#111292=DIRECTION('ref_axis',(0.,1.,0.));
#111293=DIRECTION('center_axis',(-1.,0.,0.));
#111294=DIRECTION('ref_axis',(0.,1.,0.));
#111295=DIRECTION('center_axis',(0.,1.,0.));
#111296=DIRECTION('ref_axis',(0.,0.,1.));
#111297=DIRECTION('center_axis',(0.,-1.,0.));
#111298=DIRECTION('ref_axis',(1.,0.,0.));
#111299=DIRECTION('',(-5.01606788234257E-16,-1.,0.));
#111300=DIRECTION('center_axis',(-6.19323182390956E-32,0.,1.));
#111301=DIRECTION('ref_axis',(0.656059028990495,0.754709580222783,4.06312565670714E-32));
#111302=DIRECTION('',(6.19323182390956E-32,1.23467863058847E-16,-1.));
#111303=DIRECTION('center_axis',(0.,0.,-1.));
#111304=DIRECTION('ref_axis',(-1.,0.,0.));
#111305=DIRECTION('',(-5.85782591378957E-32,-1.23467863058847E-16,1.));
#111306=DIRECTION('center_axis',(0.,-1.,0.));
#111307=DIRECTION('ref_axis',(0.,0.,-1.));
#111308=DIRECTION('center_axis',(0.,-1.,-1.23467863058847E-16));
#111309=DIRECTION('ref_axis',(1.,0.,0.));
#111310=DIRECTION('',(-5.01606788234257E-16,-1.,-1.23467863058847E-16));
#111311=DIRECTION('center_axis',(0.,-1.,0.));
#111312=DIRECTION('ref_axis',(0.,0.,-1.));
#111313=DIRECTION('center_axis',(6.20126212581678E-14,-0.483005416470283,
-0.875617363727084));
#111314=DIRECTION('ref_axis',(9.99028424960391E-30,0.875617363727084,-0.483005416470283));
#111315=DIRECTION('center_axis',(6.92361050625672E-15,-0.498898715136586,
-0.866660297945547));
#111316=DIRECTION('ref_axis',(2.25138771964303E-30,0.866660297945547,-0.498898715136586));
#111317=DIRECTION('center_axis',(0.,0.,-1.));
#111318=DIRECTION('ref_axis',(-1.,0.,0.));
#111319=DIRECTION('center_axis',(0.,0.,-1.));
#111320=DIRECTION('ref_axis',(-1.,0.,0.));
#111321=DIRECTION('',(0.,0.,-1.));
#111322=DIRECTION('center_axis',(-1.60982338570647E-12,0.,-1.));
#111323=DIRECTION('ref_axis',(-1.,0.,1.60982338570648E-12));
#111324=DIRECTION('center_axis',(0.,0.498898715136559,-0.866660297945562));
#111325=DIRECTION('ref_axis',(0.,0.866660297945562,0.498898715136559));
#111326=DIRECTION('center_axis',(1.88564486786379E-14,0.483290003559882,
-0.875460320322451));
#111327=DIRECTION('ref_axis',(3.50034193199929E-30,0.875460320322451,0.483290003559882));
#111328=DIRECTION('center_axis',(0.,1.,1.23467863058847E-16));
#111329=DIRECTION('ref_axis',(-1.,0.,0.));
#111330=DIRECTION('center_axis',(0.,1.,0.));
#111331=DIRECTION('ref_axis',(0.,0.,1.));
#111332=DIRECTION('',(5.01606788234257E-16,1.,1.23467863058847E-16));
#111333=DIRECTION('center_axis',(0.,1.,0.));
#111334=DIRECTION('ref_axis',(0.,0.,1.));
#111335=DIRECTION('',(-5.01606788234257E-16,-1.,-1.23467863058847E-16));
#111336=DIRECTION('center_axis',(0.,-1.18842113532926E-16,1.));
#111337=DIRECTION('ref_axis',(0.,1.,1.18842113532926E-16));
#111338=DIRECTION('center_axis',(0.,1.19392659184112E-16,-1.));
#111339=DIRECTION('ref_axis',(0.,1.,1.19392659184112E-16));
#111340=DIRECTION('center_axis',(-1.,5.01606788234257E-16,0.));
#111341=DIRECTION('ref_axis',(0.,-1.,0.));
#111342=DIRECTION('center_axis',(0.,-1.,0.));
#111343=DIRECTION('ref_axis',(0.,0.,-1.));
#111344=DIRECTION('center_axis',(1.,0.,0.));
#111345=DIRECTION('ref_axis',(0.,-1.,0.));
#111346=DIRECTION('center_axis',(0.,0.,1.));
#111347=DIRECTION('ref_axis',(1.,0.,0.));
#111348=DIRECTION('center_axis',(2.85977186515575E-47,0.,1.));
#111349=DIRECTION('ref_axis',(0.,-1.,0.));
#111350=DIRECTION('',(-2.85977186515575E-47,-5.70122241611331E-32,-1.));
#111351=DIRECTION('center_axis',(0.,0.,1.));
#111352=DIRECTION('ref_axis',(1.,0.,0.));
#111353=DIRECTION('center_axis',(0.,0.477110018651003,-0.878843575446074));
#111354=DIRECTION('ref_axis',(0.,0.878843575446074,0.477110018651003));
#111355=DIRECTION('center_axis',(0.,0.460605100635463,-0.887605171947863));
#111356=DIRECTION('ref_axis',(0.,0.887605171947863,0.460605100635463));
#111357=DIRECTION('center_axis',(0.,0.,-1.));
#111358=DIRECTION('ref_axis',(-1.,0.,0.));
#111359=DIRECTION('center_axis',(0.,0.,1.));
#111360=DIRECTION('ref_axis',(1.,0.,0.));
#111361=DIRECTION('center_axis',(0.,0.,-1.));
#111362=DIRECTION('ref_axis',(-1.,0.,0.));
#111363=DIRECTION('',(0.,0.,1.));
#111364=DIRECTION('center_axis',(0.,-0.477110018651024,-0.878843575446063));
#111365=DIRECTION('ref_axis',(0.,0.878843575446063,-0.477110018651024));
#111366=DIRECTION('center_axis',(0.,-0.46043947842117,-0.887691098700016));
#111367=DIRECTION('ref_axis',(0.,0.887691098700016,-0.46043947842117));
#111368=DIRECTION('center_axis',(0.,-0.635616055211064,-0.772005330524295));
#111369=DIRECTION('ref_axis',(0.,0.772005330524295,-0.635616055211064));
#111370=DIRECTION('center_axis',(0.,4.38538094726937E-12,-1.));
#111371=DIRECTION('ref_axis',(0.,1.,4.38538094726937E-12));
#111372=DIRECTION('center_axis',(0.,0.800147951883018,-0.599802680135236));
#111373=DIRECTION('ref_axis',(0.,0.599802680135236,0.800147951883018));
#111374=DIRECTION('center_axis',(1.,0.,0.));
#111375=DIRECTION('ref_axis',(0.,0.919361469586663,0.393413889230479));
#111376=DIRECTION('center_axis',(0.,-1.,-1.23467863058847E-16));
#111377=DIRECTION('ref_axis',(1.,0.,0.));
#111378=DIRECTION('center_axis',(0.,-1.,0.));
#111379=DIRECTION('ref_axis',(0.,0.,-1.));
#111380=DIRECTION('',(-4.38004274807345E-16,-1.,-1.23467863058847E-16));
#111381=DIRECTION('center_axis',(0.,-1.,0.));
#111382=DIRECTION('ref_axis',(0.,0.,-1.));
#111383=DIRECTION('',(4.38004274807345E-16,1.,1.23467863058847E-16));
#111384=DIRECTION('center_axis',(0.,0.,-1.));
#111385=DIRECTION('ref_axis',(-1.,0.,0.));
#111386=DIRECTION('center_axis',(0.,1.07494104808783E-16,-1.));
#111387=DIRECTION('ref_axis',(-1.,0.,0.));
#111388=DIRECTION('',(-1.13659195805196E-16,1.07494104808783E-16,-1.));
#111389=DIRECTION('',(1.13659195805196E-16,-1.07494104808783E-16,1.));
#111390=DIRECTION('center_axis',(0.,1.,0.));
#111391=DIRECTION('ref_axis',(-1.,0.,0.));
#111392=DIRECTION('',(4.38004274807345E-16,1.,0.));
#111393=DIRECTION('center_axis',(0.,1.,0.));
#111394=DIRECTION('ref_axis',(0.,0.,1.));
#111395=DIRECTION('center_axis',(-1.,4.38004274807345E-16,1.13659195805196E-16));
#111396=DIRECTION('ref_axis',(0.,-1.,0.));
#111397=DIRECTION('center_axis',(0.,0.,-1.));
#111398=DIRECTION('ref_axis',(-1.,0.,0.));
#111399=DIRECTION('center_axis',(1.,0.,-1.13659195805196E-16));
#111400=DIRECTION('ref_axis',(0.,-1.,0.));
#111401=DIRECTION('center_axis',(-1.13659195805195E-16,0.,-1.));
#111402=DIRECTION('ref_axis',(-1.,0.,1.13659195805195E-16));
#111403=DIRECTION('center_axis',(0.,0.,-1.));
#111404=DIRECTION('ref_axis',(-1.,0.,0.));
#111405=DIRECTION('',(-1.13659195805196E-16,0.,-1.));
#111406=DIRECTION('center_axis',(0.,-1.,0.));
#111407=DIRECTION('ref_axis',(0.,0.,-1.));
#111408=DIRECTION('center_axis',(-4.38004274807345E-16,-1.,0.));
#111409=DIRECTION('ref_axis',(0.,0.,-1.));
#111410=DIRECTION('center_axis',(0.,1.,1.23467863058847E-16));
#111411=DIRECTION('ref_axis',(-1.,0.,0.));
#111412=DIRECTION('',(-4.38004274807345E-16,-1.,-1.23467863058847E-16));
#111413=DIRECTION('center_axis',(0.,4.9783213633841E-32,-1.));
#111414=DIRECTION('ref_axis',(-1.,0.,0.));
#111415=DIRECTION('',(1.13659195805196E-16,-4.9783213633841E-32,1.));
#111416=DIRECTION('',(-1.13659195805196E-16,4.9783213633841E-32,-1.));
#111417=DIRECTION('center_axis',(0.,-1.,-1.23467863058847E-16));
#111418=DIRECTION('ref_axis',(1.,0.,0.));
#111419=DIRECTION('center_axis',(-4.38004274807345E-16,-1.,0.));
#111420=DIRECTION('ref_axis',(0.,0.,-1.));
#111421=DIRECTION('',(-4.38004274807345E-16,-1.,-1.23467863058847E-16));
#111422=DIRECTION('',(4.38004274807345E-16,1.,1.23467863058847E-16));
#111423=DIRECTION('center_axis',(-1.,4.38004274807345E-16,1.13659195805196E-16));
#111424=DIRECTION('ref_axis',(0.,-1.,0.));
#111425=DIRECTION('center_axis',(0.,-1.,0.));
#111426=DIRECTION('ref_axis',(0.,0.,-1.));
#111427=DIRECTION('center_axis',(-1.,0.,1.13659195805196E-16));
#111428=DIRECTION('ref_axis',(0.,-1.,0.));
#111429=DIRECTION('center_axis',(1.,0.,-1.13659195805196E-16));
#111430=DIRECTION('ref_axis',(0.,-1.,0.));
#111431=DIRECTION('center_axis',(1.,-5.01606788234257E-16,0.));
#111432=DIRECTION('ref_axis',(5.01606788234257E-16,1.,0.));
#111433=DIRECTION('',(1.,-5.01606788234257E-16,0.));
#111434=DIRECTION('center_axis',(1.,0.,1.13659195805196E-16));
#111435=DIRECTION('ref_axis',(0.,1.,0.));
#111436=DIRECTION('center_axis',(0.,1.,1.23467863058847E-16));
#111437=DIRECTION('ref_axis',(-1.,0.,0.));
#111438=DIRECTION('center_axis',(0.,1.,0.));
#111439=DIRECTION('ref_axis',(0.,0.,1.));
#111440=DIRECTION('center_axis',(0.,1.,0.));
#111441=DIRECTION('ref_axis',(0.,0.,1.));
#111442=DIRECTION('',(-5.01606788234257E-16,-1.,-1.23467863058847E-16));
#111443=DIRECTION('center_axis',(0.,0.973635916817664,0.228107653274998));
#111444=DIRECTION('ref_axis',(0.,-0.228107653274998,0.973635916817664));
#111445=DIRECTION('center_axis',(0.,0.489712654585584,0.871883889023499));
#111446=DIRECTION('ref_axis',(0.,-0.871883889023499,0.489712654585584));
#111447=DIRECTION('center_axis',(0.,-1.11022302462516E-13,1.));
#111448=DIRECTION('ref_axis',(0.,-1.,-1.11022302462516E-13));
#111449=DIRECTION('center_axis',(0.,-4.9783213633841E-32,-1.));
#111450=DIRECTION('ref_axis',(-1.,0.,0.));
#111451=DIRECTION('',(1.13659195805196E-16,-4.9783213633841E-32,-1.));
#111452=DIRECTION('center_axis',(0.,0.,-1.));
#111453=DIRECTION('ref_axis',(-1.,0.,0.));
#111454=DIRECTION('center_axis',(-6.24334907322839E-14,0.457979853752065,
-0.888962571516505));
#111455=DIRECTION('ref_axis',(1.27562203883084E-29,0.888962571516505,0.457979853752065));
#111456=DIRECTION('center_axis',(0.,1.,0.));
#111457=DIRECTION('ref_axis',(0.,0.,1.));
#111458=DIRECTION('center_axis',(1.,-5.01606788234257E-16,1.13659195805196E-16));
#111459=DIRECTION('ref_axis',(0.,1.,0.));
#111460=DIRECTION('center_axis',(0.,-1.,0.));
#111461=DIRECTION('ref_axis',(0.,0.,-1.));
#111462=DIRECTION('center_axis',(-1.,0.,-1.13659195805196E-16));
#111463=DIRECTION('ref_axis',(0.,1.,0.));
#111464=DIRECTION('center_axis',(0.,0.,-1.));
#111465=DIRECTION('ref_axis',(-1.,0.,0.));
#111466=DIRECTION('center_axis',(0.,-1.14024448322266E-31,-1.));
#111467=DIRECTION('ref_axis',(-1.,0.,0.));
#111468=DIRECTION('',(-1.13659195805196E-16,1.14024448322266E-31,1.));
#111469=DIRECTION('center_axis',(0.,0.,-1.));
#111470=DIRECTION('ref_axis',(-1.,0.,0.));
#111471=DIRECTION('center_axis',(1.,-5.01606788234257E-16,1.13659195805196E-16));
#111472=DIRECTION('ref_axis',(0.,1.,0.));
#111473=DIRECTION('center_axis',(-1.,0.,-1.13659195805196E-16));
#111474=DIRECTION('ref_axis',(0.,1.,0.));
#111475=DIRECTION('center_axis',(0.,1.,0.));
#111476=DIRECTION('ref_axis',(0.,0.,1.));
#111477=DIRECTION('center_axis',(0.,-1.,0.));
#111478=DIRECTION('ref_axis',(1.,0.,0.));
#111479=DIRECTION('',(-5.01606788234257E-16,-1.,0.));
#111480=DIRECTION('center_axis',(1.13659195805196E-16,0.,-1.));
#111481=DIRECTION('ref_axis',(0.,1.,0.));
#111482=DIRECTION('center_axis',(0.,0.,1.));
#111483=DIRECTION('ref_axis',(1.,0.,0.));
#111484=DIRECTION('',(-1.13659195805196E-16,-1.39441621308911E-16,1.));
#111485=DIRECTION('',(1.13659195805196E-16,1.39441621308911E-16,-1.));
#111486=DIRECTION('center_axis',(0.,0.,1.));
#111487=DIRECTION('ref_axis',(1.,0.,0.));
#111488=DIRECTION('center_axis',(0.,1.23467863058847E-16,-1.));
#111489=DIRECTION('ref_axis',(0.,1.,1.1837531408762E-16));
#111490=DIRECTION('center_axis',(0.,-1.17559414210783E-16,1.));
#111491=DIRECTION('ref_axis',(0.,1.,1.17559414210783E-16));
#111492=DIRECTION('center_axis',(-0.744016723942684,-0.668160994441905,
0.));
#111493=DIRECTION('ref_axis',(0.668160994441905,-0.744016723942684,0.));
#111494=DIRECTION('center_axis',(0.,-1.,-1.23467863058847E-16));
#111495=DIRECTION('ref_axis',(1.,0.,0.));
#111496=DIRECTION('',(5.01606788234257E-16,1.,1.23467863058847E-16));
#111497=DIRECTION('center_axis',(0.,1.,0.));
#111498=DIRECTION('ref_axis',(0.,0.,1.));
#111499=DIRECTION('',(-5.01606788234257E-16,-1.,-1.23467863058847E-16));
#111500=DIRECTION('center_axis',(0.,-1.,-1.23467863058847E-16));
#111501=DIRECTION('ref_axis',(1.,0.,0.));
#111502=DIRECTION('',(5.01606788234257E-16,1.,1.23467863058847E-16));
#111503=DIRECTION('center_axis',(0.,1.,0.));
#111504=DIRECTION('ref_axis',(0.,0.,1.));
#111505=DIRECTION('',(-5.01606788234257E-16,-1.,-1.23467863058847E-16));
#111506=DIRECTION('center_axis',(-0.473027330271494,0.,0.881047753993064));
#111507=DIRECTION('ref_axis',(0.881047753993064,0.,0.473027330271494));
#111508=DIRECTION('center_axis',(-0.452154194923616,0.,0.891939787212666));
#111509=DIRECTION('ref_axis',(0.891939787212666,0.,0.452154194923616));
#111510=DIRECTION('center_axis',(0.,0.,1.));
#111511=DIRECTION('ref_axis',(1.,0.,0.));
#111512=DIRECTION('center_axis',(0.,0.,-1.));
#111513=DIRECTION('ref_axis',(-1.,0.,0.));
#111514=DIRECTION('center_axis',(0.,0.,1.));
#111515=DIRECTION('ref_axis',(1.,0.,0.));
#111516=DIRECTION('',(0.,0.,-1.));
#111517=DIRECTION('center_axis',(0.473027330271434,0.,0.881047753993096));
#111518=DIRECTION('ref_axis',(0.881047753993096,0.,-0.473027330271434));
#111519=DIRECTION('center_axis',(0.,0.,-1.));
#111520=DIRECTION('ref_axis',(-1.,0.,0.));
#111521=DIRECTION('center_axis',(0.,0.,-1.));
#111522=DIRECTION('ref_axis',(-1.,0.,0.));
#111523=DIRECTION('',(0.,0.,1.));
#111524=DIRECTION('center_axis',(0.,0.,-1.));
#111525=DIRECTION('ref_axis',(-1.,0.,0.));
#111526=DIRECTION('center_axis',(4.18005656861882E-16,1.,0.));
#111527=DIRECTION('ref_axis',(-1.,5.9211894646675E-16,0.));
#111528=DIRECTION('center_axis',(-6.93889390390722E-16,-1.,0.));
#111529=DIRECTION('ref_axis',(-1.,6.93889390390722E-16,0.));
#111530=DIRECTION('center_axis',(-1.,0.,0.));
#111531=DIRECTION('ref_axis',(0.,0.,1.));
#111532=DIRECTION('center_axis',(1.,0.,0.));
#111533=DIRECTION('ref_axis',(0.,1.,0.));
#111534=DIRECTION('',(1.,-4.18005656861881E-16,0.));
#111535=DIRECTION('center_axis',(0.,0.,1.));
#111536=DIRECTION('ref_axis',(0.,-1.,0.));
#111537=DIRECTION('center_axis',(0.,0.,1.));
#111538=DIRECTION('ref_axis',(1.,0.,0.));
#111539=DIRECTION('',(0.,-1.23467863058847E-16,1.));
#111540=DIRECTION('',(-5.16102651992463E-32,2.15733828054269E-47,-1.));
#111541=DIRECTION('center_axis',(2.20736287103737E-8,1.,5.31880064827284E-9));
#111542=DIRECTION('ref_axis',(0.999350588281835,-2.18676396770165E-8,-0.0360333415151705));
#111543=DIRECTION('center_axis',(0.452279624303263,0.,0.891876191766604));
#111544=DIRECTION('ref_axis',(0.891876191766604,0.,-0.452279624303263));
#111545=DIRECTION('center_axis',(0.,0.,-1.));
#111546=DIRECTION('ref_axis',(-1.,0.,0.));
#111547=DIRECTION('center_axis',(-0.453032377894844,0.,-0.891494063120413));
#111548=DIRECTION('ref_axis',(-0.891494063120413,0.,0.453032377894844));
#111549=DIRECTION('center_axis',(0.,0.,1.));
#111550=DIRECTION('ref_axis',(1.,0.,0.));
#111551=DIRECTION('center_axis',(0.,0.,-1.));
#111552=DIRECTION('ref_axis',(-1.,0.,0.));
#111553=DIRECTION('',(0.,0.,1.));
#111554=DIRECTION('center_axis',(-0.45303237789485,6.28708721049444E-15,
0.89149406312041));
#111555=DIRECTION('ref_axis',(0.89149406312041,3.90721898735751E-30,0.45303237789485));
#111556=DIRECTION('center_axis',(-0.438728460697982,6.08858048281589E-15,
0.898619684724066));
#111557=DIRECTION('ref_axis',(0.898619684724066,-1.57717257184587E-30,0.438728460697982));
#111558=DIRECTION('center_axis',(1.87037530511154E-7,-0.999999999999982,
4.34091799744689E-8));
#111559=DIRECTION('ref_axis',(0.943089040187619,1.61957742669363E-7,-0.332540316770719));
#111560=DIRECTION('center_axis',(0.,0.,1.));
#111561=DIRECTION('ref_axis',(1.,0.,0.));
#111562=DIRECTION('center_axis',(0.,0.,1.));
#111563=DIRECTION('ref_axis',(0.,-1.,0.));
#111564=DIRECTION('',(5.16102651992463E-32,-2.15733828054269E-47,1.));
#111565=DIRECTION('',(0.,1.23467863058847E-16,-1.));
#111566=DIRECTION('center_axis',(1.,0.,0.));
#111567=DIRECTION('ref_axis',(0.,1.,0.));
#111568=DIRECTION('',(-1.,4.18005656861881E-16,0.));
#111569=DIRECTION('center_axis',(1.,0.,0.));
#111570=DIRECTION('ref_axis',(0.,0.,-1.));
#111571=DIRECTION('center_axis',(-4.18005656861882E-16,-1.,0.));
#111572=DIRECTION('ref_axis',(1.,-2.96059473233375E-16,0.));
#111573=DIRECTION('center_axis',(3.46944695195361E-16,1.,0.));
#111574=DIRECTION('ref_axis',(1.,-3.46944695195361E-16,0.));
#111575=DIRECTION('center_axis',(0.,0.,1.));
#111576=DIRECTION('ref_axis',(1.,0.,0.));
#111577=DIRECTION('center_axis',(0.,0.,1.));
#111578=DIRECTION('ref_axis',(1.,0.,0.));
#111579=DIRECTION('',(0.,0.,-1.));
#111580=DIRECTION('center_axis',(0.,0.,1.));
#111581=DIRECTION('ref_axis',(1.,0.,0.));
#111582=DIRECTION('center_axis',(-0.438793812561498,0.,-0.898587775377423));
#111583=DIRECTION('ref_axis',(-0.898587775377423,0.,0.438793812561498));
#111584=DIRECTION('center_axis',(-4.18005656861882E-16,-1.,0.));
#111585=DIRECTION('ref_axis',(1.,-2.96059473233375E-16,0.));
#111586=DIRECTION('center_axis',(3.46944695195361E-16,1.,0.));
#111587=DIRECTION('ref_axis',(1.,-3.46944695195361E-16,0.));
#111588=DIRECTION('center_axis',(-1.,0.,0.));
#111589=DIRECTION('ref_axis',(0.,0.,1.));
#111590=DIRECTION('center_axis',(-4.33680868994202E-16,-1.,0.));
#111591=DIRECTION('ref_axis',(1.,-4.33680868994202E-16,0.));
#111592=DIRECTION('center_axis',(4.18005656861881E-16,1.,0.));
#111593=DIRECTION('ref_axis',(-1.,4.18005656861881E-16,0.));
#111594=DIRECTION('',(4.18005656861881E-16,1.,0.));
#111595=DIRECTION('center_axis',(4.33680868994202E-16,1.,0.));
#111596=DIRECTION('ref_axis',(-1.,4.33680868994202E-16,0.));
#111597=DIRECTION('center_axis',(4.18005656861882E-16,1.,0.));
#111598=DIRECTION('ref_axis',(-1.,2.96059473233375E-16,0.));
#111599=DIRECTION('center_axis',(1.,0.,0.));
#111600=DIRECTION('ref_axis',(0.,0.,-1.));
#111601=DIRECTION('center_axis',(-3.46944695195361E-16,-1.,0.));
#111602=DIRECTION('ref_axis',(-1.,3.46944695195361E-16,0.));
#111603=DIRECTION('center_axis',(0.,0.,-1.));
#111604=DIRECTION('ref_axis',(-1.,0.,0.));
#111605=DIRECTION('center_axis',(0.,0.,-1.));
#111606=DIRECTION('ref_axis',(-1.,0.,0.));
#111607=DIRECTION('',(0.,0.,1.));
#111608=DIRECTION('center_axis',(0.,0.,-1.));
#111609=DIRECTION('ref_axis',(-1.,0.,0.));
#111610=DIRECTION('center_axis',(4.18005656861882E-16,1.,0.));
#111611=DIRECTION('ref_axis',(-1.,2.96059473233375E-16,0.));
#111612=DIRECTION('center_axis',(-3.46944695195361E-16,-1.,0.));
#111613=DIRECTION('ref_axis',(-1.,3.46944695195361E-16,0.));
#111614=DIRECTION('center_axis',(0.,0.,1.));
#111615=DIRECTION('ref_axis',(0.,-1.,0.));
#111616=DIRECTION('',(-5.16102651992463E-32,2.15733828054269E-47,-1.));
#111617=DIRECTION('center_axis',(0.,0.,-1.));
#111618=DIRECTION('ref_axis',(-1.,0.,0.));
#111619=DIRECTION('',(0.,-1.23467863058847E-16,1.));
#111620=DIRECTION('center_axis',(2.74310936473999E-7,0.99999999999996,6.28664506624393E-8));
#111621=DIRECTION('ref_axis',(-0.661953171810168,1.34459748483106E-7,0.74954519432149));
#111622=DIRECTION('center_axis',(0.434261044064412,-6.0265826227258E-15,
-0.90078707007155));
#111623=DIRECTION('ref_axis',(-0.90078707007155,1.10802520916158E-30,-0.434261044064412));
#111624=DIRECTION('center_axis',(0.445417151990703,0.,-0.895323159933044));
#111625=DIRECTION('ref_axis',(-0.895323159933044,0.,-0.445417151990703));
#111626=DIRECTION('center_axis',(0.,0.,-1.));
#111627=DIRECTION('ref_axis',(-1.,0.,0.));
#111628=DIRECTION('center_axis',(0.,0.,-1.));
#111629=DIRECTION('ref_axis',(-1.,0.,0.));
#111630=DIRECTION('',(0.,0.,-1.));
#111631=DIRECTION('center_axis',(0.,0.,-1.));
#111632=DIRECTION('ref_axis',(-1.,0.,0.));
#111633=DIRECTION('center_axis',(0.44541715199073,0.,0.895323159933031));
#111634=DIRECTION('ref_axis',(0.895323159933031,0.,-0.44541715199073));
#111635=DIRECTION('center_axis',(0.434307547312743,0.,0.900764649809921));
#111636=DIRECTION('ref_axis',(0.900764649809921,0.,-0.434307547312743));
#111637=DIRECTION('center_axis',(0.,0.,-1.));
#111638=DIRECTION('ref_axis',(-1.,0.,0.));
#111639=DIRECTION('center_axis',(-0.431774610811204,0.,-0.901981532770396));
#111640=DIRECTION('ref_axis',(-0.901981532770396,0.,0.431774610811205));
#111641=DIRECTION('center_axis',(0.,0.,1.));
#111642=DIRECTION('ref_axis',(1.,0.,0.));
#111643=DIRECTION('center_axis',(0.,0.,-1.));
#111644=DIRECTION('ref_axis',(-1.,0.,0.));
#111645=DIRECTION('',(0.,0.,1.));
#111646=DIRECTION('center_axis',(0.43177461081284,0.,-0.901981532769613));
#111647=DIRECTION('ref_axis',(-0.901981532769613,0.,-0.43177461081284));
#111648=DIRECTION('center_axis',(0.427007199080172,0.,-0.904248224733511));
#111649=DIRECTION('ref_axis',(-0.904248224733511,0.,-0.427007199080172));
#111650=DIRECTION('center_axis',(0.,0.,-1.));
#111651=DIRECTION('ref_axis',(-1.,0.,0.));
#111652=DIRECTION('center_axis',(0.,-1.,0.));
#111653=DIRECTION('ref_axis',(0.979094017787432,0.,0.203408220907771));
#111654=DIRECTION('center_axis',(0.,0.,1.));
#111655=DIRECTION('ref_axis',(0.,-1.,0.));
#111656=DIRECTION('',(0.,1.23467863058847E-16,-1.));
#111657=DIRECTION('',(5.16102651992463E-32,-2.15733828054269E-47,1.));
#111658=DIRECTION('center_axis',(0.,0.,-1.));
#111659=DIRECTION('ref_axis',(-1.,0.,0.));
#111660=DIRECTION('center_axis',(-0.427024288778512,0.,-0.904240154380022));
#111661=DIRECTION('ref_axis',(-0.904240154380022,0.,0.427024288778512));
#111662=DIRECTION('center_axis',(0.,0.,1.));
#111663=DIRECTION('ref_axis',(1.,0.,0.));
#111664=DIRECTION('center_axis',(0.,0.,-1.));
#111665=DIRECTION('ref_axis',(-1.,0.,0.));
#111666=DIRECTION('',(0.,0.,1.));
#111667=DIRECTION('',(0.,0.,-1.));
#111668=DIRECTION('center_axis',(1.,-4.18005656861882E-16,0.));
#111669=DIRECTION('ref_axis',(-4.18005656861882E-16,-1.,0.));
#111670=DIRECTION('',(0.,0.,-1.));
#111671=DIRECTION('center_axis',(0.,0.,-1.));
#111672=DIRECTION('ref_axis',(-1.,0.,0.));
#111673=DIRECTION('center_axis',(0.,0.,-1.));
#111674=DIRECTION('ref_axis',(-1.,0.,0.));
#111675=DIRECTION('',(0.,0.,1.));
#111676=DIRECTION('center_axis',(0.,0.,-1.));
#111677=DIRECTION('ref_axis',(-1.,0.,0.));
#111678=DIRECTION('center_axis',(0.,0.,1.));
#111679=DIRECTION('ref_axis',(0.,-1.,0.));
#111680=DIRECTION('',(-5.16102651992463E-32,2.15733828054269E-47,-1.));
#111681=DIRECTION('center_axis',(0.,0.,-1.));
#111682=DIRECTION('ref_axis',(-1.,0.,0.));
#111683=DIRECTION('',(0.,-1.23467863058847E-16,1.));
#111684=DIRECTION('center_axis',(0.,1.,0.));
#111685=DIRECTION('ref_axis',(0.977956433447826,0.,0.208809037826448));
#111686=DIRECTION('center_axis',(0.424945455576639,-5.89730286238743E-15,
-0.905218956819157));
#111687=DIRECTION('ref_axis',(-0.905218956819157,3.24660130849529E-29,-0.424945455576639));
#111688=DIRECTION('center_axis',(0.427566573571518,-4.42475067662884E-14,
-0.903983863331814));
#111689=DIRECTION('ref_axis',(-0.903983863331814,-2.72495173441675E-28,
-0.427566573571518));
#111690=DIRECTION('center_axis',(0.,0.,-1.));
#111691=DIRECTION('ref_axis',(-1.,0.,0.));
#111692=DIRECTION('center_axis',(0.,0.,-1.));
#111693=DIRECTION('ref_axis',(-1.,0.,0.));
#111694=DIRECTION('',(0.,0.,-1.));
#111695=DIRECTION('center_axis',(0.,0.,-1.));
#111696=DIRECTION('ref_axis',(-1.,0.,0.));
#111697=DIRECTION('center_axis',(-0.427566573571512,0.,-0.903983863331817));
#111698=DIRECTION('ref_axis',(-0.903983863331817,0.,0.427566573571512));
#111699=DIRECTION('center_axis',(-0.424954451342053,-5.8974277037113E-15,
-0.905214733797774));
#111700=DIRECTION('ref_axis',(-0.905214733797774,1.745344269554E-30,0.424954451342053));
#111701=DIRECTION('center_axis',(-0.00252749518976105,-0.999981529958737,
-0.00552734198781944));
#111702=DIRECTION('ref_axis',(0.976364750278453,-0.00127318089754541,-0.216125550141799));
#111703=DIRECTION('center_axis',(0.,0.,-1.));
#111704=DIRECTION('ref_axis',(-1.,0.,0.));
#111705=DIRECTION('center_axis',(-0.422759120858735,0.,-0.906242090023824));
#111706=DIRECTION('ref_axis',(-0.906242090023824,0.,0.422759120858735));
#111707=DIRECTION('center_axis',(0.,1.,0.));
#111708=DIRECTION('ref_axis',(0.976404651458723,0.,-0.21594896760524));
#111709=DIRECTION('center_axis',(0.,0.,1.));
#111710=DIRECTION('ref_axis',(1.,0.,0.));
#111711=DIRECTION('center_axis',(0.,0.,-1.));
#111712=DIRECTION('ref_axis',(-1.,0.,0.));
#111713=DIRECTION('',(0.,0.,1.));
#111714=DIRECTION('center_axis',(0.422759120858763,0.,-0.906242090023811));
#111715=DIRECTION('ref_axis',(-0.906242090023811,0.,-0.422759120858763));
#111716=DIRECTION('center_axis',(0.,1.,0.));
#111717=DIRECTION('ref_axis',(0.976137352210977,0.,0.217154022800736));
#111718=DIRECTION('center_axis',(0.422683101271474,0.,-0.906277549043078));
#111719=DIRECTION('ref_axis',(-0.906277549043078,0.,-0.422683101271474));
#111720=DIRECTION('center_axis',(0.,0.,-1.));
#111721=DIRECTION('ref_axis',(-1.,0.,0.));
#111722=DIRECTION('center_axis',(0.,-1.,0.));
#111723=DIRECTION('ref_axis',(0.976204192855077,0.,0.216853346416809));
#111724=DIRECTION('center_axis',(0.,0.,1.));
#111725=DIRECTION('ref_axis',(0.,-1.,0.));
#111726=DIRECTION('',(0.,1.23467863058847E-16,-1.));
#111727=DIRECTION('',(5.16102651992463E-32,-2.15733828054269E-47,1.));
#111728=DIRECTION('center_axis',(4.44089209850062E-13,0.,-1.));
#111729=DIRECTION('ref_axis',(-1.,0.,-4.44089209850062E-13));
#111730=DIRECTION('center_axis',(-0.422683349901129,0.,-0.906277433083468));
#111731=DIRECTION('ref_axis',(-0.906277433083468,0.,0.422683349901129));
#111732=DIRECTION('center_axis',(0.,0.,1.));
#111733=DIRECTION('ref_axis',(1.,0.,0.));
#111734=DIRECTION('center_axis',(0.,0.,-1.));
#111735=DIRECTION('ref_axis',(-1.,0.,0.));
#111736=DIRECTION('',(0.,0.,1.));
#111737=DIRECTION('',(0.,0.,-1.));
#111738=DIRECTION('center_axis',(1.,-4.18005656861882E-16,0.));
#111739=DIRECTION('ref_axis',(-4.18005656861882E-16,-1.,0.));
#111740=DIRECTION('center_axis',(1.,0.,0.));
#111741=DIRECTION('ref_axis',(0.,-0.00331492178303338,0.999994505631692));
#111742=DIRECTION('',(0.,0.,-1.));
#111743=DIRECTION('center_axis',(0.,0.,-1.));
#111744=DIRECTION('ref_axis',(-1.,0.,0.));
#111745=DIRECTION('center_axis',(0.,0.,-1.));
#111746=DIRECTION('ref_axis',(-1.,0.,0.));
#111747=DIRECTION('',(0.,0.,1.));
#111748=DIRECTION('center_axis',(0.,-5.55111512312578E-14,-1.));
#111749=DIRECTION('ref_axis',(0.,1.,-5.55111512312578E-14));
#111750=DIRECTION('center_axis',(0.,0.,1.));
#111751=DIRECTION('ref_axis',(0.,-1.,0.));
#111752=DIRECTION('',(-5.16102651992463E-32,2.15733828054269E-47,-1.));
#111753=DIRECTION('center_axis',(0.,0.,-1.));
#111754=DIRECTION('ref_axis',(-1.,0.,0.));
#111755=DIRECTION('',(0.,-1.23467863058847E-16,1.));
#111756=DIRECTION('center_axis',(0.,1.,0.));
#111757=DIRECTION('ref_axis',(0.976488023107232,0.,0.21557166030842));
#111758=DIRECTION('center_axis',(0.422711298276089,5.8662977014411E-15,
-0.906264397573767));
#111759=DIRECTION('ref_axis',(-0.906264397573767,-1.10286040862995E-31,
-0.422711298276089));
#111760=DIRECTION('center_axis',(0.422820321921648,5.86781070846046E-15,
-0.906213537401685));
#111761=DIRECTION('ref_axis',(-0.906213537401684,-2.1653413854129E-31,-0.422820321921648));
#111762=DIRECTION('center_axis',(-1.03393670705645E-14,-1.,-1.1317479530313E-15));
#111763=DIRECTION('ref_axis',(0.976392755984668,-1.03397437742268E-14,0.216002745493349));
#111764=DIRECTION('center_axis',(0.,0.,-1.));
#111765=DIRECTION('ref_axis',(-1.,0.,0.));
#111766=DIRECTION('center_axis',(0.,0.,-1.));
#111767=DIRECTION('ref_axis',(-1.,0.,0.));
#111768=DIRECTION('',(0.,0.,-1.));
#111769=DIRECTION('center_axis',(0.,0.,-1.));
#111770=DIRECTION('ref_axis',(-1.,0.,0.));
#111771=DIRECTION('center_axis',(0.,-1.,0.));
#111772=DIRECTION('ref_axis',(0.976124389191106,0.,-0.217212285164286));
#111773=DIRECTION('center_axis',(-0.422820321921619,0.,-0.906213537401698));
#111774=DIRECTION('ref_axis',(-0.906213537401698,0.,0.422820321921619));
#111775=DIRECTION('center_axis',(-0.00301385145090742,0.999973599361283,
-0.0066119044059187));
#111776=DIRECTION('ref_axis',(0.976009136147408,0.0015020133499738,-0.21772439025678));
#111777=DIRECTION('center_axis',(-0.422711655064036,5.86630265286877E-15,
-0.906264231156137));
#111778=DIRECTION('ref_axis',(-0.906264231156137,8.13850067779198E-31,0.422711655064036));
#111779=DIRECTION('center_axis',(0.,0.,-1.));
#111780=DIRECTION('ref_axis',(-1.,0.,0.));
#111781=DIRECTION('center_axis',(-0.427895220819097,0.,-0.903828346534991));
#111782=DIRECTION('ref_axis',(-0.903828346534991,0.,0.427895220819097));
#111783=DIRECTION('center_axis',(0.,0.,1.));
#111784=DIRECTION('ref_axis',(1.,0.,0.));
#111785=DIRECTION('center_axis',(0.,0.,-1.));
#111786=DIRECTION('ref_axis',(-1.,0.,0.));
#111787=DIRECTION('',(0.,0.,1.));
#111788=DIRECTION('center_axis',(0.427895220819092,0.,-0.903828346534994));
#111789=DIRECTION('ref_axis',(-0.903828346534994,0.,-0.427895220819092));
#111790=DIRECTION('center_axis',(0.425103688199478,0.,-0.905144659310986));
#111791=DIRECTION('ref_axis',(-0.905144659310986,0.,-0.425103688199478));
#111792=DIRECTION('center_axis',(0.,0.,-1.));
#111793=DIRECTION('ref_axis',(-1.,0.,0.));
#111794=DIRECTION('center_axis',(0.,-1.,0.));
#111795=DIRECTION('ref_axis',(0.977785987053698,0.,0.209605733512769));
#111796=DIRECTION('center_axis',(0.,0.,1.));
#111797=DIRECTION('ref_axis',(0.,-1.,0.));
#111798=DIRECTION('',(0.,1.23467863058847E-16,-1.));
#111799=DIRECTION('',(5.16102651992463E-32,-2.15733828054269E-47,1.));
#111800=DIRECTION('center_axis',(0.,0.,1.));
#111801=DIRECTION('ref_axis',(1.,0.,0.));
#111802=DIRECTION('center_axis',(-0.425113301005477,0.,-0.905140144567805));
#111803=DIRECTION('ref_axis',(-0.905140144567805,0.,0.425113301005477));
#111804=DIRECTION('center_axis',(0.,0.,1.));
#111805=DIRECTION('ref_axis',(1.,0.,0.));
#111806=DIRECTION('',(0.,0.,-1.));
#111807=DIRECTION('center_axis',(0.,0.,1.));
#111808=DIRECTION('ref_axis',(1.,0.,0.));
#111809=DIRECTION('',(0.,0.,1.));
#111810=DIRECTION('center_axis',(1.,-4.18005656861882E-16,0.));
#111811=DIRECTION('ref_axis',(-4.18005656861882E-16,-1.,0.));
#111812=DIRECTION('',(0.,0.,-1.));
#111813=DIRECTION('center_axis',(0.,0.,-1.));
#111814=DIRECTION('ref_axis',(-1.,0.,0.));
#111815=DIRECTION('center_axis',(0.,0.,-1.));
#111816=DIRECTION('ref_axis',(-1.,0.,0.));
#111817=DIRECTION('',(0.,0.,1.));
#111818=DIRECTION('center_axis',(0.,0.,-1.));
#111819=DIRECTION('ref_axis',(-1.,0.,0.));
#111820=DIRECTION('center_axis',(0.,0.,1.));
#111821=DIRECTION('ref_axis',(0.,-1.,0.));
#111822=DIRECTION('',(-5.16102651992463E-32,2.15733828054269E-47,-1.));
#111823=DIRECTION('center_axis',(0.,0.,-1.));
#111824=DIRECTION('ref_axis',(-1.,0.,0.));
#111825=DIRECTION('',(0.,-1.23467863058847E-16,1.));
#111826=DIRECTION('center_axis',(4.4207807240187E-7,0.999999999999897,9.93087227439201E-8));
#111827=DIRECTION('ref_axis',(-0.291484561047742,3.38626384751091E-8,0.956575533175924));
#111828=DIRECTION('center_axis',(0.42722596110711,0.,-0.904144887811741));
#111829=DIRECTION('ref_axis',(-0.904144887811741,0.,-0.42722596110711));
#111830=DIRECTION('center_axis',(0.432211889750627,1.1996289787948E-14,
-0.901772078941343));
#111831=DIRECTION('ref_axis',(-0.901772078941343,7.55282579686682E-29,-0.432211889750627));
#111832=DIRECTION('center_axis',(0.,0.,-1.));
#111833=DIRECTION('ref_axis',(-1.,0.,0.));
#111834=DIRECTION('center_axis',(0.,0.,-1.));
#111835=DIRECTION('ref_axis',(-1.,0.,0.));
#111836=DIRECTION('',(0.,0.,-1.));
#111837=DIRECTION('center_axis',(0.,0.,-1.));
#111838=DIRECTION('ref_axis',(-1.,0.,0.));
#111839=DIRECTION('center_axis',(-0.432211889750627,-1.54100116546287E-13,
-0.901772078941343));
#111840=DIRECTION('ref_axis',(-0.901772078941343,9.67025840811756E-28,0.432211889750627));
#111841=DIRECTION('center_axis',(-0.427243916491378,0.,-0.904136403327014));
#111842=DIRECTION('ref_axis',(-0.904136403327014,0.,0.427243916491378));
#111843=DIRECTION('center_axis',(0.,0.,-1.));
#111844=DIRECTION('ref_axis',(-1.,0.,0.));
#111845=DIRECTION('center_axis',(-0.446066534667472,0.,-0.894999802597606));
#111846=DIRECTION('ref_axis',(-0.894999802597606,0.,0.446066534667472));
#111847=DIRECTION('center_axis',(0.,0.,1.));
#111848=DIRECTION('ref_axis',(1.,0.,0.));
#111849=DIRECTION('center_axis',(0.,0.,-1.));
#111850=DIRECTION('ref_axis',(-1.,0.,0.));
#111851=DIRECTION('',(0.,0.,1.));
#111852=DIRECTION('center_axis',(-0.446066534667672,-4.96824693939355E-14,
0.894999802597506));
#111853=DIRECTION('ref_axis',(0.894999802597506,-9.63397512853712E-30,0.446066534667672));
#111854=DIRECTION('center_axis',(-0.434629636675507,0.,0.90060928205483));
#111855=DIRECTION('ref_axis',(0.90060928205483,0.,0.434629636675507));
#111856=DIRECTION('center_axis',(2.67568127619604E-7,-0.999999999999962,
6.13851297333844E-8));
#111857=DIRECTION('ref_axis',(0.690330186704652,1.40298554221222E-7,-0.723494459774435));
#111858=DIRECTION('center_axis',(0.,0.,1.));
#111859=DIRECTION('ref_axis',(1.,0.,0.));
#111860=DIRECTION('center_axis',(0.,0.,1.));
#111861=DIRECTION('ref_axis',(0.,-1.,0.));
#111862=DIRECTION('',(5.16102651992463E-32,-2.15733828054269E-47,1.));
#111863=DIRECTION('',(0.,1.23467863058847E-16,-1.));
#111864=DIRECTION('center_axis',(-4.18005656861882E-16,-1.,0.));
#111865=DIRECTION('ref_axis',(1.,0.,0.));
#111866=DIRECTION('center_axis',(0.,1.,0.));
#111867=DIRECTION('ref_axis',(1.,0.,0.));
#111868=DIRECTION('center_axis',(0.,0.,1.));
#111869=DIRECTION('ref_axis',(1.,0.,0.));
#111870=DIRECTION('center_axis',(0.,0.,1.));
#111871=DIRECTION('ref_axis',(1.,0.,0.));
#111872=DIRECTION('',(0.,0.,-1.));
#111873=DIRECTION('center_axis',(0.,0.,1.));
#111874=DIRECTION('ref_axis',(1.,0.,0.));
#111875=DIRECTION('center_axis',(-0.434677673768106,0.,-0.900586098009262));
#111876=DIRECTION('ref_axis',(-0.900586098009262,0.,0.434677673768106));
#111877=DIRECTION('center_axis',(-4.18005656861882E-16,-1.,0.));
#111878=DIRECTION('ref_axis',(1.,0.,0.));
#111879=DIRECTION('center_axis',(0.,1.,0.));
#111880=DIRECTION('ref_axis',(1.,0.,0.));
#111881=DIRECTION('center_axis',(-1.,0.,0.));
#111882=DIRECTION('ref_axis',(0.,0.,1.));
#111883=DIRECTION('center_axis',(0.,-1.,0.));
#111884=DIRECTION('ref_axis',(1.,0.,0.));
#111885=DIRECTION('center_axis',(4.18005656861881E-16,1.,0.));
#111886=DIRECTION('ref_axis',(-1.,4.18005656861881E-16,0.));
#111887=DIRECTION('',(4.18005656861881E-16,1.,0.));
#111888=DIRECTION('center_axis',(0.,1.,0.));
#111889=DIRECTION('ref_axis',(-1.,0.,0.));
#111890=DIRECTION('center_axis',(4.18005656861882E-16,1.,0.));
#111891=DIRECTION('ref_axis',(-1.,0.,0.));
#111892=DIRECTION('center_axis',(1.,0.,0.));
#111893=DIRECTION('ref_axis',(0.,0.,-1.));
#111894=DIRECTION('center_axis',(0.,-1.,0.));
#111895=DIRECTION('ref_axis',(-1.,0.,0.));
#111896=DIRECTION('center_axis',(0.,0.,-1.));
#111897=DIRECTION('ref_axis',(-1.,0.,0.));
#111898=DIRECTION('center_axis',(0.,0.,-1.));
#111899=DIRECTION('ref_axis',(-1.,0.,0.));
#111900=DIRECTION('',(0.,0.,1.));
#111901=DIRECTION('center_axis',(0.,0.,-1.));
#111902=DIRECTION('ref_axis',(-1.,0.,0.));
#111903=DIRECTION('center_axis',(4.18005656861882E-16,1.,0.));
#111904=DIRECTION('ref_axis',(-1.,0.,0.));
#111905=DIRECTION('center_axis',(0.,-1.,0.));
#111906=DIRECTION('ref_axis',(-1.,0.,0.));
#111907=DIRECTION('center_axis',(-1.,0.,0.));
#111908=DIRECTION('ref_axis',(0.,0.,1.));
#111909=DIRECTION('center_axis',(1.,0.,0.));
#111910=DIRECTION('ref_axis',(0.,1.,0.));
#111911=DIRECTION('',(1.,-4.18005656861881E-16,0.));
#111912=DIRECTION('center_axis',(0.,0.,1.));
#111913=DIRECTION('ref_axis',(0.,-1.,0.));
#111914=DIRECTION('',(-5.16102651992463E-32,2.15733828054269E-47,-1.));
#111915=DIRECTION('center_axis',(0.,0.,-1.));
#111916=DIRECTION('ref_axis',(-1.,0.,0.));
#111917=DIRECTION('',(0.,-1.23467863058847E-16,1.));
#111918=DIRECTION('center_axis',(1.7739481101835E-7,0.999999999999983,4.12226225097212E-8));
#111919=DIRECTION('ref_axis',(0.952173814460364,-1.56314836594747E-7,-0.30555691295727));
#111920=DIRECTION('center_axis',(0.439171790863778,6.20608564480709E-14,
-0.898403104463415));
#111921=DIRECTION('ref_axis',(-0.898403104463415,-1.60954096059593E-29,
-0.439171790863778));
#111922=DIRECTION('center_axis',(0.453758938247726,6.29717026090114E-15,
-0.891124472764774));
#111923=DIRECTION('ref_axis',(-0.891124472764774,1.97126653384901E-30,-0.453758938247726));
#111924=DIRECTION('center_axis',(0.,0.,-1.));
#111925=DIRECTION('ref_axis',(-1.,0.,0.));
#111926=DIRECTION('center_axis',(0.,0.,-1.));
#111927=DIRECTION('ref_axis',(-1.,0.,0.));
#111928=DIRECTION('',(0.,0.,-1.));
#111929=DIRECTION('center_axis',(0.,0.,-1.));
#111930=DIRECTION('ref_axis',(-1.,0.,0.));
#111931=DIRECTION('center_axis',(0.453758938247698,0.,0.891124472764788));
#111932=DIRECTION('ref_axis',(0.891124472764788,0.,-0.453758938247698));
#111933=DIRECTION('center_axis',(0.439239043992112,0.,0.898370225593489));
#111934=DIRECTION('ref_axis',(0.898370225593489,0.,-0.439239043992112));
#111935=DIRECTION('center_axis',(-4.18005656861882E-16,-1.,0.));
#111936=DIRECTION('ref_axis',(1.,0.,0.));
#111937=DIRECTION('center_axis',(1.,0.,0.));
#111938=DIRECTION('ref_axis',(0.,0.,-1.));
#111939=DIRECTION('center_axis',(0.,1.,0.));
#111940=DIRECTION('ref_axis',(1.,0.,0.));
#111941=DIRECTION('center_axis',(0.,0.,1.));
#111942=DIRECTION('ref_axis',(1.,0.,0.));
#111943=DIRECTION('center_axis',(0.,0.,1.));
#111944=DIRECTION('ref_axis',(1.,0.,0.));
#111945=DIRECTION('',(0.,0.,-1.));
#111946=DIRECTION('center_axis',(0.,0.,1.));
#111947=DIRECTION('ref_axis',(1.,0.,0.));
#111948=DIRECTION('center_axis',(0.452924541251067,1.8658316499269E-14,
0.891548854484436));
#111949=DIRECTION('ref_axis',(0.891548854484436,-1.10243984483832E-29,-0.452924541251067));
#111950=DIRECTION('center_axis',(0.473890079491223,-6.57654596740749E-15,
0.880584006531917));
#111951=DIRECTION('ref_axis',(0.880584006531917,-2.59399416170326E-30,-0.473890079491223));
#111952=DIRECTION('center_axis',(0.,0.,1.));
#111953=DIRECTION('ref_axis',(1.,0.,0.));
#111954=DIRECTION('center_axis',(0.,0.,1.));
#111955=DIRECTION('ref_axis',(1.,0.,0.));
#111956=DIRECTION('',(0.,0.,1.));
#111957=DIRECTION('center_axis',(0.,0.,1.));
#111958=DIRECTION('ref_axis',(1.,0.,0.));
#111959=DIRECTION('center_axis',(-0.473890079491229,6.57654596740791E-15,
0.880584006531913));
#111960=DIRECTION('ref_axis',(0.880584006531913,4.48746122839123E-29,0.473890079491229));
#111961=DIRECTION('center_axis',(-0.452796108559755,6.28380831479673E-15,
0.891614089207401));
#111962=DIRECTION('ref_axis',(0.891614089207401,-8.65475050140857E-31,0.452796108559755));
#111963=DIRECTION('center_axis',(2.01185813448576E-8,-1.,4.8563457570887E-9));
#111964=DIRECTION('ref_axis',(0.999508172280242,1.99563942576545E-8,-0.031359425138364));
#111965=DIRECTION('center_axis',(0.,0.,1.));
#111966=DIRECTION('ref_axis',(1.,0.,0.));
#111967=DIRECTION('center_axis',(0.,0.,1.));
#111968=DIRECTION('ref_axis',(0.,-1.,0.));
#111969=DIRECTION('',(5.16102651992463E-32,-2.15733828054269E-47,1.));
#111970=DIRECTION('',(0.,1.23467863058847E-16,-1.));
#111971=DIRECTION('center_axis',(1.,0.,0.));
#111972=DIRECTION('ref_axis',(0.,1.,0.));
#111973=DIRECTION('',(-1.,4.18005656861881E-16,0.));
#111974=DIRECTION('center_axis',(-4.18005656861882E-16,-1.,0.));
#111975=DIRECTION('ref_axis',(1.,0.,0.));
#111976=DIRECTION('center_axis',(0.,1.,0.));
#111977=DIRECTION('ref_axis',(1.,0.,0.));
#111978=DIRECTION('center_axis',(-1.,0.,0.));
#111979=DIRECTION('ref_axis',(0.,0.,1.));
#111980=DIRECTION('center_axis',(0.,-1.,0.));
#111981=DIRECTION('ref_axis',(1.,0.,0.));
#111982=DIRECTION('center_axis',(4.18005656861881E-16,1.,0.));
#111983=DIRECTION('ref_axis',(-1.,4.18005656861881E-16,0.));
#111984=DIRECTION('',(4.18005656861881E-16,1.,0.));
#111985=DIRECTION('center_axis',(0.,1.,0.));
#111986=DIRECTION('ref_axis',(-1.,0.,0.));
#111987=DIRECTION('center_axis',(4.18005656861882E-16,1.,0.));
#111988=DIRECTION('ref_axis',(-1.,0.,0.));
#111989=DIRECTION('center_axis',(1.,0.,0.));
#111990=DIRECTION('ref_axis',(0.,0.,-1.));
#111991=DIRECTION('center_axis',(0.,-1.,0.));
#111992=DIRECTION('ref_axis',(-1.,0.,0.));
#111993=DIRECTION('center_axis',(-4.18005656861882E-16,-1.,0.));
#111994=DIRECTION('ref_axis',(1.,-5.9211894646675E-16,0.));
#111995=DIRECTION('center_axis',(6.93889390390722E-16,1.,0.));
#111996=DIRECTION('ref_axis',(1.,-6.93889390390722E-16,0.));
#111997=DIRECTION('center_axis',(-1.,0.,0.));
#111998=DIRECTION('ref_axis',(0.,0.,1.));
#111999=DIRECTION('center_axis',(-5.78241158658935E-16,-1.,0.));
#112000=DIRECTION('ref_axis',(1.,-5.78241158658935E-16,0.));
#112001=DIRECTION('center_axis',(4.18005656861881E-16,1.,0.));
#112002=DIRECTION('ref_axis',(-1.,4.18005656861881E-16,0.));
#112003=DIRECTION('',(4.18005656861881E-16,1.,0.));
#112004=DIRECTION('center_axis',(5.78241158658935E-16,1.,0.));
#112005=DIRECTION('ref_axis',(-1.,5.78241158658935E-16,0.));
#112006=DIRECTION('center_axis',(4.18005656861882E-16,1.,0.));
#112007=DIRECTION('ref_axis',(-1.,5.9211894646675E-16,0.));
#112008=DIRECTION('center_axis',(1.,0.,0.));
#112009=DIRECTION('ref_axis',(0.,0.,-1.));
#112010=DIRECTION('center_axis',(-6.93889390390722E-16,-1.,0.));
#112011=DIRECTION('ref_axis',(-1.,6.93889390390722E-16,0.));
#112012=DIRECTION('center_axis',(0.,0.424147858891027,0.905592951495404));
#112013=DIRECTION('ref_axis',(0.,-0.905592951495404,0.424147858891027));
#112014=DIRECTION('center_axis',(0.,0.425268108821871,0.905067420482623));
#112015=DIRECTION('ref_axis',(0.,-0.905067420482623,0.425268108821871));
#112016=DIRECTION('center_axis',(0.,0.429430624963615,0.903099849597684));
#112017=DIRECTION('ref_axis',(0.,-0.903099849597684,0.429430624963615));
#112018=DIRECTION('center_axis',(0.,0.434584798675586,0.900630919278314));
#112019=DIRECTION('ref_axis',(0.,-0.900630919278314,0.434584798675586));
#112020=DIRECTION('center_axis',(0.,0.440696042277477,0.89765639212394));
#112021=DIRECTION('ref_axis',(0.,-0.89765639212394,0.440696042277477));
#112022=DIRECTION('center_axis',(-0.998868362320773,-0.00644281759551,-0.0471220209249073));
#112023=DIRECTION('ref_axis',(0.0465471507530001,-0.335857313107545,-0.940762046422451));
#112024=DIRECTION('center_axis',(0.,0.425920949091245,0.904760379948864));
#112025=DIRECTION('ref_axis',(0.,-0.904760379948864,0.425920949091245));
#112026=DIRECTION('center_axis',(0.,0.432834338283548,0.901473480254768));
#112027=DIRECTION('ref_axis',(0.,-0.901473480254768,0.432834338283548));
#112028=DIRECTION('center_axis',(-1.85986770746484E-14,0.444295746197836,
0.895880176089698));
#112029=DIRECTION('ref_axis',(-8.37014173169963E-31,-0.895880176089698,
0.444295746197836));
#112030=DIRECTION('center_axis',(0.,0.457805146562934,0.88905255625328));
#112031=DIRECTION('ref_axis',(0.,-0.88905255625328,0.457805146562934));
#112032=DIRECTION('center_axis',(0.,0.,1.));
#112033=DIRECTION('ref_axis',(1.,0.,0.));
#112034=DIRECTION('center_axis',(0.,8.19208946723988E-32,1.));
#112035=DIRECTION('ref_axis',(1.,0.,0.));
#112036=DIRECTION('',(-1.87032180698308E-16,8.19208946723987E-32,1.));
#112037=DIRECTION('center_axis',(0.,0.,1.));
#112038=DIRECTION('ref_axis',(1.,0.,0.));
#112039=DIRECTION('',(1.87032180698308E-16,-8.19208946723987E-32,-1.));
#112040=DIRECTION('center_axis',(1.,0.,1.87032180698308E-16));
#112041=DIRECTION('ref_axis',(0.,0.,-1.));
#112042=DIRECTION('center_axis',(0.,0.,1.));
#112043=DIRECTION('ref_axis',(1.,0.,0.));
#112044=DIRECTION('center_axis',(-1.,0.,0.));
#112045=DIRECTION('ref_axis',(0.,0.,-1.));
#112046=DIRECTION('center_axis',(0.,-1.,0.));
#112047=DIRECTION('ref_axis',(0.,0.,-1.));
#112048=DIRECTION('center_axis',(1.,0.,0.));
#112049=DIRECTION('ref_axis',(0.,0.,-1.));
#112050=DIRECTION('center_axis',(-1.,0.,0.));
#112051=DIRECTION('ref_axis',(0.,0.,1.));
#112052=DIRECTION('',(1.,0.,0.));
#112053=DIRECTION('',(-1.,0.,0.));
#112054=DIRECTION('center_axis',(-1.,0.,0.));
#112055=DIRECTION('ref_axis',(0.,0.,1.));
#112056=DIRECTION('center_axis',(-1.,0.,0.));
#112057=DIRECTION('ref_axis',(0.,0.,1.));
#112058=DIRECTION('center_axis',(0.,1.,0.));
#112059=DIRECTION('ref_axis',(0.,0.,1.));
#112060=DIRECTION('center_axis',(1.,0.,0.));
#112061=DIRECTION('ref_axis',(0.,0.,1.));
#112062=DIRECTION('center_axis',(0.,0.,-1.));
#112063=DIRECTION('ref_axis',(-1.,0.,0.));
#112064=DIRECTION('center_axis',(0.,0.,-1.));
#112065=DIRECTION('ref_axis',(-1.,0.,0.));
#112066=DIRECTION('center_axis',(0.,0.,1.));
#112067=DIRECTION('ref_axis',(1.,0.,0.));
#112068=DIRECTION('',(0.,0.,1.));
#112069=DIRECTION('center_axis',(0.,0.,1.));
#112070=DIRECTION('ref_axis',(1.,0.,0.));
#112071=DIRECTION('',(0.,0.,-1.));
#112072=DIRECTION('center_axis',(0.,0.466134040541469,0.884714109895668));
#112073=DIRECTION('ref_axis',(0.,-0.884714109895668,0.466134040541469));
#112074=DIRECTION('center_axis',(0.,0.450823097219337,0.892613317743783));
#112075=DIRECTION('ref_axis',(0.,-0.892613317743783,0.450823097219337));
#112076=DIRECTION('center_axis',(3.33932916167122E-16,0.999710458475598,
0.0240624025090732));
#112077=DIRECTION('ref_axis',(-2.2263435019713E-33,-0.0240624025090732,
0.999710458475598));
#112078=DIRECTION('center_axis',(0.,0.605101105507222,0.796148636947862));
#112079=DIRECTION('ref_axis',(0.,-0.796148636947862,0.605101105507222));
#112080=DIRECTION('center_axis',(-0.98202959189485,0.188726538511571,0.0004174976347577));
#112081=DIRECTION('ref_axis',(-0.153131413400455,-0.798101172975176,0.58273946830949));
#112082=DIRECTION('center_axis',(1.,0.,0.));
#112083=DIRECTION('ref_axis',(0.,-0.892435299537773,0.451175393986558));
#112084=DIRECTION('center_axis',(0.,-1.18842113532926E-16,1.));
#112085=DIRECTION('ref_axis',(0.,1.,1.18842113532926E-16));
#112086=DIRECTION('center_axis',(0.,1.19392659184112E-16,-1.));
#112087=DIRECTION('ref_axis',(0.,1.,1.19392659184112E-16));
#112088=DIRECTION('center_axis',(1.,-5.01606788234257E-16,0.));
#112089=DIRECTION('ref_axis',(0.,1.,0.));
#112090=DIRECTION('center_axis',(0.,-1.,0.));
#112091=DIRECTION('ref_axis',(0.,0.,-1.));
#112092=DIRECTION('center_axis',(-1.,0.,0.));
#112093=DIRECTION('ref_axis',(0.,1.,0.));
#112094=DIRECTION('center_axis',(0.,0.,-1.));
#112095=DIRECTION('ref_axis',(-1.,0.,0.));
#112096=DIRECTION('center_axis',(1.,0.,0.));
#112097=DIRECTION('ref_axis',(0.,1.,0.));
#112098=DIRECTION('center_axis',(-2.85977186515575E-47,0.,-1.));
#112099=DIRECTION('ref_axis',(0.,1.,0.));
#112100=DIRECTION('',(2.85977186515575E-47,5.70122241611331E-32,1.));
#112101=DIRECTION('center_axis',(0.,0.,-1.));
#112102=DIRECTION('ref_axis',(-1.,0.,0.));
#112103=DIRECTION('center_axis',(1.,-5.01606788234257E-16,0.));
#112104=DIRECTION('ref_axis',(0.,1.,0.));
#112105=DIRECTION('center_axis',(-1.,0.,0.));
#112106=DIRECTION('ref_axis',(0.,1.,0.));
#112107=DIRECTION('center_axis',(0.,1.,0.));
#112108=DIRECTION('ref_axis',(0.,0.,1.));
#112109=DIRECTION('center_axis',(0.,-0.452474032063612,-0.891777578944491));
#112110=DIRECTION('ref_axis',(0.,0.891777578944491,-0.452474032063612));
#112111=DIRECTION('center_axis',(6.4968286789756E-15,-0.468145843483589,
-0.883651214693354));
#112112=DIRECTION('ref_axis',(1.16233255777344E-30,0.883651214693354,-0.468145843483589));
#112113=DIRECTION('center_axis',(0.,0.,-1.));
#112114=DIRECTION('ref_axis',(-1.,0.,0.));
#112115=DIRECTION('center_axis',(0.,0.,-1.));
#112116=DIRECTION('ref_axis',(-1.,0.,0.));
#112117=DIRECTION('',(0.,0.,-1.));
#112118=DIRECTION('center_axis',(0.,0.,-1.));
#112119=DIRECTION('ref_axis',(-1.,0.,0.));
#112120=DIRECTION('center_axis',(6.4968286789753E-15,0.468145843483567,
-0.883651214693365));
#112121=DIRECTION('ref_axis',(-8.06613026210763E-31,0.883651214693365,0.468145843483567));
#112122=DIRECTION('center_axis',(-1.87193934265674E-16,0.452600956351886,
-0.8917131681821));
#112123=DIRECTION('ref_axis',(-4.92064035297146E-32,0.8917131681821,0.452600956351886));
#112124=DIRECTION('center_axis',(-1.,5.01606788234257E-16,0.));
#112125=DIRECTION('ref_axis',(0.,-1.,0.));
#112126=DIRECTION('center_axis',(0.,-1.,0.));
#112127=DIRECTION('ref_axis',(0.,0.,-1.));
#112128=DIRECTION('center_axis',(1.,0.,0.));
#112129=DIRECTION('ref_axis',(0.,-1.,0.));
#112130=DIRECTION('center_axis',(0.,0.,1.));
#112131=DIRECTION('ref_axis',(1.,0.,0.));
#112132=DIRECTION('center_axis',(2.85977186515575E-47,0.,1.));
#112133=DIRECTION('ref_axis',(0.,-1.,0.));
#112134=DIRECTION('',(-2.85977186515575E-47,-5.70122241611331E-32,-1.));
#112135=DIRECTION('center_axis',(0.,0.,1.));
#112136=DIRECTION('ref_axis',(1.,0.,0.));
#112137=DIRECTION('center_axis',(0.,0.,-1.));
#112138=DIRECTION('ref_axis',(-1.,0.,0.));
#112139=DIRECTION('center_axis',(0.,0.450013465461336,-0.893021769557427));
#112140=DIRECTION('ref_axis',(0.,0.893021769557427,0.450013465461336));
#112141=DIRECTION('center_axis',(0.,0.,1.));
#112142=DIRECTION('ref_axis',(1.,0.,0.));
#112143=DIRECTION('center_axis',(0.,0.,-1.));
#112144=DIRECTION('ref_axis',(-1.,0.,0.));
#112145=DIRECTION('',(0.,0.,1.));
#112146=DIRECTION('center_axis',(0.,-0.450013465459867,-0.893021769558168));
#112147=DIRECTION('ref_axis',(0.,0.893021769558168,-0.450013465459867));
#112148=DIRECTION('center_axis',(0.,-0.438949247410394,-0.898511857572202));
#112149=DIRECTION('ref_axis',(0.,0.898511857572202,-0.438949247410394));
#112150=DIRECTION('center_axis',(0.,0.439015545441723,-0.898479466020513));
#112151=DIRECTION('ref_axis',(0.,0.898479466020513,0.439015545441723));
#112152=DIRECTION('center_axis',(-1.,5.01606788234257E-16,0.));
#112153=DIRECTION('ref_axis',(0.,-1.,0.));
#112154=DIRECTION('center_axis',(1.,0.,0.));
#112155=DIRECTION('ref_axis',(0.,-1.,0.));
#112156=DIRECTION('center_axis',(0.,1.,0.));
#112157=DIRECTION('ref_axis',(0.,0.,1.));
#112158=DIRECTION('center_axis',(-1.,0.,0.));
#112159=DIRECTION('ref_axis',(0.,-1.,0.));
#112160=DIRECTION('center_axis',(1.,-5.01606788234257E-16,0.));
#112161=DIRECTION('ref_axis',(5.01606788234257E-16,1.,0.));
#112162=DIRECTION('',(1.,-5.01606788234257E-16,0.));
#112163=DIRECTION('center_axis',(1.,0.,0.));
#112164=DIRECTION('ref_axis',(0.,1.,0.));
#112165=DIRECTION('center_axis',(1.,-5.01606788234257E-16,0.));
#112166=DIRECTION('ref_axis',(0.,1.,0.));
#112167=DIRECTION('center_axis',(0.,-1.,0.));
#112168=DIRECTION('ref_axis',(0.,0.,-1.));
#112169=DIRECTION('center_axis',(-1.,6.93889390390722E-16,0.));
#112170=DIRECTION('ref_axis',(6.93889390390722E-16,1.,0.));
#112171=DIRECTION('center_axis',(0.,0.,-1.));
#112172=DIRECTION('ref_axis',(-1.,0.,0.));
#112173=DIRECTION('center_axis',(-2.85977186515575E-47,0.,-1.));
#112174=DIRECTION('ref_axis',(0.,1.,0.));
#112175=DIRECTION('',(2.85977186515575E-47,5.70122241611331E-32,1.));
#112176=DIRECTION('center_axis',(0.,0.,-1.));
#112177=DIRECTION('ref_axis',(-1.,0.,0.));
#112178=DIRECTION('center_axis',(1.,-5.01606788234257E-16,0.));
#112179=DIRECTION('ref_axis',(0.,1.,0.));
#112180=DIRECTION('center_axis',(-1.,6.93889390390722E-16,0.));
#112181=DIRECTION('ref_axis',(6.93889390390722E-16,1.,0.));
#112182=DIRECTION('center_axis',(0.,1.,0.));
#112183=DIRECTION('ref_axis',(0.,0.,1.));
#112184=DIRECTION('center_axis',(0.,-0.434444534286154,-0.900698588113075));
#112185=DIRECTION('ref_axis',(0.,0.900698588113075,-0.434444534286154));
#112186=DIRECTION('center_axis',(6.14994601925012E-15,-0.443150313610303,
-0.896447321122156));
#112187=DIRECTION('ref_axis',(-3.80752501607971E-29,0.896447321122156,-0.443150313610303));
#112188=DIRECTION('center_axis',(0.,0.,-1.));
#112189=DIRECTION('ref_axis',(-1.,0.,0.));
#112190=DIRECTION('center_axis',(0.,0.,-1.));
#112191=DIRECTION('ref_axis',(-1.,0.,0.));
#112192=DIRECTION('',(0.,0.,-1.));
#112193=DIRECTION('center_axis',(0.,0.,-1.));
#112194=DIRECTION('ref_axis',(-1.,0.,0.));
#112195=DIRECTION('center_axis',(3.10313574260842E-14,0.443150313610309,
-0.896447321122153));
#112196=DIRECTION('ref_axis',(-1.13003852554043E-30,0.896447321122153,0.443150313610309));
#112197=DIRECTION('center_axis',(4.39817443652073E-16,0.434491800625061,
-0.900675788055609));
#112198=DIRECTION('ref_axis',(-9.63119795361041E-32,0.900675788055609,0.434491800625061));
#112199=DIRECTION('center_axis',(0.,0.,-1.));
#112200=DIRECTION('ref_axis',(-1.,0.,0.));
#112201=DIRECTION('center_axis',(0.,0.430903547306764,-0.902397990311618));
#112202=DIRECTION('ref_axis',(0.,0.902397990311618,0.430903547306764));
#112203=DIRECTION('center_axis',(0.,0.,1.));
#112204=DIRECTION('ref_axis',(1.,0.,0.));
#112205=DIRECTION('center_axis',(0.,0.,-1.));
#112206=DIRECTION('ref_axis',(-1.,0.,0.));
#112207=DIRECTION('',(0.,0.,1.));
#112208=DIRECTION('center_axis',(0.,-0.430903547308298,-0.902397990310886));
#112209=DIRECTION('ref_axis',(0.,0.902397990310886,-0.430903547308298));
#112210=DIRECTION('center_axis',(0.,-0.427115883537276,-0.904196893397767));
#112211=DIRECTION('ref_axis',(0.,0.904196893397767,-0.427115883537276));
#112212=DIRECTION('center_axis',(0.,0.427133403156944,-0.904188617439729));
#112213=DIRECTION('ref_axis',(0.,0.904188617439729,0.427133403156944));
#112214=DIRECTION('center_axis',(2.85977186515575E-47,0.,1.));
#112215=DIRECTION('ref_axis',(0.,-1.,0.));
#112216=DIRECTION('center_axis',(0.,0.,1.));
#112217=DIRECTION('ref_axis',(1.,0.,0.));
#112218=DIRECTION('',(-2.85977186515575E-47,-5.70122241611331E-32,-1.));
#112219=DIRECTION('center_axis',(0.,0.,1.));
#112220=DIRECTION('ref_axis',(1.,0.,0.));
#112221=DIRECTION('',(2.85977186515575E-47,5.70122241611331E-32,1.));
#112222=DIRECTION('center_axis',(-5.01606788234257E-16,-1.,5.70122241611331E-32));
#112223=DIRECTION('ref_axis',(-1.,5.01606788234257E-16,0.));
#112224=DIRECTION('',(-2.85977186515575E-47,-5.70122241611331E-32,-1.));
#112225=DIRECTION('center_axis',(-2.85977186515575E-47,0.,-1.));
#112226=DIRECTION('ref_axis',(0.,1.,0.));
#112227=DIRECTION('center_axis',(0.,0.,-1.));
#112228=DIRECTION('ref_axis',(-1.,0.,0.));
#112229=DIRECTION('',(2.85977186515575E-47,5.70122241611331E-32,1.));
#112230=DIRECTION('center_axis',(0.,0.,-1.));
#112231=DIRECTION('ref_axis',(-1.,0.,0.));
#112232=DIRECTION('center_axis',(0.,-0.425023904828957,-0.905182125499585));
#112233=DIRECTION('ref_axis',(0.,0.905182125499585,-0.425023904828957));
#112234=DIRECTION('center_axis',(-5.01926581554439E-14,-0.427129320053956,
-0.904190546262371));
#112235=DIRECTION('ref_axis',(-3.44539770291064E-30,0.904190546262371,-0.427129320053956));
#112236=DIRECTION('center_axis',(0.,0.,-1.));
#112237=DIRECTION('ref_axis',(-1.,0.,0.));
#112238=DIRECTION('center_axis',(0.,0.,-1.));
#112239=DIRECTION('ref_axis',(-1.,0.,0.));
#112240=DIRECTION('',(0.,0.,-1.));
#112241=DIRECTION('center_axis',(0.,0.,-1.));
#112242=DIRECTION('ref_axis',(-1.,0.,0.));
#112243=DIRECTION('center_axis',(5.9276100702047E-15,0.42712932005395,-0.904190546262374));
#112244=DIRECTION('ref_axis',(3.36279389150844E-29,0.904190546262374,0.42712932005395));
#112245=DIRECTION('center_axis',(-1.25618648527741E-14,0.425033206427438,
-0.905177757920515));
#112246=DIRECTION('ref_axis',(2.68759262534439E-30,0.905177757920515,0.425033206427438));
#112247=DIRECTION('center_axis',(-0.999980559779821,0.00244847680975066,
-0.00573454651630453));
#112248=DIRECTION('ref_axis',(0.00115079471073239,0.976348942497979,0.216197636792386));
#112249=DIRECTION('center_axis',(0.,0.,-1.));
#112250=DIRECTION('ref_axis',(-1.,0.,0.));
#112251=DIRECTION('center_axis',(0.,0.422768104239746,-0.906237899250264));
#112252=DIRECTION('ref_axis',(0.,0.906237899250264,0.422768104239746));
#112253=DIRECTION('center_axis',(1.,0.,0.));
#112254=DIRECTION('ref_axis',(0.,0.976373434674857,0.216090064698084));
#112255=DIRECTION('center_axis',(0.,0.,1.));
#112256=DIRECTION('ref_axis',(1.,0.,0.));
#112257=DIRECTION('center_axis',(0.,0.,-1.));
#112258=DIRECTION('ref_axis',(-1.,0.,0.));
#112259=DIRECTION('',(0.,0.,1.));
#112260=DIRECTION('center_axis',(0.,-0.422768104239797,-0.90623789925024));
#112261=DIRECTION('ref_axis',(0.,0.90623789925024,-0.422768104239797));
#112262=DIRECTION('center_axis',(1.,0.,0.));
#112263=DIRECTION('ref_axis',(0.,0.976105817825331,-0.217295725700119));
#112264=DIRECTION('center_axis',(0.,-0.422696564637279,-0.906271269678038));
#112265=DIRECTION('ref_axis',(0.,0.906271269678038,-0.422696564637279));
#112266=DIRECTION('center_axis',(0.,0.422696864907095,-0.906271129628277));
#112267=DIRECTION('ref_axis',(0.,0.906271129628277,0.422696864907095));
#112268=DIRECTION('center_axis',(0.,0.,1.));
#112269=DIRECTION('ref_axis',(1.,0.,0.));
#112270=DIRECTION('',(5.01606788234257E-16,1.,0.));
#112271=DIRECTION('center_axis',(0.,0.,1.));
#112272=DIRECTION('ref_axis',(1.,0.,0.));
#112273=DIRECTION('',(-5.01606788234257E-16,-1.,0.));
#112274=DIRECTION('center_axis',(0.,-1.,0.));
#112275=DIRECTION('ref_axis',(1.,0.,0.));
#112276=DIRECTION('',(5.01606788234257E-16,1.,0.));
#112277=DIRECTION('center_axis',(-0.691017694403315,-0.329301163645224,
-0.643471281133376));
#112278=DIRECTION('ref_axis',(-0.681480917945783,1.81728452038657E-16,0.731835882200219));
#112279=DIRECTION('center_axis',(0.,0.,-1.));
#112280=DIRECTION('ref_axis',(-1.,0.,0.));
#112281=DIRECTION('center_axis',(0.,0.,1.));
#112282=DIRECTION('ref_axis',(0.,-1.,0.));
#112283=DIRECTION('',(0.,1.23467863058847E-16,-1.));
#112284=DIRECTION('',(-6.19323182390956E-32,-1.23467863058847E-16,1.));
#112285=DIRECTION('center_axis',(0.,0.,-1.));
#112286=DIRECTION('ref_axis',(-1.,0.,0.));
#112287=DIRECTION('center_axis',(0.999946261821081,-0.0103669398946897,
5.22173233649368E-6));
#112288=DIRECTION('ref_axis',(0.0101220853315265,0.976219669473995,-0.216547224227478));
#112289=DIRECTION('center_axis',(-1.,0.,0.));
#112290=DIRECTION('ref_axis',(0.,0.976212736710707,-0.216814881140091));
#112291=DIRECTION('center_axis',(0.,0.,-1.));
#112292=DIRECTION('ref_axis',(1.,0.,0.));
#112293=DIRECTION('center_axis',(0.,0.,1.));
#112294=DIRECTION('ref_axis',(0.,-1.,0.));
#112295=DIRECTION('center_axis',(0.,0.,-1.));
#112296=DIRECTION('ref_axis',(-1.,0.,0.));
#112297=DIRECTION('center_axis',(1.,0.,0.));
#112298=DIRECTION('ref_axis',(0.,0.978009404010872,-0.20856079609145));
#112299=DIRECTION('center_axis',(-0.998408908923169,0.0563883836225873,
-2.7843844968591E-5));
#112300=DIRECTION('ref_axis',(0.055246667114195,0.978094652824472,-0.200695430662856));
#112301=DIRECTION('center_axis',(-0.0107605169339556,0.163442104496002,
0.986494242128778));
#112302=DIRECTION('ref_axis',(0.12265223013178,-0.978886010491001,0.163519445047717));
#112303=DIRECTION('center_axis',(0.,0.,-1.));
#112304=DIRECTION('ref_axis',(-1.,0.,0.));
#112305=DIRECTION('center_axis',(0.997120695413915,-0.0758308469044614,
3.78816969998108E-5));
#112306=DIRECTION('ref_axis',(0.0744761237692872,0.979212817695212,-0.188667868620245));
#112307=DIRECTION('center_axis',(-1.,0.,0.));
#112308=DIRECTION('ref_axis',(0.,0.979170381919184,-0.203040299379802));
#112309=DIRECTION('center_axis',(0.,0.,-1.));
#112310=DIRECTION('ref_axis',(1.,0.,0.));
#112311=DIRECTION('center_axis',(0.,0.,1.));
#112312=DIRECTION('ref_axis',(0.,-1.,0.));
#112313=DIRECTION('center_axis',(0.,0.,-1.));
#112314=DIRECTION('ref_axis',(-1.,0.,0.));
#112315=DIRECTION('center_axis',(0.999999999999962,-2.70358732879246E-7,
6.19928773069953E-8));
#112316=DIRECTION('ref_axis',(-1.37951239417795E-7,-0.67866125427495,-0.734451429262638));
#112317=DIRECTION('center_axis',(-0.9932262444019,0.116196489921731,-5.62242552552882E-5));
#112318=DIRECTION('ref_axis',(0.11505091787893,0.983366096661123,-0.140550369023647));
#112319=DIRECTION('center_axis',(0.,-1.,0.));
#112320=DIRECTION('ref_axis',(1.,0.,0.));
#112321=DIRECTION('',(-5.01606788234257E-16,-1.,0.));
#112322=DIRECTION('',(5.01606788234257E-16,1.,0.));
#112323=DIRECTION('center_axis',(0.,0.,1.));
#112324=DIRECTION('ref_axis',(1.,0.,0.));
#112325=DIRECTION('center_axis',(0.,0.,1.));
#112326=DIRECTION('ref_axis',(1.,0.,0.));
#112327=DIRECTION('',(-5.01606788234257E-16,-1.,0.));
#112328=DIRECTION('center_axis',(0.,-1.,0.));
#112329=DIRECTION('ref_axis',(1.,0.,0.));
#112330=DIRECTION('',(5.01606788234257E-16,1.,0.));
#112331=DIRECTION('center_axis',(0.,0.,-1.));
#112332=DIRECTION('ref_axis',(-1.,0.,0.));
#112333=DIRECTION('center_axis',(0.991243176770489,-0.132049083222371,6.42345784418605E-5));
#112334=DIRECTION('ref_axis',(0.131204337993624,0.984846821255349,-0.113411464830016));
#112335=DIRECTION('center_axis',(-0.999999999999982,-1.83115630218257E-7,
4.25253736080571E-8));
#112336=DIRECTION('ref_axis',(1.60098201248805E-7,-0.948126339790581,-0.317893761806189));
#112337=DIRECTION('center_axis',(0.,0.,-1.));
#112338=DIRECTION('ref_axis',(1.,0.,0.));
#112339=DIRECTION('center_axis',(0.,0.,1.));
#112340=DIRECTION('ref_axis',(0.,-1.,0.));
#112341=DIRECTION('center_axis',(0.,0.,-1.));
#112342=DIRECTION('ref_axis',(-1.,0.,0.));
#112343=DIRECTION('center_axis',(1.,-2.01122486990919E-8,4.85048672787675E-9));
#112344=DIRECTION('ref_axis',(1.993567842142E-8,0.999421676189316,0.0340046050254766));
#112345=DIRECTION('center_axis',(-0.986748267175955,0.162258595028188,-7.45971144795321E-5));
#112346=DIRECTION('ref_axis',(0.162166590547152,0.986173067657473,-0.0341273722598251));
#112347=DIRECTION('center_axis',(0.,-1.,0.));
#112348=DIRECTION('ref_axis',(1.,0.,0.));
#112349=DIRECTION('',(-5.01606788234257E-16,-1.,0.));
#112350=DIRECTION('center_axis',(0.,1.23467863058847E-16,-1.));
#112351=DIRECTION('ref_axis',(-1.,0.,0.));
#112352=DIRECTION('center_axis',(0.,0.,-1.));
#112353=DIRECTION('ref_axis',(0.,1.,0.));
#112354=DIRECTION('',(2.0158362407235E-32,-1.,-1.23467863058847E-16));
#112355=DIRECTION('center_axis',(0.,1.23467863058847E-16,-1.));
#112356=DIRECTION('ref_axis',(-1.,0.,0.));
#112357=DIRECTION('',(2.0158362407235E-32,-1.,-1.23467863058847E-16));
#112358=DIRECTION('center_axis',(0.,0.,-1.));
#112359=DIRECTION('ref_axis',(0.,1.,0.));
#112360=DIRECTION('center_axis',(0.,1.23467863058847E-16,-1.));
#112361=DIRECTION('ref_axis',(-1.,0.,0.));
#112362=DIRECTION('center_axis',(0.,0.,-1.));
#112363=DIRECTION('ref_axis',(0.,-1.,0.));
#112364=DIRECTION('center_axis',(0.,1.23467863058847E-16,-1.));
#112365=DIRECTION('ref_axis',(-1.,0.,0.));
#112366=DIRECTION('center_axis',(0.,0.,-1.));
#112367=DIRECTION('ref_axis',(0.,-1.,0.));
#112368=DIRECTION('center_axis',(0.,0.,-1.));
#112369=DIRECTION('ref_axis',(0.,-1.,0.));
#112370=DIRECTION('center_axis',(0.139173100960059,-0.990268068741571,-1.22266282302934E-16));
#112371=DIRECTION('ref_axis',(6.9401346861194E-34,1.23467863058847E-16,
-1.));
#112372=DIRECTION('',(-3.43088182518023E-33,1.23467863058847E-16,-1.));
#112373=DIRECTION('',(0.990268068741571,0.139173100960059,1.71834053708117E-17));
#112374=DIRECTION('',(3.43088182518023E-33,-1.23467863058847E-16,1.));
#112375=DIRECTION('center_axis',(0.,0.,-1.));
#112376=DIRECTION('ref_axis',(0.,1.,0.));
#112377=DIRECTION('center_axis',(0.,0.,1.));
#112378=DIRECTION('ref_axis',(0.,-1.,0.));
#112379=DIRECTION('',(0.,1.23467863058847E-16,-1.));
#112380=DIRECTION('center_axis',(0.,0.,-1.));
#112381=DIRECTION('ref_axis',(0.,1.,0.));
#112382=DIRECTION('center_axis',(0.,0.,1.));
#112383=DIRECTION('ref_axis',(0.,-1.,0.));
#112384=DIRECTION('',(0.,-1.23467863058847E-16,1.));
#112385=DIRECTION('center_axis',(0.,0.,-1.));
#112386=DIRECTION('ref_axis',(0.,1.,0.));
#112387=DIRECTION('center_axis',(0.,0.,1.));
#112388=DIRECTION('ref_axis',(0.,-1.,0.));
#112389=DIRECTION('',(3.79382742684518E-34,1.23467863058847E-16,-1.));
#112390=DIRECTION('center_axis',(0.99026806874157,-0.139173100960065,-1.71834053708124E-17));
#112391=DIRECTION('ref_axis',(2.50622989185404E-33,1.23467863058847E-16,
-1.));
#112392=DIRECTION('',(0.139173100960065,0.99026806874157,1.22266282302933E-16));
#112393=DIRECTION('',(-3.79382742684518E-34,-1.23467863058847E-16,1.));
#112394=DIRECTION('center_axis',(0.,0.,1.));
#112395=DIRECTION('ref_axis',(0.,-1.,0.));
#112396=DIRECTION('',(0.,1.23467863058847E-16,-1.));
#112397=DIRECTION('center_axis',(0.,0.,-1.));
#112398=DIRECTION('ref_axis',(0.,-1.,0.));
#112399=DIRECTION('center_axis',(0.,0.,1.));
#112400=DIRECTION('ref_axis',(0.,-1.,0.));
#112401=DIRECTION('',(0.,-1.23467863058847E-16,1.));
#112402=DIRECTION('center_axis',(0.,0.,1.));
#112403=DIRECTION('ref_axis',(0.,-1.,0.));
#112404=DIRECTION('center_axis',(0.,0.,1.));
#112405=DIRECTION('ref_axis',(0.,-1.,0.));
#112406=DIRECTION('center_axis',(0.,0.,-1.));
#112407=DIRECTION('ref_axis',(0.,-1.,0.));
#112408=DIRECTION('',(3.05149908249585E-33,1.23467863058847E-16,-1.));
#112409=DIRECTION('center_axis',(0.99026806874157,0.139173100960067,1.71834053708127E-17));
#112410=DIRECTION('ref_axis',(1.48746998541713E-33,1.23467863058847E-16,
-1.));
#112411=DIRECTION('',(-0.139173100960067,0.99026806874157,1.22266282302933E-16));
#112412=DIRECTION('',(-3.05149908249585E-33,-1.23467863058847E-16,1.));
#112413=DIRECTION('center_axis',(0.,0.,-1.));
#112414=DIRECTION('ref_axis',(0.,1.,0.));
#112415=DIRECTION('center_axis',(0.,0.,1.));
#112416=DIRECTION('ref_axis',(0.,-1.,0.));
#112417=DIRECTION('',(0.,1.23467863058847E-16,-1.));
#112418=DIRECTION('center_axis',(0.,0.,-1.));
#112419=DIRECTION('ref_axis',(0.,1.,0.));
#112420=DIRECTION('center_axis',(0.,0.,1.));
#112421=DIRECTION('ref_axis',(0.,-1.,0.));
#112422=DIRECTION('',(0.,-1.23467863058847E-16,1.));
#112423=DIRECTION('center_axis',(0.,0.,-1.));
#112424=DIRECTION('ref_axis',(0.,1.,0.));
#112425=DIRECTION('center_axis',(0.,0.,1.));
#112426=DIRECTION('ref_axis',(0.,-1.,0.));
#112427=DIRECTION('',(3.43088182518023E-33,1.23467863058847E-16,-1.));
#112428=DIRECTION('center_axis',(0.139173100960059,0.990268068741571,1.22266282302934E-16));
#112429=DIRECTION('ref_axis',(8.78519494496445E-16,5.20658772030138E-33,
-1.));
#112430=DIRECTION('',(-3.43088182518023E-33,-1.23467863058847E-16,1.));
#112431=DIRECTION('',(0.990268068741571,-0.139173100960059,0.));
#112432=DIRECTION('',(-1.6326809185664E-16,-1.0052202914905E-16,1.));
#112433=DIRECTION('',(-0.990268068741571,0.139173100960059,1.71834053708117E-17));
#112434=DIRECTION('center_axis',(0.,0.,1.));
#112435=DIRECTION('ref_axis',(1.,0.,0.));
#112436=DIRECTION('center_axis',(0.990268068741572,-0.139173100960052,0.));
#112437=DIRECTION('ref_axis',(0.139173100960052,0.990268068741572,0.));
#112438=DIRECTION('center_axis',(0.,-1.0052202914905E-16,1.));
#112439=DIRECTION('ref_axis',(1.,0.,0.));
#112440=DIRECTION('center_axis',(0.,0.,1.));
#112441=DIRECTION('ref_axis',(1.,0.,0.));
#112442=DIRECTION('',(1.6326809185664E-16,1.00522029149049E-16,-1.));
#112443=DIRECTION('center_axis',(0.,-1.,0.));
#112444=DIRECTION('ref_axis',(0.,0.,-1.));
#112445=DIRECTION('center_axis',(2.0158362407235E-32,-1.,0.));
#112446=DIRECTION('ref_axis',(0.,0.,-1.));
#112447=DIRECTION('center_axis',(-1.41612495910826E-31,-1.,0.));
#112448=DIRECTION('ref_axis',(0.,0.,-1.));
#112449=DIRECTION('',(-2.0158362407235E-32,1.,1.23467863058847E-16));
#112450=DIRECTION('center_axis',(0.,-1.,0.));
#112451=DIRECTION('ref_axis',(0.,0.,-1.));
#112452=DIRECTION('center_axis',(2.0158362407235E-32,-1.,0.));
#112453=DIRECTION('ref_axis',(0.,0.,-1.));
#112454=DIRECTION('',(-2.0158362407235E-32,1.,1.23467863058847E-16));
#112455=DIRECTION('center_axis',(0.,7.15121221728469E-32,1.));
#112456=DIRECTION('ref_axis',(1.,0.,0.));
#112457=DIRECTION('',(-1.6326809185664E-16,7.15121221728469E-32,1.));
#112458=DIRECTION('',(1.6326809185664E-16,-7.15121221728469E-32,-1.));
#112459=DIRECTION('center_axis',(0.,0.,1.));
#112460=DIRECTION('ref_axis',(1.,0.,0.));
#112461=DIRECTION('center_axis',(-1.,0.,0.));
#112462=DIRECTION('ref_axis',(0.,0.,-1.));
#112463=DIRECTION('center_axis',(0.,-1.,0.));
#112464=DIRECTION('ref_axis',(0.,0.,-1.));
#112465=DIRECTION('center_axis',(1.,0.,0.));
#112466=DIRECTION('ref_axis',(0.,0.,-1.));
#112467=DIRECTION('center_axis',(-4.38004274807345E-16,-1.,0.));
#112468=DIRECTION('ref_axis',(-1.,4.38004274807345E-16,0.));
#112469=DIRECTION('',(-1.,4.38004274807345E-16,0.));
#112470=DIRECTION('center_axis',(-1.,0.,0.));
#112471=DIRECTION('ref_axis',(0.,0.,1.));
#112472=DIRECTION('center_axis',(0.,1.,0.));
#112473=DIRECTION('ref_axis',(0.,0.,1.));
#112474=DIRECTION('center_axis',(1.,0.,0.));
#112475=DIRECTION('ref_axis',(0.,0.,1.));
#112476=DIRECTION('center_axis',(0.,0.,-1.));
#112477=DIRECTION('ref_axis',(-1.,0.,0.));
#112478=DIRECTION('',(0.,0.,1.));
#112479=DIRECTION('center_axis',(0.,0.,1.));
#112480=DIRECTION('ref_axis',(-1.,0.,0.));
#112481=DIRECTION('',(0.,0.,-1.));
#112482=DIRECTION('center_axis',(0.,1.,0.));
#112483=DIRECTION('ref_axis',(1.,0.,0.));
#112484=DIRECTION('',(-1.,0.,0.));
#112485=DIRECTION('',(-1.87032180698308E-16,0.,1.));
#112486=DIRECTION('center_axis',(0.,0.,1.));
#112487=DIRECTION('ref_axis',(1.,0.,0.));
#112488=DIRECTION('center_axis',(0.,0.,1.));
#112489=DIRECTION('ref_axis',(-1.,0.,0.));
#112490=DIRECTION('',(1.87032180698308E-16,0.,-1.));
#112491=DIRECTION('center_axis',(-1.,0.,0.));
#112492=DIRECTION('ref_axis',(0.,0.,-1.));
#112493=DIRECTION('center_axis',(0.,-1.,0.));
#112494=DIRECTION('ref_axis',(0.,0.,-1.));
#112495=DIRECTION('center_axis',(1.,0.,0.));
#112496=DIRECTION('ref_axis',(0.,0.,-1.));
#112497=DIRECTION('center_axis',(-4.38004274807345E-16,-1.,0.));
#112498=DIRECTION('ref_axis',(-1.,4.38004274807345E-16,0.));
#112499=DIRECTION('',(-1.,4.38004274807345E-16,0.));
#112500=DIRECTION('center_axis',(-1.,0.,0.));
#112501=DIRECTION('ref_axis',(0.,0.,1.));
#112502=DIRECTION('center_axis',(0.,1.,0.));
#112503=DIRECTION('ref_axis',(0.,0.,1.));
#112504=DIRECTION('center_axis',(1.,0.,0.));
#112505=DIRECTION('ref_axis',(0.,0.,1.));
#112506=DIRECTION('center_axis',(0.,0.,-1.));
#112507=DIRECTION('ref_axis',(-1.,0.,0.));
#112508=DIRECTION('',(0.,0.,1.));
#112509=DIRECTION('center_axis',(0.,0.,1.));
#112510=DIRECTION('ref_axis',(-1.,0.,0.));
#112511=DIRECTION('',(0.,0.,-1.));
#112512=DIRECTION('center_axis',(0.,1.,0.));
#112513=DIRECTION('ref_axis',(1.,0.,0.));
#112514=DIRECTION('',(-1.,0.,0.));
#112515=DIRECTION('',(-1.87032180698308E-16,0.,1.));
#112516=DIRECTION('center_axis',(0.,0.,1.));
#112517=DIRECTION('ref_axis',(1.,0.,0.));
#112518=DIRECTION('center_axis',(0.,0.,1.));
#112519=DIRECTION('ref_axis',(-1.,0.,0.));
#112520=DIRECTION('',(1.87032180698308E-16,0.,-1.));
#112521=DIRECTION('center_axis',(-1.,0.,0.));
#112522=DIRECTION('ref_axis',(0.,0.,-1.));
#112523=DIRECTION('center_axis',(0.,-1.,0.));
#112524=DIRECTION('ref_axis',(0.,0.,-1.));
#112525=DIRECTION('center_axis',(1.,0.,0.));
#112526=DIRECTION('ref_axis',(0.,0.,-1.));
#112527=DIRECTION('center_axis',(-4.38004274807345E-16,-1.,0.));
#112528=DIRECTION('ref_axis',(-1.,4.38004274807345E-16,0.));
#112529=DIRECTION('center_axis',(-6.15557891118788E-9,-1.,7.989575083689E-9));
#112530=DIRECTION('ref_axis',(0.717962811290552,1.14191836403356E-9,0.696081461902102));
#112531=DIRECTION('',(-1.,4.38004274807345E-16,0.));
#112532=DIRECTION('center_axis',(1.79937481368581E-15,0.983475799774124,
-0.181039640020212));
#112533=DIRECTION('ref_axis',(-3.24346588047852E-31,0.181039640020212,0.983475799774124));
#112534=DIRECTION('center_axis',(0.,1.,0.));
#112535=DIRECTION('ref_axis',(0.,0.,1.));
#112536=DIRECTION('center_axis',(1.,0.,0.));
#112537=DIRECTION('ref_axis',(0.,0.000252653767738075,-0.999999968083036));
#112538=DIRECTION('center_axis',(-0.988033841711791,0.154018907555706,0.00820388612708266));
#112539=DIRECTION('ref_axis',(-0.0369034044335798,-0.184421063066604,-0.982154270081129));
#112540=DIRECTION('center_axis',(0.,0.,-1.));
#112541=DIRECTION('ref_axis',(-1.,0.,0.));
#112542=DIRECTION('',(0.,0.,1.));
#112543=DIRECTION('center_axis',(0.,0.,1.));
#112544=DIRECTION('ref_axis',(-1.,0.,0.));
#112545=DIRECTION('',(0.,0.,-1.));
#112546=DIRECTION('center_axis',(0.,0.,-1.));
#112547=DIRECTION('ref_axis',(-1.,0.,0.));
#112548=DIRECTION('center_axis',(0.,1.,0.));
#112549=DIRECTION('ref_axis',(1.,0.,0.));
#112550=DIRECTION('',(-1.,0.,0.));
#112551=DIRECTION('',(-1.87032180698308E-16,0.,1.));
#112552=DIRECTION('center_axis',(3.552570199055E-14,-1.,-2.23044154114413E-16));
#112553=DIRECTION('ref_axis',(-0.00256148703537234,1.37530068325002E-16,
-0.999996719386703));
#112554=DIRECTION('center_axis',(0.,0.,1.));
#112555=DIRECTION('ref_axis',(1.,0.,0.));
#112556=DIRECTION('center_axis',(0.,0.,1.));
#112557=DIRECTION('ref_axis',(-1.,0.,0.));
#112558=DIRECTION('',(1.87032180698308E-16,0.,-1.));
#112559=DIRECTION('center_axis',(0.,0.,-1.));
#112560=DIRECTION('ref_axis',(-1.,0.,0.));
#112561=DIRECTION('center_axis',(0.,-1.,0.));
#112562=DIRECTION('ref_axis',(0.,0.,-1.));
#112563=DIRECTION('center_axis',(0.991674892658728,-0.128766868407894,-2.95080255278421E-5));
#112564=DIRECTION('ref_axis',(-0.0290207967337628,-0.223275175385041,-0.974323349516841));
#112565=DIRECTION('center_axis',(-0.998076185175213,0.0619994224918331,
1.40275800867403E-5));
#112566=DIRECTION('ref_axis',(0.0133447743819902,0.214605257625009,0.976609697062443));
#112567=DIRECTION('center_axis',(0.,1.,0.));
#112568=DIRECTION('ref_axis',(0.,0.,1.));
#112569=DIRECTION('center_axis',(0.,0.,-1.));
#112570=DIRECTION('ref_axis',(-1.,0.,0.));
#112571=DIRECTION('',(0.,0.,1.));
#112572=DIRECTION('center_axis',(0.,0.,1.));
#112573=DIRECTION('ref_axis',(-1.,0.,0.));
#112574=DIRECTION('',(0.,0.,-1.));
#112575=DIRECTION('center_axis',(0.,0.,-1.));
#112576=DIRECTION('ref_axis',(-1.,0.,0.));
#112577=DIRECTION('center_axis',(0.,1.,0.));
#112578=DIRECTION('ref_axis',(1.,0.,0.));
#112579=DIRECTION('',(-1.,0.,0.));
#112580=DIRECTION('',(-1.87032180698308E-16,0.,1.));
#112581=DIRECTION('center_axis',(0.,0.,1.));
#112582=DIRECTION('ref_axis',(1.,0.,0.));
#112583=DIRECTION('center_axis',(0.,0.,1.));
#112584=DIRECTION('ref_axis',(-1.,0.,0.));
#112585=DIRECTION('',(1.87032180698308E-16,0.,-1.));
#112586=DIRECTION('center_axis',(0.,0.,-1.));
#112587=DIRECTION('ref_axis',(-1.,0.,0.));
#112588=DIRECTION('center_axis',(-0.716305556970081,0.650473286312467,0.252568511195758));
#112589=DIRECTION('ref_axis',(-0.672268907563029,-0.740307041655023,-6.62280424422414E-17));
#112590=DIRECTION('center_axis',(-0.488849591387095,0.481564692142823,0.727407399111432));
#112591=DIRECTION('ref_axis',(0.82998476161361,2.33877977530395E-17,0.557786066058662));
#112592=DIRECTION('center_axis',(0.,1.,0.));
#112593=DIRECTION('ref_axis',(0.,0.,1.));
#112594=DIRECTION('center_axis',(0.,-1.,0.));
#112595=DIRECTION('ref_axis',(0.,0.,-1.));
#112596=DIRECTION('center_axis',(0.,1.,0.));
#112597=DIRECTION('ref_axis',(0.,0.,1.));
#112598=DIRECTION('',(4.38004274807345E-16,1.,0.));
#112599=DIRECTION('',(0.,-1.,0.));
#112600=DIRECTION('center_axis',(-4.38004274807345E-16,-1.,0.));
#112601=DIRECTION('ref_axis',(1.,0.,0.));
#112602=DIRECTION('center_axis',(-0.366954554655378,9.16653140031321E-14,
0.930238869762855));
#112603=DIRECTION('ref_axis',(0.930238869762855,-2.79622788237931E-29,0.366954554655378));
#112604=DIRECTION('center_axis',(0.,-1.,0.));
#112605=DIRECTION('ref_axis',(1.,0.,0.));
#112606=DIRECTION('center_axis',(9.37295054023422E-45,1.,-2.02617679489732E-30));
#112607=DIRECTION('ref_axis',(1.,-4.97841222228891E-60,4.62592926927148E-15));
#112608=DIRECTION('center_axis',(-1.,0.,0.));
#112609=DIRECTION('ref_axis',(0.,0.,1.));
#112610=DIRECTION('center_axis',(0.,1.,0.));
#112611=DIRECTION('ref_axis',(1.,0.,0.));
#112612=DIRECTION('',(-1.,0.,0.));
#112613=DIRECTION('',(-1.87032180698308E-16,0.,1.));
#112614=DIRECTION('center_axis',(0.,0.,1.));
#112615=DIRECTION('ref_axis',(1.,0.,0.));
#112616=DIRECTION('center_axis',(0.,0.,1.));
#112617=DIRECTION('ref_axis',(-1.,0.,0.));
#112618=DIRECTION('',(1.87032180698308E-16,0.,-1.));
#112619=DIRECTION('center_axis',(-1.,5.01606788234257E-16,0.));
#112620=DIRECTION('ref_axis',(0.,-1.,0.));
#112621=DIRECTION('center_axis',(1.,0.,0.));
#112622=DIRECTION('ref_axis',(0.,-1.,0.));
#112623=DIRECTION('center_axis',(0.,1.,0.));
#112624=DIRECTION('ref_axis',(0.,0.,1.));
#112625=DIRECTION('center_axis',(-1.,0.,0.));
#112626=DIRECTION('ref_axis',(0.,-1.,0.));
#112627=DIRECTION('center_axis',(1.,-5.01606788234257E-16,0.));
#112628=DIRECTION('ref_axis',(5.01606788234257E-16,1.,0.));
#112629=DIRECTION('',(1.,-5.01606788234257E-16,0.));
#112630=DIRECTION('center_axis',(1.,-4.38004274807346E-16,-5.40794518211031E-32));
#112631=DIRECTION('ref_axis',(4.38004274807346E-16,1.,5.80597460094347E-63));
#112632=DIRECTION('',(-1.,4.38004274807345E-16,5.40794518211031E-32));
#112633=DIRECTION('center_axis',(-1.,0.,0.));
#112634=DIRECTION('ref_axis',(0.,0.,1.));
#112635=DIRECTION('',(1.,-4.38004274807345E-16,-5.40794518211031E-32));
#112636=DIRECTION('center_axis',(0.,0.,-1.));
#112637=DIRECTION('ref_axis',(0.,1.,0.));
#112638=DIRECTION('center_axis',(0.,0.,-1.));
#112639=DIRECTION('ref_axis',(0.,1.,0.));
#112640=DIRECTION('',(0.,0.,-1.));
#112641=DIRECTION('center_axis',(0.,0.,-1.));
#112642=DIRECTION('ref_axis',(0.,1.,0.));
#112643=DIRECTION('center_axis',(0.,0.,-1.));
#112644=DIRECTION('ref_axis',(0.,1.,0.));
#112645=DIRECTION('center_axis',(0.,1.23467863058847E-16,-1.));
#112646=DIRECTION('ref_axis',(-1.,0.,0.));
#112647=DIRECTION('center_axis',(0.,0.,-1.));
#112648=DIRECTION('ref_axis',(0.,1.,0.));
#112649=DIRECTION('center_axis',(0.,0.,-1.));
#112650=DIRECTION('ref_axis',(0.,1.,0.));
#112651=DIRECTION('center_axis',(0.,0.,1.));
#112652=DIRECTION('ref_axis',(-1.,0.,0.));
#112653=DIRECTION('',(0.,0.,-1.));
#112654=DIRECTION('center_axis',(0.,1.,1.23467863058847E-16));
#112655=DIRECTION('ref_axis',(-1.,0.,0.));
#112656=DIRECTION('center_axis',(0.,-1.,-2.77555756156289E-14));
#112657=DIRECTION('ref_axis',(0.,2.77555756156289E-14,-1.));
#112658=DIRECTION('',(-4.38004274807345E-16,-1.,-1.23467863058847E-16));
#112659=DIRECTION('',(4.38004274807345E-16,1.,1.23467863058847E-16));
#112660=DIRECTION('center_axis',(0.,1.,1.23467863058847E-16));
#112661=DIRECTION('ref_axis',(-1.,0.,0.));
#112662=DIRECTION('center_axis',(0.,-1.,0.));
#112663=DIRECTION('ref_axis',(0.,0.,-1.));
#112664=DIRECTION('',(-4.38004274807345E-16,-1.,-1.23467863058847E-16));
#112665=DIRECTION('center_axis',(0.,-1.,0.));
#112666=DIRECTION('ref_axis',(0.,0.,-1.));
#112667=DIRECTION('',(4.38004274807345E-16,1.,1.23467863058847E-16));
#112668=DIRECTION('center_axis',(0.740307041655026,-0.672268907563025,0.));
#112669=DIRECTION('ref_axis',(0.672268907563025,0.740307041655026,0.));
#112670=DIRECTION('center_axis',(0.,0.,-1.));
#112671=DIRECTION('ref_axis',(0.,1.,0.));
#112672=DIRECTION('center_axis',(0.,1.23467863058847E-16,-1.));
#112673=DIRECTION('ref_axis',(0.,1.,1.19418947186571E-16));
#112674=DIRECTION('center_axis',(0.71239495798367,-0.701778757044872,0.));
#112675=DIRECTION('ref_axis',(0.701778757044872,0.71239495798367,0.));
#112676=DIRECTION('center_axis',(1.76945321870477E-31,-1.17608371252665E-16,
1.));
#112677=DIRECTION('ref_axis',(3.01980662698042E-14,1.,1.17608371252665E-16));
#112678=DIRECTION('center_axis',(1.,0.,0.));
#112679=DIRECTION('ref_axis',(0.,0.,-1.));
#112680=DIRECTION('center_axis',(0.,0.,-1.));
#112681=DIRECTION('ref_axis',(0.,1.,0.));
#112682=DIRECTION('center_axis',(-1.,4.38004274807346E-16,5.40794518211031E-32));
#112683=DIRECTION('ref_axis',(-4.38004274807346E-16,-1.,-5.80597460094347E-63));
#112684=DIRECTION('',(1.,-4.38004274807345E-16,-5.40794518211031E-32));
#112685=DIRECTION('',(-1.,4.38004274807345E-16,5.40794518211031E-32));
#112686=DIRECTION('center_axis',(0.,0.,-1.));
#112687=DIRECTION('ref_axis',(0.,1.,0.));
#112688=DIRECTION('center_axis',(0.,0.,-1.));
#112689=DIRECTION('ref_axis',(0.,1.,0.));
#112690=DIRECTION('',(0.,0.,-1.));
#112691=DIRECTION('center_axis',(0.,0.,-1.));
#112692=DIRECTION('ref_axis',(0.,1.,0.));
#112693=DIRECTION('center_axis',(0.,1.23467863058847E-16,-1.));
#112694=DIRECTION('ref_axis',(-1.,0.,0.));
#112695=DIRECTION('center_axis',(0.,0.,-1.));
#112696=DIRECTION('ref_axis',(0.,1.,0.));
#112697=DIRECTION('center_axis',(0.,0.,-1.));
#112698=DIRECTION('ref_axis',(0.,1.,0.));
#112699=DIRECTION('center_axis',(0.,0.,1.));
#112700=DIRECTION('ref_axis',(-1.,0.,0.));
#112701=DIRECTION('',(0.,0.,-1.));
#112702=DIRECTION('center_axis',(-1.,4.38004274807346E-16,5.40794518211031E-32));
#112703=DIRECTION('ref_axis',(-4.38004274807346E-16,-1.,-5.80597460094347E-63));
#112704=DIRECTION('',(-1.,4.38004274807345E-16,5.40794518211031E-32));
#112705=DIRECTION('center_axis',(-1.,0.,0.));
#112706=DIRECTION('ref_axis',(0.,0.,1.));
#112707=DIRECTION('',(1.,-4.38004274807345E-16,-5.40794518211031E-32));
#112708=DIRECTION('center_axis',(0.,1.23467863058847E-16,-1.));
#112709=DIRECTION('ref_axis',(-1.,0.,0.));
#112710=DIRECTION('',(-0.0871557427476402,-0.996194698091747,-1.22998030563942E-16));
#112711=DIRECTION('center_axis',(0.,-1.17559414210783E-16,1.));
#112712=DIRECTION('ref_axis',(0.,1.,1.17559414210783E-16));
#112713=DIRECTION('center_axis',(-4.18005656861882E-16,-1.,0.));
#112714=DIRECTION('ref_axis',(-1.,4.18005656861882E-16,0.));
#112715=DIRECTION('',(1.08020383274181E-17,-4.51531312649963E-33,1.));
#112716=DIRECTION('',(1.,-4.18005656861881E-16,0.));
#112717=DIRECTION('center_axis',(0.,0.,-1.));
#112718=DIRECTION('ref_axis',(-1.,0.,0.));
#112719=DIRECTION('center_axis',(0.,0.,-1.));
#112720=DIRECTION('ref_axis',(-1.,0.,0.));
#112721=DIRECTION('center_axis',(1.,0.,0.));
#112722=DIRECTION('ref_axis',(0.,1.,0.));
#112723=DIRECTION('',(-1.,4.18005656861881E-16,0.));
#112724=DIRECTION('center_axis',(0.,0.,-1.));
#112725=DIRECTION('ref_axis',(0.,-1.,0.));
#112726=DIRECTION('',(-0.0871557427476402,-0.996194698091747,0.));
#112727=DIRECTION('',(1.,-4.18005656861881E-16,0.));
#112728=DIRECTION('center_axis',(1.,0.,0.));
#112729=DIRECTION('ref_axis',(0.,1.,0.));
#112730=DIRECTION('',(-1.,4.18005656861881E-16,0.));
#112731=DIRECTION('center_axis',(4.18005656861882E-16,1.,0.));
#112732=DIRECTION('ref_axis',(1.,-4.18005656861882E-16,0.));
#112733=DIRECTION('',(-1.08020383274181E-17,4.51531312649963E-33,-1.));
#112734=DIRECTION('center_axis',(0.,0.,-1.));
#112735=DIRECTION('ref_axis',(-1.,0.,0.));
#112736=DIRECTION('center_axis',(0.,1.23467863058847E-16,-1.));
#112737=DIRECTION('ref_axis',(-1.,0.,0.));
#112738=DIRECTION('',(-0.0871557427476402,-0.996194698091747,-1.22998030563942E-16));
#112739=DIRECTION('center_axis',(0.,0.,1.));
#112740=DIRECTION('ref_axis',(1.,0.,0.));
#112741=DIRECTION('center_axis',(-4.18005656861882E-16,-1.,0.));
#112742=DIRECTION('ref_axis',(-1.,4.18005656861882E-16,0.));
#112743=DIRECTION('',(1.08020383274181E-17,-4.51531312649963E-33,1.));
#112744=DIRECTION('',(1.,-4.18005656861881E-16,0.));
#112745=DIRECTION('center_axis',(1.,0.,0.));
#112746=DIRECTION('ref_axis',(0.,1.,0.));
#112747=DIRECTION('',(-1.,4.18005656861881E-16,0.));
#112748=DIRECTION('center_axis',(0.,0.,-1.));
#112749=DIRECTION('ref_axis',(0.,-1.,0.));
#112750=DIRECTION('',(-0.0871557427476402,-0.996194698091747,0.));
#112751=DIRECTION('',(1.,-4.38004274807345E-16,0.));
#112752=DIRECTION('center_axis',(-1.,0.,0.));
#112753=DIRECTION('ref_axis',(0.,-1.,0.));
#112754=DIRECTION('',(-1.,4.38004274807345E-16,0.));
#112755=DIRECTION('center_axis',(4.38004274807345E-16,1.,0.));
#112756=DIRECTION('ref_axis',(1.,-4.38004274807345E-16,0.));
#112757=DIRECTION('',(-1.08020383274181E-17,4.73133896404192E-33,-1.));
#112758=DIRECTION('center_axis',(0.,0.,-1.));
#112759=DIRECTION('ref_axis',(-1.,0.,0.));
#112760=DIRECTION('center_axis',(4.18005656861882E-16,1.,0.));
#112761=DIRECTION('ref_axis',(1.,-4.18005656861882E-16,0.));
#112762=DIRECTION('',(-1.,4.18005656861881E-16,0.));
#112763=DIRECTION('',(-1.08020383274181E-17,4.51531312649963E-33,-1.));
#112764=DIRECTION('center_axis',(1.38777878078144E-14,0.,1.));
#112765=DIRECTION('ref_axis',(1.,0.,-1.38777878078144E-14));
#112766=DIRECTION('center_axis',(0.,1.23467863058847E-16,-1.));
#112767=DIRECTION('ref_axis',(0.,1.,1.1837531408762E-16));
#112768=DIRECTION('center_axis',(-4.18005656861882E-16,-1.,0.));
#112769=DIRECTION('ref_axis',(-1.,4.18005656861882E-16,0.));
#112770=DIRECTION('',(-1.08020383274202E-17,4.51531312650048E-33,1.));
#112771=DIRECTION('',(1.,-4.18005656861881E-16,0.));
#112772=DIRECTION('center_axis',(1.,0.,0.));
#112773=DIRECTION('ref_axis',(0.,1.,0.));
#112774=DIRECTION('',(-1.,4.18005656861881E-16,0.));
#112775=DIRECTION('center_axis',(0.,0.,-1.));
#112776=DIRECTION('ref_axis',(0.,-1.,0.));
#112777=DIRECTION('',(0.0871557427476566,-0.996194698091746,0.));
#112778=DIRECTION('',(1.,-4.18005656861881E-16,0.));
#112779=DIRECTION('center_axis',(1.,0.,0.));
#112780=DIRECTION('ref_axis',(0.,1.,0.));
#112781=DIRECTION('',(-1.,4.18005656861881E-16,0.));
#112782=DIRECTION('center_axis',(4.18005656861882E-16,1.,0.));
#112783=DIRECTION('ref_axis',(1.,-4.18005656861882E-16,0.));
#112784=DIRECTION('',(1.08020383274202E-17,-4.51531312650048E-33,-1.));
#112785=DIRECTION('center_axis',(0.,0.,-1.));
#112786=DIRECTION('ref_axis',(-1.,0.,0.));
#112787=DIRECTION('center_axis',(0.,1.23467863058847E-16,-1.));
#112788=DIRECTION('ref_axis',(-1.,0.,0.));
#112789=DIRECTION('center_axis',(-3.98829513817191E-31,-1.17559414210783E-16,
1.));
#112790=DIRECTION('ref_axis',(-6.75015598972095E-14,1.,1.17559414210783E-16));
#112791=DIRECTION('',(0.0871557427476566,-0.996194698091746,-1.22998030563941E-16));
#112792=DIRECTION('center_axis',(0.,1.23467863058847E-16,-1.));
#112793=DIRECTION('ref_axis',(0.,1.,1.1837531408762E-16));
#112794=DIRECTION('center_axis',(0.0835592633859915,-0.955086750882199,
-0.284301156859544));
#112795=DIRECTION('ref_axis',(2.48475885091778E-18,0.285298901444289,-0.958438593147564));
#112796=DIRECTION('center_axis',(0.,0.,1.));
#112797=DIRECTION('ref_axis',(1.,0.,0.));
#112798=DIRECTION('center_axis',(0.,-1.,0.));
#112799=DIRECTION('ref_axis',(0.964920734333665,0.,-0.26254138045836));
#112800=DIRECTION('center_axis',(-4.18005656861882E-16,-1.,0.));
#112801=DIRECTION('ref_axis',(-1.,4.18005656861882E-16,0.));
#112802=DIRECTION('',(-1.08020383274202E-17,4.51531312650048E-33,1.));
#112803=DIRECTION('',(1.,-4.18005656861881E-16,0.));
#112804=DIRECTION('center_axis',(-4.38004274807345E-16,-1.,0.));
#112805=DIRECTION('ref_axis',(-1.,4.38004274807345E-16,0.));
#112806=DIRECTION('',(-1.08020383274202E-17,4.73133896404282E-33,1.));
#112807=DIRECTION('',(1.,-4.38004274807345E-16,0.));
#112808=DIRECTION('center_axis',(0.,0.,-1.));
#112809=DIRECTION('ref_axis',(-1.,0.,0.));
#112810=DIRECTION('center_axis',(-1.,0.,0.));
#112811=DIRECTION('ref_axis',(0.,-1.,0.));
#112812=DIRECTION('',(-1.,4.38004274807345E-16,0.));
#112813=DIRECTION('center_axis',(0.,0.,-1.));
#112814=DIRECTION('ref_axis',(0.,-1.,0.));
#112815=DIRECTION('',(0.0871557427476566,-0.996194698091746,0.));
#112816=DIRECTION('',(1.,-4.18005656861881E-16,0.));
#112817=DIRECTION('center_axis',(1.,0.,0.));
#112818=DIRECTION('ref_axis',(0.,1.,0.));
#112819=DIRECTION('',(-1.,4.18005656861881E-16,0.));
#112820=DIRECTION('center_axis',(4.18005656861882E-16,1.,0.));
#112821=DIRECTION('ref_axis',(1.,-4.18005656861882E-16,0.));
#112822=DIRECTION('',(1.08020383274202E-17,-4.51531312650048E-33,-1.));
#112823=DIRECTION('center_axis',(0.,0.,-1.));
#112824=DIRECTION('ref_axis',(-1.,0.,0.));
#112825=DIRECTION('center_axis',(0.,0.,1.));
#112826=DIRECTION('ref_axis',(1.,0.,0.));
#112827=DIRECTION('center_axis',(0.,1.23467863058847E-16,-1.));
#112828=DIRECTION('ref_axis',(-1.,0.,0.));
#112829=DIRECTION('',(0.0871557427476566,-0.996194698091746,-1.22998030563941E-16));
#112830=DIRECTION('center_axis',(1.,0.,1.87032180698308E-16));
#112831=DIRECTION('ref_axis',(-1.87032180698308E-16,0.,1.));
#112832=DIRECTION('',(0.,-1.,0.));
#112833=DIRECTION('',(-1.87032180698308E-16,-1.07104667533214E-16,1.));
#112834=DIRECTION('',(0.,1.,0.));
#112835=DIRECTION('center_axis',(0.,-1.,0.));
#112836=DIRECTION('ref_axis',(0.,0.,-1.));
#112837=DIRECTION('',(0.,-1.,0.));
#112838=DIRECTION('center_axis',(0.,0.,1.));
#112839=DIRECTION('ref_axis',(1.,0.,0.));
#112840=DIRECTION('',(0.996194698091746,-0.0871557427476568,0.));
#112841=DIRECTION('',(4.38004274807345E-16,1.,0.));
#112842=DIRECTION('center_axis',(4.38004274807346E-16,1.,0.));
#112843=DIRECTION('ref_axis',(-1.,4.38004274807346E-16,0.));
#112844=DIRECTION('',(-4.38004274807345E-16,-1.,0.));
#112845=DIRECTION('center_axis',(1.,-4.38004274807345E-16,0.));
#112846=DIRECTION('ref_axis',(-4.38004274807345E-16,-1.,0.));
#112847=DIRECTION('',(5.40794518211031E-32,1.23467863058847E-16,-1.));
#112848=DIRECTION('center_axis',(0.,0.,-1.));
#112849=DIRECTION('ref_axis',(-1.,0.,0.));
#112850=DIRECTION('center_axis',(0.,0.,1.));
#112851=DIRECTION('ref_axis',(1.,0.,0.));
#112852=DIRECTION('center_axis',(1.,0.,1.87032180698308E-16));
#112853=DIRECTION('ref_axis',(-1.87032180698308E-16,0.,1.));
#112854=DIRECTION('',(-1.87032180698308E-16,-1.07104667533214E-16,1.));
#112855=DIRECTION('',(0.,1.,0.));
#112856=DIRECTION('',(0.,-1.,0.));
#112857=DIRECTION('center_axis',(0.,-1.,0.));
#112858=DIRECTION('ref_axis',(0.,0.,-1.));
#112859=DIRECTION('',(0.,-1.,0.));
#112860=DIRECTION('center_axis',(0.,0.,1.));
#112861=DIRECTION('ref_axis',(1.,0.,0.));
#112862=DIRECTION('',(0.996194698091746,-0.0871557427476568,0.));
#112863=DIRECTION('',(0.,1.,0.));
#112864=DIRECTION('center_axis',(0.,-1.,0.));
#112865=DIRECTION('ref_axis',(0.,0.,-1.));
#112866=DIRECTION('',(0.,-1.,0.));
#112867=DIRECTION('center_axis',(-1.,0.,0.));
#112868=DIRECTION('ref_axis',(0.,0.,1.));
#112869=DIRECTION('',(0.,1.23467863058847E-16,-1.));
#112870=DIRECTION('',(0.,1.,0.));
#112871=DIRECTION('center_axis',(0.,0.,1.));
#112872=DIRECTION('ref_axis',(1.,0.,0.));
#112873=DIRECTION('center_axis',(0.,0.,1.));
#112874=DIRECTION('ref_axis',(1.,0.,0.));
#112875=DIRECTION('center_axis',(0.,1.23467863058847E-16,-1.));
#112876=DIRECTION('ref_axis',(-1.,0.,0.));
#112877=DIRECTION('',(0.996194698091746,-0.0871557427476568,-1.07609333103598E-17));
#112878=DIRECTION('center_axis',(-1.,5.01606788234257E-16,0.));
#112879=DIRECTION('ref_axis',(0.,0.,1.));
#112880=DIRECTION('',(-6.19323182390956E-32,-1.23467863058847E-16,1.));
#112881=DIRECTION('',(-5.01606788234257E-16,-1.,0.));
#112882=DIRECTION('center_axis',(0.,-1.,0.));
#112883=DIRECTION('ref_axis',(1.,0.,0.));
#112884=DIRECTION('',(5.01606788234257E-16,1.,0.));
#112885=DIRECTION('center_axis',(0.,0.,-1.));
#112886=DIRECTION('ref_axis',(0.,-1.,0.));
#112887=DIRECTION('',(-0.996194698091747,-0.0871557427476402,0.));
#112888=DIRECTION('',(-5.01606788234257E-16,-1.,0.));
#112889=DIRECTION('center_axis',(0.,-1.,0.));
#112890=DIRECTION('ref_axis',(1.,0.,0.));
#112891=DIRECTION('',(5.01606788234257E-16,1.,0.));
#112892=DIRECTION('center_axis',(1.,-5.01606788234257E-16,0.));
#112893=DIRECTION('ref_axis',(-5.01606788234257E-16,-1.,0.));
#112894=DIRECTION('',(6.19323182390956E-32,1.23467863058847E-16,-1.));
#112895=DIRECTION('center_axis',(0.,0.,-1.));
#112896=DIRECTION('ref_axis',(-1.,0.,0.));
#112897=DIRECTION('center_axis',(0.,1.23467863058847E-16,-1.));
#112898=DIRECTION('ref_axis',(-1.,0.,0.));
#112899=DIRECTION('center_axis',(0.,-1.17559414210783E-16,1.));
#112900=DIRECTION('ref_axis',(0.,1.,1.17559414210783E-16));
#112901=DIRECTION('',(-0.996194698091747,-0.0871557427476402,-1.07609333103578E-17));
#112902=DIRECTION('center_axis',(0.,1.23467863058847E-16,-1.));
#112903=DIRECTION('ref_axis',(0.,1.,1.1837531408762E-16));
#112904=DIRECTION('center_axis',(-1.,5.01606788234257E-16,0.));
#112905=DIRECTION('ref_axis',(0.,0.,1.));
#112906=DIRECTION('',(-6.19323182390956E-32,-1.23467863058847E-16,1.));
#112907=DIRECTION('',(-5.01606788234257E-16,-1.,0.));
#112908=DIRECTION('center_axis',(0.,0.,-1.));
#112909=DIRECTION('ref_axis',(-1.,0.,0.));
#112910=DIRECTION('center_axis',(0.,0.,1.));
#112911=DIRECTION('ref_axis',(1.,0.,0.));
#112912=DIRECTION('center_axis',(-1.,4.38004274807345E-16,1.13659195805196E-16));
#112913=DIRECTION('ref_axis',(1.13659195805196E-16,0.,1.));
#112914=DIRECTION('',(1.13659195805196E-16,-1.13523971920422E-16,1.));
#112915=DIRECTION('',(-4.38004274807345E-16,-1.,0.));
#112916=DIRECTION('center_axis',(0.,1.,0.));
#112917=DIRECTION('ref_axis',(-1.,0.,0.));
#112918=DIRECTION('',(4.38004274807345E-16,1.,0.));
#112919=DIRECTION('center_axis',(0.,0.,-1.));
#112920=DIRECTION('ref_axis',(0.,-1.,0.));
#112921=DIRECTION('',(-0.996194698091747,-0.0871557427476402,0.));
#112922=DIRECTION('',(-5.01606788234257E-16,-1.,0.));
#112923=DIRECTION('center_axis',(0.,-1.,0.));
#112924=DIRECTION('ref_axis',(1.,0.,0.));
#112925=DIRECTION('',(5.01606788234257E-16,1.,0.));
#112926=DIRECTION('center_axis',(1.,-5.01606788234257E-16,1.13659195805196E-16));
#112927=DIRECTION('ref_axis',(-5.01606788234257E-16,-1.,-5.42661491374937E-48));
#112928=DIRECTION('',(1.13659195805196E-16,1.33411754197273E-16,-1.));
#112929=DIRECTION('center_axis',(0.,0.,-1.));
#112930=DIRECTION('ref_axis',(-1.,0.,0.));
#112931=DIRECTION('center_axis',(0.,0.,-1.));
#112932=DIRECTION('ref_axis',(-1.,0.,0.));
#112933=DIRECTION('center_axis',(0.,1.23467863058847E-16,-1.));
#112934=DIRECTION('ref_axis',(-1.,0.,0.));
#112935=DIRECTION('',(-0.996194698091747,-0.0871557427476402,-1.07609333103578E-17));
#112936=DIRECTION('center_axis',(4.18005656861882E-16,1.,0.));
#112937=DIRECTION('ref_axis',(1.,-4.18005656861882E-16,0.));
#112938=DIRECTION('',(-1.,4.18005656861881E-16,0.));
#112939=DIRECTION('',(-5.16102651992463E-32,2.15733828054269E-47,-1.));
#112940=DIRECTION('center_axis',(2.32688276946506E-8,1.,-5.60873972379676E-9));
#112941=DIRECTION('ref_axis',(0.999404101594694,-2.30613634711969E-8,0.0345172669210846));
#112942=DIRECTION('center_axis',(0.,0.,1.));
#112943=DIRECTION('ref_axis',(1.,0.,0.));
#112944=DIRECTION('center_axis',(-0.161942099399832,-0.986800258756125,
7.590006713781E-5));
#112945=DIRECTION('ref_axis',(0.986128889721933,-0.161834757970274,-0.0368690109508116));
#112946=DIRECTION('center_axis',(0.,-1.18842113532926E-16,1.));
#112947=DIRECTION('ref_axis',(0.,1.,1.18842113532926E-16));
#112948=DIRECTION('center_axis',(0.,1.19033121480991E-16,-1.));
#112949=DIRECTION('ref_axis',(0.,-1.,-1.19033121480991E-16));
#112950=DIRECTION('center_axis',(-4.18005656861882E-16,-1.,0.));
#112951=DIRECTION('ref_axis',(-1.,4.18005656861882E-16,0.));
#112952=DIRECTION('center_axis',(1.8411653907608E-7,-0.999999999999982,
-4.27391046394874E-8));
#112953=DIRECTION('ref_axis',(0.944128962271366,1.59743963266783E-7,0.329576247020879));
#112954=DIRECTION('',(5.16102651992463E-32,-2.15733828054269E-47,1.));
#112955=DIRECTION('',(1.,-4.18005656861881E-16,0.));
#112956=DIRECTION('center_axis',(0.131559425275772,0.991308283854165,-6.31127399035659E-5));
#112957=DIRECTION('ref_axis',(0.984955559835192,-0.130723532319353,-0.113021693703886));
#112958=DIRECTION('center_axis',(0.,0.,-1.));
#112959=DIRECTION('ref_axis',(-1.,0.,0.));
#112960=DIRECTION('center_axis',(1.,0.,0.));
#112961=DIRECTION('ref_axis',(0.,1.,0.));
#112962=DIRECTION('',(-1.,4.18005656861881E-16,0.));
#112963=DIRECTION('center_axis',(0.,0.,-1.));
#112964=DIRECTION('ref_axis',(0.,-1.,0.));
#112965=DIRECTION('center_axis',(0.,0.,-1.));
#112966=DIRECTION('ref_axis',(-1.,0.,0.));
#112967=DIRECTION('',(1.,-4.18005656861881E-16,0.));
#112968=DIRECTION('center_axis',(1.,0.,0.));
#112969=DIRECTION('ref_axis',(0.,1.,0.));
#112970=DIRECTION('',(-1.,4.18005656861881E-16,0.));
#112971=DIRECTION('center_axis',(4.18005656861882E-16,1.,0.));
#112972=DIRECTION('ref_axis',(1.,-4.18005656861882E-16,0.));
#112973=DIRECTION('',(-5.16102651992463E-32,2.15733828054269E-47,-1.));
#112974=DIRECTION('center_axis',(2.74436147249812E-7,0.99999999999996,-6.29034153387323E-8));
#112975=DIRECTION('ref_axis',(0.660475707378147,-1.3402754171038E-7,0.750847414567913));
#112976=DIRECTION('center_axis',(0.,0.,1.));
#112977=DIRECTION('ref_axis',(1.,0.,0.));
#112978=DIRECTION('center_axis',(-0.115639749300789,-0.993291218694044,
5.69820218245346E-5));
#112979=DIRECTION('ref_axis',(0.983118122834487,-0.114463578413279,-0.142747489544376));
#112980=DIRECTION('center_axis',(0.,-1.18842113532926E-16,1.));
#112981=DIRECTION('ref_axis',(0.,1.,1.18842113532926E-16));
#112982=DIRECTION('center_axis',(-4.72661011967866E-32,1.19033121480991E-16,
-1.));
#112983=DIRECTION('ref_axis',(-1.06581410364015E-14,-1.,-1.19033121480991E-16));
#112984=DIRECTION('center_axis',(-4.18005656861882E-16,-1.,0.));
#112985=DIRECTION('ref_axis',(-1.,4.18005656861882E-16,0.));
#112986=DIRECTION('center_axis',(4.47342289204968E-7,-0.999999999999895,
-1.00433397542106E-7));
#112987=DIRECTION('ref_axis',(-0.286876404864124,-3.21200065696789E-8,-0.957967602965901));
#112988=DIRECTION('',(5.16102651992463E-32,-2.15733828054269E-47,1.));
#112989=DIRECTION('center_axis',(0.0751032200622623,0.997175764329397,-3.7018408260164E-5));
#112990=DIRECTION('ref_axis',(0.979395211524647,-0.0737710402502458,-0.187996950142784));
#112991=DIRECTION('center_axis',(0.,0.,-1.));
#112992=DIRECTION('ref_axis',(-1.,0.,0.));
#112993=DIRECTION('center_axis',(-0.159867238682005,-0.0103393831144628,
-0.987084374890517));
#112994=DIRECTION('ref_axis',(0.98052069011386,0.11392960656718,-0.159997565625503));
#112995=DIRECTION('center_axis',(4.18005656861882E-16,1.,0.));
#112996=DIRECTION('ref_axis',(1.,-4.18005656861882E-16,0.));
#112997=DIRECTION('',(-5.16102651992463E-32,2.15733828054269E-47,-1.));
#112998=DIRECTION('center_axis',(0.,1.,0.));
#112999=DIRECTION('ref_axis',(0.977685721591009,0.,-0.210072915429545));
#113000=DIRECTION('center_axis',(0.,0.,-1.));
#113001=DIRECTION('ref_axis',(-1.,0.,0.));
#113002=DIRECTION('center_axis',(-0.0555987775761959,-0.998453191267193,
2.79354816923995E-5));
#113003=DIRECTION('ref_axis',(0.977794512058442,-0.054454062847614,-0.20236760419539));
#113004=DIRECTION('center_axis',(0.,-1.18842113532926E-16,1.));
#113005=DIRECTION('ref_axis',(0.,1.,1.18842113532926E-16));
#113006=DIRECTION('center_axis',(0.,1.19033121480991E-16,-1.));
#113007=DIRECTION('ref_axis',(0.,-1.,-1.19033121480991E-16));
#113008=DIRECTION('center_axis',(-4.18005656861882E-16,-1.,0.));
#113009=DIRECTION('ref_axis',(-1.,4.18005656861882E-16,0.));
#113010=DIRECTION('center_axis',(0.,-1.,0.));
#113011=DIRECTION('ref_axis',(0.976470143643405,0.,-0.215652634050752));
#113012=DIRECTION('',(5.16102651992463E-32,-2.15733828054269E-47,1.));
#113013=DIRECTION('center_axis',(0.00945202350686712,0.99995532861701,-4.69828733081355E-6));
#113014=DIRECTION('ref_axis',(0.976474172799545,-0.00923108138389767,-0.215436712265873));
#113015=DIRECTION('center_axis',(0.,0.,-1.));
#113016=DIRECTION('ref_axis',(-1.,0.,0.));
#113017=DIRECTION('center_axis',(-0.0305144215778958,2.78804702901659E-8,
-0.999534326612031));
#113018=DIRECTION('ref_axis',(0.99952008198814,-0.00533875532879332,-0.0305139868578466));
#113019=DIRECTION('center_axis',(4.18005656861882E-16,1.,0.));
#113020=DIRECTION('ref_axis',(1.,-4.18005656861882E-16,0.));
#113021=DIRECTION('',(-5.16102651992463E-32,2.15733828054269E-47,-1.));
#113022=DIRECTION('center_axis',(0.,1.,0.));
#113023=DIRECTION('ref_axis',(0.976222312485803,0.,-0.216771761548571));
#113024=DIRECTION('center_axis',(0.,0.,-1.));
#113025=DIRECTION('ref_axis',(-1.,0.,0.));
#113026=DIRECTION('center_axis',(0.0113199996393415,-0.999935926735075,
-5.71253473801473E-6));
#113027=DIRECTION('ref_axis',(0.976230462447886,0.0110528731720008,-0.216453039210427));
#113028=DIRECTION('center_axis',(0.,-1.18842113532926E-16,1.));
#113029=DIRECTION('ref_axis',(0.,1.,1.18842113532926E-16));
#113030=DIRECTION('center_axis',(-1.96942088319945E-31,1.19033121480991E-16,
-1.));
#113031=DIRECTION('ref_axis',(-4.44089209850063E-14,-1.,-1.19033121480991E-16));
#113032=DIRECTION('center_axis',(-4.18005656861882E-16,-1.,0.));
#113033=DIRECTION('ref_axis',(-1.,4.18005656861882E-16,0.));
#113034=DIRECTION('center_axis',(0.,-1.,0.));
#113035=DIRECTION('ref_axis',(0.978069789124882,0.,-0.208277429408972));
#113036=DIRECTION('',(5.16102651992463E-32,-2.15733828054269E-47,1.));
#113037=DIRECTION('center_axis',(-0.0573828197059871,0.998352248055229,
2.83841706920683E-5));
#113038=DIRECTION('ref_axis',(0.978154360176249,0.0562275849658862,-0.200131222844156));
#113039=DIRECTION('center_axis',(0.,0.,-1.));
#113040=DIRECTION('ref_axis',(-1.,0.,0.));
#113041=DIRECTION('center_axis',(-0.167640680088922,0.0112856983933777,
-0.985783564171719));
#113042=DIRECTION('ref_axis',(0.977940174982197,-0.124494780023978,-0.167732119472009));
#113043=DIRECTION('center_axis',(4.18005656861882E-16,1.,0.));
#113044=DIRECTION('ref_axis',(1.,-4.18005656861882E-16,0.));
#113045=DIRECTION('',(-5.16102651992463E-32,2.15733828054269E-47,-1.));
#113046=DIRECTION('center_axis',(0.,1.,0.));
#113047=DIRECTION('ref_axis',(0.979260396969467,0.,-0.202605712967828));
#113048=DIRECTION('center_axis',(0.,0.,-1.));
#113049=DIRECTION('ref_axis',(-1.,0.,0.));
#113050=DIRECTION('center_axis',(0.0768213995086415,-0.997044869150772,
-3.84402733247989E-5));
#113051=DIRECTION('ref_axis',(0.979293407027384,0.0754609081712752,-0.187856525813356));
#113052=DIRECTION('center_axis',(0.,-1.18842113532926E-16,1.));
#113053=DIRECTION('ref_axis',(0.,1.,1.18842113532926E-16));
#113054=DIRECTION('center_axis',(0.,1.19033121480991E-16,-1.));
#113055=DIRECTION('ref_axis',(0.,-1.,-1.19033121480991E-16));
#113056=DIRECTION('center_axis',(-4.18005656861882E-16,-1.,0.));
#113057=DIRECTION('ref_axis',(-1.,4.18005656861882E-16,0.));
#113058=DIRECTION('center_axis',(2.65375038641309E-7,-0.999999999999963,
-6.08902664370013E-8));
#113059=DIRECTION('ref_axis',(-0.699850500391891,-1.4222958468278E-7,-0.714289351104438));
#113060=DIRECTION('',(5.16102651992463E-32,-2.15733828054269E-47,1.));
#113061=DIRECTION('',(1.,-4.18005656861881E-16,0.));
#113062=DIRECTION('center_axis',(-0.117125163318625,0.993117159703197,5.67506910983411E-5));
#113063=DIRECTION('ref_axis',(0.98346589789016,0.115994870303608,-0.139068392348335));
#113064=DIRECTION('center_axis',(0.,0.,-1.));
#113065=DIRECTION('ref_axis',(-1.,0.,0.));
#113066=DIRECTION('center_axis',(1.,0.,0.));
#113067=DIRECTION('ref_axis',(0.,1.,0.));
#113068=DIRECTION('',(-1.,4.18005656861881E-16,0.));
#113069=DIRECTION('center_axis',(0.,0.,-1.));
#113070=DIRECTION('ref_axis',(0.,-1.,0.));
#113071=DIRECTION('center_axis',(0.,0.,-1.));
#113072=DIRECTION('ref_axis',(-1.,0.,0.));
#113073=DIRECTION('',(1.,-4.18005656861881E-16,0.));
#113074=DIRECTION('center_axis',(1.,0.,0.));
#113075=DIRECTION('ref_axis',(0.,1.,0.));
#113076=DIRECTION('',(-1.,4.18005656861881E-16,0.));
#113077=DIRECTION('center_axis',(4.18005656861882E-16,1.,0.));
#113078=DIRECTION('ref_axis',(1.,-4.18005656861882E-16,0.));
#113079=DIRECTION('',(-5.16102651992463E-32,2.15733828054269E-47,-1.));
#113080=DIRECTION('center_axis',(1.78035294390513E-7,0.999999999999983,
-4.13792835849922E-8));
#113081=DIRECTION('ref_axis',(0.953984227519048,-1.57435003701598E-7,0.299856788558906));
#113082=DIRECTION('center_axis',(0.,0.,1.));
#113083=DIRECTION('ref_axis',(1.,0.,0.));
#113084=DIRECTION('center_axis',(0.132927043042659,-0.991125823009864,-6.47375843459798E-5));
#113085=DIRECTION('ref_axis',(0.984931431928559,0.132103559132877,-0.111618654639735));
#113086=DIRECTION('center_axis',(0.,-1.18842113532926E-16,1.));
#113087=DIRECTION('ref_axis',(0.,1.,1.18842113532926E-16));
#113088=DIRECTION('center_axis',(9.84710441599736E-32,1.19033121480991E-16,
-1.));
#113089=DIRECTION('ref_axis',(2.22044604925031E-14,-1.,-1.19033121480991E-16));
#113090=DIRECTION('center_axis',(0.,0.,1.));
#113091=DIRECTION('ref_axis',(1.,0.,0.));
#113092=DIRECTION('center_axis',(0.,-1.,0.));
#113093=DIRECTION('ref_axis',(0.949353414893388,0.,0.314210269772112));
#113094=DIRECTION('center_axis',(-4.18005656861882E-16,-1.,0.));
#113095=DIRECTION('ref_axis',(-1.,4.18005656861882E-16,0.));
#113096=DIRECTION('',(5.16102651992463E-32,-2.15733828054269E-47,1.));
#113097=DIRECTION('',(1.,-4.18005656861881E-16,0.));
#113098=DIRECTION('center_axis',(1.,0.,0.));
#113099=DIRECTION('ref_axis',(0.,1.,0.));
#113100=DIRECTION('',(-1.,4.18005656861881E-16,0.));
#113101=DIRECTION('center_axis',(0.,0.,-1.));
#113102=DIRECTION('ref_axis',(0.,-1.,0.));
#113103=DIRECTION('center_axis',(0.,0.,1.));
#113104=DIRECTION('ref_axis',(-1.,-1.5419764230905E-14,0.));
#113105=DIRECTION('',(1.,-4.18005656861881E-16,0.));
#113106=DIRECTION('center_axis',(1.,0.,0.));
#113107=DIRECTION('ref_axis',(0.,1.,0.));
#113108=DIRECTION('center_axis',(0.985034259178296,-0.172358661647933,-3.73628995927113E-11));
#113109=DIRECTION('ref_axis',(-0.0884978163252629,-0.505767334680601,-0.858118604667059));
#113110=DIRECTION('center_axis',(1.,0.,0.));
#113111=DIRECTION('ref_axis',(0.,1.,0.));
#113112=DIRECTION('center_axis',(0.985034259164998,0.172358661723926,1.4184662739622E-13));
#113113=DIRECTION('ref_axis',(0.0566474313388088,-0.323741551509226,0.944448239105306));
#113114=DIRECTION('',(-1.,4.18005656861881E-16,0.));
#113115=DIRECTION('center_axis',(0.,0.,-1.));
#113116=DIRECTION('ref_axis',(0.,-1.,0.));
#113117=DIRECTION('center_axis',(0.,0.,1.));
#113118=DIRECTION('ref_axis',(-1.,2.69845874040837E-15,0.));
#113119=DIRECTION('',(1.,-4.18005656861881E-16,0.));
#113120=DIRECTION('center_axis',(1.,0.,0.));
#113121=DIRECTION('ref_axis',(0.,1.,0.));
#113122=DIRECTION('center_axis',(1.,0.,1.87032180698308E-16));
#113123=DIRECTION('ref_axis',(-1.87032180698308E-16,0.,1.));
#113124=DIRECTION('center_axis',(1.,0.,0.));
#113125=DIRECTION('ref_axis',(0.,0.97671957347062,-0.214520103485359));
#113126=DIRECTION('',(-1.87032180698308E-16,-1.23467863058847E-16,1.));
#113127=DIRECTION('',(0.,-1.,0.));
#113128=DIRECTION('center_axis',(-0.00150472629281886,-0.0576832079807129,
-0.998333803552618));
#113129=DIRECTION('ref_axis',(0.0662281834101546,0.996137339756707,-0.0576561190561847));
#113130=DIRECTION('center_axis',(-1.,0.,0.));
#113131=DIRECTION('ref_axis',(0.,0.,1.));
#113132=DIRECTION('',(0.,1.23467863058847E-16,-1.));
#113133=DIRECTION('center_axis',(-1.,0.,0.));
#113134=DIRECTION('ref_axis',(0.,0.977150339649859,-0.212549320681494));
#113135=DIRECTION('',(0.,1.,0.));
#113136=DIRECTION('center_axis',(0.,0.,1.));
#113137=DIRECTION('ref_axis',(1.,0.,0.));
#113138=DIRECTION('center_axis',(0.998974276838322,0.045281273125727,-2.27917889832281E-5));
#113139=DIRECTION('ref_axis',(0.0443009274833836,-0.977241931984893,0.207450317412498));
#113140=DIRECTION('center_axis',(0.,-1.18842113532926E-16,1.));
#113141=DIRECTION('ref_axis',(0.,1.,1.18842113532926E-16));
#113142=DIRECTION('center_axis',(0.,0.,1.));
#113143=DIRECTION('ref_axis',(0.,-1.,0.));
#113144=DIRECTION('center_axis',(0.,1.19033121480991E-16,-1.));
#113145=DIRECTION('ref_axis',(0.,-1.,-1.19033121480991E-16));
#113146=DIRECTION('center_axis',(1.,0.,1.87032180698308E-16));
#113147=DIRECTION('ref_axis',(-1.87032180698308E-16,0.,1.));
#113148=DIRECTION('center_axis',(0.999999999999922,3.86396291419339E-7,
-8.7347856309549E-8));
#113149=DIRECTION('ref_axis',(-5.51687615636349E-8,0.354181556536311,0.935176681172875));
#113150=DIRECTION('',(-1.87032180698308E-16,-1.23467863058847E-16,1.));
#113151=DIRECTION('',(0.,-1.,0.));
#113152=DIRECTION('center_axis',(-0.995792257730495,-0.0916393879573366,
4.49311545952089E-5));
#113153=DIRECTION('ref_axis',(0.0902711933575697,-0.980840233260372,0.172637042570649));
#113154=DIRECTION('center_axis',(0.,0.,-1.));
#113155=DIRECTION('ref_axis',(-1.,0.,0.));
#113156=DIRECTION('center_axis',(-0.049502590584409,-0.39010562996265,-0.91943846504096));
#113157=DIRECTION('ref_axis',(0.184301157644048,0.901190701629574,-0.392286123368467));
#113158=DIRECTION('center_axis',(-1.,0.,0.));
#113159=DIRECTION('ref_axis',(0.,0.,1.));
#113160=DIRECTION('',(0.,1.23467863058847E-16,-1.));
#113161=DIRECTION('center_axis',(-0.999999999999951,3.06438016471383E-7,
-6.99460036508937E-8));
#113162=DIRECTION('ref_axis',(1.06561681951965E-7,0.539875486057826,0.841744889829344));
#113163=DIRECTION('',(0.,1.,0.));
#113164=DIRECTION('center_axis',(0.,0.,1.));
#113165=DIRECTION('ref_axis',(1.,0.,0.));
#113166=DIRECTION('center_axis',(0.994006408314,0.109321806185977,-5.40642036517117E-5));
#113167=DIRECTION('ref_axis',(0.10805711689382,-0.982431998566189,0.152154617681619));
#113168=DIRECTION('center_axis',(0.,-1.18842113532926E-16,1.));
#113169=DIRECTION('ref_axis',(0.,1.,1.18842113532926E-16));
#113170=DIRECTION('center_axis',(0.,1.19033121480991E-16,-1.));
#113171=DIRECTION('ref_axis',(0.,-1.,-1.19033121480991E-16));
#113172=DIRECTION('center_axis',(0.,0.,1.));
#113173=DIRECTION('ref_axis',(1.,0.,0.));
#113174=DIRECTION('center_axis',(0.999999999999995,9.8647085618326E-8,-2.32552699791606E-8));
#113175=DIRECTION('ref_axis',(9.49367917791162E-8,-0.992051753854412,-0.125830511698778));
#113176=DIRECTION('center_axis',(-0.989231594111401,-0.146358629503497,
6.91496543724644E-5));
#113177=DIRECTION('ref_axis',(0.145900204554444,-0.986095533541962,0.0795533094193093));
#113178=DIRECTION('center_axis',(1.,0.,1.87032180698308E-16));
#113179=DIRECTION('ref_axis',(-1.87032180698308E-16,0.,1.));
#113180=DIRECTION('',(-1.87032180698308E-16,-1.23467863058847E-16,1.));
#113181=DIRECTION('',(0.,1.,0.));
#113182=DIRECTION('',(0.,-1.,0.));
#113183=DIRECTION('center_axis',(0.,-1.,0.));
#113184=DIRECTION('ref_axis',(0.,0.,-1.));
#113185=DIRECTION('',(0.,-1.,0.));
#113186=DIRECTION('center_axis',(0.,0.,1.));
#113187=DIRECTION('ref_axis',(1.,0.,0.));
#113188=DIRECTION('center_axis',(0.,0.,-1.));
#113189=DIRECTION('ref_axis',(1.,-1.23459581198307E-13,0.));
#113190=DIRECTION('',(0.,1.,0.));
#113191=DIRECTION('center_axis',(0.,-1.,0.));
#113192=DIRECTION('ref_axis',(0.,0.,-1.));
#113193=DIRECTION('',(0.,-1.,0.));
#113194=DIRECTION('center_axis',(-1.,0.,0.));
#113195=DIRECTION('ref_axis',(0.,0.,1.));
#113196=DIRECTION('',(0.,1.23467863058847E-16,-1.));
#113197=DIRECTION('center_axis',(-1.,0.,0.));
#113198=DIRECTION('ref_axis',(0.,-0.558140143909497,-0.829746696140868));
#113199=DIRECTION('',(0.,1.,0.));
#113200=DIRECTION('center_axis',(0.,0.,1.));
#113201=DIRECTION('ref_axis',(1.,0.,0.));
#113202=DIRECTION('center_axis',(0.,1.23467863058847E-16,-1.));
#113203=DIRECTION('ref_axis',(0.,1.,1.1837531408762E-16));
#113204=DIRECTION('center_axis',(0.,1.19212619247436E-16,-1.));
#113205=DIRECTION('ref_axis',(0.,1.,1.19212619247436E-16));
#113206=DIRECTION('center_axis',(0.,-1.,0.));
#113207=DIRECTION('ref_axis',(1.,0.,0.));
#113208=DIRECTION('',(-5.01606788234257E-16,-1.,0.));
#113209=DIRECTION('',(5.01606788234257E-16,1.,0.));
#113210=DIRECTION('center_axis',(1.,-5.01606788234257E-16,0.));
#113211=DIRECTION('ref_axis',(-5.01606788234257E-16,-1.,0.));
#113212=DIRECTION('',(6.19323182390956E-32,1.23467863058847E-16,-1.));
#113213=DIRECTION('center_axis',(1.,-2.12838232963581E-8,-5.13483277355434E-9));
#113214=DIRECTION('ref_axis',(2.11055106046707E-8,0.999470690690628,-0.0325321141397118));
#113215=DIRECTION('',(6.19323182390956E-32,1.23467863058847E-16,-1.));
#113216=DIRECTION('center_axis',(0.,0.,-1.));
#113217=DIRECTION('ref_axis',(-1.,0.,0.));
#113218=DIRECTION('center_axis',(-0.986715031900344,0.162460579946267,7.60619890862346E-5));
#113219=DIRECTION('ref_axis',(0.162362454938592,0.986102575671949,0.0352156709358418));
#113220=DIRECTION('center_axis',(0.,-1.18842113532926E-16,1.));
#113221=DIRECTION('ref_axis',(0.,1.,1.18842113532926E-16));
#113222=DIRECTION('center_axis',(-5.51437847295852E-32,1.19033121480991E-16,
-1.));
#113223=DIRECTION('ref_axis',(-1.24344978758017E-14,-1.,-1.19033121480991E-16));
#113224=DIRECTION('center_axis',(-1.,5.01606788234257E-16,0.));
#113225=DIRECTION('ref_axis',(0.,0.,1.));
#113226=DIRECTION('',(-6.19323182390956E-32,-1.23467863058847E-16,1.));
#113227=DIRECTION('center_axis',(-0.999999999999983,-1.80161300130045E-7,
-4.18470807107181E-8));
#113228=DIRECTION('ref_axis',(1.57783577543169E-7,-0.949012696634457,0.315237849292515));
#113229=DIRECTION('',(-6.19323182390956E-32,-1.23467863058847E-16,1.));
#113230=DIRECTION('',(-5.01606788234257E-16,-1.,0.));
#113231=DIRECTION('center_axis',(0.991217376526726,-0.132242612086272,-6.34040519857628E-5));
#113232=DIRECTION('ref_axis',(0.131422968750417,0.985020258821126,0.111638223726418));
#113233=DIRECTION('center_axis',(0.,0.,-1.));
#113234=DIRECTION('ref_axis',(-1.,0.,0.));
#113235=DIRECTION('center_axis',(0.,-1.,0.));
#113236=DIRECTION('ref_axis',(1.,0.,0.));
#113237=DIRECTION('',(5.01606788234257E-16,1.,0.));
#113238=DIRECTION('center_axis',(0.,0.,-1.));
#113239=DIRECTION('ref_axis',(0.,-1.,0.));
#113240=DIRECTION('center_axis',(0.,0.,-1.));
#113241=DIRECTION('ref_axis',(-1.,0.,0.));
#113242=DIRECTION('',(-5.01606788234257E-16,-1.,0.));
#113243=DIRECTION('center_axis',(0.,-1.,0.));
#113244=DIRECTION('ref_axis',(1.,0.,0.));
#113245=DIRECTION('',(5.01606788234257E-16,1.,0.));
#113246=DIRECTION('center_axis',(1.,-5.01606788234257E-16,0.));
#113247=DIRECTION('ref_axis',(-5.01606788234257E-16,-1.,0.));
#113248=DIRECTION('',(6.19323182390956E-32,1.23467863058847E-16,-1.));
#113249=DIRECTION('center_axis',(0.999999999999961,-2.7050082141817E-7,
-6.20337418949715E-8));
#113250=DIRECTION('ref_axis',(1.37645784434391E-7,0.677526577092017,-0.735498291863385));
#113251=DIRECTION('',(6.19323182390956E-32,1.23467863058847E-16,-1.));
#113252=DIRECTION('center_axis',(0.,0.,-1.));
#113253=DIRECTION('ref_axis',(-1.,0.,0.));
#113254=DIRECTION('center_axis',(0.,0.,-1.));
#113255=DIRECTION('ref_axis',(-1.,0.,0.));
#113256=DIRECTION('center_axis',(-0.993204090877291,0.116385697482287,5.73251750129611E-5));
#113257=DIRECTION('ref_axis',(0.115221510518281,0.983199503181504,0.141572385928648));
#113258=DIRECTION('center_axis',(0.,-1.18842113532926E-16,1.));
#113259=DIRECTION('ref_axis',(0.,1.,1.18842113532926E-16));
#113260=DIRECTION('center_axis',(-6.69603100287811E-32,1.19033121480991E-16,
-1.));
#113261=DIRECTION('ref_axis',(-1.50990331349022E-14,-1.,-1.19033121480991E-16));
#113262=DIRECTION('center_axis',(-1.,5.01606788234257E-16,0.));
#113263=DIRECTION('ref_axis',(0.,0.,1.));
#113264=DIRECTION('',(-6.19323182390956E-32,-1.23467863058847E-16,1.));
#113265=DIRECTION('center_axis',(-0.999999999999896,-4.44492331285063E-7,
-9.98246615501216E-8));
#113266=DIRECTION('ref_axis',(-3.30569703989997E-8,0.289344971519085,-0.957224888652932));
#113267=DIRECTION('',(-6.19323182390956E-32,-1.23467863058847E-16,1.));
#113268=DIRECTION('center_axis',(0.997110719027039,-0.0759619154585161,
-3.74333490112874E-5));
#113269=DIRECTION('ref_axis',(0.0746245599506448,0.979463680395188,0.187302092457309));
#113270=DIRECTION('center_axis',(0.,0.,-1.));
#113271=DIRECTION('ref_axis',(-1.,0.,0.));
#113272=DIRECTION('center_axis',(-0.0109863751058524,0.174010750210057,
-0.984682465759072));
#113273=DIRECTION('ref_axis',(0.115492347803954,-0.977930751386158,-0.174106183382538));
#113274=DIRECTION('center_axis',(1.,-5.01606788234257E-16,0.));
#113275=DIRECTION('ref_axis',(-5.01606788234257E-16,-1.,0.));
#113276=DIRECTION('',(6.19323182390956E-32,1.23467863058847E-16,-1.));
#113277=DIRECTION('center_axis',(1.,0.,0.));
#113278=DIRECTION('ref_axis',(0.,0.97773854081723,0.20982694250404));
#113279=DIRECTION('',(6.19323182390956E-32,1.23467863058847E-16,-1.));
#113280=DIRECTION('center_axis',(0.,0.,-1.));
#113281=DIRECTION('ref_axis',(-1.,0.,0.));
#113282=DIRECTION('center_axis',(0.,0.,-1.));
#113283=DIRECTION('ref_axis',(-1.,0.,0.));
#113284=DIRECTION('center_axis',(-0.998403025832976,0.0564924526119683,
2.83803315785685E-5));
#113285=DIRECTION('ref_axis',(0.0553351197097672,0.977847823027442,0.201870402801399));
#113286=DIRECTION('center_axis',(0.,-1.18842113532926E-16,1.));
#113287=DIRECTION('ref_axis',(0.,1.,1.18842113532926E-16));
#113288=DIRECTION('center_axis',(-1.73309037721552E-31,1.19033121480991E-16,
-1.));
#113289=DIRECTION('ref_axis',(-3.90798504668055E-14,-1.,-1.19033121480991E-16));
#113290=DIRECTION('center_axis',(-1.,5.01606788234257E-16,0.));
#113291=DIRECTION('ref_axis',(0.,0.,1.));
#113292=DIRECTION('',(-6.19323182390956E-32,-1.23467863058847E-16,1.));
#113293=DIRECTION('center_axis',(-1.,0.,0.));
#113294=DIRECTION('ref_axis',(0.,0.976478786201388,0.215613497023408));
#113295=DIRECTION('',(-6.19323182390956E-32,-1.23467863058847E-16,1.));
#113296=DIRECTION('',(-2.85977186515575E-47,-5.70122241611331E-32,-1.));
#113297=DIRECTION('center_axis',(0.999946064618564,-0.0103859437316171,
-5.16237906977087E-6));
#113298=DIRECTION('ref_axis',(0.0101433645819431,0.976483796643044,0.215352053736538));
#113299=DIRECTION('center_axis',(0.,0.,-1.));
#113300=DIRECTION('ref_axis',(-1.,0.,0.));
#113301=DIRECTION('center_axis',(0.,0.,1.));
#113302=DIRECTION('ref_axis',(1.,0.,0.));
#113303=DIRECTION('center_axis',(2.85977186515575E-47,0.,1.));
#113304=DIRECTION('ref_axis',(0.,-1.,0.));
#113305=DIRECTION('center_axis',(1.0547118733939E-12,0.,1.));
#113306=DIRECTION('ref_axis',(1.,0.,-1.0547118733939E-12));
#113307=DIRECTION('',(2.85977186515575E-47,5.70122241611331E-32,1.));
#113308=DIRECTION('center_axis',(0.,0.,1.));
#113309=DIRECTION('ref_axis',(1.,0.,0.));
#113310=DIRECTION('center_axis',(-0.91200931366711,-0.410169491533009,-5.52463721181358E-12));
#113311=DIRECTION('ref_axis',(0.410169491533009,-0.91200931366711,-2.38205677224627E-27));
#113312=DIRECTION('center_axis',(0.,0.,-1.));
#113313=DIRECTION('ref_axis',(1.,0.,0.));
#113314=DIRECTION('center_axis',(-0.908150397510606,-0.418644067796653,
0.));
#113315=DIRECTION('ref_axis',(0.418644067796653,-0.908150397510606,0.));
#113316=DIRECTION('center_axis',(0.,0.,1.));
#113317=DIRECTION('ref_axis',(0.,-1.,0.));
#113318=DIRECTION('',(0.,-1.23467863058847E-16,1.));
#113319=DIRECTION('center_axis',(1.5706724042304E-30,1.99810034797076E-44,
-1.));
#113320=DIRECTION('ref_axis',(1.27213054904966E-14,-1.,2.98704733337335E-59));
#113321=DIRECTION('center_axis',(-0.999990764844661,-0.00426925256430225,
0.000493667835992639));
#113322=DIRECTION('ref_axis',(0.00426925308452771,-0.999990886697524,1.74890393922737E-21));
#113323=DIRECTION('center_axis',(0.,0.,-1.));
#113324=DIRECTION('ref_axis',(-1.,0.,0.));
#113325=DIRECTION('center_axis',(0.,0.,1.));
#113326=DIRECTION('ref_axis',(0.,-1.,0.));
#113327=DIRECTION('',(0.,1.23467863058847E-16,-1.));
#113328=DIRECTION('center_axis',(0.,-6.17339315294237E-17,1.));
#113329=DIRECTION('ref_axis',(0.,-1.,0.));
#113330=DIRECTION('center_axis',(-8.2246118621519E-31,1.09573841495595E-44,
-1.));
#113331=DIRECTION('ref_axis',(-1.33226762955019E-14,-1.,1.36906336112945E-59));
#113332=DIRECTION('center_axis',(0.,0.,1.));
#113333=DIRECTION('ref_axis',(0.664473794614039,0.747311565728258,0.));
#113334=DIRECTION('center_axis',(-1.66533453693774E-13,-1.96105155259282E-14,
-1.));
#113335=DIRECTION('ref_axis',(-1.,3.15330219577248E-42,1.66533453693774E-13));
#113336=DIRECTION('',(0.,-1.23467863058847E-16,1.));
#113337=DIRECTION('center_axis',(-0.99077695153738,-0.134510490459868,0.0163694917007939));
#113338=DIRECTION('ref_axis',(0.134528515815408,-0.990909722645057,-8.11100475129765E-19));
#113339=DIRECTION('center_axis',(0.00303671055821314,-0.143796114085276,
-0.989602675806285));
#113340=DIRECTION('ref_axis',(0.135485018598647,-0.980423214395597,0.142878026335506));
#113341=DIRECTION('center_axis',(-0.989571111262359,-0.142966967401199,
0.017591531686721));
#113342=DIRECTION('ref_axis',(0.142989093957737,-0.989724264130745,-6.72869096378782E-19));
#113343=DIRECTION('center_axis',(0.,0.,-1.));
#113344=DIRECTION('ref_axis',(-1.,0.,0.));
#113345=DIRECTION('center_axis',(0.,0.,1.));
#113346=DIRECTION('ref_axis',(0.,-1.,0.));
#113347=DIRECTION('',(0.,1.23467863058847E-16,-1.));
#113348=DIRECTION('center_axis',(0.,-6.17339315294237E-17,1.));
#113349=DIRECTION('ref_axis',(0.,-1.,0.));
#113350=DIRECTION('center_axis',(2.19322982990717E-31,7.79191761746451E-46,
-1.));
#113351=DIRECTION('ref_axis',(3.5527136788005E-15,-1.,-1.0890276736257E-60));
#113352=DIRECTION('center_axis',(0.,0.,1.));
#113353=DIRECTION('ref_axis',(0.610293066582435,0.792175720961838,0.));
#113354=DIRECTION('center_axis',(0.,0.,-1.));
#113355=DIRECTION('ref_axis',(-1.,0.,0.));
#113356=DIRECTION('',(0.,-1.23467863058847E-16,1.));
#113357=DIRECTION('center_axis',(-0.962287669136798,-0.272033898305467,
-2.53734057564779E-13));
#113358=DIRECTION('ref_axis',(0.272033898305467,-0.962287669136798,2.03523668564842E-29));
#113359=DIRECTION('center_axis',(0.,0.,1.));
#113360=DIRECTION('ref_axis',(1.,0.,0.));
#113361=DIRECTION('center_axis',(0.,0.,-1.));
#113362=DIRECTION('ref_axis',(1.,0.,0.));
#113363=DIRECTION('center_axis',(-0.959851548777671,-0.280508474576272,
0.));
#113364=DIRECTION('ref_axis',(0.280508474576272,-0.959851548777671,0.));
#113365=DIRECTION('center_axis',(0.,0.,-1.));
#113366=DIRECTION('ref_axis',(-1.,0.,0.));
#113367=DIRECTION('center_axis',(0.,0.,1.));
#113368=DIRECTION('ref_axis',(0.,-1.,0.));
#113369=DIRECTION('',(0.,1.23467863058847E-16,-1.));
#113370=DIRECTION('center_axis',(0.,-6.17339315294237E-17,1.));
#113371=DIRECTION('ref_axis',(0.,-1.,0.));
#113372=DIRECTION('center_axis',(1.37076864369198E-30,3.04371781932207E-44,
-1.));
#113373=DIRECTION('ref_axis',(2.22044604925031E-14,-1.,3.98272977783113E-59));
#113374=DIRECTION('center_axis',(0.,0.,1.));
#113375=DIRECTION('ref_axis',(0.550808342809402,0.834631756819474,0.));
#113376=DIRECTION('center_axis',(0.,0.,-1.));
#113377=DIRECTION('ref_axis',(-1.,0.,0.));
#113378=DIRECTION('',(0.,-1.23467863058847E-16,1.));
#113379=DIRECTION('center_axis',(0.,0.,-1.));
#113380=DIRECTION('ref_axis',(0.,1.,0.));
#113381=DIRECTION('',(0.,0.,-1.));
#113382=DIRECTION('center_axis',(0.,0.,-1.));
#113383=DIRECTION('ref_axis',(0.,1.,0.));
#113384=DIRECTION('center_axis',(0.,0.,-1.));
#113385=DIRECTION('ref_axis',(0.,1.,0.));
#113386=DIRECTION('',(0.,0.,-1.));
#113387=DIRECTION('center_axis',(0.,0.,-1.));
#113388=DIRECTION('ref_axis',(0.,-1.,0.));
#113389=DIRECTION('center_axis',(0.,-1.23467863058847E-16,1.));
#113390=DIRECTION('ref_axis',(0.,-1.,0.));
#113391=DIRECTION('center_axis',(0.902736181373369,0.430194591829591,-1.25279811715363E-14));
#113392=DIRECTION('ref_axis',(-0.430194591829591,0.902736181373369,2.66752875008673E-30));
#113393=DIRECTION('center_axis',(0.,0.,1.));
#113394=DIRECTION('ref_axis',(0.,-1.,0.));
#113395=DIRECTION('center_axis',(0.990268068741571,0.139173100960064,0.));
#113396=DIRECTION('ref_axis',(-0.139173100960064,0.990268068741571,0.));
#113397=DIRECTION('center_axis',(0.990268068741571,0.139173100960064,1.71834053708117E-17));
#113398=DIRECTION('ref_axis',(-0.139173100960064,0.990268068741571,-7.54967553857625E-35));
#113399=DIRECTION('',(-0.990268068741571,-0.139173100960059,-1.71834053708117E-17));
#113400=DIRECTION('center_axis',(0.990268068741571,0.139173100960064,7.72565905471723E-15));
#113401=DIRECTION('ref_axis',(-0.139173100960064,0.990268068741571,-6.67502150120727E-33));
#113402=DIRECTION('center_axis',(0.,-1.23467863058847E-16,1.));
#113403=DIRECTION('ref_axis',(0.,-1.,0.));
#113404=DIRECTION('center_axis',(3.11538328111815E-31,7.86084147552191E-46,
-1.));
#113405=DIRECTION('ref_axis',(2.52323414687536E-15,-1.,-6.22301527786114E-61));
#113406=DIRECTION('center_axis',(0.728126055379271,0.685443248911113,0.));
#113407=DIRECTION('ref_axis',(-0.685443248911113,0.728126055379271,0.));
#113408=DIRECTION('center_axis',(0.,-1.23467863058847E-16,1.));
#113409=DIRECTION('ref_axis',(0.,-1.,0.));
#113410=DIRECTION('center_axis',(0.,0.,-1.));
#113411=DIRECTION('ref_axis',(0.,-1.,0.));
#113412=DIRECTION('center_axis',(0.685443248911113,0.728126055379271,1.18468586241421E-15));
#113413=DIRECTION('ref_axis',(-0.728126055379271,0.685443248911113,-2.6468713136043E-31));
#113414=DIRECTION('center_axis',(0.,-1.23467863058847E-16,1.));
#113415=DIRECTION('ref_axis',(0.,-1.,0.));
#113416=DIRECTION('center_axis',(-1.24615331244726E-30,1.2577346360835E-44,
-1.));
#113417=DIRECTION('ref_axis',(-1.00929365875014E-14,-1.,-9.95682444457783E-60));
#113418=DIRECTION('center_axis',(0.139173100960064,0.990268068741571,3.86282952735861E-15));
#113419=DIRECTION('ref_axis',(-0.990268068741571,0.139173100960064,3.00533800087463E-32));
#113420=DIRECTION('center_axis',(0.139173100960064,0.990268068741571,1.22266282302934E-16));
#113421=DIRECTION('ref_axis',(-0.990268068741571,0.139173100960064,-6.46427645420959E-34));
#113422=DIRECTION('',(-0.139173100960065,-0.99026806874157,-1.22266282302933E-16));
#113423=DIRECTION('center_axis',(0.139173100960068,0.99026806874157,0.));
#113424=DIRECTION('ref_axis',(-0.99026806874157,0.139173100960068,0.));
#113425=DIRECTION('center_axis',(0.,-1.23467863058847E-16,1.));
#113426=DIRECTION('ref_axis',(0.,-1.,0.));
#113427=DIRECTION('center_axis',(0.,0.,1.));
#113428=DIRECTION('ref_axis',(0.,-1.,0.));
#113429=DIRECTION('center_axis',(0.425784239486448,0.90482472413443,-1.18178866550092E-14));
#113430=DIRECTION('ref_axis',(-0.90482472413443,0.425784239486448,3.74967935723291E-30));
#113431=DIRECTION('center_axis',(0.,-1.23467863058847E-16,1.));
#113432=DIRECTION('ref_axis',(0.,-1.,0.));
#113433=DIRECTION('center_axis',(-2.19322982990717E-31,3.89595880873225E-46,
-1.));
#113434=DIRECTION('ref_axis',(-1.77635683940025E-15,-1.,-5.4451383681285E-61));
#113435=DIRECTION('center_axis',(-0.425784239486454,0.904824724134427,0.));
#113436=DIRECTION('ref_axis',(-0.904824724134427,-0.425784239486454,0.));
#113437=DIRECTION('center_axis',(0.,-1.23467863058847E-16,1.));
#113438=DIRECTION('ref_axis',(0.,-1.,0.));
#113439=DIRECTION('center_axis',(0.,0.,1.));
#113440=DIRECTION('ref_axis',(0.,-1.,0.));
#113441=DIRECTION('center_axis',(-0.139173100960068,0.99026806874157,0.));
#113442=DIRECTION('ref_axis',(-0.99026806874157,-0.139173100960068,0.));
#113443=DIRECTION('center_axis',(-0.139173100960068,0.99026806874157,1.22266282302933E-16));
#113444=DIRECTION('ref_axis',(-0.99026806874157,-0.139173100960068,-6.9848527780828E-33));
#113445=DIRECTION('',(0.139173100960067,-0.99026806874157,-1.22266282302933E-16));
#113446=DIRECTION('center_axis',(-0.139173100960068,0.99026806874157,2.36226307343407E-14));
#113447=DIRECTION('ref_axis',(-0.99026806874157,-0.139173100960068,-1.46728138438144E-30));
#113448=DIRECTION('center_axis',(0.,-1.23467863058847E-16,1.));
#113449=DIRECTION('ref_axis',(0.,-1.,0.));
#113450=DIRECTION('center_axis',(-6.23076656223629E-31,3.14433659020876E-45,
-1.));
#113451=DIRECTION('ref_axis',(-5.04646829375071E-15,-1.,1.86690458335834E-60));
#113452=DIRECTION('center_axis',(-0.685443248911113,0.728126055379271,1.18468586241421E-15));
#113453=DIRECTION('ref_axis',(-0.728126055379271,-0.685443248911113,2.6468713136043E-31));
#113454=DIRECTION('center_axis',(0.,-1.23467863058847E-16,1.));
#113455=DIRECTION('ref_axis',(0.,-1.,0.));
#113456=DIRECTION('center_axis',(0.,0.,-1.));
#113457=DIRECTION('ref_axis',(0.,-1.,0.));
#113458=DIRECTION('center_axis',(-0.728126055379271,0.685443248911113,-1.18468586241421E-15));
#113459=DIRECTION('ref_axis',(-0.685443248911113,-0.728126055379271,2.48798705504199E-31));
#113460=DIRECTION('center_axis',(0.,-1.23467863058847E-16,1.));
#113461=DIRECTION('ref_axis',(0.,-1.,0.));
#113462=DIRECTION('center_axis',(3.11538328111815E-31,7.86084147552189E-46,
-1.));
#113463=DIRECTION('ref_axis',(2.52323414687536E-15,-1.,3.11150763893057E-61));
#113464=DIRECTION('center_axis',(-0.990268068741571,0.139173100960064,3.86282952735861E-15));
#113465=DIRECTION('ref_axis',(-0.139173100960064,-0.990268068741571,3.33751075060364E-33));
#113466=DIRECTION('center_axis',(-0.990268068741571,0.139173100960064,1.71834053708117E-17));
#113467=DIRECTION('ref_axis',(-0.139173100960064,-0.990268068741571,7.54967553857625E-35));
#113468=DIRECTION('',(0.990268068741571,-0.139173100960059,-1.71834053708117E-17));
#113469=DIRECTION('center_axis',(-0.990268068741572,0.139173100960051,1.7605559658208E-14));
#113470=DIRECTION('ref_axis',(-0.139173100960051,-0.990268068741572,2.08829111071605E-30));
#113471=DIRECTION('center_axis',(0.,-1.23467863058847E-16,1.));
#113472=DIRECTION('ref_axis',(0.,-1.,0.));
#113473=DIRECTION('center_axis',(0.,0.,1.));
#113474=DIRECTION('ref_axis',(0.,-1.,0.));
#113475=DIRECTION('center_axis',(-0.904824724134424,0.42578423948646,0.));
#113476=DIRECTION('ref_axis',(-0.42578423948646,-0.904824724134424,0.));
#113477=DIRECTION('center_axis',(0.,0.,-1.));
#113478=DIRECTION('ref_axis',(0.,-1.,0.));
#113479=DIRECTION('center_axis',(0.,0.,1.));
#113480=DIRECTION('ref_axis',(0.,-1.,0.));
#113481=DIRECTION('',(0.,1.23467863058847E-16,-1.));
#113482=DIRECTION('center_axis',(0.,0.,1.));
#113483=DIRECTION('ref_axis',(1.,0.,0.));
#113484=DIRECTION('center_axis',(0.990268068741572,-0.139173100960052,0.));
#113485=DIRECTION('ref_axis',(0.139173100960052,0.990268068741572,0.));
#113486=DIRECTION('center_axis',(0.990268068741571,-0.139173100960059,0.));
#113487=DIRECTION('ref_axis',(0.139173100960059,0.990268068741571,0.));
#113488=DIRECTION('',(-0.990268068741571,0.139173100960059,0.));
#113489=DIRECTION('center_axis',(0.,0.,1.));
#113490=DIRECTION('ref_axis',(1.,0.,0.));
#113491=DIRECTION('center_axis',(0.904824724134427,-0.425784239486454,0.));
#113492=DIRECTION('ref_axis',(0.425784239486454,0.904824724134427,0.));
#113493=DIRECTION('center_axis',(0.,0.,-1.));
#113494=DIRECTION('ref_axis',(1.,-1.5419764230905E-15,0.));
#113495=DIRECTION('center_axis',(0.,-1.,0.));
#113496=DIRECTION('ref_axis',(0.,0.,-1.));
#113497=DIRECTION('',(0.,1.,0.));
#113498=DIRECTION('',(0.,-1.,0.));
#113499=DIRECTION('center_axis',(0.,1.,0.));
#113500=DIRECTION('ref_axis',(0.,0.,-1.));
#113501=DIRECTION('center_axis',(-1.,0.,-1.6326809185664E-16));
#113502=DIRECTION('ref_axis',(-1.6326809185664E-16,0.,1.));
#113503=DIRECTION('',(1.6326809185664E-16,0.,-1.));
#113504=DIRECTION('',(0.,-1.,0.));
#113505=DIRECTION('center_axis',(0.,-1.,0.));
#113506=DIRECTION('ref_axis',(0.,0.,-1.));
#113507=DIRECTION('center_axis',(0.,-1.,0.));
#113508=DIRECTION('ref_axis',(0.,0.,-1.));
#113509=DIRECTION('',(0.,1.,0.));
#113510=DIRECTION('center_axis',(1.,0.,0.));
#113511=DIRECTION('ref_axis',(0.,1.,0.));
#113512=DIRECTION('',(1.,-4.38004274807345E-16,0.));
#113513=DIRECTION('center_axis',(0.,-1.,0.));
#113514=DIRECTION('ref_axis',(0.,0.,-1.));
#113515=DIRECTION('center_axis',(0.,1.,0.));
#113516=DIRECTION('ref_axis',(0.,0.,1.));
#113517=DIRECTION('',(0.,-1.,0.));
#113518=DIRECTION('center_axis',(0.,0.,-1.));
#113519=DIRECTION('ref_axis',(-1.,0.,0.));
#113520=DIRECTION('center_axis',(-1.,0.,0.));
#113521=DIRECTION('ref_axis',(0.,0.,1.));
#113522=DIRECTION('center_axis',(0.,0.,-1.));
#113523=DIRECTION('ref_axis',(-1.,0.,0.));
#113524=DIRECTION('center_axis',(1.,0.,0.));
#113525=DIRECTION('ref_axis',(0.,0.,-1.));
#113526=DIRECTION('center_axis',(-1.,0.,0.));
#113527=DIRECTION('ref_axis',(0.,0.,1.));
#113528=DIRECTION('',(1.,0.,0.));
#113529=DIRECTION('center_axis',(0.,0.,-1.));
#113530=DIRECTION('ref_axis',(-1.,0.,0.));
#113531=DIRECTION('center_axis',(0.,-1.,0.));
#113532=DIRECTION('ref_axis',(0.,0.,-1.));
#113533=DIRECTION('center_axis',(0.,0.,-1.));
#113534=DIRECTION('ref_axis',(-1.,0.,0.));
#113535=DIRECTION('center_axis',(0.,-1.,0.));
#113536=DIRECTION('ref_axis',(0.,0.,-1.));
#113537=DIRECTION('',(0.,1.,0.));
#113538=DIRECTION('center_axis',(1.,0.,0.));
#113539=DIRECTION('ref_axis',(0.,1.,0.));
#113540=DIRECTION('',(1.,-4.38004274807345E-16,0.));
#113541=DIRECTION('center_axis',(0.,-1.,0.));
#113542=DIRECTION('ref_axis',(0.,0.,-1.));
#113543=DIRECTION('center_axis',(0.,1.,0.));
#113544=DIRECTION('ref_axis',(0.,0.,1.));
#113545=DIRECTION('',(0.,-1.,0.));
#113546=DIRECTION('center_axis',(0.,0.,-1.));
#113547=DIRECTION('ref_axis',(-1.,0.,0.));
#113548=DIRECTION('center_axis',(-1.,0.,0.));
#113549=DIRECTION('ref_axis',(0.,0.,1.));
#113550=DIRECTION('center_axis',(0.,0.,-1.));
#113551=DIRECTION('ref_axis',(-1.,0.,0.));
#113552=DIRECTION('center_axis',(1.,0.,0.));
#113553=DIRECTION('ref_axis',(0.,0.,-1.));
#113554=DIRECTION('center_axis',(-1.,0.,0.));
#113555=DIRECTION('ref_axis',(0.,0.,1.));
#113556=DIRECTION('',(1.,0.,0.));
#113557=DIRECTION('center_axis',(0.,0.,-1.));
#113558=DIRECTION('ref_axis',(-1.,0.,0.));
#113559=DIRECTION('center_axis',(0.,-1.,0.));
#113560=DIRECTION('ref_axis',(0.,0.,-1.));
#113561=DIRECTION('center_axis',(0.,0.,-1.));
#113562=DIRECTION('ref_axis',(-1.,0.,0.));
#113563=DIRECTION('center_axis',(0.,-1.,0.));
#113564=DIRECTION('ref_axis',(0.,0.,-1.));
#113565=DIRECTION('',(0.,1.,0.));
#113566=DIRECTION('center_axis',(1.,0.,0.));
#113567=DIRECTION('ref_axis',(0.,1.,0.));
#113568=DIRECTION('',(1.,-4.38004274807345E-16,0.));
#113569=DIRECTION('center_axis',(1.,0.,-1.73472347597681E-14));
#113570=DIRECTION('ref_axis',(-1.73472347597681E-14,0.,-1.));
#113571=DIRECTION('center_axis',(0.950554487276066,-0.310557831521497,3.79371153572051E-14));
#113572=DIRECTION('ref_axis',(0.310557831521497,0.950554487276066,1.69736969313821E-30));
#113573=DIRECTION('center_axis',(0.,0.,-1.));
#113574=DIRECTION('ref_axis',(-1.,0.,0.));
#113575=DIRECTION('center_axis',(0.,0.,-1.));
#113576=DIRECTION('ref_axis',(-1.,0.,0.));
#113577=DIRECTION('center_axis',(0.,-1.,0.));
#113578=DIRECTION('ref_axis',(0.,0.,-1.));
#113579=DIRECTION('center_axis',(0.,1.,0.));
#113580=DIRECTION('ref_axis',(0.,0.,1.));
#113581=DIRECTION('',(0.,-1.,0.));
#113582=DIRECTION('center_axis',(0.,0.,-1.));
#113583=DIRECTION('ref_axis',(-1.,0.,0.));
#113584=DIRECTION('center_axis',(-1.,0.,0.));
#113585=DIRECTION('ref_axis',(0.,0.,1.));
#113586=DIRECTION('center_axis',(0.,0.,-1.));
#113587=DIRECTION('ref_axis',(-1.,0.,0.));
#113588=DIRECTION('center_axis',(1.,0.,0.));
#113589=DIRECTION('ref_axis',(0.,0.,-1.));
#113590=DIRECTION('center_axis',(-1.,0.,0.));
#113591=DIRECTION('ref_axis',(0.,0.,1.));
#113592=DIRECTION('',(1.,0.,0.));
#113593=DIRECTION('center_axis',(0.,0.,-1.));
#113594=DIRECTION('ref_axis',(-1.,0.,0.));
#113595=DIRECTION('center_axis',(0.,-1.,0.));
#113596=DIRECTION('ref_axis',(0.,0.,-1.));
#113597=DIRECTION('center_axis',(0.,0.,-1.));
#113598=DIRECTION('ref_axis',(-1.,0.,0.));
#113599=DIRECTION('center_axis',(0.,-1.,0.));
#113600=DIRECTION('ref_axis',(0.,0.,-1.));
#113601=DIRECTION('',(0.,1.,0.));
#113602=DIRECTION('center_axis',(0.,0.,-1.));
#113603=DIRECTION('ref_axis',(-1.,0.,0.));
#113604=DIRECTION('center_axis',(0.,0.,-1.));
#113605=DIRECTION('ref_axis',(-1.,0.,0.));
#113606=DIRECTION('center_axis',(0.,-1.,0.));
#113607=DIRECTION('ref_axis',(0.,0.,-1.));
#113608=DIRECTION('center_axis',(0.,1.,0.));
#113609=DIRECTION('ref_axis',(0.,0.,1.));
#113610=DIRECTION('',(0.,-1.,0.));
#113611=DIRECTION('center_axis',(0.,0.,-1.));
#113612=DIRECTION('ref_axis',(-1.,0.,0.));
#113613=DIRECTION('center_axis',(-1.,0.,0.));
#113614=DIRECTION('ref_axis',(0.,0.,1.));
#113615=DIRECTION('center_axis',(0.,0.,-1.));
#113616=DIRECTION('ref_axis',(-1.,0.,0.));
#113617=DIRECTION('center_axis',(1.,0.,0.));
#113618=DIRECTION('ref_axis',(0.,0.,-1.));
#113619=DIRECTION('center_axis',(-1.,0.,0.));
#113620=DIRECTION('ref_axis',(0.,0.,1.));
#113621=DIRECTION('',(1.,0.,0.));
#113622=DIRECTION('center_axis',(0.,0.,-1.));
#113623=DIRECTION('ref_axis',(-1.,0.,0.));
#113624=DIRECTION('center_axis',(0.,-1.,0.));
#113625=DIRECTION('ref_axis',(0.,0.,-1.));
#113626=DIRECTION('center_axis',(0.,0.,-1.));
#113627=DIRECTION('ref_axis',(-1.,0.,0.));
#113628=DIRECTION('center_axis',(0.,-1.,0.));
#113629=DIRECTION('ref_axis',(0.,0.,-1.));
#113630=DIRECTION('center_axis',(0.,-1.,0.));
#113631=DIRECTION('ref_axis',(0.,0.,-1.));
#113632=DIRECTION('',(0.,1.,0.));
#113633=DIRECTION('center_axis',(0.,-1.,0.));
#113634=DIRECTION('ref_axis',(0.,0.,-1.));
#113635=DIRECTION('center_axis',(0.,1.,0.));
#113636=DIRECTION('ref_axis',(0.,0.,-1.));
#113637=DIRECTION('',(0.,1.,0.));
#113638=DIRECTION('center_axis',(1.,0.,0.));
#113639=DIRECTION('ref_axis',(0.,0.,-1.));
#113640=DIRECTION('center_axis',(-1.,0.,0.));
#113641=DIRECTION('ref_axis',(0.,0.,1.));
#113642=DIRECTION('',(1.,0.,0.));
#113643=DIRECTION('center_axis',(0.,0.,-1.));
#113644=DIRECTION('ref_axis',(-1.,0.,0.));
#113645=DIRECTION('center_axis',(0.,0.,-1.));
#113646=DIRECTION('ref_axis',(-1.,0.,0.));
#113647=DIRECTION('center_axis',(0.,0.423401464461212,0.905942161449671));
#113648=DIRECTION('ref_axis',(0.,-0.905942161449671,0.423401464461211));
#113649=DIRECTION('center_axis',(0.999426495211847,-0.0338626728150633,
-7.64099929122785E-6));
#113650=DIRECTION('ref_axis',(-0.00722436375911664,-0.213000171029248,-0.97702545294879));
#113651=DIRECTION('center_axis',(6.703313282803E-15,0.423071618151431,0.90609624539269));
#113652=DIRECTION('ref_axis',(-9.44993610611347E-31,-0.90609624539269,0.423071618151431));
#113653=DIRECTION('center_axis',(-0.999690772268051,-0.0248668391563904,
1.23482154850145E-5));
#113654=DIRECTION('ref_axis',(0.0242988167036592,-0.976749496966587,0.213002318490482));
#113655=DIRECTION('center_axis',(0.,0.,-1.));
#113656=DIRECTION('ref_axis',(-1.,0.,0.));
#113657=DIRECTION('center_axis',(0.,-1.,0.));
#113658=DIRECTION('ref_axis',(1.,0.,0.));
#113659=DIRECTION('',(5.01606788234257E-16,1.,0.));
#113660=DIRECTION('center_axis',(0.,0.,-1.));
#113661=DIRECTION('ref_axis',(0.,-1.,0.));
#113662=DIRECTION('center_axis',(0.,0.,1.));
#113663=DIRECTION('ref_axis',(-1.,-5.55111512312579E-15,0.));
#113664=DIRECTION('center_axis',(0.,0.,-1.));
#113665=DIRECTION('ref_axis',(-1.,0.,0.));
#113666=DIRECTION('center_axis',(0.,1.23467863058847E-16,-1.));
#113667=DIRECTION('ref_axis',(-1.,0.,0.));
#113668=DIRECTION('',(-0.996194698091747,-0.0871557427476402,-1.07609333103578E-17));
#113669=DIRECTION('',(-0.0871557427476402,-0.996194698091747,-1.22998030563942E-16));
#113670=DIRECTION('center_axis',(0.,0.,-1.));
#113671=DIRECTION('ref_axis',(0.,1.,0.));
#113672=DIRECTION('',(-0.707106781186547,-0.707106781186548,-8.73049632275231E-17));
#113673=DIRECTION('center_axis',(0.,0.,-1.));
#113674=DIRECTION('ref_axis',(0.,1.,0.));
#113675=DIRECTION('center_axis',(0.,1.23467863058847E-16,-1.));
#113676=DIRECTION('ref_axis',(-1.,0.,0.));
#113677=DIRECTION('',(0.0871557427476566,-0.996194698091746,-1.22998030563941E-16));
#113678=DIRECTION('',(0.996194698091746,-0.0871557427476568,-1.07609333103598E-17));
#113679=DIRECTION('center_axis',(0.,0.,-1.));
#113680=DIRECTION('ref_axis',(0.,1.,0.));
#113681=DIRECTION('',(0.707106781186547,-0.707106781186548,-8.73049632275231E-17));
#113682=DIRECTION('center_axis',(0.,0.,-1.));
#113683=DIRECTION('ref_axis',(0.,1.,0.));
#113684=DIRECTION('center_axis',(-0.0871557427476394,-0.996194698091747,
-1.22998030563942E-16));
#113685=DIRECTION('ref_axis',(0.996194698091747,-0.0871557427476394,8.16488070285074E-35));
#113686=DIRECTION('',(0.0871557427476402,0.996194698091747,1.22998030563942E-16));
#113687=DIRECTION('center_axis',(0.0871557427476394,0.996194698091747,0.));
#113688=DIRECTION('ref_axis',(-0.996194698091747,0.0871557427476394,0.));
#113689=DIRECTION('center_axis',(0.,4.51531312649963E-33,-1.));
#113690=DIRECTION('ref_axis',(-1.,0.,0.));
#113691=DIRECTION('center_axis',(0.,0.,-1.));
#113692=DIRECTION('ref_axis',(-1.,0.,0.));
#113693=DIRECTION('',(-1.08020383274181E-17,4.42963887209064E-33,-1.));
#113694=DIRECTION('center_axis',(0.,0.,-1.));
#113695=DIRECTION('ref_axis',(-1.,0.,0.));
#113696=DIRECTION('center_axis',(-0.0871557427476469,-0.996194698091747,
1.3824978635387E-14));
#113697=DIRECTION('ref_axis',(0.996194698091747,-0.0871557427476469,-9.13671722807069E-31));
#113698=DIRECTION('center_axis',(0.0871557427476469,0.996194698091747,0.));
#113699=DIRECTION('ref_axis',(-0.996194698091747,0.0871557427476469,0.));
#113700=DIRECTION('center_axis',(-0.0871557427476469,-0.996194698091747,
0.));
#113701=DIRECTION('ref_axis',(0.996194698091747,-0.0871557427476469,0.));
#113702=DIRECTION('',(0.0871557427476402,0.996194698091747,0.));
#113703=DIRECTION('center_axis',(0.,0.,-1.));
#113704=DIRECTION('ref_axis',(-1.,0.,0.));
#113705=DIRECTION('center_axis',(0.,-4.51531312649963E-33,1.));
#113706=DIRECTION('ref_axis',(1.,0.,0.));
#113707=DIRECTION('',(1.08020383274181E-17,-4.42963887209064E-33,1.));
#113708=DIRECTION('center_axis',(-0.0871557427476394,-0.996194698091747,
-1.22998030563942E-16));
#113709=DIRECTION('ref_axis',(0.996194698091747,-0.0871557427476394,8.16488070285074E-35));
#113710=DIRECTION('',(0.0871557427476402,0.996194698091747,1.22998030563942E-16));
#113711=DIRECTION('center_axis',(0.,-4.51531312649963E-33,1.));
#113712=DIRECTION('ref_axis',(-0.737277336810104,-0.675590207615682,-3.0505013325817E-33));
#113713=DIRECTION('center_axis',(0.,0.,1.));
#113714=DIRECTION('ref_axis',(1.,0.,0.));
#113715=DIRECTION('',(-1.08020383274181E-17,4.42963887209064E-33,-1.));
#113716=DIRECTION('center_axis',(-0.0871557427476469,-0.996194698091747,
0.));
#113717=DIRECTION('ref_axis',(0.996194698091747,-0.0871557427476469,0.));
#113718=DIRECTION('center_axis',(0.0871557427476469,0.996194698091747,0.));
#113719=DIRECTION('ref_axis',(-0.996194698091747,0.0871557427476469,0.));
#113720=DIRECTION('center_axis',(-0.0871557427476469,-0.996194698091747,
1.3824978635387E-14));
#113721=DIRECTION('ref_axis',(0.996194698091747,-0.0871557427476469,-9.13671722807069E-31));
#113722=DIRECTION('',(0.0871557427476402,0.996194698091747,0.));
#113723=DIRECTION('center_axis',(0.,0.,-1.));
#113724=DIRECTION('ref_axis',(-1.,0.,0.));
#113725=DIRECTION('center_axis',(0.,-4.73133896404192E-33,1.));
#113726=DIRECTION('ref_axis',(1.,0.,0.));
#113727=DIRECTION('',(1.08020383274181E-17,-4.62223186652937E-33,1.));
#113728=DIRECTION('center_axis',(-0.0871557427476394,-0.996194698091747,
-1.22998030563942E-16));
#113729=DIRECTION('ref_axis',(0.996194698091747,-0.0871557427476394,8.16488070285074E-35));
#113730=DIRECTION('',(0.0871557427476402,0.996194698091747,1.22998030563942E-16));
#113731=DIRECTION('center_axis',(0.0871557427476394,0.996194698091747,0.));
#113732=DIRECTION('ref_axis',(-0.996194698091747,0.0871557427476394,0.));
#113733=DIRECTION('center_axis',(-0.0690733635565107,-0.78951215817867,
-0.609835570080205));
#113734=DIRECTION('ref_axis',(3.95541556389227E-18,0.611295598907861,-0.791402357057319));
#113735=DIRECTION('center_axis',(-0.996194698091743,0.0871557427476822,
-4.52226792607938E-16));
#113736=DIRECTION('ref_axis',(0.039915296454851,0.456233926159048,0.888964213976255));
#113737=DIRECTION('center_axis',(0.,0.,1.));
#113738=DIRECTION('ref_axis',(1.,0.,0.));
#113739=DIRECTION('center_axis',(0.,4.51531312649963E-33,-1.));
#113740=DIRECTION('ref_axis',(-1.,0.,0.));
#113741=DIRECTION('',(1.08020383274181E-17,-4.42963887209064E-33,1.));
#113742=DIRECTION('center_axis',(0.,-4.51531312650048E-33,-1.));
#113743=DIRECTION('ref_axis',(-1.,0.,0.));
#113744=DIRECTION('',(1.08020383274202E-17,-4.37133056147834E-33,-1.));
#113745=DIRECTION('center_axis',(0.,0.,-1.));
#113746=DIRECTION('ref_axis',(-1.,0.,0.));
#113747=DIRECTION('center_axis',(0.0871557427476538,-0.996194698091746,
-6.91248931769351E-15));
#113748=DIRECTION('ref_axis',(0.996194698091746,0.0871557427476538,2.78649888037662E-32));
#113749=DIRECTION('center_axis',(-0.0871557427476538,0.996194698091746,
0.));
#113750=DIRECTION('ref_axis',(-0.996194698091746,-0.0871557427476538,0.));
#113751=DIRECTION('center_axis',(0.0871557427476538,-0.996194698091746,
-6.91248931769351E-15));
#113752=DIRECTION('ref_axis',(0.996194698091746,0.0871557427476538,2.78649888037662E-32));
#113753=DIRECTION('',(-0.0871557427476566,0.996194698091746,0.));
#113754=DIRECTION('center_axis',(0.,0.,-1.));
#113755=DIRECTION('ref_axis',(-1.,0.,0.));
#113756=DIRECTION('center_axis',(0.,4.51531312650048E-33,1.));
#113757=DIRECTION('ref_axis',(-0.737277336810102,0.675590207615685,-3.05050133258229E-33));
#113758=DIRECTION('',(-1.08020383274202E-17,4.37133056147834E-33,1.));
#113759=DIRECTION('center_axis',(0.0871557427476572,-0.996194698091746,
-1.22998030563942E-16));
#113760=DIRECTION('ref_axis',(0.996194698091746,0.0871557427476572,1.44426287624373E-33));
#113761=DIRECTION('',(-0.0871557427476566,0.996194698091746,1.22998030563941E-16));
#113762=DIRECTION('center_axis',(0.0871557427476607,-0.996194698091745,
0.));
#113763=DIRECTION('ref_axis',(0.996194698091745,0.0871557427476607,0.));
#113764=DIRECTION('center_axis',(0.,4.51531312650048E-33,1.));
#113765=DIRECTION('ref_axis',(1.,0.,0.));
#113766=DIRECTION('center_axis',(0.,0.,1.));
#113767=DIRECTION('ref_axis',(1.,0.,0.));
#113768=DIRECTION('',(1.08020383274202E-17,-4.37133056147834E-33,-1.));
#113769=DIRECTION('center_axis',(0.0479130906931042,-0.547649132616206,
0.835335120346889));
#113770=DIRECTION('ref_axis',(2.39380283931159E-17,-0.836295598856108,-0.54827882626808));
#113771=DIRECTION('center_axis',(-0.996194698091723,-0.0871557427479135,
-1.21464724749175E-13));
#113772=DIRECTION('ref_axis',(-0.0257890725821804,0.294770448454491,-0.955220030387392));
#113773=DIRECTION('center_axis',(0.0871557427476572,-0.996194698091746,
-1.22998030563942E-16));
#113774=DIRECTION('ref_axis',(0.996194698091746,0.0871557427476572,1.44426287624373E-33));
#113775=DIRECTION('',(-0.0871557427476566,0.996194698091746,1.22998030563941E-16));
#113776=DIRECTION('center_axis',(-0.0871557427476572,0.996194698091746,
0.));
#113777=DIRECTION('ref_axis',(-0.996194698091746,-0.0871557427476572,0.));
#113778=DIRECTION('center_axis',(0.,-4.73133896404282E-33,-1.));
#113779=DIRECTION('ref_axis',(-1.,0.,0.));
#113780=DIRECTION('',(1.08020383274202E-17,-4.56392355591706E-33,-1.));
#113781=DIRECTION('center_axis',(0.,0.,-1.));
#113782=DIRECTION('ref_axis',(-1.,0.,0.));
#113783=DIRECTION('center_axis',(-0.0871557427476538,0.996194698091746,
0.));
#113784=DIRECTION('ref_axis',(-0.996194698091746,-0.0871557427476538,0.));
#113785=DIRECTION('center_axis',(-0.0871557427476538,0.996194698091746,
0.));
#113786=DIRECTION('ref_axis',(-0.996194698091746,-0.0871557427476538,0.));
#113787=DIRECTION('',(-0.0871557427476566,0.996194698091746,0.));
#113788=DIRECTION('center_axis',(-0.0871557427476538,0.996194698091746,
0.));
#113789=DIRECTION('ref_axis',(-0.996194698091746,-0.0871557427476538,0.));
#113790=DIRECTION('center_axis',(0.,0.,1.));
#113791=DIRECTION('ref_axis',(1.,0.,0.));
#113792=DIRECTION('center_axis',(0.,4.51531312650048E-33,1.));
#113793=DIRECTION('ref_axis',(-0.737277336810104,0.675590207615683,-3.05050133258228E-33));
#113794=DIRECTION('',(-1.08020383274202E-17,4.37133056147834E-33,1.));
#113795=DIRECTION('center_axis',(0.0871557427476572,-0.996194698091746,
-1.22998030563942E-16));
#113796=DIRECTION('ref_axis',(0.996194698091746,0.0871557427476572,1.44426287624373E-33));
#113797=DIRECTION('',(-0.0871557427476566,0.996194698091746,1.22998030563941E-16));
#113798=DIRECTION('center_axis',(0.707106781186548,-0.707106781186548,-8.7304963227523E-17));
#113799=DIRECTION('ref_axis',(0.707106781186548,0.707106781186548,2.5701266908181E-33));
#113800=DIRECTION('center_axis',(-0.707106781186544,0.707106781186551,0.));
#113801=DIRECTION('ref_axis',(-0.707106781186551,-0.707106781186544,0.));
#113802=DIRECTION('center_axis',(-0.707106781186548,0.707106781186548,0.));
#113803=DIRECTION('ref_axis',(-0.707106781186548,-0.707106781186548,0.));
#113804=DIRECTION('',(-0.707106781186547,0.707106781186548,8.73049632275231E-17));
#113805=DIRECTION('center_axis',(0.,-1.07104667533214E-16,1.));
#113806=DIRECTION('ref_axis',(1.,0.,0.));
#113807=DIRECTION('center_axis',(0.,0.,1.));
#113808=DIRECTION('ref_axis',(1.,0.,0.));
#113809=DIRECTION('',(1.87032180698308E-16,1.07104667533214E-16,-1.));
#113810=DIRECTION('center_axis',(0.996194698091745,-0.0871557427476607,
-1.2095289040845E-15));
#113811=DIRECTION('ref_axis',(0.0871557427476607,0.996194698091745,-5.51367835803032E-32));
#113812=DIRECTION('center_axis',(-0.996194698091746,0.0871557427476572,
0.));
#113813=DIRECTION('ref_axis',(-0.0871557427476572,-0.996194698091746,0.));
#113814=DIRECTION('center_axis',(0.996194698091745,-0.0871557427476607,
0.));
#113815=DIRECTION('ref_axis',(0.0871557427476607,0.996194698091745,0.));
#113816=DIRECTION('',(-0.996194698091746,0.0871557427476568,1.54074395550979E-33));
#113817=DIRECTION('center_axis',(0.,0.,-1.));
#113818=DIRECTION('ref_axis',(-1.,0.,0.));
#113819=DIRECTION('center_axis',(-5.40794518211031E-32,0.,1.));
#113820=DIRECTION('ref_axis',(0.,-1.,0.));
#113821=DIRECTION('',(-5.23852944873328E-32,-1.23467863058847E-16,1.));
#113822=DIRECTION('center_axis',(0.996194698091746,-0.0871557427476572,
-1.07609333103598E-17));
#113823=DIRECTION('ref_axis',(0.0871557427476572,0.996194698091746,-1.48387871229006E-34));
#113824=DIRECTION('',(-0.996194698091746,0.0871557427476568,1.07609333103598E-17));
#113825=DIRECTION('center_axis',(-0.996194698091746,0.0871557427476538,
0.));
#113826=DIRECTION('ref_axis',(-0.0871557427476538,-0.996194698091746,0.));
#113827=DIRECTION('center_axis',(-0.955086750882198,0.0835592633859996,
-0.284301156859545));
#113828=DIRECTION('ref_axis',(-0.28529890144429,-2.70823414235005E-19,0.958438593147564));
#113829=DIRECTION('center_axis',(0.,1.07104667533214E-16,-1.));
#113830=DIRECTION('ref_axis',(-1.,0.,0.));
#113831=DIRECTION('center_axis',(0.,0.,-1.));
#113832=DIRECTION('ref_axis',(-1.,0.,0.));
#113833=DIRECTION('',(1.87032180698308E-16,1.07104667533214E-16,-1.));
#113834=DIRECTION('center_axis',(-0.996194698091745,0.0871557427476607,
0.));
#113835=DIRECTION('ref_axis',(-0.0871557427476607,-0.996194698091745,0.));
#113836=DIRECTION('center_axis',(-0.996194698091746,0.0871557427476572,
0.));
#113837=DIRECTION('ref_axis',(-0.0871557427476572,-0.996194698091746,0.));
#113838=DIRECTION('',(-0.996194698091746,0.0871557427476568,1.54074395550979E-33));
#113839=DIRECTION('center_axis',(-0.996194698091746,0.0871557427476538,
0.));
#113840=DIRECTION('ref_axis',(-0.0871557427476538,-0.996194698091746,0.));
#113841=DIRECTION('center_axis',(0.,0.,1.));
#113842=DIRECTION('ref_axis',(1.,0.,0.));
#113843=DIRECTION('center_axis',(0.,0.,1.));
#113844=DIRECTION('ref_axis',(0.,-1.,0.));
#113845=DIRECTION('',(1.54074395550979E-33,-1.23467863058847E-16,1.));
#113846=DIRECTION('center_axis',(0.996194698091746,-0.0871557427476572,
-1.07609333103598E-17));
#113847=DIRECTION('ref_axis',(0.0871557427476572,0.996194698091746,-1.48387871229006E-34));
#113848=DIRECTION('',(-0.996194698091746,0.0871557427476568,1.07609333103598E-17));
#113849=DIRECTION('center_axis',(-0.913306614095669,0.407272671129681,2.94898912583324E-15));
#113850=DIRECTION('ref_axis',(-0.407272671129681,-0.913306614095669,-7.93980541862816E-31));
#113851=DIRECTION('center_axis',(-0.707106781186548,-0.707106781186548,
-8.7304963227523E-17));
#113852=DIRECTION('ref_axis',(0.707106781186548,-0.707106781186548,-2.5701266908181E-33));
#113853=DIRECTION('center_axis',(0.707106781186544,0.707106781186551,0.));
#113854=DIRECTION('ref_axis',(-0.707106781186551,0.707106781186544,0.));
#113855=DIRECTION('center_axis',(0.707106781186548,0.707106781186548,0.));
#113856=DIRECTION('ref_axis',(-0.707106781186548,0.707106781186548,0.));
#113857=DIRECTION('',(0.707106781186547,0.707106781186548,8.73049632275231E-17));
#113858=DIRECTION('center_axis',(6.19323182390956E-32,0.,-1.));
#113859=DIRECTION('ref_axis',(0.,1.,0.));
#113860=DIRECTION('',(6.16356212163056E-32,1.23467863058847E-16,-1.));
#113861=DIRECTION('center_axis',(0.,0.,-1.));
#113862=DIRECTION('ref_axis',(-1.,0.,0.));
#113863=DIRECTION('center_axis',(-0.996194698091747,-0.0871557427476457,
3.00690150789426E-14));
#113864=DIRECTION('ref_axis',(0.0871557427476457,-0.996194698091747,1.22577679051452E-30));
#113865=DIRECTION('center_axis',(0.996194698091747,0.0871557427476457,0.));
#113866=DIRECTION('ref_axis',(-0.0871557427476457,0.996194698091747,0.));
#113867=DIRECTION('center_axis',(-0.996194698091747,-0.0871557427476457,
0.));
#113868=DIRECTION('ref_axis',(0.0871557427476457,-0.996194698091747,0.));
#113869=DIRECTION('',(0.996194698091747,0.0871557427476402,1.54074395550979E-33));
#113870=DIRECTION('center_axis',(0.,0.,-1.));
#113871=DIRECTION('ref_axis',(-1.,0.,0.));
#113872=DIRECTION('center_axis',(-6.19323182390956E-32,0.,1.));
#113873=DIRECTION('ref_axis',(0.675590207615642,0.737277336810141,4.18408677372686E-32));
#113874=DIRECTION('',(-6.16356212163056E-32,-1.23467863058847E-16,1.));
#113875=DIRECTION('center_axis',(-0.996194698091747,-0.0871557427476409,
-1.07609333103578E-17));
#113876=DIRECTION('ref_axis',(0.0871557427476409,-0.996194698091747,2.79703111108876E-34));
#113877=DIRECTION('',(0.996194698091747,0.0871557427476402,1.07609333103578E-17));
#113878=DIRECTION('center_axis',(-0.996194698091747,-0.08715574274764,0.));
#113879=DIRECTION('ref_axis',(0.08715574274764,-0.996194698091747,0.));
#113880=DIRECTION('center_axis',(6.19323182390956E-32,0.,-1.));
#113881=DIRECTION('ref_axis',(0.,1.,0.));
#113882=DIRECTION('',(6.16356212163056E-32,1.23467863058847E-16,-1.));
#113883=DIRECTION('center_axis',(0.,0.,-1.));
#113884=DIRECTION('ref_axis',(-1.,0.,0.));
#113885=DIRECTION('center_axis',(-0.919081670180344,-0.0804092269952343,
0.385776152389619));
#113886=DIRECTION('ref_axis',(0.387029378450866,1.43097488374089E-17,0.922067383771889));
#113887=DIRECTION('center_axis',(-0.996194698091747,-0.0871557427476409,
-1.07609333103578E-17));
#113888=DIRECTION('ref_axis',(0.0871557427476409,-0.996194698091747,2.79703111108876E-34));
#113889=DIRECTION('',(0.996194698091747,0.0871557427476402,1.07609333103578E-17));
#113890=DIRECTION('center_axis',(0.996194698091747,0.0871557427476394,1.20952890408421E-15));
#113891=DIRECTION('ref_axis',(-0.0871557427476394,0.996194698091747,1.39857739234396E-32));
#113892=DIRECTION('center_axis',(0.,1.13523971920422E-16,-1.));
#113893=DIRECTION('ref_axis',(-1.,0.,0.));
#113894=DIRECTION('center_axis',(0.,0.,1.));
#113895=DIRECTION('ref_axis',(1.,0.,0.));
#113896=DIRECTION('',(-1.13659195805196E-16,1.13523971920422E-16,-1.));
#113897=DIRECTION('center_axis',(-0.996194698091747,-0.0871557427476457,
1.3824978635387E-14));
#113898=DIRECTION('ref_axis',(0.0871557427476457,-0.996194698091747,6.24837364119099E-31));
#113899=DIRECTION('center_axis',(0.996194698091747,0.0871557427476457,0.));
#113900=DIRECTION('ref_axis',(-0.0871557427476457,0.996194698091747,0.));
#113901=DIRECTION('center_axis',(-0.996194698091747,-0.0871557427476457,
0.));
#113902=DIRECTION('ref_axis',(0.0871557427476457,-0.996194698091747,0.));
#113903=DIRECTION('',(0.996194698091747,0.0871557427476402,1.54074395550979E-33));
#113904=DIRECTION('center_axis',(0.,0.,-1.));
#113905=DIRECTION('ref_axis',(-1.,0.,0.));
#113906=DIRECTION('center_axis',(-1.13659195805196E-16,0.,1.));
#113907=DIRECTION('ref_axis',(0.675590207615648,0.737277336810135,7.67870396914601E-17));
#113908=DIRECTION('',(-1.13659195805196E-16,-1.33411754197273E-16,1.));
#113909=DIRECTION('center_axis',(-0.996194698091747,-0.0871557427476409,
-1.07609333103578E-17));
#113910=DIRECTION('ref_axis',(0.0871557427476409,-0.996194698091747,2.79703111108876E-34));
#113911=DIRECTION('',(0.996194698091747,0.0871557427476402,1.07609333103578E-17));
#113912=DIRECTION('center_axis',(-0.405419774737912,0.90915150463265,0.0952803645860425));
#113913=DIRECTION('ref_axis',(-0.913306614095667,-0.407272671129684,-4.7539503937481E-18));
#113914=DIRECTION('center_axis',(0.,0.,1.));
#113915=DIRECTION('ref_axis',(1.,0.,0.));
#113916=DIRECTION('center_axis',(0.,0.,-1.));
#113917=DIRECTION('ref_axis',(0.,1.,0.));
#113918=DIRECTION('',(0.,-1.23467863058847E-16,1.));
#113919=DIRECTION('center_axis',(0.,-1.23467863058847E-16,1.));
#113920=DIRECTION('ref_axis',(0.,-1.,-1.21694324257719E-16));
#113921=DIRECTION('center_axis',(0.,-1.18842113532929E-16,1.));
#113922=DIRECTION('ref_axis',(0.,-1.,-1.18842113532929E-16));
#113923=DIRECTION('center_axis',(0.,0.,-1.));
#113924=DIRECTION('ref_axis',(0.,1.,0.));
#113925=DIRECTION('',(0.,1.23467863058847E-16,-1.));
#113926=DIRECTION('center_axis',(0.,0.,-1.));
#113927=DIRECTION('ref_axis',(-1.,0.,0.));
#113928=DIRECTION('center_axis',(-0.279133941838593,0.960252176521172,2.49865799020366E-15));
#113929=DIRECTION('ref_axis',(-0.960252176521172,-0.279133941838593,3.84227067759201E-30));
#113930=DIRECTION('center_axis',(0.,0.,-1.));
#113931=DIRECTION('ref_axis',(-1.,0.,0.));
#113932=DIRECTION('center_axis',(0.,0.,1.));
#113933=DIRECTION('ref_axis',(-1.,0.,0.));
#113934=DIRECTION('center_axis',(-0.270643175546941,0.962679734662503,0.));
#113935=DIRECTION('ref_axis',(-0.962679734662504,-0.270643175546941,0.));
#113936=DIRECTION('center_axis',(0.,0.,1.));
#113937=DIRECTION('ref_axis',(1.,0.,0.));
#113938=DIRECTION('center_axis',(0.,0.,-1.));
#113939=DIRECTION('ref_axis',(0.,1.,0.));
#113940=DIRECTION('',(0.,-1.23467863058847E-16,1.));
#113941=DIRECTION('center_axis',(0.,-1.23467863058847E-16,1.));
#113942=DIRECTION('ref_axis',(0.,-1.,-1.21694324257719E-16));
#113943=DIRECTION('center_axis',(0.,-1.18842113532929E-16,1.));
#113944=DIRECTION('ref_axis',(0.,-1.,-1.18842113532929E-16));
#113945=DIRECTION('center_axis',(0.,0.,-1.));
#113946=DIRECTION('ref_axis',(0.,1.,0.));
#113947=DIRECTION('',(0.,1.23467863058847E-16,-1.));
#113948=DIRECTION('center_axis',(0.,0.,-1.));
#113949=DIRECTION('ref_axis',(-1.,0.,0.));
#113950=DIRECTION('center_axis',(0.141334929101325,-0.989809819863889,-0.0173481502454526));
#113951=DIRECTION('ref_axis',(0.989958799240908,0.1413562018643,-1.53957070961197E-18));
#113952=DIRECTION('center_axis',(0.132860127107541,-0.991003467296,-0.0161342626814395));
#113953=DIRECTION('ref_axis',(0.991132478736687,0.132877423188709,7.57324997548269E-19));
#113954=DIRECTION('center_axis',(0.14258112270268,0.00286725800189432,0.989778966376026));
#113955=DIRECTION('ref_axis',(0.97964031348631,0.142384138292289,-0.141533082193549));
#113956=DIRECTION('center_axis',(0.,0.,-1.));
#113957=DIRECTION('ref_axis',(-1.,0.,0.));
#113958=DIRECTION('center_axis',(0.,0.,-1.));
#113959=DIRECTION('ref_axis',(0.,1.,0.));
#113960=DIRECTION('',(0.,-1.23467863058847E-16,1.));
#113961=DIRECTION('center_axis',(0.,-1.23467863058847E-16,1.));
#113962=DIRECTION('ref_axis',(0.,-1.,-1.21694324257719E-16));
#113963=DIRECTION('center_axis',(0.,-1.18842113532929E-16,1.));
#113964=DIRECTION('ref_axis',(0.,-1.,-1.18842113532929E-16));
#113965=DIRECTION('center_axis',(0.,0.,-1.));
#113966=DIRECTION('ref_axis',(0.,1.,0.));
#113967=DIRECTION('',(0.,1.23467863058847E-16,-1.));
#113968=DIRECTION('center_axis',(3.91353616180368E-12,0.,-1.));
#113969=DIRECTION('ref_axis',(-1.,0.,-3.91353616180368E-12));
#113970=DIRECTION('center_axis',(0.00235261362124023,-0.999997195602435,
-0.000272022820600068));
#113971=DIRECTION('ref_axis',(0.999997232600541,0.00235261370828272,8.12493746167259E-22));
#113972=DIRECTION('center_axis',(-0.00620231251671424,-0.999980508301815,
0.000717172147678158));
#113973=DIRECTION('ref_axis',(0.999980765464846,-0.00620231411175082,5.84684475171815E-22));
#113974=DIRECTION('center_axis',(0.115833873408401,-1.74164817710871E-9,
0.993268601019486));
#113975=DIRECTION('ref_axis',(0.993265814819633,0.00236857700963695,-0.115833548480737));
#113976=DIRECTION('center_axis',(0.,0.,-1.));
#113977=DIRECTION('ref_axis',(-1.,0.,0.));
#113978=DIRECTION('center_axis',(0.,0.,-1.));
#113979=DIRECTION('ref_axis',(0.,1.,0.));
#113980=DIRECTION('',(0.,-1.23467863058847E-16,1.));
#113981=DIRECTION('center_axis',(0.,-1.23467863058847E-16,1.));
#113982=DIRECTION('ref_axis',(0.,-1.,-1.21694324257719E-16));
#113983=DIRECTION('center_axis',(0.,-1.18842113532929E-16,1.));
#113984=DIRECTION('ref_axis',(0.,-1.,-1.18842113532929E-16));
#113985=DIRECTION('center_axis',(0.,0.,-1.));
#113986=DIRECTION('ref_axis',(0.,1.,0.));
#113987=DIRECTION('',(0.,1.23467863058847E-16,-1.));
#113988=DIRECTION('center_axis',(6.61970478432749E-12,0.,-1.));
#113989=DIRECTION('ref_axis',(-1.,0.,-6.61970478432749E-12));
#113990=DIRECTION('center_axis',(-0.136675079747296,-0.990475586151279,
0.0166744059669382));
#113991=DIRECTION('ref_axis',(0.990613308713893,-0.136694083993833,9.06110283290218E-19));
#113992=DIRECTION('center_axis',(-0.14514509610524,-0.989248239790814,0.0179114808817288));
#113993=DIRECTION('ref_axis',(0.989406963861029,-0.145168384517086,-1.21343959465114E-18));
#113994=DIRECTION('center_axis',(0.145269618843932,-0.00325155863630697,
0.989386762195338));
#113995=DIRECTION('ref_axis',(0.979906495320475,-0.137666580604216,-0.144330083535927));
#113996=DIRECTION('center_axis',(1.18805075949821E-12,7.25808302348696E-12,
-1.));
#113997=DIRECTION('ref_axis',(-5.87747175411144E-39,1.,7.25808302348696E-12));
#113998=DIRECTION('center_axis',(0.,0.,-1.));
#113999=DIRECTION('ref_axis',(0.,1.,0.));
#114000=DIRECTION('',(0.,-1.23467863058847E-16,1.));
#114001=DIRECTION('center_axis',(0.,-1.23467863058847E-16,1.));
#114002=DIRECTION('ref_axis',(0.,-1.,-1.21694324257719E-16));
#114003=DIRECTION('center_axis',(0.,-1.18842113532929E-16,1.));
#114004=DIRECTION('ref_axis',(0.,-1.,-1.18842113532929E-16));
#114005=DIRECTION('center_axis',(0.,0.,-1.));
#114006=DIRECTION('ref_axis',(0.,1.,0.));
#114007=DIRECTION('',(0.,1.23467863058847E-16,-1.));
#114008=DIRECTION('center_axis',(0.,0.,-1.));
#114009=DIRECTION('ref_axis',(-1.,0.,0.));
#114010=DIRECTION('center_axis',(0.274464020377229,0.96159736975429,0.));
#114011=DIRECTION('ref_axis',(-0.96159736975429,0.274464020377229,0.));
#114012=DIRECTION('center_axis',(0.,0.,-1.));
#114013=DIRECTION('ref_axis',(-1.,0.,0.));
#114014=DIRECTION('center_axis',(0.,0.,1.));
#114015=DIRECTION('ref_axis',(-1.,0.,0.));
#114016=DIRECTION('center_axis',(0.282954786668892,0.959133248668381,0.));
#114017=DIRECTION('ref_axis',(-0.959133248668381,0.282954786668892,0.));
#114018=DIRECTION('center_axis',(0.,0.,1.));
#114019=DIRECTION('ref_axis',(1.,0.,0.));
#114020=DIRECTION('center_axis',(0.,0.,-1.));
#114021=DIRECTION('ref_axis',(0.,1.,0.));
#114022=DIRECTION('',(0.,-1.23467863058847E-16,1.));
#114023=DIRECTION('center_axis',(0.,-1.23467863058847E-16,1.));
#114024=DIRECTION('ref_axis',(0.,-1.,-1.21694324257719E-16));
#114025=DIRECTION('center_axis',(0.,-1.18842113532929E-16,1.));
#114026=DIRECTION('ref_axis',(0.,-1.,-1.18842113532929E-16));
#114027=DIRECTION('center_axis',(0.,0.,-1.));
#114028=DIRECTION('ref_axis',(0.,1.,0.));
#114029=DIRECTION('center_axis',(0.,0.,1.));
#114030=DIRECTION('ref_axis',(1.,0.,0.));
#114031=DIRECTION('',(0.,1.23467863058847E-16,-1.));
#114032=DIRECTION('center_axis',(-0.388071473886494,-0.870248040119286,
0.303428541544968));
#114033=DIRECTION('ref_axis',(0.913306614096678,-0.407272671127417,-4.84423453041484E-17));
#114034=DIRECTION('center_axis',(0.0871557427476569,0.996194698091746,1.22998030563941E-16));
#114035=DIRECTION('ref_axis',(1.41124413247282E-15,4.52989727324155E-33,
-1.));
#114036=DIRECTION('',(1.54074395550979E-33,-1.23467863058847E-16,1.));
#114037=DIRECTION('',(0.996194698091746,-0.0871557427476568,0.));
#114038=DIRECTION('',(-3.08148791101958E-33,1.23467863058847E-16,-1.));
#114039=DIRECTION('center_axis',(0.,1.23467863058847E-16,-1.));
#114040=DIRECTION('ref_axis',(0.,1.,0.));
#114041=DIRECTION('center_axis',(5.71153601538325E-31,-2.64211616260596E-45,
1.));
#114042=DIRECTION('ref_axis',(4.62592926927148E-15,1.,1.24460305557223E-60));
#114043=DIRECTION('center_axis',(0.707106781186548,0.707106781186547,8.7304963227523E-17));
#114044=DIRECTION('ref_axis',(2.16153073061992E-33,1.23467863058847E-16,
-1.));
#114045=DIRECTION('',(1.23259516440783E-32,1.23467863058847E-16,-1.));
#114046=DIRECTION('',(-1.23259516440783E-32,-1.23467863058847E-16,1.));
#114047=DIRECTION('',(0.707106781186547,-0.707106781186548,0.));
#114048=DIRECTION('center_axis',(-1.67127905768941E-33,0.,-1.));
#114049=DIRECTION('ref_axis',(0.,1.,0.));
#114050=DIRECTION('center_axis',(5.71153601538325E-31,-2.64211616260596E-45,
1.));
#114051=DIRECTION('ref_axis',(4.62592926927148E-15,1.,1.24460305557223E-60));
#114052=DIRECTION('center_axis',(0.,1.23467863058847E-16,-1.));
#114053=DIRECTION('ref_axis',(0.,1.,0.));
#114054=DIRECTION('center_axis',(-2.85576800769162E-31,-6.6052904065149E-46,
1.));
#114055=DIRECTION('ref_axis',(-2.31296463463574E-15,1.,3.11150763893057E-61));
#114056=DIRECTION('center_axis',(0.996194698091746,0.0871557427476566,1.07609333103598E-17));
#114057=DIRECTION('ref_axis',(1.4714164960684E-33,1.23467863058847E-16,
-1.));
#114058=DIRECTION('',(0.,-1.23467863058847E-16,1.));
#114059=DIRECTION('',(0.0871557427476566,-0.996194698091746,-3.51482972517089E-16));
#114060=DIRECTION('',(0.,1.23467863058847E-16,-1.));
#114061=DIRECTION('center_axis',(-4.26141870503966E-34,0.,-1.));
#114062=DIRECTION('ref_axis',(0.,1.,0.));
#114063=DIRECTION('center_axis',(-2.85576800769162E-31,-6.6052904065149E-46,
1.));
#114064=DIRECTION('ref_axis',(-2.31296463463574E-15,1.,3.11150763893057E-61));
#114065=DIRECTION('center_axis',(0.272999209159005,-0.962014257585904,0.));
#114066=DIRECTION('ref_axis',(0.962014257585904,0.272999209159004,0.));
#114067=DIRECTION('center_axis',(0.,0.,-1.));
#114068=DIRECTION('ref_axis',(-1.,0.,0.));
#114069=DIRECTION('center_axis',(-0.384110320270104,0.923287204428827,0.));
#114070=DIRECTION('ref_axis',(-0.923287204428827,-0.384110320270104,0.));
#114071=DIRECTION('center_axis',(0.,0.,-1.));
#114072=DIRECTION('ref_axis',(-1.,0.,0.));
#114073=DIRECTION('center_axis',(-0.886109103059821,-0.368607756298431,
-0.280960814832168));
#114074=DIRECTION('ref_axis',(-0.25934119650515,-0.10807938690911,0.959719224523834));
#114075=DIRECTION('center_axis',(0.,1.18842113532929E-16,-1.));
#114076=DIRECTION('ref_axis',(0.,1.,1.18842113532929E-16));
#114077=DIRECTION('center_axis',(0.,0.,1.));
#114078=DIRECTION('ref_axis',(-1.,1.78263170299393E-15,0.));
#114079=DIRECTION('',(0.,1.23467863058847E-16,-1.));
#114080=DIRECTION('',(0.,-1.23467863058847E-16,1.));
#114081=DIRECTION('center_axis',(0.,0.,-1.));
#114082=DIRECTION('ref_axis',(0.,1.,0.));
#114083=DIRECTION('center_axis',(0.,0.,-1.));
#114084=DIRECTION('ref_axis',(0.,1.,0.));
#114085=DIRECTION('center_axis',(-0.334110320282714,-0.942533974921107,
0.));
#114086=DIRECTION('ref_axis',(0.942533974921107,-0.334110320282714,0.));
#114087=DIRECTION('center_axis',(0.,0.,-1.));
#114088=DIRECTION('ref_axis',(-1.,0.,0.));
#114089=DIRECTION('center_axis',(-0.222999209171599,-0.974818625544692,
0.));
#114090=DIRECTION('ref_axis',(0.974818625544692,-0.222999209171599,0.));
#114091=DIRECTION('center_axis',(0.,0.,-1.));
#114092=DIRECTION('ref_axis',(-1.,0.,0.));
#114093=DIRECTION('center_axis',(0.,0.,-1.));
#114094=DIRECTION('ref_axis',(0.688859710772108,-0.724894681229603,0.));
#114095=DIRECTION('',(0.,1.23467863058847E-16,-1.));
#114096=DIRECTION('center_axis',(0.,4.63518112781003E-12,-1.));
#114097=DIRECTION('ref_axis',(0.,1.,4.63518112781003E-12));
#114098=DIRECTION('center_axis',(-0.997624402707396,0.0684293228260734,
-0.00793592466417746));
#114099=DIRECTION('ref_axis',(-0.0684314777296081,-0.997655818835204,-3.0788904879186E-19));
#114100=DIRECTION('center_axis',(0.00012024518356205,0.117893637119934,
0.993026221138057));
#114101=DIRECTION('ref_axis',(0.0688956039867685,0.990665697053439,-0.117621734526076));
#114102=DIRECTION('center_axis',(-0.996993498376656,0.0769676640255834,
-0.00894107874490511));
#114103=DIRECTION('ref_axis',(-0.07697074071877,-0.997033352036532,7.99587428479913E-19));
#114104=DIRECTION('center_axis',(0.,0.,1.));
#114105=DIRECTION('ref_axis',(1.,0.,0.));
#114106=DIRECTION('center_axis',(0.,0.,-1.));
#114107=DIRECTION('ref_axis',(0.,1.,0.));
#114108=DIRECTION('',(0.,-1.23467863058847E-16,1.));
#114109=DIRECTION('center_axis',(0.,-1.23467863058847E-16,1.));
#114110=DIRECTION('ref_axis',(0.,-1.,-1.21694324257719E-16));
#114111=DIRECTION('center_axis',(0.,-1.18842113532929E-16,1.));
#114112=DIRECTION('ref_axis',(0.,-1.,-1.18842113532929E-16));
#114113=DIRECTION('center_axis',(0.,0.,-1.));
#114114=DIRECTION('ref_axis',(0.634315526883886,-0.773074260568814,0.));
#114115=DIRECTION('',(0.,1.23467863058847E-16,-1.));
#114116=DIRECTION('center_axis',(0.,-1.38777878078144E-14,-1.));
#114117=DIRECTION('ref_axis',(0.,1.,-1.38777878078144E-14));
#114118=DIRECTION('center_axis',(-0.976728808322011,0.212349635823786,-0.0301407889639504));
#114119=DIRECTION('ref_axis',(-0.212446157929364,-0.977172773863994,-1.17576428045677E-20));
#114120=DIRECTION('center_axis',(0.0251527414239144,0.25401807230836,0.966872358969686));
#114121=DIRECTION('ref_axis',(0.213030566219325,0.943601106365079,-0.253446108517911));
#114122=DIRECTION('center_axis',(-0.974807460973989,0.220687770576049,-0.0323623538639763));
#114123=DIRECTION('ref_axis',(-0.220803427003966,-0.975318330917298,-7.28333184199878E-18));
#114124=DIRECTION('center_axis',(2.7755575615626E-13,5.13478148889134E-13,
1.));
#114125=DIRECTION('ref_axis',(-1.14794370197489E-40,-1.,5.13478148889134E-13));
#114126=DIRECTION('center_axis',(0.,0.,-1.));
#114127=DIRECTION('ref_axis',(0.,1.,0.));
#114128=DIRECTION('',(0.,-1.23467863058847E-16,1.));
#114129=DIRECTION('center_axis',(0.,-1.23467863058847E-16,1.));
#114130=DIRECTION('ref_axis',(0.,-1.,-1.21694324257719E-16));
#114131=DIRECTION('center_axis',(0.,-1.18842113532929E-16,1.));
#114132=DIRECTION('ref_axis',(0.,-1.,-1.18842113532929E-16));
#114133=DIRECTION('center_axis',(0.,0.,-1.));
#114134=DIRECTION('ref_axis',(0.574616980402509,-0.818422461711006,0.));
#114135=DIRECTION('center_axis',(0.,0.,-1.));
#114136=DIRECTION('ref_axis',(-1.,0.,0.));
#114137=DIRECTION('',(0.,1.23467863058847E-16,-1.));
#114138=DIRECTION('center_axis',(-0.934252508717439,0.356612184249462,0.));
#114139=DIRECTION('ref_axis',(-0.356612184249462,-0.934252508717439,0.));
#114140=DIRECTION('center_axis',(0.,0.,1.));
#114141=DIRECTION('ref_axis',(1.,0.,0.));
#114142=DIRECTION('center_axis',(0.,0.,1.));
#114143=DIRECTION('ref_axis',(1.,0.,0.));
#114144=DIRECTION('center_axis',(-0.930967150605313,0.365102950541111,0.));
#114145=DIRECTION('ref_axis',(-0.365102950541111,-0.930967150605313,0.));
#114146=DIRECTION('center_axis',(0.,0.,1.));
#114147=DIRECTION('ref_axis',(1.,0.,0.));
#114148=DIRECTION('center_axis',(0.,0.,-1.));
#114149=DIRECTION('ref_axis',(0.,1.,0.));
#114150=DIRECTION('',(0.,-1.23467863058847E-16,1.));
#114151=DIRECTION('center_axis',(0.,1.23467863058847E-16,-1.));
#114152=DIRECTION('ref_axis',(0.,1.,1.21694324257719E-16));
#114153=DIRECTION('center_axis',(4.39608526712911E-31,-1.18842113532929E-16,
1.));
#114154=DIRECTION('ref_axis',(9.50350909079134E-14,1.,1.18842113532929E-16));
#114155=DIRECTION('center_axis',(0.,0.,-1.));
#114156=DIRECTION('ref_axis',(0.,1.,0.));
#114157=DIRECTION('',(0.,1.23467863058847E-16,-1.));
#114158=DIRECTION('center_axis',(0.,0.,-1.));
#114159=DIRECTION('ref_axis',(0.,1.,0.));
#114160=DIRECTION('center_axis',(0.,0.,-1.));
#114161=DIRECTION('ref_axis',(-1.,0.,0.));
#114162=DIRECTION('center_axis',(-0.911656491798923,-0.41095308851605,5.08035184938228E-15));
#114163=DIRECTION('ref_axis',(0.41095308851605,-0.911656491798923,7.81754519040083E-31));
#114164=DIRECTION('center_axis',(-0.911086081553275,-0.412216147184822,
0.));
#114165=DIRECTION('ref_axis',(0.412216147184823,-0.911086081553275,0.));
#114166=DIRECTION('center_axis',(0.,0.,1.));
#114167=DIRECTION('ref_axis',(-1.,0.,0.));
#114168=DIRECTION('center_axis',(0.,0.,-1.));
#114169=DIRECTION('ref_axis',(-1.,0.,0.));
#114170=DIRECTION('center_axis',(0.,0.,-1.));
#114171=DIRECTION('ref_axis',(0.,1.,0.));
#114172=DIRECTION('',(0.,-1.23467863058847E-16,1.));
#114173=DIRECTION('center_axis',(0.,-1.23467863058847E-16,1.));
#114174=DIRECTION('ref_axis',(0.,-1.,-1.21694324257719E-16));
#114175=DIRECTION('center_axis',(0.,-1.18842113532929E-16,1.));
#114176=DIRECTION('ref_axis',(0.,-1.,-1.18842113532929E-16));
#114177=DIRECTION('center_axis',(0.,0.,-1.));
#114178=DIRECTION('ref_axis',(0.,1.,0.));
#114179=DIRECTION('',(0.,1.23467863058847E-16,-1.));
#114180=DIRECTION('center_axis',(0.,0.,-1.));
#114181=DIRECTION('ref_axis',(-1.,0.,0.));
#114182=DIRECTION('center_axis',(-0.959694777166788,-0.28104436425374,-1.95400042656926E-13));
#114183=DIRECTION('ref_axis',(0.28104436425374,-0.959694777166788,-3.56742184214581E-30));
#114184=DIRECTION('center_axis',(0.,0.,-1.));
#114185=DIRECTION('ref_axis',(-1.,0.,0.));
#114186=DIRECTION('center_axis',(-0.962140601075499,-0.272553597962085,
1.24636926569648E-14));
#114187=DIRECTION('ref_axis',(0.272553597962085,-0.962140601075499,-4.52904126028793E-31));
#114188=DIRECTION('center_axis',(0.,0.,1.));
#114189=DIRECTION('ref_axis',(-1.,0.,0.));
#114190=DIRECTION('center_axis',(0.,0.,-1.));
#114191=DIRECTION('ref_axis',(-1.,0.,0.));
#114192=DIRECTION('center_axis',(0.,0.,-1.));
#114193=DIRECTION('ref_axis',(0.,1.,0.));
#114194=DIRECTION('',(0.,-1.23467863058847E-16,1.));
#114195=DIRECTION('center_axis',(0.,-1.23467863058847E-16,1.));
#114196=DIRECTION('ref_axis',(0.,-1.,-1.21694324257719E-16));
#114197=DIRECTION('center_axis',(0.,-1.18842113532929E-16,1.));
#114198=DIRECTION('ref_axis',(0.,-1.,-1.18842113532929E-16));
#114199=DIRECTION('center_axis',(0.,0.,-1.));
#114200=DIRECTION('ref_axis',(0.,1.,0.));
#114201=DIRECTION('',(0.,1.23467863058847E-16,-1.));
#114202=DIRECTION('center_axis',(0.,1.38777878078144E-14,-1.));
#114203=DIRECTION('ref_axis',(0.,1.,1.38777878078144E-14));
#114204=DIRECTION('center_axis',(-0.989538255790606,-0.14315195982541,-0.0179320028170335));
#114205=DIRECTION('ref_axis',(0.143174981115239,-0.989697390510176,-2.48873089681965E-18));
#114206=DIRECTION('center_axis',(-0.99074835547853,-0.134685218959648,-0.0166609696710313));
#114207=DIRECTION('ref_axis',(0.13470391634661,-0.99088589399632,2.11341644556228E-18));
#114208=DIRECTION('center_axis',(0.0035180468195045,-0.149207652782241,
0.988799625656174));
#114209=DIRECTION('ref_axis',(0.144246054961535,-0.978388820119922,-0.148149898050527));
#114210=DIRECTION('center_axis',(-5.55111512312579E-13,-6.5495003047383E-14,
-1.));
#114211=DIRECTION('ref_axis',(-1.,7.99467207819295E-41,5.55111512312579E-13));
#114212=DIRECTION('center_axis',(-5.55111512312579E-13,-6.5495003047383E-14,
-1.));
#114213=DIRECTION('ref_axis',(-1.,7.99467207819295E-41,5.55111512312579E-13));
#114214=DIRECTION('center_axis',(0.,0.,-1.));
#114215=DIRECTION('ref_axis',(0.,1.,0.));
#114216=DIRECTION('',(0.,-1.23467863058847E-16,1.));
#114217=DIRECTION('center_axis',(0.,-1.23467863058847E-16,1.));
#114218=DIRECTION('ref_axis',(0.,-1.,-1.21694324257719E-16));
#114219=DIRECTION('center_axis',(0.,-1.18842113532929E-16,1.));
#114220=DIRECTION('ref_axis',(0.,-1.,-1.18842113532929E-16));
#114221=DIRECTION('center_axis',(0.,0.,-1.));
#114222=DIRECTION('ref_axis',(0.,1.,0.));
#114223=DIRECTION('',(0.,1.23467863058847E-16,-1.));
#114224=DIRECTION('center_axis',(0.,1.38777878078144E-14,-1.));
#114225=DIRECTION('ref_axis',(0.,1.,1.38777878078144E-14));
#114226=DIRECTION('center_axis',(0.999990739418254,0.00427492665558239,
0.00049606433434234));
#114227=DIRECTION('ref_axis',(-0.00427492718156908,0.999990862457049,1.90763185875202E-22));
#114228=DIRECTION('center_axis',(0.,1.18842113532929E-16,-1.));
#114229=DIRECTION('ref_axis',(1.22464679914735E-16,-1.,-1.18842113532929E-16));
#114230=DIRECTION('center_axis',(0.,0.,1.));
#114231=DIRECTION('ref_axis',(-1.,0.,0.));
#114232=DIRECTION('center_axis',(7.9520675071357E-13,-0.116240704649149,
0.99322107236137));
#114233=DIRECTION('ref_axis',(0.00430412409636137,-0.993211872368101,-0.116239627936495));
#114234=DIRECTION('',(0.,-1.23467863058847E-16,1.));
#114235=DIRECTION('center_axis',(0.996194698091747,-0.0871557427476402,
-1.07609333103578E-17));
#114236=DIRECTION('ref_axis',(-4.87735489362744E-35,1.23467863058847E-16,
-1.));
#114237=DIRECTION('',(1.54660695142382E-33,-1.23467863058847E-16,1.));
#114238=DIRECTION('',(-0.0871557427476402,-0.996194698091747,0.));
#114239=DIRECTION('',(-1.54660695142382E-33,1.23467863058847E-16,-1.));
#114240=DIRECTION('center_axis',(0.,1.23467863058847E-16,-1.));
#114241=DIRECTION('ref_axis',(0.,1.,0.));
#114242=DIRECTION('center_axis',(-2.85576800769162E-31,-6.6052904065149E-46,
1.));
#114243=DIRECTION('ref_axis',(-2.31296463463574E-15,1.,3.11150763893057E-61));
#114244=DIRECTION('center_axis',(0.707106781186548,-0.707106781186547,-8.7304963227523E-17));
#114245=DIRECTION('ref_axis',(-2.16153073061992E-33,1.23467863058847E-16,
-1.));
#114246=DIRECTION('',(-1.23259516440783E-32,1.23467863058847E-16,-1.));
#114247=DIRECTION('',(-8.71576399210526E-33,-1.23467863058847E-16,1.));
#114248=DIRECTION('',(-0.707106781186547,-0.707106781186548,0.));
#114249=DIRECTION('center_axis',(1.35502005093696E-32,0.,-1.));
#114250=DIRECTION('ref_axis',(0.,1.,0.));
#114251=DIRECTION('center_axis',(-2.85576800769162E-31,-6.6052904065149E-46,
1.));
#114252=DIRECTION('ref_axis',(-2.31296463463574E-15,1.,3.11150763893057E-61));
#114253=DIRECTION('center_axis',(0.,1.23467863058847E-16,-1.));
#114254=DIRECTION('ref_axis',(0.,1.,0.));
#114255=DIRECTION('center_axis',(0.,0.,1.));
#114256=DIRECTION('ref_axis',(0.,1.,0.));
#114257=DIRECTION('center_axis',(0.0871557427476402,-0.996194698091747,
-1.22998030563942E-16));
#114258=DIRECTION('ref_axis',(1.53780943396195E-34,1.23467863058847E-16,
-1.));
#114259=DIRECTION('',(6.15711282612512E-33,-1.23467863058847E-16,1.));
#114260=DIRECTION('',(-0.996194698091747,-0.0871557427476402,0.));
#114261=DIRECTION('',(5.86299591403052E-36,1.23467863058847E-16,-1.));
#114262=DIRECTION('center_axis',(-5.61645494961161E-33,0.,-1.));
#114263=DIRECTION('ref_axis',(0.,1.,0.));
#114264=DIRECTION('center_axis',(0.,0.,1.));
#114265=DIRECTION('ref_axis',(0.,1.,0.));
#114266=DIRECTION('center_axis',(-0.970284356147939,-0.241967494127993,
1.34486472837252E-14));
#114267=DIRECTION('ref_axis',(0.241967494127993,-0.970284356147939,-2.62269727666659E-30));
#114268=DIRECTION('center_axis',(0.,0.,-1.));
#114269=DIRECTION('ref_axis',(-1.,0.,0.));
#114270=DIRECTION('center_axis',(0.,0.,-1.));
#114271=DIRECTION('ref_axis',(-1.,0.,0.));
#114272=DIRECTION('center_axis',(0.,0.,-1.));
#114273=DIRECTION('ref_axis',(0.,1.,0.));
#114274=DIRECTION('center_axis',(0.,0.,-1.));
#114275=DIRECTION('ref_axis',(0.,1.,0.));
#114276=DIRECTION('center_axis',(-7.4257679719932E-13,0.0392139963569502,
-0.999230835437797));
#114277=DIRECTION('ref_axis',(-0.00367973466771379,-0.9992240703987,-0.0392137308685247));
#114278=DIRECTION('center_axis',(0.,-1.,0.));
#114279=DIRECTION('ref_axis',(-0.00205411287980643,0.,0.999997890307913));
#114280=DIRECTION('center_axis',(-5.01606788234257E-16,-1.,5.70122241611331E-32));
#114281=DIRECTION('ref_axis',(-1.,5.01606788234257E-16,0.));
#114282=DIRECTION('center_axis',(0.,-1.,0.));
#114283=DIRECTION('ref_axis',(0.00228223725611616,0.,-0.999997395693162));
#114284=DIRECTION('center_axis',(-1.45825811553708E-13,0.0304934853273349,
0.999534965547775));
#114285=DIRECTION('ref_axis',(0.00367477153576914,-0.999528216691971,0.030493279435453));
#114286=DIRECTION('center_axis',(7.06462337057814E-14,0.115836593517192,
0.993268283799665));
#114287=DIRECTION('ref_axis',(0.00429820688470854,-0.993259108648899,0.115835523495903));
#114288=DIRECTION('center_axis',(0.,0.,1.));
#114289=DIRECTION('ref_axis',(0.,-1.,0.));
#114290=DIRECTION('center_axis',(0.,0.,1.));
#114291=DIRECTION('ref_axis',(0.,-1.,0.));
#114292=DIRECTION('center_axis',(0.,-1.23467863058847E-16,1.));
#114293=DIRECTION('ref_axis',(0.,-1.,0.));
#114294=DIRECTION('center_axis',(2.19322982990717E-31,3.89595880873225E-46,
-1.));
#114295=DIRECTION('ref_axis',(1.77635683940025E-15,-1.,-5.4451383681285E-61));
#114296=DIRECTION('center_axis',(0.,-1.23467863058847E-16,1.));
#114297=DIRECTION('ref_axis',(0.,-1.,-1.23467863058847E-16));
#114298=DIRECTION('center_axis',(2.19322982990717E-31,3.89595880873225E-46,
-1.));
#114299=DIRECTION('ref_axis',(1.77635683940025E-15,-1.,-5.4451383681285E-61));
#114300=DIRECTION('center_axis',(0.,-1.23467863058847E-16,1.));
#114301=DIRECTION('ref_axis',(1.22464679914735E-16,1.,0.));
#114302=DIRECTION('center_axis',(0.,0.,1.));
#114303=DIRECTION('ref_axis',(0.,-1.,0.));
#114304=DIRECTION('center_axis',(0.,0.,1.));
#114305=DIRECTION('ref_axis',(1.22464679914735E-16,1.,0.));
#114306=DIRECTION('center_axis',(0.,0.,-1.));
#114307=DIRECTION('ref_axis',(1.,-8.89601782552209E-16,0.));
#114308=DIRECTION('center_axis',(0.,0.,1.));
#114309=DIRECTION('ref_axis',(1.,0.,0.));
#114310=DIRECTION('center_axis',(0.,0.,1.));
#114311=DIRECTION('ref_axis',(1.,0.,0.));
#114312=DIRECTION('center_axis',(0.,0.,1.));
#114313=DIRECTION('ref_axis',(1.,0.,0.));
#114314=DIRECTION('',(-1.,0.,0.));
#114315=DIRECTION('center_axis',(0.,-1.,0.));
#114316=DIRECTION('ref_axis',(0.,0.,-1.));
#114317=DIRECTION('',(1.,0.,0.));
#114318=DIRECTION('center_axis',(0.,0.,-1.));
#114319=DIRECTION('ref_axis',(0.,-1.,0.));
#114320=DIRECTION('center_axis',(0.,0.,-1.));
#114321=DIRECTION('ref_axis',(-1.,0.,0.));
#114322=DIRECTION('center_axis',(0.,0.,-1.));
#114323=DIRECTION('ref_axis',(-1.,0.,0.));
#114324=DIRECTION('center_axis',(0.,0.,1.));
#114325=DIRECTION('ref_axis',(0.,-1.,0.));
#114326=DIRECTION('center_axis',(0.,-1.18842113532926E-16,1.));
#114327=DIRECTION('ref_axis',(0.,1.,1.18842113532926E-16));
#114328=DIRECTION('center_axis',(0.,1.19033121480991E-16,-1.));
#114329=DIRECTION('ref_axis',(0.,-1.,-1.19033121480991E-16));
#114330=DIRECTION('center_axis',(0.,-1.23467863058847E-16,1.));
#114331=DIRECTION('ref_axis',(-1.22464679914735E-16,1.,1.21694324257719E-16));
#114332=DIRECTION('center_axis',(0.,-1.18842113532929E-16,1.));
#114333=DIRECTION('ref_axis',(0.,-1.,-1.18842113532929E-16));
#114334=DIRECTION('center_axis',(0.,1.18842113532929E-16,-1.));
#114335=DIRECTION('ref_axis',(0.,1.,1.18842113532929E-16));
#114336=DIRECTION('center_axis',(0.,0.,1.));
#114337=DIRECTION('ref_axis',(-1.,1.78263170299393E-15,0.));
#114338=DIRECTION('center_axis',(0.,0.,-1.));
#114339=DIRECTION('ref_axis',(0.,1.,0.));
#114340=DIRECTION('center_axis',(0.,0.,-1.));
#114341=DIRECTION('ref_axis',(0.,1.,0.));
#114342=DIRECTION('center_axis',(0.,0.,-1.));
#114343=DIRECTION('ref_axis',(0.,-1.,0.));
#114344=DIRECTION('center_axis',(-0.5,0.866025403784438,1.0692630595994E-16));
#114345=DIRECTION('ref_axis',(2.13852611919879E-16,5.48307457472744E-35,
1.));
#114346=DIRECTION('',(0.,1.23467863058847E-16,-1.));
#114347=DIRECTION('',(0.,1.23467863058847E-16,-1.));
#114348=DIRECTION('center_axis',(-1.,0.,0.));
#114349=DIRECTION('ref_axis',(0.,0.,1.));
#114350=DIRECTION('',(0.,1.23467863058847E-16,-1.));
#114351=DIRECTION('center_axis',(-0.5,-0.866025403784439,-1.0692630595994E-16));
#114352=DIRECTION('ref_axis',(-0.866025403784439,0.5,-9.26929360883051E-34));
#114353=DIRECTION('',(0.,1.23467863058847E-16,-1.));
#114354=DIRECTION('center_axis',(0.5,-0.866025403784439,-1.0692630595994E-16));
#114355=DIRECTION('ref_axis',(-4.5474696259435E-34,1.23467863058847E-16,
-1.));
#114356=DIRECTION('',(0.,1.23467863058847E-16,-1.));
#114357=DIRECTION('center_axis',(1.,0.,0.));
#114358=DIRECTION('ref_axis',(0.,1.,0.));
#114359=DIRECTION('',(0.,1.23467863058847E-16,-1.));
#114360=DIRECTION('center_axis',(0.5,0.866025403784439,1.0692630595994E-16));
#114361=DIRECTION('ref_axis',(2.1385261191988E-16,-4.09037363277686E-33,
-1.));
#114362=DIRECTION('center_axis',(0.,0.,-1.));
#114363=DIRECTION('ref_axis',(0.,1.,0.));
#114364=DIRECTION('',(-1.06057523872491E-16,-0.866025403784439,-0.5));
#114365=DIRECTION('center_axis',(0.,0.,-1.));
#114366=DIRECTION('ref_axis',(0.,1.,0.));
#114367=DIRECTION('center_axis',(0.,0.,-1.));
#114368=DIRECTION('ref_axis',(0.,1.,0.));
#114369=DIRECTION('center_axis',(0.,0.,-1.));
#114370=DIRECTION('ref_axis',(0.,1.,0.));
#114371=DIRECTION('center_axis',(0.,0.,-1.));
#114372=DIRECTION('ref_axis',(0.,1.,0.));
#114373=DIRECTION('center_axis',(0.,0.,-1.));
#114374=DIRECTION('ref_axis',(0.,1.,0.));
#114375=DIRECTION('center_axis',(0.,0.,-1.));
#114376=DIRECTION('ref_axis',(0.,1.,0.));
#114377=DIRECTION('center_axis',(0.,0.,-1.));
#114378=DIRECTION('ref_axis',(0.,1.,0.));
#114379=DIRECTION('center_axis',(0.,0.,-1.));
#114380=DIRECTION('ref_axis',(0.,1.,0.));
#114381=DIRECTION('center_axis',(0.,0.,-1.));
#114382=DIRECTION('ref_axis',(0.,1.,0.));
#114383=DIRECTION('center_axis',(0.,0.,-1.));
#114384=DIRECTION('ref_axis',(0.,1.,0.));
#114385=DIRECTION('center_axis',(0.,0.,-1.));
#114386=DIRECTION('ref_axis',(0.,1.,0.));
#114387=DIRECTION('center_axis',(0.,0.,-1.));
#114388=DIRECTION('ref_axis',(0.,1.,0.));
#114389=DIRECTION('center_axis',(0.,1.23467863058847E-16,-1.));
#114390=DIRECTION('ref_axis',(0.,1.,0.));
#114391=DIRECTION('center_axis',(0.,0.,-1.));
#114392=DIRECTION('ref_axis',(0.,1.,0.));
#114393=DIRECTION('center_axis',(-1.,0.,0.));
#114394=DIRECTION('ref_axis',(0.,-1.,0.));
#114395=DIRECTION('center_axis',(0.,0.,1.));
#114396=DIRECTION('ref_axis',(0.,1.,0.));
#114397=DIRECTION('center_axis',(0.,0.,1.));
#114398=DIRECTION('ref_axis',(0.,1.,0.));
#114399=DIRECTION('center_axis',(0.,1.23467863058847E-16,-1.));
#114400=DIRECTION('ref_axis',(-1.,0.,0.));
#114401=DIRECTION('center_axis',(0.,0.,-1.));
#114402=DIRECTION('ref_axis',(0.,1.,0.));
#114403=DIRECTION('center_axis',(0.,1.23467863058847E-16,-1.));
#114404=DIRECTION('ref_axis',(-1.,0.,0.));
#114405=DIRECTION('center_axis',(0.,0.,1.));
#114406=DIRECTION('ref_axis',(0.,-1.,0.));
#114407=DIRECTION('',(0.,0.,-1.));
#114408=DIRECTION('center_axis',(0.,0.,-1.));
#114409=DIRECTION('ref_axis',(-1.,0.,0.));
#114410=DIRECTION('center_axis',(0.,0.,-1.));
#114411=DIRECTION('ref_axis',(1.,0.,0.));
#114412=DIRECTION('',(-0.707106781186552,8.65956056235499E-17,0.707106781186543));
#114413=DIRECTION('center_axis',(0.,0.,1.));
#114414=DIRECTION('ref_axis',(1.,0.,0.));
#114415=DIRECTION('center_axis',(0.,0.,1.));
#114416=DIRECTION('ref_axis',(1.,0.,0.));
#114417=DIRECTION('center_axis',(0.,0.,-1.));
#114418=DIRECTION('ref_axis',(-1.,0.,0.));
#114419=DIRECTION('center_axis',(0.,0.,1.));
#114420=DIRECTION('ref_axis',(1.,0.,0.));
#114421=DIRECTION('',(0.,0.,1.));
#114422=DIRECTION('center_axis',(0.,1.23467863058847E-16,-1.));
#114423=DIRECTION('ref_axis',(-1.,0.,0.));
#114424=DIRECTION('center_axis',(0.,0.,-1.));
#114425=DIRECTION('ref_axis',(0.,1.,0.));
#114426=DIRECTION('center_axis',(0.,0.,-1.));
#114427=DIRECTION('ref_axis',(-1.,0.,0.));
#114428=DIRECTION('center_axis',(0.,0.,1.));
#114429=DIRECTION('ref_axis',(1.,0.,0.));
#114430=DIRECTION('',(0.,0.,1.));
#114431=DIRECTION('center_axis',(0.,0.,1.));
#114432=DIRECTION('ref_axis',(1.,0.,0.));
#114433=DIRECTION('center_axis',(-0.592966514233392,-0.805227118891249,
0.));
#114434=DIRECTION('ref_axis',(0.805227118891249,-0.592966514233392,0.));
#114435=DIRECTION('center_axis',(0.807208114890536,0.590266938981735,-2.28940150095415E-14));
#114436=DIRECTION('ref_axis',(-0.590266938981735,0.807208114890536,-1.47426480814321E-30));
#114437=DIRECTION('center_axis',(0.,-1.23467863058847E-16,1.));
#114438=DIRECTION('ref_axis',(0.,-1.,0.));
#114439=DIRECTION('center_axis',(0.,0.,-1.));
#114440=DIRECTION('ref_axis',(0.,-1.,0.));
#114441=DIRECTION('center_axis',(-1.,0.,0.));
#114442=DIRECTION('ref_axis',(0.,1.,0.));
#114443=DIRECTION('center_axis',(0.,0.,1.));
#114444=DIRECTION('ref_axis',(0.,1.,0.));
#114445=DIRECTION('center_axis',(0.,0.,1.));
#114446=DIRECTION('ref_axis',(0.,1.,0.));
#114447=DIRECTION('center_axis',(-0.168369768252295,0.882882757183484,-0.438371598312161));
#114448=DIRECTION('ref_axis',(-2.05714353600353E-15,-0.444720469017533,
-0.895669416937313));
#114449=DIRECTION('center_axis',(-0.507675385487887,-0.517400512911953,
0.688884904906599));
#114450=DIRECTION('ref_axis',(-1.34605780150592E-16,0.799589295572927,0.600547215800049));
#114451=DIRECTION('center_axis',(-0.506894799267393,-0.516604973631544,
0.690055768539632));
#114452=DIRECTION('ref_axis',(-4.2861068992561E-17,0.800521374177574,0.599304204461181));
#114453=DIRECTION('center_axis',(0.,0.,1.));
#114454=DIRECTION('ref_axis',(1.,0.,0.));
#114455=DIRECTION('center_axis',(-0.663838127753914,0.747876286654537,9.2338686945498E-17));
#114456=DIRECTION('ref_axis',(0.747876286654537,0.663838127753914,1.66533453693772E-13));
#114457=DIRECTION('center_axis',(-0.187328576766759,0.982297309538482,0.));
#114458=DIRECTION('ref_axis',(-0.982297309538482,-0.187328576766759,0.));
#114459=DIRECTION('center_axis',(-0.668574108837973,0.743645521059268,0.));
#114460=DIRECTION('ref_axis',(-0.743645521059268,-0.668574108837973,0.));
#114461=DIRECTION('center_axis',(0.,-1.23467863058847E-16,1.));
#114462=DIRECTION('ref_axis',(0.,-1.,0.));
#114463=DIRECTION('center_axis',(-0.679956281045645,0.733252654865004,0.));
#114464=DIRECTION('ref_axis',(-0.733252654865004,-0.679956281045645,0.));
#114465=DIRECTION('center_axis',(0.,0.,-1.));
#114466=DIRECTION('ref_axis',(0.,-1.,0.));
#114467=DIRECTION('center_axis',(5.71153601538328E-31,-2.64211616260599E-45,
1.));
#114468=DIRECTION('ref_axis',(-4.6259292692715E-15,-1.,-3.11150763893057E-61));
#114469=DIRECTION('center_axis',(-0.775870249713592,0.63089250717485,-1.27793330397298E-14));
#114470=DIRECTION('ref_axis',(-0.63089250717485,-0.775870249713592,-7.13011169472736E-30));
#114471=DIRECTION('center_axis',(0.,-1.23467863058847E-16,1.));
#114472=DIRECTION('ref_axis',(0.,-1.,0.));
#114473=DIRECTION('center_axis',(-0.746021307914873,0.665922073621968,0.));
#114474=DIRECTION('ref_axis',(-0.665922073621968,-0.746021307914873,0.));
#114475=DIRECTION('center_axis',(0.,0.,-1.));
#114476=DIRECTION('ref_axis',(0.,-1.,0.));
#114477=DIRECTION('center_axis',(2.41254715360152E-30,-4.7140880421464E-44,
1.));
#114478=DIRECTION('ref_axis',(-1.95398793972133E-14,-1.,1.49352366668667E-58));
#114479=DIRECTION('center_axis',(0.507468854451513,0.517190025527329,-0.68919506618715));
#114480=DIRECTION('ref_axis',(-1.08020880515219E-16,-0.799836347973839,
-0.600218140728745));
#114481=DIRECTION('center_axis',(0.,-1.23467863058847E-16,1.));
#114482=DIRECTION('ref_axis',(0.,-1.,0.));
#114483=DIRECTION('center_axis',(-0.923323390669864,0.38402332773141,-1.28136860937081E-14));
#114484=DIRECTION('ref_axis',(-0.38402332773141,-0.923323390669864,2.90201745723254E-30));
#114485=DIRECTION('center_axis',(0.,0.,-1.));
#114486=DIRECTION('ref_axis',(0.,-1.,0.));
#114487=DIRECTION('center_axis',(-6.28268961692158E-30,-3.19696055675322E-43,
1.));
#114488=DIRECTION('ref_axis',(5.08852219619863E-14,-1.,-2.38963786669868E-58));
#114489=DIRECTION('center_axis',(0.511561679834273,0.521361253861094,-0.682998602266158));
#114490=DIRECTION('ref_axis',(1.21631079100244E-16,-0.79488081246627,-0.606765600518819));
#114491=DIRECTION('center_axis',(-0.987526870499689,0.134244619791538,-0.0822743100737742));
#114492=DIRECTION('ref_axis',(-0.134701294632915,-0.990886250396188,-7.62230551969098E-18));
#114493=DIRECTION('center_axis',(0.887573437172827,-0.12065692809958,-0.444584411925099));
#114494=DIRECTION('ref_axis',(-0.447856331161543,-5.04904183848934E-18,
-0.89410553439654));
#114495=DIRECTION('center_axis',(0.502571259550305,0.589216419045832,0.632650093338194));
#114496=DIRECTION('ref_axis',(-0.234843565694733,-0.611220822461641,0.755815854452061));
#114497=DIRECTION('center_axis',(0.,0.,1.));
#114498=DIRECTION('ref_axis',(1.,0.,0.));
#114499=DIRECTION('center_axis',(0.606371999687993,-0.771616335224111,0.192148976603301));
#114500=DIRECTION('ref_axis',(0.786267832350933,0.617885827487704,-3.1641897774151E-17));
#114501=DIRECTION('center_axis',(-0.645804421056786,-0.763502881293522,
-1.01980482580395E-14));
#114502=DIRECTION('ref_axis',(0.763502881293522,-0.645804421056786,-6.9816295225584E-30));
#114503=DIRECTION('center_axis',(0.48724015249101,-0.488874385354372,-0.723601319197887));
#114504=DIRECTION('ref_axis',(-1.47352524967685E-15,-0.828613098245121,
0.559821697879442));
#114505=DIRECTION('center_axis',(0.488418020654004,-0.490056204158282,-0.722006062208899));
#114506=DIRECTION('ref_axis',(3.20373038523992E-15,-0.827409999881363,0.561598336977882));
#114507=DIRECTION('center_axis',(-0.753146254930614,-0.657853113304171,
-3.00335537434998E-14));
#114508=DIRECTION('ref_axis',(0.657853113304171,-0.753146254930614,-2.96993835591878E-30));
#114509=DIRECTION('center_axis',(-0.171101227036283,-0.869601781127171,
-0.463159920942141));
#114510=DIRECTION('ref_axis',(-4.21773228904835E-17,-0.470092156192753,
0.882617337630554));
#114511=DIRECTION('center_axis',(0.484433158250521,-0.486057976285942,-0.727373465886845));
#114512=DIRECTION('ref_axis',(-3.34045680200078E-15,-0.831447136037245,
0.555603869654868));
#114513=DIRECTION('center_axis',(1.,0.,0.));
#114514=DIRECTION('ref_axis',(0.,-1.,0.));
#114515=DIRECTION('center_axis',(-0.193053842425666,-0.981173356447606,
0.00539059570228739));
#114516=DIRECTION('ref_axis',(0.981187612482096,-0.193056647416463,-1.03740416739262E-18));
#114517=DIRECTION('center_axis',(-0.663957144707683,-0.747700087626819,
0.0102707815899847));
#114518=DIRECTION('ref_axis',(0.747739527797473,-0.663992167551103,3.3311423852743E-19));
#114519=DIRECTION('center_axis',(0.485576620175616,-0.487205273451398,-0.725841833638689));
#114520=DIRECTION('ref_axis',(1.3020744827461E-16,-0.830298240911906,0.557319326004935));
#114521=DIRECTION('center_axis',(-0.210025631952355,-0.977695880078777,
0.));
#114522=DIRECTION('ref_axis',(0.977695880078777,-0.210025631952355,0.));
#114523=DIRECTION('center_axis',(0.869253009153379,0.170328745809824,-0.464098399510975));
#114524=DIRECTION('ref_axis',(-0.470980702241858,8.1123542202202E-17,-0.882143513333157));
#114525=DIRECTION('center_axis',(0.,1.23467863058847E-16,-1.));
#114526=DIRECTION('ref_axis',(0.,1.,0.));
#114527=DIRECTION('center_axis',(-0.67420688908099,-0.738542531419643,0.));
#114528=DIRECTION('ref_axis',(0.738542531419643,-0.67420688908099,0.));
#114529=DIRECTION('center_axis',(0.,0.,1.));
#114530=DIRECTION('ref_axis',(0.,1.,0.));
#114531=DIRECTION('center_axis',(-4.28365201153744E-31,1.48619034146585E-45,
-1.));
#114532=DIRECTION('ref_axis',(3.46944695195361E-15,1.,1.24460305557223E-60));
#114533=DIRECTION('center_axis',(1.,0.,0.));
#114534=DIRECTION('ref_axis',(0.,-1.,0.));
#114535=DIRECTION('center_axis',(0.752788125817861,0.658228853504028,0.00669432912290745));
#114536=DIRECTION('ref_axis',(0.658243602947644,-0.752804994124312,-1.11021690861332E-13));
#114537=DIRECTION('center_axis',(0.981331609270135,0.192290369398073,0.00356180909645361));
#114538=DIRECTION('ref_axis',(-0.192291589154029,0.981337834153263,-1.28820063606849E-18));
#114539=DIRECTION('center_axis',(0.,1.23467863058847E-16,-1.));
#114540=DIRECTION('ref_axis',(0.,1.,0.));
#114541=DIRECTION('center_axis',(-0.74079592940915,-0.671730147433353,0.));
#114542=DIRECTION('ref_axis',(0.671730147433353,-0.74079592940915,0.));
#114543=DIRECTION('center_axis',(0.,0.,1.));
#114544=DIRECTION('ref_axis',(0.,1.,0.));
#114545=DIRECTION('center_axis',(-1.64492525510334E-30,2.19148451090235E-44,
-1.));
#114546=DIRECTION('ref_axis',(1.33226996430588E-14,1.,1.74244427780112E-59));
#114547=DIRECTION('center_axis',(0.979119873047182,0.203283728330798,0.));
#114548=DIRECTION('ref_axis',(-0.203283728330798,0.979119873047182,0.));
#114549=DIRECTION('center_axis',(0.,1.23467863058847E-16,-1.));
#114550=DIRECTION('ref_axis',(0.,1.,0.));
#114551=DIRECTION('center_axis',(-2.57019120692247E-30,5.35028522927707E-44,
-1.));
#114552=DIRECTION('ref_axis',(2.08166817117217E-14,1.,-1.99136488891557E-59));
#114553=DIRECTION('center_axis',(0.,0.,1.));
#114554=DIRECTION('ref_axis',(0.,1.,0.));
#114555=DIRECTION('center_axis',(0.,-1.23467863058847E-16,1.));
#114556=DIRECTION('ref_axis',(0.,-1.,0.));
#114557=DIRECTION('center_axis',(0.777162624242377,0.629299813666508,0.));
#114558=DIRECTION('ref_axis',(-0.629299813666508,0.777162624242377,0.));
#114559=DIRECTION('center_axis',(0.,0.,-1.));
#114560=DIRECTION('ref_axis',(0.,-1.,0.));
#114561=DIRECTION('center_axis',(0.982297019165463,0.187330099393145,0.));
#114562=DIRECTION('ref_axis',(-0.187330099393145,0.982297019165463,0.));
#114563=DIRECTION('center_axis',(4.46763300492346E-31,-1.61659432440069E-45,
1.));
#114564=DIRECTION('ref_axis',(-3.61845819166247E-15,-1.,1.86690458335834E-60));
#114565=DIRECTION('center_axis',(0.,-1.23467863058847E-16,1.));
#114566=DIRECTION('ref_axis',(0.,-1.,0.));
#114567=DIRECTION('center_axis',(0.635030358342585,0.772487180465338,0.));
#114568=DIRECTION('ref_axis',(-0.772487180465338,0.635030358342585,0.));
#114569=DIRECTION('center_axis',(0.,0.,-1.));
#114570=DIRECTION('ref_axis',(0.,-1.,0.));
#114571=DIRECTION('center_axis',(1.09661491495359E-30,-9.73989702183063E-45,
1.));
#114572=DIRECTION('ref_axis',(-8.88178419700125E-15,-1.,2.48920611114446E-60));
#114573=DIRECTION('center_axis',(0.,-1.23467863058847E-16,1.));
#114574=DIRECTION('ref_axis',(0.,-1.,0.));
#114575=DIRECTION('center_axis',(0.0394959395290733,0.999219730970479,0.));
#114576=DIRECTION('ref_axis',(-0.999219730970479,0.0394959395290733,0.));
#114577=DIRECTION('center_axis',(0.,0.,-1.));
#114578=DIRECTION('ref_axis',(0.,-1.,0.));
#114579=DIRECTION('center_axis',(6.70144950738521E-31,-3.63733722990157E-45,
1.));
#114580=DIRECTION('ref_axis',(-5.42768728749372E-15,-1.,2.48920611114446E-60));
#114581=DIRECTION('center_axis',(0.,-1.23467863058847E-16,1.));
#114582=DIRECTION('ref_axis',(0.,-1.,-1.33055111034894E-16));
#114583=DIRECTION('center_axis',(-0.0394959395290663,0.999219730970479,
0.));
#114584=DIRECTION('ref_axis',(-0.999219730970479,-0.0394959395290663,0.));
#114585=DIRECTION('center_axis',(0.,1.29997489681772E-16,-1.));
#114586=DIRECTION('ref_axis',(0.,-1.,-1.29997489681772E-16));
#114587=DIRECTION('center_axis',(0.,-1.30058395245648E-16,1.));
#114588=DIRECTION('ref_axis',(0.,-1.,-1.30058395245648E-16));
#114589=DIRECTION('center_axis',(0.,-1.23467863058847E-16,1.));
#114590=DIRECTION('ref_axis',(0.,-1.,0.));
#114591=DIRECTION('center_axis',(-0.635030358342616,0.772487180465313,0.));
#114592=DIRECTION('ref_axis',(-0.772487180465313,-0.635030358342616,0.));
#114593=DIRECTION('center_axis',(0.,0.,-1.));
#114594=DIRECTION('ref_axis',(0.,-1.,0.));
#114595=DIRECTION('center_axis',(-5.21223850574408E-31,-2.20036449710098E-45,
1.));
#114596=DIRECTION('ref_axis',(4.22153455693958E-15,-1.,-9.33452291679171E-61));
#114597=DIRECTION('center_axis',(0.,-1.23467863058847E-16,1.));
#114598=DIRECTION('ref_axis',(0.,-1.,0.));
#114599=DIRECTION('center_axis',(-0.774287490710421,0.632834008037937,0.));
#114600=DIRECTION('ref_axis',(-0.632834008037937,-0.774287490710421,0.));
#114601=DIRECTION('center_axis',(0.,0.,-1.));
#114602=DIRECTION('ref_axis',(0.,-1.,0.));
#114603=DIRECTION('center_axis',(0.,0.,1.));
#114604=DIRECTION('ref_axis',(0.,-1.,0.));
#114605=DIRECTION('center_axis',(0.,-1.23467863058847E-16,1.));
#114606=DIRECTION('ref_axis',(0.,-1.,0.));
#114607=DIRECTION('center_axis',(-0.999225121087074,0.0393593367388477,
0.));
#114608=DIRECTION('ref_axis',(-0.0393593367388477,-0.999225121087074,0.));
#114609=DIRECTION('center_axis',(0.,0.,-1.));
#114610=DIRECTION('ref_axis',(0.,-1.,0.));
#114611=DIRECTION('center_axis',(5.21223850574404E-31,-2.20036449710094E-45,
1.));
#114612=DIRECTION('ref_axis',(-4.22153455693955E-15,-1.,2.48920611114446E-60));
#114613=DIRECTION('center_axis',(0.,0.,-1.));
#114614=DIRECTION('ref_axis',(-0.751703367637011,-0.659501362457407,0.));
#114615=DIRECTION('center_axis',(0.659496851377394,-0.751707325375577,0.));
#114616=DIRECTION('ref_axis',(0.751707325375577,0.659496851377394,0.));
#114617=DIRECTION('center_axis',(-0.00318935089126825,-0.00297677156874421,
0.999990483390677));
#114618=DIRECTION('ref_axis',(-0.747789842767528,-0.663921177326532,-0.0043613473913037));
#114619=DIRECTION('center_axis',(0.657034976183429,-0.753860093168249,1.01740733956786E-14));
#114620=DIRECTION('ref_axis',(0.753860093168249,0.657034976183429,-8.45764823615526E-31));
#114621=DIRECTION('center_axis',(-0.00280476608066071,-0.00263885430337773,
0.999992584840107));
#114622=DIRECTION('ref_axis',(0.937191712771117,-0.348810515489431,0.00170815606344439));
#114623=DIRECTION('center_axis',(0.768895279480121,0.207195498703726,-0.604871948853723));
#114624=DIRECTION('ref_axis',(-0.618289095466814,1.21523947502978E-17,-0.785950758271044));
#114625=DIRECTION('center_axis',(0.202724571193613,0.760898522337225,-0.616389638896853));
#114626=DIRECTION('ref_axis',(-1.87348493224475E-17,-0.629459870756021,
-0.777032992290426));
#114627=DIRECTION('center_axis',(0.767736348840716,0.206883199723352,-0.606448876939313));
#114628=DIRECTION('ref_axis',(-0.619859127336644,-1.17584790122141E-16,
-0.784713108248775));
#114629=DIRECTION('center_axis',(0.260190354028299,-0.965557341472079,1.40549396816343E-10));
#114630=DIRECTION('ref_axis',(-0.58403426831887,-0.15738069260472,-0.796326121023605));
#114631=DIRECTION('center_axis',(-0.243334995703589,0.96954396966785,0.0277951568918529));
#114632=DIRECTION('ref_axis',(-0.594809401908895,-0.126526334687349,-0.793846875682815));
#114633=DIRECTION('center_axis',(0.202457297762738,0.759895348634851,-0.617713608159743));
#114634=DIRECTION('ref_axis',(5.55058625584594E-17,-0.630776296546234,-0.775964730973913));
#114635=DIRECTION('center_axis',(0.966468863382725,-0.256741605888852,0.00465659932972454));
#114636=DIRECTION('ref_axis',(-0.154910761359747,-0.597411475844062,-0.786830467473625));
#114637=DIRECTION('center_axis',(-0.966292363520655,0.25744721439873,-4.29897349204163E-11));
#114638=DIRECTION('ref_axis',(-0.159028116924834,-0.596889950284185,-0.786404759190256));
#114639=DIRECTION('center_axis',(0.578576029254642,0.155909851599689,-0.800588468906525));
#114640=DIRECTION('ref_axis',(-0.810499837678775,1.21842170142303E-15,-0.585738860860947));
#114641=DIRECTION('center_axis',(0.153941565569776,0.577798286012631,-0.801530495409122));
#114642=DIRECTION('ref_axis',(-1.29290181198153E-17,-0.811200037627138,
-0.584768756820788));
#114643=DIRECTION('center_axis',(0.0544019837731304,-0.025960154057113,
-0.998181593981215));
#114644=DIRECTION('ref_axis',(-0.998518116145471,-1.61274188638027E-18,
-0.054420324597515));
#114645=DIRECTION('center_axis',(-0.025995718416376,0.0542003143889016,
-0.998191639187667));
#114646=DIRECTION('ref_axis',(1.6064497712818E-18,-0.99852908789078,-0.0542186373492239));
#114647=DIRECTION('center_axis',(0.734334158412678,-0.678788143523695,2.48736119588291E-13));
#114648=DIRECTION('ref_axis',(0.678788143523695,0.734334158412678,-6.81231552358944E-29));
#114649=DIRECTION('center_axis',(-0.680870844883917,0.73240350394237,1.91708814121709E-12));
#114650=DIRECTION('ref_axis',(-0.73240350394237,-0.680870844883917,-1.31317411609931E-27));
#114651=DIRECTION('center_axis',(0.,-1.23467863058847E-16,1.));
#114652=DIRECTION('ref_axis',(0.,-1.,0.));
#114653=DIRECTION('center_axis',(0.,0.,-1.));
#114654=DIRECTION('ref_axis',(0.,1.,0.));
#114655=DIRECTION('center_axis',(-9.86953423458227E-31,-7.88931658768281E-45,
1.));
#114656=DIRECTION('ref_axis',(7.99360577730113E-15,-1.,2.48920611114446E-60));
#114657=DIRECTION('center_axis',(0.0255375237255525,0.0535186253292443,
0.998240247447895));
#114658=DIRECTION('ref_axis',(-2.96412751937958E-19,0.998565915482956,-0.0535360853601283));
#114659=DIRECTION('center_axis',(-0.682537484892591,-0.730850587819765,
8.37209378123771E-13));
#114660=DIRECTION('ref_axis',(0.730850587819765,-0.682537484892591,3.92323810141884E-28));
#114661=DIRECTION('center_axis',(0.,-1.23467863058847E-16,1.));
#114662=DIRECTION('ref_axis',(0.,-1.,0.));
#114663=DIRECTION('center_axis',(-0.735878524541007,-0.677113577710085,
5.64206319996869E-13));
#114664=DIRECTION('ref_axis',(0.677113577710085,-0.735878524541007,-1.38055872491966E-28));
#114665=DIRECTION('center_axis',(0.,0.,1.));
#114666=DIRECTION('ref_axis',(0.,-1.,0.));
#114667=DIRECTION('center_axis',(5.92172054074936E-30,2.84015397156581E-43,
-1.));
#114668=DIRECTION('ref_axis',(-4.79616346638068E-14,1.,-2.78791084448179E-58));
#114669=DIRECTION('center_axis',(-0.152544532818274,0.577842847451632,0.801765432752152));
#114670=DIRECTION('ref_axis',(4.14384419008336E-17,0.811259933931047,-0.58468565879299));
#114671=DIRECTION('center_axis',(-0.0536778879072088,-0.0251150971461135,
0.998242413567548));
#114672=DIRECTION('ref_axis',(0.998557392321894,-9.29874389531901E-20,0.0536948250700053));
#114673=DIRECTION('center_axis',(-0.19315692461333,0.731683694333232,0.653704347485004));
#114674=DIRECTION('ref_axis',(-3.51224977473848E-17,0.66625127354731,-0.745727323152764));
#114675=DIRECTION('center_axis',(-0.576537673896198,0.156770156178271,0.801889910592596));
#114676=DIRECTION('ref_axis',(0.811929324239482,3.97972821433516E-17,0.583755747243673));
#114677=DIRECTION('center_axis',(-0.193538145022295,0.733127767631913,0.651971366509586));
#114678=DIRECTION('ref_axis',(1.09087611421558E-16,0.664535912353125,-0.747256328974871));
#114679=DIRECTION('center_axis',(0.967398007177023,0.253182433216653,0.00630485689132568));
#114680=DIRECTION('ref_axis',(-0.16111421782421,0.634435934472465,-0.755998183770929));
#114681=DIRECTION('center_axis',(-0.966876318105823,-0.255245343710962,
-5.9860823738661E-11));
#114682=DIRECTION('ref_axis',(-0.166411982471238,0.630373124957365,-0.758245854206588));
#114683=DIRECTION('center_axis',(-0.72784499809572,0.197913127261801,0.656560776169652));
#114684=DIRECTION('ref_axis',(0.669809908048189,2.97308687105849E-17,0.742532616846207));
#114685=DIRECTION('center_axis',(-0.72888212476865,0.19819513920631,0.655323992379136));
#114686=DIRECTION('ref_axis',(0.668587032943078,1.18015531912611E-16,0.743633901446385));
#114687=DIRECTION('center_axis',(0.262389207131878,0.964962125671627,-2.3868460211661E-11));
#114688=DIRECTION('ref_axis',(-0.633554268004896,0.172273913779853,-0.754274941996453));
#114689=DIRECTION('center_axis',(-0.257377402244523,-0.96626185396935,0.00974178513293261));
#114690=DIRECTION('ref_axis',(-0.635976884577247,0.161793976065296,-0.754556897518273));
#114691=DIRECTION('center_axis',(0.70592193778968,-0.708289642552581,-8.74510085926821E-17));
#114692=DIRECTION('ref_axis',(-0.708289642552581,-0.70592193778968,-3.19694546253078E-33));
#114693=DIRECTION('',(-0.70592193778968,0.708289642552581,8.74510085926821E-17));
#114694=DIRECTION('center_axis',(-0.705921937789676,0.708289642552585,-6.53108990768421E-15));
#114695=DIRECTION('ref_axis',(-0.708289642552585,-0.705921937789676,-2.24639971032546E-30));
#114696=DIRECTION('',(0.70592193778968,-0.708289642552581,-8.74510085926821E-17));
#114697=DIRECTION('center_axis',(0.,0.,-1.));
#114698=DIRECTION('ref_axis',(0.,1.,0.));
#114699=DIRECTION('center_axis',(0.,0.,1.));
#114700=DIRECTION('ref_axis',(0.,1.,0.));
#114701=DIRECTION('center_axis',(-0.74079592940915,-0.671730147433353,0.));
#114702=DIRECTION('ref_axis',(0.671730147433353,-0.74079592940915,0.));
#114703=DIRECTION('center_axis',(0.,1.23467863058847E-16,-1.));
#114704=DIRECTION('ref_axis',(0.,1.,0.));
#114705=DIRECTION('center_axis',(0.,0.,1.));
#114706=DIRECTION('ref_axis',(0.,1.,0.));
#114707=DIRECTION('center_axis',(-0.674206889080985,-0.738542531419647,
0.));
#114708=DIRECTION('ref_axis',(0.738542531419647,-0.674206889080985,0.));
#114709=DIRECTION('center_axis',(-2.41254715360153E-30,4.71408804214643E-44,
-1.));
#114710=DIRECTION('ref_axis',(1.95398793972133E-14,1.,5.9740946667467E-59));
#114711=DIRECTION('center_axis',(0.,0.,1.));
#114712=DIRECTION('ref_axis',(0.,1.,0.));
#114713=DIRECTION('center_axis',(0.7059219377897,-0.708289642552562,-2.19056695270365E-17));
#114714=DIRECTION('ref_axis',(0.708289642552562,0.7059219377897,4.72941823813195E-33));
#114715=DIRECTION('center_axis',(0.,0.,-1.));
#114716=DIRECTION('ref_axis',(0.,1.,0.));
#114717=DIRECTION('center_axis',(0.,0.,1.));
#114718=DIRECTION('ref_axis',(0.,1.,0.));
#114719=DIRECTION('center_axis',(-0.7059219377897,0.708289642552561,8.74510085926797E-17));
#114720=DIRECTION('ref_axis',(0.708289642552561,0.7059219377897,-8.55019604084016E-33));
#114721=DIRECTION('',(-0.7059219377897,0.708289642552561,8.74510085926797E-17));
#114722=DIRECTION('',(0.7059219377897,-0.708289642552561,-8.74510085926797E-17));
#114723=DIRECTION('center_axis',(-0.964962125666191,0.262389207151869,3.23966346967465E-17));
#114724=DIRECTION('ref_axis',(0.262389207151869,0.964962125666191,-4.57090956622107E-33));
#114725=DIRECTION('',(-0.964962125666191,0.262389207151869,3.23966346967465E-17));
#114726=DIRECTION('center_axis',(-0.964962125666191,0.26238920715187,2.42758782660955E-15));
#114727=DIRECTION('ref_axis',(-0.26238920715187,-0.964962125666191,2.22950724024121E-31));
#114728=DIRECTION('',(0.964962125666191,-0.262389207151869,-3.23966346967465E-17));
#114729=DIRECTION('center_axis',(0.,0.,-1.));
#114730=DIRECTION('ref_axis',(0.,1.,0.));
#114731=DIRECTION('center_axis',(0.,0.,1.));
#114732=DIRECTION('ref_axis',(0.,1.,0.));
#114733=DIRECTION('center_axis',(-0.735878524541004,-0.677113577710087,
0.));
#114734=DIRECTION('ref_axis',(0.677113577710087,-0.735878524541004,0.));
#114735=DIRECTION('center_axis',(0.,1.23467863058847E-16,-1.));
#114736=DIRECTION('ref_axis',(0.,1.,0.));
#114737=DIRECTION('center_axis',(-0.682537484892593,-0.730850587819763,
0.));
#114738=DIRECTION('ref_axis',(0.730850587819763,-0.682537484892593,0.));
#114739=DIRECTION('center_axis',(4.93476711729114E-30,1.97232914692071E-43,
-1.));
#114740=DIRECTION('ref_axis',(-3.99680288865056E-14,1.,0.));
#114741=DIRECTION('center_axis',(0.,0.,1.));
#114742=DIRECTION('ref_axis',(0.,1.,0.));
#114743=DIRECTION('center_axis',(0.255245343760721,-0.966876318092687,-2.36149381309596E-15));
#114744=DIRECTION('ref_axis',(0.966876318092687,0.255245343760721,9.80822191756775E-31));
#114745=DIRECTION('center_axis',(-5.71153601538325E-31,2.64211616260596E-45,
-1.));
#114746=DIRECTION('ref_axis',(4.62592926927148E-15,1.,1.24460305557223E-60));
#114747=DIRECTION('center_axis',(0.,0.,1.));
#114748=DIRECTION('ref_axis',(0.,1.,0.));
#114749=DIRECTION('center_axis',(0.255245343760725,-0.966876318092686,-1.1937815283711E-16));
#114750=DIRECTION('ref_axis',(-0.966876318092686,-0.255245343760725,-8.61241374820812E-33));
#114751=DIRECTION('',(-0.255245343760725,0.966876318092686,1.1937815283711E-16));
#114752=DIRECTION('',(0.255245343760725,-0.966876318092686,-1.1937815283711E-16));
#114753=DIRECTION('center_axis',(0.257447214431338,0.966292363511968,1.19306053212906E-16));
#114754=DIRECTION('ref_axis',(0.966292363511968,-0.257447214431338,-1.5335664280992E-33));
#114755=DIRECTION('',(-0.257447214431338,-0.966292363511968,-1.19306053212906E-16));
#114756=DIRECTION('center_axis',(-0.257447214431328,-0.96629236351197,1.78800005081742E-14));
#114757=DIRECTION('ref_axis',(0.96629236351197,-0.257447214431328,-3.12759209575828E-30));
#114758=DIRECTION('',(0.257447214431338,0.966292363511968,1.19306053212906E-16));
#114759=DIRECTION('center_axis',(0.680870844883904,-0.732403503942382,0.));
#114760=DIRECTION('ref_axis',(0.732403503942382,0.680870844883904,0.));
#114761=DIRECTION('center_axis',(0.,0.,-1.));
#114762=DIRECTION('ref_axis',(0.,-1.,0.));
#114763=DIRECTION('center_axis',(0.,0.,1.));
#114764=DIRECTION('ref_axis',(0.,-1.,0.));
#114765=DIRECTION('center_axis',(0.,-1.23467863058847E-16,1.));
#114766=DIRECTION('ref_axis',(0.,-1.,0.));
#114767=DIRECTION('center_axis',(0.734334158412675,-0.678788143523698,0.));
#114768=DIRECTION('ref_axis',(0.678788143523698,0.734334158412675,0.));
#114769=DIRECTION('center_axis',(0.,0.,-1.));
#114770=DIRECTION('ref_axis',(0.,-1.,0.));
#114771=DIRECTION('center_axis',(4.05747518532827E-30,-1.33339190228861E-43,
1.));
#114772=DIRECTION('ref_axis',(-3.28626015289047E-14,-1.,2.58877435559024E-58));
#114773=DIRECTION('center_axis',(0.,0.,1.));
#114774=DIRECTION('ref_axis',(0.,-1.,0.));
#114775=DIRECTION('center_axis',(0.965557341499939,0.260190353924909,-4.11871123919569E-15));
#114776=DIRECTION('ref_axis',(-0.260190353924909,0.965557341499939,-2.2632930465492E-31));
#114777=DIRECTION('center_axis',(0.,0.,-1.));
#114778=DIRECTION('ref_axis',(0.,-1.,0.));
#114779=DIRECTION('center_axis',(-0.965557341499939,-0.260190353924911,
-3.21251469876339E-17));
#114780=DIRECTION('ref_axis',(-0.260190353924911,0.965557341499939,-9.87488652925334E-34));
#114781=DIRECTION('',(-0.965557341499939,-0.260190353924911,-3.21251469876339E-17));
#114782=DIRECTION('',(0.965557341499939,0.260190353924911,3.21251469876339E-17));
#114783=DIRECTION('center_axis',(-0.700366780446484,-0.713783141330072,
-8.81292791474553E-17));
#114784=DIRECTION('ref_axis',(-0.713783141330072,0.700366780446484,-8.54636793605324E-33));
#114785=DIRECTION('',(-0.700366780446485,-0.713783141330072,-8.81292791474553E-17));
#114786=DIRECTION('center_axis',(-0.700366780446484,-0.713783141330073,
0.));
#114787=DIRECTION('ref_axis',(0.713783141330073,-0.700366780446484,0.));
#114788=DIRECTION('',(0.700366780446485,0.713783141330072,8.81292791474553E-17));
#114789=DIRECTION('center_axis',(0.679956281045647,-0.733252654865001,0.));
#114790=DIRECTION('ref_axis',(0.733252654865001,0.679956281045647,0.));
#114791=DIRECTION('center_axis',(0.,0.,-1.));
#114792=DIRECTION('ref_axis',(0.,-1.,0.));
#114793=DIRECTION('center_axis',(0.,0.,1.));
#114794=DIRECTION('ref_axis',(0.,-1.,0.));
#114795=DIRECTION('center_axis',(0.,-1.23467863058847E-16,1.));
#114796=DIRECTION('ref_axis',(0.,-1.,0.));
#114797=DIRECTION('center_axis',(0.746021307914879,-0.665922073621961,1.23220336456872E-14));
#114798=DIRECTION('ref_axis',(0.665922073621961,0.746021307914879,1.41534494748923E-30));
#114799=DIRECTION('center_axis',(0.,0.,-1.));
#114800=DIRECTION('ref_axis',(0.,-1.,0.));
#114801=DIRECTION('center_axis',(3.28984144636074E-30,-8.76588974171719E-44,
1.));
#114802=DIRECTION('ref_axis',(-2.66453258755498E-14,-1.,1.59309191113245E-58));
#114803=DIRECTION('center_axis',(0.,0.,1.));
#114804=DIRECTION('ref_axis',(0.,-1.,0.));
#114805=DIRECTION('center_axis',(0.700366780446456,0.7137831413301,0.));
#114806=DIRECTION('ref_axis',(-0.7137831413301,0.700366780446456,0.));
#114807=DIRECTION('center_axis',(0.,0.,-1.));
#114808=DIRECTION('ref_axis',(0.,-1.,0.));
#114809=DIRECTION('center_axis',(0.700366780446451,0.713783141330105,8.81292791474594E-17));
#114810=DIRECTION('ref_axis',(0.713783141330105,-0.700366780446451,4.73735951537523E-32));
#114811=DIRECTION('',(-0.700366780446451,-0.713783141330105,-8.81292791474594E-17));
#114812=DIRECTION('',(0.700366780446451,0.713783141330105,8.81292791474594E-17));
#114813=DIRECTION('center_axis',(0.,0.,-1.));
#114814=DIRECTION('ref_axis',(0.,1.,0.));
#114815=DIRECTION('',(0.,1.23467863058847E-16,-1.));
#114816=DIRECTION('',(6.16297582203915E-33,-1.23467863058847E-16,1.));
#114817=DIRECTION('center_axis',(0.,0.,-1.));
#114818=DIRECTION('ref_axis',(0.,1.,0.));
#114819=DIRECTION('',(-7.37292681274632E-34,1.23467863058847E-16,-1.));
#114820=DIRECTION('',(0.,-1.23467863058847E-16,1.));
#114821=DIRECTION('center_axis',(0.,0.,1.));
#114822=DIRECTION('ref_axis',(0.,-1.,0.));
#114823=DIRECTION('',(0.,1.23467863058847E-16,-1.));
#114824=DIRECTION('',(0.,-1.23467863058847E-16,1.));
#114825=DIRECTION('center_axis',(0.,0.,1.));
#114826=DIRECTION('ref_axis',(0.0252625808996282,0.999680850074808,0.));
#114827=DIRECTION('',(5.83684288299471E-35,1.23467863058847E-16,-1.));
#114828=DIRECTION('',(0.,-1.23467863058847E-16,1.));
#114829=DIRECTION('center_axis',(0.,0.,1.));
#114830=DIRECTION('ref_axis',(0.,-1.,0.));
#114831=DIRECTION('',(3.52789515968553E-33,1.23467863058847E-16,-1.));
#114832=DIRECTION('',(0.,-1.23467863058847E-16,1.));
#114833=DIRECTION('center_axis',(0.,0.,1.));
#114834=DIRECTION('ref_axis',(0.,-1.,0.));
#114835=DIRECTION('',(-1.21605822285869E-32,-1.23467863058847E-16,1.));
#114836=DIRECTION('',(0.,1.23467863058847E-16,-1.));
#114837=DIRECTION('center_axis',(0.,0.,-1.));
#114838=DIRECTION('ref_axis',(-0.239106811829941,-0.970993271107746,0.));
#114839=DIRECTION('',(0.,1.23467863058847E-16,-1.));
#114840=DIRECTION('',(6.62645671305077E-33,-1.23467863058847E-16,1.));
#114841=DIRECTION('center_axis',(0.,0.,-1.));
#114842=DIRECTION('ref_axis',(0.,1.,0.));
#114843=DIRECTION('',(6.16297582203915E-33,1.23467863058847E-16,-1.));
#114844=DIRECTION('',(0.,-1.23467863058847E-16,1.));
#114845=DIRECTION('center_axis',(0.,1.23467863058847E-16,-1.));
#114846=DIRECTION('ref_axis',(0.,1.,0.));
#114847=DIRECTION('center_axis',(0.,0.,-1.));
#114848=DIRECTION('ref_axis',(0.,1.,0.));
#114849=DIRECTION('center_axis',(0.,-1.,0.));
#114850=DIRECTION('ref_axis',(0.,0.,1.));
#114851=DIRECTION('center_axis',(0.,0.,1.));
#114852=DIRECTION('ref_axis',(0.,1.,0.));
#114853=DIRECTION('center_axis',(-0.994416787801726,-0.105523704152657,
0.));
#114854=DIRECTION('ref_axis',(0.105523704152657,-0.994416787801726,0.));
#114855=DIRECTION('center_axis',(-7.82779334765923E-17,1.,0.));
#114856=DIRECTION('ref_axis',(0.,0.,1.));
#114857=DIRECTION('center_axis',(0.,-1.,0.));
#114858=DIRECTION('ref_axis',(0.,0.,1.));
#114859=DIRECTION('',(-7.82779334765923E-17,1.,1.23467863058847E-16));
#114860=DIRECTION('',(7.82779334765923E-17,-1.,-1.23467863058847E-16));
#114861=DIRECTION('center_axis',(0.,1.23467863058847E-16,-1.));
#114862=DIRECTION('ref_axis',(0.,1.,1.38375392967352E-16));
#114863=DIRECTION('center_axis',(-0.992522955047552,-0.122058116090968,
0.));
#114864=DIRECTION('ref_axis',(0.122058116090968,-0.992522955047552,0.));
#114865=DIRECTION('center_axis',(6.16166569047948E-31,1.35428930001789E-16,
-1.));
#114866=DIRECTION('ref_axis',(5.15143483426073E-14,1.,1.35428930001789E-16));
#114867=DIRECTION('center_axis',(0.,-1.35726946151947E-16,1.));
#114868=DIRECTION('ref_axis',(0.,1.,1.35726946151947E-16));
#114869=DIRECTION('center_axis',(0.,1.23467863058847E-16,-1.));
#114870=DIRECTION('ref_axis',(0.,1.,0.));
#114871=DIRECTION('center_axis',(-1.,0.,0.));
#114872=DIRECTION('ref_axis',(0.,0.,1.));
#114873=DIRECTION('center_axis',(0.,0.,1.));
#114874=DIRECTION('ref_axis',(0.,1.,0.));
#114875=DIRECTION('center_axis',(0.,0.,-1.));
#114876=DIRECTION('ref_axis',(0.,1.,0.));
#114877=DIRECTION('center_axis',(0.,1.23467863058847E-16,-1.));
#114878=DIRECTION('ref_axis',(0.,1.,0.));
#114879=DIRECTION('center_axis',(-0.848949186868299,-0.528474481990998,
0.));
#114880=DIRECTION('ref_axis',(0.528474481990998,-0.848949186868299,0.));
#114881=DIRECTION('center_axis',(-2.06796993660427E-30,3.463654065723E-44,
-1.));
#114882=DIRECTION('ref_axis',(1.67490542508106E-14,1.,-2.09093313336134E-58));
#114883=DIRECTION('center_axis',(0.,0.,1.));
#114884=DIRECTION('ref_axis',(0.,1.,0.));
#114885=DIRECTION('center_axis',(-1.,0.,-1.17757899099328E-32));
#114886=DIRECTION('ref_axis',(0.,1.,0.));
#114887=DIRECTION('center_axis',(-1.,0.,0.));
#114888=DIRECTION('ref_axis',(0.,0.,1.));
#114889=DIRECTION('',(1.,9.53753439817791E-17,1.17757899099328E-32));
#114890=DIRECTION('',(-1.,-9.53753439817791E-17,-1.17757899099328E-32));
#114891=DIRECTION('center_axis',(0.,1.23467863058847E-16,-1.));
#114892=DIRECTION('ref_axis',(0.,1.,0.));
#114893=DIRECTION('center_axis',(-0.787431540449703,-0.616402116402116,
0.));
#114894=DIRECTION('ref_axis',(0.616402116402116,-0.787431540449703,0.));
#114895=DIRECTION('center_axis',(-7.6763044046751E-31,4.77254954069701E-45,
-1.));
#114896=DIRECTION('ref_axis',(6.21724893790088E-15,1.,-1.86690458335834E-60));
#114897=DIRECTION('center_axis',(0.,0.,1.));
#114898=DIRECTION('ref_axis',(0.,1.,0.));
#114899=DIRECTION('center_axis',(0.,1.23467863058847E-16,-1.));
#114900=DIRECTION('ref_axis',(0.,1.,0.));
#114901=DIRECTION('center_axis',(0.,1.,0.));
#114902=DIRECTION('ref_axis',(0.,0.,-1.));
#114903=DIRECTION('center_axis',(0.,0.,1.));
#114904=DIRECTION('ref_axis',(0.,1.,0.));
#114905=DIRECTION('center_axis',(0.,0.,-1.));
#114906=DIRECTION('ref_axis',(0.,1.,0.));
#114907=DIRECTION('center_axis',(0.,1.23467863058847E-16,-1.));
#114908=DIRECTION('ref_axis',(0.,1.,0.));
#114909=DIRECTION('center_axis',(0.,-1.,0.));
#114910=DIRECTION('ref_axis',(0.,0.,1.));
#114911=DIRECTION('center_axis',(-3.56971000961454E-31,1.03207662601796E-45,
-1.));
#114912=DIRECTION('ref_axis',(2.89120579329468E-15,1.,-3.11150763893057E-61));
#114913=DIRECTION('center_axis',(0.,0.,1.));
#114914=DIRECTION('ref_axis',(0.,1.,0.));
#114915=DIRECTION('center_axis',(0.,-1.,0.));
#114916=DIRECTION('ref_axis',(0.,0.,-1.));
#114917=DIRECTION('',(0.,1.,1.23467863058847E-16));
#114918=DIRECTION('',(0.,-1.,-1.23467863058847E-16));
#114919=DIRECTION('center_axis',(0.,1.23467863058847E-16,-1.));
#114920=DIRECTION('ref_axis',(0.,1.,0.));
#114921=DIRECTION('center_axis',(0.,0.,-1.));
#114922=DIRECTION('ref_axis',(0.,1.,0.));
#114923=DIRECTION('center_axis',(0.,-1.,0.));
#114924=DIRECTION('ref_axis',(0.,0.,1.));
#114925=DIRECTION('center_axis',(0.,0.,1.));
#114926=DIRECTION('ref_axis',(0.,1.,0.));
#114927=DIRECTION('center_axis',(-0.998440322660918,-0.0558294016156522,
0.));
#114928=DIRECTION('ref_axis',(0.0558294016156522,-0.998440322660918,0.));
#114929=DIRECTION('center_axis',(-5.87084501074442E-17,1.,0.));
#114930=DIRECTION('ref_axis',(0.,0.,1.));
#114931=DIRECTION('center_axis',(0.,-1.,0.));
#114932=DIRECTION('ref_axis',(0.,0.,1.));
#114933=DIRECTION('',(-5.87084501074442E-17,1.,1.23467863058847E-16));
#114934=DIRECTION('',(5.87084501074442E-17,-1.,-1.23467863058847E-16));
#114935=DIRECTION('center_axis',(0.,1.23467863058847E-16,-1.));
#114936=DIRECTION('ref_axis',(0.,1.,1.38375392967352E-16));
#114937=DIRECTION('center_axis',(-0.995642397459837,-0.0932535059953692,
0.));
#114938=DIRECTION('ref_axis',(0.0932535059953692,-0.995642397459837,0.));
#114939=DIRECTION('center_axis',(8.0739067668352E-31,1.35428930001789E-16,
-1.));
#114940=DIRECTION('ref_axis',(6.75015598972095E-14,1.,1.35428930001789E-16));
#114941=DIRECTION('center_axis',(0.,-1.35726946151947E-16,1.));
#114942=DIRECTION('ref_axis',(0.,1.,1.35726946151947E-16));
#114943=DIRECTION('center_axis',(0.,1.23467863058847E-16,-1.));
#114944=DIRECTION('ref_axis',(0.,1.,0.));
#114945=DIRECTION('center_axis',(-1.,0.,0.));
#114946=DIRECTION('ref_axis',(0.,0.,1.));
#114947=DIRECTION('center_axis',(0.,0.,1.));
#114948=DIRECTION('ref_axis',(0.,1.,0.));
#114949=DIRECTION('center_axis',(0.,0.,-1.));
#114950=DIRECTION('ref_axis',(0.,1.,0.));
#114951=DIRECTION('center_axis',(0.,1.23467863058847E-16,-1.));
#114952=DIRECTION('ref_axis',(0.,1.,0.));
#114953=DIRECTION('center_axis',(0.,-1.,0.));
#114954=DIRECTION('ref_axis',(0.,0.,1.));
#114955=DIRECTION('center_axis',(0.,0.,-1.));
#114956=DIRECTION('ref_axis',(0.,1.,0.));
#114957=DIRECTION('center_axis',(0.,0.,1.));
#114958=DIRECTION('ref_axis',(0.,1.,0.));
#114959=DIRECTION('center_axis',(-1.,0.,-1.17757899099328E-32));
#114960=DIRECTION('ref_axis',(0.,1.,0.));
#114961=DIRECTION('center_axis',(-1.,0.,0.));
#114962=DIRECTION('ref_axis',(0.,0.,1.));
#114963=DIRECTION('',(1.,9.53753439817791E-17,1.17757899099328E-32));
#114964=DIRECTION('',(-1.,-9.53753439817791E-17,-1.17757899099328E-32));
#114965=DIRECTION('center_axis',(-7.82779334765923E-17,-1.,0.));
#114966=DIRECTION('ref_axis',(0.,0.,-1.));
#114967=DIRECTION('center_axis',(0.,-1.,0.));
#114968=DIRECTION('ref_axis',(0.,0.,1.));
#114969=DIRECTION('',(7.82779334765923E-17,1.,1.23467863058847E-16));
#114970=DIRECTION('',(-7.82779334765923E-17,-1.,-1.23467863058847E-16));
#114971=DIRECTION('center_axis',(0.,1.23467863058847E-16,-1.));
#114972=DIRECTION('ref_axis',(0.,1.,0.));
#114973=DIRECTION('center_axis',(0.,0.,-1.));
#114974=DIRECTION('ref_axis',(0.,1.,0.));
#114975=DIRECTION('center_axis',(0.,0.,1.));
#114976=DIRECTION('ref_axis',(0.,1.,0.));
#114977=DIRECTION('center_axis',(0.,1.23467863058847E-16,-1.));
#114978=DIRECTION('ref_axis',(0.,1.,0.));
#114979=DIRECTION('center_axis',(0.,0.,-1.));
#114980=DIRECTION('ref_axis',(0.,1.,0.));
#114981=DIRECTION('center_axis',(0.,-1.,0.));
#114982=DIRECTION('ref_axis',(0.,0.,1.));
#114983=DIRECTION('center_axis',(0.,0.,1.));
#114984=DIRECTION('ref_axis',(0.,1.,0.));
#114985=DIRECTION('center_axis',(-0.999981180102553,-0.00613509907864248,
0.));
#114986=DIRECTION('ref_axis',(0.00613509907864248,-0.999981180102553,0.));
#114987=DIRECTION('center_axis',(-6.11546355285877E-17,1.,0.));
#114988=DIRECTION('ref_axis',(0.,0.,1.));
#114989=DIRECTION('center_axis',(0.,-1.,0.));
#114990=DIRECTION('ref_axis',(0.,0.,1.));
#114991=DIRECTION('',(-6.11546355285877E-17,1.,1.23467863058847E-16));
#114992=DIRECTION('',(6.11546355285877E-17,-1.,-1.23467863058847E-16));
#114993=DIRECTION('center_axis',(0.,1.23467863058847E-16,-1.));
#114994=DIRECTION('ref_axis',(0.,1.,1.38375392967352E-16));
#114995=DIRECTION('center_axis',(-0.999050847451757,-0.0435592034583644,
0.));
#114996=DIRECTION('ref_axis',(0.0435592034583644,-0.999050847451757,0.));
#114997=DIRECTION('center_axis',(-6.37413692118567E-32,1.35428930001789E-16,
-1.));
#114998=DIRECTION('ref_axis',(-5.32907051820075E-15,1.,1.35428930001789E-16));
#114999=DIRECTION('center_axis',(0.,-1.35726946151947E-16,1.));
#115000=DIRECTION('ref_axis',(0.,1.,1.35726946151947E-16));
#115001=DIRECTION('center_axis',(0.,1.23467863058847E-16,-1.));
#115002=DIRECTION('ref_axis',(0.,1.,0.));
#115003=DIRECTION('center_axis',(-1.,0.,0.));
#115004=DIRECTION('ref_axis',(0.,0.,1.));
#115005=DIRECTION('center_axis',(0.,0.,1.));
#115006=DIRECTION('ref_axis',(0.,1.,0.));
#115007=DIRECTION('center_axis',(0.,0.,-1.));
#115008=DIRECTION('ref_axis',(0.,1.,0.));
#115009=DIRECTION('center_axis',(0.,1.23467863058847E-16,-1.));
#115010=DIRECTION('ref_axis',(0.,1.,0.));
#115011=DIRECTION('center_axis',(0.,-1.,0.));
#115012=DIRECTION('ref_axis',(0.,0.,1.));
#115013=DIRECTION('center_axis',(-1.78485500480727E-31,2.58019156504489E-46,
-1.));
#115014=DIRECTION('ref_axis',(1.44560289664734E-15,1.,-3.88938454866321E-62));
#115015=DIRECTION('center_axis',(0.,0.,1.));
#115016=DIRECTION('ref_axis',(0.,1.,0.));
#115017=DIRECTION('center_axis',(-1.,0.,-1.17757899099328E-32));
#115018=DIRECTION('ref_axis',(0.,1.,0.));
#115019=DIRECTION('center_axis',(-1.,0.,0.));
#115020=DIRECTION('ref_axis',(0.,0.,1.));
#115021=DIRECTION('',(1.,9.53753439817791E-17,1.17757899099328E-32));
#115022=DIRECTION('',(-1.,-9.53753439817791E-17,-1.17757899099328E-32));
#115023=DIRECTION('center_axis',(0.,-1.,-1.23467863058847E-16));
#115024=DIRECTION('ref_axis',(-1.,0.,0.));
#115025=DIRECTION('center_axis',(0.,-1.,0.));
#115026=DIRECTION('ref_axis',(0.,0.,1.));
#115027=DIRECTION('',(-3.13111733906369E-16,1.,1.23467863058847E-16));
#115028=DIRECTION('',(3.13111733906369E-16,-1.,-1.23467863058847E-16));
#115029=DIRECTION('center_axis',(0.,1.23467863058847E-16,-1.));
#115030=DIRECTION('ref_axis',(0.,1.,0.));
#115031=DIRECTION('center_axis',(0.,0.,-1.));
#115032=DIRECTION('ref_axis',(0.,1.,0.));
#115033=DIRECTION('center_axis',(0.,0.,1.));
#115034=DIRECTION('ref_axis',(0.,1.,0.));
#115035=DIRECTION('center_axis',(0.,1.23467863058847E-16,-1.));
#115036=DIRECTION('ref_axis',(0.,1.,0.));
#115037=DIRECTION('center_axis',(-1.,-4.81867632215781E-16,0.));
#115038=DIRECTION('ref_axis',(4.81867632215781E-16,-1.,0.));
#115039=DIRECTION('center_axis',(0.,0.,-1.));
#115040=DIRECTION('ref_axis',(0.,1.,0.));
#115041=DIRECTION('center_axis',(0.,-1.,0.));
#115042=DIRECTION('ref_axis',(0.,0.,1.));
#115043=DIRECTION('center_axis',(0.,0.,1.));
#115044=DIRECTION('ref_axis',(0.,1.,0.));
#115045=DIRECTION('center_axis',(-6.11546355285877E-17,1.,0.));
#115046=DIRECTION('ref_axis',(0.,0.,1.));
#115047=DIRECTION('center_axis',(0.,-1.,0.));
#115048=DIRECTION('ref_axis',(0.,0.,1.));
#115049=DIRECTION('',(-6.11546355285877E-17,1.,1.23467863058847E-16));
#115050=DIRECTION('',(6.11546355285877E-17,-1.,-1.23467863058847E-16));
#115051=DIRECTION('center_axis',(1.,0.,5.88789495496639E-32));
#115052=DIRECTION('ref_axis',(0.,-1.,0.));
#115053=DIRECTION('center_axis',(-1.,0.,0.));
#115054=DIRECTION('ref_axis',(0.,0.,1.));
#115055=DIRECTION('',(1.,4.76876719908896E-16,5.88789495496639E-32));
#115056=DIRECTION('',(-1.,-4.76876719908896E-16,-5.88789495496639E-32));
#115057=DIRECTION('center_axis',(0.,1.23467863058847E-16,-1.));
#115058=DIRECTION('ref_axis',(0.,1.,0.));
#115059=DIRECTION('center_axis',(-1.,0.,0.));
#115060=DIRECTION('ref_axis',(0.,0.,1.));
#115061=DIRECTION('center_axis',(0.,0.,1.));
#115062=DIRECTION('ref_axis',(0.,1.,0.));
#115063=DIRECTION('center_axis',(0.,0.,-1.));
#115064=DIRECTION('ref_axis',(0.,1.,0.));
#115065=DIRECTION('center_axis',(0.,1.23467863058847E-16,-1.));
#115066=DIRECTION('ref_axis',(0.,1.,0.));
#115067=DIRECTION('center_axis',(0.,-1.,0.));
#115068=DIRECTION('ref_axis',(0.,0.,1.));
#115069=DIRECTION('center_axis',(0.,0.,-1.));
#115070=DIRECTION('ref_axis',(0.,1.,0.));
#115071=DIRECTION('center_axis',(0.,0.,1.));
#115072=DIRECTION('ref_axis',(0.,1.,0.));
#115073=DIRECTION('center_axis',(-1.,0.,-1.5273745825629E-32));
#115074=DIRECTION('ref_axis',(0.,1.,0.));
#115075=DIRECTION('center_axis',(-1.,0.,0.));
#115076=DIRECTION('ref_axis',(0.,0.,1.));
#115077=DIRECTION('',(1.,1.23706245878324E-16,1.52737458256291E-32));
#115078=DIRECTION('',(-1.,-1.23706245878324E-16,-1.52737458256291E-32));
#115079=DIRECTION('center_axis',(0.,-1.,-1.23467863058847E-16));
#115080=DIRECTION('ref_axis',(-1.,0.,0.));
#115081=DIRECTION('center_axis',(0.,-1.,0.));
#115082=DIRECTION('ref_axis',(0.,0.,1.));
#115083=DIRECTION('',(-3.13111733906369E-16,1.,1.23467863058847E-16));
#115084=DIRECTION('',(3.13111733906369E-16,-1.,-1.23467863058847E-16));
#115085=DIRECTION('center_axis',(0.,1.23467863058847E-16,-1.));
#115086=DIRECTION('ref_axis',(0.,1.,0.));
#115087=DIRECTION('center_axis',(-1.78485500480727E-31,2.58019156504489E-46,
-1.));
#115088=DIRECTION('ref_axis',(1.44560289664734E-15,1.,-3.88938454866321E-62));
#115089=DIRECTION('center_axis',(0.,0.,1.));
#115090=DIRECTION('ref_axis',(0.,1.,0.));
#115091=DIRECTION('center_axis',(0.,1.23467863058847E-16,-1.));
#115092=DIRECTION('ref_axis',(0.,1.,0.));
#115093=DIRECTION('center_axis',(-1.,0.,0.));
#115094=DIRECTION('ref_axis',(0.,0.,1.));
#115095=DIRECTION('center_axis',(0.,0.,-1.));
#115096=DIRECTION('ref_axis',(0.,1.,0.));
#115097=DIRECTION('center_axis',(0.,-1.,0.));
#115098=DIRECTION('ref_axis',(0.,0.,1.));
#115099=DIRECTION('center_axis',(0.,0.,1.));
#115100=DIRECTION('ref_axis',(0.,1.,0.));
#115101=DIRECTION('center_axis',(-6.11546355285877E-17,1.,0.));
#115102=DIRECTION('ref_axis',(0.,0.,1.));
#115103=DIRECTION('center_axis',(0.,-1.,0.));
#115104=DIRECTION('ref_axis',(0.,0.,1.));
#115105=DIRECTION('',(-6.11546355285877E-17,1.,1.23467863058847E-16));
#115106=DIRECTION('',(6.11546355285877E-17,-1.,-1.23467863058847E-16));
#115107=DIRECTION('center_axis',(1.,0.,-1.5273745825629E-32));
#115108=DIRECTION('ref_axis',(0.,-1.,0.));
#115109=DIRECTION('center_axis',(-1.,0.,0.));
#115110=DIRECTION('ref_axis',(0.,0.,1.));
#115111=DIRECTION('',(1.,-1.23706245878324E-16,-1.52737458256291E-32));
#115112=DIRECTION('',(-1.,1.23706245878324E-16,1.52737458256291E-32));
#115113=DIRECTION('center_axis',(0.,1.23467863058847E-16,-1.));
#115114=DIRECTION('ref_axis',(0.,1.,0.));
#115115=DIRECTION('center_axis',(-0.995922166025996,-0.0902166238455439,
0.));
#115116=DIRECTION('ref_axis',(0.0902166238455439,-0.995922166025996,0.));
#115117=DIRECTION('center_axis',(0.,0.,1.));
#115118=DIRECTION('ref_axis',(0.,1.,0.));
#115119=DIRECTION('center_axis',(1.11553437800454E-31,1.00788733009566E-46,
-1.));
#115120=DIRECTION('ref_axis',(-9.03501810404587E-16,1.,1.55575381946529E-61));
#115121=DIRECTION('center_axis',(0.,1.23467863058847E-16,-1.));
#115122=DIRECTION('ref_axis',(0.,1.,0.));
#115123=DIRECTION('center_axis',(0.,-1.,0.));
#115124=DIRECTION('ref_axis',(0.,0.,1.));
#115125=DIRECTION('center_axis',(1.78485500480727E-31,2.58019156504489E-46,
-1.));
#115126=DIRECTION('ref_axis',(-1.44560289664734E-15,1.,-3.88938454866321E-62));
#115127=DIRECTION('center_axis',(0.,0.,1.));
#115128=DIRECTION('ref_axis',(0.,1.,0.));
#115129=DIRECTION('center_axis',(0.,1.23467863058847E-16,-1.));
#115130=DIRECTION('ref_axis',(0.,1.,0.));
#115131=DIRECTION('center_axis',(-0.913440670994017,-0.406971916198157,
-3.63370493544251E-16));
#115132=DIRECTION('ref_axis',(0.406971916198157,-0.913440670994017,6.94755181634254E-32));
#115133=DIRECTION('center_axis',(-5.48307457476793E-31,2.43497425545765E-45,
-1.));
#115134=DIRECTION('ref_axis',(4.44089209850063E-15,1.,-3.42265840282363E-60));
#115135=DIRECTION('center_axis',(0.,0.,1.));
#115136=DIRECTION('ref_axis',(0.,1.,0.));
#115137=DIRECTION('center_axis',(0.,-1.,-1.23467863058847E-16));
#115138=DIRECTION('ref_axis',(-1.,0.,0.));
#115139=DIRECTION('center_axis',(3.61400724161834E-16,-1.,-1.20466908053943E-16));
#115140=DIRECTION('ref_axis',(1.,3.61400724161834E-16,-2.73691106313441E-47));
#115141=DIRECTION('',(-3.13111733906369E-16,1.,1.23467863058847E-16));
#115142=DIRECTION('',(3.13111733906369E-16,-1.,-1.23467863058847E-16));
#115143=DIRECTION('center_axis',(0.,1.23467863058847E-16,-1.));
#115144=DIRECTION('ref_axis',(0.,1.,0.));
#115145=DIRECTION('center_axis',(-0.99836765577839,-0.0571141304368959,
4.12821761995348E-17));
#115146=DIRECTION('ref_axis',(0.0571141304368959,-0.99836765577839,1.08996476499831E-33));
#115147=DIRECTION('center_axis',(0.,0.,1.));
#115148=DIRECTION('ref_axis',(0.,1.,0.));
#115149=DIRECTION('center_axis',(0.,0.,-1.));
#115150=DIRECTION('ref_axis',(0.,1.,0.));
#115151=DIRECTION('center_axis',(0.,1.23467863058847E-16,-1.));
#115152=DIRECTION('ref_axis',(-0.686617021913638,-0.727019301819729,0.));
#115153=DIRECTION('center_axis',(0.,0.,1.));
#115154=DIRECTION('ref_axis',(0.,1.,0.));
#115155=DIRECTION('center_axis',(-1.78485500480727E-31,2.58019156504489E-46,
-1.));
#115156=DIRECTION('ref_axis',(1.44560289664734E-15,1.,0.));
#115157=DIRECTION('center_axis',(0.,1.23467863058847E-16,-1.));
#115158=DIRECTION('ref_axis',(0.,1.,0.));
#115159=DIRECTION('center_axis',(-1.,0.,0.));
#115160=DIRECTION('ref_axis',(0.,0.,1.));
#115161=DIRECTION('center_axis',(0.,0.,-1.));
#115162=DIRECTION('ref_axis',(0.,1.,0.));
#115163=DIRECTION('center_axis',(0.,-1.,0.));
#115164=DIRECTION('ref_axis',(0.,0.,1.));
#115165=DIRECTION('center_axis',(0.,0.,1.));
#115166=DIRECTION('ref_axis',(0.,1.,0.));
#115167=DIRECTION('center_axis',(-5.87084501074442E-17,1.,0.));
#115168=DIRECTION('ref_axis',(0.,0.,1.));
#115169=DIRECTION('center_axis',(4.81867632215779E-16,-1.,-1.20466908053945E-16));
#115170=DIRECTION('ref_axis',(1.,4.81867632215779E-16,1.09476442525376E-47));
#115171=DIRECTION('',(-5.87084501074442E-17,1.,1.23467863058847E-16));
#115172=DIRECTION('',(5.87084501074442E-17,-1.,-1.23467863058847E-16));
#115173=DIRECTION('center_axis',(1.,0.,-1.5273745825629E-32));
#115174=DIRECTION('ref_axis',(0.,-1.,0.));
#115175=DIRECTION('center_axis',(-1.,0.,0.));
#115176=DIRECTION('ref_axis',(0.,0.,1.));
#115177=DIRECTION('',(1.,-1.23706245878324E-16,-1.52737458256291E-32));
#115178=DIRECTION('',(-1.,1.23706245878324E-16,1.52737458256291E-32));
#115179=DIRECTION('center_axis',(0.,1.23467863058847E-16,-1.));
#115180=DIRECTION('ref_axis',(0.,1.,0.));
#115181=DIRECTION('center_axis',(-1.,0.,0.));
#115182=DIRECTION('ref_axis',(0.,0.,1.));
#115183=DIRECTION('center_axis',(0.,0.,1.));
#115184=DIRECTION('ref_axis',(0.,1.,0.));
#115185=DIRECTION('center_axis',(0.,0.,-1.));
#115186=DIRECTION('ref_axis',(0.,1.,0.));
#115187=DIRECTION('center_axis',(0.,1.23467863058847E-16,-1.));
#115188=DIRECTION('ref_axis',(0.,1.,0.));
#115189=DIRECTION('center_axis',(0.,-1.,0.));
#115190=DIRECTION('ref_axis',(0.,0.,1.));
#115191=DIRECTION('center_axis',(3.56971000961454E-31,1.03207662601796E-45,
-1.));
#115192=DIRECTION('ref_axis',(-2.89120579329468E-15,1.,-3.11150763893057E-61));
#115193=DIRECTION('center_axis',(0.,0.,1.));
#115194=DIRECTION('ref_axis',(0.,1.,0.));
#115195=DIRECTION('center_axis',(-1.,0.,4.58212374768871E-32));
#115196=DIRECTION('ref_axis',(0.,1.,0.));
#115197=DIRECTION('center_axis',(-1.,0.,0.));
#115198=DIRECTION('ref_axis',(0.,0.,1.));
#115199=DIRECTION('',(1.,-3.71118737634973E-16,-4.58212374768871E-32));
#115200=DIRECTION('',(-1.,3.71118737634973E-16,4.58212374768871E-32));
#115201=DIRECTION('center_axis',(-7.82779334765923E-17,-1.,0.));
#115202=DIRECTION('ref_axis',(0.,0.,-1.));
#115203=DIRECTION('center_axis',(-1.20466908053945E-16,-1.,-1.20466908053943E-16));
#115204=DIRECTION('ref_axis',(1.,-1.20466908053945E-16,2.73691106313441E-48));
#115205=DIRECTION('',(7.82779334765923E-17,1.,1.23467863058847E-16));
#115206=DIRECTION('',(-7.82779334765923E-17,-1.,-1.23467863058847E-16));
#115207=DIRECTION('center_axis',(0.,1.23467863058847E-16,-1.));
#115208=DIRECTION('ref_axis',(0.,1.,0.));
#115209=DIRECTION('center_axis',(0.,0.,-1.));
#115210=DIRECTION('ref_axis',(0.,1.,0.));
#115211=DIRECTION('center_axis',(0.,0.,1.));
#115212=DIRECTION('ref_axis',(0.,1.,0.));
#115213=DIRECTION('center_axis',(0.,1.23467863058847E-16,-1.));
#115214=DIRECTION('ref_axis',(0.,1.,0.));
#115215=DIRECTION('center_axis',(-1.,0.,0.));
#115216=DIRECTION('ref_axis',(0.,0.,1.));
#115217=DIRECTION('center_axis',(0.,0.,-1.));
#115218=DIRECTION('ref_axis',(0.,1.,0.));
#115219=DIRECTION('center_axis',(0.,-1.,0.));
#115220=DIRECTION('ref_axis',(0.,0.,1.));
#115221=DIRECTION('center_axis',(0.,0.,1.));
#115222=DIRECTION('ref_axis',(0.,1.,0.));
#115223=DIRECTION('center_axis',(-5.87084501074442E-17,1.,0.));
#115224=DIRECTION('ref_axis',(0.,0.,1.));
#115225=DIRECTION('center_axis',(0.,-1.,0.));
#115226=DIRECTION('ref_axis',(0.,0.,1.));
#115227=DIRECTION('',(-5.87084501074442E-17,1.,1.23467863058847E-16));
#115228=DIRECTION('',(5.87084501074442E-17,-1.,-1.23467863058847E-16));
#115229=DIRECTION('center_axis',(1.,0.,5.88789495496639E-32));
#115230=DIRECTION('ref_axis',(0.,-1.,0.));
#115231=DIRECTION('center_axis',(-1.,0.,0.));
#115232=DIRECTION('ref_axis',(0.,0.,1.));
#115233=DIRECTION('',(1.,4.76876719908896E-16,5.88789495496639E-32));
#115234=DIRECTION('',(-1.,-4.76876719908896E-16,-5.88789495496639E-32));
#115235=DIRECTION('center_axis',(0.,1.23467863058847E-16,-1.));
#115236=DIRECTION('ref_axis',(0.,1.,0.));
#115237=DIRECTION('center_axis',(-1.,0.,0.));
#115238=DIRECTION('ref_axis',(0.,0.,1.));
#115239=DIRECTION('center_axis',(0.,0.,1.));
#115240=DIRECTION('ref_axis',(0.,1.,0.));
#115241=DIRECTION('center_axis',(1.78485500480727E-31,2.58019156504489E-46,
-1.));
#115242=DIRECTION('ref_axis',(-1.44560289664734E-15,1.,-3.88938454866321E-62));
#115243=DIRECTION('center_axis',(0.,1.23467863058847E-16,-1.));
#115244=DIRECTION('ref_axis',(0.,1.,0.));
#115245=DIRECTION('center_axis',(0.,-1.,0.));
#115246=DIRECTION('ref_axis',(0.,0.,1.));
#115247=DIRECTION('center_axis',(0.,0.,-1.));
#115248=DIRECTION('ref_axis',(0.,1.,0.));
#115249=DIRECTION('center_axis',(0.,0.,1.));
#115250=DIRECTION('ref_axis',(0.,1.,0.));
#115251=DIRECTION('center_axis',(-1.,0.,-1.5273745825629E-32));
#115252=DIRECTION('ref_axis',(0.,1.,0.));
#115253=DIRECTION('center_axis',(-1.,0.,0.));
#115254=DIRECTION('ref_axis',(0.,0.,1.));
#115255=DIRECTION('',(1.,1.23706245878324E-16,1.52737458256291E-32));
#115256=DIRECTION('',(-1.,-1.23706245878324E-16,-1.52737458256291E-32));
#115257=DIRECTION('center_axis',(-7.82779334765923E-17,-1.,0.));
#115258=DIRECTION('ref_axis',(0.,0.,-1.));
#115259=DIRECTION('center_axis',(0.,-1.,0.));
#115260=DIRECTION('ref_axis',(0.,0.,1.));
#115261=DIRECTION('',(7.82779334765923E-17,1.,1.23467863058847E-16));
#115262=DIRECTION('',(-7.82779334765923E-17,-1.,-1.23467863058847E-16));
#115263=DIRECTION('center_axis',(0.,1.23467863058847E-16,-1.));
#115264=DIRECTION('ref_axis',(0.,1.,0.));
#115265=DIRECTION('center_axis',(0.,0.,-1.));
#115266=DIRECTION('ref_axis',(0.,1.,0.));
#115267=DIRECTION('center_axis',(0.,0.,1.));
#115268=DIRECTION('ref_axis',(0.,1.,0.));
#115269=DIRECTION('center_axis',(0.,1.23467863058847E-16,-1.));
#115270=DIRECTION('ref_axis',(0.,1.,0.));
#115271=DIRECTION('center_axis',(-1.,0.,0.));
#115272=DIRECTION('ref_axis',(0.,0.,1.));
#115273=DIRECTION('center_axis',(0.,0.,-1.));
#115274=DIRECTION('ref_axis',(0.,1.,0.));
#115275=DIRECTION('center_axis',(0.,-1.,0.));
#115276=DIRECTION('ref_axis',(0.,0.,1.));
#115277=DIRECTION('center_axis',(0.,0.,1.));
#115278=DIRECTION('ref_axis',(0.,1.,0.));
#115279=DIRECTION('center_axis',(-7.82779334765923E-17,1.,0.));
#115280=DIRECTION('ref_axis',(0.,0.,1.));
#115281=DIRECTION('center_axis',(0.,-1.,0.));
#115282=DIRECTION('ref_axis',(0.,0.,1.));
#115283=DIRECTION('',(-7.82779334765923E-17,1.,1.23467863058847E-16));
#115284=DIRECTION('',(7.82779334765923E-17,-1.,-1.23467863058847E-16));
#115285=DIRECTION('center_axis',(1.,0.,5.88789495496639E-32));
#115286=DIRECTION('ref_axis',(0.,-1.,0.));
#115287=DIRECTION('center_axis',(-1.,0.,0.));
#115288=DIRECTION('ref_axis',(0.,0.,1.));
#115289=DIRECTION('',(1.,4.76876719908896E-16,5.88789495496639E-32));
#115290=DIRECTION('',(-1.,-4.76876719908896E-16,-5.88789495496639E-32));
#115291=DIRECTION('center_axis',(0.,1.23467863058847E-16,-1.));
#115292=DIRECTION('ref_axis',(0.,1.,0.));
#115293=DIRECTION('center_axis',(-1.,0.,0.));
#115294=DIRECTION('ref_axis',(0.,0.,1.));
#115295=DIRECTION('center_axis',(0.,0.,1.));
#115296=DIRECTION('ref_axis',(0.,1.,0.));
#115297=DIRECTION('center_axis',(0.,0.,-1.));
#115298=DIRECTION('ref_axis',(0.,1.,0.));
#115299=DIRECTION('center_axis',(0.,1.23467863058847E-16,-1.));
#115300=DIRECTION('ref_axis',(0.,1.,0.));
#115301=DIRECTION('center_axis',(0.,-1.,0.));
#115302=DIRECTION('ref_axis',(0.,0.,1.));
#115303=DIRECTION('center_axis',(0.,0.,-1.));
#115304=DIRECTION('ref_axis',(0.,1.,0.));
#115305=DIRECTION('center_axis',(0.,0.,1.));
#115306=DIRECTION('ref_axis',(0.,1.,0.));
#115307=DIRECTION('center_axis',(-1.,0.,-1.5273745825629E-32));
#115308=DIRECTION('ref_axis',(0.,1.,0.));
#115309=DIRECTION('center_axis',(-1.,0.,0.));
#115310=DIRECTION('ref_axis',(0.,0.,1.));
#115311=DIRECTION('',(1.,1.23706245878324E-16,1.52737458256291E-32));
#115312=DIRECTION('',(-1.,-1.23706245878324E-16,-1.52737458256291E-32));
#115313=DIRECTION('center_axis',(0.,-1.,0.));
#115314=DIRECTION('ref_axis',(0.,0.,-1.));
#115315=DIRECTION('center_axis',(0.,-1.,0.));
#115316=DIRECTION('ref_axis',(0.,0.,1.));
#115317=DIRECTION('',(0.,1.,1.23467863058847E-16));
#115318=DIRECTION('',(0.,-1.,-1.23467863058847E-16));
#115319=DIRECTION('center_axis',(0.,1.23467863058847E-16,-1.));
#115320=DIRECTION('ref_axis',(0.,1.,0.));
#115321=DIRECTION('center_axis',(0.,0.,-1.));
#115322=DIRECTION('ref_axis',(0.,1.,0.));
#115323=DIRECTION('center_axis',(0.,0.,1.));
#115324=DIRECTION('ref_axis',(0.,1.,0.));
#115325=DIRECTION('center_axis',(0.,1.23467863058847E-16,-1.));
#115326=DIRECTION('ref_axis',(0.,1.,0.));
#115327=DIRECTION('center_axis',(-1.,0.,0.));
#115328=DIRECTION('ref_axis',(0.,0.,1.));
#115329=DIRECTION('center_axis',(0.,0.,-1.));
#115330=DIRECTION('ref_axis',(0.,1.,0.));
#115331=DIRECTION('center_axis',(0.,-1.,0.));
#115332=DIRECTION('ref_axis',(0.,0.,1.));
#115333=DIRECTION('center_axis',(0.,0.,1.));
#115334=DIRECTION('ref_axis',(0.,1.,0.));
#115335=DIRECTION('center_axis',(-7.82779334765923E-17,1.,0.));
#115336=DIRECTION('ref_axis',(0.,0.,1.));
#115337=DIRECTION('center_axis',(-4.57774250604992E-15,-1.,-1.20466908053943E-16));
#115338=DIRECTION('ref_axis',(1.,-4.57774250604992E-15,-3.50324616081204E-46));
#115339=DIRECTION('',(-7.82779334765923E-17,1.,1.23467863058847E-16));
#115340=DIRECTION('',(7.82779334765923E-17,-1.,-1.23467863058847E-16));
#115341=DIRECTION('center_axis',(1.,0.,-1.5273745825629E-32));
#115342=DIRECTION('ref_axis',(0.,-1.,0.));
#115343=DIRECTION('center_axis',(-1.,0.,0.));
#115344=DIRECTION('ref_axis',(0.,0.,1.));
#115345=DIRECTION('',(1.,-1.23706245878324E-16,-1.52737458256291E-32));
#115346=DIRECTION('',(-1.,1.23706245878324E-16,1.52737458256291E-32));
#115347=DIRECTION('center_axis',(0.,1.23467863058847E-16,-1.));
#115348=DIRECTION('ref_axis',(0.,1.,0.));
#115349=DIRECTION('center_axis',(-1.,0.,0.));
#115350=DIRECTION('ref_axis',(0.,0.,1.));
#115351=DIRECTION('center_axis',(0.,0.,1.));
#115352=DIRECTION('ref_axis',(0.,1.,0.));
#115353=DIRECTION('center_axis',(0.,0.,-1.));
#115354=DIRECTION('ref_axis',(0.,1.,0.));
#115355=DIRECTION('center_axis',(0.,1.23467863058847E-16,-1.));
#115356=DIRECTION('ref_axis',(0.,1.,0.));
#115357=DIRECTION('center_axis',(0.,-1.,0.));
#115358=DIRECTION('ref_axis',(0.,0.,1.));
#115359=DIRECTION('center_axis',(0.,0.,-1.));
#115360=DIRECTION('ref_axis',(0.,1.,0.));
#115361=DIRECTION('center_axis',(0.,0.,1.));
#115362=DIRECTION('ref_axis',(0.,1.,0.));
#115363=DIRECTION('center_axis',(-1.,0.,4.58212374768871E-32));
#115364=DIRECTION('ref_axis',(0.,1.,0.));
#115365=DIRECTION('center_axis',(-1.,0.,0.));
#115366=DIRECTION('ref_axis',(0.,0.,1.));
#115367=DIRECTION('',(1.,-3.71118737634973E-16,-4.58212374768871E-32));
#115368=DIRECTION('',(-1.,3.71118737634973E-16,4.58212374768871E-32));
#115369=DIRECTION('center_axis',(0.,-1.,0.));
#115370=DIRECTION('ref_axis',(0.,0.,-1.));
#115371=DIRECTION('center_axis',(0.,-1.,-1.20466908053943E-16));
#115372=DIRECTION('ref_axis',(0.,-1.20466908053943E-16,1.));
#115373=DIRECTION('',(0.,1.,1.23467863058847E-16));
#115374=DIRECTION('',(0.,-1.,-1.23467863058847E-16));
#115375=DIRECTION('center_axis',(0.,1.23467863058847E-16,-1.));
#115376=DIRECTION('ref_axis',(0.,1.,0.));
#115377=DIRECTION('center_axis',(0.,0.,-1.));
#115378=DIRECTION('ref_axis',(0.,1.,0.));
#115379=DIRECTION('center_axis',(0.,0.,1.));
#115380=DIRECTION('ref_axis',(0.,1.,0.));
#115381=DIRECTION('center_axis',(0.,1.23467863058847E-16,-1.));
#115382=DIRECTION('ref_axis',(0.,1.,0.));
#115383=DIRECTION('center_axis',(-1.,0.,0.));
#115384=DIRECTION('ref_axis',(0.,0.,1.));
#115385=DIRECTION('center_axis',(0.,0.,-1.));
#115386=DIRECTION('ref_axis',(0.,1.,0.));
#115387=DIRECTION('center_axis',(0.,-1.,0.));
#115388=DIRECTION('ref_axis',(0.,0.,1.));
#115389=DIRECTION('center_axis',(0.,0.,1.));
#115390=DIRECTION('ref_axis',(0.,1.,0.));
#115391=DIRECTION('center_axis',(0.,1.,0.));
#115392=DIRECTION('ref_axis',(0.,0.,1.));
#115393=DIRECTION('center_axis',(-3.61400724161836E-16,-1.,-1.20466908053943E-16));
#115394=DIRECTION('ref_axis',(1.,-3.61400724161836E-16,1.09476442525376E-47));
#115395=DIRECTION('',(0.,1.,1.23467863058847E-16));
#115396=DIRECTION('',(0.,-1.,-1.23467863058847E-16));
#115397=DIRECTION('center_axis',(1.,0.,-1.5273745825629E-32));
#115398=DIRECTION('ref_axis',(0.,-1.,0.));
#115399=DIRECTION('center_axis',(-1.,0.,0.));
#115400=DIRECTION('ref_axis',(0.,0.,1.));
#115401=DIRECTION('',(1.,-1.23706245878324E-16,-1.52737458256291E-32));
#115402=DIRECTION('',(-1.,1.23706245878324E-16,1.52737458256291E-32));
#115403=DIRECTION('center_axis',(0.,1.23467863058847E-16,-1.));
#115404=DIRECTION('ref_axis',(0.,1.,0.));
#115405=DIRECTION('center_axis',(-1.,0.,0.));
#115406=DIRECTION('ref_axis',(0.,0.,1.));
#115407=DIRECTION('center_axis',(0.,0.,1.));
#115408=DIRECTION('ref_axis',(0.,1.,0.));
#115409=DIRECTION('center_axis',(0.,0.,-1.));
#115410=DIRECTION('ref_axis',(0.,1.,0.));
#115411=DIRECTION('center_axis',(0.,1.23467863058847E-16,-1.));
#115412=DIRECTION('ref_axis',(0.,1.,0.));
#115413=DIRECTION('center_axis',(-0.0294983404866172,-0.999564829267485,
0.));
#115414=DIRECTION('ref_axis',(0.999564829267485,-0.0294983404866172,0.));
#115415=DIRECTION('center_axis',(0.,0.,-1.));
#115416=DIRECTION('ref_axis',(0.,1.,0.));
#115417=DIRECTION('center_axis',(0.,0.,1.));
#115418=DIRECTION('ref_axis',(0.,1.,0.));
#115419=DIRECTION('center_axis',(-1.,0.,4.58212374768871E-32));
#115420=DIRECTION('ref_axis',(0.,1.,0.));
#115421=DIRECTION('center_axis',(-1.,0.,0.));
#115422=DIRECTION('ref_axis',(0.,0.,1.));
#115423=DIRECTION('',(1.,-3.71118737634973E-16,-4.58212374768871E-32));
#115424=DIRECTION('',(-1.,3.71118737634973E-16,4.58212374768871E-32));
#115425=DIRECTION('center_axis',(0.,1.23467863058847E-16,-1.));
#115426=DIRECTION('ref_axis',(0.,1.,1.25697703075927E-16));
#115427=DIRECTION('center_axis',(-0.0175200318846342,-0.999846512462169,
-1.20448417884836E-16));
#115428=DIRECTION('ref_axis',(0.999846512462169,-0.0175200318846342,1.51017636338582E-32));
#115429=DIRECTION('center_axis',(1.11644282221188E-31,1.22833149346405E-16,
-1.));
#115430=DIRECTION('ref_axis',(-1.75897069864052E-13,1.,1.22833149346405E-16));
#115431=DIRECTION('center_axis',(0.,-1.22914743790472E-16,1.));
#115432=DIRECTION('ref_axis',(0.,1.,1.22914743790472E-16));
#115433=DIRECTION('center_axis',(0.,1.23467863058847E-16,-1.));
#115434=DIRECTION('ref_axis',(0.,1.,0.));
#115435=DIRECTION('center_axis',(0.,0.,-1.));
#115436=DIRECTION('ref_axis',(0.,1.,0.));
#115437=DIRECTION('center_axis',(0.,0.,1.));
#115438=DIRECTION('ref_axis',(0.,1.,0.));
#115439=DIRECTION('center_axis',(0.,1.23467863058847E-16,-1.));
#115440=DIRECTION('ref_axis',(0.,1.,0.));
#115441=DIRECTION('center_axis',(-1.,0.,0.));
#115442=DIRECTION('ref_axis',(0.,0.,1.));
#115443=DIRECTION('center_axis',(0.,0.,-1.));
#115444=DIRECTION('ref_axis',(0.,1.,0.));
#115445=DIRECTION('center_axis',(0.,-1.,0.));
#115446=DIRECTION('ref_axis',(0.,0.,1.));
#115447=DIRECTION('center_axis',(0.,0.,1.));
#115448=DIRECTION('ref_axis',(0.,1.,0.));
#115449=DIRECTION('center_axis',(0.,1.,0.));
#115450=DIRECTION('ref_axis',(0.,0.,1.));
#115451=DIRECTION('center_axis',(0.,-1.,0.));
#115452=DIRECTION('ref_axis',(0.,0.,1.));
#115453=DIRECTION('',(0.,1.,1.23467863058847E-16));
#115454=DIRECTION('',(0.,-1.,-1.23467863058847E-16));
#115455=DIRECTION('center_axis',(1.,0.,5.88789495496639E-32));
#115456=DIRECTION('ref_axis',(0.,-1.,0.));
#115457=DIRECTION('center_axis',(-1.,0.,0.));
#115458=DIRECTION('ref_axis',(0.,0.,1.));
#115459=DIRECTION('',(1.,4.76876719908896E-16,5.88789495496639E-32));
#115460=DIRECTION('',(-1.,-4.76876719908896E-16,-5.88789495496639E-32));
#115461=DIRECTION('center_axis',(0.,1.23467863058847E-16,-1.));
#115462=DIRECTION('ref_axis',(0.,1.,0.));
#115463=DIRECTION('center_axis',(-1.,0.,0.));
#115464=DIRECTION('ref_axis',(0.,0.,1.));
#115465=DIRECTION('center_axis',(0.,0.,1.));
#115466=DIRECTION('ref_axis',(0.,1.,0.));
#115467=DIRECTION('center_axis',(0.,0.,-1.));
#115468=DIRECTION('ref_axis',(0.,1.,0.));
#115469=DIRECTION('center_axis',(0.,1.23467863058847E-16,-1.));
#115470=DIRECTION('ref_axis',(0.,1.,0.));
#115471=DIRECTION('center_axis',(-0.646912564190485,-0.762564183719962,
0.));
#115472=DIRECTION('ref_axis',(0.762564183719962,-0.646912564190485,0.));
#115473=DIRECTION('center_axis',(0.,0.,-1.));
#115474=DIRECTION('ref_axis',(0.,1.,0.));
#115475=DIRECTION('center_axis',(0.,0.,1.));
#115476=DIRECTION('ref_axis',(0.,1.,0.));
#115477=DIRECTION('center_axis',(-1.,0.,-1.5273745825629E-32));
#115478=DIRECTION('ref_axis',(0.,1.,0.));
#115479=DIRECTION('center_axis',(-1.,0.,0.));
#115480=DIRECTION('ref_axis',(0.,0.,1.));
#115481=DIRECTION('',(1.,1.23706245878324E-16,1.52737458256291E-32));
#115482=DIRECTION('',(-1.,-1.23706245878324E-16,-1.52737458256291E-32));
#115483=DIRECTION('center_axis',(0.,1.23467863058847E-16,-1.));
#115484=DIRECTION('ref_axis',(0.,1.,0.));
#115485=DIRECTION('center_axis',(-0.55837318130784,-0.829589892896582,0.));
#115486=DIRECTION('ref_axis',(0.829589892896582,-0.55837318130784,0.));
#115487=DIRECTION('center_axis',(-6.57968948972152E-31,3.50636292785903E-45,
-1.));
#115488=DIRECTION('ref_axis',(5.32907051820075E-15,1.,0.));
#115489=DIRECTION('center_axis',(0.,0.,1.));
#115490=DIRECTION('ref_axis',(0.,1.,0.));
#115491=DIRECTION('center_axis',(0.,1.23467863058847E-16,-1.));
#115492=DIRECTION('ref_axis',(0.,1.,0.));
#115493=DIRECTION('center_axis',(0.0331928226750539,0.999448966442441,0.));
#115494=DIRECTION('ref_axis',(-0.99944896644244,0.0331928226750539,0.));
#115495=DIRECTION('center_axis',(0.,0.,1.));
#115496=DIRECTION('ref_axis',(0.,1.,0.));
#115497=DIRECTION('center_axis',(0.,0.,-1.));
#115498=DIRECTION('ref_axis',(0.,1.,0.));
#115499=DIRECTION('center_axis',(0.,1.23467863058847E-16,-1.));
#115500=DIRECTION('ref_axis',(0.,1.,0.));
#115501=DIRECTION('center_axis',(-0.03879684915621,-0.999247118832749,0.));
#115502=DIRECTION('ref_axis',(0.999247118832749,-0.03879684915621,0.));
#115503=DIRECTION('center_axis',(-1.18169710663102E-30,1.13098908268507E-44,
-1.));
#115504=DIRECTION('ref_axis',(9.57088814332033E-15,1.,-2.7381267222589E-59));
#115505=DIRECTION('center_axis',(0.,0.,1.));
#115506=DIRECTION('ref_axis',(0.,1.,0.));
#115507=DIRECTION('center_axis',(0.,1.23467863058847E-16,-1.));
#115508=DIRECTION('ref_axis',(0.,1.,1.25697703075927E-16));
#115509=DIRECTION('center_axis',(1.18920911416235E-31,1.22833149346405E-16,
-1.));
#115510=DIRECTION('ref_axis',(-1.87361497136383E-13,1.,1.22833149346405E-16));
#115511=DIRECTION('center_axis',(0.,-1.22914743790472E-16,1.));
#115512=DIRECTION('ref_axis',(0.,1.,1.22914743790472E-16));
#115513=DIRECTION('center_axis',(0.,1.23467863058847E-16,-1.));
#115514=DIRECTION('ref_axis',(0.,1.,0.));
#115515=DIRECTION('center_axis',(-1.,0.,0.));
#115516=DIRECTION('ref_axis',(0.,0.,1.));
#115517=DIRECTION('center_axis',(0.,0.,-1.));
#115518=DIRECTION('ref_axis',(0.,1.,0.));
#115519=DIRECTION('center_axis',(0.,-1.,-9.63735264431547E-16));
#115520=DIRECTION('ref_axis',(0.,-9.63735264431547E-16,1.));
#115521=DIRECTION('center_axis',(0.,0.,1.));
#115522=DIRECTION('ref_axis',(0.,1.,0.));
#115523=DIRECTION('center_axis',(0.,1.,0.));
#115524=DIRECTION('ref_axis',(0.,0.,1.));
#115525=DIRECTION('center_axis',(-3.85494105772624E-15,-1.,0.));
#115526=DIRECTION('ref_axis',(1.,-3.85494105772625E-15,0.));
#115527=DIRECTION('',(0.,1.,1.23467863058847E-16));
#115528=DIRECTION('',(0.,-1.,-1.23467863058847E-16));
#115529=DIRECTION('center_axis',(1.,0.,4.58212374768871E-32));
#115530=DIRECTION('ref_axis',(0.,-1.,0.));
#115531=DIRECTION('center_axis',(-1.,0.,0.));
#115532=DIRECTION('ref_axis',(0.,0.,1.));
#115533=DIRECTION('',(1.,3.71118737634973E-16,4.58212374768871E-32));
#115534=DIRECTION('',(-1.,-3.71118737634973E-16,-4.58212374768871E-32));
#115535=DIRECTION('center_axis',(0.,1.23467863058847E-16,-1.));
#115536=DIRECTION('ref_axis',(0.,1.,0.));
#115537=DIRECTION('center_axis',(-1.,0.,0.));
#115538=DIRECTION('ref_axis',(0.,0.,1.));
#115539=DIRECTION('center_axis',(0.,0.,1.));
#115540=DIRECTION('ref_axis',(0.,1.,0.));
#115541=DIRECTION('center_axis',(0.,0.,-1.));
#115542=DIRECTION('ref_axis',(0.,1.,0.));
#115543=DIRECTION('center_axis',(0.,1.23467863058847E-16,-1.));
#115544=DIRECTION('ref_axis',(0.,1.,0.));
#115545=DIRECTION('center_axis',(-0.0138255496962061,-0.999904422520272,
0.));
#115546=DIRECTION('ref_axis',(0.999904422520272,-0.0138255496962061,0.));
#115547=DIRECTION('center_axis',(0.,0.,-1.));
#115548=DIRECTION('ref_axis',(0.,1.,0.));
#115549=DIRECTION('center_axis',(0.,0.,1.));
#115550=DIRECTION('ref_axis',(0.,1.,0.));
#115551=DIRECTION('center_axis',(-1.,0.,4.58212374768871E-32));
#115552=DIRECTION('ref_axis',(0.,1.,0.));
#115553=DIRECTION('center_axis',(-1.,0.,0.));
#115554=DIRECTION('ref_axis',(0.,0.,1.));
#115555=DIRECTION('',(1.,-3.71118737634973E-16,-4.58212374768871E-32));
#115556=DIRECTION('',(-1.,3.71118737634973E-16,4.58212374768871E-32));
#115557=DIRECTION('center_axis',(0.,1.23467863058847E-16,-1.));
#115558=DIRECTION('ref_axis',(0.,1.,1.25697703075927E-16));
#115559=DIRECTION('center_axis',(-0.00184724109421639,-0.999998293848714,
0.));
#115560=DIRECTION('ref_axis',(0.999998293848714,-0.00184724109421639,0.));
#115561=DIRECTION('center_axis',(5.51984300367294E-32,1.22833149346405E-16,
-1.));
#115562=DIRECTION('ref_axis',(-8.69658697372547E-14,1.,1.22833149346405E-16));
#115563=DIRECTION('center_axis',(0.,-1.22914743790472E-16,1.));
#115564=DIRECTION('ref_axis',(0.,1.,1.22914743790472E-16));
#115565=DIRECTION('center_axis',(0.,1.23467863058847E-16,-1.));
#115566=DIRECTION('ref_axis',(0.,1.,0.));
#115567=DIRECTION('center_axis',(0.,0.,-1.));
#115568=DIRECTION('ref_axis',(0.,1.,0.));
#115569=DIRECTION('center_axis',(0.,0.,1.));
#115570=DIRECTION('ref_axis',(0.,1.,0.));
#115571=DIRECTION('center_axis',(0.,1.23467863058847E-16,-1.));
#115572=DIRECTION('ref_axis',(0.,1.,0.));
#115573=DIRECTION('center_axis',(-1.,0.,0.));
#115574=DIRECTION('ref_axis',(0.,0.,1.));
#115575=DIRECTION('center_axis',(0.,0.,-1.));
#115576=DIRECTION('ref_axis',(0.,1.,0.));
#115577=DIRECTION('center_axis',(0.,-1.,-9.63735264431547E-16));
#115578=DIRECTION('ref_axis',(0.,-9.63735264431547E-16,1.));
#115579=DIRECTION('center_axis',(0.,0.,1.));
#115580=DIRECTION('ref_axis',(0.,1.,0.));
#115581=DIRECTION('center_axis',(-7.82779334765923E-17,1.,0.));
#115582=DIRECTION('ref_axis',(0.,0.,1.));
#115583=DIRECTION('center_axis',(-3.85494105772624E-15,-1.,0.));
#115584=DIRECTION('ref_axis',(1.,-3.85494105772625E-15,0.));
#115585=DIRECTION('',(-7.82779334765923E-17,1.,1.23467863058847E-16));
#115586=DIRECTION('',(7.82779334765923E-17,-1.,-1.23467863058847E-16));
#115587=DIRECTION('center_axis',(1.,0.,4.58212374768871E-32));
#115588=DIRECTION('ref_axis',(0.,-1.,0.));
#115589=DIRECTION('center_axis',(-1.,0.,0.));
#115590=DIRECTION('ref_axis',(0.,0.,1.));
#115591=DIRECTION('',(1.,3.71118737634973E-16,4.58212374768871E-32));
#115592=DIRECTION('',(-1.,-3.71118737634973E-16,-4.58212374768871E-32));
#115593=DIRECTION('center_axis',(0.,1.23467863058847E-16,-1.));
#115594=DIRECTION('ref_axis',(0.,1.,0.));
#115595=DIRECTION('center_axis',(-1.,0.,0.));
#115596=DIRECTION('ref_axis',(0.,0.,1.));
#115597=DIRECTION('center_axis',(0.,0.,1.));
#115598=DIRECTION('ref_axis',(0.,1.,0.));
#115599=DIRECTION('center_axis',(0.,0.,-1.));
#115600=DIRECTION('ref_axis',(0.,1.,0.));
#115601=DIRECTION('center_axis',(0.,1.23467863058847E-16,-1.));
#115602=DIRECTION('ref_axis',(0.,1.,0.));
#115603=DIRECTION('center_axis',(0.,-1.,0.));
#115604=DIRECTION('ref_axis',(0.,0.,1.));
#115605=DIRECTION('center_axis',(0.,0.,-1.));
#115606=DIRECTION('ref_axis',(0.,1.,0.));
#115607=DIRECTION('center_axis',(0.,0.,1.));
#115608=DIRECTION('ref_axis',(0.,1.,0.));
#115609=DIRECTION('center_axis',(-1.,0.,4.58212374768871E-32));
#115610=DIRECTION('ref_axis',(0.,1.,0.));
#115611=DIRECTION('center_axis',(-1.,0.,0.));
#115612=DIRECTION('ref_axis',(0.,0.,1.));
#115613=DIRECTION('',(1.,-3.71118737634973E-16,-4.58212374768871E-32));
#115614=DIRECTION('',(-1.,3.71118737634973E-16,4.58212374768871E-32));
#115615=DIRECTION('center_axis',(0.,-1.,0.));
#115616=DIRECTION('ref_axis',(0.,0.,-1.));
#115617=DIRECTION('center_axis',(0.,-1.,0.));
#115618=DIRECTION('ref_axis',(0.,0.,1.));
#115619=DIRECTION('',(0.,1.,1.23467863058847E-16));
#115620=DIRECTION('',(0.,-1.,-1.23467863058847E-16));
#115621=DIRECTION('center_axis',(0.,1.23467863058847E-16,-1.));
#115622=DIRECTION('ref_axis',(0.,1.,0.));
#115623=DIRECTION('center_axis',(0.,0.,-1.));
#115624=DIRECTION('ref_axis',(0.,1.,0.));
#115625=DIRECTION('center_axis',(0.,0.,1.));
#115626=DIRECTION('ref_axis',(0.,1.,0.));
#115627=DIRECTION('center_axis',(0.,1.23467863058847E-16,-1.));
#115628=DIRECTION('ref_axis',(0.,1.,0.));
#115629=DIRECTION('center_axis',(0.0972343474872435,0.995261514210577,0.));
#115630=DIRECTION('ref_axis',(-0.995261514210577,0.0972343474872435,0.));
#115631=DIRECTION('center_axis',(1.78485500480727E-31,2.58019156504489E-46,
-1.));
#115632=DIRECTION('ref_axis',(-1.44560289664734E-15,1.,-3.88938454866321E-62));
#115633=DIRECTION('center_axis',(-1.,0.,0.));
#115634=DIRECTION('ref_axis',(0.,0.,1.));
#115635=DIRECTION('center_axis',(0.,0.,1.));
#115636=DIRECTION('ref_axis',(0.,1.,0.));
#115637=DIRECTION('center_axis',(-1.,0.,4.58212374768871E-32));
#115638=DIRECTION('ref_axis',(0.,1.,0.));
#115639=DIRECTION('center_axis',(-1.,0.,0.));
#115640=DIRECTION('ref_axis',(0.,0.,1.));
#115641=DIRECTION('',(1.,-3.71118737634973E-16,-4.58212374768871E-32));
#115642=DIRECTION('',(-1.,3.71118737634973E-16,4.58212374768871E-32));
#115643=DIRECTION('center_axis',(0.,1.23467863058847E-16,-1.));
#115644=DIRECTION('ref_axis',(0.,1.,0.));
#115645=DIRECTION('center_axis',(0.359814015251205,0.933024048151389,0.));
#115646=DIRECTION('ref_axis',(-0.933024048151389,0.359814015251205,0.));
#115647=DIRECTION('center_axis',(0.,0.,1.));
#115648=DIRECTION('ref_axis',(0.,1.,0.));
#115649=DIRECTION('center_axis',(-9.86953423458227E-31,7.88931658768281E-45,
-1.));
#115650=DIRECTION('ref_axis',(7.99360577730113E-15,1.,-2.48920611114446E-60));
#115651=DIRECTION('center_axis',(0.,1.23467863058847E-16,-1.));
#115652=DIRECTION('ref_axis',(0.,1.,0.));
#115653=DIRECTION('center_axis',(0.,1.,0.));
#115654=DIRECTION('ref_axis',(0.,0.,-1.));
#115655=DIRECTION('center_axis',(0.,0.,1.));
#115656=DIRECTION('ref_axis',(0.,1.,0.));
#115657=DIRECTION('center_axis',(0.,0.,-1.));
#115658=DIRECTION('ref_axis',(0.,1.,0.));
#115659=DIRECTION('center_axis',(0.,1.23467863058847E-16,-1.));
#115660=DIRECTION('ref_axis',(0.,1.,0.));
#115661=DIRECTION('center_axis',(0.,1.,0.));
#115662=DIRECTION('ref_axis',(0.,0.,-1.));
#115663=DIRECTION('center_axis',(0.,0.,-1.));
#115664=DIRECTION('ref_axis',(0.,1.,0.));
#115665=DIRECTION('center_axis',(0.,0.,1.));
#115666=DIRECTION('ref_axis',(0.,1.,0.));
#115667=DIRECTION('center_axis',(-7.82779334765923E-17,-1.,0.));
#115668=DIRECTION('ref_axis',(0.,0.,-1.));
#115669=DIRECTION('center_axis',(0.,1.,0.));
#115670=DIRECTION('ref_axis',(0.,0.,-1.));
#115671=DIRECTION('',(-7.82779334765923E-17,-1.,-1.23467863058847E-16));
#115672=DIRECTION('',(7.82779334765923E-17,1.,1.23467863058847E-16));
#115673=DIRECTION('center_axis',(-5.87084501074442E-17,1.,0.));
#115674=DIRECTION('ref_axis',(0.,0.,1.));
#115675=DIRECTION('center_axis',(0.,1.,0.));
#115676=DIRECTION('ref_axis',(0.,0.,-1.));
#115677=DIRECTION('',(5.87084501074442E-17,-1.,-1.23467863058847E-16));
#115678=DIRECTION('',(-5.87084501074442E-17,1.,1.23467863058847E-16));
#115679=DIRECTION('center_axis',(0.,1.23467863058847E-16,-1.));
#115680=DIRECTION('ref_axis',(0.,1.,0.));
#115681=DIRECTION('center_axis',(1.,0.,0.));
#115682=DIRECTION('ref_axis',(0.,0.,-1.));
#115683=DIRECTION('center_axis',(0.,0.,1.));
#115684=DIRECTION('ref_axis',(0.,1.,0.));
#115685=DIRECTION('center_axis',(3.56971000961454E-31,1.03207662601795E-45,
-1.));
#115686=DIRECTION('ref_axis',(-2.89120579329468E-15,1.,-2.1780553472514E-60));
#115687=DIRECTION('center_axis',(0.,1.23467863058847E-16,-1.));
#115688=DIRECTION('ref_axis',(0.,1.,0.));
#115689=DIRECTION('center_axis',(-1.,0.,0.));
#115690=DIRECTION('ref_axis',(0.,0.,1.));
#115691=DIRECTION('center_axis',(0.,0.,-1.));
#115692=DIRECTION('ref_axis',(0.,1.,0.));
#115693=DIRECTION('center_axis',(0.,0.,1.));
#115694=DIRECTION('ref_axis',(0.,1.,0.));
#115695=DIRECTION('center_axis',(1.,0.,4.58212374768871E-32));
#115696=DIRECTION('ref_axis',(0.,-1.,0.));
#115697=DIRECTION('',(1.,3.71118737634973E-16,4.58212374768871E-32));
#115698=DIRECTION('',(-1.,-3.71118737634973E-16,-4.58212374768871E-32));
#115699=DIRECTION('center_axis',(0.,1.23467863058847E-16,-1.));
#115700=DIRECTION('ref_axis',(0.,1.,0.));
#115701=DIRECTION('center_axis',(7.70988211545246E-15,1.,0.));
#115702=DIRECTION('ref_axis',(-1.,7.70988211545246E-15,0.));
#115703=DIRECTION('center_axis',(1.78485500480727E-31,2.58019156504489E-46,
-1.));
#115704=DIRECTION('ref_axis',(-1.44560289664734E-15,1.,-3.88938454866321E-62));
#115705=DIRECTION('center_axis',(-1.,0.,0.));
#115706=DIRECTION('ref_axis',(0.,0.,1.));
#115707=DIRECTION('center_axis',(0.,0.,1.));
#115708=DIRECTION('ref_axis',(0.,1.,0.));
#115709=DIRECTION('center_axis',(-1.,0.,4.07299888683441E-32));
#115710=DIRECTION('ref_axis',(0.,1.,0.));
#115711=DIRECTION('center_axis',(-1.,0.,0.));
#115712=DIRECTION('ref_axis',(0.,0.,1.));
#115713=DIRECTION('',(1.,-3.29883322342198E-16,-4.07299888683441E-32));
#115714=DIRECTION('',(-1.,3.29883322342198E-16,4.07299888683441E-32));
#115715=DIRECTION('center_axis',(-5.87084501074442E-17,1.,0.));
#115716=DIRECTION('ref_axis',(0.,0.,1.));
#115717=DIRECTION('center_axis',(0.,1.,0.));
#115718=DIRECTION('ref_axis',(0.,0.,-1.));
#115719=DIRECTION('',(5.87084501074442E-17,-1.,-1.23467863058847E-16));
#115720=DIRECTION('',(-5.87084501074442E-17,1.,1.23467863058847E-16));
#115721=DIRECTION('center_axis',(0.,1.23467863058847E-16,-1.));
#115722=DIRECTION('ref_axis',(0.,1.,0.));
#115723=DIRECTION('center_axis',(0.,1.,0.));
#115724=DIRECTION('ref_axis',(0.,0.,-1.));
#115725=DIRECTION('center_axis',(0.,0.,1.));
#115726=DIRECTION('ref_axis',(0.,1.,0.));
#115727=DIRECTION('center_axis',(0.,0.,-1.));
#115728=DIRECTION('ref_axis',(0.,1.,0.));
#115729=DIRECTION('center_axis',(0.,1.23467863058847E-16,-1.));
#115730=DIRECTION('ref_axis',(0.,1.,0.));
#115731=DIRECTION('center_axis',(-0.359814015251208,0.933024048151388,0.));
#115732=DIRECTION('ref_axis',(-0.933024048151388,-0.359814015251207,0.));
#115733=DIRECTION('center_axis',(0.,0.,-1.));
#115734=DIRECTION('ref_axis',(0.,1.,0.));
#115735=DIRECTION('center_axis',(0.,0.,1.));
#115736=DIRECTION('ref_axis',(0.,1.,0.));
#115737=DIRECTION('center_axis',(-7.82779334765923E-17,-1.,0.));
#115738=DIRECTION('ref_axis',(0.,0.,-1.));
#115739=DIRECTION('center_axis',(-3.85494105772624E-15,1.,0.));
#115740=DIRECTION('ref_axis',(-1.,-3.85494105772625E-15,0.));
#115741=DIRECTION('',(-7.82779334765923E-17,-1.,-1.23467863058847E-16));
#115742=DIRECTION('',(7.82779334765923E-17,1.,1.23467863058847E-16));
#115743=DIRECTION('center_axis',(0.,1.23467863058847E-16,-1.));
#115744=DIRECTION('ref_axis',(0.,1.,0.));
#115745=DIRECTION('center_axis',(-0.0972343474872435,0.995261514210577,
0.));
#115746=DIRECTION('ref_axis',(-0.995261514210577,-0.0972343474872435,0.));
#115747=DIRECTION('center_axis',(0.,0.,1.));
#115748=DIRECTION('ref_axis',(0.,1.,0.));
#115749=DIRECTION('center_axis',(-8.77291931962869E-31,6.2335340939716E-45,
-1.));
#115750=DIRECTION('ref_axis',(7.105427357601E-15,1.,-3.73380916671668E-60));
#115751=DIRECTION('center_axis',(0.,1.23467863058847E-16,-1.));
#115752=DIRECTION('ref_axis',(0.,1.,0.));
#115753=DIRECTION('center_axis',(1.,0.,0.));
#115754=DIRECTION('ref_axis',(0.,0.,-1.));
#115755=DIRECTION('center_axis',(0.,0.,1.));
#115756=DIRECTION('ref_axis',(0.,1.,0.));
#115757=DIRECTION('center_axis',(0.,0.,-1.));
#115758=DIRECTION('ref_axis',(0.,1.,0.));
#115759=DIRECTION('center_axis',(0.,1.23467863058847E-16,-1.));
#115760=DIRECTION('ref_axis',(0.,1.,0.));
#115761=DIRECTION('center_axis',(-1.,0.,0.));
#115762=DIRECTION('ref_axis',(0.,0.,1.));
#115763=DIRECTION('center_axis',(0.,0.,-1.));
#115764=DIRECTION('ref_axis',(0.,1.,0.));
#115765=DIRECTION('center_axis',(0.,0.,1.));
#115766=DIRECTION('ref_axis',(0.,1.,0.));
#115767=DIRECTION('center_axis',(1.,0.,4.58212374768871E-32));
#115768=DIRECTION('ref_axis',(0.,-1.,0.));
#115769=DIRECTION('',(1.,3.71118737634973E-16,4.58212374768871E-32));
#115770=DIRECTION('',(-1.,-3.71118737634973E-16,-4.58212374768871E-32));
#115771=DIRECTION('center_axis',(0.,1.23467863058847E-16,-1.));
#115772=DIRECTION('ref_axis',(0.,1.,0.));
#115773=DIRECTION('center_axis',(0.,1.,0.));
#115774=DIRECTION('ref_axis',(0.,0.,-1.));
#115775=DIRECTION('center_axis',(0.,0.,-1.));
#115776=DIRECTION('ref_axis',(0.,1.,0.));
#115777=DIRECTION('center_axis',(-1.,0.,0.));
#115778=DIRECTION('ref_axis',(0.,0.,1.));
#115779=DIRECTION('center_axis',(0.,0.,1.));
#115780=DIRECTION('ref_axis',(0.,1.,0.));
#115781=DIRECTION('center_axis',(-1.,0.,4.07299888683441E-32));
#115782=DIRECTION('ref_axis',(0.,1.,0.));
#115783=DIRECTION('center_axis',(-1.,0.,0.));
#115784=DIRECTION('ref_axis',(0.,0.,1.));
#115785=DIRECTION('',(1.,-3.29883322342198E-16,-4.07299888683441E-32));
#115786=DIRECTION('',(-1.,3.29883322342198E-16,4.07299888683441E-32));
#115787=DIRECTION('center_axis',(-7.82779334765923E-17,1.,0.));
#115788=DIRECTION('ref_axis',(0.,0.,1.));
#115789=DIRECTION('center_axis',(0.,1.,0.));
#115790=DIRECTION('ref_axis',(0.,0.,-1.));
#115791=DIRECTION('',(7.82779334765923E-17,-1.,-1.23467863058847E-16));
#115792=DIRECTION('',(-7.82779334765923E-17,1.,1.23467863058847E-16));
#115793=DIRECTION('center_axis',(0.,1.23467863058847E-16,-1.));
#115794=DIRECTION('ref_axis',(0.,1.,0.));
#115795=DIRECTION('center_axis',(0.,1.,0.));
#115796=DIRECTION('ref_axis',(0.,0.,-1.));
#115797=DIRECTION('center_axis',(0.,0.,1.));
#115798=DIRECTION('ref_axis',(0.,1.,0.));
#115799=DIRECTION('center_axis',(0.,0.,-1.));
#115800=DIRECTION('ref_axis',(0.,1.,0.));
#115801=DIRECTION('center_axis',(0.,1.23467863058847E-16,-1.));
#115802=DIRECTION('ref_axis',(0.,1.,0.));
#115803=DIRECTION('center_axis',(-1.,0.,0.));
#115804=DIRECTION('ref_axis',(0.,0.,1.));
#115805=DIRECTION('center_axis',(0.,0.,-1.));
#115806=DIRECTION('ref_axis',(0.,1.,0.));
#115807=DIRECTION('center_axis',(0.,0.,1.));
#115808=DIRECTION('ref_axis',(0.,1.,0.));
#115809=DIRECTION('center_axis',(0.,-1.,0.));
#115810=DIRECTION('ref_axis',(0.,0.,-1.));
#115811=DIRECTION('center_axis',(-3.85494105772624E-15,1.,0.));
#115812=DIRECTION('ref_axis',(-1.,-3.85494105772625E-15,0.));
#115813=DIRECTION('',(0.,-1.,-1.23467863058847E-16));
#115814=DIRECTION('',(0.,1.,1.23467863058847E-16));
#115815=DIRECTION('center_axis',(1.,0.,4.58212374768871E-32));
#115816=DIRECTION('ref_axis',(0.,-1.,0.));
#115817=DIRECTION('center_axis',(-1.,0.,0.));
#115818=DIRECTION('ref_axis',(0.,0.,1.));
#115819=DIRECTION('',(1.,3.71118737634973E-16,4.58212374768871E-32));
#115820=DIRECTION('',(-1.,-3.71118737634973E-16,-4.58212374768871E-32));
#115821=DIRECTION('center_axis',(0.,1.23467863058847E-16,-1.));
#115822=DIRECTION('ref_axis',(0.,1.,0.));
#115823=DIRECTION('center_axis',(0.,0.,-1.));
#115824=DIRECTION('ref_axis',(0.,1.,0.));
#115825=DIRECTION('center_axis',(0.,0.,1.));
#115826=DIRECTION('ref_axis',(0.,1.,0.));
#115827=DIRECTION('center_axis',(0.,1.23467863058847E-16,-1.));
#115828=DIRECTION('ref_axis',(0.,1.,0.));
#115829=DIRECTION('center_axis',(0.,1.,0.));
#115830=DIRECTION('ref_axis',(0.,0.,-1.));
#115831=DIRECTION('center_axis',(0.,0.,-1.));
#115832=DIRECTION('ref_axis',(0.,1.,0.));
#115833=DIRECTION('center_axis',(-1.,0.,0.));
#115834=DIRECTION('ref_axis',(0.,0.,1.));
#115835=DIRECTION('center_axis',(0.,0.,1.));
#115836=DIRECTION('ref_axis',(0.,1.,0.));
#115837=DIRECTION('center_axis',(-1.,0.,4.07299888683441E-32));
#115838=DIRECTION('ref_axis',(0.,1.,0.));
#115839=DIRECTION('center_axis',(-1.,0.,0.));
#115840=DIRECTION('ref_axis',(0.,0.,1.));
#115841=DIRECTION('',(1.,-3.29883322342198E-16,-4.07299888683441E-32));
#115842=DIRECTION('',(-1.,3.29883322342198E-16,4.07299888683441E-32));
#115843=DIRECTION('center_axis',(0.,1.,0.));
#115844=DIRECTION('ref_axis',(0.,0.,1.));
#115845=DIRECTION('center_axis',(0.,1.,0.));
#115846=DIRECTION('ref_axis',(0.,0.,-1.));
#115847=DIRECTION('',(0.,-1.,-1.23467863058847E-16));
#115848=DIRECTION('',(0.,1.,1.23467863058847E-16));
#115849=DIRECTION('center_axis',(0.,1.23467863058847E-16,-1.));
#115850=DIRECTION('ref_axis',(0.,1.,0.));
#115851=DIRECTION('center_axis',(-0.0138255496962003,0.999904422520272,
-3.41098746684905E-15));
#115852=DIRECTION('ref_axis',(-0.999904422520272,-0.0138255496962003,-3.38006024551251E-32));
#115853=DIRECTION('center_axis',(0.,0.,1.));
#115854=DIRECTION('ref_axis',(0.,1.,0.));
#115855=DIRECTION('center_axis',(0.,0.,-1.));
#115856=DIRECTION('ref_axis',(0.,1.,0.));
#115857=DIRECTION('center_axis',(0.,1.23467863058847E-16,-1.));
#115858=DIRECTION('ref_axis',(0.,1.,0.));
#115859=DIRECTION('center_axis',(-1.,0.,0.));
#115860=DIRECTION('ref_axis',(0.,0.,1.));
#115861=DIRECTION('center_axis',(0.,0.,-1.));
#115862=DIRECTION('ref_axis',(0.,1.,0.));
#115863=DIRECTION('center_axis',(0.,0.,1.));
#115864=DIRECTION('ref_axis',(0.,1.,0.));
#115865=DIRECTION('center_axis',(0.,1.23467863058847E-16,-1.));
#115866=DIRECTION('ref_axis',(0.,1.,1.25697703075927E-16));
#115867=DIRECTION('center_axis',(-0.00184724109421639,0.999998293848714,
0.));
#115868=DIRECTION('ref_axis',(-0.999998293848714,-0.00184724109421639,0.));
#115869=DIRECTION('center_axis',(0.,-1.22914743790472E-16,1.));
#115870=DIRECTION('ref_axis',(0.,1.,1.22914743790472E-16));
#115871=DIRECTION('center_axis',(0.,1.22833149346405E-16,-1.));
#115872=DIRECTION('ref_axis',(0.,1.,1.22833149346405E-16));
#115873=DIRECTION('center_axis',(1.,0.,4.58212374768871E-32));
#115874=DIRECTION('ref_axis',(0.,-1.,0.));
#115875=DIRECTION('center_axis',(-1.,0.,0.));
#115876=DIRECTION('ref_axis',(0.,0.,1.));
#115877=DIRECTION('',(1.,3.71118737634973E-16,4.58212374768871E-32));
#115878=DIRECTION('',(-1.,-3.71118737634973E-16,-4.58212374768871E-32));
#115879=DIRECTION('center_axis',(0.,1.23467863058847E-16,-1.));
#115880=DIRECTION('ref_axis',(0.,1.,0.));
#115881=DIRECTION('center_axis',(0.,0.,-1.));
#115882=DIRECTION('ref_axis',(0.,1.,0.));
#115883=DIRECTION('center_axis',(0.,0.,1.));
#115884=DIRECTION('ref_axis',(0.,1.,0.));
#115885=DIRECTION('center_axis',(0.,1.23467863058847E-16,-1.));
#115886=DIRECTION('ref_axis',(0.,1.,0.));
#115887=DIRECTION('center_axis',(0.,-1.,0.));
#115888=DIRECTION('ref_axis',(0.,0.,1.));
#115889=DIRECTION('center_axis',(0.,0.,-1.));
#115890=DIRECTION('ref_axis',(0.,1.,0.));
#115891=DIRECTION('center_axis',(1.,0.,0.));
#115892=DIRECTION('ref_axis',(0.,0.,-1.));
#115893=DIRECTION('center_axis',(0.,0.,1.));
#115894=DIRECTION('ref_axis',(0.,1.,0.));
#115895=DIRECTION('center_axis',(1.,0.,4.07299888683441E-32));
#115896=DIRECTION('ref_axis',(0.,-1.,0.));
#115897=DIRECTION('center_axis',(1.,0.,0.));
#115898=DIRECTION('ref_axis',(0.,0.,-1.));
#115899=DIRECTION('',(-1.,-3.29883322342198E-16,-4.07299888683441E-32));
#115900=DIRECTION('',(1.,3.29883322342198E-16,4.07299888683441E-32));
#115901=DIRECTION('center_axis',(0.,-1.,0.));
#115902=DIRECTION('ref_axis',(0.,0.,-1.));
#115903=DIRECTION('center_axis',(0.,-1.,0.));
#115904=DIRECTION('ref_axis',(0.,0.,1.));
#115905=DIRECTION('',(0.,1.,1.23467863058847E-16));
#115906=DIRECTION('',(0.,-1.,-1.23467863058847E-16));
#115907=DIRECTION('center_axis',(0.,1.23467863058847E-16,-1.));
#115908=DIRECTION('ref_axis',(0.,1.,0.));
#115909=DIRECTION('center_axis',(0.,-1.,0.));
#115910=DIRECTION('ref_axis',(0.,0.,1.));
#115911=DIRECTION('center_axis',(0.,0.,1.));
#115912=DIRECTION('ref_axis',(0.,1.,0.));
#115913=DIRECTION('center_axis',(0.,0.,-1.));
#115914=DIRECTION('ref_axis',(0.,1.,0.));
#115915=DIRECTION('center_axis',(0.,1.23467863058847E-16,-1.));
#115916=DIRECTION('ref_axis',(0.,1.,0.));
#115917=DIRECTION('center_axis',(1.,0.,0.));
#115918=DIRECTION('ref_axis',(0.,0.,-1.));
#115919=DIRECTION('center_axis',(0.,0.,-1.));
#115920=DIRECTION('ref_axis',(0.,1.,0.));
#115921=DIRECTION('center_axis',(0.,0.,1.));
#115922=DIRECTION('ref_axis',(0.,1.,0.));
#115923=DIRECTION('center_axis',(-7.82779334765923E-17,1.,0.));
#115924=DIRECTION('ref_axis',(0.,0.,1.));
#115925=DIRECTION('center_axis',(1.5419764230905E-14,-1.,0.));
#115926=DIRECTION('ref_axis',(1.,1.5419764230905E-14,0.));
#115927=DIRECTION('',(-7.82779334765923E-17,1.,1.23467863058847E-16));
#115928=DIRECTION('',(7.82779334765923E-17,-1.,-1.23467863058847E-16));
#115929=DIRECTION('center_axis',(-1.,0.,4.07299888683445E-32));
#115930=DIRECTION('ref_axis',(0.,1.,0.));
#115931=DIRECTION('center_axis',(1.,0.,0.));
#115932=DIRECTION('ref_axis',(0.,0.,-1.));
#115933=DIRECTION('',(-1.,3.29883322342202E-16,4.07299888683446E-32));
#115934=DIRECTION('',(1.,-3.29883322342202E-16,-4.07299888683446E-32));
#115935=DIRECTION('center_axis',(0.,1.23467863058847E-16,-1.));
#115936=DIRECTION('ref_axis',(0.,1.,0.));
#115937=DIRECTION('center_axis',(0.,0.,-1.));
#115938=DIRECTION('ref_axis',(0.,1.,0.));
#115939=DIRECTION('center_axis',(0.,0.,1.));
#115940=DIRECTION('ref_axis',(0.,1.,0.));
#115941=DIRECTION('center_axis',(0.,1.23467863058847E-16,-1.));
#115942=DIRECTION('ref_axis',(0.,1.,0.));
#115943=DIRECTION('center_axis',(0.,-1.,0.));
#115944=DIRECTION('ref_axis',(0.,0.,1.));
#115945=DIRECTION('center_axis',(0.,0.,-1.));
#115946=DIRECTION('ref_axis',(0.,1.,0.));
#115947=DIRECTION('center_axis',(1.,0.,0.));
#115948=DIRECTION('ref_axis',(0.,0.,-1.));
#115949=DIRECTION('center_axis',(0.,0.,1.));
#115950=DIRECTION('ref_axis',(0.,1.,0.));
#115951=DIRECTION('center_axis',(1.,0.,4.07299888683441E-32));
#115952=DIRECTION('ref_axis',(0.,-1.,0.));
#115953=DIRECTION('center_axis',(1.,0.,0.));
#115954=DIRECTION('ref_axis',(0.,0.,-1.));
#115955=DIRECTION('',(-1.,-3.29883322342198E-16,-4.07299888683441E-32));
#115956=DIRECTION('',(1.,3.29883322342198E-16,4.07299888683441E-32));
#115957=DIRECTION('center_axis',(-7.82779334765923E-17,-1.,0.));
#115958=DIRECTION('ref_axis',(0.,0.,-1.));
#115959=DIRECTION('center_axis',(0.,-1.,0.));
#115960=DIRECTION('ref_axis',(0.,0.,1.));
#115961=DIRECTION('',(7.82779334765923E-17,1.,1.23467863058847E-16));
#115962=DIRECTION('',(-7.82779334765923E-17,-1.,-1.23467863058847E-16));
#115963=DIRECTION('center_axis',(0.,1.23467863058847E-16,-1.));
#115964=DIRECTION('ref_axis',(0.,1.,0.));
#115965=DIRECTION('center_axis',(0.,-1.,0.));
#115966=DIRECTION('ref_axis',(0.,0.,1.));
#115967=DIRECTION('center_axis',(0.,0.,1.));
#115968=DIRECTION('ref_axis',(0.,1.,0.));
#115969=DIRECTION('center_axis',(0.,0.,-1.));
#115970=DIRECTION('ref_axis',(0.,1.,0.));
#115971=DIRECTION('center_axis',(0.,1.23467863058847E-16,-1.));
#115972=DIRECTION('ref_axis',(0.,1.,0.));
#115973=DIRECTION('center_axis',(1.,0.,0.));
#115974=DIRECTION('ref_axis',(0.,0.,-1.));
#115975=DIRECTION('center_axis',(0.,0.,-1.));
#115976=DIRECTION('ref_axis',(0.,1.,0.));
#115977=DIRECTION('center_axis',(0.,0.,1.));
#115978=DIRECTION('ref_axis',(0.,1.,0.));
#115979=DIRECTION('center_axis',(-5.87084501074442E-17,1.,0.));
#115980=DIRECTION('ref_axis',(0.,0.,1.));
#115981=DIRECTION('center_axis',(1.5419764230905E-14,-1.,-5.94422822341731E-29));
#115982=DIRECTION('ref_axis',(1.,1.5419764230905E-14,1.59309191113245E-57));
#115983=DIRECTION('',(-5.87084501074442E-17,1.,1.23467863058847E-16));
#115984=DIRECTION('',(5.87084501074442E-17,-1.,-1.23467863058847E-16));
#115985=DIRECTION('center_axis',(-1.,0.,4.07299888683445E-32));
#115986=DIRECTION('ref_axis',(0.,1.,0.));
#115987=DIRECTION('center_axis',(1.,0.,0.));
#115988=DIRECTION('ref_axis',(0.,0.,-1.));
#115989=DIRECTION('',(-1.,3.29883322342202E-16,4.07299888683446E-32));
#115990=DIRECTION('',(1.,-3.29883322342202E-16,-4.07299888683446E-32));
#115991=DIRECTION('center_axis',(0.,1.23467863058847E-16,-1.));
#115992=DIRECTION('ref_axis',(0.,1.,0.));
#115993=DIRECTION('center_axis',(0.,0.,-1.));
#115994=DIRECTION('ref_axis',(0.,1.,0.));
#115995=DIRECTION('center_axis',(0.,0.,1.));
#115996=DIRECTION('ref_axis',(0.,1.,0.));
#115997=DIRECTION('center_axis',(0.,1.23467863058847E-16,-1.));
#115998=DIRECTION('ref_axis',(0.,1.,0.));
#115999=DIRECTION('center_axis',(0.,1.,0.));
#116000=DIRECTION('ref_axis',(0.,0.,-1.));
#116001=DIRECTION('center_axis',(0.,0.,-1.));
#116002=DIRECTION('ref_axis',(0.,1.,0.));
#116003=DIRECTION('center_axis',(-1.,4.81867632215781E-16,7.43028527927166E-30));
#116004=DIRECTION('ref_axis',(-4.81867632215781E-16,-1.,1.36218908067985E-60));
#116005=DIRECTION('center_axis',(0.,0.,1.));
#116006=DIRECTION('ref_axis',(0.,1.,0.));
#116007=DIRECTION('center_axis',(-1.,0.,4.07299888683445E-32));
#116008=DIRECTION('ref_axis',(0.,1.,0.));
#116009=DIRECTION('center_axis',(-1.,0.,0.));
#116010=DIRECTION('ref_axis',(0.,0.,1.));
#116011=DIRECTION('',(1.,-3.29883322342202E-16,-4.07299888683446E-32));
#116012=DIRECTION('',(-1.,3.29883322342202E-16,4.07299888683446E-32));
#116013=DIRECTION('center_axis',(-6.11546355285877E-17,1.,0.));
#116014=DIRECTION('ref_axis',(0.,0.,1.));
#116015=DIRECTION('center_axis',(0.,1.,0.));
#116016=DIRECTION('ref_axis',(0.,0.,-1.));
#116017=DIRECTION('',(6.11546355285877E-17,-1.,-1.23467863058847E-16));
#116018=DIRECTION('',(-6.11546355285877E-17,1.,1.23467863058847E-16));
#116019=DIRECTION('center_axis',(0.,1.23467863058847E-16,-1.));
#116020=DIRECTION('ref_axis',(0.,1.,0.));
#116021=DIRECTION('center_axis',(0.,1.,0.));
#116022=DIRECTION('ref_axis',(0.,0.,-1.));
#116023=DIRECTION('center_axis',(0.,0.,1.));
#116024=DIRECTION('ref_axis',(0.,1.,0.));
#116025=DIRECTION('center_axis',(0.,0.,-1.));
#116026=DIRECTION('ref_axis',(0.,1.,0.));
#116027=DIRECTION('center_axis',(0.,1.23467863058847E-16,-1.));
#116028=DIRECTION('ref_axis',(0.,1.,0.));
#116029=DIRECTION('center_axis',(-0.995922166025996,0.0902166238455435,
0.));
#116030=DIRECTION('ref_axis',(-0.0902166238455435,-0.995922166025996,0.));
#116031=DIRECTION('center_axis',(1.11553437800454E-31,1.00788733009566E-46,
-1.));
#116032=DIRECTION('ref_axis',(-9.03501810404587E-16,1.,1.16681536459896E-61));
#116033=DIRECTION('center_axis',(0.,0.,1.));
#116034=DIRECTION('ref_axis',(0.,1.,0.));
#116035=DIRECTION('center_axis',(0.,-1.,-1.23467863058847E-16));
#116036=DIRECTION('ref_axis',(-1.,0.,0.));
#116037=DIRECTION('center_axis',(0.,1.,0.));
#116038=DIRECTION('ref_axis',(0.,0.,-1.));
#116039=DIRECTION('',(3.13111733906369E-16,-1.,-1.23467863058847E-16));
#116040=DIRECTION('',(-3.13111733906369E-16,1.,1.23467863058847E-16));
#116041=DIRECTION('center_axis',(0.,1.23467863058847E-16,-1.));
#116042=DIRECTION('ref_axis',(0.,1.,0.));
#116043=DIRECTION('center_axis',(-0.913440670994019,0.406971916198153,0.));
#116044=DIRECTION('ref_axis',(-0.406971916198153,-0.913440670994019,0.));
#116045=DIRECTION('center_axis',(0.,0.,1.));
#116046=DIRECTION('ref_axis',(0.,1.,0.));
#116047=DIRECTION('center_axis',(0.,0.,-1.));
#116048=DIRECTION('ref_axis',(0.,1.,0.));
#116049=DIRECTION('center_axis',(0.,1.23467863058847E-16,-1.));
#116050=DIRECTION('ref_axis',(0.,1.,0.));
#116051=DIRECTION('center_axis',(0.,0.,-1.));
#116052=DIRECTION('ref_axis',(0.,1.,0.));
#116053=DIRECTION('center_axis',(0.99836765577839,-0.0571141304368842,0.));
#116054=DIRECTION('ref_axis',(0.0571141304368842,0.99836765577839,0.));
#116055=DIRECTION('center_axis',(0.,0.,1.));
#116056=DIRECTION('ref_axis',(0.,1.,0.));
#116057=DIRECTION('center_axis',(0.,1.23467863058847E-16,-1.));
#116058=DIRECTION('ref_axis',(0.,1.,0.));
#116059=DIRECTION('center_axis',(0.,0.,1.));
#116060=DIRECTION('ref_axis',(0.,1.,0.));
#116061=DIRECTION('center_axis',(0.,0.,-1.));
#116062=DIRECTION('ref_axis',(0.,1.,0.));
#116063=DIRECTION('center_axis',(0.,1.23467863058847E-16,-1.));
#116064=DIRECTION('ref_axis',(0.,1.,0.));
#116065=DIRECTION('center_axis',(0.,1.,0.));
#116066=DIRECTION('ref_axis',(0.,0.,-1.));
#116067=DIRECTION('center_axis',(0.,0.,-1.));
#116068=DIRECTION('ref_axis',(0.,1.,0.));
#116069=DIRECTION('center_axis',(-1.,0.,0.));
#116070=DIRECTION('ref_axis',(0.,0.,1.));
#116071=DIRECTION('center_axis',(0.,0.,1.));
#116072=DIRECTION('ref_axis',(0.,1.,0.));
#116073=DIRECTION('center_axis',(-1.,0.,4.07299888683445E-32));
#116074=DIRECTION('ref_axis',(0.,1.,0.));
#116075=DIRECTION('center_axis',(-1.,0.,0.));
#116076=DIRECTION('ref_axis',(0.,0.,1.));
#116077=DIRECTION('',(1.,-3.29883322342202E-16,-4.07299888683446E-32));
#116078=DIRECTION('',(-1.,3.29883322342202E-16,4.07299888683446E-32));
#116079=DIRECTION('center_axis',(0.,1.,0.));
#116080=DIRECTION('ref_axis',(0.,0.,1.));
#116081=DIRECTION('center_axis',(0.,1.,0.));
#116082=DIRECTION('ref_axis',(0.,0.,-1.));
#116083=DIRECTION('',(0.,-1.,-1.23467863058847E-16));
#116084=DIRECTION('',(0.,1.,1.23467863058847E-16));
#116085=DIRECTION('center_axis',(0.,1.23467863058847E-16,-1.));
#116086=DIRECTION('ref_axis',(0.,1.,0.));
#116087=DIRECTION('center_axis',(-0.0294983404866249,0.999564829267484,
0.));
#116088=DIRECTION('ref_axis',(-0.999564829267484,-0.0294983404866249,0.));
#116089=DIRECTION('center_axis',(0.,0.,1.));
#116090=DIRECTION('ref_axis',(0.,1.,0.));
#116091=DIRECTION('center_axis',(0.,0.,-1.));
#116092=DIRECTION('ref_axis',(0.,1.,0.));
#116093=DIRECTION('center_axis',(0.,1.23467863058847E-16,-1.));
#116094=DIRECTION('ref_axis',(0.,1.,0.));
#116095=DIRECTION('center_axis',(-1.,0.,0.));
#116096=DIRECTION('ref_axis',(0.,0.,1.));
#116097=DIRECTION('center_axis',(0.,0.,-1.));
#116098=DIRECTION('ref_axis',(0.,1.,0.));
#116099=DIRECTION('center_axis',(0.,0.,1.));
#116100=DIRECTION('ref_axis',(0.,1.,0.));
#116101=DIRECTION('center_axis',(0.,1.23467863058847E-16,-1.));
#116102=DIRECTION('ref_axis',(0.,1.,1.25697703075927E-16));
#116103=DIRECTION('center_axis',(-0.0175200318846409,0.999846512462168,
7.7086987446295E-15));
#116104=DIRECTION('ref_axis',(-0.999846512462168,-0.0175200318846409,1.3995963210887E-31));
#116105=DIRECTION('center_axis',(0.,-1.22914743790472E-16,1.));
#116106=DIRECTION('ref_axis',(0.,1.,1.22914743790472E-16));
#116107=DIRECTION('center_axis',(-1.09981052690886E-31,1.22833149346405E-16,
-1.));
#116108=DIRECTION('ref_axis',(1.73276629344662E-13,1.,1.22833149346405E-16));
#116109=DIRECTION('center_axis',(1.,0.,4.07299888683441E-32));
#116110=DIRECTION('ref_axis',(0.,-1.,0.));
#116111=DIRECTION('center_axis',(-1.,0.,0.));
#116112=DIRECTION('ref_axis',(0.,0.,1.));
#116113=DIRECTION('',(1.,3.29883322342198E-16,4.07299888683441E-32));
#116114=DIRECTION('',(-1.,-3.29883322342198E-16,-4.07299888683441E-32));
#116115=DIRECTION('center_axis',(0.,1.23467863058847E-16,-1.));
#116116=DIRECTION('ref_axis',(0.,1.,0.));
#116117=DIRECTION('center_axis',(0.,0.,-1.));
#116118=DIRECTION('ref_axis',(0.,1.,0.));
#116119=DIRECTION('center_axis',(0.,0.,1.));
#116120=DIRECTION('ref_axis',(0.,1.,0.));
#116121=DIRECTION('center_axis',(0.,1.23467863058847E-16,-1.));
#116122=DIRECTION('ref_axis',(0.,1.,0.));
#116123=DIRECTION('center_axis',(-1.5419764230905E-14,1.,0.));
#116124=DIRECTION('ref_axis',(-1.,-1.5419764230905E-14,0.));
#116125=DIRECTION('center_axis',(0.,0.,-1.));
#116126=DIRECTION('ref_axis',(0.,1.,0.));
#116127=DIRECTION('center_axis',(-1.,0.,0.));
#116128=DIRECTION('ref_axis',(0.,0.,1.));
#116129=DIRECTION('center_axis',(0.,0.,1.));
#116130=DIRECTION('ref_axis',(0.,1.,0.));
#116131=DIRECTION('center_axis',(-1.,0.,7.06547394595967E-32));
#116132=DIRECTION('ref_axis',(0.,1.,0.));
#116133=DIRECTION('center_axis',(-1.,0.,0.));
#116134=DIRECTION('ref_axis',(0.,0.,1.));
#116135=DIRECTION('',(1.,-5.72252063890675E-16,-7.06547394595967E-32));
#116136=DIRECTION('',(-1.,5.72252063890675E-16,7.06547394595967E-32));
#116137=DIRECTION('center_axis',(0.,1.,0.));
#116138=DIRECTION('ref_axis',(0.,0.,1.));
#116139=DIRECTION('center_axis',(0.,1.,0.));
#116140=DIRECTION('ref_axis',(0.,0.,-1.));
#116141=DIRECTION('',(0.,-1.,-1.23467863058847E-16));
#116142=DIRECTION('',(0.,1.,1.23467863058847E-16));
#116143=DIRECTION('center_axis',(0.,1.23467863058847E-16,-1.));
#116144=DIRECTION('ref_axis',(0.,1.,0.));
#116145=DIRECTION('center_axis',(-0.64691256419049,0.762564183719958,0.));
#116146=DIRECTION('ref_axis',(-0.762564183719958,-0.64691256419049,0.));
#116147=DIRECTION('center_axis',(0.,0.,1.));
#116148=DIRECTION('ref_axis',(0.,1.,0.));
#116149=DIRECTION('center_axis',(0.,0.,-1.));
#116150=DIRECTION('ref_axis',(0.,1.,0.));
#116151=DIRECTION('center_axis',(0.,1.23467863058847E-16,-1.));
#116152=DIRECTION('ref_axis',(0.,1.,0.));
#116153=DIRECTION('center_axis',(-1.,0.,0.));
#116154=DIRECTION('ref_axis',(0.,0.,1.));
#116155=DIRECTION('center_axis',(0.,0.,-1.));
#116156=DIRECTION('ref_axis',(0.,1.,0.));
#116157=DIRECTION('center_axis',(0.,0.,1.));
#116158=DIRECTION('ref_axis',(0.,1.,0.));
#116159=DIRECTION('center_axis',(0.,1.23467863058847E-16,-1.));
#116160=DIRECTION('ref_axis',(0.,1.,0.));
#116161=DIRECTION('center_axis',(-0.55837318130784,0.829589892896582,0.));
#116162=DIRECTION('ref_axis',(-0.829589892896582,-0.55837318130784,0.));
#116163=DIRECTION('center_axis',(0.,0.,1.));
#116164=DIRECTION('ref_axis',(0.,1.,0.));
#116165=DIRECTION('center_axis',(0.,0.,-1.));
#116166=DIRECTION('ref_axis',(0.,1.,0.));
#116167=DIRECTION('center_axis',(1.,0.,4.07299888683445E-32));
#116168=DIRECTION('ref_axis',(0.,-1.,0.));
#116169=DIRECTION('center_axis',(-1.,0.,0.));
#116170=DIRECTION('ref_axis',(0.,0.,1.));
#116171=DIRECTION('',(1.,3.29883322342202E-16,4.07299888683446E-32));
#116172=DIRECTION('',(-1.,-3.29883322342202E-16,-4.07299888683446E-32));
#116173=DIRECTION('center_axis',(0.,1.23467863058847E-16,-1.));
#116174=DIRECTION('ref_axis',(0.,1.,0.));
#116175=DIRECTION('center_axis',(-0.03879684915621,0.999247118832749,5.83634271056011E-15));
#116176=DIRECTION('ref_axis',(-0.999247118832749,-0.03879684915621,-4.4574149748685E-34));
#116177=DIRECTION('center_axis',(0.,0.,1.));
#116178=DIRECTION('ref_axis',(0.,1.,0.));
#116179=DIRECTION('center_axis',(0.,0.,-1.));
#116180=DIRECTION('ref_axis',(0.,1.,0.));
#116181=DIRECTION('center_axis',(0.,1.23467863058847E-16,-1.));
#116182=DIRECTION('ref_axis',(0.,1.,0.));
#116183=DIRECTION('center_axis',(0.0331928226750423,-0.999448966442441,
0.));
#116184=DIRECTION('ref_axis',(0.999448966442441,0.0331928226750423,0.));
#116185=DIRECTION('center_axis',(0.,0.,-1.));
#116186=DIRECTION('ref_axis',(0.,1.,0.));
#116187=DIRECTION('center_axis',(0.,0.,1.));
#116188=DIRECTION('ref_axis',(0.,1.,0.));
#116189=DIRECTION('center_axis',(0.,1.23467863058847E-16,-1.));
#116190=DIRECTION('ref_axis',(0.,1.,1.25697703075927E-16));
#116191=DIRECTION('center_axis',(-1.17257681885938E-31,1.22833149346405E-16,
-1.));
#116192=DIRECTION('ref_axis',(1.84741056616993E-13,1.,1.22833149346405E-16));
#116193=DIRECTION('center_axis',(0.,-1.22914743790472E-16,1.));
#116194=DIRECTION('ref_axis',(0.,1.,1.22914743790472E-16));
#116195=DIRECTION('center_axis',(0.,1.23467863058847E-16,-1.));
#116196=DIRECTION('ref_axis',(0.,1.,0.));
#116197=DIRECTION('center_axis',(0.,1.,0.));
#116198=DIRECTION('ref_axis',(0.,0.,-1.));
#116199=DIRECTION('center_axis',(0.,0.,-1.));
#116200=DIRECTION('ref_axis',(0.,1.,0.));
#116201=DIRECTION('center_axis',(-1.,0.,0.));
#116202=DIRECTION('ref_axis',(0.,0.,1.));
#116203=DIRECTION('center_axis',(0.,0.,1.));
#116204=DIRECTION('ref_axis',(0.,1.,0.));
#116205=DIRECTION('center_axis',(-1.,0.,7.06547394595967E-32));
#116206=DIRECTION('ref_axis',(0.,1.,0.));
#116207=DIRECTION('center_axis',(-1.,0.,0.));
#116208=DIRECTION('ref_axis',(0.,0.,1.));
#116209=DIRECTION('',(1.,-5.72252063890675E-16,-7.06547394595967E-32));
#116210=DIRECTION('',(-1.,5.72252063890675E-16,7.06547394595967E-32));
#116211=DIRECTION('center_axis',(-7.82779334765923E-17,1.,0.));
#116212=DIRECTION('ref_axis',(0.,0.,1.));
#116213=DIRECTION('center_axis',(0.,1.,0.));
#116214=DIRECTION('ref_axis',(0.,0.,-1.));
#116215=DIRECTION('',(7.82779334765923E-17,-1.,-1.23467863058847E-16));
#116216=DIRECTION('',(-7.82779334765923E-17,1.,1.23467863058847E-16));
#116217=DIRECTION('center_axis',(0.,1.23467863058847E-16,-1.));
#116218=DIRECTION('ref_axis',(0.,1.,0.));
#116219=DIRECTION('center_axis',(0.,1.,0.));
#116220=DIRECTION('ref_axis',(0.,0.,-1.));
#116221=DIRECTION('center_axis',(0.,0.,1.));
#116222=DIRECTION('ref_axis',(0.,1.,0.));
#116223=DIRECTION('center_axis',(0.,0.,-1.));
#116224=DIRECTION('ref_axis',(0.,1.,0.));
#116225=DIRECTION('center_axis',(0.,1.23467863058847E-16,-1.));
#116226=DIRECTION('ref_axis',(0.,1.,0.));
#116227=DIRECTION('center_axis',(-1.,0.,0.));
#116228=DIRECTION('ref_axis',(0.,0.,1.));
#116229=DIRECTION('center_axis',(0.,0.,-1.));
#116230=DIRECTION('ref_axis',(0.,1.,0.));
#116231=DIRECTION('center_axis',(0.,0.,1.));
#116232=DIRECTION('ref_axis',(0.,1.,0.));
#116233=DIRECTION('center_axis',(0.,-1.,0.));
#116234=DIRECTION('ref_axis',(0.,0.,-1.));
#116235=DIRECTION('center_axis',(1.5419764230905E-14,1.,0.));
#116236=DIRECTION('ref_axis',(-1.,1.5419764230905E-14,0.));
#116237=DIRECTION('',(0.,-1.,-1.23467863058847E-16));
#116238=DIRECTION('',(0.,1.,1.23467863058847E-16));
#116239=DIRECTION('center_axis',(1.,0.,4.07299888683445E-32));
#116240=DIRECTION('ref_axis',(0.,-1.,0.));
#116241=DIRECTION('center_axis',(-1.,0.,0.));
#116242=DIRECTION('ref_axis',(0.,0.,1.));
#116243=DIRECTION('',(1.,3.29883322342202E-16,4.07299888683446E-32));
#116244=DIRECTION('',(-1.,-3.29883322342202E-16,-4.07299888683446E-32));
#116245=DIRECTION('center_axis',(0.,1.23467863058847E-16,-1.));
#116246=DIRECTION('ref_axis',(0.,1.,0.));
#116247=DIRECTION('center_axis',(0.,0.,-1.));
#116248=DIRECTION('ref_axis',(0.,1.,0.));
#116249=DIRECTION('center_axis',(0.,0.,1.));
#116250=DIRECTION('ref_axis',(0.,1.,0.));
#116251=DIRECTION('center_axis',(0.,1.23467863058847E-16,-1.));
#116252=DIRECTION('ref_axis',(0.,1.,0.));
#116253=DIRECTION('center_axis',(-1.5419764230905E-14,-1.,0.));
#116254=DIRECTION('ref_axis',(1.,-1.5419764230905E-14,0.));
#116255=DIRECTION('center_axis',(0.,0.,-1.));
#116256=DIRECTION('ref_axis',(0.,1.,0.));
#116257=DIRECTION('center_axis',(1.,0.,0.));
#116258=DIRECTION('ref_axis',(0.,0.,-1.));
#116259=DIRECTION('center_axis',(0.,0.,1.));
#116260=DIRECTION('ref_axis',(0.,1.,0.));
#116261=DIRECTION('center_axis',(1.,0.,-2.35515798198655E-32));
#116262=DIRECTION('ref_axis',(0.,-1.,0.));
#116263=DIRECTION('center_axis',(1.,0.,0.));
#116264=DIRECTION('ref_axis',(0.,0.,-1.));
#116265=DIRECTION('',(-1.,1.90750687963558E-16,2.35515798198656E-32));
#116266=DIRECTION('',(1.,-1.90750687963558E-16,-2.35515798198656E-32));
#116267=DIRECTION('center_axis',(0.,-1.,0.));
#116268=DIRECTION('ref_axis',(0.,0.,-1.));
#116269=DIRECTION('center_axis',(0.,-1.,0.));
#116270=DIRECTION('ref_axis',(0.,0.,1.));
#116271=DIRECTION('',(0.,1.,1.23467863058847E-16));
#116272=DIRECTION('',(0.,-1.,-1.23467863058847E-16));
#116273=DIRECTION('center_axis',(0.,1.23467863058847E-16,-1.));
#116274=DIRECTION('ref_axis',(0.,1.,0.));
#116275=DIRECTION('center_axis',(0.,-1.,0.));
#116276=DIRECTION('ref_axis',(0.,0.,1.));
#116277=DIRECTION('center_axis',(0.,0.,1.));
#116278=DIRECTION('ref_axis',(0.,1.,0.));
#116279=DIRECTION('center_axis',(0.,0.,-1.));
#116280=DIRECTION('ref_axis',(0.,1.,0.));
#116281=DIRECTION('center_axis',(0.,1.23467863058847E-16,-1.));
#116282=DIRECTION('ref_axis',(0.,1.,0.));
#116283=DIRECTION('center_axis',(0.787431540449696,-0.616402116402125,0.));
#116284=DIRECTION('ref_axis',(0.616402116402125,0.787431540449696,0.));
#116285=DIRECTION('center_axis',(0.,0.,-1.));
#116286=DIRECTION('ref_axis',(0.,1.,0.));
#116287=DIRECTION('center_axis',(0.,0.,1.));
#116288=DIRECTION('ref_axis',(0.,1.,0.));
#116289=DIRECTION('center_axis',(-7.82779334765923E-17,1.,0.));
#116290=DIRECTION('ref_axis',(0.,0.,1.));
#116291=DIRECTION('center_axis',(0.,-1.,0.));
#116292=DIRECTION('ref_axis',(0.,0.,1.));
#116293=DIRECTION('',(-7.82779334765923E-17,1.,1.23467863058847E-16));
#116294=DIRECTION('',(7.82779334765923E-17,-1.,-1.23467863058847E-16));
#116295=DIRECTION('center_axis',(0.,1.23467863058847E-16,-1.));
#116296=DIRECTION('ref_axis',(0.,1.,0.));
#116297=DIRECTION('center_axis',(0.873059908686793,-0.487612957009766,0.));
#116298=DIRECTION('ref_axis',(0.487612957009766,0.873059908686793,0.));
#116299=DIRECTION('center_axis',(0.,0.,-1.));
#116300=DIRECTION('ref_axis',(0.,1.,0.));
#116301=DIRECTION('center_axis',(0.,0.,1.));
#116302=DIRECTION('ref_axis',(0.,1.,0.));
#116303=DIRECTION('center_axis',(0.,1.23467863058847E-16,-1.));
#116304=DIRECTION('ref_axis',(0.695782815675814,-0.718252235228152,0.));
#116305=DIRECTION('center_axis',(-0.99949512518498,0.0317725468205174,0.));
#116306=DIRECTION('ref_axis',(-0.0317725468205174,-0.99949512518498,0.));
#116307=DIRECTION('center_axis',(0.,0.,1.));
#116308=DIRECTION('ref_axis',(0.,1.,0.));
#116309=DIRECTION('center_axis',(0.,0.,-1.));
#116310=DIRECTION('ref_axis',(0.,1.,0.));
#116311=DIRECTION('center_axis',(0.,1.23467863058847E-16,-1.));
#116312=DIRECTION('ref_axis',(0.,1.,0.));
#116313=DIRECTION('center_axis',(0.999425898115847,-0.0338802918425069,
0.));
#116314=DIRECTION('ref_axis',(0.0338802918425069,0.999425898115847,0.));
#116315=DIRECTION('center_axis',(0.,0.,-1.));
#116316=DIRECTION('ref_axis',(0.,1.,0.));
#116317=DIRECTION('center_axis',(0.,0.,1.));
#116318=DIRECTION('ref_axis',(0.,1.,0.));
#116319=DIRECTION('center_axis',(0.,1.23467863058847E-16,-1.));
#116320=DIRECTION('ref_axis',(0.,1.,1.25697703075927E-16));
#116321=DIRECTION('center_axis',(0.,1.22833149346405E-16,-1.));
#116322=DIRECTION('ref_axis',(0.,1.,1.22833149346405E-16));
#116323=DIRECTION('center_axis',(0.,-1.22914743790472E-16,1.));
#116324=DIRECTION('ref_axis',(0.,1.,1.22914743790472E-16));
#116325=DIRECTION('center_axis',(0.,1.23467863058847E-16,-1.));
#116326=DIRECTION('ref_axis',(0.,1.,0.));
#116327=DIRECTION('center_axis',(-1.5419764230905E-14,-1.,0.));
#116328=DIRECTION('ref_axis',(1.,-1.5419764230905E-14,0.));
#116329=DIRECTION('center_axis',(0.,0.,-1.));
#116330=DIRECTION('ref_axis',(0.,1.,0.));
#116331=DIRECTION('center_axis',(1.,0.,0.));
#116332=DIRECTION('ref_axis',(0.,0.,-1.));
#116333=DIRECTION('center_axis',(0.,0.,1.));
#116334=DIRECTION('ref_axis',(0.,1.,0.));
#116335=DIRECTION('center_axis',(1.,0.,-2.35515798198655E-32));
#116336=DIRECTION('ref_axis',(0.,-1.,0.));
#116337=DIRECTION('center_axis',(1.,0.,0.));
#116338=DIRECTION('ref_axis',(0.,0.,-1.));
#116339=DIRECTION('',(-1.,1.90750687963558E-16,2.35515798198656E-32));
#116340=DIRECTION('',(1.,-1.90750687963558E-16,-2.35515798198656E-32));
#116341=DIRECTION('center_axis',(-7.82779334765923E-17,-1.,0.));
#116342=DIRECTION('ref_axis',(0.,0.,-1.));
#116343=DIRECTION('center_axis',(0.,-1.,0.));
#116344=DIRECTION('ref_axis',(0.,0.,1.));
#116345=DIRECTION('',(7.82779334765923E-17,1.,1.23467863058847E-16));
#116346=DIRECTION('',(-7.82779334765923E-17,-1.,-1.23467863058847E-16));
#116347=DIRECTION('center_axis',(0.,1.23467863058847E-16,-1.));
#116348=DIRECTION('ref_axis',(0.,1.,0.));
#116349=DIRECTION('center_axis',(0.,-1.,0.));
#116350=DIRECTION('ref_axis',(0.,0.,1.));
#116351=DIRECTION('center_axis',(0.,0.,1.));
#116352=DIRECTION('ref_axis',(0.,1.,0.));
#116353=DIRECTION('center_axis',(0.,0.,-1.));
#116354=DIRECTION('ref_axis',(0.,1.,0.));
#116355=DIRECTION('center_axis',(0.,1.23467863058847E-16,-1.));
#116356=DIRECTION('ref_axis',(0.,1.,0.));
#116357=DIRECTION('center_axis',(0.99960573342019,-0.0280780646320843,0.));
#116358=DIRECTION('ref_axis',(0.0280780646320843,0.99960573342019,0.));
#116359=DIRECTION('center_axis',(0.,0.,-1.));
#116360=DIRECTION('ref_axis',(0.,1.,0.));
#116361=DIRECTION('center_axis',(0.,0.,1.));
#116362=DIRECTION('ref_axis',(0.,1.,0.));
#116363=DIRECTION('center_axis',(-5.87084501074442E-17,1.,0.));
#116364=DIRECTION('ref_axis',(0.,0.,1.));
#116365=DIRECTION('center_axis',(0.,-1.,0.));
#116366=DIRECTION('ref_axis',(0.,0.,1.));
#116367=DIRECTION('',(-5.87084501074442E-17,1.,1.23467863058847E-16));
#116368=DIRECTION('',(5.87084501074442E-17,-1.,-1.23467863058847E-16));
#116369=DIRECTION('center_axis',(0.,1.23467863058847E-16,-1.));
#116370=DIRECTION('ref_axis',(0.,1.,1.25697703075927E-16));
#116371=DIRECTION('center_axis',(0.999858703750256,-0.0168098939573669,
0.));
#116372=DIRECTION('ref_axis',(0.0168098939573669,0.999858703750256,0.));
#116373=DIRECTION('center_axis',(0.,1.22833149346405E-16,-1.));
#116374=DIRECTION('ref_axis',(0.,1.,1.22833149346405E-16));
#116375=DIRECTION('center_axis',(0.,-1.22914743790472E-16,1.));
#116376=DIRECTION('ref_axis',(0.,1.,1.22914743790472E-16));
#116377=DIRECTION('center_axis',(0.,1.23467863058847E-16,-1.));
#116378=DIRECTION('ref_axis',(0.701138397908224,-0.713025207814344,0.));
#116379=DIRECTION('center_axis',(0.,0.,-1.));
#116380=DIRECTION('ref_axis',(0.,1.,0.));
#116381=DIRECTION('center_axis',(0.,0.,1.));
#116382=DIRECTION('ref_axis',(0.,1.,0.));
#116383=DIRECTION('center_axis',(0.,1.23467863058847E-16,-1.));
#116384=DIRECTION('ref_axis',(0.,1.,0.));
#116385=DIRECTION('center_axis',(-1.5419764230905E-14,1.,0.));
#116386=DIRECTION('ref_axis',(-1.,-1.5419764230905E-14,0.));
#116387=DIRECTION('center_axis',(0.,0.,-1.));
#116388=DIRECTION('ref_axis',(0.,1.,0.));
#116389=DIRECTION('center_axis',(-1.,0.,0.));
#116390=DIRECTION('ref_axis',(0.,0.,1.));
#116391=DIRECTION('center_axis',(0.,0.,1.));
#116392=DIRECTION('ref_axis',(0.,1.,0.));
#116393=DIRECTION('center_axis',(-1.,0.,7.06547394595967E-32));
#116394=DIRECTION('ref_axis',(0.,1.,0.));
#116395=DIRECTION('center_axis',(-1.,0.,0.));
#116396=DIRECTION('ref_axis',(0.,0.,1.));
#116397=DIRECTION('',(1.,-5.72252063890675E-16,-7.06547394595967E-32));
#116398=DIRECTION('',(-1.,5.72252063890675E-16,7.06547394595967E-32));
#116399=DIRECTION('center_axis',(-5.87084501074442E-17,1.,0.));
#116400=DIRECTION('ref_axis',(0.,0.,1.));
#116401=DIRECTION('center_axis',(0.,1.,0.));
#116402=DIRECTION('ref_axis',(0.,0.,-1.));
#116403=DIRECTION('',(5.87084501074442E-17,-1.,-1.23467863058847E-16));
#116404=DIRECTION('',(-5.87084501074442E-17,1.,1.23467863058847E-16));
#116405=DIRECTION('center_axis',(0.,1.23467863058847E-16,-1.));
#116406=DIRECTION('ref_axis',(0.,1.,0.));
#116407=DIRECTION('center_axis',(0.,1.,0.));
#116408=DIRECTION('ref_axis',(0.,0.,-1.));
#116409=DIRECTION('center_axis',(0.,0.,1.));
#116410=DIRECTION('ref_axis',(0.,1.,0.));
#116411=DIRECTION('center_axis',(0.,0.,-1.));
#116412=DIRECTION('ref_axis',(0.,1.,0.));
#116413=DIRECTION('center_axis',(0.,1.23467863058847E-16,-1.));
#116414=DIRECTION('ref_axis',(0.,1.,0.));
#116415=DIRECTION('center_axis',(-1.,0.,0.));
#116416=DIRECTION('ref_axis',(0.,0.,1.));
#116417=DIRECTION('center_axis',(0.,0.,-1.));
#116418=DIRECTION('ref_axis',(0.,1.,0.));
#116419=DIRECTION('center_axis',(0.,0.,1.));
#116420=DIRECTION('ref_axis',(0.,1.,0.));
#116421=DIRECTION('center_axis',(-7.82779334765923E-17,-1.,0.));
#116422=DIRECTION('ref_axis',(0.,0.,-1.));
#116423=DIRECTION('center_axis',(1.5419764230905E-14,1.,0.));
#116424=DIRECTION('ref_axis',(-1.,1.5419764230905E-14,0.));
#116425=DIRECTION('',(-7.82779334765923E-17,-1.,-1.23467863058847E-16));
#116426=DIRECTION('',(7.82779334765923E-17,1.,1.23467863058847E-16));
#116427=DIRECTION('center_axis',(1.,0.,4.07299888683445E-32));
#116428=DIRECTION('ref_axis',(0.,-1.,0.));
#116429=DIRECTION('center_axis',(-1.,0.,0.));
#116430=DIRECTION('ref_axis',(0.,0.,1.));
#116431=DIRECTION('',(1.,3.29883322342202E-16,4.07299888683446E-32));
#116432=DIRECTION('',(-1.,-3.29883322342202E-16,-4.07299888683446E-32));
#116433=DIRECTION('center_axis',(0.,1.23467863058847E-16,-1.));
#116434=DIRECTION('ref_axis',(0.,1.,0.));
#116435=DIRECTION('center_axis',(0.,0.,-1.));
#116436=DIRECTION('ref_axis',(0.,1.,0.));
#116437=DIRECTION('center_axis',(0.,0.,1.));
#116438=DIRECTION('ref_axis',(0.,1.,0.));
#116439=DIRECTION('center_axis',(0.,1.23467863058847E-16,-1.));
#116440=DIRECTION('ref_axis',(0.,1.,0.));
#116441=DIRECTION('center_axis',(0.,-1.,0.));
#116442=DIRECTION('ref_axis',(0.,0.,1.));
#116443=DIRECTION('center_axis',(0.,0.,-1.));
#116444=DIRECTION('ref_axis',(0.,1.,0.));
#116445=DIRECTION('center_axis',(1.,0.,0.));
#116446=DIRECTION('ref_axis',(0.,0.,-1.));
#116447=DIRECTION('center_axis',(0.,0.,1.));
#116448=DIRECTION('ref_axis',(0.,1.,0.));
#116449=DIRECTION('center_axis',(1.,0.,-2.35515798198655E-32));
#116450=DIRECTION('ref_axis',(0.,-1.,0.));
#116451=DIRECTION('center_axis',(1.,-4.81867632215781E-16,0.));
#116452=DIRECTION('ref_axis',(4.81867632215781E-16,1.,0.));
#116453=DIRECTION('',(-1.,1.90750687963558E-16,2.35515798198656E-32));
#116454=DIRECTION('',(1.,-1.90750687963558E-16,-2.35515798198656E-32));
#116455=DIRECTION('center_axis',(0.,-1.,-1.23467863058847E-16));
#116456=DIRECTION('ref_axis',(-1.,0.,0.));
#116457=DIRECTION('center_axis',(0.,-1.,0.));
#116458=DIRECTION('ref_axis',(0.,0.,1.));
#116459=DIRECTION('',(-3.13111733906369E-16,1.,1.23467863058847E-16));
#116460=DIRECTION('',(3.13111733906369E-16,-1.,-1.23467863058847E-16));
#116461=DIRECTION('center_axis',(0.,1.23467863058847E-16,-1.));
#116462=DIRECTION('ref_axis',(0.,1.,0.));
#116463=DIRECTION('center_axis',(0.,-1.,0.));
#116464=DIRECTION('ref_axis',(0.,0.,1.));
#116465=DIRECTION('center_axis',(0.,0.,1.));
#116466=DIRECTION('ref_axis',(0.,1.,0.));
#116467=DIRECTION('center_axis',(0.,0.,-1.));
#116468=DIRECTION('ref_axis',(0.,1.,0.));
#116469=DIRECTION('center_axis',(0.,1.23467863058847E-16,-1.));
#116470=DIRECTION('ref_axis',(0.,1.,0.));
#116471=DIRECTION('center_axis',(0.999913989288144,-0.0131154117689341,
0.));
#116472=DIRECTION('ref_axis',(0.0131154117689341,0.999913989288144,0.));
#116473=DIRECTION('center_axis',(0.,0.,-1.));
#116474=DIRECTION('ref_axis',(0.,1.,0.));
#116475=DIRECTION('center_axis',(0.,0.,1.));
#116476=DIRECTION('ref_axis',(0.,1.,0.));
#116477=DIRECTION('center_axis',(-6.11546355285877E-17,1.,0.));
#116478=DIRECTION('ref_axis',(0.,0.,1.));
#116479=DIRECTION('center_axis',(0.,-1.,0.));
#116480=DIRECTION('ref_axis',(0.,0.,1.));
#116481=DIRECTION('',(-6.11546355285877E-17,1.,1.23467863058847E-16));
#116482=DIRECTION('',(6.11546355285877E-17,-1.,-1.23467863058847E-16));
#116483=DIRECTION('center_axis',(0.,1.23467863058847E-16,-1.));
#116484=DIRECTION('ref_axis',(0.,1.,1.25697703075927E-16));
#116485=DIRECTION('center_axis',(0.999998293848715,-0.00184724109421639,
0.));
#116486=DIRECTION('ref_axis',(0.00184724109421639,0.999998293848714,0.));
#116487=DIRECTION('center_axis',(0.,1.22833149346405E-16,-1.));
#116488=DIRECTION('ref_axis',(0.,1.,1.22833149346405E-16));
#116489=DIRECTION('center_axis',(0.,-1.22914743790472E-16,1.));
#116490=DIRECTION('ref_axis',(0.,1.,1.22914743790472E-16));
#116491=DIRECTION('center_axis',(0.,1.23467863058847E-16,-1.));
#116492=DIRECTION('ref_axis',(0.706453380948024,-0.707759578209371,0.));
#116493=DIRECTION('center_axis',(0.,0.,-1.));
#116494=DIRECTION('ref_axis',(0.,1.,0.));
#116495=DIRECTION('center_axis',(0.,0.,1.));
#116496=DIRECTION('ref_axis',(0.,1.,0.));
#116497=DIRECTION('center_axis',(0.,1.23467863058847E-16,-1.));
#116498=DIRECTION('ref_axis',(0.,1.,0.));
#116499=DIRECTION('center_axis',(0.,1.,0.));
#116500=DIRECTION('ref_axis',(0.,0.,-1.));
#116501=DIRECTION('center_axis',(0.,0.,-1.));
#116502=DIRECTION('ref_axis',(0.,1.,0.));
#116503=DIRECTION('center_axis',(-1.,4.81867632215781E-16,-7.43028527927166E-30));
#116504=DIRECTION('ref_axis',(-4.81867632215781E-16,-1.,-1.36218908067985E-60));
#116505=DIRECTION('center_axis',(0.,0.,1.));
#116506=DIRECTION('ref_axis',(0.,1.,0.));
#116507=DIRECTION('center_axis',(-1.,0.,7.06547394595967E-32));
#116508=DIRECTION('ref_axis',(0.,1.,0.));
#116509=DIRECTION('center_axis',(-1.,0.,0.));
#116510=DIRECTION('ref_axis',(0.,0.,1.));
#116511=DIRECTION('',(1.,-5.72252063890675E-16,-7.06547394595967E-32));
#116512=DIRECTION('',(-1.,5.72252063890675E-16,7.06547394595967E-32));
#116513=DIRECTION('center_axis',(-6.11546355285877E-17,1.,0.));
#116514=DIRECTION('ref_axis',(0.,0.,1.));
#116515=DIRECTION('center_axis',(0.,1.,0.));
#116516=DIRECTION('ref_axis',(0.,0.,-1.));
#116517=DIRECTION('',(6.11546355285877E-17,-1.,-1.23467863058847E-16));
#116518=DIRECTION('',(-6.11546355285877E-17,1.,1.23467863058847E-16));
#116519=DIRECTION('center_axis',(0.,1.23467863058847E-16,-1.));
#116520=DIRECTION('ref_axis',(0.,1.,0.));
#116521=DIRECTION('center_axis',(0.,1.,0.));
#116522=DIRECTION('ref_axis',(0.,0.,-1.));
#116523=DIRECTION('center_axis',(0.,0.,1.));
#116524=DIRECTION('ref_axis',(0.,1.,0.));
#116525=DIRECTION('center_axis',(1.78485500480727E-31,2.58019156504489E-46,
-1.));
#116526=DIRECTION('ref_axis',(-1.44560289664734E-15,1.,-3.88938454866321E-62));
#116527=DIRECTION('center_axis',(0.,1.23467863058847E-16,-1.));
#116528=DIRECTION('ref_axis',(0.,1.,0.));
#116529=DIRECTION('center_axis',(-1.,-4.81867632215781E-16,0.));
#116530=DIRECTION('ref_axis',(4.81867632215781E-16,-1.,0.));
#116531=DIRECTION('center_axis',(0.,0.,-1.));
#116532=DIRECTION('ref_axis',(0.,1.,0.));
#116533=DIRECTION('center_axis',(0.,0.,1.));
#116534=DIRECTION('ref_axis',(0.,1.,0.));
#116535=DIRECTION('center_axis',(0.,-1.,-1.23467863058847E-16));
#116536=DIRECTION('ref_axis',(-1.,0.,0.));
#116537=DIRECTION('center_axis',(0.,1.,0.));
#116538=DIRECTION('ref_axis',(0.,0.,-1.));
#116539=DIRECTION('',(3.13111733906369E-16,-1.,-1.23467863058847E-16));
#116540=DIRECTION('',(-3.13111733906369E-16,1.,1.23467863058847E-16));
#116541=DIRECTION('center_axis',(1.,0.,4.07299888683445E-32));
#116542=DIRECTION('ref_axis',(0.,-1.,0.));
#116543=DIRECTION('center_axis',(-1.,0.,0.));
#116544=DIRECTION('ref_axis',(0.,0.,1.));
#116545=DIRECTION('',(1.,3.29883322342202E-16,4.07299888683446E-32));
#116546=DIRECTION('',(-1.,-3.29883322342202E-16,-4.07299888683446E-32));
#116547=DIRECTION('center_axis',(0.,1.23467863058847E-16,-1.));
#116548=DIRECTION('ref_axis',(0.,1.,0.));
#116549=DIRECTION('center_axis',(0.,0.,-1.));
#116550=DIRECTION('ref_axis',(0.,1.,0.));
#116551=DIRECTION('center_axis',(0.,0.,1.));
#116552=DIRECTION('ref_axis',(0.,1.,0.));
#116553=DIRECTION('center_axis',(0.,1.23467863058847E-16,-1.));
#116554=DIRECTION('ref_axis',(0.,1.,0.));
#116555=DIRECTION('center_axis',(0.699822617100543,-0.714316669688274,0.));
#116556=DIRECTION('ref_axis',(0.714316669688274,0.699822617100543,0.));
#116557=DIRECTION('center_axis',(0.,0.,-1.));
#116558=DIRECTION('ref_axis',(0.,1.,0.));
#116559=DIRECTION('center_axis',(1.,0.,0.));
#116560=DIRECTION('ref_axis',(0.,0.,-1.));
#116561=DIRECTION('center_axis',(0.,0.,1.));
#116562=DIRECTION('ref_axis',(0.,1.,0.));
#116563=DIRECTION('center_axis',(1.,0.,-2.35515798198655E-32));
#116564=DIRECTION('ref_axis',(0.,-1.,0.));
#116565=DIRECTION('center_axis',(1.,0.,0.));
#116566=DIRECTION('ref_axis',(0.,0.,-1.));
#116567=DIRECTION('',(-1.,1.90750687963558E-16,2.35515798198656E-32));
#116568=DIRECTION('',(1.,-1.90750687963558E-16,-2.35515798198656E-32));
#116569=DIRECTION('center_axis',(0.,1.23467863058847E-16,-1.));
#116570=DIRECTION('ref_axis',(0.,1.,0.));
#116571=DIRECTION('center_axis',(0.74298130529014,-0.669312169312168,0.));
#116572=DIRECTION('ref_axis',(0.669312169312168,0.742981305290139,0.));
#116573=DIRECTION('center_axis',(0.,0.,-1.));
#116574=DIRECTION('ref_axis',(0.,1.,0.));
#116575=DIRECTION('center_axis',(0.,0.,1.));
#116576=DIRECTION('ref_axis',(0.,1.,0.));
#116577=DIRECTION('center_axis',(0.,1.23467863058847E-16,-1.));
#116578=DIRECTION('ref_axis',(0.,1.,0.));
#116579=DIRECTION('center_axis',(0.,-1.,0.));
#116580=DIRECTION('ref_axis',(0.,0.,1.));
#116581=DIRECTION('center_axis',(0.,0.,1.));
#116582=DIRECTION('ref_axis',(0.,1.,0.));
#116583=DIRECTION('center_axis',(0.,0.,-1.));
#116584=DIRECTION('ref_axis',(0.,1.,0.));
#116585=DIRECTION('center_axis',(0.,1.23467863058847E-16,-1.));
#116586=DIRECTION('ref_axis',(0.406625030395211,-0.913595142640379,0.));
#116587=DIRECTION('center_axis',(0.,1.,0.));
#116588=DIRECTION('ref_axis',(0.,0.,-1.));
#116589=DIRECTION('center_axis',(0.,0.,-1.));
#116590=DIRECTION('ref_axis',(0.,1.,0.));
#116591=DIRECTION('center_axis',(0.,0.,1.));
#116592=DIRECTION('ref_axis',(0.,1.,0.));
#116593=DIRECTION('center_axis',(0.,1.,0.));
#116594=DIRECTION('ref_axis',(0.,0.,1.));
#116595=DIRECTION('',(0.,-1.,-1.23467863058847E-16));
#116596=DIRECTION('',(0.,1.,1.23467863058847E-16));
#116597=DIRECTION('center_axis',(0.,1.23467863058847E-16,-1.));
#116598=DIRECTION('ref_axis',(0.,1.,0.));
#116599=DIRECTION('center_axis',(0.,0.,-1.));
#116600=DIRECTION('ref_axis',(0.,1.,0.));
#116601=DIRECTION('center_axis',(0.,-1.,0.));
#116602=DIRECTION('ref_axis',(0.,0.,1.));
#116603=DIRECTION('center_axis',(0.,0.,1.));
#116604=DIRECTION('ref_axis',(0.,1.,0.));
#116605=DIRECTION('center_axis',(-0.742981305290128,-0.669312169312181,
0.));
#116606=DIRECTION('ref_axis',(0.669312169312181,-0.742981305290128,0.));
#116607=DIRECTION('center_axis',(0.,1.,0.));
#116608=DIRECTION('ref_axis',(0.,0.,1.));
#116609=DIRECTION('center_axis',(0.,-1.,0.));
#116610=DIRECTION('ref_axis',(0.,0.,1.));
#116611=DIRECTION('',(0.,1.,1.23467863058847E-16));
#116612=DIRECTION('',(0.,-1.,-1.23467863058847E-16));
#116613=DIRECTION('center_axis',(0.,1.23467863058847E-16,-1.));
#116614=DIRECTION('ref_axis',(0.,1.,0.));
#116615=DIRECTION('center_axis',(-0.699822617100527,-0.714316669688289,
0.));
#116616=DIRECTION('ref_axis',(0.714316669688289,-0.699822617100527,0.));
#116617=DIRECTION('center_axis',(-1.20627640644894E-30,1.17852753964151E-44,
-1.));
#116618=DIRECTION('ref_axis',(9.76996261670138E-15,1.,-4.97841222228891E-60));
#116619=DIRECTION('center_axis',(0.,0.,1.));
#116620=DIRECTION('ref_axis',(0.,1.,0.));
#116621=DIRECTION('center_axis',(0.,1.23467863058847E-16,-1.));
#116622=DIRECTION('ref_axis',(0.,1.,0.));
#116623=DIRECTION('center_axis',(-1.,0.,0.));
#116624=DIRECTION('ref_axis',(0.,0.,1.));
#116625=DIRECTION('center_axis',(0.,0.,1.));
#116626=DIRECTION('ref_axis',(0.,1.,0.));
#116627=DIRECTION('center_axis',(0.,0.,-1.));
#116628=DIRECTION('ref_axis',(0.,1.,0.));
#116629=DIRECTION('center_axis',(0.,1.23467863058847E-16,-1.));
#116630=DIRECTION('ref_axis',(0.,1.,0.));
#116631=DIRECTION('center_axis',(1.,0.,0.));
#116632=DIRECTION('ref_axis',(0.,0.,-1.));
#116633=DIRECTION('center_axis',(0.,0.,-1.));
#116634=DIRECTION('ref_axis',(0.,1.,0.));
#116635=DIRECTION('center_axis',(0.,0.,1.));
#116636=DIRECTION('ref_axis',(0.,1.,0.));
#116637=DIRECTION('center_axis',(-1.,0.,-1.17757899099328E-32));
#116638=DIRECTION('ref_axis',(0.,1.,0.));
#116639=DIRECTION('',(-1.,-9.53753439817791E-17,-1.17757899099328E-32));
#116640=DIRECTION('',(1.,9.53753439817791E-17,1.17757899099328E-32));
#116641=DIRECTION('center_axis',(0.,1.23467863058847E-16,-1.));
#116642=DIRECTION('ref_axis',(0.,1.,0.));
#116643=DIRECTION('center_axis',(-0.87305990868679,0.487612957009772,0.));
#116644=DIRECTION('ref_axis',(-0.487612957009772,-0.87305990868679,0.));
#116645=DIRECTION('center_axis',(0.,0.,1.));
#116646=DIRECTION('ref_axis',(0.,1.,0.));
#116647=DIRECTION('center_axis',(-0.999425898115847,0.0338802918424838,
-7.7054558576033E-15));
#116648=DIRECTION('ref_axis',(-0.0338802918424838,-0.999425898115847,2.67737997453887E-33));
#116649=DIRECTION('center_axis',(0.,0.,-1.));
#116650=DIRECTION('ref_axis',(0.,1.,0.));
#116651=DIRECTION('center_axis',(0.,1.23467863058847E-16,-1.));
#116652=DIRECTION('ref_axis',(0.,1.,0.));
#116653=DIRECTION('center_axis',(-0.55837318130784,0.829589892896582,0.));
#116654=DIRECTION('ref_axis',(-0.829589892896582,-0.55837318130784,0.));
#116655=DIRECTION('center_axis',(0.,0.,1.));
#116656=DIRECTION('ref_axis',(0.,1.,0.));
#116657=DIRECTION('center_axis',(4.38645965981435E-31,1.5583835234929E-45,
-1.));
#116658=DIRECTION('ref_axis',(-3.5527136788005E-15,1.,-1.24460305557223E-60));
#116659=DIRECTION('center_axis',(0.,1.23467863058847E-16,-1.));
#116660=DIRECTION('ref_axis',(0.,1.,0.));
#116661=DIRECTION('center_axis',(-0.03879684915621,0.999247118832749,5.83634271056011E-15));
#116662=DIRECTION('ref_axis',(-0.999247118832749,-0.03879684915621,-4.4574149748685E-34));
#116663=DIRECTION('center_axis',(0.,0.,1.));
#116664=DIRECTION('ref_axis',(0.,1.,0.));
#116665=DIRECTION('center_axis',(6.64132094812011E-31,3.57235825122499E-45,
-1.));
#116666=DIRECTION('ref_axis',(-5.37898752240871E-15,1.,2.61366641670168E-59));
#116667=DIRECTION('center_axis',(0.,1.23467863058847E-16,-1.));
#116668=DIRECTION('ref_axis',(0.,1.,1.24777965780772E-16));
#116669=DIRECTION('center_axis',(0.0387968491562139,0.999247118832749,0.));
#116670=DIRECTION('ref_axis',(-0.999247118832749,0.0387968491562139,0.));
#116671=DIRECTION('center_axis',(0.,-1.22014183466588E-16,1.));
#116672=DIRECTION('ref_axis',(0.,1.,1.22014183466588E-16));
#116673=DIRECTION('center_axis',(4.09030343683335E-32,1.21933779888604E-16,
-1.));
#116674=DIRECTION('ref_axis',(-2.66628532023081E-14,1.,1.21933779888604E-16));
#116675=DIRECTION('center_axis',(0.,1.23467863058847E-16,-1.));
#116676=DIRECTION('ref_axis',(0.,1.,0.));
#116677=DIRECTION('center_axis',(0.55837318130784,0.829589892896582,0.));
#116678=DIRECTION('ref_axis',(-0.829589892896582,0.55837318130784,0.));
#116679=DIRECTION('center_axis',(0.,0.,1.));
#116680=DIRECTION('ref_axis',(0.,1.,0.));
#116681=DIRECTION('center_axis',(-1.32826418962402E-31,1.42894330048999E-46,
-1.));
#116682=DIRECTION('ref_axis',(1.07579750448174E-15,1.,9.14005368935855E-61));
#116683=DIRECTION('center_axis',(0.,1.23467863058847E-16,-1.));
#116684=DIRECTION('ref_axis',(0.,1.,0.));
#116685=DIRECTION('center_axis',(0.848949186868297,0.528474481991002,8.14895191435076E-15));
#116686=DIRECTION('ref_axis',(-0.528474481991002,0.848949186868297,-1.25969070483717E-30));
#116687=DIRECTION('center_axis',(0.,0.,1.));
#116688=DIRECTION('ref_axis',(0.,1.,0.));
#116689=DIRECTION('center_axis',(-1.53526088093502E-30,1.90901981627881E-44,
-1.));
#116690=DIRECTION('ref_axis',(1.24344978758017E-14,1.,2.98704733337335E-59));
#116691=DIRECTION('center_axis',(0.,1.23467863058847E-16,-1.));
#116692=DIRECTION('ref_axis',(0.,1.,0.));
#116693=DIRECTION('center_axis',(0.992522955047552,0.122058116090968,0.));
#116694=DIRECTION('ref_axis',(-0.122058116090968,0.992522955047552,0.));
#116695=DIRECTION('center_axis',(0.,0.,1.));
#116696=DIRECTION('ref_axis',(0.,1.,0.));
#116697=DIRECTION('center_axis',(-1.32826418962402E-31,1.42894330048999E-46,
-1.));
#116698=DIRECTION('ref_axis',(1.07579750448174E-15,1.,5.05619991326218E-61));
#116699=DIRECTION('center_axis',(0.,1.23467863058847E-16,-1.));
#116700=DIRECTION('ref_axis',(0.,1.,0.));
#116701=DIRECTION('center_axis',(-0.87305990868679,0.487612957009772,0.));
#116702=DIRECTION('ref_axis',(-0.487612957009772,-0.87305990868679,0.));
#116703=DIRECTION('center_axis',(0.,0.,1.));
#116704=DIRECTION('ref_axis',(0.,1.,0.));
#116705=DIRECTION('center_axis',(-0.999425898115848,0.0338802918424761,
0.));
#116706=DIRECTION('ref_axis',(-0.0338802918424761,-0.999425898115848,0.));
#116707=DIRECTION('center_axis',(-4.46213751201822E-31,1.61261972815309E-45,
-1.));
#116708=DIRECTION('ref_axis',(3.61400724161835E-15,1.,1.6490990486332E-59));
#116709=DIRECTION('center_axis',(0.,1.23467863058847E-16,-1.));
#116710=DIRECTION('ref_axis',(0.,1.,0.));
#116711=DIRECTION('center_axis',(-0.55837318130784,0.829589892896582,0.));
#116712=DIRECTION('ref_axis',(-0.829589892896582,-0.55837318130784,0.));
#116713=DIRECTION('center_axis',(0.,0.,1.));
#116714=DIRECTION('ref_axis',(0.,1.,0.));
#116715=DIRECTION('center_axis',(4.38645965981435E-31,1.5583835234929E-45,
-1.));
#116716=DIRECTION('ref_axis',(-3.5527136788005E-15,1.,-1.24460305557223E-60));
#116717=DIRECTION('center_axis',(0.,1.23467863058847E-16,-1.));
#116718=DIRECTION('ref_axis',(0.,1.,0.));
#116719=DIRECTION('center_axis',(-0.0387968491561946,0.99924711883275,0.));
#116720=DIRECTION('ref_axis',(-0.99924711883275,-0.0387968491561946,0.));
#116721=DIRECTION('center_axis',(0.,0.,1.));
#116722=DIRECTION('ref_axis',(0.,1.,0.));
#116723=DIRECTION('center_axis',(-8.92427502403635E-31,6.45047891261223E-45,
-1.));
#116724=DIRECTION('ref_axis',(7.2280144832367E-15,1.,3.73380916671669E-60));
#116725=DIRECTION('center_axis',(0.,1.23467863058847E-16,-1.));
#116726=DIRECTION('ref_axis',(0.,1.,1.25162611019057E-16));
#116727=DIRECTION('center_axis',(0.0387968491562177,0.999247118832749,0.));
#116728=DIRECTION('ref_axis',(-0.999247118832749,0.0387968491562177,0.));
#116729=DIRECTION('center_axis',(0.,-1.22309905988566E-16,1.));
#116730=DIRECTION('ref_axis',(0.,1.,1.22309905988566E-16));
#116731=DIRECTION('center_axis',(3.29067448743359E-32,1.22229112323298E-16,
-1.));
#116732=DIRECTION('ref_axis',(-2.65644604115968E-14,1.,1.22229112323298E-16));
#116733=DIRECTION('center_axis',(0.,1.23467863058847E-16,-1.));
#116734=DIRECTION('ref_axis',(0.,1.,0.));
#116735=DIRECTION('center_axis',(0.55837318130784,0.829589892896582,0.));
#116736=DIRECTION('ref_axis',(-0.829589892896582,0.55837318130784,0.));
#116737=DIRECTION('center_axis',(0.,0.,1.));
#116738=DIRECTION('ref_axis',(0.,1.,0.));
#116739=DIRECTION('center_axis',(0.,0.,-1.));
#116740=DIRECTION('ref_axis',(0.,1.,0.));
#116741=DIRECTION('center_axis',(0.,1.23467863058847E-16,-1.));
#116742=DIRECTION('ref_axis',(0.,1.,0.));
#116743=DIRECTION('center_axis',(0.848949186868305,0.528474481990989,0.));
#116744=DIRECTION('ref_axis',(-0.528474481990989,0.848949186868305,0.));
#116745=DIRECTION('center_axis',(0.,0.,1.));
#116746=DIRECTION('ref_axis',(0.,1.,0.));
#116747=DIRECTION('center_axis',(-1.53526088093502E-30,1.90901981627881E-44,
-1.));
#116748=DIRECTION('ref_axis',(1.24344978758017E-14,1.,3.23596794448779E-59));
#116749=DIRECTION('center_axis',(0.,1.23467863058847E-16,-1.));
#116750=DIRECTION('ref_axis',(0.,1.,0.));
#116751=DIRECTION('center_axis',(0.992522955047553,0.12205811609096,0.));
#116752=DIRECTION('ref_axis',(-0.12205811609096,0.992522955047552,0.));
#116753=DIRECTION('center_axis',(0.,0.,1.));
#116754=DIRECTION('ref_axis',(0.,1.,0.));
#116755=DIRECTION('center_axis',(1.42788400384582E-30,1.65132260162873E-44,
-1.));
#116756=DIRECTION('ref_axis',(-1.15648231731787E-14,1.,-2.48920611114446E-60));
#116757=DIRECTION('center_axis',(0.,1.23467863058847E-16,-1.));
#116758=DIRECTION('ref_axis',(0.,1.,0.));
#116759=DIRECTION('center_axis',(-0.689680595319751,0.724113717892013,0.));
#116760=DIRECTION('ref_axis',(-0.724113717892013,-0.689680595319751,0.));
#116761=DIRECTION('center_axis',(0.,0.,-1.));
#116762=DIRECTION('ref_axis',(0.,1.,0.));
#116763=DIRECTION('center_axis',(0.,0.,1.));
#116764=DIRECTION('ref_axis',(0.,1.,0.));
#116765=DIRECTION('center_axis',(0.68968059531976,-0.724113717892004,-8.94047733597239E-17));
#116766=DIRECTION('ref_axis',(-0.724113717892004,-0.68968059531976,2.34589631629098E-32));
#116767=DIRECTION('center_axis',(-0.689680595319751,0.724113717892013,0.));
#116768=DIRECTION('ref_axis',(-0.724113717892013,-0.689680595319751,0.));
#116769=DIRECTION('',(0.689680595319752,-0.724113717892012,-8.94047733597238E-17));
#116770=DIRECTION('',(-0.689680595319752,0.724113717892012,8.94047733597238E-17));
#116771=DIRECTION('center_axis',(0.,1.23467863058847E-16,-1.));
#116772=DIRECTION('ref_axis',(0.,1.,0.));
#116773=DIRECTION('center_axis',(0.,0.,-1.));
#116774=DIRECTION('ref_axis',(0.,1.,0.));
#116775=DIRECTION('center_axis',(0.,0.,1.));
#116776=DIRECTION('ref_axis',(0.,1.,0.));
#116777=DIRECTION('center_axis',(-0.635568809204586,-0.772044227208691,
0.));
#116778=DIRECTION('ref_axis',(0.772044227208691,-0.635568809204586,0.));
#116779=DIRECTION('center_axis',(0.,1.23467863058847E-16,-1.));
#116780=DIRECTION('ref_axis',(0.,1.,0.));
#116781=DIRECTION('center_axis',(-0.120708341042265,-0.992688015643799,
0.));
#116782=DIRECTION('ref_axis',(0.992688015643799,-0.120708341042265,0.));
#116783=DIRECTION('center_axis',(-2.19322982990717E-31,3.89595880873225E-46,
-1.));
#116784=DIRECTION('ref_axis',(1.77635683940025E-15,1.,7.77876909732643E-62));
#116785=DIRECTION('center_axis',(0.,0.,1.));
#116786=DIRECTION('ref_axis',(0.,1.,0.));
#116787=DIRECTION('center_axis',(0.,1.23467863058847E-16,-1.));
#116788=DIRECTION('ref_axis',(0.,1.,0.));
#116789=DIRECTION('center_axis',(1.,0.,0.));
#116790=DIRECTION('ref_axis',(0.,0.,-1.));
#116791=DIRECTION('center_axis',(0.,0.,-1.));
#116792=DIRECTION('ref_axis',(0.,1.,0.));
#116793=DIRECTION('center_axis',(0.,0.,1.));
#116794=DIRECTION('ref_axis',(0.,1.,0.));
#116795=DIRECTION('center_axis',(-1.,0.,4.58212374768871E-32));
#116796=DIRECTION('ref_axis',(0.,1.,0.));
#116797=DIRECTION('center_axis',(1.,0.,0.));
#116798=DIRECTION('ref_axis',(0.,0.,-1.));
#116799=DIRECTION('',(-1.,3.71118737634973E-16,4.58212374768871E-32));
#116800=DIRECTION('',(1.,-3.71118737634973E-16,-4.58212374768871E-32));
#116801=DIRECTION('center_axis',(0.,1.23467863058847E-16,-1.));
#116802=DIRECTION('ref_axis',(0.,1.,0.));
#116803=DIRECTION('center_axis',(0.,0.,-1.));
#116804=DIRECTION('ref_axis',(0.,1.,0.));
#116805=DIRECTION('center_axis',(0.,0.,1.));
#116806=DIRECTION('ref_axis',(0.,1.,0.));
#116807=DIRECTION('center_axis',(0.,1.23467863058847E-16,-1.));
#116808=DIRECTION('ref_axis',(0.,1.,0.));
#116809=DIRECTION('center_axis',(-1.,0.,0.));
#116810=DIRECTION('ref_axis',(0.,0.,1.));
#116811=DIRECTION('center_axis',(0.,0.,-1.));
#116812=DIRECTION('ref_axis',(0.,1.,0.));
#116813=DIRECTION('center_axis',(0.,0.,1.));
#116814=DIRECTION('ref_axis',(0.,1.,0.));
#116815=DIRECTION('center_axis',(1.,0.,4.58212374768871E-32));
#116816=DIRECTION('ref_axis',(0.,-1.,0.));
#116817=DIRECTION('center_axis',(-1.,0.,0.));
#116818=DIRECTION('ref_axis',(0.,0.,1.));
#116819=DIRECTION('',(1.,3.71118737634973E-16,4.58212374768871E-32));
#116820=DIRECTION('',(-1.,-3.71118737634973E-16,-4.58212374768871E-32));
#116821=DIRECTION('center_axis',(0.,1.23467863058847E-16,-1.));
#116822=DIRECTION('ref_axis',(0.,1.,0.));
#116823=DIRECTION('center_axis',(0.120708341042269,-0.992688015643799,0.));
#116824=DIRECTION('ref_axis',(0.992688015643799,0.120708341042269,0.));
#116825=DIRECTION('center_axis',(1.78485500480727E-31,2.58019156504489E-46,
-1.));
#116826=DIRECTION('ref_axis',(-1.44560289664734E-15,1.,-3.88938454866321E-62));
#116827=DIRECTION('center_axis',(0.,0.,1.));
#116828=DIRECTION('ref_axis',(0.,1.,0.));
#116829=DIRECTION('center_axis',(0.,1.23467863058847E-16,-1.));
#116830=DIRECTION('ref_axis',(0.,1.,0.));
#116831=DIRECTION('center_axis',(0.635568809204587,-0.77204422720869,0.));
#116832=DIRECTION('ref_axis',(0.77204422720869,0.635568809204587,0.));
#116833=DIRECTION('center_axis',(6.57968948972152E-31,3.50636292785902E-45,
-1.));
#116834=DIRECTION('ref_axis',(-5.32907051820075E-15,1.,-4.3561106945028E-60));
#116835=DIRECTION('center_axis',(0.,0.,1.));
#116836=DIRECTION('ref_axis',(0.,1.,0.));
#116837=DIRECTION('center_axis',(0.,1.23467863058847E-16,-1.));
#116838=DIRECTION('ref_axis',(-0.0361435302645206,-0.999346609150208,0.));
#116839=DIRECTION('center_axis',(0.689680595319753,0.724113717892011,0.));
#116840=DIRECTION('ref_axis',(-0.724113717892011,0.689680595319753,0.));
#116841=DIRECTION('center_axis',(1.78485500480727E-31,2.58019156504489E-46,
-1.));
#116842=DIRECTION('ref_axis',(-1.44560289664734E-15,1.,-3.88938454866321E-62));
#116843=DIRECTION('center_axis',(0.,0.,1.));
#116844=DIRECTION('ref_axis',(0.,1.,0.));
#116845=DIRECTION('center_axis',(-0.689680595319751,-0.724113717892013,
-8.9404773359724E-17));
#116846=DIRECTION('ref_axis',(-0.724113717892013,0.689680595319751,4.19197973383322E-33));
#116847=DIRECTION('center_axis',(0.689680595319753,0.724113717892011,0.));
#116848=DIRECTION('ref_axis',(-0.724113717892011,0.689680595319753,0.));
#116849=DIRECTION('',(-0.689680595319751,-0.724113717892013,-8.9404773359724E-17));
#116850=DIRECTION('',(0.689680595319751,0.724113717892013,8.9404773359724E-17));
#116851=DIRECTION('center_axis',(0.,1.23467863058847E-16,-1.));
#116852=DIRECTION('ref_axis',(0.,1.,0.));
#116853=DIRECTION('center_axis',(-8.92427502403635E-32,6.45047891261222E-47,
-1.));
#116854=DIRECTION('ref_axis',(7.2280144832367E-16,1.,-6.80642296016062E-62));
#116855=DIRECTION('center_axis',(0.,0.,1.));
#116856=DIRECTION('ref_axis',(0.,1.,0.));
#116857=DIRECTION('center_axis',(0.,1.23467863058847E-16,-1.));
#116858=DIRECTION('ref_axis',(0.,1.,0.));
#116859=DIRECTION('center_axis',(1.92747052886312E-15,1.,0.));
#116860=DIRECTION('ref_axis',(-1.,1.92747052886312E-15,0.));
#116861=DIRECTION('center_axis',(0.,0.,-1.));
#116862=DIRECTION('ref_axis',(0.,1.,0.));
#116863=DIRECTION('center_axis',(0.,0.,1.));
#116864=DIRECTION('ref_axis',(0.,1.,0.));
#116865=DIRECTION('center_axis',(-6.11546355285877E-17,1.,0.));
#116866=DIRECTION('ref_axis',(0.,0.,1.));
#116867=DIRECTION('center_axis',(0.,1.,0.));
#116868=DIRECTION('ref_axis',(0.,0.,-1.));
#116869=DIRECTION('',(6.11546355285877E-17,-1.,-1.23467863058847E-16));
#116870=DIRECTION('',(-6.11546355285877E-17,1.,1.23467863058847E-16));
#116871=DIRECTION('center_axis',(0.,1.23467863058847E-16,-1.));
#116872=DIRECTION('ref_axis',(0.,1.,0.));
#116873=DIRECTION('center_axis',(0.,0.,-1.));
#116874=DIRECTION('ref_axis',(0.,1.,0.));
#116875=DIRECTION('center_axis',(0.,0.,1.));
#116876=DIRECTION('ref_axis',(0.,1.,0.));
#116877=DIRECTION('center_axis',(-0.992688015643799,-0.120708341042267,
-1.45413606216828E-17));
#116878=DIRECTION('ref_axis',(0.120708341042267,-0.992688015643799,-1.06337197076866E-33));
#116879=DIRECTION('center_axis',(0.,1.23467863058847E-16,-1.));
#116880=DIRECTION('ref_axis',(0.,1.,0.));
#116881=DIRECTION('center_axis',(-0.802069210224766,-0.597231095983306,
0.));
#116882=DIRECTION('ref_axis',(0.597231095983306,-0.802069210224766,0.));
#116883=DIRECTION('center_axis',(8.77291931962869E-31,6.2335340939716E-45,
-1.));
#116884=DIRECTION('ref_axis',(-7.105427357601E-15,1.,-4.97841222228891E-60));
#116885=DIRECTION('center_axis',(0.,0.,1.));
#116886=DIRECTION('ref_axis',(0.,1.,0.));
#116887=DIRECTION('center_axis',(0.,1.23467863058847E-16,-1.));
#116888=DIRECTION('ref_axis',(0.,1.,0.));
#116889=DIRECTION('center_axis',(0.689680595319753,-0.724113717892012,0.));
#116890=DIRECTION('ref_axis',(0.724113717892012,0.689680595319752,0.));
#116891=DIRECTION('center_axis',(0.,0.,-1.));
#116892=DIRECTION('ref_axis',(0.,1.,0.));
#116893=DIRECTION('center_axis',(0.,0.,1.));
#116894=DIRECTION('ref_axis',(0.,1.,0.));
#116895=DIRECTION('center_axis',(-0.68968059531976,0.724113717892004,8.94047733597239E-17));
#116896=DIRECTION('ref_axis',(0.724113717892004,0.68968059531976,-2.34589631629098E-32));
#116897=DIRECTION('center_axis',(0.689680595319752,-0.724113717892012,0.));
#116898=DIRECTION('ref_axis',(0.724113717892012,0.689680595319752,0.));
#116899=DIRECTION('',(-0.689680595319752,0.724113717892012,8.94047733597238E-17));
#116900=DIRECTION('',(0.689680595319752,-0.724113717892012,-8.94047733597238E-17));
#116901=DIRECTION('center_axis',(0.,1.23467863058847E-16,-1.));
#116902=DIRECTION('ref_axis',(-0.0950205176920742,-0.995475314218052,0.));
#116903=DIRECTION('center_axis',(0.,0.,-1.));
#116904=DIRECTION('ref_axis',(0.,1.,0.));
#116905=DIRECTION('center_axis',(0.,0.,1.));
#116906=DIRECTION('ref_axis',(0.,1.,0.));
#116907=DIRECTION('center_axis',(0.,1.23467863058847E-16,-1.));
#116908=DIRECTION('ref_axis',(0.,1.,0.));
#116909=DIRECTION('center_axis',(0.,0.,1.));
#116910=DIRECTION('ref_axis',(0.,1.,0.));
#116911=DIRECTION('center_axis',(-0.689680595319753,-0.724113717892011,
0.));
#116912=DIRECTION('ref_axis',(0.724113717892011,-0.689680595319753,0.));
#116913=DIRECTION('center_axis',(-1.60636950432654E-30,2.08995516768636E-44,
-1.));
#116914=DIRECTION('ref_axis',(1.30104260698261E-14,1.,2.24028550003001E-59));
#116915=DIRECTION('center_axis',(0.689680595319751,0.724113717892013,8.9404773359724E-17));
#116916=DIRECTION('ref_axis',(0.724113717892013,-0.689680595319751,-4.19197973383322E-33));
#116917=DIRECTION('center_axis',(-0.689680595319752,-0.724113717892012,
0.));
#116918=DIRECTION('ref_axis',(0.724113717892012,-0.689680595319752,0.));
#116919=DIRECTION('',(0.689680595319751,0.724113717892013,8.9404773359724E-17));
#116920=DIRECTION('',(-0.689680595319751,-0.724113717892013,-8.9404773359724E-17));
#116921=DIRECTION('center_axis',(0.,1.23467863058847E-16,-1.));
#116922=DIRECTION('ref_axis',(0.,1.,0.));
#116923=DIRECTION('center_axis',(0.802069210224767,-0.597231095983305,0.));
#116924=DIRECTION('ref_axis',(0.597231095983305,0.802069210224766,0.));
#116925=DIRECTION('center_axis',(0.,0.,-1.));
#116926=DIRECTION('ref_axis',(0.,1.,0.));
#116927=DIRECTION('center_axis',(0.,0.,1.));
#116928=DIRECTION('ref_axis',(0.,1.,0.));
#116929=DIRECTION('center_axis',(0.,1.23467863058847E-16,-1.));
#116930=DIRECTION('ref_axis',(0.,1.,0.));
#116931=DIRECTION('center_axis',(0.992688015643799,-0.120708341042267,0.));
#116932=DIRECTION('ref_axis',(0.120708341042267,0.992688015643799,0.));
#116933=DIRECTION('center_axis',(0.,0.,-1.));
#116934=DIRECTION('ref_axis',(0.,1.,0.));
#116935=DIRECTION('center_axis',(0.,0.,1.));
#116936=DIRECTION('ref_axis',(0.,1.,0.));
#116937=DIRECTION('center_axis',(0.,1.23467863058847E-16,-1.));
#116938=DIRECTION('ref_axis',(0.663057938251906,-0.748568080084325,0.));
#116939=DIRECTION('center_axis',(0.,1.,0.));
#116940=DIRECTION('ref_axis',(0.,0.,-1.));
#116941=DIRECTION('center_axis',(0.,0.,-1.));
#116942=DIRECTION('ref_axis',(0.,1.,0.));
#116943=DIRECTION('center_axis',(0.,0.,1.));
#116944=DIRECTION('ref_axis',(0.,1.,0.));
#116945=DIRECTION('center_axis',(-6.11546355285877E-17,1.,0.));
#116946=DIRECTION('ref_axis',(0.,0.,1.));
#116947=DIRECTION('center_axis',(0.,1.,0.));
#116948=DIRECTION('ref_axis',(0.,0.,-1.));
#116949=DIRECTION('',(6.11546355285877E-17,-1.,-1.23467863058847E-16));
#116950=DIRECTION('',(-6.11546355285877E-17,1.,1.23467863058847E-16));
#116951=DIRECTION('center_axis',(0.,1.23467863058847E-16,-1.));
#116952=DIRECTION('ref_axis',(0.,1.,0.));
#116953=DIRECTION('center_axis',(-2.23106875600908E-31,4.03154932038264E-46,
-1.));
#116954=DIRECTION('ref_axis',(1.80700362080917E-15,1.,2.33363072919793E-61));
#116955=DIRECTION('center_axis',(0.,0.,1.));
#116956=DIRECTION('ref_axis',(0.,1.,0.));
#116957=DIRECTION('center_axis',(0.,-1.23467863058847E-16,1.));
#116958=DIRECTION('ref_axis',(0.,-1.,0.));
#116959=DIRECTION('center_axis',(-0.777162624242383,-0.6292998136665,-1.36800580655942E-15));
#116960=DIRECTION('ref_axis',(0.6292998136665,-0.777162624242383,-6.36525986617897E-32));
#116961=DIRECTION('center_axis',(-7.93261518924905E-31,5.09657996678154E-45,
-1.));
#116962=DIRECTION('ref_axis',(6.42484205421795E-15,1.,4.3561106945028E-60));
#116963=DIRECTION('center_axis',(-0.982297019165463,-0.187330099393146,
-5.41061232187394E-15));
#116964=DIRECTION('ref_axis',(0.187330099393146,-0.982297019165463,5.34128931770042E-31));
#116965=DIRECTION('center_axis',(0.,0.,1.));
#116966=DIRECTION('ref_axis',(0.,-1.,0.));
#116967=DIRECTION('center_axis',(0.,-1.23467863058847E-16,1.));
#116968=DIRECTION('ref_axis',(0.,-1.,0.));
#116969=DIRECTION('center_axis',(-0.6350303583426,-0.772487180465326,0.));
#116970=DIRECTION('ref_axis',(0.772487180465326,-0.6350303583426,0.));
#116971=DIRECTION('center_axis',(-3.28984474486076E-31,8.76590731964757E-46,
-1.));
#116972=DIRECTION('ref_axis',(2.66453525910037E-15,1.,-6.22301527786114E-61));
#116973=DIRECTION('center_axis',(0.,0.,1.));
#116974=DIRECTION('ref_axis',(0.,-1.,0.));
#116975=DIRECTION('center_axis',(0.,-1.23467863058847E-16,1.));
#116976=DIRECTION('ref_axis',(0.,-1.,0.));
#116977=DIRECTION('center_axis',(-0.0394959395290685,-0.999219730970479,
7.30821690739571E-16));
#116978=DIRECTION('ref_axis',(0.999219730970479,-0.0394959395290685,1.49001220711228E-32));
#116979=DIRECTION('center_axis',(-1.22040233680755E-31,1.206291116398E-46,
-1.));
#116980=DIRECTION('ref_axis',(9.88437239110456E-16,1.,0.));
#116981=DIRECTION('center_axis',(-4.09907119868247E-31,-1.3608711024552E-45,
1.));
#116982=DIRECTION('ref_axis',(3.31994990204759E-15,-1.,-9.33452291679171E-61));
#116983=DIRECTION('center_axis',(0.,-1.23467863058847E-16,1.));
#116984=DIRECTION('ref_axis',(0.,-1.,-1.32864206562206E-16));
#116985=DIRECTION('center_axis',(0.0394959395290708,-0.999219730970479,
0.));
#116986=DIRECTION('ref_axis',(0.999219730970479,0.0394959395290708,0.));
#116987=DIRECTION('center_axis',(2.45193654393607E-31,1.29750229435012E-16,
-1.));
#116988=DIRECTION('ref_axis',(3.90288690140516E-14,1.,1.29750229435012E-16));
#116989=DIRECTION('center_axis',(0.,-1.29932421951445E-16,1.));
#116990=DIRECTION('ref_axis',(0.,-1.,-1.29932421951445E-16));
#116991=DIRECTION('center_axis',(0.,-1.23467863058847E-16,1.));
#116992=DIRECTION('ref_axis',(0.,-1.,0.));
#116993=DIRECTION('center_axis',(0.6350303583426,-0.772487180465326,1.66587444809586E-15));
#116994=DIRECTION('ref_axis',(0.772487180465326,0.6350303583426,9.8727026228538E-31));
#116995=DIRECTION('center_axis',(1.22040233680755E-31,1.20629111639801E-46,
-1.));
#116996=DIRECTION('ref_axis',(-9.88437239110458E-16,1.,-1.75022304689845E-61));
#116997=DIRECTION('center_axis',(3.41589266556873E-31,-9.45049376705E-46,
1.));
#116998=DIRECTION('ref_axis',(-2.766624918373E-15,-1.,6.22301527786114E-61));
#116999=DIRECTION('center_axis',(0.,-1.23467863058847E-16,1.));
#117000=DIRECTION('ref_axis',(0.,-1.,0.));
#117001=DIRECTION('center_axis',(0.77428749071043,-0.632834008037926,-3.58179916610815E-15));
#117002=DIRECTION('ref_axis',(0.632834008037926,0.77428749071043,7.75406439997931E-31));
#117003=DIRECTION('center_axis',(-1.09661491495359E-30,9.73989702183063E-45,
-1.));
#117004=DIRECTION('ref_axis',(8.88178419700125E-15,1.,-2.48920611114446E-60));
#117005=DIRECTION('center_axis',(-3.28984474486076E-31,-8.76590731964757E-46,
1.));
#117006=DIRECTION('ref_axis',(2.66453525910038E-15,-1.,4.66726145839586E-61));
#117007=DIRECTION('center_axis',(0.,-1.23467863058847E-16,1.));
#117008=DIRECTION('ref_axis',(0.,-1.,0.));
#117009=DIRECTION('center_axis',(0.999225121087074,-0.0393593367388569,
7.28294031357568E-16));
#117010=DIRECTION('ref_axis',(0.0393593367388569,0.999225121087074,-1.34329260515414E-32));
#117011=DIRECTION('center_axis',(-2.4408046736151E-31,4.82516446559199E-46,
-1.));
#117012=DIRECTION('ref_axis',(1.97687447822091E-15,1.,-3.11150763893057E-61));
#117013=DIRECTION('center_axis',(6.83178533113742E-31,-3.78019750681997E-45,
1.));
#117014=DIRECTION('ref_axis',(-5.53324983674598E-15,-1.,5.60071375007503E-60));
#117015=DIRECTION('center_axis',(-1.,0.,0.));
#117016=DIRECTION('ref_axis',(0.,-7.86407975776152E-14,-1.));
#117017=DIRECTION('center_axis',(-0.994526788819783,0.10448189469861,1.81517644375859E-14));
#117018=DIRECTION('ref_axis',(-0.10448189469861,-0.994526788819783,-2.86631910367634E-30));
#117019=DIRECTION('center_axis',(-0.993679318607912,-0.112256009954549,
-1.48651952901285E-13));
#117020=DIRECTION('ref_axis',(0.112256009954549,-0.993679318607912,-2.2981091857326E-29));
#117021=DIRECTION('center_axis',(-0.991556456479175,-0.129675724846491,
3.15431192506052E-12));
#117022=DIRECTION('ref_axis',(0.129675724846491,-0.991556456479175,7.41046500628616E-29));
#117023=DIRECTION('center_axis',(0.000137331807541708,-0.00219823298717573,
-0.999997574452913));
#117024=DIRECTION('ref_axis',(-0.11217860466933,0.993685625182725,-0.00219976354633589));
#117025=DIRECTION('center_axis',(-2.53853736684102E-13,2.16212897560678E-12,
1.));
#117026=DIRECTION('ref_axis',(-0.129669785749043,0.991557233176077,-2.17675059075509E-12));
#117027=DIRECTION('center_axis',(-0.858927270467749,-0.512097592307192,
1.49780811271862E-14));
#117028=DIRECTION('ref_axis',(0.512097592307192,-0.858927270467749,-6.01293732495529E-30));
#117029=DIRECTION('center_axis',(-0.536899969302814,-0.843645910890723,
-1.46316605705353E-12));
#117030=DIRECTION('ref_axis',(0.843645910890723,-0.536899969302814,1.20303121328766E-28));
#117031=DIRECTION('center_axis',(-0.040766102180794,-0.99916871694073,-1.55671748522919E-15));
#117032=DIRECTION('ref_axis',(0.99916871694073,-0.040766102180794,-1.4838474346331E-32));
#117033=DIRECTION('center_axis',(-0.0297586090124609,-0.999557114521048,
7.26582357398889E-15));
#117034=DIRECTION('ref_axis',(0.999557114521048,-0.0297586090124609,1.68195404251657E-31));
#117035=DIRECTION('center_axis',(-0.0210932860527463,5.46714727619952E-5,
-0.999777510396452));
#117036=DIRECTION('ref_axis',(-0.998923256585619,0.0413287487753403,0.0210775230292068));
#117037=DIRECTION('center_axis',(0.,0.,1.));
#117038=DIRECTION('ref_axis',(-0.999557147327683,0.0297575070552604,0.));
#117039=DIRECTION('center_axis',(0.233238585379144,-0.972419540265587,4.54398481782876E-15));
#117040=DIRECTION('ref_axis',(0.972419540265587,0.233238585379145,-6.30780798053809E-30));
#117041=DIRECTION('center_axis',(-0.229570335512527,-0.973292073867175,
-1.03212124729447E-14));
#117042=DIRECTION('ref_axis',(0.973292073867175,-0.229570335512527,2.98849951310675E-30));
#117043=DIRECTION('center_axis',(0.0298379862379757,-0.999554748164033,
-8.0054834066732E-15));
#117044=DIRECTION('ref_axis',(0.999554748164032,0.0298379862379757,9.39450193490723E-31));
#117045=DIRECTION('center_axis',(0.0407665603815583,-0.999168698246025,
-4.49007546874249E-14));
#117046=DIRECTION('ref_axis',(0.999168698246025,0.0407665603815583,1.08335075317432E-30));
#117047=DIRECTION('center_axis',(-0.0206791468565618,0.000130026885512925,
-0.999786155124332));
#117048=DIRECTION('ref_axis',(-0.9993253707471,-0.0303600651974135,0.0206656677215903));
#117049=DIRECTION('center_axis',(-5.11490712329098E-12,-1.76010917473445E-13,
1.));
#117050=DIRECTION('ref_axis',(-0.999168739570265,-0.040765547531809,-5.11784665730284E-12));
#117051=DIRECTION('center_axis',(0.536601093577061,-0.843836042351772,2.84249428416013E-15));
#117052=DIRECTION('ref_axis',(0.843836042351772,0.536601093577061,2.98189956073675E-31));
#117053=DIRECTION('center_axis',(0.882960425292266,-0.469447427693135,5.17032777304292E-14));
#117054=DIRECTION('ref_axis',(0.469447427693135,0.882960425292266,-2.22396706740103E-29));
#117055=DIRECTION('center_axis',(0.999360062311266,-0.0357696219888033,
-1.64961351615811E-15));
#117056=DIRECTION('ref_axis',(0.0357696219888033,0.999360062311266,4.316049615934E-32));
#117057=DIRECTION('center_axis',(0.999556853338411,-0.0297673805400138,
-1.82491045181999E-14));
#117058=DIRECTION('ref_axis',(0.0297673805400138,0.999556853338411,-8.47827291376735E-32));
#117059=DIRECTION('center_axis',(1.57626159414375E-5,-0.0233282309877023,
-0.999727859665081));
#117060=DIRECTION('ref_axis',(-0.0363487305279994,-0.999067219538478,0.023312242119934));
#117061=DIRECTION('center_axis',(-3.70157306512969E-13,-1.12910217712061E-11,
1.));
#117062=DIRECTION('ref_axis',(-0.0297644531368429,-0.999556940513878,-1.12970184589887E-11));
#117063=DIRECTION('center_axis',(0.972436723729276,0.233166932352493,0.));
#117064=DIRECTION('ref_axis',(-0.233166932352493,0.972436723729276,0.));
#117065=DIRECTION('center_axis',(-0.635093426738814,0.772416788158568,0.00535207286497078));
#117066=DIRECTION('ref_axis',(-0.77242785121363,-0.635102522959478,9.38368926324323E-20));
#117067=DIRECTION('center_axis',(0.00691691416309599,0.00571143710532978,
0.999959767082982));
#117068=DIRECTION('ref_axis',(-0.755062687525124,-0.655591277438894,0.0089674329312478));
#117069=DIRECTION('center_axis',(-0.563237659270021,0.823253026831934,-0.0708363818393295));
#117070=DIRECTION('ref_axis',(-0.825326289137892,-0.564656104596307,-9.62895252096333E-18));
#117071=DIRECTION('center_axis',(0.507471952069715,0.412437854735,0.756549558088658));
#117072=DIRECTION('ref_axis',(-0.587169164883915,-0.477074009384416,0.653936358814375));
#117073=DIRECTION('center_axis',(-0.341333328819756,-0.277129686002563,
-0.898159615977553));
#117074=DIRECTION('ref_axis',(-0.751460582051474,-0.493539243236486,0.437865286370611));
#117075=DIRECTION('center_axis',(-0.0353652067153621,0.980391286708013,
-0.193861360515669));
#117076=DIRECTION('ref_axis',(3.63487303375728E-18,-0.193982705344839,-0.981004949032928));
#117077=DIRECTION('center_axis',(-0.0385934612262193,0.999254003953662,
-0.00140724310442582));
#117078=DIRECTION('ref_axis',(-0.999254993383049,-0.0385934994402315,-2.19294060248386E-20));
#117079=DIRECTION('center_axis',(0.0149227809046296,-0.000160750066432761,
0.999888636183795));
#117080=DIRECTION('ref_axis',(-0.999085030892015,-0.0400869256955743,0.0149043428496258));
#117081=DIRECTION('center_axis',(0.0362455094603874,-7.24243967428071E-6,
-0.999342915615808));
#117082=DIRECTION('ref_axis',(-0.99884239871172,-0.0316458184758586,-0.036227126698248));
#117083=DIRECTION('center_axis',(-0.460561989867266,-0.543327519921019,
0.701910150650338));
#117084=DIRECTION('ref_axis',(1.68332661555862E-16,0.790771035553874,0.612112056186654));
#117085=DIRECTION('center_axis',(-0.469907551033905,-0.216399115636686,
0.855779361887735));
#117086=DIRECTION('ref_axis',(-0.876549208984677,-2.3138118535155E-14,-0.481312252314792));
#117087=DIRECTION('center_axis',(0.488505761670049,-0.207277391256933,-0.847583744469469));
#117088=DIRECTION('ref_axis',(-0.866400038259138,1.13916389737517E-16,-0.499350551921758));
#117089=DIRECTION('center_axis',(-0.485723325571869,0.464849177451359,0.740262178703059));
#117090=DIRECTION('ref_axis',(0.836086106459356,-1.21161241824207E-16,0.548598234216658));
#117091=DIRECTION('center_axis',(0.0366457249192154,-0.000264295716704561,
-0.999328284895869));
#117092=DIRECTION('ref_axis',(-0.998575905634023,0.0387881617069405,-0.0366283933388643));
#117093=DIRECTION('center_axis',(0.0387718059368437,0.999247421633299,0.00115647031964687));
#117094=DIRECTION('ref_axis',(-0.999248089842511,0.0387718318640339,-1.43119761272989E-20));
#117095=DIRECTION('center_axis',(0.015774878482318,-2.06992946781092E-6,
0.999875568860738));
#117096=DIRECTION('ref_axis',(-0.99934939359657,0.0324376701882913,0.0157666442505599));
#117097=DIRECTION('center_axis',(0.0362051861961663,0.986513040328005,0.159628336316885));
#117098=DIRECTION('ref_axis',(-3.13261606677306E-17,0.159733060933468,-0.987160244967769));
#117099=DIRECTION('center_axis',(0.586558422242651,0.80833932738343,0.0503661503543409));
#117100=DIRECTION('ref_axis',(-0.809366559200372,0.587303816476745,6.0201141129801E-17));
#117101=DIRECTION('center_axis',(0.635108704314869,0.772391525947514,-0.00694725470670599));
#117102=DIRECTION('ref_axis',(-0.772410166108943,0.635124031423434,-3.90764897276796E-18));
#117103=DIRECTION('center_axis',(0.533623207912185,-0.432878874101261,0.726541225488501));
#117104=DIRECTION('ref_axis',(-0.613440310270918,0.393261638349251,0.684862226683281));
#117105=DIRECTION('center_axis',(-0.367164830643458,0.297433524522046,-0.88131906006222));
#117106=DIRECTION('ref_axis',(-0.67960514144709,0.561137496245174,0.472505621158498));
#117107=DIRECTION('center_axis',(0.00311221115432024,-0.00394761201357374,
0.999987365170741));
#117108=DIRECTION('ref_axis',(-0.641176102355285,-0.767393078417564,-0.0010339077811091));
#117109=DIRECTION('center_axis',(0.119709524432718,0.500158371272784,-0.857619515522967));
#117110=DIRECTION('ref_axis',(-5.19703601812987E-17,-0.863831361964004,
-0.503781081510029));
#117111=DIRECTION('center_axis',(-0.501099625553759,-0.466384922602348,
0.728961088974634));
#117112=DIRECTION('ref_axis',(0.824074180962238,-2.20209609654532E-16,0.566481901097834));
#117113=DIRECTION('center_axis',(-0.089444411535165,0.865796085392892,0.492338131535099));
#117114=DIRECTION('ref_axis',(0.983291169652569,0.155450651542661,-0.0947289323187182));
#117115=DIRECTION('center_axis',(-0.254850131470821,0.841789549783716,0.475858975290195));
#117116=DIRECTION('ref_axis',(-0.487493726574647,-0.536841697226028,0.688586130175333));
#117117=DIRECTION('center_axis',(-2.30425867295841E-5,0.030784145628616,
-0.999526055611836));
#117118=DIRECTION('ref_axis',(-0.0383802756263916,-0.99878963808956,-0.0307605800947844));
#117119=DIRECTION('center_axis',(-0.999263201609641,0.0383614667420372,
0.00120489761000603));
#117120=DIRECTION('ref_axis',(-0.0383614945882391,-0.999263926964722,2.87536200646804E-20));
#117121=DIRECTION('center_axis',(-4.00197585461019E-5,0.0159615005705134,
0.999872606334405));
#117122=DIRECTION('ref_axis',(-0.0321201706221352,-0.999356707583681,0.0159519793978996));
#117123=DIRECTION('center_axis',(-0.974363720155827,0.0344964635874725,
0.222318093829667));
#117124=DIRECTION('ref_axis',(0.222450491940089,1.26241972147447E-18,0.974943987434977));
#117125=DIRECTION('center_axis',(-0.836810598831192,0.541308500745221,0.0820556439542334));
#117126=DIRECTION('ref_axis',(-0.543140105176027,-0.839642082169167,1.69471490770742E-17));
#117127=DIRECTION('center_axis',(-0.774120577489127,0.632943886852024,-0.0109255482495788));
#117128=DIRECTION('ref_axis',(-0.632981666732123,-0.774166784085331,5.39501067277511E-19));
#117129=DIRECTION('center_axis',(-0.266671211339203,-0.334921826443821,
-0.903722211309657));
#117130=DIRECTION('ref_axis',(-0.574038792157477,-0.698019134436299,0.428075639413392));
#117131=DIRECTION('center_axis',(0.0102380851882465,0.0116065194865278,
0.999880227985876));
#117132=DIRECTION('ref_axis',(0.775942434655157,-0.630803416456049,-0.000622807196781762));
#117133=DIRECTION('center_axis',(-1.07824096236302E-8,-0.998305357148899,
-0.0581929023834511));
#117134=DIRECTION('ref_axis',(0.,0.058192902383451,-0.998305357148899));
#117135=DIRECTION('center_axis',(-1.,0.,0.));
#117136=DIRECTION('ref_axis',(0.,-6.93889390390722E-15,-1.));
#117137=DIRECTION('center_axis',(-2.31017521133305E-9,0.986382705137784,
0.164466285314247));
#117138=DIRECTION('ref_axis',(0.99999903088274,0.000228972993696964,-0.00137324613565508));
#117139=DIRECTION('center_axis',(-0.99999635393917,-0.000157155077313813,
0.00269581354111146));
#117140=DIRECTION('ref_axis',(0.00269581357440168,1.24619272072387E-21,
0.999996366287984));
#117141=DIRECTION('center_axis',(-8.12532577157186E-9,-0.998207006171548,
-0.0598562680931181));
#117142=DIRECTION('ref_axis',(0.999311726713681,0.00222038745151431,-0.0370289445175939));
#117143=DIRECTION('center_axis',(0.244344449131117,-0.492606745559265,-0.835245104390514));
#117144=DIRECTION('ref_axis',(-4.32889927015855E-17,-0.86135403585069,0.508005142615435));
#117145=DIRECTION('center_axis',(-0.982994797178248,-0.183632204703407,
0.000664918236953841));
#117146=DIRECTION('ref_axis',(0.183632245296812,-0.982995014477312,5.7655403569157E-20));
#117147=DIRECTION('center_axis',(0.000179526560883581,-0.00456486630691949,
-0.999989564828461));
#117148=DIRECTION('ref_axis',(0.986444685005576,0.164093132907876,-0.000571976160476437));
#117149=DIRECTION('center_axis',(0.330813257101916,0.830741130674896,-0.447696060660149));
#117150=DIRECTION('ref_axis',(-0.932375699002072,0.214461635172499,-0.291001310906903));
#117151=DIRECTION('center_axis',(-0.433391148275503,0.470797811534069,0.768453989026781));
#117152=DIRECTION('ref_axis',(8.06979081629128E-16,0.852695228537141,-0.522408697506075));
#117153=DIRECTION('center_axis',(-0.96720597488598,-0.18129103740974,0.177893681449798));
#117154=DIRECTION('ref_axis',(0.184229551589837,-0.982883244501099,1.61805378326746E-17));
#117155=DIRECTION('center_axis',(-0.831503844166329,-0.548952032819844,
0.0851646804701234));
#117156=DIRECTION('ref_axis',(0.550953708881667,-0.834535805504794,3.15287181374443E-17));
#117157=DIRECTION('center_axis',(-0.777065025633406,-0.629380269512156,
-0.00710086516978589));
#117158=DIRECTION('ref_axis',(0.62939613750826,-0.777084617071837,1.0927692862107E-18));
#117159=DIRECTION('center_axis',(-0.295452400444952,0.370381022938362,-0.880639413675341));
#117160=DIRECTION('ref_axis',(-0.467331061476171,0.747944548358106,0.471360405168853));
#117161=DIRECTION('center_axis',(0.429530667833731,-0.537702321291583,0.725520240288272));
#117162=DIRECTION('ref_axis',(-0.451971122885174,0.567540558793691,0.68820042008274));
#117163=DIRECTION('center_axis',(0.,0.,-1.));
#117164=DIRECTION('ref_axis',(0.,1.,0.));
#117165=DIRECTION('center_axis',(0.,0.,1.));
#117166=DIRECTION('ref_axis',(0.,1.,0.));
#117167=DIRECTION('',(0.,1.23467863058847E-16,-1.));
#117168=DIRECTION('',(3.82498197630791E-33,-1.23467863058847E-16,1.));
#117169=DIRECTION('center_axis',(0.,0.,-1.));
#117170=DIRECTION('ref_axis',(0.,1.,0.));
#117171=DIRECTION('',(0.,-1.23467863058847E-16,1.));
#117172=DIRECTION('center_axis',(0.,0.,1.));
#117173=DIRECTION('ref_axis',(0.,1.,0.));
#117174=DIRECTION('',(0.,1.23467863058847E-16,-1.));
#117175=DIRECTION('center_axis',(0.,0.,-1.));
#117176=DIRECTION('ref_axis',(0.,1.,0.));
#117177=DIRECTION('',(0.,-1.23467863058847E-16,1.));
#117178=DIRECTION('center_axis',(0.,0.,1.));
#117179=DIRECTION('ref_axis',(0.,1.,0.));
#117180=DIRECTION('',(0.,1.23467863058847E-16,-1.));
#117181=DIRECTION('center_axis',(0.,0.,-1.));
#117182=DIRECTION('ref_axis',(0.,1.,0.));
#117183=DIRECTION('',(0.,-1.23467863058847E-16,1.));
#117184=DIRECTION('center_axis',(0.,0.,1.));
#117185=DIRECTION('ref_axis',(0.,1.,0.));
#117186=DIRECTION('',(0.,1.23467863058847E-16,-1.));
#117187=DIRECTION('center_axis',(0.,0.,-1.));
#117188=DIRECTION('ref_axis',(0.,1.,0.));
#117189=DIRECTION('',(0.,-1.23467863058847E-16,1.));
#117190=DIRECTION('center_axis',(0.,0.,1.));
#117191=DIRECTION('ref_axis',(0.,1.,0.));
#117192=DIRECTION('',(0.,1.23467863058847E-16,-1.));
#117193=DIRECTION('center_axis',(0.,0.,-1.));
#117194=DIRECTION('ref_axis',(0.,1.,0.));
#117195=DIRECTION('',(0.,-1.23467863058847E-16,1.));
#117196=DIRECTION('center_axis',(0.,0.,1.));
#117197=DIRECTION('ref_axis',(0.,1.,0.));
#117198=DIRECTION('',(0.,1.23467863058847E-16,-1.));
#117199=DIRECTION('center_axis',(0.,0.,-1.));
#117200=DIRECTION('ref_axis',(0.,1.,0.));
#117201=DIRECTION('',(0.,-1.23467863058847E-16,1.));
#117202=DIRECTION('center_axis',(0.,0.,1.));
#117203=DIRECTION('ref_axis',(0.,1.,0.));
#117204=DIRECTION('',(-1.27503726478586E-32,1.23467863058847E-16,-1.));
#117205=DIRECTION('center_axis',(0.,0.,-1.));
#117206=DIRECTION('ref_axis',(-0.0950205176920726,-0.995475314218053,0.));
#117207=DIRECTION('',(0.,-1.23467863058847E-16,1.));
#117208=DIRECTION('center_axis',(0.,0.,1.));
#117209=DIRECTION('ref_axis',(0.,1.,0.));
#117210=DIRECTION('',(0.,1.23467863058847E-16,-1.));
#117211=DIRECTION('center_axis',(0.,0.,-1.));
#117212=DIRECTION('ref_axis',(0.,1.,0.));
#117213=DIRECTION('',(0.,-1.23467863058847E-16,1.));
#117214=DIRECTION('center_axis',(0.,0.,1.));
#117215=DIRECTION('ref_axis',(0.,1.,0.));
#117216=DIRECTION('',(0.,1.23467863058847E-16,-1.));
#117217=DIRECTION('center_axis',(0.,0.,-1.));
#117218=DIRECTION('ref_axis',(0.,1.,0.));
#117219=DIRECTION('center_axis',(0.,0.,1.));
#117220=DIRECTION('ref_axis',(0.,1.,0.));
#117221=DIRECTION('',(0.,1.23467863058847E-16,-1.));
#117222=DIRECTION('',(0.,-1.23467863058847E-16,1.));
#117223=DIRECTION('center_axis',(0.,0.,-1.));
#117224=DIRECTION('ref_axis',(0.,1.,0.));
#117225=DIRECTION('',(0.,-1.23467863058847E-16,1.));
#117226=DIRECTION('center_axis',(0.,0.,1.));
#117227=DIRECTION('ref_axis',(0.,1.,0.));
#117228=DIRECTION('',(0.,1.23467863058847E-16,-1.));
#117229=DIRECTION('center_axis',(-1.3684555315672E-48,0.,1.));
#117230=DIRECTION('ref_axis',(0.,-1.,0.));
#117231=DIRECTION('',(0.,-1.23467863058847E-16,1.));
#117232=DIRECTION('center_axis',(0.,0.,1.));
#117233=DIRECTION('ref_axis',(0.,1.,0.));
#117234=DIRECTION('',(1.3684555315672E-48,1.23467863058847E-16,-1.));
#117235=DIRECTION('center_axis',(0.,0.,-1.));
#117236=DIRECTION('ref_axis',(0.,1.,0.));
#117237=DIRECTION('',(0.,-1.23467863058847E-16,1.));
#117238=DIRECTION('center_axis',(0.,0.,1.));
#117239=DIRECTION('ref_axis',(0.,1.,0.));
#117240=DIRECTION('',(0.,1.23467863058847E-16,-1.));
#117241=DIRECTION('center_axis',(0.,0.,1.));
#117242=DIRECTION('ref_axis',(0.,-1.,0.));
#117243=DIRECTION('',(0.,-1.23467863058847E-16,1.));
#117244=DIRECTION('center_axis',(0.,0.,1.));
#117245=DIRECTION('ref_axis',(0.,1.,0.));
#117246=DIRECTION('',(0.,1.23467863058847E-16,-1.));
#117247=DIRECTION('center_axis',(0.,0.,-1.));
#117248=DIRECTION('ref_axis',(0.,1.,0.));
#117249=DIRECTION('',(0.,-1.23467863058847E-16,1.));
#117250=DIRECTION('center_axis',(0.,0.,1.));
#117251=DIRECTION('ref_axis',(0.,1.,0.));
#117252=DIRECTION('',(0.,1.23467863058847E-16,-1.));
#117253=DIRECTION('center_axis',(0.,0.,-1.));
#117254=DIRECTION('ref_axis',(0.,1.,0.));
#117255=DIRECTION('',(0.,-1.23467863058847E-16,1.));
#117256=DIRECTION('center_axis',(0.,0.,1.));
#117257=DIRECTION('ref_axis',(0.,1.,0.));
#117258=DIRECTION('',(0.,1.23467863058847E-16,-1.));
#117259=DIRECTION('center_axis',(0.,0.,1.));
#117260=DIRECTION('ref_axis',(0.,-1.,0.));
#117261=DIRECTION('',(0.,-1.23467863058847E-16,1.));
#117262=DIRECTION('center_axis',(0.,0.,1.));
#117263=DIRECTION('ref_axis',(0.,1.,0.));
#117264=DIRECTION('',(0.,1.23467863058847E-16,-1.));
#117265=DIRECTION('center_axis',(1.3684555315672E-48,0.,-1.));
#117266=DIRECTION('ref_axis',(0.,1.,0.));
#117267=DIRECTION('',(-1.3684555315672E-48,-1.23467863058847E-16,1.));
#117268=DIRECTION('center_axis',(0.,0.,1.));
#117269=DIRECTION('ref_axis',(0.,1.,0.));
#117270=DIRECTION('',(0.,1.23467863058847E-16,-1.));
#117271=DIRECTION('center_axis',(0.,0.,-1.));
#117272=DIRECTION('ref_axis',(-0.686617021913642,-0.727019301819726,0.));
#117273=DIRECTION('',(0.,-1.23467863058847E-16,1.));
#117274=DIRECTION('center_axis',(0.,0.,1.));
#117275=DIRECTION('ref_axis',(0.,1.,0.));
#117276=DIRECTION('',(0.,1.23467863058847E-16,-1.));
#117277=DIRECTION('center_axis',(0.,0.,1.));
#117278=DIRECTION('ref_axis',(0.,-1.,0.));
#117279=DIRECTION('',(0.,-1.23467863058847E-16,1.));
#117280=DIRECTION('center_axis',(0.,0.,1.));
#117281=DIRECTION('ref_axis',(0.,1.,0.));
#117282=DIRECTION('',(0.,1.23467863058847E-16,-1.));
#117283=DIRECTION('center_axis',(0.,0.,-1.));
#117284=DIRECTION('ref_axis',(0.,1.,0.));
#117285=DIRECTION('',(0.,-1.23467863058847E-16,1.));
#117286=DIRECTION('center_axis',(0.,0.,1.));
#117287=DIRECTION('ref_axis',(0.,1.,0.));
#117288=DIRECTION('',(0.,1.23467863058847E-16,-1.));
#117289=DIRECTION('center_axis',(0.,0.,-1.));
#117290=DIRECTION('ref_axis',(0.,1.,0.));
#117291=DIRECTION('',(0.,-1.23467863058847E-16,1.));
#117292=DIRECTION('center_axis',(0.,0.,1.));
#117293=DIRECTION('ref_axis',(0.,1.,0.));
#117294=DIRECTION('',(0.,1.23467863058847E-16,-1.));
#117295=DIRECTION('center_axis',(0.,0.,-1.));
#117296=DIRECTION('ref_axis',(0.,1.,0.));
#117297=DIRECTION('',(0.,-1.23467863058847E-16,1.));
#117298=DIRECTION('center_axis',(0.,0.,1.));
#117299=DIRECTION('ref_axis',(0.,1.,0.));
#117300=DIRECTION('',(0.,1.23467863058847E-16,-1.));
#117301=DIRECTION('center_axis',(0.,0.,1.));
#117302=DIRECTION('ref_axis',(0.,-1.,0.));
#117303=DIRECTION('',(0.,-1.23467863058847E-16,1.));
#117304=DIRECTION('center_axis',(0.,0.,1.));
#117305=DIRECTION('ref_axis',(0.,1.,0.));
#117306=DIRECTION('',(0.,1.23467863058847E-16,-1.));
#117307=DIRECTION('center_axis',(0.,0.,-1.));
#117308=DIRECTION('ref_axis',(0.,1.,0.));
#117309=DIRECTION('',(0.,-1.23467863058847E-16,1.));
#117310=DIRECTION('center_axis',(0.,0.,1.));
#117311=DIRECTION('ref_axis',(0.,1.,0.));
#117312=DIRECTION('',(0.,1.23467863058847E-16,-1.));
#117313=DIRECTION('center_axis',(0.,0.,1.));
#117314=DIRECTION('ref_axis',(0.,-1.,0.));
#117315=DIRECTION('',(0.,-1.23467863058847E-16,1.));
#117316=DIRECTION('center_axis',(0.,0.,1.));
#117317=DIRECTION('ref_axis',(0.,1.,0.));
#117318=DIRECTION('',(0.,1.23467863058847E-16,-1.));
#117319=DIRECTION('center_axis',(0.,0.,-1.));
#117320=DIRECTION('ref_axis',(0.,1.,0.));
#117321=DIRECTION('',(0.,-1.23467863058847E-16,1.));
#117322=DIRECTION('center_axis',(0.,0.,1.));
#117323=DIRECTION('ref_axis',(0.,1.,0.));
#117324=DIRECTION('',(0.,1.23467863058847E-16,-1.));
#117325=DIRECTION('center_axis',(0.,0.,-1.));
#117326=DIRECTION('ref_axis',(0.,1.,0.));
#117327=DIRECTION('center_axis',(0.,0.,1.));
#117328=DIRECTION('ref_axis',(0.,1.,0.));
#117329=DIRECTION('',(0.,1.23467863058847E-16,-1.));
#117330=DIRECTION('',(0.,-1.23467863058847E-16,1.));
#117331=DIRECTION('center_axis',(0.,0.,1.));
#117332=DIRECTION('ref_axis',(0.,-1.,0.));
#117333=DIRECTION('',(0.,-1.23467863058847E-16,1.));
#117334=DIRECTION('center_axis',(0.,0.,1.));
#117335=DIRECTION('ref_axis',(0.,1.,0.));
#117336=DIRECTION('',(0.,1.23467863058847E-16,-1.));
#117337=DIRECTION('center_axis',(0.,0.,-1.));
#117338=DIRECTION('ref_axis',(0.,1.,0.));
#117339=DIRECTION('',(0.,-1.23467863058847E-16,1.));
#117340=DIRECTION('center_axis',(0.,0.,1.));
#117341=DIRECTION('ref_axis',(0.,1.,0.));
#117342=DIRECTION('',(0.,1.23467863058847E-16,-1.));
#117343=DIRECTION('center_axis',(0.,0.,1.));
#117344=DIRECTION('ref_axis',(0.,-1.,0.));
#117345=DIRECTION('',(0.,-1.23467863058847E-16,1.));
#117346=DIRECTION('center_axis',(0.,0.,1.));
#117347=DIRECTION('ref_axis',(0.,1.,0.));
#117348=DIRECTION('',(0.,1.23467863058847E-16,-1.));
#117349=DIRECTION('center_axis',(0.,0.,-1.));
#117350=DIRECTION('ref_axis',(0.,1.,0.));
#117351=DIRECTION('',(0.,-1.23467863058847E-16,1.));
#117352=DIRECTION('center_axis',(0.,0.,1.));
#117353=DIRECTION('ref_axis',(0.,1.,0.));
#117354=DIRECTION('',(0.,1.23467863058847E-16,-1.));
#117355=DIRECTION('center_axis',(0.,0.,1.));
#117356=DIRECTION('ref_axis',(0.,-1.,0.));
#117357=DIRECTION('',(0.,-1.23467863058847E-16,1.));
#117358=DIRECTION('center_axis',(0.,0.,1.));
#117359=DIRECTION('ref_axis',(0.,1.,0.));
#117360=DIRECTION('',(0.,1.23467863058847E-16,-1.));
#117361=DIRECTION('center_axis',(0.,0.,-1.));
#117362=DIRECTION('ref_axis',(0.,1.,0.));
#117363=DIRECTION('',(0.,-1.23467863058847E-16,1.));
#117364=DIRECTION('center_axis',(0.,0.,1.));
#117365=DIRECTION('ref_axis',(0.,1.,0.));
#117366=DIRECTION('',(0.,1.23467863058847E-16,-1.));
#117367=DIRECTION('center_axis',(0.,0.,1.));
#117368=DIRECTION('ref_axis',(0.,-1.,0.));
#117369=DIRECTION('',(0.,-1.23467863058847E-16,1.));
#117370=DIRECTION('center_axis',(0.,0.,1.));
#117371=DIRECTION('ref_axis',(0.,1.,0.));
#117372=DIRECTION('',(0.,1.23467863058847E-16,-1.));
#117373=DIRECTION('center_axis',(0.,0.,-1.));
#117374=DIRECTION('ref_axis',(0.,1.,0.));
#117375=DIRECTION('',(0.,-1.23467863058847E-16,1.));
#117376=DIRECTION('center_axis',(0.,0.,1.));
#117377=DIRECTION('ref_axis',(0.,1.,0.));
#117378=DIRECTION('',(0.,1.23467863058847E-16,-1.));
#117379=DIRECTION('center_axis',(0.,0.,1.));
#117380=DIRECTION('ref_axis',(0.,-1.,0.));
#117381=DIRECTION('',(0.,-1.23467863058847E-16,1.));
#117382=DIRECTION('center_axis',(0.,0.,1.));
#117383=DIRECTION('ref_axis',(0.,1.,0.));
#117384=DIRECTION('',(0.,1.23467863058847E-16,-1.));
#117385=DIRECTION('center_axis',(0.,0.,-1.));
#117386=DIRECTION('ref_axis',(0.,1.,0.));
#117387=DIRECTION('',(0.,-1.23467863058847E-16,1.));
#117388=DIRECTION('center_axis',(0.,0.,1.));
#117389=DIRECTION('ref_axis',(0.,1.,0.));
#117390=DIRECTION('',(0.,1.23467863058847E-16,-1.));
#117391=DIRECTION('center_axis',(0.,0.,-1.));
#117392=DIRECTION('ref_axis',(0.695782815675814,-0.718252235228151,0.));
#117393=DIRECTION('',(0.,-1.23467863058847E-16,1.));
#117394=DIRECTION('center_axis',(0.,0.,1.));
#117395=DIRECTION('ref_axis',(0.,1.,0.));
#117396=DIRECTION('',(0.,1.23467863058847E-16,-1.));
#117397=DIRECTION('center_axis',(0.,0.,-1.));
#117398=DIRECTION('ref_axis',(0.,1.,0.));
#117399=DIRECTION('',(0.,-1.23467863058847E-16,1.));
#117400=DIRECTION('center_axis',(0.,0.,1.));
#117401=DIRECTION('ref_axis',(0.,1.,0.));
#117402=DIRECTION('',(0.,1.23467863058847E-16,-1.));
#117403=DIRECTION('center_axis',(0.,0.,1.));
#117404=DIRECTION('ref_axis',(0.,-1.,0.));
#117405=DIRECTION('',(0.,-1.23467863058847E-16,1.));
#117406=DIRECTION('center_axis',(0.,0.,1.));
#117407=DIRECTION('ref_axis',(0.,1.,0.));
#117408=DIRECTION('',(0.,1.23467863058847E-16,-1.));
#117409=DIRECTION('center_axis',(0.,0.,-1.));
#117410=DIRECTION('ref_axis',(0.,1.,0.));
#117411=DIRECTION('',(0.,-1.23467863058847E-16,1.));
#117412=DIRECTION('center_axis',(0.,0.,1.));
#117413=DIRECTION('ref_axis',(0.,1.,0.));
#117414=DIRECTION('',(0.,1.23467863058847E-16,-1.));
#117415=DIRECTION('center_axis',(0.,0.,-1.));
#117416=DIRECTION('ref_axis',(0.,1.,0.));
#117417=DIRECTION('',(0.,-1.23467863058847E-16,1.));
#117418=DIRECTION('center_axis',(0.,0.,1.));
#117419=DIRECTION('ref_axis',(0.,1.,0.));
#117420=DIRECTION('',(0.,1.23467863058847E-16,-1.));
#117421=DIRECTION('center_axis',(0.,0.,-1.));
#117422=DIRECTION('ref_axis',(0.,1.,0.));
#117423=DIRECTION('',(0.,-1.23467863058847E-16,1.));
#117424=DIRECTION('center_axis',(0.,0.,1.));
#117425=DIRECTION('ref_axis',(0.,1.,0.));
#117426=DIRECTION('',(0.,1.23467863058847E-16,-1.));
#117427=DIRECTION('center_axis',(0.,0.,1.));
#117428=DIRECTION('ref_axis',(0.,-1.,0.));
#117429=DIRECTION('',(0.,-1.23467863058847E-16,1.));
#117430=DIRECTION('center_axis',(0.,0.,1.));
#117431=DIRECTION('ref_axis',(0.,1.,0.));
#117432=DIRECTION('',(0.,1.23467863058847E-16,-1.));
#117433=DIRECTION('center_axis',(0.,0.,-1.));
#117434=DIRECTION('ref_axis',(0.,1.,0.));
#117435=DIRECTION('',(0.,-1.23467863058847E-16,1.));
#117436=DIRECTION('center_axis',(0.,0.,1.));
#117437=DIRECTION('ref_axis',(0.,1.,0.));
#117438=DIRECTION('',(0.,1.23467863058847E-16,-1.));
#117439=DIRECTION('center_axis',(0.,0.,1.));
#117440=DIRECTION('ref_axis',(0.,-1.,0.));
#117441=DIRECTION('',(0.,-1.23467863058847E-16,1.));
#117442=DIRECTION('center_axis',(0.,0.,1.));
#117443=DIRECTION('ref_axis',(0.,1.,0.));
#117444=DIRECTION('',(0.,1.23467863058847E-16,-1.));
#117445=DIRECTION('center_axis',(0.,0.,-1.));
#117446=DIRECTION('ref_axis',(0.,1.,0.));
#117447=DIRECTION('',(0.,-1.23467863058847E-16,1.));
#117448=DIRECTION('center_axis',(0.,0.,1.));
#117449=DIRECTION('ref_axis',(0.,1.,0.));
#117450=DIRECTION('',(0.,1.23467863058847E-16,-1.));
#117451=DIRECTION('center_axis',(0.,0.,1.));
#117452=DIRECTION('ref_axis',(0.,-1.,0.));
#117453=DIRECTION('',(0.,-1.23467863058847E-16,1.));
#117454=DIRECTION('center_axis',(0.,0.,1.));
#117455=DIRECTION('ref_axis',(0.,1.,0.));
#117456=DIRECTION('',(0.,1.23467863058847E-16,-1.));
#117457=DIRECTION('center_axis',(0.,0.,-1.));
#117458=DIRECTION('ref_axis',(0.,1.,0.));
#117459=DIRECTION('',(0.,-1.23467863058847E-16,1.));
#117460=DIRECTION('center_axis',(0.,0.,1.));
#117461=DIRECTION('ref_axis',(0.,1.,0.));
#117462=DIRECTION('',(0.,1.23467863058847E-16,-1.));
#117463=DIRECTION('center_axis',(0.,0.,1.));
#117464=DIRECTION('ref_axis',(0.,-1.,0.));
#117465=DIRECTION('',(0.,-1.23467863058847E-16,1.));
#117466=DIRECTION('center_axis',(0.,0.,1.));
#117467=DIRECTION('ref_axis',(0.,1.,0.));
#117468=DIRECTION('',(0.,1.23467863058847E-16,-1.));
#117469=DIRECTION('center_axis',(0.,0.,-1.));
#117470=DIRECTION('ref_axis',(0.,1.,0.));
#117471=DIRECTION('',(0.,-1.23467863058847E-16,1.));
#117472=DIRECTION('center_axis',(0.,0.,1.));
#117473=DIRECTION('ref_axis',(0.,1.,0.));
#117474=DIRECTION('',(0.,1.23467863058847E-16,-1.));
#117475=DIRECTION('center_axis',(0.,0.,1.));
#117476=DIRECTION('ref_axis',(0.,-1.,0.));
#117477=DIRECTION('',(0.,-1.23467863058847E-16,1.));
#117478=DIRECTION('center_axis',(0.,0.,1.));
#117479=DIRECTION('ref_axis',(0.,1.,0.));
#117480=DIRECTION('',(0.,1.23467863058847E-16,-1.));
#117481=DIRECTION('center_axis',(0.,0.,-1.));
#117482=DIRECTION('ref_axis',(0.,1.,0.));
#117483=DIRECTION('',(0.,-1.23467863058847E-16,1.));
#117484=DIRECTION('center_axis',(0.,0.,1.));
#117485=DIRECTION('ref_axis',(0.,1.,0.));
#117486=DIRECTION('',(0.,1.23467863058847E-16,-1.));
#117487=DIRECTION('center_axis',(0.,0.,1.));
#117488=DIRECTION('ref_axis',(0.,-1.,0.));
#117489=DIRECTION('',(0.,-1.23467863058847E-16,1.));
#117490=DIRECTION('center_axis',(0.,0.,1.));
#117491=DIRECTION('ref_axis',(0.,1.,0.));
#117492=DIRECTION('',(0.,1.23467863058847E-16,-1.));
#117493=DIRECTION('center_axis',(0.,0.,-1.));
#117494=DIRECTION('ref_axis',(0.,1.,0.));
#117495=DIRECTION('',(0.,-1.23467863058847E-16,1.));
#117496=DIRECTION('center_axis',(0.,0.,1.));
#117497=DIRECTION('ref_axis',(0.,1.,0.));
#117498=DIRECTION('',(0.,1.23467863058847E-16,-1.));
#117499=DIRECTION('center_axis',(0.,0.,-1.));
#117500=DIRECTION('ref_axis',(0.,1.,0.));
#117501=DIRECTION('',(0.,-1.23467863058847E-16,1.));
#117502=DIRECTION('center_axis',(0.,0.,1.));
#117503=DIRECTION('ref_axis',(0.,1.,0.));
#117504=DIRECTION('',(0.,1.23467863058847E-16,-1.));
#117505=DIRECTION('center_axis',(0.,0.,-1.));
#117506=DIRECTION('ref_axis',(0.406625030395207,-0.91359514264038,0.));
#117507=DIRECTION('',(0.,-1.23467863058847E-16,1.));
#117508=DIRECTION('center_axis',(0.,0.,1.));
#117509=DIRECTION('ref_axis',(0.,1.,0.));
#117510=DIRECTION('',(0.,1.23467863058847E-16,-1.));
#117511=DIRECTION('center_axis',(0.,0.,-1.));
#117512=DIRECTION('ref_axis',(0.,1.,0.));
#117513=DIRECTION('',(0.,-1.23467863058847E-16,1.));
#117514=DIRECTION('center_axis',(0.,0.,1.));
#117515=DIRECTION('ref_axis',(0.,1.,0.));
#117516=DIRECTION('',(0.,1.23467863058847E-16,-1.));
#117517=DIRECTION('center_axis',(0.,0.,-1.));
#117518=DIRECTION('ref_axis',(0.,1.,0.));
#117519=DIRECTION('',(0.,-1.23467863058847E-16,1.));
#117520=DIRECTION('center_axis',(0.,0.,1.));
#117521=DIRECTION('ref_axis',(0.,1.,0.));
#117522=DIRECTION('',(0.,1.23467863058847E-16,-1.));
#117523=DIRECTION('center_axis',(0.,0.,1.));
#117524=DIRECTION('ref_axis',(0.,-1.,0.));
#117525=DIRECTION('',(0.,-1.23467863058847E-16,1.));
#117526=DIRECTION('center_axis',(0.,0.,1.));
#117527=DIRECTION('ref_axis',(0.,1.,0.));
#117528=DIRECTION('',(0.,1.23467863058847E-16,-1.));
#117529=DIRECTION('center_axis',(0.,0.,-1.));
#117530=DIRECTION('ref_axis',(0.,1.,0.));
#117531=DIRECTION('',(0.,-1.23467863058847E-16,1.));
#117532=DIRECTION('center_axis',(0.,0.,1.));
#117533=DIRECTION('ref_axis',(0.,1.,0.));
#117534=DIRECTION('',(0.,1.23467863058847E-16,-1.));
#117535=DIRECTION('center_axis',(0.,0.,1.));
#117536=DIRECTION('ref_axis',(0.,-1.,0.));
#117537=DIRECTION('',(0.,-1.23467863058847E-16,1.));
#117538=DIRECTION('center_axis',(0.,0.,1.));
#117539=DIRECTION('ref_axis',(0.,1.,0.));
#117540=DIRECTION('',(0.,1.23467863058847E-16,-1.));
#117541=DIRECTION('center_axis',(0.,0.,-1.));
#117542=DIRECTION('ref_axis',(0.,1.,0.));
#117543=DIRECTION('',(0.,-1.23467863058847E-16,1.));
#117544=DIRECTION('center_axis',(0.,0.,1.));
#117545=DIRECTION('ref_axis',(0.,1.,0.));
#117546=DIRECTION('',(0.,1.23467863058847E-16,-1.));
#117547=DIRECTION('center_axis',(0.,0.,1.));
#117548=DIRECTION('ref_axis',(0.,-1.,0.));
#117549=DIRECTION('',(0.,-1.23467863058847E-16,1.));
#117550=DIRECTION('center_axis',(0.,0.,1.));
#117551=DIRECTION('ref_axis',(0.,1.,0.));
#117552=DIRECTION('',(0.,1.23467863058847E-16,-1.));
#117553=DIRECTION('center_axis',(0.,0.,-1.));
#117554=DIRECTION('ref_axis',(0.,1.,0.));
#117555=DIRECTION('',(0.,-1.23467863058847E-16,1.));
#117556=DIRECTION('center_axis',(0.,0.,1.));
#117557=DIRECTION('ref_axis',(0.,1.,0.));
#117558=DIRECTION('',(0.,1.23467863058847E-16,-1.));
#117559=DIRECTION('center_axis',(0.,0.,-1.));
#117560=DIRECTION('ref_axis',(0.,1.,0.));
#117561=DIRECTION('',(0.,-1.23467863058847E-16,1.));
#117562=DIRECTION('center_axis',(0.,0.,1.));
#117563=DIRECTION('ref_axis',(0.,1.,0.));
#117564=DIRECTION('',(0.,1.23467863058847E-16,-1.));
#117565=DIRECTION('center_axis',(0.,0.,-1.));
#117566=DIRECTION('ref_axis',(0.,1.,0.));
#117567=DIRECTION('',(0.,-1.23467863058847E-16,1.));
#117568=DIRECTION('center_axis',(0.,0.,1.));
#117569=DIRECTION('ref_axis',(0.,1.,0.));
#117570=DIRECTION('',(0.,1.23467863058847E-16,-1.));
#117571=DIRECTION('center_axis',(0.,0.,1.));
#117572=DIRECTION('ref_axis',(0.,-1.,0.));
#117573=DIRECTION('',(0.,-1.23467863058847E-16,1.));
#117574=DIRECTION('center_axis',(0.,0.,1.));
#117575=DIRECTION('ref_axis',(0.,1.,0.));
#117576=DIRECTION('',(0.,1.23467863058847E-16,-1.));
#117577=DIRECTION('center_axis',(0.,0.,-1.));
#117578=DIRECTION('ref_axis',(0.,1.,0.));
#117579=DIRECTION('',(0.,-1.23467863058847E-16,1.));
#117580=DIRECTION('center_axis',(0.,0.,1.));
#117581=DIRECTION('ref_axis',(0.,1.,0.));
#117582=DIRECTION('',(0.,1.23467863058847E-16,-1.));
#117583=DIRECTION('center_axis',(0.,0.,-1.));
#117584=DIRECTION('ref_axis',(0.,1.,0.));
#117585=DIRECTION('',(0.,-1.23467863058847E-16,1.));
#117586=DIRECTION('center_axis',(0.,0.,1.));
#117587=DIRECTION('ref_axis',(0.,1.,0.));
#117588=DIRECTION('',(0.,1.23467863058847E-16,-1.));
#117589=DIRECTION('center_axis',(0.,0.,-1.));
#117590=DIRECTION('ref_axis',(0.,1.,0.));
#117591=DIRECTION('',(0.,-1.23467863058847E-16,1.));
#117592=DIRECTION('center_axis',(0.,0.,1.));
#117593=DIRECTION('ref_axis',(0.,1.,0.));
#117594=DIRECTION('',(0.,1.23467863058847E-16,-1.));
#117595=DIRECTION('center_axis',(0.,0.,1.));
#117596=DIRECTION('ref_axis',(0.,-1.,0.));
#117597=DIRECTION('',(0.,-1.23467863058847E-16,1.));
#117598=DIRECTION('center_axis',(0.,0.,1.));
#117599=DIRECTION('ref_axis',(0.,1.,0.));
#117600=DIRECTION('',(0.,1.23467863058847E-16,-1.));
#117601=DIRECTION('center_axis',(0.,0.,-1.));
#117602=DIRECTION('ref_axis',(0.,1.,0.));
#117603=DIRECTION('',(0.,-1.23467863058847E-16,1.));
#117604=DIRECTION('center_axis',(0.,0.,1.));
#117605=DIRECTION('ref_axis',(0.,1.,0.));
#117606=DIRECTION('',(0.,1.23467863058847E-16,-1.));
#117607=DIRECTION('center_axis',(0.,0.,-1.));
#117608=DIRECTION('ref_axis',(0.,1.,0.));
#117609=DIRECTION('',(0.,-1.23467863058847E-16,1.));
#117610=DIRECTION('center_axis',(0.,0.,1.));
#117611=DIRECTION('ref_axis',(0.,1.,0.));
#117612=DIRECTION('',(0.,1.23467863058847E-16,-1.));
#117613=DIRECTION('center_axis',(0.,0.,-1.));
#117614=DIRECTION('ref_axis',(0.,1.,0.));
#117615=DIRECTION('',(0.,-1.23467863058847E-16,1.));
#117616=DIRECTION('center_axis',(0.,0.,1.));
#117617=DIRECTION('ref_axis',(0.,1.,0.));
#117618=DIRECTION('',(0.,1.23467863058847E-16,-1.));
#117619=DIRECTION('center_axis',(0.,0.,1.));
#117620=DIRECTION('ref_axis',(0.,-1.,0.));
#117621=DIRECTION('',(0.,-1.23467863058847E-16,1.));
#117622=DIRECTION('center_axis',(0.,0.,1.));
#117623=DIRECTION('ref_axis',(0.,1.,0.));
#117624=DIRECTION('',(0.,1.23467863058847E-16,-1.));
#117625=DIRECTION('center_axis',(0.,0.,-1.));
#117626=DIRECTION('ref_axis',(0.,1.,0.));
#117627=DIRECTION('',(0.,-1.23467863058847E-16,1.));
#117628=DIRECTION('center_axis',(0.,0.,1.));
#117629=DIRECTION('ref_axis',(0.,1.,0.));
#117630=DIRECTION('',(0.,1.23467863058847E-16,-1.));
#117631=DIRECTION('center_axis',(0.,0.,-1.));
#117632=DIRECTION('ref_axis',(0.,1.,0.));
#117633=DIRECTION('',(0.,-1.23467863058847E-16,1.));
#117634=DIRECTION('center_axis',(0.,0.,1.));
#117635=DIRECTION('ref_axis',(0.,1.,0.));
#117636=DIRECTION('',(0.,1.23467863058847E-16,-1.));
#117637=DIRECTION('center_axis',(0.,0.,-1.));
#117638=DIRECTION('ref_axis',(0.,1.,0.));
#117639=DIRECTION('',(0.,-1.23467863058847E-16,1.));
#117640=DIRECTION('center_axis',(0.,0.,1.));
#117641=DIRECTION('ref_axis',(0.,1.,0.));
#117642=DIRECTION('',(0.,1.23467863058847E-16,-1.));
#117643=DIRECTION('center_axis',(0.,0.,1.));
#117644=DIRECTION('ref_axis',(0.,-1.,0.));
#117645=DIRECTION('',(0.,-1.23467863058847E-16,1.));
#117646=DIRECTION('center_axis',(0.,0.,1.));
#117647=DIRECTION('ref_axis',(0.,1.,0.));
#117648=DIRECTION('',(0.,1.23467863058847E-16,-1.));
#117649=DIRECTION('center_axis',(0.,0.,-1.));
#117650=DIRECTION('ref_axis',(0.,1.,0.));
#117651=DIRECTION('',(0.,-1.23467863058847E-16,1.));
#117652=DIRECTION('center_axis',(0.,0.,1.));
#117653=DIRECTION('ref_axis',(0.,1.,0.));
#117654=DIRECTION('',(0.,1.23467863058847E-16,-1.));
#117655=DIRECTION('center_axis',(0.,0.,-1.));
#117656=DIRECTION('ref_axis',(0.,1.,0.));
#117657=DIRECTION('',(0.,-1.23467863058847E-16,1.));
#117658=DIRECTION('center_axis',(0.,0.,1.));
#117659=DIRECTION('ref_axis',(0.,1.,0.));
#117660=DIRECTION('',(0.,1.23467863058847E-16,-1.));
#117661=DIRECTION('center_axis',(0.,0.,-1.));
#117662=DIRECTION('ref_axis',(0.,1.,0.));
#117663=DIRECTION('',(0.,-1.23467863058847E-16,1.));
#117664=DIRECTION('center_axis',(0.,0.,1.));
#117665=DIRECTION('ref_axis',(0.,1.,0.));
#117666=DIRECTION('',(0.,1.23467863058847E-16,-1.));
#117667=DIRECTION('center_axis',(0.,0.,-1.));
#117668=DIRECTION('ref_axis',(0.,1.,0.));
#117669=DIRECTION('',(0.,-1.23467863058847E-16,1.));
#117670=DIRECTION('center_axis',(0.,0.,1.));
#117671=DIRECTION('ref_axis',(0.,1.,0.));
#117672=DIRECTION('',(0.,1.23467863058847E-16,-1.));
#117673=DIRECTION('center_axis',(0.,0.,-1.));
#117674=DIRECTION('ref_axis',(0.,1.,0.));
#117675=DIRECTION('center_axis',(0.,0.,1.));
#117676=DIRECTION('ref_axis',(0.,1.,0.));
#117677=DIRECTION('',(0.,1.23467863058847E-16,-1.));
#117678=DIRECTION('',(0.,-1.23467863058847E-16,1.));
#117679=DIRECTION('center_axis',(0.,0.,1.));
#117680=DIRECTION('ref_axis',(0.,-1.,0.));
#117681=DIRECTION('',(0.,-1.23467863058847E-16,1.));
#117682=DIRECTION('center_axis',(0.,0.,1.));
#117683=DIRECTION('ref_axis',(0.,1.,0.));
#117684=DIRECTION('',(0.,1.23467863058847E-16,-1.));
#117685=DIRECTION('center_axis',(0.,0.,-1.));
#117686=DIRECTION('ref_axis',(0.,1.,0.));
#117687=DIRECTION('',(0.,-1.23467863058847E-16,1.));
#117688=DIRECTION('center_axis',(0.,0.,1.));
#117689=DIRECTION('ref_axis',(0.,1.,0.));
#117690=DIRECTION('',(0.,1.23467863058847E-16,-1.));
#117691=DIRECTION('center_axis',(0.,0.,1.));
#117692=DIRECTION('ref_axis',(0.,-1.,0.));
#117693=DIRECTION('',(0.,-1.23467863058847E-16,1.));
#117694=DIRECTION('center_axis',(0.,0.,1.));
#117695=DIRECTION('ref_axis',(0.,1.,0.));
#117696=DIRECTION('',(0.,1.23467863058847E-16,-1.));
#117697=DIRECTION('center_axis',(1.3684555315672E-48,0.,-1.));
#117698=DIRECTION('ref_axis',(0.,1.,0.));
#117699=DIRECTION('',(-1.3684555315672E-48,-1.23467863058847E-16,1.));
#117700=DIRECTION('center_axis',(0.,0.,1.));
#117701=DIRECTION('ref_axis',(0.,1.,0.));
#117702=DIRECTION('',(0.,1.23467863058847E-16,-1.));
#117703=DIRECTION('center_axis',(0.,0.,-1.));
#117704=DIRECTION('ref_axis',(0.701138397908223,-0.713025207814346,0.));
#117705=DIRECTION('',(0.,-1.23467863058847E-16,1.));
#117706=DIRECTION('center_axis',(0.,0.,1.));
#117707=DIRECTION('ref_axis',(0.,1.,0.));
#117708=DIRECTION('',(1.3684555315672E-48,1.23467863058847E-16,-1.));
#117709=DIRECTION('center_axis',(0.,0.,1.));
#117710=DIRECTION('ref_axis',(0.,-1.,0.));
#117711=DIRECTION('',(0.,-1.23467863058847E-16,1.));
#117712=DIRECTION('center_axis',(0.,0.,1.));
#117713=DIRECTION('ref_axis',(0.,1.,0.));
#117714=DIRECTION('',(0.,1.23467863058847E-16,-1.));
#117715=DIRECTION('center_axis',(1.3684555315672E-48,0.,-1.));
#117716=DIRECTION('ref_axis',(0.,1.,0.));
#117717=DIRECTION('',(-1.3684555315672E-48,-1.23467863058847E-16,1.));
#117718=DIRECTION('center_axis',(0.,0.,1.));
#117719=DIRECTION('ref_axis',(0.,1.,0.));
#117720=DIRECTION('',(0.,1.23467863058847E-16,-1.));
#117721=DIRECTION('center_axis',(-1.3684555315672E-48,0.,1.));
#117722=DIRECTION('ref_axis',(0.,-1.,0.));
#117723=DIRECTION('',(0.,-1.23467863058847E-16,1.));
#117724=DIRECTION('center_axis',(0.,0.,1.));
#117725=DIRECTION('ref_axis',(0.,1.,0.));
#117726=DIRECTION('',(1.3684555315672E-48,1.23467863058847E-16,-1.));
#117727=DIRECTION('center_axis',(0.,0.,-1.));
#117728=DIRECTION('ref_axis',(0.,1.,0.));
#117729=DIRECTION('',(0.,-1.23467863058847E-16,1.));
#117730=DIRECTION('center_axis',(0.,0.,1.));
#117731=DIRECTION('ref_axis',(0.,1.,0.));
#117732=DIRECTION('',(0.,1.23467863058847E-16,-1.));
#117733=DIRECTION('center_axis',(0.,0.,1.));
#117734=DIRECTION('ref_axis',(0.,-1.,0.));
#117735=DIRECTION('',(0.,-1.23467863058847E-16,1.));
#117736=DIRECTION('center_axis',(0.,0.,1.));
#117737=DIRECTION('ref_axis',(0.,1.,0.));
#117738=DIRECTION('',(0.,1.23467863058847E-16,-1.));
#117739=DIRECTION('center_axis',(1.3684555315672E-48,0.,-1.));
#117740=DIRECTION('ref_axis',(0.,1.,0.));
#117741=DIRECTION('',(-1.3684555315672E-48,-1.23467863058847E-16,1.));
#117742=DIRECTION('center_axis',(0.,0.,1.));
#117743=DIRECTION('ref_axis',(0.,1.,0.));
#117744=DIRECTION('',(0.,1.23467863058847E-16,-1.));
#117745=DIRECTION('center_axis',(-1.3684555315672E-48,0.,1.));
#117746=DIRECTION('ref_axis',(0.,-1.,0.));
#117747=DIRECTION('',(0.,-1.23467863058847E-16,1.));
#117748=DIRECTION('center_axis',(0.,0.,1.));
#117749=DIRECTION('ref_axis',(0.,1.,0.));
#117750=DIRECTION('',(1.3684555315672E-48,1.23467863058847E-16,-1.));
#117751=DIRECTION('center_axis',(0.,0.,-1.));
#117752=DIRECTION('ref_axis',(0.,1.,0.));
#117753=DIRECTION('',(0.,-1.23467863058847E-16,1.));
#117754=DIRECTION('center_axis',(0.,0.,1.));
#117755=DIRECTION('ref_axis',(0.,1.,0.));
#117756=DIRECTION('',(0.,1.23467863058847E-16,-1.));
#117757=DIRECTION('center_axis',(0.,0.,1.));
#117758=DIRECTION('ref_axis',(0.,-1.,0.));
#117759=DIRECTION('',(0.,-1.23467863058847E-16,1.));
#117760=DIRECTION('center_axis',(0.,0.,1.));
#117761=DIRECTION('ref_axis',(0.,1.,0.));
#117762=DIRECTION('',(0.,1.23467863058847E-16,-1.));
#117763=DIRECTION('center_axis',(1.3684555315672E-48,0.,-1.));
#117764=DIRECTION('ref_axis',(0.,1.,0.));
#117765=DIRECTION('',(-1.3684555315672E-48,-1.23467863058847E-16,1.));
#117766=DIRECTION('center_axis',(0.,0.,1.));
#117767=DIRECTION('ref_axis',(0.,1.,0.));
#117768=DIRECTION('',(0.,1.23467863058847E-16,-1.));
#117769=DIRECTION('center_axis',(-1.3684555315672E-48,0.,1.));
#117770=DIRECTION('ref_axis',(0.,-1.,0.));
#117771=DIRECTION('',(0.,-1.23467863058847E-16,1.));
#117772=DIRECTION('center_axis',(0.,0.,1.));
#117773=DIRECTION('ref_axis',(0.,1.,0.));
#117774=DIRECTION('',(1.3684555315672E-48,1.23467863058847E-16,-1.));
#117775=DIRECTION('center_axis',(0.,0.,-1.));
#117776=DIRECTION('ref_axis',(0.,1.,0.));
#117777=DIRECTION('',(0.,-1.23467863058847E-16,1.));
#117778=DIRECTION('center_axis',(0.,0.,1.));
#117779=DIRECTION('ref_axis',(0.,1.,0.));
#117780=DIRECTION('',(0.,1.23467863058847E-16,-1.));
#117781=DIRECTION('center_axis',(0.,0.,-1.));
#117782=DIRECTION('ref_axis',(0.,1.,0.));
#117783=DIRECTION('',(0.,-1.23467863058847E-16,1.));
#117784=DIRECTION('center_axis',(0.,0.,1.));
#117785=DIRECTION('ref_axis',(0.,1.,0.));
#117786=DIRECTION('',(0.,1.23467863058847E-16,-1.));
#117787=DIRECTION('center_axis',(0.,0.,1.));
#117788=DIRECTION('ref_axis',(0.,-1.,0.));
#117789=DIRECTION('',(0.,-1.23467863058847E-16,1.));
#117790=DIRECTION('center_axis',(0.,0.,1.));
#117791=DIRECTION('ref_axis',(0.,1.,0.));
#117792=DIRECTION('',(0.,1.23467863058847E-16,-1.));
#117793=DIRECTION('center_axis',(1.3684555315672E-48,0.,-1.));
#117794=DIRECTION('ref_axis',(0.,1.,0.));
#117795=DIRECTION('',(-1.3684555315672E-48,-1.23467863058847E-16,1.));
#117796=DIRECTION('center_axis',(0.,0.,1.));
#117797=DIRECTION('ref_axis',(0.,1.,0.));
#117798=DIRECTION('',(0.,1.23467863058847E-16,-1.));
#117799=DIRECTION('center_axis',(-1.3684555315672E-48,0.,1.));
#117800=DIRECTION('ref_axis',(0.,-1.,0.));
#117801=DIRECTION('',(0.,-1.23467863058847E-16,1.));
#117802=DIRECTION('center_axis',(0.,0.,1.));
#117803=DIRECTION('ref_axis',(0.,1.,0.));
#117804=DIRECTION('',(1.3684555315672E-48,1.23467863058847E-16,-1.));
#117805=DIRECTION('center_axis',(0.,0.,-1.));
#117806=DIRECTION('ref_axis',(0.,1.,0.));
#117807=DIRECTION('',(0.,-1.23467863058847E-16,1.));
#117808=DIRECTION('center_axis',(0.,0.,1.));
#117809=DIRECTION('ref_axis',(0.,1.,0.));
#117810=DIRECTION('',(0.,1.23467863058847E-16,-1.));
#117811=DIRECTION('center_axis',(0.,0.,-1.));
#117812=DIRECTION('ref_axis',(0.,1.,0.));
#117813=DIRECTION('',(0.,-1.23467863058847E-16,1.));
#117814=DIRECTION('center_axis',(0.,0.,1.));
#117815=DIRECTION('ref_axis',(0.,1.,0.));
#117816=DIRECTION('',(0.,1.23467863058847E-16,-1.));
#117817=DIRECTION('center_axis',(0.,0.,-1.));
#117818=DIRECTION('ref_axis',(0.,1.,0.));
#117819=DIRECTION('center_axis',(0.,0.,1.));
#117820=DIRECTION('ref_axis',(0.,1.,0.));
#117821=DIRECTION('',(0.,1.23467863058847E-16,-1.));
#117822=DIRECTION('',(-1.3684555315672E-48,-1.23467863058847E-16,1.));
#117823=DIRECTION('center_axis',(-1.3684555315672E-48,0.,1.));
#117824=DIRECTION('ref_axis',(0.,-1.,0.));
#117825=DIRECTION('',(-1.3684555315672E-48,-1.23467863058847E-16,1.));
#117826=DIRECTION('center_axis',(0.,0.,1.));
#117827=DIRECTION('ref_axis',(0.,1.,0.));
#117828=DIRECTION('',(1.3684555315672E-48,1.23467863058847E-16,-1.));
#117829=DIRECTION('center_axis',(0.,0.,-1.));
#117830=DIRECTION('ref_axis',(0.,1.,0.));
#117831=DIRECTION('',(0.,-1.23467863058847E-16,1.));
#117832=DIRECTION('center_axis',(0.,0.,1.));
#117833=DIRECTION('ref_axis',(0.,1.,0.));
#117834=DIRECTION('',(0.,1.23467863058847E-16,-1.));
#117835=DIRECTION('center_axis',(0.,0.,1.));
#117836=DIRECTION('ref_axis',(0.,-1.,0.));
#117837=DIRECTION('',(0.,-1.23467863058847E-16,1.));
#117838=DIRECTION('center_axis',(0.,0.,1.));
#117839=DIRECTION('ref_axis',(0.,1.,0.));
#117840=DIRECTION('',(0.,1.23467863058847E-16,-1.));
#117841=DIRECTION('center_axis',(0.,0.,-1.));
#117842=DIRECTION('ref_axis',(0.,1.,0.));
#117843=DIRECTION('',(0.,-1.23467863058847E-16,1.));
#117844=DIRECTION('center_axis',(0.,0.,1.));
#117845=DIRECTION('ref_axis',(0.,1.,0.));
#117846=DIRECTION('',(0.,1.23467863058847E-16,-1.));
#117847=DIRECTION('center_axis',(0.,0.,-1.));
#117848=DIRECTION('ref_axis',(0.706453380948025,-0.707759578209369,0.));
#117849=DIRECTION('',(0.,-1.23467863058847E-16,1.));
#117850=DIRECTION('center_axis',(0.,0.,1.));
#117851=DIRECTION('ref_axis',(0.,1.,0.));
#117852=DIRECTION('',(0.,1.23467863058847E-16,-1.));
#117853=DIRECTION('center_axis',(0.,0.,1.));
#117854=DIRECTION('ref_axis',(0.,-1.,0.));
#117855=DIRECTION('',(0.,-1.23467863058847E-16,1.));
#117856=DIRECTION('center_axis',(0.,0.,1.));
#117857=DIRECTION('ref_axis',(0.,1.,0.));
#117858=DIRECTION('',(0.,1.23467863058847E-16,-1.));
#117859=DIRECTION('center_axis',(0.,0.,-1.));
#117860=DIRECTION('ref_axis',(0.,1.,0.));
#117861=DIRECTION('',(0.,-1.23467863058847E-16,1.));
#117862=DIRECTION('center_axis',(0.,0.,1.));
#117863=DIRECTION('ref_axis',(0.,1.,0.));
#117864=DIRECTION('',(0.,1.23467863058847E-16,-1.));
#117865=DIRECTION('center_axis',(0.,0.,1.));
#117866=DIRECTION('ref_axis',(0.,-1.,0.));
#117867=DIRECTION('',(0.,-1.23467863058847E-16,1.));
#117868=DIRECTION('center_axis',(0.,0.,1.));
#117869=DIRECTION('ref_axis',(0.,1.,0.));
#117870=DIRECTION('',(0.,1.23467863058847E-16,-1.));
#117871=DIRECTION('center_axis',(0.,0.,-1.));
#117872=DIRECTION('ref_axis',(0.,1.,0.));
#117873=DIRECTION('',(0.,-1.23467863058847E-16,1.));
#117874=DIRECTION('center_axis',(0.,0.,1.));
#117875=DIRECTION('ref_axis',(0.,1.,0.));
#117876=DIRECTION('',(0.,1.23467863058847E-16,-1.));
#117877=DIRECTION('center_axis',(0.,0.,-1.));
#117878=DIRECTION('ref_axis',(0.,1.,0.));
#117879=DIRECTION('',(0.,-1.23467863058847E-16,1.));
#117880=DIRECTION('center_axis',(0.,0.,1.));
#117881=DIRECTION('ref_axis',(0.,1.,0.));
#117882=DIRECTION('',(0.,1.23467863058847E-16,-1.));
#117883=DIRECTION('center_axis',(0.,0.,1.));
#117884=DIRECTION('ref_axis',(0.,-1.,0.));
#117885=DIRECTION('',(0.,-1.23467863058847E-16,1.));
#117886=DIRECTION('center_axis',(0.,0.,1.));
#117887=DIRECTION('ref_axis',(0.,1.,0.));
#117888=DIRECTION('',(0.,1.23467863058847E-16,-1.));
#117889=DIRECTION('center_axis',(0.,0.,-1.));
#117890=DIRECTION('ref_axis',(0.,1.,0.));
#117891=DIRECTION('',(0.,-1.23467863058847E-16,1.));
#117892=DIRECTION('center_axis',(0.,0.,1.));
#117893=DIRECTION('ref_axis',(0.,1.,0.));
#117894=DIRECTION('',(0.,1.23467863058847E-16,-1.));
#117895=DIRECTION('center_axis',(0.,0.,1.));
#117896=DIRECTION('ref_axis',(0.,-1.,0.));
#117897=DIRECTION('',(0.,-1.23467863058847E-16,1.));
#117898=DIRECTION('center_axis',(0.,0.,1.));
#117899=DIRECTION('ref_axis',(0.,1.,0.));
#117900=DIRECTION('',(0.,1.23467863058847E-16,-1.));
#117901=DIRECTION('center_axis',(0.,0.,-1.));
#117902=DIRECTION('ref_axis',(0.,1.,0.));
#117903=DIRECTION('',(0.,-1.23467863058847E-16,1.));
#117904=DIRECTION('center_axis',(0.,0.,1.));
#117905=DIRECTION('ref_axis',(0.,1.,0.));
#117906=DIRECTION('',(0.,1.23467863058847E-16,-1.));
#117907=DIRECTION('center_axis',(0.,0.,-1.));
#117908=DIRECTION('ref_axis',(0.,1.,0.));
#117909=DIRECTION('',(0.,-1.23467863058847E-16,1.));
#117910=DIRECTION('center_axis',(0.,0.,1.));
#117911=DIRECTION('ref_axis',(0.,1.,0.));
#117912=DIRECTION('',(0.,1.23467863058847E-16,-1.));
#117913=DIRECTION('center_axis',(0.,0.,-1.));
#117914=DIRECTION('ref_axis',(0.,1.,0.));
#117915=DIRECTION('center_axis',(0.,0.,1.));
#117916=DIRECTION('ref_axis',(0.,1.,0.));
#117917=DIRECTION('',(0.,1.23467863058847E-16,-1.));
#117918=DIRECTION('',(0.,-1.23467863058847E-16,1.));
#117919=DIRECTION('center_axis',(0.,0.,1.));
#117920=DIRECTION('ref_axis',(0.,-1.,0.));
#117921=DIRECTION('',(0.,-1.23467863058847E-16,1.));
#117922=DIRECTION('center_axis',(0.,0.,1.));
#117923=DIRECTION('ref_axis',(0.,1.,0.));
#117924=DIRECTION('',(0.,1.23467863058847E-16,-1.));
#117925=DIRECTION('center_axis',(0.,0.,-1.));
#117926=DIRECTION('ref_axis',(-0.0361435302645155,-0.999346609150208,0.));
#117927=DIRECTION('',(0.,-1.23467863058847E-16,1.));
#117928=DIRECTION('center_axis',(0.,0.,1.));
#117929=DIRECTION('ref_axis',(0.,1.,0.));
#117930=DIRECTION('',(1.27503726478586E-32,1.23467863058847E-16,-1.));
#117931=DIRECTION('center_axis',(0.,0.,-1.));
#117932=DIRECTION('ref_axis',(0.,1.,0.));
#117933=DIRECTION('',(0.,-1.23467863058847E-16,1.));
#117934=DIRECTION('center_axis',(0.,0.,1.));
#117935=DIRECTION('ref_axis',(0.,1.,0.));
#117936=DIRECTION('',(0.,1.23467863058847E-16,-1.));
#117937=DIRECTION('center_axis',(0.,0.,-1.));
#117938=DIRECTION('ref_axis',(0.,1.,0.));
#117939=DIRECTION('',(0.,-1.23467863058847E-16,1.));
#117940=DIRECTION('center_axis',(0.,0.,1.));
#117941=DIRECTION('ref_axis',(0.,1.,0.));
#117942=DIRECTION('',(0.,1.23467863058847E-16,-1.));
#117943=DIRECTION('center_axis',(0.,0.,-1.));
#117944=DIRECTION('ref_axis',(0.,1.,0.));
#117945=DIRECTION('center_axis',(0.,0.,1.));
#117946=DIRECTION('ref_axis',(0.,1.,0.));
#117947=DIRECTION('',(0.,1.23467863058847E-16,-1.));
#117948=DIRECTION('',(0.,-1.23467863058847E-16,1.));
#117949=DIRECTION('center_axis',(0.,0.,-1.));
#117950=DIRECTION('ref_axis',(0.663057938251906,-0.748568080084324,0.));
#117951=DIRECTION('',(0.,-1.23467863058847E-16,1.));
#117952=DIRECTION('center_axis',(0.,0.,1.));
#117953=DIRECTION('ref_axis',(0.,1.,0.));
#117954=DIRECTION('',(0.,1.23467863058847E-16,-1.));
#117955=DIRECTION('center_axis',(0.,0.,-1.));
#117956=DIRECTION('ref_axis',(0.,1.,0.));
#117957=DIRECTION('center_axis',(0.,0.,1.));
#117958=DIRECTION('ref_axis',(0.,1.,0.));
#117959=DIRECTION('',(0.,1.23467863058847E-16,-1.));
#117960=DIRECTION('',(0.,-1.23467863058847E-16,1.));
#117961=DIRECTION('center_axis',(0.,0.,-1.));
#117962=DIRECTION('ref_axis',(0.,1.,0.));
#117963=DIRECTION('',(-3.82498197630791E-33,-1.23467863058847E-16,1.));
#117964=DIRECTION('center_axis',(0.,0.,1.));
#117965=DIRECTION('ref_axis',(0.,1.,0.));
#117966=DIRECTION('',(0.,1.23467863058847E-16,-1.));
#117967=DIRECTION('center_axis',(0.,0.,-1.));
#117968=DIRECTION('ref_axis',(0.,1.,0.));
#117969=DIRECTION('',(0.,-1.23467863058847E-16,1.));
#117970=DIRECTION('center_axis',(0.,0.,1.));
#117971=DIRECTION('ref_axis',(0.,1.,0.));
#117972=DIRECTION('',(1.3684555315672E-48,1.23467863058847E-16,-1.));
#117973=DIRECTION('center_axis',(0.,0.,-1.));
#117974=DIRECTION('ref_axis',(0.,1.,0.));
#117975=DIRECTION('',(-1.3684555315672E-48,-1.23467863058847E-16,1.));
#117976=DIRECTION('center_axis',(0.,0.,1.));
#117977=DIRECTION('ref_axis',(0.,1.,0.));
#117978=DIRECTION('',(0.,1.23467863058847E-16,-1.));
#117979=DIRECTION('center_axis',(0.,0.,-1.));
#117980=DIRECTION('ref_axis',(0.,1.,0.));
#117981=DIRECTION('',(0.,-1.23467863058847E-16,1.));
#117982=DIRECTION('center_axis',(0.,0.,1.));
#117983=DIRECTION('ref_axis',(0.,1.,0.));
#117984=DIRECTION('center_axis',(0.,0.,-1.));
#117985=DIRECTION('ref_axis',(0.,1.,0.));
#117986=DIRECTION('center_axis',(0.,0.,1.));
#117987=DIRECTION('ref_axis',(0.,1.,0.));
#117988=DIRECTION('',(0.,1.23467863058847E-16,-1.));
#117989=DIRECTION('center_axis',(0.,0.,-1.));
#117990=DIRECTION('ref_axis',(0.,1.,0.));
#117991=DIRECTION('center_axis',(0.,0.,-1.));
#117992=DIRECTION('ref_axis',(0.,1.,0.));
#117993=DIRECTION('center_axis',(0.,0.,-1.));
#117994=DIRECTION('ref_axis',(0.,1.,0.));
#117995=DIRECTION('center_axis',(-5.48307457476793E-31,2.43497425545765E-45,
-1.));
#117996=DIRECTION('ref_axis',(4.44089209850063E-15,1.,-3.42265840282363E-60));
#117997=DIRECTION('center_axis',(0.,0.,-1.));
#117998=DIRECTION('ref_axis',(0.,1.,0.));
#117999=DIRECTION('center_axis',(0.,0.,-1.));
#118000=DIRECTION('ref_axis',(0.,1.,0.));
#118001=DIRECTION('center_axis',(-0.724113717892013,0.689680595319751,8.51533892972833E-17));
#118002=DIRECTION('ref_axis',(1.17596707800504E-16,6.08324121309175E-33,
1.));
#118003=DIRECTION('',(0.689680595319751,0.724113717892013,8.9404773359724E-17));
#118004=DIRECTION('center_axis',(0.724113717892013,-0.689680595319751,-8.51533892972834E-17));
#118005=DIRECTION('ref_axis',(4.33608168928332E-33,1.23467863058847E-16,
-1.));
#118006=DIRECTION('',(-0.689680595319751,-0.724113717892013,-8.9404773359724E-17));
#118007=DIRECTION('center_axis',(0.,0.,-1.));
#118008=DIRECTION('ref_axis',(0.,1.,0.));
#118009=DIRECTION('center_axis',(2.19322982990717E-31,3.89595880873225E-46,
-1.));
#118010=DIRECTION('ref_axis',(-1.77635683940025E-15,1.,7.77876909732643E-62));
#118011=DIRECTION('center_axis',(0.,0.,-1.));
#118012=DIRECTION('ref_axis',(0.,1.,0.));
#118013=DIRECTION('center_axis',(-4.38645965981435E-31,1.5583835234929E-45,
-1.));
#118014=DIRECTION('ref_axis',(3.5527136788005E-15,1.,-9.33452291679171E-61));
#118015=DIRECTION('center_axis',(0.,0.,-1.));
#118016=DIRECTION('ref_axis',(0.,1.,0.));
#118017=DIRECTION('center_axis',(7.6763044046751E-31,4.77254954069701E-45,
-1.));
#118018=DIRECTION('ref_axis',(-6.21724893790088E-15,1.,-1.86690458335834E-60));
#118019=DIRECTION('center_axis',(0.724113717892013,0.689680595319752,8.51533892972834E-17));
#118020=DIRECTION('ref_axis',(1.94663562866425E-33,1.23467863058847E-16,
-1.));
#118021=DIRECTION('',(0.689680595319752,-0.724113717892012,-8.94047733597238E-17));
#118022=DIRECTION('center_axis',(-0.724113717892013,-0.689680595319752,
-8.51533892972833E-17));
#118023=DIRECTION('ref_axis',(-0.689680595319752,0.724113717892013,-1.8658423912347E-33));
#118024=DIRECTION('',(-0.689680595319752,0.724113717892012,8.94047733597238E-17));
#118025=DIRECTION('center_axis',(0.,0.,-1.));
#118026=DIRECTION('ref_axis',(0.,1.,0.));
#118027=DIRECTION('center_axis',(-1.09661491495359E-31,9.73989702183063E-47,
-1.));
#118028=DIRECTION('ref_axis',(8.88178419700125E-16,1.,0.));
#118029=DIRECTION('center_axis',(0.,0.,-1.));
#118030=DIRECTION('ref_axis',(0.,1.,0.));
#118031=DIRECTION('center_axis',(-9.86953423458227E-31,7.88931658768281E-45,
-1.));
#118032=DIRECTION('ref_axis',(7.99360577730113E-15,1.,-2.48920611114446E-60));
#118033=DIRECTION('center_axis',(-1.,0.,0.));
#118034=DIRECTION('ref_axis',(0.,0.,1.));
#118035=DIRECTION('',(0.,1.,0.));
#118036=DIRECTION('center_axis',(1.,0.,0.));
#118037=DIRECTION('ref_axis',(0.,1.,0.));
#118038=DIRECTION('',(0.,-1.,0.));
#118039=DIRECTION('center_axis',(1.,0.,0.));
#118040=DIRECTION('ref_axis',(0.,1.,0.));
#118041=DIRECTION('',(0.,-1.,0.));
#118042=DIRECTION('center_axis',(-1.,0.,0.));
#118043=DIRECTION('ref_axis',(0.,0.,1.));
#118044=DIRECTION('',(0.,1.,0.));
#118045=DIRECTION('center_axis',(1.,0.,0.));
#118046=DIRECTION('ref_axis',(0.,1.,0.));
#118047=DIRECTION('',(0.,-1.,0.));
#118048=DIRECTION('center_axis',(-1.,0.,0.));
#118049=DIRECTION('ref_axis',(0.,0.,1.));
#118050=DIRECTION('',(0.,1.,0.));
#118051=DIRECTION('center_axis',(1.,0.,0.));
#118052=DIRECTION('ref_axis',(0.,1.,0.));
#118053=DIRECTION('',(0.,-1.,0.));
#118054=DIRECTION('center_axis',(-1.,0.,0.));
#118055=DIRECTION('ref_axis',(0.,0.,1.));
#118056=DIRECTION('',(0.,1.,0.));
#118057=DIRECTION('center_axis',(1.,0.,0.));
#118058=DIRECTION('ref_axis',(0.,1.,0.));
#118059=DIRECTION('',(0.,-1.,0.));
#118060=DIRECTION('center_axis',(-1.,0.,0.));
#118061=DIRECTION('ref_axis',(0.,0.,1.));
#118062=DIRECTION('',(0.,1.,0.));
#118063=DIRECTION('center_axis',(1.,0.,0.));
#118064=DIRECTION('ref_axis',(0.,1.,0.));
#118065=DIRECTION('',(0.,-1.,0.));
#118066=DIRECTION('center_axis',(-1.,0.,0.));
#118067=DIRECTION('ref_axis',(0.,0.,1.));
#118068=DIRECTION('',(0.,1.,0.));
#118069=DIRECTION('center_axis',(1.,0.,0.));
#118070=DIRECTION('ref_axis',(0.,1.,0.));
#118071=DIRECTION('',(0.,-1.,0.));
#118072=DIRECTION('center_axis',(-1.,0.,0.));
#118073=DIRECTION('ref_axis',(0.,0.,1.));
#118074=DIRECTION('',(0.,1.,0.));
#118075=DIRECTION('center_axis',(1.,0.,0.));
#118076=DIRECTION('ref_axis',(0.,1.,0.));
#118077=DIRECTION('',(0.,-1.,0.));
#118078=DIRECTION('center_axis',(-1.,0.,0.));
#118079=DIRECTION('ref_axis',(0.,0.,1.));
#118080=DIRECTION('',(0.,1.,0.));
#118081=DIRECTION('center_axis',(-1.,7.82779334765923E-17,9.66480917101747E-33));
#118082=DIRECTION('ref_axis',(9.66480917101747E-33,0.,1.));
#118083=DIRECTION('',(7.82779334765923E-17,1.,0.));
#118084=DIRECTION('center_axis',(1.,7.82779334765923E-17,9.66480917101747E-33));
#118085=DIRECTION('ref_axis',(-7.82779334765923E-17,1.,1.39213059235047E-65));
#118086=DIRECTION('',(7.82779334765923E-17,-1.,0.));
#118087=DIRECTION('center_axis',(1.,7.82779334765923E-17,9.66480917101747E-33));
#118088=DIRECTION('ref_axis',(-7.82779334765923E-17,1.,1.39213059235047E-65));
#118089=DIRECTION('',(7.82779334765923E-17,-1.,0.));
#118090=DIRECTION('center_axis',(-1.,7.82779334765923E-17,9.66480917101747E-33));
#118091=DIRECTION('ref_axis',(9.66480917101747E-33,0.,1.));
#118092=DIRECTION('',(7.82779334765923E-17,1.,0.));
#118093=DIRECTION('center_axis',(1.,7.82779334765923E-17,9.66480917101747E-33));
#118094=DIRECTION('ref_axis',(-7.82779334765923E-17,1.,1.39213059235047E-65));
#118095=DIRECTION('',(7.82779334765923E-17,-1.,0.));
#118096=DIRECTION('center_axis',(-1.,7.82779334765923E-17,9.66480917101747E-33));
#118097=DIRECTION('ref_axis',(9.66480917101747E-33,0.,1.));
#118098=DIRECTION('',(7.82779334765923E-17,1.,0.));
#118099=DIRECTION('center_axis',(1.,7.82779334765923E-17,9.66480917101747E-33));
#118100=DIRECTION('ref_axis',(-7.82779334765923E-17,1.,1.39213059235047E-65));
#118101=DIRECTION('',(7.82779334765923E-17,-1.,0.));
#118102=DIRECTION('center_axis',(-1.,7.82779334765923E-17,9.66480917101747E-33));
#118103=DIRECTION('ref_axis',(9.66480917101747E-33,0.,1.));
#118104=DIRECTION('',(7.82779334765923E-17,1.,0.));
#118105=DIRECTION('center_axis',(1.,7.82779334765923E-17,9.66480917101747E-33));
#118106=DIRECTION('ref_axis',(-7.82779334765923E-17,1.,1.39213059235047E-65));
#118107=DIRECTION('',(7.82779334765923E-17,-1.,0.));
#118108=DIRECTION('center_axis',(-1.,7.82779334765923E-17,9.66480917101747E-33));
#118109=DIRECTION('ref_axis',(9.66480917101747E-33,0.,1.));
#118110=DIRECTION('',(7.82779334765923E-17,1.,0.));
#118111=DIRECTION('center_axis',(1.,7.82779334765923E-17,9.66480917101747E-33));
#118112=DIRECTION('ref_axis',(-7.82779334765923E-17,1.,1.39213059235047E-65));
#118113=DIRECTION('',(7.82779334765923E-17,-1.,0.));
#118114=DIRECTION('center_axis',(-1.,7.82779334765923E-17,9.66480917101747E-33));
#118115=DIRECTION('ref_axis',(9.66480917101747E-33,0.,1.));
#118116=DIRECTION('',(7.82779334765923E-17,1.,0.));
#118117=DIRECTION('center_axis',(1.,7.82779334765923E-17,9.66480917101747E-33));
#118118=DIRECTION('ref_axis',(-7.82779334765923E-17,1.,1.39213059235047E-65));
#118119=DIRECTION('',(7.82779334765923E-17,-1.,0.));
#118120=DIRECTION('center_axis',(-1.,7.82779334765923E-17,9.66480917101747E-33));
#118121=DIRECTION('ref_axis',(9.66480917101747E-33,0.,1.));
#118122=DIRECTION('',(7.82779334765923E-17,1.,0.));
#118123=DIRECTION('center_axis',(1.,7.82779334765923E-17,9.66480917101747E-33));
#118124=DIRECTION('ref_axis',(-7.82779334765923E-17,1.,1.39213059235047E-65));
#118125=DIRECTION('',(7.82779334765923E-17,-1.,0.));
#118126=DIRECTION('center_axis',(-1.,7.82779334765923E-17,9.66480917101747E-33));
#118127=DIRECTION('ref_axis',(9.66480917101747E-33,0.,1.));
#118128=DIRECTION('',(7.82779334765923E-17,1.,0.));
#118129=DIRECTION('center_axis',(0.,-1.,-1.23467863058847E-16));
#118130=DIRECTION('ref_axis',(0.,1.23467863058847E-16,-1.));
#118131=DIRECTION('',(0.,-1.23467863058847E-16,1.));
#118132=DIRECTION('',(-1.,0.,0.));
#118133=DIRECTION('',(0.,-1.23467863058847E-16,1.));
#118134=DIRECTION('',(1.,0.,0.));
#118135=DIRECTION('center_axis',(1.,7.82779334765923E-17,9.66480917101747E-33));
#118136=DIRECTION('ref_axis',(-7.82779334765923E-17,1.,1.39213059235047E-65));
#118137=DIRECTION('',(0.,-1.23467863058847E-16,1.));
#118138=DIRECTION('',(7.82779334765923E-17,-1.,0.));
#118139=DIRECTION('',(-7.82779334765923E-17,1.,1.23467863058847E-16));
#118140=DIRECTION('center_axis',(-1.,7.82779334765923E-17,9.66480917101747E-33));
#118141=DIRECTION('ref_axis',(9.66480917101747E-33,0.,1.));
#118142=DIRECTION('',(7.82779334765923E-17,1.,0.));
#118143=DIRECTION('',(0.,1.23467863058847E-16,-1.));
#118144=DIRECTION('',(-7.82779334765923E-17,-1.,-1.23467863058847E-16));
#118145=DIRECTION('center_axis',(-1.,-3.13111733906369E-16,-3.86592366840699E-32));
#118146=DIRECTION('ref_axis',(-3.13111733906369E-16,1.,9.91259258008946E-64));
#118147=DIRECTION('',(-3.13111733906369E-16,1.,0.));
#118148=DIRECTION('center_axis',(1.,5.87084501074442E-17,7.2486068782631E-33));
#118149=DIRECTION('ref_axis',(-5.87084501074442E-17,1.,-2.58656569862219E-65));
#118150=DIRECTION('',(5.87084501074442E-17,-1.,0.));
#118151=DIRECTION('center_axis',(1.,5.87084501074442E-17,7.2486068782631E-33));
#118152=DIRECTION('ref_axis',(-5.87084501074442E-17,1.,-2.58656569862219E-65));
#118153=DIRECTION('',(5.87084501074442E-17,-1.,0.));
#118154=DIRECTION('center_axis',(-1.,-3.13111733906369E-16,-3.86592366840699E-32));
#118155=DIRECTION('ref_axis',(-3.13111733906369E-16,1.,9.91259258008946E-64));
#118156=DIRECTION('',(-3.13111733906369E-16,1.,0.));
#118157=DIRECTION('center_axis',(1.,5.87084501074442E-17,7.2486068782631E-33));
#118158=DIRECTION('ref_axis',(-5.87084501074442E-17,1.,-2.58656569862219E-65));
#118159=DIRECTION('',(5.87084501074442E-17,-1.,0.));
#118160=DIRECTION('center_axis',(-1.,-3.13111733906369E-16,-3.86592366840699E-32));
#118161=DIRECTION('ref_axis',(-3.13111733906369E-16,1.,9.91259258008946E-64));
#118162=DIRECTION('',(-3.13111733906369E-16,1.,0.));
#118163=DIRECTION('center_axis',(1.,5.87084501074442E-17,7.2486068782631E-33));
#118164=DIRECTION('ref_axis',(-5.87084501074442E-17,1.,-2.58656569862219E-65));
#118165=DIRECTION('',(5.87084501074442E-17,-1.,0.));
#118166=DIRECTION('center_axis',(-1.,-3.13111733906369E-16,-3.86592366840699E-32));
#118167=DIRECTION('ref_axis',(-3.13111733906369E-16,1.,9.91259258008946E-64));
#118168=DIRECTION('',(-3.13111733906369E-16,1.,0.));
#118169=DIRECTION('center_axis',(1.,5.87084501074442E-17,7.2486068782631E-33));
#118170=DIRECTION('ref_axis',(-5.87084501074442E-17,1.,-2.58656569862219E-65));
#118171=DIRECTION('',(5.87084501074442E-17,-1.,0.));
#118172=DIRECTION('center_axis',(1.,5.87084501074442E-17,7.2486068782631E-33));
#118173=DIRECTION('ref_axis',(-5.87084501074442E-17,1.,-2.58656569862219E-65));
#118174=DIRECTION('',(5.87084501074442E-17,-1.,0.));
#118175=DIRECTION('center_axis',(1.,5.87084501074442E-17,7.2486068782631E-33));
#118176=DIRECTION('ref_axis',(-5.87084501074442E-17,1.,-2.58656569862219E-65));
#118177=DIRECTION('',(5.87084501074442E-17,-1.,0.));
#118178=DIRECTION('center_axis',(-1.,-3.13111733906369E-16,-3.86592366840699E-32));
#118179=DIRECTION('ref_axis',(-3.13111733906369E-16,1.,9.91259258008946E-64));
#118180=DIRECTION('',(-3.13111733906369E-16,1.,0.));
#118181=DIRECTION('center_axis',(1.,5.87084501074442E-17,7.2486068782631E-33));
#118182=DIRECTION('ref_axis',(-5.87084501074442E-17,1.,-2.58656569862219E-65));
#118183=DIRECTION('',(5.87084501074442E-17,-1.,0.));
#118184=DIRECTION('center_axis',(-1.,-3.13111733906369E-16,-3.86592366840699E-32));
#118185=DIRECTION('ref_axis',(-3.13111733906369E-16,1.,9.91259258008946E-64));
#118186=DIRECTION('',(-3.13111733906369E-16,1.,0.));
#118187=DIRECTION('center_axis',(1.,6.11546355285877E-17,7.5506321648574E-33));
#118188=DIRECTION('ref_axis',(-6.11546355285877E-17,1.,2.57447640954701E-65));
#118189=DIRECTION('',(6.11546355285877E-17,-1.,0.));
#118190=DIRECTION('center_axis',(1.,6.11546355285877E-17,7.5506321648574E-33));
#118191=DIRECTION('ref_axis',(-6.11546355285877E-17,1.,2.57447640954701E-65));
#118192=DIRECTION('',(6.11546355285877E-17,-1.,0.));
#118193=DIRECTION('center_axis',(1.,6.11546355285877E-17,7.5506321648574E-33));
#118194=DIRECTION('ref_axis',(-6.11546355285877E-17,1.,2.57447640954701E-65));
#118195=DIRECTION('',(6.11546355285877E-17,-1.,0.));
#118196=DIRECTION('center_axis',(1.,6.11546355285877E-17,7.5506321648574E-33));
#118197=DIRECTION('ref_axis',(-6.11546355285877E-17,1.,2.57447640954701E-65));
#118198=DIRECTION('',(6.11546355285877E-17,-1.,0.));
#118199=DIRECTION('center_axis',(1.,6.11546355285877E-17,7.5506321648574E-33));
#118200=DIRECTION('ref_axis',(-6.11546355285877E-17,1.,2.57447640954701E-65));
#118201=DIRECTION('',(6.11546355285877E-17,-1.,0.));
#118202=DIRECTION('center_axis',(1.,6.11546355285877E-17,7.5506321648574E-33));
#118203=DIRECTION('ref_axis',(-6.11546355285877E-17,1.,2.57447640954701E-65));
#118204=DIRECTION('',(6.11546355285877E-17,-1.,0.));
#118205=DIRECTION('center_axis',(1.,6.11546355285877E-17,7.5506321648574E-33));
#118206=DIRECTION('ref_axis',(-6.11546355285877E-17,1.,2.57447640954701E-65));
#118207=DIRECTION('',(6.11546355285877E-17,-1.,0.));
#118208=DIRECTION('center_axis',(1.,6.11546355285877E-17,7.5506321648574E-33));
#118209=DIRECTION('ref_axis',(-6.11546355285877E-17,1.,2.57447640954701E-65));
#118210=DIRECTION('',(6.11546355285877E-17,-1.,0.));
#118211=DIRECTION('center_axis',(0.,0.,-1.));
#118212=DIRECTION('ref_axis',(0.,1.,0.));
#118213=DIRECTION('',(0.,1.23467863058847E-16,-1.));
#118214=DIRECTION('center_axis',(0.,0.,1.));
#118215=DIRECTION('ref_axis',(0.,1.,0.));
#118216=DIRECTION('',(0.,1.23467863058847E-16,-1.));
#118217=DIRECTION('center_axis',(0.,0.,1.));
#118218=DIRECTION('ref_axis',(0.,1.,0.));
#118219=DIRECTION('center_axis',(0.,0.,-1.));
#118220=DIRECTION('ref_axis',(0.,1.,0.));
#118221=DIRECTION('center_axis',(-2.19322982990717E-31,3.89595880873225E-46,
-1.));
#118222=DIRECTION('ref_axis',(1.77635683940025E-15,1.,1.55575381946529E-61));
#118223=DIRECTION('',(0.,1.23467863058847E-16,-1.));
#118224=DIRECTION('center_axis',(0.,0.,1.));
#118225=DIRECTION('ref_axis',(0.,1.,0.));
#118226=DIRECTION('center_axis',(0.,0.,-1.));
#118227=DIRECTION('ref_axis',(0.,1.,0.));
#118228=DIRECTION('center_axis',(0.,0.,1.));
#118229=DIRECTION('ref_axis',(0.,1.,0.));
#118230=DIRECTION('',(0.,1.23467863058847E-16,-1.));
#118231=DIRECTION('center_axis',(0.,0.,1.));
#118232=DIRECTION('ref_axis',(0.,1.,0.));
#118233=DIRECTION('center_axis',(0.,1.22462808028055E-16,-1.));
#118234=DIRECTION('ref_axis',(0.,1.,1.22462808028055E-16));
#118235=DIRECTION('center_axis',(0.,-1.22462808028055E-16,1.));
#118236=DIRECTION('ref_axis',(0.,1.,1.22462808028055E-16));
#118237=DIRECTION('',(0.,1.23467863058847E-16,-1.));
#118238=DIRECTION('center_axis',(0.,-1.22462808028055E-16,1.));
#118239=DIRECTION('ref_axis',(0.,1.,1.22462808028055E-16));
#118240=DIRECTION('center_axis',(0.,0.,-1.));
#118241=DIRECTION('ref_axis',(0.,1.,0.));
#118242=DIRECTION('center_axis',(0.,0.,1.));
#118243=DIRECTION('ref_axis',(0.,1.,0.));
#118244=DIRECTION('',(0.,1.23467863058847E-16,-1.));
#118245=DIRECTION('center_axis',(0.,0.,1.));
#118246=DIRECTION('ref_axis',(0.,1.,0.));
#118247=DIRECTION('center_axis',(0.,0.,-1.));
#118248=DIRECTION('ref_axis',(0.,1.,0.));
#118249=DIRECTION('center_axis',(4.38645965981435E-31,1.5583835234929E-45,
-1.));
#118250=DIRECTION('ref_axis',(-3.5527136788005E-15,1.,-9.33452291679171E-61));
#118251=DIRECTION('',(0.,1.23467863058847E-16,-1.));
#118252=DIRECTION('center_axis',(0.,0.,1.));
#118253=DIRECTION('ref_axis',(0.,1.,0.));
#118254=DIRECTION('center_axis',(0.,0.,-1.));
#118255=DIRECTION('ref_axis',(0.,1.,0.));
#118256=DIRECTION('center_axis',(0.,0.,1.));
#118257=DIRECTION('ref_axis',(0.,1.,0.));
#118258=DIRECTION('',(0.,1.23467863058847E-16,-1.));
#118259=DIRECTION('center_axis',(0.,0.,1.));
#118260=DIRECTION('ref_axis',(0.,1.,0.));
#118261=DIRECTION('center_axis',(0.,-1.23467863058847E-16,1.));
#118262=DIRECTION('ref_axis',(0.,-1.,-1.23467863058847E-16));
#118263=DIRECTION('',(-0.700366780446485,-0.713783141330072,-8.81292791474553E-17));
#118264=DIRECTION('center_axis',(0.,0.,1.));
#118265=DIRECTION('ref_axis',(0.,-1.,0.));
#118266=DIRECTION('',(0.700366780446451,0.713783141330105,8.81292791474594E-17));
#118267=DIRECTION('center_axis',(0.713783141330072,-0.700366780446485,-8.64727897391324E-17));
#118268=DIRECTION('ref_axis',(-4.34651812646493E-33,1.23467863058847E-16,
-1.));
#118269=DIRECTION('',(0.0133576962200374,0.0136135788205688,-0.999818104668739));
#118270=DIRECTION('center_axis',(0.,1.23467863058847E-16,-1.));
#118271=DIRECTION('ref_axis',(-1.,0.,0.));
#118272=DIRECTION('center_axis',(-7.1617481931302E-31,4.1541690210802E-45,
-1.));
#118273=DIRECTION('ref_axis',(5.80049578546342E-15,1.,-2.48920611114446E-60));
#118274=DIRECTION('',(-0.70592193778968,0.708289642552581,8.74510085926821E-17));
#118275=DIRECTION('center_axis',(-0.708289642552581,-0.70592193778968,-8.71586731452524E-17));
#118276=DIRECTION('ref_axis',(-0.70592193778968,0.708289642552581,-2.39349531189888E-34));
#118277=DIRECTION('',(0.0134621338381862,-0.0135072866467963,-0.999818145544461));
#118278=DIRECTION('center_axis',(-0.966292363511968,0.257447214431338,3.17864574162902E-17));
#118279=DIRECTION('ref_axis',(3.28952795412384E-17,-9.22328292945695E-37,
1.));
#118280=DIRECTION('',(0.,1.23467863058847E-16,-1.));
#118281=DIRECTION('',(-0.257447214431338,-0.966292363511968,-1.19306053212906E-16));
#118282=DIRECTION('center_axis',(0.260190353924911,-0.965557341499939,-1.19215301615779E-16));
#118283=DIRECTION('ref_axis',(-3.12701465369725E-33,1.23467863058847E-16,
-1.));
#118284=DIRECTION('',(0.965557341499939,0.260190353924911,3.21251469876339E-17));
#118285=DIRECTION('',(0.,1.23467863058847E-16,-1.));
#118286=DIRECTION('center_axis',(0.,0.,-1.));
#118287=DIRECTION('ref_axis',(0.,1.,0.));
#118288=DIRECTION('center_axis',(0.,0.,-1.));
#118289=DIRECTION('ref_axis',(0.,-1.,0.));
#118290=DIRECTION('center_axis',(-4.93476711729114E-30,-1.97232914692071E-43,
1.));
#118291=DIRECTION('ref_axis',(3.99680288865056E-14,-1.,0.));
#118292=DIRECTION('center_axis',(-0.966876318092686,-0.255245343760725,
-3.15145971498576E-17));
#118293=DIRECTION('ref_axis',(-0.255245343760725,0.966876318092686,-1.94208817023009E-34));
#118294=DIRECTION('',(0.255245343760725,-0.966876318092686,-1.1937815283711E-16));
#118295=DIRECTION('',(0.,1.23467863058847E-16,-1.));
#118296=DIRECTION('center_axis',(0.262389207151869,0.964962125666191,1.19141811588728E-16));
#118297=DIRECTION('ref_axis',(4.54065214350716E-16,-4.72048517437092E-33,
-1.));
#118298=DIRECTION('',(0.,1.23467863058847E-16,-1.));
#118299=DIRECTION('',(-0.964962125666191,0.262389207151869,3.23966346967465E-17));
#118300=DIRECTION('center_axis',(0.,0.,-1.));
#118301=DIRECTION('ref_axis',(0.,1.,0.));
#118302=DIRECTION('center_axis',(0.,0.,-1.));
#118303=DIRECTION('ref_axis',(0.,-1.,0.));
#118304=DIRECTION('center_axis',(0.,0.,1.));
#118305=DIRECTION('ref_axis',(0.,1.,0.));
#118306=DIRECTION('center_axis',(0.,0.,-1.));
#118307=DIRECTION('ref_axis',(0.,1.,0.));
#118308=DIRECTION('center_axis',(0.,0.,1.));
#118309=DIRECTION('ref_axis',(0.,1.,0.));
#118310=DIRECTION('',(0.,1.23467863058847E-16,-1.));
#118311=DIRECTION('center_axis',(0.,0.,1.));
#118312=DIRECTION('ref_axis',(0.,1.,0.));
#118313=DIRECTION('',(0.,1.23467863058847E-16,-1.));
#118314=DIRECTION('center_axis',(0.,0.,-1.));
#118315=DIRECTION('ref_axis',(0.,1.,0.));
#118316=DIRECTION('center_axis',(0.,0.,1.));
#118317=DIRECTION('ref_axis',(0.,1.,0.));
#118318=DIRECTION('',(0.,1.23467863058847E-16,-1.));
#118319=DIRECTION('center_axis',(0.,0.,1.));
#118320=DIRECTION('ref_axis',(0.,1.,0.));
#118321=DIRECTION('',(0.,1.23467863058847E-16,-1.));
#118322=DIRECTION('center_axis',(0.,0.,-1.));
#118323=DIRECTION('ref_axis',(0.,1.,0.));
#118324=DIRECTION('center_axis',(0.,0.,1.));
#118325=DIRECTION('ref_axis',(0.,1.,0.));
#118326=DIRECTION('',(0.,1.23467863058847E-16,-1.));
#118327=DIRECTION('center_axis',(0.,0.,1.));
#118328=DIRECTION('ref_axis',(0.,1.,0.));
#118329=DIRECTION('center_axis',(0.,0.,-1.));
#118330=DIRECTION('ref_axis',(0.,1.,0.));
#118331=DIRECTION('center_axis',(0.,0.,1.));
#118332=DIRECTION('ref_axis',(0.,1.,0.));
#118333=DIRECTION('',(0.,1.23467863058847E-16,-1.));
#118334=DIRECTION('center_axis',(0.,0.,1.));
#118335=DIRECTION('ref_axis',(0.,1.,0.));
#118336=DIRECTION('center_axis',(0.,1.21568833848598E-16,-1.));
#118337=DIRECTION('ref_axis',(0.,1.,1.21568833848598E-16));
#118338=DIRECTION('center_axis',(0.,-1.21568833848598E-16,1.));
#118339=DIRECTION('ref_axis',(0.,1.,1.21568833848598E-16));
#118340=DIRECTION('center_axis',(0.,-1.21568833848598E-16,1.));
#118341=DIRECTION('ref_axis',(0.,1.,1.21568833848598E-16));
#118342=DIRECTION('center_axis',(0.,0.,-1.));
#118343=DIRECTION('ref_axis',(0.,1.,0.));
#118344=DIRECTION('center_axis',(0.,0.,1.));
#118345=DIRECTION('ref_axis',(0.,1.,0.));
#118346=DIRECTION('',(0.,1.23467863058847E-16,-1.));
#118347=DIRECTION('center_axis',(0.,0.,1.));
#118348=DIRECTION('ref_axis',(0.,1.,0.));
#118349=DIRECTION('',(0.,1.23467863058847E-16,-1.));
#118350=DIRECTION('center_axis',(0.,0.,-1.));
#118351=DIRECTION('ref_axis',(0.,1.,0.));
#118352=DIRECTION('center_axis',(0.,0.,1.));
#118353=DIRECTION('ref_axis',(0.,1.,0.));
#118354=DIRECTION('center_axis',(0.,0.,1.));
#118355=DIRECTION('ref_axis',(0.,1.,0.));
#118356=DIRECTION('center_axis',(0.,0.,1.));
#118357=DIRECTION('ref_axis',(0.,1.,0.));
#118358=DIRECTION('center_axis',(9.45862666529894E-32,-7.24606518465966E-47,
1.));
#118359=DIRECTION('ref_axis',(-7.66080049574581E-16,-1.,2.91703841149741E-62));
#118360=DIRECTION('',(-0.000686915141868458,-0.0174388829355556,0.999847695156391));
#118361=DIRECTION('',(-0.0110444763156131,-0.0135131799871829,0.999847695156391));
#118362=DIRECTION('center_axis',(0.,0.,1.));
#118363=DIRECTION('ref_axis',(0.,1.,0.));
#118364=DIRECTION('',(-0.013481760241072,-0.011082807913809,0.999847695156391));
#118365=DIRECTION('center_axis',(4.38645965981435E-31,-1.5583835234929E-45,
1.));
#118366=DIRECTION('ref_axis',(-3.5527136788005E-15,-1.,1.24460305557223E-60));
#118367=DIRECTION('center_axis',(0.,0.,1.));
#118368=DIRECTION('ref_axis',(0.,1.,0.));
#118369=DIRECTION('center_axis',(1.89172533305981E-31,-2.89842607386392E-46,
1.));
#118370=DIRECTION('ref_axis',(-1.53216009914918E-15,-1.,7.38983064246011E-61));
#118371=DIRECTION('center_axis',(-0.49830877570858,-0.40695051295028,-0.765558387101415));
#118372=DIRECTION('ref_axis',(-0.616776838376874,-0.454175066156573,0.642892946705359));
#118373=DIRECTION('',(-0.0174387888650499,-0.000689299189283617,0.999847695156391));
#118374=DIRECTION('center_axis',(0.,0.,1.));
#118375=DIRECTION('ref_axis',(0.,1.,0.));
#118376=DIRECTION('center_axis',(-6.62103866570927E-31,-3.55057194048325E-45,
1.));
#118377=DIRECTION('ref_axis',(5.36256034702207E-15,-1.,-1.86690458335834E-60));
#118378=DIRECTION('',(-0.0174387888650499,0.000689299189283565,0.999847695156391));
#118379=DIRECTION('center_axis',(0.524694313011686,-0.428071664090414,0.735833220435214));
#118380=DIRECTION('ref_axis',(-0.586317116676987,0.444960261348595,0.676936189394668));
#118381=DIRECTION('',(-0.0134817602410721,0.0110828079138087,0.999847695156391));
#118382=DIRECTION('center_axis',(0.,0.,1.));
#118383=DIRECTION('ref_axis',(0.,1.,0.));
#118384=DIRECTION('',(-0.0109827961190146,0.0135633579861438,0.999847695156391));
#118385=DIRECTION('center_axis',(1.09661491495359E-30,-9.73989702183064E-45,
1.));
#118386=DIRECTION('ref_axis',(-8.88178419700126E-15,-1.,3.73380916671668E-60));
#118387=DIRECTION('center_axis',(0.,0.,1.));
#118388=DIRECTION('ref_axis',(0.,1.,0.));
#118389=DIRECTION('center_axis',(0.,0.,1.));
#118390=DIRECTION('ref_axis',(0.,-1.,0.));
#118391=DIRECTION('center_axis',(-0.424375096187792,0.528257078927607,-0.735425207820941));
#118392=DIRECTION('ref_axis',(-0.426055759035728,0.600170551540012,0.676957752933407));
#118393=DIRECTION('',(-0.003269361032546,0.0171434468206077,0.999847695156391));
#118394=DIRECTION('center_axis',(0.,-1.30002649721837E-16,1.));
#118395=DIRECTION('ref_axis',(0.,1.,1.30002649721837E-16));
#118396=DIRECTION('center_axis',(0.,-1.30002742469137E-16,1.));
#118397=DIRECTION('ref_axis',(0.,-1.,-1.30002742469137E-16));
#118398=DIRECTION('',(-0.0174387888650499,-0.000689299189283839,0.999847695156391));
#118399=DIRECTION('center_axis',(2.57572279529701E-31,-1.30052077910778E-16,
1.));
#118400=DIRECTION('ref_axis',(3.91196650355621E-14,-1.,-1.30052077910778E-16));
#118401=DIRECTION('',(-0.0174387888650499,0.000689299189283565,0.999847695156391));
#118402=DIRECTION('center_axis',(0.,0.,1.));
#118403=DIRECTION('ref_axis',(0.,1.,0.));
#118404=DIRECTION('center_axis',(2.14851878863042E-31,-3.73873238811768E-46,
1.));
#118405=DIRECTION('ref_axis',(-1.74014414391086E-15,-1.,-5.4451383681285E-61));
#118406=DIRECTION('center_axis',(-2.96506482541439E-31,-7.12056498031345E-46,
1.));
#118407=DIRECTION('ref_axis',(2.40148711734095E-15,-1.,1.0890276736257E-60));
#118408=DIRECTION('',(-0.013481760241072,0.0110828079138088,0.999847695156391));
#118409=DIRECTION('center_axis',(0.,0.,1.));
#118410=DIRECTION('ref_axis',(0.,1.,0.));
#118411=DIRECTION('center_axis',(0.,0.,1.));
#118412=DIRECTION('ref_axis',(0.,-1.,0.));
#118413=DIRECTION('center_axis',(0.,0.,1.));
#118414=DIRECTION('ref_axis',(0.,-1.,0.));
#118415=DIRECTION('',(-0.0109827961190146,0.0135633579861438,0.999847695156391));
#118416=DIRECTION('center_axis',(0.,0.,1.));
#118417=DIRECTION('ref_axis',(0.,1.,0.));
#118418=DIRECTION('center_axis',(-3.58086464771735E-31,-1.03853677447713E-45,
1.));
#118419=DIRECTION('ref_axis',(2.90024023985143E-15,-1.,1.55575381946529E-61));
#118420=DIRECTION('center_axis',(0.,0.,1.));
#118421=DIRECTION('ref_axis',(0.,-1.,0.));
#118422=DIRECTION('',(-0.0032693610325459,0.0171434468206077,0.999847695156391));
#118423=DIRECTION('center_axis',(0.,0.,1.));
#118424=DIRECTION('ref_axis',(0.,1.,0.));
#118425=DIRECTION('center_axis',(-2.14851878863041E-31,-3.73873238811767E-46,
1.));
#118426=DIRECTION('ref_axis',(1.74014414391086E-15,-1.,-6.22301527786114E-61));
#118427=DIRECTION('',(-0.000686915141868465,-0.0174388829355556,0.999847695156391));
#118428=DIRECTION('center_axis',(9.63646068259673E-31,-7.52109676045604E-45,
1.));
#118429=DIRECTION('ref_axis',(-7.80483313135807E-15,-1.,-3.73380916671668E-60));
#118430=DIRECTION('',(-0.0110444763156131,-0.0135131799871829,0.999847695156391));
#118431=DIRECTION('center_axis',(0.,0.,1.));
#118432=DIRECTION('ref_axis',(0.,1.,0.));
#118433=DIRECTION('center_axis',(1.09661491495359E-30,-9.73989702183063E-45,
1.));
#118434=DIRECTION('ref_axis',(-8.88178419700125E-15,-1.,2.48920611114446E-60));
#118435=DIRECTION('center_axis',(7.6763044046751E-31,-4.77254954069701E-45,
1.));
#118436=DIRECTION('ref_axis',(-6.21724893790088E-15,-1.,1.86690458335834E-60));
#118437=DIRECTION('',(-0.013481760241072,-0.011082807913809,0.999847695156391));
#118438=DIRECTION('center_axis',(0.,0.,1.));
#118439=DIRECTION('ref_axis',(0.,-1.,0.));
#118440=DIRECTION('center_axis',(-2.14851878863042E-31,-3.73873238811769E-46,
1.));
#118441=DIRECTION('ref_axis',(1.74014414391087E-15,-1.,2.33363072919793E-61));
#118442=DIRECTION('center_axis',(2.22379861906079E-31,-4.00531780142632E-46,
1.));
#118443=DIRECTION('ref_axis',(-1.80111533800572E-15,-1.,8.55664600705907E-61));
#118444=DIRECTION('center_axis',(0.,-1.30362731016209E-16,1.));
#118445=DIRECTION('ref_axis',(0.,1.,1.30362731016209E-16));
#118446=DIRECTION('center_axis',(0.,-1.30357480714758E-16,1.));
#118447=DIRECTION('ref_axis',(0.,-1.,-1.30357480714758E-16));
#118448=DIRECTION('center_axis',(9.64693417405135E-8,-8.44902797496882E-7,
0.999999999999638));
#118449=DIRECTION('ref_axis',(-0.131285471389456,0.9913446045656,8.50254852648554E-7));
#118450=DIRECTION('center_axis',(0.,1.23467863058847E-16,-1.));
#118451=DIRECTION('ref_axis',(-1.,0.,0.));
#118452=DIRECTION('center_axis',(0.,-1.21568833848598E-16,1.));
#118453=DIRECTION('ref_axis',(0.,1.,1.21568833848598E-16));
#118454=DIRECTION('center_axis',(2.34983671542145E-7,7.16718722586561E-6,
0.999999999974288));
#118455=DIRECTION('ref_axis',(-0.0297033272165618,-0.999558758803525,7.17100456465166E-6));
#118456=DIRECTION('center_axis',(0.,-1.21568833848598E-16,1.));
#118457=DIRECTION('ref_axis',(0.,1.,1.21568833848598E-16));
#118458=DIRECTION('center_axis',(0.,1.23467863058847E-16,-1.));
#118459=DIRECTION('ref_axis',(-1.,0.,0.));
#118460=DIRECTION('center_axis',(0.,0.,1.));
#118461=DIRECTION('ref_axis',(0.,1.,0.));
#118462=DIRECTION('center_axis',(0.,-1.23467863058847E-16,1.));
#118463=DIRECTION('ref_axis',(0.,-1.,-1.23467863058847E-16));
#118464=DIRECTION('center_axis',(0.,0.,1.));
#118465=DIRECTION('ref_axis',(0.,1.,0.));
#118466=DIRECTION('center_axis',(0.,1.23467863058847E-16,-1.));
#118467=DIRECTION('ref_axis',(-1.,0.,0.));
#118468=DIRECTION('center_axis',(0.,-1.30925187718918E-16,1.));
#118469=DIRECTION('ref_axis',(0.,1.,1.30925187718918E-16));
#118470=DIRECTION('center_axis',(0.,1.23467863058847E-16,-1.));
#118471=DIRECTION('ref_axis',(-1.,0.,0.));
#118472=DIRECTION('center_axis',(0.,-1.30925187718918E-16,1.));
#118473=DIRECTION('ref_axis',(0.,1.,1.30925187718918E-16));
#118474=DIRECTION('center_axis',(0.,1.23467863058847E-16,-1.));
#118475=DIRECTION('ref_axis',(-1.,0.,0.));
#118476=DIRECTION('center_axis',(0.,-1.21568833848598E-16,1.));
#118477=DIRECTION('ref_axis',(0.,1.,1.21568833848598E-16));
#118478=DIRECTION('center_axis',(0.,1.23467863058847E-16,-1.));
#118479=DIRECTION('ref_axis',(-1.,0.,0.));
#118480=DIRECTION('center_axis',(0.,-1.21568833848598E-16,1.));
#118481=DIRECTION('ref_axis',(0.,1.,1.21568833848598E-16));
#118482=DIRECTION('center_axis',(0.,1.23467863058847E-16,-1.));
#118483=DIRECTION('ref_axis',(-1.,0.,0.));
#118484=DIRECTION('center_axis',(0.,-1.21568833848598E-16,1.));
#118485=DIRECTION('ref_axis',(0.,1.,1.21568833848598E-16));
#118486=DIRECTION('center_axis',(0.,1.23467863058847E-16,-1.));
#118487=DIRECTION('ref_axis',(-1.,0.,0.));
#118488=DIRECTION('center_axis',(0.,-1.21568833848598E-16,1.));
#118489=DIRECTION('ref_axis',(0.,1.,1.21568833848598E-16));
#118490=DIRECTION('center_axis',(0.,1.23467863058847E-16,-1.));
#118491=DIRECTION('ref_axis',(-1.,0.,0.));
#118492=DIRECTION('center_axis',(7.1617481931302E-31,4.1541690210802E-45,
-1.));
#118493=DIRECTION('ref_axis',(-5.80049578546342E-15,1.,-2.48920611114446E-60));
#118494=DIRECTION('',(0.7059219377897,-0.708289642552561,-8.74510085926797E-17));
#118495=DIRECTION('center_axis',(0.,1.21568833848598E-16,-1.));
#118496=DIRECTION('ref_axis',(0.,1.,1.21568833848598E-16));
#118497=DIRECTION('center_axis',(0.,-1.21568833848598E-16,1.));
#118498=DIRECTION('ref_axis',(0.,1.,1.21568833848598E-16));
#118499=DIRECTION('center_axis',(0.,1.21568833848598E-16,-1.));
#118500=DIRECTION('ref_axis',(0.,1.,1.21568833848598E-16));
#118501=DIRECTION('center_axis',(0.,-1.21568833848598E-16,1.));
#118502=DIRECTION('ref_axis',(0.,1.,1.21568833848598E-16));
#118503=DIRECTION('center_axis',(0.,1.21568833848598E-16,-1.));
#118504=DIRECTION('ref_axis',(0.,1.,1.21568833848598E-16));
#118505=DIRECTION('center_axis',(0.,-1.21568833848598E-16,1.));
#118506=DIRECTION('ref_axis',(0.,1.,1.21568833848598E-16));
#118507=DIRECTION('center_axis',(0.,1.21568833848598E-16,-1.));
#118508=DIRECTION('ref_axis',(0.,1.,1.21568833848598E-16));
#118509=DIRECTION('center_axis',(0.,-1.21568833848598E-16,1.));
#118510=DIRECTION('ref_axis',(0.,1.,1.21568833848598E-16));
#118511=DIRECTION('center_axis',(0.,1.21568833848598E-16,-1.));
#118512=DIRECTION('ref_axis',(0.,1.,1.21568833848598E-16));
#118513=DIRECTION('center_axis',(0.,-1.21568833848598E-16,1.));
#118514=DIRECTION('ref_axis',(0.,1.,1.21568833848598E-16));
#118515=DIRECTION('center_axis',(-0.713783141330105,0.700366780446451,8.64727897391283E-17));
#118516=DIRECTION('ref_axis',(1.21147145025014E-16,-2.46367577887085E-33,
1.));
#118517=DIRECTION('',(-0.0133579710326364,-0.0136138588975274,0.999818097183587));
#118518=DIRECTION('center_axis',(0.,0.,-1.));
#118519=DIRECTION('ref_axis',(0.705510697508504,-0.708699270283993,0.));
#118520=DIRECTION('',(-0.0134623247494151,0.0135074781986352,0.999818140386068));
#118521=DIRECTION('center_axis',(0.708289642552561,0.7059219377897,8.71586731452549E-17));
#118522=DIRECTION('ref_axis',(-2.22539097861278E-34,1.23467863058847E-16,
-1.));
#118523=DIRECTION('center_axis',(0.,0.,-1.));
#118524=DIRECTION('ref_axis',(0.,1.,0.));
#118525=DIRECTION('center_axis',(0.,0.,-1.));
#118526=DIRECTION('ref_axis',(0.,1.,0.));
#118527=DIRECTION('',(0.,1.23467863058847E-16,-1.));
#118528=DIRECTION('center_axis',(0.,0.,1.));
#118529=DIRECTION('ref_axis',(0.,1.,0.));
#118530=DIRECTION('',(0.,1.23467863058847E-16,-1.));
#118531=DIRECTION('center_axis',(0.,0.,-1.));
#118532=DIRECTION('ref_axis',(0.,1.,0.));
#118533=DIRECTION('center_axis',(0.,0.,1.));
#118534=DIRECTION('ref_axis',(0.,1.,0.));
#118535=DIRECTION('',(0.,1.23467863058847E-16,-1.));
#118536=DIRECTION('center_axis',(0.,0.,-1.));
#118537=DIRECTION('ref_axis',(0.,1.,0.));
#118538=DIRECTION('center_axis',(0.,0.,1.));
#118539=DIRECTION('ref_axis',(0.,1.,0.));
#118540=DIRECTION('',(0.,1.23467863058847E-16,-1.));
#118541=DIRECTION('center_axis',(0.,1.22914743790472E-16,-1.));
#118542=DIRECTION('ref_axis',(0.,1.,1.22914743790472E-16));
#118543=DIRECTION('center_axis',(0.,-1.22914743790472E-16,1.));
#118544=DIRECTION('ref_axis',(0.,1.,1.22914743790472E-16));
#118545=DIRECTION('center_axis',(0.,0.,-1.));
#118546=DIRECTION('ref_axis',(0.,1.,0.));
#118547=DIRECTION('',(0.,1.23467863058847E-16,-1.));
#118548=DIRECTION('center_axis',(0.,0.,1.));
#118549=DIRECTION('ref_axis',(0.,1.,0.));
#118550=DIRECTION('',(0.,1.23467863058847E-16,-1.));
#118551=DIRECTION('center_axis',(0.,0.,-1.));
#118552=DIRECTION('ref_axis',(0.,1.,0.));
#118553=DIRECTION('center_axis',(0.,0.,1.));
#118554=DIRECTION('ref_axis',(0.,1.,0.));
#118555=DIRECTION('center_axis',(0.,0.,-1.));
#118556=DIRECTION('ref_axis',(0.,1.,0.));
#118557=DIRECTION('',(0.,1.23467863058847E-16,-1.));
#118558=DIRECTION('center_axis',(0.,0.,1.));
#118559=DIRECTION('ref_axis',(0.,1.,0.));
#118560=DIRECTION('',(0.,1.23467863058847E-16,-1.));
#118561=DIRECTION('center_axis',(0.,1.23467863058847E-16,-1.));
#118562=DIRECTION('ref_axis',(-1.,0.,0.));
#118563=DIRECTION('center_axis',(0.,0.,1.));
#118564=DIRECTION('ref_axis',(0.,1.,0.));
#118565=DIRECTION('center_axis',(0.,0.,-1.));
#118566=DIRECTION('ref_axis',(0.,1.,0.));
#118567=DIRECTION('',(-2.13730336808358E-18,-0.0174524064372818,-0.999847695156391));
#118568=DIRECTION('center_axis',(0.,0.,1.));
#118569=DIRECTION('ref_axis',(0.,-1.,0.));
#118570=DIRECTION('center_axis',(0.,0.,1.));
#118571=DIRECTION('ref_axis',(0.,-1.,0.));
#118572=DIRECTION('center_axis',(0.,1.23467863058847E-16,-1.));
#118573=DIRECTION('ref_axis',(-1.,0.,0.));
#118574=DIRECTION('center_axis',(0.,0.,1.));
#118575=DIRECTION('ref_axis',(0.,1.,0.));
#118576=DIRECTION('center_axis',(0.,0.,-1.));
#118577=DIRECTION('ref_axis',(0.,1.,0.));
#118578=DIRECTION('',(-2.13730336808358E-18,-0.0174524064372818,-0.999847695156391));
#118579=DIRECTION('center_axis',(0.,-1.23467863058847E-16,1.));
#118580=DIRECTION('ref_axis',(0.,-1.,-1.23467863058847E-16));
#118581=DIRECTION('center_axis',(0.713783141330072,-0.700366780446485,-8.64727897391324E-17));
#118582=DIRECTION('ref_axis',(-4.34651812646493E-33,1.23467863058847E-16,
-1.));
#118583=DIRECTION('center_axis',(-0.713783141330105,0.700366780446451,8.64727897391283E-17));
#118584=DIRECTION('ref_axis',(1.21147145025014E-16,-2.46367577887085E-33,
1.));
#118585=DIRECTION('center_axis',(0.,0.,1.));
#118586=DIRECTION('ref_axis',(0.,-1.,0.));
#118587=DIRECTION('center_axis',(0.,1.23467863058847E-16,-1.));
#118588=DIRECTION('ref_axis',(-1.,0.,0.));
#118589=DIRECTION('center_axis',(0.,0.,-1.));
#118590=DIRECTION('ref_axis',(0.,1.,0.));
#118591=DIRECTION('center_axis',(-0.708289642552581,-0.70592193778968,-8.71586731452524E-17));
#118592=DIRECTION('ref_axis',(-0.70592193778968,0.708289642552581,-2.39349531189888E-34));
#118593=DIRECTION('center_axis',(0.708289642552561,0.7059219377897,8.71586731452549E-17));
#118594=DIRECTION('ref_axis',(-2.22539097861278E-34,1.23467863058847E-16,
-1.));
#118595=DIRECTION('center_axis',(0.,0.,1.));
#118596=DIRECTION('ref_axis',(0.,-1.,0.));
#118597=DIRECTION('center_axis',(-0.966292363511968,0.257447214431338,3.17864574162902E-17));
#118598=DIRECTION('ref_axis',(3.28952795412384E-17,-9.22328292945695E-37,
1.));
#118599=DIRECTION('center_axis',(0.260190353924911,-0.965557341499939,-1.19215301615779E-16));
#118600=DIRECTION('ref_axis',(-3.12701465369725E-33,1.23467863058847E-16,
-1.));
#118601=DIRECTION('center_axis',(0.,0.,-1.));
#118602=DIRECTION('ref_axis',(0.,1.,0.));
#118603=DIRECTION('center_axis',(-0.966876318092686,-0.255245343760725,
-3.15145971498576E-17));
#118604=DIRECTION('ref_axis',(-0.255245343760725,0.966876318092686,-1.94208817023009E-34));
#118605=DIRECTION('center_axis',(0.262389207151869,0.964962125666191,1.19141811588728E-16));
#118606=DIRECTION('ref_axis',(4.54065214350716E-16,-4.72048517437092E-33,
-1.));
#118607=DIRECTION('center_axis',(0.,0.,-1.));
#118608=DIRECTION('ref_axis',(0.,1.,0.));
#118609=DIRECTION('center_axis',(0.,0.,-1.));
#118610=DIRECTION('ref_axis',(0.,1.,0.));
#118611=DIRECTION('',(0.,1.23467863058847E-16,-1.));
#118612=DIRECTION('center_axis',(0.,0.,1.));
#118613=DIRECTION('ref_axis',(0.,1.,0.));
#118614=DIRECTION('',(0.,1.23467863058847E-16,-1.));
#118615=DIRECTION('center_axis',(0.,0.,-1.));
#118616=DIRECTION('ref_axis',(0.,1.,0.));
#118617=DIRECTION('',(0.,1.23467863058847E-16,-1.));
#118618=DIRECTION('center_axis',(0.,0.,1.));
#118619=DIRECTION('ref_axis',(0.,1.,0.));
#118620=DIRECTION('center_axis',(0.,1.22229112323298E-16,-1.));
#118621=DIRECTION('ref_axis',(0.,1.,1.22229112323298E-16));
#118622=DIRECTION('',(0.,1.23467863058847E-16,-1.));
#118623=DIRECTION('center_axis',(0.,-1.22229112323298E-16,1.));
#118624=DIRECTION('ref_axis',(0.,1.,1.22229112323298E-16));
#118625=DIRECTION('center_axis',(0.,0.,-1.));
#118626=DIRECTION('ref_axis',(0.,1.,0.));
#118627=DIRECTION('',(0.,1.23467863058847E-16,-1.));
#118628=DIRECTION('center_axis',(0.,0.,1.));
#118629=DIRECTION('ref_axis',(0.,1.,0.));
#118630=DIRECTION('center_axis',(0.,0.,-1.));
#118631=DIRECTION('ref_axis',(0.,1.,0.));
#118632=DIRECTION('',(0.,1.23467863058847E-16,-1.));
#118633=DIRECTION('center_axis',(0.,0.,1.));
#118634=DIRECTION('ref_axis',(0.,1.,0.));
#118635=DIRECTION('center_axis',(0.,0.,-1.));
#118636=DIRECTION('ref_axis',(0.,1.,0.));
#118637=DIRECTION('',(0.,1.23467863058847E-16,-1.));
#118638=DIRECTION('center_axis',(0.,0.,1.));
#118639=DIRECTION('ref_axis',(0.,1.,0.));
#118640=DIRECTION('center_axis',(0.,0.,-1.));
#118641=DIRECTION('ref_axis',(0.,1.,0.));
#118642=DIRECTION('center_axis',(0.,0.,1.));
#118643=DIRECTION('ref_axis',(0.,1.,0.));
#118644=DIRECTION('',(0.,1.23467863058847E-16,-1.));
#118645=DIRECTION('center_axis',(0.,0.,-1.));
#118646=DIRECTION('ref_axis',(0.,1.,0.));
#118647=DIRECTION('',(0.,1.23467863058847E-16,-1.));
#118648=DIRECTION('center_axis',(0.,0.,1.));
#118649=DIRECTION('ref_axis',(0.,1.,0.));
#118650=DIRECTION('',(0.,1.23467863058847E-16,-1.));
#118651=DIRECTION('center_axis',(0.,0.,-1.));
#118652=DIRECTION('ref_axis',(0.,1.,0.));
#118653=DIRECTION('',(0.,1.23467863058847E-16,-1.));
#118654=DIRECTION('center_axis',(0.,0.,1.));
#118655=DIRECTION('ref_axis',(0.,1.,0.));
#118656=DIRECTION('',(0.,1.23467863058847E-16,-1.));
#118657=DIRECTION('center_axis',(0.,0.,-1.));
#118658=DIRECTION('ref_axis',(0.,1.,0.));
#118659=DIRECTION('center_axis',(0.,0.,1.));
#118660=DIRECTION('ref_axis',(0.,1.,0.));
#118661=DIRECTION('',(0.,1.23467863058847E-16,-1.));
#118662=DIRECTION('center_axis',(0.,0.,-1.));
#118663=DIRECTION('ref_axis',(0.,1.,0.));
#118664=DIRECTION('center_axis',(0.,0.,1.));
#118665=DIRECTION('ref_axis',(0.,1.,0.));
#118666=DIRECTION('',(0.,1.23467863058847E-16,-1.));
#118667=DIRECTION('center_axis',(0.,1.22014183466588E-16,-1.));
#118668=DIRECTION('ref_axis',(0.,1.,1.22014183466588E-16));
#118669=DIRECTION('center_axis',(0.,-1.22014183466588E-16,1.));
#118670=DIRECTION('ref_axis',(0.,1.,1.22014183466588E-16));
#118671=DIRECTION('',(0.,1.23467863058847E-16,-1.));
#118672=DIRECTION('center_axis',(0.,0.,-1.));
#118673=DIRECTION('ref_axis',(0.,1.,0.));
#118674=DIRECTION('center_axis',(0.,0.,1.));
#118675=DIRECTION('ref_axis',(0.,1.,0.));
#118676=DIRECTION('',(0.,1.23467863058847E-16,-1.));
#118677=DIRECTION('center_axis',(0.,0.,-1.));
#118678=DIRECTION('ref_axis',(0.,1.,0.));
#118679=DIRECTION('center_axis',(0.,0.,1.));
#118680=DIRECTION('ref_axis',(0.,1.,0.));
#118681=DIRECTION('',(-0.459549353210719,-0.545727376107149,0.700711083779054));
#118682=DIRECTION('',(-0.595667475496749,-0.42912133257888,0.678995685230073));
#118683=DIRECTION('',(-0.580626046021037,0.392567954055243,0.713276801901518));
#118684=DIRECTION('',(0.484796374610729,-0.46748816331627,-0.739207205270264));
#118685=DIRECTION('center_axis',(0.,0.,1.));
#118686=DIRECTION('ref_axis',(0.,1.,0.));
#118687=DIRECTION('',(-0.0110444763156131,-0.0135131799871829,0.999847695156391));
#118688=DIRECTION('',(-0.000686915141868466,-0.0174388829355556,0.999847695156391));
#118689=DIRECTION('center_axis',(0.,0.,1.));
#118690=DIRECTION('ref_axis',(0.,1.,0.));
#118691=DIRECTION('',(-0.013481760241072,-0.011082807913809,0.999847695156391));
#118692=DIRECTION('center_axis',(0.,0.,1.));
#118693=DIRECTION('ref_axis',(0.,1.,0.));
#118694=DIRECTION('',(-0.0174387888650499,-0.000689299189283616,0.999847695156391));
#118695=DIRECTION('center_axis',(0.,0.,1.));
#118696=DIRECTION('ref_axis',(0.,1.,0.));
#118697=DIRECTION('',(-0.0134817602410721,0.0110828079138087,0.999847695156391));
#118698=DIRECTION('',(-0.0174387888650499,0.000689299189283565,0.999847695156391));
#118699=DIRECTION('center_axis',(0.,0.,1.));
#118700=DIRECTION('ref_axis',(0.,1.,0.));
#118701=DIRECTION('',(-0.0109827961190146,0.0135633579861438,0.999847695156391));
#118702=DIRECTION('center_axis',(0.,0.,1.));
#118703=DIRECTION('ref_axis',(0.,1.,0.));
#118704=DIRECTION('',(-0.00326936103254579,0.0171434468206077,0.999847695156391));
#118705=DIRECTION('center_axis',(0.,-1.29698951474901E-16,1.));
#118706=DIRECTION('ref_axis',(0.,1.,1.29698951474901E-16));
#118707=DIRECTION('',(-0.0174387888650499,-0.000689299189283839,0.999847695156391));
#118708=DIRECTION('center_axis',(0.,-1.29698951474901E-16,1.));
#118709=DIRECTION('ref_axis',(0.,1.,1.29698951474901E-16));
#118710=DIRECTION('',(-0.0174387888650499,0.000689299189283565,0.999847695156391));
#118711=DIRECTION('center_axis',(0.,0.,1.));
#118712=DIRECTION('ref_axis',(0.,1.,0.));
#118713=DIRECTION('center_axis',(0.,0.,1.));
#118714=DIRECTION('ref_axis',(0.,1.,0.));
#118715=DIRECTION('',(-0.0134817602410721,0.0110828079138088,0.999847695156391));
#118716=DIRECTION('center_axis',(0.,0.,1.));
#118717=DIRECTION('ref_axis',(0.,1.,0.));
#118718=DIRECTION('center_axis',(0.,0.,1.));
#118719=DIRECTION('ref_axis',(0.,1.,0.));
#118720=DIRECTION('',(-0.0109827961190146,0.0135633579861438,0.999847695156391));
#118721=DIRECTION('center_axis',(0.,0.,1.));
#118722=DIRECTION('ref_axis',(0.,1.,0.));
#118723=DIRECTION('center_axis',(0.,0.,1.));
#118724=DIRECTION('ref_axis',(0.,1.,0.));
#118725=DIRECTION('',(-0.0032693610325459,0.0171434468206077,0.999847695156391));
#118726=DIRECTION('center_axis',(0.,0.,1.));
#118727=DIRECTION('ref_axis',(0.,1.,0.));
#118728=DIRECTION('',(-0.000686915141868473,-0.0174388829355556,0.999847695156391));
#118729=DIRECTION('center_axis',(0.,0.,1.));
#118730=DIRECTION('ref_axis',(0.,1.,0.));
#118731=DIRECTION('',(-0.0110444763156131,-0.0135131799871829,0.999847695156391));
#118732=DIRECTION('center_axis',(0.,0.,1.));
#118733=DIRECTION('ref_axis',(0.,1.,0.));
#118734=DIRECTION('center_axis',(0.,0.,1.));
#118735=DIRECTION('ref_axis',(0.,1.,0.));
#118736=DIRECTION('',(-0.013481760241072,-0.011082807913809,0.999847695156391));
#118737=DIRECTION('center_axis',(0.,0.,1.));
#118738=DIRECTION('ref_axis',(0.,-1.,0.));
#118739=DIRECTION('center_axis',(0.,0.,1.));
#118740=DIRECTION('ref_axis',(0.,-1.,0.));
#118741=DIRECTION('center_axis',(0.,-1.30057350048735E-16,1.));
#118742=DIRECTION('ref_axis',(0.,1.,1.30057350048735E-16));
#118743=DIRECTION('center_axis',(0.,1.23467863058847E-16,-1.));
#118744=DIRECTION('ref_axis',(-1.,0.,0.));
#118745=DIRECTION('center_axis',(0.,-1.23467863058847E-16,1.));
#118746=DIRECTION('ref_axis',(0.,-1.,-1.23467863058847E-16));
#118747=DIRECTION('center_axis',(0.,1.22914743790472E-16,-1.));
#118748=DIRECTION('ref_axis',(0.,1.,1.22914743790472E-16));
#118749=DIRECTION('center_axis',(0.,-1.22914743790472E-16,1.));
#118750=DIRECTION('ref_axis',(0.,1.,1.22914743790472E-16));
#118751=DIRECTION('center_axis',(0.,1.22914743790472E-16,-1.));
#118752=DIRECTION('ref_axis',(0.,1.,1.22914743790472E-16));
#118753=DIRECTION('center_axis',(0.,-1.22914743790472E-16,1.));
#118754=DIRECTION('ref_axis',(0.,1.,1.22914743790472E-16));
#118755=DIRECTION('center_axis',(0.,1.22914743790472E-16,-1.));
#118756=DIRECTION('ref_axis',(0.,1.,1.22914743790472E-16));
#118757=DIRECTION('center_axis',(0.,-1.22914743790472E-16,1.));
#118758=DIRECTION('ref_axis',(0.,1.,1.22914743790472E-16));
#118759=DIRECTION('center_axis',(0.,1.22914743790472E-16,-1.));
#118760=DIRECTION('ref_axis',(0.,1.,1.22914743790472E-16));
#118761=DIRECTION('center_axis',(0.,-1.22914743790472E-16,1.));
#118762=DIRECTION('ref_axis',(0.,1.,1.22914743790472E-16));
#118763=DIRECTION('center_axis',(0.,1.22914743790472E-16,-1.));
#118764=DIRECTION('ref_axis',(0.,1.,1.22914743790472E-16));
#118765=DIRECTION('center_axis',(0.,-1.22914743790472E-16,1.));
#118766=DIRECTION('ref_axis',(0.,1.,1.22914743790472E-16));
#118767=DIRECTION('center_axis',(3.29883322342201E-16,1.,1.23467863058847E-16));
#118768=DIRECTION('ref_axis',(1.,-3.29883322342202E-16,0.));
#118769=DIRECTION('',(-1.,3.29883322342202E-16,0.));
#118770=DIRECTION('center_axis',(3.29883322342201E-16,-1.,-1.23467863058847E-16));
#118771=DIRECTION('ref_axis',(1.07891492167253E-48,1.23467863058847E-16,
-1.));
#118772=DIRECTION('',(1.,3.29883322342202E-16,0.));
#118773=DIRECTION('center_axis',(3.71118737634973E-16,1.,1.23467863058847E-16));
#118774=DIRECTION('ref_axis',(1.,-3.71118737634973E-16,0.));
#118775=DIRECTION('',(-1.,3.71118737634973E-16,0.));
#118776=DIRECTION('center_axis',(3.71118737634973E-16,-1.,-1.23467863058847E-16));
#118777=DIRECTION('ref_axis',(9.86109193995912E-49,1.23467863058847E-16,
-1.));
#118778=DIRECTION('',(1.,3.71118737634973E-16,0.));
#118779=DIRECTION('center_axis',(5.72252063890675E-16,1.,1.23467863058847E-16));
#118780=DIRECTION('ref_axis',(1.,-5.72252063890675E-16,0.));
#118781=DIRECTION('',(-1.,5.72252063890675E-16,0.));
#118782=DIRECTION('center_axis',(-1.90750687963558E-16,-1.,-1.23467863058847E-16));
#118783=DIRECTION('ref_axis',(-1.,1.90750687963558E-16,0.));
#118784=DIRECTION('',(1.,-1.90750687963558E-16,0.));
#118785=DIRECTION('center_axis',(-1.23706245878324E-16,-1.,-1.23467863058847E-16));
#118786=DIRECTION('ref_axis',(-1.,1.23706245878324E-16,0.));
#118787=DIRECTION('',(1.,-1.23706245878324E-16,0.));
#118788=DIRECTION('center_axis',(-1.23706245878324E-16,1.,1.23467863058847E-16));
#118789=DIRECTION('ref_axis',(1.,1.23706245878324E-16,0.));
#118790=DIRECTION('',(-1.,-1.23706245878324E-16,0.));
#118791=DIRECTION('center_axis',(4.76876719908896E-16,-1.,-1.23467863058847E-16));
#118792=DIRECTION('ref_axis',(8.72767235901404E-49,1.23467863058847E-16,
-1.));
#118793=DIRECTION('',(1.,4.76876719908896E-16,0.));
#118794=DIRECTION('center_axis',(-9.53753439817791E-17,1.,1.23467863058847E-16));
#118795=DIRECTION('ref_axis',(4.60419424770999E-49,1.23467863058847E-16,
-1.));
#118796=DIRECTION('',(-1.,-9.53753439817791E-17,0.));
#118797=DIRECTION('center_axis',(0.,1.35726946151947E-16,-1.));
#118798=DIRECTION('ref_axis',(0.,1.,1.35726946151947E-16));
#118799=DIRECTION('center_axis',(0.,-1.35726946151947E-16,1.));
#118800=DIRECTION('ref_axis',(0.,1.,1.35726946151947E-16));
#118801=DIRECTION('center_axis',(0.,1.22914743790472E-16,-1.));
#118802=DIRECTION('ref_axis',(0.,1.,1.22914743790472E-16));
#118803=DIRECTION('center_axis',(0.,-1.22914743790472E-16,1.));
#118804=DIRECTION('ref_axis',(0.,1.,1.22914743790472E-16));
#118805=DIRECTION('center_axis',(0.,1.34087697701688E-16,-1.));
#118806=DIRECTION('ref_axis',(0.,1.,1.34087697701688E-16));
#118807=DIRECTION('center_axis',(1.86759697420978E-30,1.34087697701688E-16,
-1.));
#118808=DIRECTION('ref_axis',(1.75859327100625E-13,1.,1.34087697701688E-16));
#118809=DIRECTION('center_axis',(0.,-1.34087697701688E-16,1.));
#118810=DIRECTION('ref_axis',(0.,1.,1.34087697701688E-16));
#118811=DIRECTION('center_axis',(3.29883322342201E-16,1.,1.23467863058847E-16));
#118812=DIRECTION('ref_axis',(1.,-3.29883322342202E-16,0.));
#118813=DIRECTION('',(-1.,3.29883322342202E-16,0.));
#118814=DIRECTION('center_axis',(3.29883322342201E-16,-1.,-1.23467863058847E-16));
#118815=DIRECTION('ref_axis',(1.07891492167253E-48,1.23467863058847E-16,
-1.));
#118816=DIRECTION('',(1.,3.29883322342202E-16,0.));
#118817=DIRECTION('center_axis',(3.29883322342198E-16,1.,1.23467863058847E-16));
#118818=DIRECTION('ref_axis',(1.,-3.29883322342198E-16,0.));
#118819=DIRECTION('',(-1.,3.29883322342198E-16,0.));
#118820=DIRECTION('center_axis',(3.29883322342198E-16,-1.,-1.23467863058847E-16));
#118821=DIRECTION('ref_axis',(8.54897290170095E-49,1.23467863058847E-16,
-1.));
#118822=DIRECTION('',(1.,3.29883322342198E-16,0.));
#118823=DIRECTION('center_axis',(3.71118737634973E-16,1.,1.23467863058847E-16));
#118824=DIRECTION('ref_axis',(1.,-3.71118737634973E-16,0.));
#118825=DIRECTION('',(-1.,3.71118737634973E-16,0.));
#118826=DIRECTION('center_axis',(3.71118737634973E-16,-1.,-1.23467863058847E-16));
#118827=DIRECTION('ref_axis',(9.86109193995912E-49,1.23467863058847E-16,
-1.));
#118828=DIRECTION('',(1.,3.71118737634973E-16,0.));
#118829=DIRECTION('center_axis',(3.71118737634973E-16,1.,1.23467863058847E-16));
#118830=DIRECTION('ref_axis',(1.,-3.71118737634973E-16,0.));
#118831=DIRECTION('',(-1.,3.71118737634973E-16,0.));
#118832=DIRECTION('center_axis',(3.71118737634973E-16,-1.,-1.23467863058847E-16));
#118833=DIRECTION('ref_axis',(9.86109193995912E-49,1.23467863058847E-16,
-1.));
#118834=DIRECTION('',(1.,3.71118737634973E-16,0.));
#118835=DIRECTION('center_axis',(5.72252063890675E-16,1.,1.23467863058847E-16));
#118836=DIRECTION('ref_axis',(1.,-5.72252063890675E-16,0.));
#118837=DIRECTION('',(-1.,5.72252063890675E-16,0.));
#118838=DIRECTION('center_axis',(-1.90750687963558E-16,-1.,-1.23467863058847E-16));
#118839=DIRECTION('ref_axis',(-1.,1.90750687963558E-16,0.));
#118840=DIRECTION('',(1.,-1.90750687963558E-16,0.));
#118841=DIRECTION('center_axis',(-1.23706245878324E-16,-1.,-1.23467863058847E-16));
#118842=DIRECTION('ref_axis',(-1.,1.23706245878324E-16,0.));
#118843=DIRECTION('',(1.,-1.23706245878324E-16,0.));
#118844=DIRECTION('center_axis',(-1.23706245878324E-16,1.,1.23467863058847E-16));
#118845=DIRECTION('ref_axis',(1.,1.23706245878324E-16,0.));
#118846=DIRECTION('',(-1.,-1.23706245878324E-16,0.));
#118847=DIRECTION('center_axis',(4.76876719908896E-16,-1.,-1.23467863058847E-16));
#118848=DIRECTION('ref_axis',(8.72767235901404E-49,1.23467863058847E-16,
-1.));
#118849=DIRECTION('',(1.,4.76876719908896E-16,0.));
#118850=DIRECTION('center_axis',(-9.53753439817791E-17,1.,1.23467863058847E-16));
#118851=DIRECTION('ref_axis',(4.60419424770999E-49,1.23467863058847E-16,
-1.));
#118852=DIRECTION('',(-1.,-9.53753439817791E-17,0.));
#118853=DIRECTION('center_axis',(0.,1.35726946151947E-16,-1.));
#118854=DIRECTION('ref_axis',(0.,1.,1.35726946151947E-16));
#118855=DIRECTION('center_axis',(0.,-1.35726946151947E-16,1.));
#118856=DIRECTION('ref_axis',(0.,1.,1.35726946151947E-16));
#118857=DIRECTION('center_axis',(0.,1.35726946151947E-16,-1.));
#118858=DIRECTION('ref_axis',(0.,1.,1.35726946151947E-16));
#118859=DIRECTION('center_axis',(0.,-1.35726946151947E-16,1.));
#118860=DIRECTION('ref_axis',(0.,1.,1.35726946151947E-16));
#118861=DIRECTION('center_axis',(0.,1.22914743790472E-16,-1.));
#118862=DIRECTION('ref_axis',(0.,1.,1.22914743790472E-16));
#118863=DIRECTION('center_axis',(0.,-1.22914743790472E-16,1.));
#118864=DIRECTION('ref_axis',(0.,1.,1.22914743790472E-16));
#118865=DIRECTION('center_axis',(0.,1.22914743790472E-16,-1.));
#118866=DIRECTION('ref_axis',(0.,1.,1.22914743790472E-16));
#118867=DIRECTION('center_axis',(0.,-1.22914743790472E-16,1.));
#118868=DIRECTION('ref_axis',(0.,1.,1.22914743790472E-16));
#118869=DIRECTION('center_axis',(0.,0.,-1.));
#118870=DIRECTION('ref_axis',(0.,1.,0.));
#118871=DIRECTION('center_axis',(0.,0.,1.));
#118872=DIRECTION('ref_axis',(0.,1.,0.));
#118873=DIRECTION('center_axis',(0.,0.,-1.));
#118874=DIRECTION('ref_axis',(0.,1.,0.));
#118875=DIRECTION('center_axis',(0.,0.,1.));
#118876=DIRECTION('ref_axis',(0.,1.,0.));
#118877=DIRECTION('center_axis',(0.,0.,-1.));
#118878=DIRECTION('ref_axis',(0.,1.,0.));
#118879=DIRECTION('center_axis',(0.,0.,1.));
#118880=DIRECTION('ref_axis',(0.,1.,0.));
#118881=DIRECTION('center_axis',(0.,0.,-1.));
#118882=DIRECTION('ref_axis',(0.,1.,0.));
#118883=DIRECTION('center_axis',(0.,0.,1.));
#118884=DIRECTION('ref_axis',(0.,1.,0.));
#118885=DIRECTION('center_axis',(3.29883322342201E-16,1.,1.23467863058847E-16));
#118886=DIRECTION('ref_axis',(1.,-3.29883322342202E-16,0.));
#118887=DIRECTION('',(-1.,3.29883322342202E-16,0.));
#118888=DIRECTION('center_axis',(3.29883322342201E-16,1.,1.23467863058847E-16));
#118889=DIRECTION('ref_axis',(1.,-3.29883322342202E-16,0.));
#118890=DIRECTION('',(-1.,3.29883322342202E-16,0.));
#118891=DIRECTION('center_axis',(3.29883322342201E-16,-1.,-1.23467863058847E-16));
#118892=DIRECTION('ref_axis',(1.07891492167253E-48,1.23467863058847E-16,
-1.));
#118893=DIRECTION('',(1.,3.29883322342202E-16,0.));
#118894=DIRECTION('center_axis',(3.29883322342201E-16,-1.,-1.23467863058847E-16));
#118895=DIRECTION('ref_axis',(1.07891492167253E-48,1.23467863058847E-16,
-1.));
#118896=DIRECTION('',(1.,3.29883322342202E-16,0.));
#118897=DIRECTION('center_axis',(3.29883322342198E-16,1.,1.23467863058847E-16));
#118898=DIRECTION('ref_axis',(1.,-3.29883322342198E-16,0.));
#118899=DIRECTION('',(-1.,3.29883322342198E-16,0.));
#118900=DIRECTION('center_axis',(3.29883322342198E-16,1.,1.23467863058847E-16));
#118901=DIRECTION('ref_axis',(1.,-3.29883322342198E-16,0.));
#118902=DIRECTION('',(-1.,3.29883322342198E-16,0.));
#118903=DIRECTION('center_axis',(3.29883322342198E-16,-1.,-1.23467863058847E-16));
#118904=DIRECTION('ref_axis',(8.54897290170095E-49,1.23467863058847E-16,
-1.));
#118905=DIRECTION('',(1.,3.29883322342198E-16,0.));
#118906=DIRECTION('center_axis',(3.29883322342198E-16,-1.,-1.23467863058847E-16));
#118907=DIRECTION('ref_axis',(8.54897290170095E-49,1.23467863058847E-16,
-1.));
#118908=DIRECTION('',(1.,3.29883322342198E-16,0.));
#118909=DIRECTION('center_axis',(3.71118737634973E-16,1.,1.23467863058847E-16));
#118910=DIRECTION('ref_axis',(1.,-3.71118737634973E-16,0.));
#118911=DIRECTION('',(-1.,3.71118737634973E-16,0.));
#118912=DIRECTION('center_axis',(3.71118737634973E-16,1.,1.23467863058847E-16));
#118913=DIRECTION('ref_axis',(1.,-3.71118737634973E-16,0.));
#118914=DIRECTION('',(-1.,3.71118737634973E-16,0.));
#118915=DIRECTION('center_axis',(3.71118737634973E-16,-1.,-1.23467863058847E-16));
#118916=DIRECTION('ref_axis',(9.86109193995912E-49,1.23467863058847E-16,
-1.));
#118917=DIRECTION('',(1.,3.71118737634973E-16,0.));
#118918=DIRECTION('center_axis',(3.71118737634973E-16,-1.,-1.23467863058847E-16));
#118919=DIRECTION('ref_axis',(9.86109193995912E-49,1.23467863058847E-16,
-1.));
#118920=DIRECTION('',(1.,3.71118737634973E-16,0.));
#118921=DIRECTION('center_axis',(3.71118737634973E-16,1.,1.23467863058847E-16));
#118922=DIRECTION('ref_axis',(1.,-3.71118737634973E-16,0.));
#118923=DIRECTION('',(-1.,3.71118737634973E-16,0.));
#118924=DIRECTION('center_axis',(3.71118737634973E-16,1.,1.23467863058847E-16));
#118925=DIRECTION('ref_axis',(1.,-3.71118737634973E-16,0.));
#118926=DIRECTION('',(-1.,3.71118737634973E-16,0.));
#118927=DIRECTION('center_axis',(3.71118737634973E-16,-1.,-1.23467863058847E-16));
#118928=DIRECTION('ref_axis',(9.86109193995912E-49,1.23467863058847E-16,
-1.));
#118929=DIRECTION('',(1.,3.71118737634973E-16,0.));
#118930=DIRECTION('center_axis',(3.71118737634973E-16,-1.,-1.23467863058847E-16));
#118931=DIRECTION('ref_axis',(9.86109193995912E-49,1.23467863058847E-16,
-1.));
#118932=DIRECTION('',(1.,3.71118737634973E-16,0.));
#118933=DIRECTION('center_axis',(5.72252063890675E-16,1.,1.23467863058847E-16));
#118934=DIRECTION('ref_axis',(1.,-5.72252063890675E-16,0.));
#118935=DIRECTION('',(-1.,5.72252063890675E-16,0.));
#118936=DIRECTION('center_axis',(5.72252063890675E-16,1.,1.23467863058847E-16));
#118937=DIRECTION('ref_axis',(1.,-5.72252063890675E-16,0.));
#118938=DIRECTION('',(-1.,5.72252063890675E-16,0.));
#118939=DIRECTION('center_axis',(-1.90750687963558E-16,-1.,-1.23467863058847E-16));
#118940=DIRECTION('ref_axis',(-1.,1.90750687963558E-16,0.));
#118941=DIRECTION('',(1.,-1.90750687963558E-16,0.));
#118942=DIRECTION('center_axis',(-1.90750687963558E-16,-1.,-1.23467863058847E-16));
#118943=DIRECTION('ref_axis',(-1.,1.90750687963558E-16,0.));
#118944=DIRECTION('',(1.,-1.90750687963558E-16,0.));
#118945=DIRECTION('center_axis',(-1.23706245878324E-16,-1.,-1.23467863058847E-16));
#118946=DIRECTION('ref_axis',(-1.,1.23706245878324E-16,0.));
#118947=DIRECTION('',(1.,-1.23706245878324E-16,0.));
#118948=DIRECTION('center_axis',(-1.23706245878324E-16,-1.,-1.23467863058847E-16));
#118949=DIRECTION('ref_axis',(-1.,1.23706245878324E-16,0.));
#118950=DIRECTION('',(1.,-1.23706245878324E-16,0.));
#118951=DIRECTION('center_axis',(-1.23706245878324E-16,1.,1.23467863058847E-16));
#118952=DIRECTION('ref_axis',(1.,1.23706245878324E-16,0.));
#118953=DIRECTION('',(-1.,-1.23706245878324E-16,0.));
#118954=DIRECTION('center_axis',(-1.23706245878324E-16,1.,1.23467863058847E-16));
#118955=DIRECTION('ref_axis',(1.,1.23706245878324E-16,0.));
#118956=DIRECTION('',(-1.,-1.23706245878324E-16,0.));
#118957=DIRECTION('center_axis',(4.76876719908896E-16,-1.,-1.23467863058847E-16));
#118958=DIRECTION('ref_axis',(8.72767235901404E-49,1.23467863058847E-16,
-1.));
#118959=DIRECTION('',(1.,4.76876719908896E-16,0.));
#118960=DIRECTION('center_axis',(4.76876719908896E-16,-1.,-1.23467863058847E-16));
#118961=DIRECTION('ref_axis',(8.72767235901404E-49,1.23467863058847E-16,
-1.));
#118962=DIRECTION('',(1.,4.76876719908896E-16,0.));
#118963=DIRECTION('center_axis',(-9.53753439817791E-17,1.,1.23467863058847E-16));
#118964=DIRECTION('ref_axis',(4.60419424770999E-49,1.23467863058847E-16,
-1.));
#118965=DIRECTION('',(-1.,-9.53753439817791E-17,0.));
#118966=DIRECTION('center_axis',(-9.53753439817791E-17,1.,1.23467863058847E-16));
#118967=DIRECTION('ref_axis',(4.60419424770999E-49,1.23467863058847E-16,
-1.));
#118968=DIRECTION('',(-1.,-9.53753439817791E-17,0.));
#118969=DIRECTION('center_axis',(-0.592966514233392,0.805227118891249,0.));
#118970=DIRECTION('ref_axis',(-0.805227118891249,-0.592966514233392,0.));
#118971=DIRECTION('center_axis',(0.807208114890536,-0.590266938981735,2.28940150095415E-14));
#118972=DIRECTION('ref_axis',(0.590266938981735,0.807208114890536,-1.47426480814321E-30));
#118973=DIRECTION('center_axis',(0.,1.23467863058847E-16,-1.));
#118974=DIRECTION('ref_axis',(-0.705921937789672,-0.708289642552589,0.));
#118975=DIRECTION('center_axis',(-1.06667316881548E-30,-9.2152858313306E-45,
1.));
#118976=DIRECTION('ref_axis',(-8.63927780386936E-15,1.,6.22301527786114E-60));
#118977=DIRECTION('center_axis',(0.,0.,-1.));
#118978=DIRECTION('ref_axis',(0.,-1.,0.));
#118979=DIRECTION('center_axis',(0.,0.,-1.));
#118980=DIRECTION('ref_axis',(0.,-1.,0.));
#118981=DIRECTION('center_axis',(0.,-1.23467863058847E-16,1.));
#118982=DIRECTION('ref_axis',(0.,-1.,0.));
#118983=DIRECTION('center_axis',(0.,0.,1.));
#118984=DIRECTION('ref_axis',(0.,-1.,0.));
#118985=DIRECTION('center_axis',(-1.,0.,0.));
#118986=DIRECTION('ref_axis',(0.,1.,0.));
#118987=DIRECTION('center_axis',(0.,0.,-1.));
#118988=DIRECTION('ref_axis',(0.,1.,0.));
#118989=DIRECTION('center_axis',(0.,0.,-1.));
#118990=DIRECTION('ref_axis',(0.,1.,0.));
#118991=DIRECTION('center_axis',(-0.168369768252295,-0.882882757183484,
0.438371598312161));
#118992=DIRECTION('ref_axis',(2.05714353600353E-15,-0.444720469017533,-0.895669416937313));
#118993=DIRECTION('center_axis',(-0.507675385487887,0.517400512911953,-0.688884904906599));
#118994=DIRECTION('ref_axis',(1.34605780150592E-16,0.799589295572927,0.600547215800049));
#118995=DIRECTION('center_axis',(-0.506894799267393,0.516604973631544,-0.690055768539632));
#118996=DIRECTION('ref_axis',(4.2861068992561E-17,0.800521374177574,0.599304204461181));
#118997=DIRECTION('center_axis',(0.,0.,1.));
#118998=DIRECTION('ref_axis',(1.,0.,0.));
#118999=DIRECTION('center_axis',(-0.663838127753914,-0.747876286654537,
-9.2338686945498E-17));
#119000=DIRECTION('ref_axis',(-0.747876286654537,0.663838127753914,1.66533453693772E-13));
#119001=DIRECTION('center_axis',(-0.187328576766759,-0.982297309538482,
0.));
#119002=DIRECTION('ref_axis',(0.982297309538482,-0.187328576766759,0.));
#119003=DIRECTION('center_axis',(-0.668574108837973,-0.743645521059268,
0.));
#119004=DIRECTION('ref_axis',(0.743645521059268,-0.668574108837973,0.));
#119005=DIRECTION('center_axis',(0.,-1.23467863058847E-16,1.));
#119006=DIRECTION('ref_axis',(0.,-1.,0.));
#119007=DIRECTION('center_axis',(-0.679956281045645,-0.733252654865004,
0.));
#119008=DIRECTION('ref_axis',(0.733252654865004,-0.679956281045645,0.));
#119009=DIRECTION('center_axis',(5.71153601538328E-31,2.64211616260599E-45,
-1.));
#119010=DIRECTION('ref_axis',(4.6259292692715E-15,-1.,-3.11150763893057E-61));
#119011=DIRECTION('center_axis',(0.,0.,1.));
#119012=DIRECTION('ref_axis',(0.,-1.,0.));
#119013=DIRECTION('center_axis',(-0.775870249713592,-0.63089250717485,1.27793330397298E-14));
#119014=DIRECTION('ref_axis',(0.63089250717485,-0.775870249713592,-7.13011169472736E-30));
#119015=DIRECTION('center_axis',(0.,-1.23467863058847E-16,1.));
#119016=DIRECTION('ref_axis',(0.,-1.,0.));
#119017=DIRECTION('center_axis',(-0.746021307914873,-0.665922073621968,
0.));
#119018=DIRECTION('ref_axis',(0.665922073621968,-0.746021307914873,0.));
#119019=DIRECTION('center_axis',(2.41254715360152E-30,4.7140880421464E-44,
-1.));
#119020=DIRECTION('ref_axis',(1.95398793972133E-14,-1.,1.49352366668667E-58));
#119021=DIRECTION('center_axis',(0.,0.,1.));
#119022=DIRECTION('ref_axis',(0.,-1.,0.));
#119023=DIRECTION('center_axis',(0.507468854451513,-0.517190025527329,0.68919506618715));
#119024=DIRECTION('ref_axis',(1.08020880515219E-16,-0.799836347973839,-0.600218140728745));
#119025=DIRECTION('center_axis',(0.,-1.23467863058847E-16,1.));
#119026=DIRECTION('ref_axis',(0.,-1.,0.));
#119027=DIRECTION('center_axis',(-0.923323390669864,-0.38402332773141,1.28136860937081E-14));
#119028=DIRECTION('ref_axis',(0.38402332773141,-0.923323390669864,2.90201745723254E-30));
#119029=DIRECTION('center_axis',(-6.28268961692158E-30,3.19696055675322E-43,
-1.));
#119030=DIRECTION('ref_axis',(-5.08852219619863E-14,-1.,-2.38963786669868E-58));
#119031=DIRECTION('center_axis',(0.,0.,1.));
#119032=DIRECTION('ref_axis',(0.,-1.,0.));
#119033=DIRECTION('center_axis',(0.511561679834273,-0.521361253861094,0.682998602266158));
#119034=DIRECTION('ref_axis',(-1.21631079100244E-16,-0.79488081246627,-0.606765600518819));
#119035=DIRECTION('center_axis',(-0.987526870499689,-0.134244619791538,
0.0822743100737742));
#119036=DIRECTION('ref_axis',(0.134701294632915,-0.990886250396188,-7.62230551969098E-18));
#119037=DIRECTION('center_axis',(0.887573437172827,0.12065692809958,0.444584411925099));
#119038=DIRECTION('ref_axis',(0.447856331161543,-5.04904183848934E-18,-0.89410553439654));
#119039=DIRECTION('center_axis',(0.502574642452133,-0.589207696134777,-0.632655529952643));
#119040=DIRECTION('ref_axis',(-0.234516419283699,0.611436391027521,-0.755743070635512));
#119041=DIRECTION('center_axis',(0.,0.,1.));
#119042=DIRECTION('ref_axis',(1.,0.,0.));
#119043=DIRECTION('center_axis',(0.606371999687993,0.771616335224111,-0.192148976603301));
#119044=DIRECTION('ref_axis',(-0.786267832350933,0.617885827487704,-3.1641897774151E-17));
#119045=DIRECTION('center_axis',(-0.645804421056786,0.763502881293522,1.01980482580395E-14));
#119046=DIRECTION('ref_axis',(-0.763502881293522,-0.645804421056786,-6.9816295225584E-30));
#119047=DIRECTION('center_axis',(0.48724015249101,0.488874385354372,0.723601319197887));
#119048=DIRECTION('ref_axis',(1.47352524967685E-15,-0.828613098245121,0.559821697879442));
#119049=DIRECTION('center_axis',(0.488418020654004,0.490056204158282,0.722006062208899));
#119050=DIRECTION('ref_axis',(-3.20373038523992E-15,-0.827409999881363,
0.561598336977882));
#119051=DIRECTION('center_axis',(-0.753146254930614,0.657853113304171,3.00335537434998E-14));
#119052=DIRECTION('ref_axis',(-0.657853113304171,-0.753146254930614,-2.96993835591878E-30));
#119053=DIRECTION('center_axis',(-0.171101227036283,0.869601781127171,0.463159920942141));
#119054=DIRECTION('ref_axis',(4.21773228904835E-17,-0.470092156192753,0.882617337630554));
#119055=DIRECTION('center_axis',(0.484433158250521,0.486057976285942,0.727373465886845));
#119056=DIRECTION('ref_axis',(3.34045680200078E-15,-0.831447136037245,0.555603869654868));
#119057=DIRECTION('center_axis',(1.,0.,0.));
#119058=DIRECTION('ref_axis',(0.,-1.,0.));
#119059=DIRECTION('center_axis',(-0.193053842425666,0.981173356447606,-0.00539059570228739));
#119060=DIRECTION('ref_axis',(-0.981187612482096,-0.193056647416463,-1.03740416739262E-18));
#119061=DIRECTION('center_axis',(-0.663957144707683,0.747700087626819,-0.0102707815899847));
#119062=DIRECTION('ref_axis',(-0.747739527797473,-0.663992167551103,3.3311423852743E-19));
#119063=DIRECTION('center_axis',(0.485576620175616,0.487205273451398,0.725841833638689));
#119064=DIRECTION('ref_axis',(-1.3020744827461E-16,-0.830298240911906,0.557319326004935));
#119065=DIRECTION('center_axis',(-0.210025631952355,0.977695880078777,0.));
#119066=DIRECTION('ref_axis',(-0.977695880078777,-0.210025631952355,0.));
#119067=DIRECTION('center_axis',(0.869253009153379,-0.170328745809824,0.464098399510975));
#119068=DIRECTION('ref_axis',(0.470980702241858,8.1123542202202E-17,-0.882143513333157));
#119069=DIRECTION('center_axis',(0.,1.23467863058847E-16,-1.));
#119070=DIRECTION('ref_axis',(0.,1.,0.));
#119071=DIRECTION('center_axis',(-0.67420688908099,0.738542531419643,0.));
#119072=DIRECTION('ref_axis',(-0.738542531419643,-0.67420688908099,0.));
#119073=DIRECTION('center_axis',(-4.28365201153744E-31,-1.48619034146585E-45,
1.));
#119074=DIRECTION('ref_axis',(-3.46944695195361E-15,1.,1.24460305557223E-60));
#119075=DIRECTION('center_axis',(0.,0.,-1.));
#119076=DIRECTION('ref_axis',(0.,1.,0.));
#119077=DIRECTION('center_axis',(1.,0.,0.));
#119078=DIRECTION('ref_axis',(0.,-1.,0.));
#119079=DIRECTION('center_axis',(0.752788125817861,-0.658228853504028,-0.00669432912290745));
#119080=DIRECTION('ref_axis',(-0.658243602947644,-0.752804994124312,-1.11021690861332E-13));
#119081=DIRECTION('center_axis',(0.981331609270135,-0.192290369398073,-0.00356180909645361));
#119082=DIRECTION('ref_axis',(0.192291589154029,0.981337834153263,-1.28820063606849E-18));
#119083=DIRECTION('center_axis',(0.,1.23467863058847E-16,-1.));
#119084=DIRECTION('ref_axis',(0.,1.,0.));
#119085=DIRECTION('center_axis',(-0.74079592940915,0.671730147433353,0.));
#119086=DIRECTION('ref_axis',(-0.671730147433353,-0.74079592940915,0.));
#119087=DIRECTION('center_axis',(-1.64492525510334E-30,-2.19148451090235E-44,
1.));
#119088=DIRECTION('ref_axis',(-1.33226996430588E-14,1.,1.74244427780112E-59));
#119089=DIRECTION('center_axis',(0.,0.,-1.));
#119090=DIRECTION('ref_axis',(0.,1.,0.));
#119091=DIRECTION('center_axis',(0.979119873047182,-0.203283728330798,0.));
#119092=DIRECTION('ref_axis',(0.203283728330798,0.979119873047182,0.));
#119093=DIRECTION('center_axis',(0.,1.23467863058847E-16,-1.));
#119094=DIRECTION('ref_axis',(0.,1.,0.));
#119095=DIRECTION('center_axis',(0.,0.,-1.));
#119096=DIRECTION('ref_axis',(0.,1.,0.));
#119097=DIRECTION('center_axis',(-2.57019120692247E-30,-5.35028522927707E-44,
1.));
#119098=DIRECTION('ref_axis',(-2.08166817117217E-14,1.,-1.99136488891557E-59));
#119099=DIRECTION('center_axis',(0.,-1.23467863058847E-16,1.));
#119100=DIRECTION('ref_axis',(1.22464679914735E-16,1.,1.21959207089992E-16));
#119101=DIRECTION('center_axis',(2.7383203336382E-32,1.19614019798162E-16,
-1.));
#119102=DIRECTION('ref_axis',(7.105427357601E-15,-1.,-1.19614019798162E-16));
#119103=DIRECTION('center_axis',(0.,-1.19356871810915E-16,1.));
#119104=DIRECTION('ref_axis',(0.,-1.,-1.19356871810915E-16));
#119105=DIRECTION('center_axis',(0.982297019165463,-0.187330099393145,0.));
#119106=DIRECTION('ref_axis',(0.187330099393145,0.982297019165463,0.));
#119107=DIRECTION('center_axis',(0.,-1.23467863058847E-16,1.));
#119108=DIRECTION('ref_axis',(0.,-1.,0.));
#119109=DIRECTION('center_axis',(0.777162624242377,-0.629299813666508,0.));
#119110=DIRECTION('ref_axis',(0.629299813666508,0.777162624242377,0.));
#119111=DIRECTION('center_axis',(4.46763300492346E-31,1.61659432440069E-45,
-1.));
#119112=DIRECTION('ref_axis',(3.61845819166247E-15,-1.,1.86690458335834E-60));
#119113=DIRECTION('center_axis',(0.,0.,1.));
#119114=DIRECTION('ref_axis',(0.,-1.,0.));
#119115=DIRECTION('center_axis',(0.,-1.23467863058847E-16,1.));
#119116=DIRECTION('ref_axis',(0.,-1.,0.));
#119117=DIRECTION('center_axis',(0.635030358342585,-0.772487180465338,0.));
#119118=DIRECTION('ref_axis',(0.772487180465338,0.635030358342585,0.));
#119119=DIRECTION('center_axis',(1.09661491495359E-30,9.73989702183063E-45,
-1.));
#119120=DIRECTION('ref_axis',(8.88178419700125E-15,-1.,2.48920611114446E-60));
#119121=DIRECTION('center_axis',(0.,0.,1.));
#119122=DIRECTION('ref_axis',(0.,-1.,0.));
#119123=DIRECTION('center_axis',(0.,-1.23467863058847E-16,1.));
#119124=DIRECTION('ref_axis',(0.,-1.,0.));
#119125=DIRECTION('center_axis',(0.0394959395290733,-0.999219730970479,
0.));
#119126=DIRECTION('ref_axis',(0.999219730970479,0.0394959395290733,0.));
#119127=DIRECTION('center_axis',(6.70144950738521E-31,3.63733722990157E-45,
-1.));
#119128=DIRECTION('ref_axis',(5.42768728749372E-15,-1.,2.48920611114446E-60));
#119129=DIRECTION('center_axis',(0.,0.,1.));
#119130=DIRECTION('ref_axis',(0.,-1.,0.));
#119131=DIRECTION('center_axis',(0.,-1.23467863058847E-16,1.));
#119132=DIRECTION('ref_axis',(0.,-1.,-1.33055111034894E-16));
#119133=DIRECTION('center_axis',(-0.0394959395290663,-0.999219730970479,
0.));
#119134=DIRECTION('ref_axis',(0.999219730970479,-0.0394959395290663,0.));
#119135=DIRECTION('center_axis',(0.,1.30058395245648E-16,-1.));
#119136=DIRECTION('ref_axis',(0.,-1.,-1.30058395245648E-16));
#119137=DIRECTION('center_axis',(0.,-1.29997489681772E-16,1.));
#119138=DIRECTION('ref_axis',(0.,-1.,-1.29997489681772E-16));
#119139=DIRECTION('center_axis',(0.,-1.23467863058847E-16,1.));
#119140=DIRECTION('ref_axis',(0.,-1.,0.));
#119141=DIRECTION('center_axis',(-0.635030358342616,-0.772487180465313,
0.));
#119142=DIRECTION('ref_axis',(0.772487180465313,-0.635030358342616,0.));
#119143=DIRECTION('center_axis',(-5.21223850574408E-31,2.20036449710098E-45,
-1.));
#119144=DIRECTION('ref_axis',(-4.22153455693958E-15,-1.,-9.33452291679171E-61));
#119145=DIRECTION('center_axis',(0.,0.,1.));
#119146=DIRECTION('ref_axis',(0.,-1.,0.));
#119147=DIRECTION('center_axis',(0.,-1.23467863058847E-16,1.));
#119148=DIRECTION('ref_axis',(0.,-1.,0.));
#119149=DIRECTION('center_axis',(-0.774287490710421,-0.632834008037937,
0.));
#119150=DIRECTION('ref_axis',(0.632834008037937,-0.774287490710421,0.));
#119151=DIRECTION('center_axis',(0.,0.,-1.));
#119152=DIRECTION('ref_axis',(0.,-1.,0.));
#119153=DIRECTION('center_axis',(0.,0.,1.));
#119154=DIRECTION('ref_axis',(0.,-1.,0.));
#119155=DIRECTION('center_axis',(0.,-1.23467863058847E-16,1.));
#119156=DIRECTION('ref_axis',(0.,-1.,0.));
#119157=DIRECTION('center_axis',(-0.999225121087074,-0.0393593367388477,
0.));
#119158=DIRECTION('ref_axis',(0.0393593367388477,-0.999225121087074,0.));
#119159=DIRECTION('center_axis',(5.21223850574404E-31,2.20036449710094E-45,
-1.));
#119160=DIRECTION('ref_axis',(4.22153455693955E-15,-1.,2.48920611114446E-60));
#119161=DIRECTION('center_axis',(0.,0.,1.));
#119162=DIRECTION('ref_axis',(0.,-1.,0.));
#119163=DIRECTION('center_axis',(0.,-1.23467863058847E-16,1.));
#119164=DIRECTION('ref_axis',(0.,-1.,-1.33055111034894E-16));
#119165=DIRECTION('center_axis',(0.,-1.29997489681772E-16,1.));
#119166=DIRECTION('ref_axis',(0.,-1.,-1.29997489681772E-16));
#119167=DIRECTION('center_axis',(-3.39506970834015E-31,1.30058395245648E-16,
-1.));
#119168=DIRECTION('ref_axis',(5.15143483426073E-14,-1.,-1.30058395245648E-16));
#119169=DIRECTION('center_axis',(0.,0.,1.));
#119170=DIRECTION('ref_axis',(0.75170336763964,-0.659501362454411,0.));
#119171=DIRECTION('center_axis',(-0.00318936290742699,0.00297678217545832,
-0.999990483320779));
#119172=DIRECTION('ref_axis',(0.747789842749455,-0.6639211772416,-0.00436136341903465));
#119173=DIRECTION('center_axis',(0.659496851377394,0.751707325375577,0.));
#119174=DIRECTION('ref_axis',(-0.751707325375577,0.659496851377394,0.));
#119175=DIRECTION('center_axis',(0.657034976183429,0.753860093168249,-1.01740733956786E-14));
#119176=DIRECTION('ref_axis',(-0.753860093168249,0.657034976183429,-8.45764823615526E-31));
#119177=DIRECTION('center_axis',(-0.00280476608066071,0.00263885430337773,
-0.999992584840107));
#119178=DIRECTION('ref_axis',(0.937191712771117,0.348810515489431,-0.00170815606344439));
#119179=DIRECTION('center_axis',(0.768895279480121,-0.207195498703726,0.604871948853723));
#119180=DIRECTION('ref_axis',(0.618289095466814,1.21523947502978E-17,-0.785950758271044));
#119181=DIRECTION('center_axis',(0.202724571193613,-0.760898522337225,0.616389638896853));
#119182=DIRECTION('ref_axis',(1.87348493224475E-17,-0.629459870756021,-0.777032992290426));
#119183=DIRECTION('center_axis',(0.767736348840716,-0.206883199723352,0.606448876939313));
#119184=DIRECTION('ref_axis',(0.619859127336644,-1.17584790122141E-16,-0.784713108248775));
#119185=DIRECTION('center_axis',(-0.243334995703589,-0.96954396966785,-0.0277951568918529));
#119186=DIRECTION('ref_axis',(0.594809401908895,-0.126526334687349,-0.793846875682815));
#119187=DIRECTION('center_axis',(0.260190354028299,0.965557341472079,-1.40549396816343E-10));
#119188=DIRECTION('ref_axis',(0.58403426831887,-0.15738069260472,-0.796326121023605));
#119189=DIRECTION('center_axis',(0.202457297762738,-0.759895348634851,0.617713608159743));
#119190=DIRECTION('ref_axis',(-5.55058625584594E-17,-0.630776296546234,
-0.775964730973913));
#119191=DIRECTION('center_axis',(-0.966292363520655,-0.25744721439873,4.29897349204163E-11));
#119192=DIRECTION('ref_axis',(0.159028116924834,-0.596889950284185,-0.786404759190256));
#119193=DIRECTION('center_axis',(0.966468863382725,0.256741605888852,-0.00465659932972454));
#119194=DIRECTION('ref_axis',(0.154910761359747,-0.597411475844062,-0.786830467473625));
#119195=DIRECTION('center_axis',(0.578576029254642,-0.155909851599689,0.800588468906525));
#119196=DIRECTION('ref_axis',(0.810499837678775,1.21842170142303E-15,-0.585738860860947));
#119197=DIRECTION('center_axis',(0.153941565569776,-0.577798286012631,0.801530495409122));
#119198=DIRECTION('ref_axis',(1.29290181198153E-17,-0.811200037627138,-0.584768756820788));
#119199=DIRECTION('center_axis',(0.0544019837731304,0.025960154057113,0.998181593981215));
#119200=DIRECTION('ref_axis',(0.998518116145471,-1.61274188638027E-18,-0.054420324597515));
#119201=DIRECTION('center_axis',(-0.025995718416376,-0.0542003143889016,
0.998191639187667));
#119202=DIRECTION('ref_axis',(-1.6064497712818E-18,-0.99852908789078,-0.0542186373492239));
#119203=DIRECTION('center_axis',(0.734334158412678,0.678788143523695,-2.48736119588291E-13));
#119204=DIRECTION('ref_axis',(-0.678788143523695,0.734334158412678,-6.81231552358944E-29));
#119205=DIRECTION('center_axis',(-0.680870844883917,-0.73240350394237,-1.91708814121709E-12));
#119206=DIRECTION('ref_axis',(0.73240350394237,-0.680870844883917,-1.31317411609931E-27));
#119207=DIRECTION('center_axis',(0.,-1.23467863058847E-16,1.));
#119208=DIRECTION('ref_axis',(0.,-1.,0.));
#119209=DIRECTION('center_axis',(-9.86953423458227E-31,7.88931658768281E-45,
-1.));
#119210=DIRECTION('ref_axis',(-7.99360577730113E-15,-1.,2.48920611114446E-60));
#119211=DIRECTION('center_axis',(0.,0.,1.));
#119212=DIRECTION('ref_axis',(0.,1.,0.));
#119213=DIRECTION('center_axis',(0.0255375237255525,-0.0535186253292443,
-0.998240247447895));
#119214=DIRECTION('ref_axis',(2.96412751937958E-19,0.998565915482956,-0.0535360853601283));
#119215=DIRECTION('center_axis',(-0.682537484892591,0.730850587819765,-8.37209378123771E-13));
#119216=DIRECTION('ref_axis',(-0.730850587819765,-0.682537484892591,3.92323810141884E-28));
#119217=DIRECTION('center_axis',(0.,-1.23467863058847E-16,1.));
#119218=DIRECTION('ref_axis',(0.,-1.,0.));
#119219=DIRECTION('center_axis',(-0.735878524541007,0.677113577710085,-5.64206319996869E-13));
#119220=DIRECTION('ref_axis',(-0.677113577710085,-0.735878524541007,-1.38055872491966E-28));
#119221=DIRECTION('center_axis',(5.92172054074936E-30,-2.84015397156581E-43,
1.));
#119222=DIRECTION('ref_axis',(4.79616346638068E-14,1.,-2.78791084448179E-58));
#119223=DIRECTION('center_axis',(0.,0.,-1.));
#119224=DIRECTION('ref_axis',(0.,-1.,0.));
#119225=DIRECTION('center_axis',(-0.152544532818274,-0.577842847451632,
-0.801765432752152));
#119226=DIRECTION('ref_axis',(-4.14384419008336E-17,0.811259933931047,-0.58468565879299));
#119227=DIRECTION('center_axis',(-0.0536778879072088,0.0251150971461135,
-0.998242413567548));
#119228=DIRECTION('ref_axis',(-0.998557392321894,-9.29874389531901E-20,
0.0536948250700053));
#119229=DIRECTION('center_axis',(-0.19315692461333,-0.731683694333232,-0.653704347485004));
#119230=DIRECTION('ref_axis',(3.51224977473848E-17,0.66625127354731,-0.745727323152764));
#119231=DIRECTION('center_axis',(-0.576537673896198,-0.156770156178271,
-0.801889910592596));
#119232=DIRECTION('ref_axis',(-0.811929324239482,3.97972821433516E-17,0.583755747243673));
#119233=DIRECTION('center_axis',(-0.193538145022295,-0.733127767631913,
-0.651971366509586));
#119234=DIRECTION('ref_axis',(-1.09087611421558E-16,0.664535912353125,-0.747256328974871));
#119235=DIRECTION('center_axis',(-0.966876318111592,0.25524534368911,8.60979798737377E-11));
#119236=DIRECTION('ref_axis',(0.166411982437669,0.630373124965737,-0.758245854206995));
#119237=DIRECTION('center_axis',(0.967398007177023,-0.253182433216653,-0.00630485689132568));
#119238=DIRECTION('ref_axis',(0.16111421782421,0.634435934472465,-0.755998183770929));
#119239=DIRECTION('center_axis',(-0.72784499809572,-0.197913127261801,-0.656560776169652));
#119240=DIRECTION('ref_axis',(-0.669809908048189,2.97308687105849E-17,0.742532616846207));
#119241=DIRECTION('center_axis',(-0.72888212476865,-0.19819513920631,-0.655323992379136));
#119242=DIRECTION('ref_axis',(-0.668587032943078,1.18015531912611E-16,0.743633901446385));
#119243=DIRECTION('center_axis',(-0.257377402244523,0.96626185396935,-0.00974178513293261));
#119244=DIRECTION('ref_axis',(0.635976884577247,0.161793976065296,-0.754556897518273));
#119245=DIRECTION('center_axis',(0.262389207131878,-0.964962125671627,2.3868460211661E-11));
#119246=DIRECTION('ref_axis',(0.633554268004896,0.172273913779853,-0.754274941996453));
#119247=DIRECTION('center_axis',(-0.70592193778968,-0.708289642552581,-8.74510085926821E-17));
#119248=DIRECTION('ref_axis',(0.708289642552581,-0.70592193778968,-3.19694546253078E-33));
#119249=DIRECTION('',(0.70592193778968,0.708289642552581,8.74510085926821E-17));
#119250=DIRECTION('',(-0.70592193778968,-0.708289642552581,-8.74510085926821E-17));
#119251=DIRECTION('center_axis',(-0.705921937789676,-0.708289642552585,
6.53108990768421E-15));
#119252=DIRECTION('ref_axis',(0.708289642552585,-0.705921937789676,-2.24639971032546E-30));
#119253=DIRECTION('center_axis',(0.,0.,1.));
#119254=DIRECTION('ref_axis',(0.,1.,0.));
#119255=DIRECTION('center_axis',(-0.74079592940915,0.671730147433353,0.));
#119256=DIRECTION('ref_axis',(-0.671730147433353,-0.74079592940915,0.));
#119257=DIRECTION('center_axis',(0.,0.,-1.));
#119258=DIRECTION('ref_axis',(0.,1.,0.));
#119259=DIRECTION('center_axis',(0.,1.23467863058847E-16,-1.));
#119260=DIRECTION('ref_axis',(0.,1.,0.));
#119261=DIRECTION('center_axis',(0.,0.,-1.));
#119262=DIRECTION('ref_axis',(0.,1.,0.));
#119263=DIRECTION('center_axis',(0.,0.,-1.));
#119264=DIRECTION('ref_axis',(0.,1.,0.));
#119265=DIRECTION('center_axis',(-2.41254715360153E-30,-4.71408804214643E-44,
1.));
#119266=DIRECTION('ref_axis',(-1.95398793972133E-14,1.,5.9740946667467E-59));
#119267=DIRECTION('center_axis',(-0.674206889080985,0.738542531419647,0.));
#119268=DIRECTION('ref_axis',(-0.738542531419647,-0.674206889080985,0.));
#119269=DIRECTION('center_axis',(0.7059219377897,0.708289642552562,2.19056695270365E-17));
#119270=DIRECTION('ref_axis',(-0.708289642552562,0.7059219377897,4.72941823813195E-33));
#119271=DIRECTION('center_axis',(0.,0.,-1.));
#119272=DIRECTION('ref_axis',(0.,1.,0.));
#119273=DIRECTION('center_axis',(0.,0.,1.));
#119274=DIRECTION('ref_axis',(0.,1.,0.));
#119275=DIRECTION('center_axis',(0.7059219377897,0.708289642552561,8.74510085926797E-17));
#119276=DIRECTION('ref_axis',(-0.708289642552561,0.7059219377897,-8.55019604084016E-33));
#119277=DIRECTION('',(0.7059219377897,0.708289642552561,8.74510085926797E-17));
#119278=DIRECTION('',(-0.7059219377897,-0.708289642552561,-8.74510085926797E-17));
#119279=DIRECTION('center_axis',(0.964962125666191,0.262389207151869,3.23966346967465E-17));
#119280=DIRECTION('ref_axis',(-0.262389207151869,0.964962125666191,-4.57090956622107E-33));
#119281=DIRECTION('',(0.964962125666191,0.262389207151869,3.23966346967465E-17));
#119282=DIRECTION('',(-0.964962125666191,-0.262389207151869,-3.23966346967465E-17));
#119283=DIRECTION('center_axis',(-0.964962125666191,-0.26238920715187,-2.42758782660955E-15));
#119284=DIRECTION('ref_axis',(0.26238920715187,-0.964962125666191,2.22950724024121E-31));
#119285=DIRECTION('center_axis',(0.,0.,1.));
#119286=DIRECTION('ref_axis',(0.,1.,0.));
#119287=DIRECTION('center_axis',(-0.735878524541004,0.677113577710087,0.));
#119288=DIRECTION('ref_axis',(-0.677113577710087,-0.735878524541004,0.));
#119289=DIRECTION('center_axis',(0.,0.,-1.));
#119290=DIRECTION('ref_axis',(0.,1.,0.));
#119291=DIRECTION('center_axis',(0.,1.23467863058847E-16,-1.));
#119292=DIRECTION('ref_axis',(0.,1.,0.));
#119293=DIRECTION('center_axis',(-0.682537484892593,0.730850587819763,0.));
#119294=DIRECTION('ref_axis',(-0.730850587819763,-0.682537484892593,0.));
#119295=DIRECTION('center_axis',(0.,0.,-1.));
#119296=DIRECTION('ref_axis',(0.,1.,0.));
#119297=DIRECTION('center_axis',(4.93476711729114E-30,-1.97232914692071E-43,
1.));
#119298=DIRECTION('ref_axis',(3.99680288865056E-14,1.,0.));
#119299=DIRECTION('center_axis',(0.255245343760721,0.966876318092687,2.36149381309596E-15));
#119300=DIRECTION('ref_axis',(-0.966876318092687,0.255245343760721,9.80822191756775E-31));
#119301=DIRECTION('center_axis',(0.,0.,-1.));
#119302=DIRECTION('ref_axis',(0.,1.,0.));
#119303=DIRECTION('center_axis',(-5.71153601538325E-31,-2.64211616260596E-45,
1.));
#119304=DIRECTION('ref_axis',(-4.62592926927148E-15,1.,1.24460305557223E-60));
#119305=DIRECTION('center_axis',(-0.255245343760725,-0.966876318092686,
-1.1937815283711E-16));
#119306=DIRECTION('ref_axis',(0.966876318092686,-0.255245343760725,-8.61241374820812E-33));
#119307=DIRECTION('',(-0.255245343760725,-0.966876318092686,-1.1937815283711E-16));
#119308=DIRECTION('',(0.255245343760725,0.966876318092686,1.1937815283711E-16));
#119309=DIRECTION('center_axis',(-0.257447214431338,0.966292363511968,1.19306053212906E-16));
#119310=DIRECTION('ref_axis',(-0.966292363511968,-0.257447214431338,-1.5335664280992E-33));
#119311=DIRECTION('',(0.257447214431338,-0.966292363511968,-1.19306053212906E-16));
#119312=DIRECTION('',(-0.257447214431338,0.966292363511968,1.19306053212906E-16));
#119313=DIRECTION('center_axis',(-0.257447214431328,0.96629236351197,-1.78800005081742E-14));
#119314=DIRECTION('ref_axis',(-0.96629236351197,-0.257447214431328,-3.12759209575828E-30));
#119315=DIRECTION('center_axis',(0.680870844883904,0.732403503942382,0.));
#119316=DIRECTION('ref_axis',(-0.732403503942382,0.680870844883904,0.));
#119317=DIRECTION('center_axis',(0.,0.,-1.));
#119318=DIRECTION('ref_axis',(0.,-1.,0.));
#119319=DIRECTION('center_axis',(0.,0.,1.));
#119320=DIRECTION('ref_axis',(0.,-1.,0.));
#119321=DIRECTION('center_axis',(0.,-1.23467863058847E-16,1.));
#119322=DIRECTION('ref_axis',(0.,-1.,0.));
#119323=DIRECTION('center_axis',(0.734334158412675,0.678788143523698,0.));
#119324=DIRECTION('ref_axis',(-0.678788143523698,0.734334158412675,0.));
#119325=DIRECTION('center_axis',(4.05747518532827E-30,1.33339190228861E-43,
-1.));
#119326=DIRECTION('ref_axis',(3.28626015289047E-14,-1.,2.58877435559024E-58));
#119327=DIRECTION('center_axis',(0.,0.,1.));
#119328=DIRECTION('ref_axis',(0.,-1.,0.));
#119329=DIRECTION('center_axis',(-1.14230720307665E-30,1.05684646504238E-44,
-1.));
#119330=DIRECTION('ref_axis',(-9.25185853854296E-15,-1.,-3.73380916671668E-60));
#119331=DIRECTION('center_axis',(0.,0.,1.));
#119332=DIRECTION('ref_axis',(0.,-1.,0.));
#119333=DIRECTION('center_axis',(0.965557341499939,-0.260190353924909,4.11871123919569E-15));
#119334=DIRECTION('ref_axis',(0.260190353924909,0.965557341499939,-2.2632930465492E-31));
#119335=DIRECTION('center_axis',(0.965557341499939,-0.260190353924911,-3.21251469876339E-17));
#119336=DIRECTION('ref_axis',(0.260190353924911,0.965557341499939,-9.87488652925334E-34));
#119337=DIRECTION('',(-0.965557341499939,0.260190353924911,3.21251469876339E-17));
#119338=DIRECTION('',(0.965557341499939,-0.260190353924911,-3.21251469876339E-17));
#119339=DIRECTION('center_axis',(0.700366780446484,-0.713783141330072,-8.81292791474553E-17));
#119340=DIRECTION('ref_axis',(0.713783141330072,0.700366780446484,-8.54636793605324E-33));
#119341=DIRECTION('',(0.700366780446485,-0.713783141330072,-8.81292791474553E-17));
#119342=DIRECTION('',(-0.700366780446485,0.713783141330072,8.81292791474553E-17));
#119343=DIRECTION('center_axis',(-0.700366780446484,0.713783141330073,0.));
#119344=DIRECTION('ref_axis',(-0.713783141330073,-0.700366780446484,0.));
#119345=DIRECTION('center_axis',(0.679956281045647,0.733252654865001,0.));
#119346=DIRECTION('ref_axis',(-0.733252654865001,0.679956281045647,0.));
#119347=DIRECTION('center_axis',(0.,0.,-1.));
#119348=DIRECTION('ref_axis',(0.,-1.,0.));
#119349=DIRECTION('center_axis',(0.,0.,1.));
#119350=DIRECTION('ref_axis',(0.,-1.,0.));
#119351=DIRECTION('center_axis',(0.,-1.23467863058847E-16,1.));
#119352=DIRECTION('ref_axis',(0.,-1.,0.));
#119353=DIRECTION('center_axis',(0.746021307914879,0.665922073621961,-1.23220336456872E-14));
#119354=DIRECTION('ref_axis',(-0.665922073621961,0.746021307914879,1.41534494748923E-30));
#119355=DIRECTION('center_axis',(3.28984144636074E-30,8.76588974171719E-44,
-1.));
#119356=DIRECTION('ref_axis',(2.66453258755498E-14,-1.,1.59309191113245E-58));
#119357=DIRECTION('center_axis',(0.,0.,1.));
#119358=DIRECTION('ref_axis',(0.,-1.,0.));
#119359=DIRECTION('center_axis',(0.,0.,-1.));
#119360=DIRECTION('ref_axis',(0.,-1.,0.));
#119361=DIRECTION('center_axis',(0.,0.,1.));
#119362=DIRECTION('ref_axis',(0.,-1.,0.));
#119363=DIRECTION('center_axis',(0.700366780446456,-0.7137831413301,0.));
#119364=DIRECTION('ref_axis',(0.7137831413301,0.700366780446456,0.));
#119365=DIRECTION('center_axis',(-0.700366780446451,0.713783141330105,8.81292791474594E-17));
#119366=DIRECTION('ref_axis',(-0.713783141330105,-0.700366780446451,4.73735951537523E-32));
#119367=DIRECTION('',(0.700366780446451,-0.713783141330105,-8.81292791474594E-17));
#119368=DIRECTION('',(-0.700366780446451,0.713783141330105,8.81292791474594E-17));
#119369=DIRECTION('center_axis',(0.,0.,-1.));
#119370=DIRECTION('ref_axis',(0.,1.,0.));
#119371=DIRECTION('',(0.,1.23467863058847E-16,-1.));
#119372=DIRECTION('',(-6.16297582203915E-33,-1.23467863058847E-16,1.));
#119373=DIRECTION('center_axis',(0.,0.,-1.));
#119374=DIRECTION('ref_axis',(0.,1.,0.));
#119375=DIRECTION('',(0.,-1.23467863058847E-16,1.));
#119376=DIRECTION('',(7.37292681274632E-34,1.23467863058847E-16,-1.));
#119377=DIRECTION('center_axis',(0.,0.,1.));
#119378=DIRECTION('ref_axis',(0.,-1.,0.));
#119379=DIRECTION('',(0.,1.23467863058847E-16,-1.));
#119380=DIRECTION('',(0.,-1.23467863058847E-16,1.));
#119381=DIRECTION('center_axis',(0.,0.,1.));
#119382=DIRECTION('ref_axis',(-0.0252625808996327,0.999680850074807,0.));
#119383=DIRECTION('',(-5.83684288299471E-35,1.23467863058847E-16,-1.));
#119384=DIRECTION('',(0.,-1.23467863058847E-16,1.));
#119385=DIRECTION('center_axis',(0.,0.,1.));
#119386=DIRECTION('ref_axis',(0.,-1.,0.));
#119387=DIRECTION('',(-3.52789515968553E-33,1.23467863058847E-16,-1.));
#119388=DIRECTION('',(0.,-1.23467863058847E-16,1.));
#119389=DIRECTION('center_axis',(0.,0.,1.));
#119390=DIRECTION('ref_axis',(0.,-1.,0.));
#119391=DIRECTION('',(0.,1.23467863058847E-16,-1.));
#119392=DIRECTION('',(1.21605822285869E-32,-1.23467863058847E-16,1.));
#119393=DIRECTION('center_axis',(0.,0.,-1.));
#119394=DIRECTION('ref_axis',(0.239106811829941,-0.970993271107746,0.));
#119395=DIRECTION('',(-6.62645671305077E-33,-1.23467863058847E-16,1.));
#119396=DIRECTION('',(0.,1.23467863058847E-16,-1.));
#119397=DIRECTION('center_axis',(0.,0.,-1.));
#119398=DIRECTION('ref_axis',(0.,1.,0.));
#119399=DIRECTION('',(0.,-1.23467863058847E-16,1.));
#119400=DIRECTION('',(-6.16297582203915E-33,1.23467863058847E-16,-1.));
#119401=DIRECTION('center_axis',(0.,1.23467863058847E-16,-1.));
#119402=DIRECTION('ref_axis',(0.,1.,0.));
#119403=DIRECTION('center_axis',(4.99759401346035E-30,-2.02287018699519E-43,
1.));
#119404=DIRECTION('ref_axis',(4.04768811061255E-14,1.,2.78791084448179E-58));
#119405=DIRECTION('center_axis',(-0.994416787801726,0.105523704152657,0.));
#119406=DIRECTION('ref_axis',(-0.105523704152657,-0.994416787801726,0.));
#119407=DIRECTION('center_axis',(0.,0.,-1.));
#119408=DIRECTION('ref_axis',(0.,1.,0.));
#119409=DIRECTION('center_axis',(0.,1.,0.));
#119410=DIRECTION('ref_axis',(0.,0.,1.));
#119411=DIRECTION('center_axis',(7.82779334765923E-17,1.,0.));
#119412=DIRECTION('ref_axis',(0.,0.,1.));
#119413=DIRECTION('center_axis',(0.,1.,0.));
#119414=DIRECTION('ref_axis',(0.,0.,1.));
#119415=DIRECTION('',(-7.82779334765923E-17,-1.,-1.23467863058847E-16));
#119416=DIRECTION('',(7.82779334765923E-17,1.,1.23467863058847E-16));
#119417=DIRECTION('center_axis',(0.,1.23467863058847E-16,-1.));
#119418=DIRECTION('ref_axis',(0.,1.,1.38375392967352E-16));
#119419=DIRECTION('center_axis',(-0.992522955047552,0.122058116090968,0.));
#119420=DIRECTION('ref_axis',(-0.122058116090968,-0.992522955047552,0.));
#119421=DIRECTION('center_axis',(0.,1.35726946151947E-16,-1.));
#119422=DIRECTION('ref_axis',(0.,1.,1.35726946151947E-16));
#119423=DIRECTION('center_axis',(6.16166569047948E-31,-1.35428930001789E-16,
1.));
#119424=DIRECTION('ref_axis',(-5.15143483426073E-14,1.,1.35428930001789E-16));
#119425=DIRECTION('center_axis',(0.,1.23467863058847E-16,-1.));
#119426=DIRECTION('ref_axis',(0.,1.,0.));
#119427=DIRECTION('center_axis',(-1.,0.,0.));
#119428=DIRECTION('ref_axis',(0.,0.,1.));
#119429=DIRECTION('center_axis',(0.,0.,1.));
#119430=DIRECTION('ref_axis',(0.,1.,0.));
#119431=DIRECTION('center_axis',(0.,0.,-1.));
#119432=DIRECTION('ref_axis',(0.,1.,0.));
#119433=DIRECTION('center_axis',(0.,1.23467863058847E-16,-1.));
#119434=DIRECTION('ref_axis',(0.,1.,0.));
#119435=DIRECTION('center_axis',(-0.848949186868299,0.528474481990998,0.));
#119436=DIRECTION('ref_axis',(-0.528474481990998,-0.848949186868299,0.));
#119437=DIRECTION('center_axis',(0.,0.,-1.));
#119438=DIRECTION('ref_axis',(0.,1.,0.));
#119439=DIRECTION('center_axis',(-2.06796993660427E-30,-3.463654065723E-44,
1.));
#119440=DIRECTION('ref_axis',(-1.67490542508106E-14,1.,-2.09093313336134E-58));
#119441=DIRECTION('center_axis',(1.,0.,-1.17757899099328E-32));
#119442=DIRECTION('ref_axis',(0.,1.,0.));
#119443=DIRECTION('center_axis',(-1.,0.,0.));
#119444=DIRECTION('ref_axis',(0.,0.,1.));
#119445=DIRECTION('',(1.,-9.53753439817791E-17,-1.17757899099328E-32));
#119446=DIRECTION('',(-1.,9.53753439817791E-17,1.17757899099328E-32));
#119447=DIRECTION('center_axis',(0.,1.23467863058847E-16,-1.));
#119448=DIRECTION('ref_axis',(0.,1.,0.));
#119449=DIRECTION('center_axis',(-0.787431540449703,0.616402116402116,0.));
#119450=DIRECTION('ref_axis',(-0.616402116402116,-0.787431540449703,0.));
#119451=DIRECTION('center_axis',(0.,0.,-1.));
#119452=DIRECTION('ref_axis',(0.,1.,0.));
#119453=DIRECTION('center_axis',(-7.6763044046751E-31,-4.77254954069701E-45,
1.));
#119454=DIRECTION('ref_axis',(-6.21724893790088E-15,1.,-1.86690458335834E-60));
#119455=DIRECTION('center_axis',(0.,1.23467863058847E-16,-1.));
#119456=DIRECTION('ref_axis',(0.,1.,0.));
#119457=DIRECTION('center_axis',(0.,-1.,0.));
#119458=DIRECTION('ref_axis',(0.,0.,-1.));
#119459=DIRECTION('center_axis',(0.,0.,1.));
#119460=DIRECTION('ref_axis',(0.,1.,0.));
#119461=DIRECTION('center_axis',(0.,0.,-1.));
#119462=DIRECTION('ref_axis',(0.,1.,0.));
#119463=DIRECTION('center_axis',(0.,1.23467863058847E-16,-1.));
#119464=DIRECTION('ref_axis',(0.,1.,0.));
#119465=DIRECTION('center_axis',(0.,1.,0.));
#119466=DIRECTION('ref_axis',(0.,0.,1.));
#119467=DIRECTION('center_axis',(0.,0.,-1.));
#119468=DIRECTION('ref_axis',(0.,1.,0.));
#119469=DIRECTION('center_axis',(-3.56971000961454E-31,-1.03207662601796E-45,
1.));
#119470=DIRECTION('ref_axis',(-2.89120579329468E-15,1.,-3.11150763893057E-61));
#119471=DIRECTION('center_axis',(0.,-1.,0.));
#119472=DIRECTION('ref_axis',(0.,0.,-1.));
#119473=DIRECTION('',(0.,-1.,-1.23467863058847E-16));
#119474=DIRECTION('',(0.,1.,1.23467863058847E-16));
#119475=DIRECTION('center_axis',(0.,1.23467863058847E-16,-1.));
#119476=DIRECTION('ref_axis',(0.,1.,0.));
#119477=DIRECTION('center_axis',(3.56971000961454E-30,-1.03207662601796E-43,
1.));
#119478=DIRECTION('ref_axis',(2.89120579329468E-14,1.,-3.98272977783113E-59));
#119479=DIRECTION('center_axis',(-0.998440322660918,0.0558294016156522,
0.));
#119480=DIRECTION('ref_axis',(-0.0558294016156522,-0.998440322660918,0.));
#119481=DIRECTION('center_axis',(0.,0.,-1.));
#119482=DIRECTION('ref_axis',(0.,1.,0.));
#119483=DIRECTION('center_axis',(0.,1.,0.));
#119484=DIRECTION('ref_axis',(0.,0.,1.));
#119485=DIRECTION('center_axis',(5.87084501074442E-17,1.,0.));
#119486=DIRECTION('ref_axis',(0.,0.,1.));
#119487=DIRECTION('center_axis',(0.,1.,0.));
#119488=DIRECTION('ref_axis',(0.,0.,1.));
#119489=DIRECTION('',(-5.87084501074442E-17,-1.,-1.23467863058847E-16));
#119490=DIRECTION('',(5.87084501074442E-17,1.,1.23467863058847E-16));
#119491=DIRECTION('center_axis',(0.,1.23467863058847E-16,-1.));
#119492=DIRECTION('ref_axis',(0.,1.,1.38375392967352E-16));
#119493=DIRECTION('center_axis',(-0.995642397459837,0.0932535059953692,
0.));
#119494=DIRECTION('ref_axis',(-0.0932535059953692,-0.995642397459837,0.));
#119495=DIRECTION('center_axis',(0.,1.35726946151947E-16,-1.));
#119496=DIRECTION('ref_axis',(0.,1.,1.35726946151947E-16));
#119497=DIRECTION('center_axis',(8.0739067668352E-31,-1.35428930001789E-16,
1.));
#119498=DIRECTION('ref_axis',(-6.75015598972095E-14,1.,1.35428930001789E-16));
#119499=DIRECTION('center_axis',(0.,1.23467863058847E-16,-1.));
#119500=DIRECTION('ref_axis',(0.,1.,0.));
#119501=DIRECTION('center_axis',(-1.,0.,0.));
#119502=DIRECTION('ref_axis',(0.,0.,1.));
#119503=DIRECTION('center_axis',(0.,0.,1.));
#119504=DIRECTION('ref_axis',(0.,1.,0.));
#119505=DIRECTION('center_axis',(0.,0.,-1.));
#119506=DIRECTION('ref_axis',(0.,1.,0.));
#119507=DIRECTION('center_axis',(0.,1.23467863058847E-16,-1.));
#119508=DIRECTION('ref_axis',(0.,1.,0.));
#119509=DIRECTION('center_axis',(0.,1.,0.));
#119510=DIRECTION('ref_axis',(0.,0.,1.));
#119511=DIRECTION('center_axis',(0.,0.,-1.));
#119512=DIRECTION('ref_axis',(0.,1.,0.));
#119513=DIRECTION('center_axis',(0.,0.,1.));
#119514=DIRECTION('ref_axis',(0.,1.,0.));
#119515=DIRECTION('center_axis',(1.,0.,-1.17757899099328E-32));
#119516=DIRECTION('ref_axis',(0.,1.,0.));
#119517=DIRECTION('center_axis',(-1.,0.,0.));
#119518=DIRECTION('ref_axis',(0.,0.,1.));
#119519=DIRECTION('',(1.,-9.53753439817791E-17,-1.17757899099328E-32));
#119520=DIRECTION('',(-1.,9.53753439817791E-17,1.17757899099328E-32));
#119521=DIRECTION('center_axis',(7.82779334765923E-17,-1.,0.));
#119522=DIRECTION('ref_axis',(0.,0.,-1.));
#119523=DIRECTION('center_axis',(0.,1.,0.));
#119524=DIRECTION('ref_axis',(0.,0.,1.));
#119525=DIRECTION('',(7.82779334765923E-17,-1.,-1.23467863058847E-16));
#119526=DIRECTION('',(-7.82779334765923E-17,1.,1.23467863058847E-16));
#119527=DIRECTION('center_axis',(0.,1.23467863058847E-16,-1.));
#119528=DIRECTION('ref_axis',(0.,1.,0.));
#119529=DIRECTION('center_axis',(0.,0.,-1.));
#119530=DIRECTION('ref_axis',(0.,1.,0.));
#119531=DIRECTION('center_axis',(0.,0.,1.));
#119532=DIRECTION('ref_axis',(0.,1.,0.));
#119533=DIRECTION('center_axis',(0.,1.23467863058847E-16,-1.));
#119534=DIRECTION('ref_axis',(0.,1.,0.));
#119535=DIRECTION('center_axis',(-6.13543907902499E-30,-3.04885917353938E-43,
1.));
#119536=DIRECTION('ref_axis',(-4.96925995722523E-14,1.,2.78791084448179E-58));
#119537=DIRECTION('center_axis',(-0.999981180102553,0.00613509907864248,
0.));
#119538=DIRECTION('ref_axis',(-0.00613509907864248,-0.999981180102553,0.));
#119539=DIRECTION('center_axis',(0.,0.,-1.));
#119540=DIRECTION('ref_axis',(0.,1.,0.));
#119541=DIRECTION('center_axis',(0.,1.,0.));
#119542=DIRECTION('ref_axis',(0.,0.,1.));
#119543=DIRECTION('center_axis',(6.11546355285877E-17,1.,0.));
#119544=DIRECTION('ref_axis',(0.,0.,1.));
#119545=DIRECTION('center_axis',(0.,1.,0.));
#119546=DIRECTION('ref_axis',(0.,0.,1.));
#119547=DIRECTION('',(-6.11546355285877E-17,-1.,-1.23467863058847E-16));
#119548=DIRECTION('',(6.11546355285877E-17,1.,1.23467863058847E-16));
#119549=DIRECTION('center_axis',(0.,1.23467863058847E-16,-1.));
#119550=DIRECTION('ref_axis',(0.,1.,1.38375392967352E-16));
#119551=DIRECTION('center_axis',(-0.999050847451757,0.0435592034583644,
0.));
#119552=DIRECTION('ref_axis',(-0.0435592034583644,-0.999050847451757,0.));
#119553=DIRECTION('center_axis',(0.,1.35726946151947E-16,-1.));
#119554=DIRECTION('ref_axis',(0.,1.,1.35726946151947E-16));
#119555=DIRECTION('center_axis',(-6.37413692118567E-32,-1.35428930001789E-16,
1.));
#119556=DIRECTION('ref_axis',(5.32907051820075E-15,1.,1.35428930001789E-16));
#119557=DIRECTION('center_axis',(0.,1.23467863058847E-16,-1.));
#119558=DIRECTION('ref_axis',(0.,1.,0.));
#119559=DIRECTION('center_axis',(-1.,0.,0.));
#119560=DIRECTION('ref_axis',(0.,0.,1.));
#119561=DIRECTION('center_axis',(0.,0.,1.));
#119562=DIRECTION('ref_axis',(0.,1.,0.));
#119563=DIRECTION('center_axis',(0.,0.,-1.));
#119564=DIRECTION('ref_axis',(0.,1.,0.));
#119565=DIRECTION('center_axis',(0.,1.23467863058847E-16,-1.));
#119566=DIRECTION('ref_axis',(0.,1.,0.));
#119567=DIRECTION('center_axis',(0.,1.,0.));
#119568=DIRECTION('ref_axis',(0.,0.,1.));
#119569=DIRECTION('center_axis',(0.,0.,-1.));
#119570=DIRECTION('ref_axis',(0.,1.,0.));
#119571=DIRECTION('center_axis',(-1.78485500480727E-31,-2.58019156504489E-46,
1.));
#119572=DIRECTION('ref_axis',(-1.44560289664734E-15,1.,-3.88938454866321E-62));
#119573=DIRECTION('center_axis',(1.,0.,-1.17757899099328E-32));
#119574=DIRECTION('ref_axis',(0.,1.,0.));
#119575=DIRECTION('center_axis',(-1.,0.,0.));
#119576=DIRECTION('ref_axis',(0.,0.,1.));
#119577=DIRECTION('',(1.,-9.53753439817791E-17,-1.17757899099328E-32));
#119578=DIRECTION('',(-1.,9.53753439817791E-17,1.17757899099328E-32));
#119579=DIRECTION('center_axis',(0.,-1.,-1.23467863058847E-16));
#119580=DIRECTION('ref_axis',(1.,0.,0.));
#119581=DIRECTION('center_axis',(0.,1.,0.));
#119582=DIRECTION('ref_axis',(0.,0.,1.));
#119583=DIRECTION('',(-3.13111733906369E-16,-1.,-1.23467863058847E-16));
#119584=DIRECTION('',(3.13111733906369E-16,1.,1.23467863058847E-16));
#119585=DIRECTION('center_axis',(0.,1.23467863058847E-16,-1.));
#119586=DIRECTION('ref_axis',(0.,1.,0.));
#119587=DIRECTION('center_axis',(0.,0.,-1.));
#119588=DIRECTION('ref_axis',(0.,1.,0.));
#119589=DIRECTION('center_axis',(0.,0.,1.));
#119590=DIRECTION('ref_axis',(0.,1.,0.));
#119591=DIRECTION('center_axis',(0.,1.23467863058847E-16,-1.));
#119592=DIRECTION('ref_axis',(0.,1.,0.));
#119593=DIRECTION('center_axis',(-1.,4.81867632215781E-16,0.));
#119594=DIRECTION('ref_axis',(-4.81867632215781E-16,-1.,0.));
#119595=DIRECTION('center_axis',(0.,0.,-1.));
#119596=DIRECTION('ref_axis',(0.,1.,0.));
#119597=DIRECTION('center_axis',(0.,1.,0.));
#119598=DIRECTION('ref_axis',(0.,0.,1.));
#119599=DIRECTION('center_axis',(0.,0.,1.));
#119600=DIRECTION('ref_axis',(0.,1.,0.));
#119601=DIRECTION('center_axis',(6.11546355285877E-17,1.,0.));
#119602=DIRECTION('ref_axis',(0.,0.,1.));
#119603=DIRECTION('center_axis',(0.,1.,0.));
#119604=DIRECTION('ref_axis',(0.,0.,1.));
#119605=DIRECTION('',(-6.11546355285877E-17,-1.,-1.23467863058847E-16));
#119606=DIRECTION('',(6.11546355285877E-17,1.,1.23467863058847E-16));
#119607=DIRECTION('center_axis',(-1.,0.,5.88789495496639E-32));
#119608=DIRECTION('ref_axis',(0.,-1.,0.));
#119609=DIRECTION('center_axis',(-1.,0.,0.));
#119610=DIRECTION('ref_axis',(0.,0.,1.));
#119611=DIRECTION('',(1.,-4.76876719908896E-16,-5.88789495496639E-32));
#119612=DIRECTION('',(-1.,4.76876719908896E-16,5.88789495496639E-32));
#119613=DIRECTION('center_axis',(0.,1.23467863058847E-16,-1.));
#119614=DIRECTION('ref_axis',(0.,1.,0.));
#119615=DIRECTION('center_axis',(-1.,0.,0.));
#119616=DIRECTION('ref_axis',(0.,0.,1.));
#119617=DIRECTION('center_axis',(0.,0.,1.));
#119618=DIRECTION('ref_axis',(0.,1.,0.));
#119619=DIRECTION('center_axis',(0.,0.,-1.));
#119620=DIRECTION('ref_axis',(0.,1.,0.));
#119621=DIRECTION('center_axis',(0.,1.23467863058847E-16,-1.));
#119622=DIRECTION('ref_axis',(0.,1.,0.));
#119623=DIRECTION('center_axis',(0.,1.,0.));
#119624=DIRECTION('ref_axis',(0.,0.,1.));
#119625=DIRECTION('center_axis',(0.,0.,-1.));
#119626=DIRECTION('ref_axis',(0.,1.,0.));
#119627=DIRECTION('center_axis',(0.,0.,1.));
#119628=DIRECTION('ref_axis',(0.,1.,0.));
#119629=DIRECTION('center_axis',(1.,0.,-1.5273745825629E-32));
#119630=DIRECTION('ref_axis',(0.,1.,0.));
#119631=DIRECTION('center_axis',(-1.,0.,0.));
#119632=DIRECTION('ref_axis',(0.,0.,1.));
#119633=DIRECTION('',(1.,-1.23706245878324E-16,-1.52737458256291E-32));
#119634=DIRECTION('',(-1.,1.23706245878324E-16,1.52737458256291E-32));
#119635=DIRECTION('center_axis',(0.,-1.,-1.23467863058847E-16));
#119636=DIRECTION('ref_axis',(1.,0.,0.));
#119637=DIRECTION('center_axis',(0.,1.,0.));
#119638=DIRECTION('ref_axis',(0.,0.,1.));
#119639=DIRECTION('',(-3.13111733906369E-16,-1.,-1.23467863058847E-16));
#119640=DIRECTION('',(3.13111733906369E-16,1.,1.23467863058847E-16));
#119641=DIRECTION('center_axis',(0.,1.23467863058847E-16,-1.));
#119642=DIRECTION('ref_axis',(0.,1.,0.));
#119643=DIRECTION('center_axis',(0.,0.,-1.));
#119644=DIRECTION('ref_axis',(0.,1.,0.));
#119645=DIRECTION('center_axis',(-1.78485500480727E-31,-2.58019156504489E-46,
1.));
#119646=DIRECTION('ref_axis',(-1.44560289664734E-15,1.,-3.88938454866321E-62));
#119647=DIRECTION('center_axis',(0.,1.23467863058847E-16,-1.));
#119648=DIRECTION('ref_axis',(0.,1.,0.));
#119649=DIRECTION('center_axis',(-1.,0.,0.));
#119650=DIRECTION('ref_axis',(0.,0.,1.));
#119651=DIRECTION('center_axis',(0.,0.,-1.));
#119652=DIRECTION('ref_axis',(0.,1.,0.));
#119653=DIRECTION('center_axis',(0.,1.,0.));
#119654=DIRECTION('ref_axis',(0.,0.,1.));
#119655=DIRECTION('center_axis',(0.,0.,1.));
#119656=DIRECTION('ref_axis',(0.,1.,0.));
#119657=DIRECTION('center_axis',(6.11546355285877E-17,1.,0.));
#119658=DIRECTION('ref_axis',(0.,0.,1.));
#119659=DIRECTION('center_axis',(0.,1.,0.));
#119660=DIRECTION('ref_axis',(0.,0.,1.));
#119661=DIRECTION('',(-6.11546355285877E-17,-1.,-1.23467863058847E-16));
#119662=DIRECTION('',(6.11546355285877E-17,1.,1.23467863058847E-16));
#119663=DIRECTION('center_axis',(-1.,0.,-1.5273745825629E-32));
#119664=DIRECTION('ref_axis',(0.,-1.,0.));
#119665=DIRECTION('center_axis',(-1.,0.,0.));
#119666=DIRECTION('ref_axis',(0.,0.,1.));
#119667=DIRECTION('',(1.,1.23706245878324E-16,1.52737458256291E-32));
#119668=DIRECTION('',(-1.,-1.23706245878324E-16,-1.52737458256291E-32));
#119669=DIRECTION('center_axis',(0.,1.23467863058847E-16,-1.));
#119670=DIRECTION('ref_axis',(0.,1.,0.));
#119671=DIRECTION('center_axis',(-0.995922166025996,0.0902166238455439,
0.));
#119672=DIRECTION('ref_axis',(-0.0902166238455439,-0.995922166025996,0.));
#119673=DIRECTION('center_axis',(1.11553437800454E-31,-1.00788733009566E-46,
1.));
#119674=DIRECTION('ref_axis',(9.03501810404587E-16,1.,1.55575381946529E-61));
#119675=DIRECTION('center_axis',(0.,0.,-1.));
#119676=DIRECTION('ref_axis',(0.,1.,0.));
#119677=DIRECTION('center_axis',(0.,1.23467863058847E-16,-1.));
#119678=DIRECTION('ref_axis',(0.,1.,0.));
#119679=DIRECTION('center_axis',(0.,1.,0.));
#119680=DIRECTION('ref_axis',(0.,0.,1.));
#119681=DIRECTION('center_axis',(0.,0.,-1.));
#119682=DIRECTION('ref_axis',(0.,1.,0.));
#119683=DIRECTION('center_axis',(1.78485500480727E-31,-2.58019156504489E-46,
1.));
#119684=DIRECTION('ref_axis',(1.44560289664734E-15,1.,-3.88938454866321E-62));
#119685=DIRECTION('center_axis',(0.,1.23467863058847E-16,-1.));
#119686=DIRECTION('ref_axis',(0.,1.,0.));
#119687=DIRECTION('center_axis',(-0.913440670994017,0.406971916198157,3.63370493544251E-16));
#119688=DIRECTION('ref_axis',(-0.406971916198157,-0.913440670994017,6.94755181634254E-32));
#119689=DIRECTION('center_axis',(0.,0.,-1.));
#119690=DIRECTION('ref_axis',(0.,1.,0.));
#119691=DIRECTION('center_axis',(-5.48307457476793E-31,-2.43497425545765E-45,
1.));
#119692=DIRECTION('ref_axis',(-4.44089209850063E-15,1.,-3.42265840282363E-60));
#119693=DIRECTION('center_axis',(0.,-1.,-1.23467863058847E-16));
#119694=DIRECTION('ref_axis',(1.,0.,0.));
#119695=DIRECTION('center_axis',(3.61400724161834E-16,1.,1.20466908053943E-16));
#119696=DIRECTION('ref_axis',(-1.,3.61400724161834E-16,-2.73691106313441E-47));
#119697=DIRECTION('',(-3.13111733906369E-16,-1.,-1.23467863058847E-16));
#119698=DIRECTION('',(3.13111733906369E-16,1.,1.23467863058847E-16));
#119699=DIRECTION('center_axis',(0.,1.23467863058847E-16,-1.));
#119700=DIRECTION('ref_axis',(0.,1.,0.));
#119701=DIRECTION('center_axis',(-0.99836765577839,0.0571141304368959,-4.12821761995348E-17));
#119702=DIRECTION('ref_axis',(-0.0571141304368959,-0.99836765577839,1.08996476499831E-33));
#119703=DIRECTION('center_axis',(0.,0.,1.));
#119704=DIRECTION('ref_axis',(0.,1.,0.));
#119705=DIRECTION('center_axis',(0.,0.,-1.));
#119706=DIRECTION('ref_axis',(0.,1.,0.));
#119707=DIRECTION('center_axis',(0.,1.23467863058847E-16,-1.));
#119708=DIRECTION('ref_axis',(0.686617021913638,-0.727019301819729,0.));
#119709=DIRECTION('center_axis',(-1.78485500480727E-31,-2.58019156504489E-46,
1.));
#119710=DIRECTION('ref_axis',(-1.44560289664734E-15,1.,0.));
#119711=DIRECTION('center_axis',(0.,0.,-1.));
#119712=DIRECTION('ref_axis',(0.,1.,0.));
#119713=DIRECTION('center_axis',(0.,1.23467863058847E-16,-1.));
#119714=DIRECTION('ref_axis',(0.,1.,0.));
#119715=DIRECTION('center_axis',(-1.,0.,0.));
#119716=DIRECTION('ref_axis',(0.,0.,1.));
#119717=DIRECTION('center_axis',(0.,0.,-1.));
#119718=DIRECTION('ref_axis',(0.,1.,0.));
#119719=DIRECTION('center_axis',(0.,1.,0.));
#119720=DIRECTION('ref_axis',(0.,0.,1.));
#119721=DIRECTION('center_axis',(0.,0.,1.));
#119722=DIRECTION('ref_axis',(0.,1.,0.));
#119723=DIRECTION('center_axis',(5.87084501074442E-17,1.,0.));
#119724=DIRECTION('ref_axis',(0.,0.,1.));
#119725=DIRECTION('center_axis',(4.81867632215779E-16,1.,1.20466908053945E-16));
#119726=DIRECTION('ref_axis',(-1.,4.81867632215779E-16,1.09476442525376E-47));
#119727=DIRECTION('',(-5.87084501074442E-17,-1.,-1.23467863058847E-16));
#119728=DIRECTION('',(5.87084501074442E-17,1.,1.23467863058847E-16));
#119729=DIRECTION('center_axis',(-1.,0.,-1.5273745825629E-32));
#119730=DIRECTION('ref_axis',(0.,-1.,0.));
#119731=DIRECTION('center_axis',(-1.,0.,0.));
#119732=DIRECTION('ref_axis',(0.,0.,1.));
#119733=DIRECTION('',(1.,1.23706245878324E-16,1.52737458256291E-32));
#119734=DIRECTION('',(-1.,-1.23706245878324E-16,-1.52737458256291E-32));
#119735=DIRECTION('center_axis',(0.,1.23467863058847E-16,-1.));
#119736=DIRECTION('ref_axis',(0.,1.,0.));
#119737=DIRECTION('center_axis',(-1.,0.,0.));
#119738=DIRECTION('ref_axis',(0.,0.,1.));
#119739=DIRECTION('center_axis',(0.,0.,1.));
#119740=DIRECTION('ref_axis',(0.,1.,0.));
#119741=DIRECTION('center_axis',(0.,0.,-1.));
#119742=DIRECTION('ref_axis',(0.,1.,0.));
#119743=DIRECTION('center_axis',(0.,1.23467863058847E-16,-1.));
#119744=DIRECTION('ref_axis',(0.,1.,0.));
#119745=DIRECTION('center_axis',(0.,1.,0.));
#119746=DIRECTION('ref_axis',(0.,0.,1.));
#119747=DIRECTION('center_axis',(0.,0.,-1.));
#119748=DIRECTION('ref_axis',(0.,1.,0.));
#119749=DIRECTION('center_axis',(3.56971000961454E-31,-1.03207662601796E-45,
1.));
#119750=DIRECTION('ref_axis',(2.89120579329468E-15,1.,-3.11150763893057E-61));
#119751=DIRECTION('center_axis',(1.,0.,4.58212374768871E-32));
#119752=DIRECTION('ref_axis',(0.,1.,0.));
#119753=DIRECTION('center_axis',(-1.,0.,0.));
#119754=DIRECTION('ref_axis',(0.,0.,1.));
#119755=DIRECTION('',(1.,3.71118737634973E-16,4.58212374768871E-32));
#119756=DIRECTION('',(-1.,-3.71118737634973E-16,-4.58212374768871E-32));
#119757=DIRECTION('center_axis',(7.82779334765923E-17,-1.,0.));
#119758=DIRECTION('ref_axis',(0.,0.,-1.));
#119759=DIRECTION('center_axis',(-1.20466908053945E-16,1.,1.20466908053943E-16));
#119760=DIRECTION('ref_axis',(-1.,-1.20466908053945E-16,2.73691106313441E-48));
#119761=DIRECTION('',(7.82779334765923E-17,-1.,-1.23467863058847E-16));
#119762=DIRECTION('',(-7.82779334765923E-17,1.,1.23467863058847E-16));
#119763=DIRECTION('center_axis',(0.,1.23467863058847E-16,-1.));
#119764=DIRECTION('ref_axis',(0.,1.,0.));
#119765=DIRECTION('center_axis',(0.,0.,-1.));
#119766=DIRECTION('ref_axis',(0.,1.,0.));
#119767=DIRECTION('center_axis',(0.,0.,1.));
#119768=DIRECTION('ref_axis',(0.,1.,0.));
#119769=DIRECTION('center_axis',(0.,1.23467863058847E-16,-1.));
#119770=DIRECTION('ref_axis',(0.,1.,0.));
#119771=DIRECTION('center_axis',(-1.,0.,0.));
#119772=DIRECTION('ref_axis',(0.,0.,1.));
#119773=DIRECTION('center_axis',(0.,0.,-1.));
#119774=DIRECTION('ref_axis',(0.,1.,0.));
#119775=DIRECTION('center_axis',(0.,1.,0.));
#119776=DIRECTION('ref_axis',(0.,0.,1.));
#119777=DIRECTION('center_axis',(0.,0.,1.));
#119778=DIRECTION('ref_axis',(0.,1.,0.));
#119779=DIRECTION('center_axis',(5.87084501074442E-17,1.,0.));
#119780=DIRECTION('ref_axis',(0.,0.,1.));
#119781=DIRECTION('center_axis',(0.,1.,0.));
#119782=DIRECTION('ref_axis',(0.,0.,1.));
#119783=DIRECTION('',(-5.87084501074442E-17,-1.,-1.23467863058847E-16));
#119784=DIRECTION('',(5.87084501074442E-17,1.,1.23467863058847E-16));
#119785=DIRECTION('center_axis',(-1.,0.,5.88789495496639E-32));
#119786=DIRECTION('ref_axis',(0.,-1.,0.));
#119787=DIRECTION('center_axis',(-1.,0.,0.));
#119788=DIRECTION('ref_axis',(0.,0.,1.));
#119789=DIRECTION('',(1.,-4.76876719908896E-16,-5.88789495496639E-32));
#119790=DIRECTION('',(-1.,4.76876719908896E-16,5.88789495496639E-32));
#119791=DIRECTION('center_axis',(0.,1.23467863058847E-16,-1.));
#119792=DIRECTION('ref_axis',(0.,1.,0.));
#119793=DIRECTION('center_axis',(-1.,0.,0.));
#119794=DIRECTION('ref_axis',(0.,0.,1.));
#119795=DIRECTION('center_axis',(1.78485500480727E-31,-2.58019156504489E-46,
1.));
#119796=DIRECTION('ref_axis',(1.44560289664734E-15,1.,-3.88938454866321E-62));
#119797=DIRECTION('center_axis',(0.,0.,-1.));
#119798=DIRECTION('ref_axis',(0.,1.,0.));
#119799=DIRECTION('center_axis',(0.,1.23467863058847E-16,-1.));
#119800=DIRECTION('ref_axis',(0.,1.,0.));
#119801=DIRECTION('center_axis',(0.,1.,0.));
#119802=DIRECTION('ref_axis',(0.,0.,1.));
#119803=DIRECTION('center_axis',(0.,0.,-1.));
#119804=DIRECTION('ref_axis',(0.,1.,0.));
#119805=DIRECTION('center_axis',(0.,0.,1.));
#119806=DIRECTION('ref_axis',(0.,1.,0.));
#119807=DIRECTION('center_axis',(1.,0.,-1.5273745825629E-32));
#119808=DIRECTION('ref_axis',(0.,1.,0.));
#119809=DIRECTION('center_axis',(-1.,0.,0.));
#119810=DIRECTION('ref_axis',(0.,0.,1.));
#119811=DIRECTION('',(1.,-1.23706245878324E-16,-1.52737458256291E-32));
#119812=DIRECTION('',(-1.,1.23706245878324E-16,1.52737458256291E-32));
#119813=DIRECTION('center_axis',(7.82779334765923E-17,-1.,0.));
#119814=DIRECTION('ref_axis',(0.,0.,-1.));
#119815=DIRECTION('center_axis',(0.,1.,0.));
#119816=DIRECTION('ref_axis',(0.,0.,1.));
#119817=DIRECTION('',(7.82779334765923E-17,-1.,-1.23467863058847E-16));
#119818=DIRECTION('',(-7.82779334765923E-17,1.,1.23467863058847E-16));
#119819=DIRECTION('center_axis',(0.,1.23467863058847E-16,-1.));
#119820=DIRECTION('ref_axis',(0.,1.,0.));
#119821=DIRECTION('center_axis',(0.,0.,-1.));
#119822=DIRECTION('ref_axis',(0.,1.,0.));
#119823=DIRECTION('center_axis',(0.,0.,1.));
#119824=DIRECTION('ref_axis',(0.,1.,0.));
#119825=DIRECTION('center_axis',(0.,1.23467863058847E-16,-1.));
#119826=DIRECTION('ref_axis',(0.,1.,0.));
#119827=DIRECTION('center_axis',(-1.,0.,0.));
#119828=DIRECTION('ref_axis',(0.,0.,1.));
#119829=DIRECTION('center_axis',(0.,0.,-1.));
#119830=DIRECTION('ref_axis',(0.,1.,0.));
#119831=DIRECTION('center_axis',(0.,1.,0.));
#119832=DIRECTION('ref_axis',(0.,0.,1.));
#119833=DIRECTION('center_axis',(0.,0.,1.));
#119834=DIRECTION('ref_axis',(0.,1.,0.));
#119835=DIRECTION('center_axis',(7.82779334765923E-17,1.,0.));
#119836=DIRECTION('ref_axis',(0.,0.,1.));
#119837=DIRECTION('center_axis',(0.,1.,0.));
#119838=DIRECTION('ref_axis',(0.,0.,1.));
#119839=DIRECTION('',(-7.82779334765923E-17,-1.,-1.23467863058847E-16));
#119840=DIRECTION('',(7.82779334765923E-17,1.,1.23467863058847E-16));
#119841=DIRECTION('center_axis',(-1.,0.,5.88789495496639E-32));
#119842=DIRECTION('ref_axis',(0.,-1.,0.));
#119843=DIRECTION('center_axis',(-1.,0.,0.));
#119844=DIRECTION('ref_axis',(0.,0.,1.));
#119845=DIRECTION('',(1.,-4.76876719908896E-16,-5.88789495496639E-32));
#119846=DIRECTION('',(-1.,4.76876719908896E-16,5.88789495496639E-32));
#119847=DIRECTION('center_axis',(0.,1.23467863058847E-16,-1.));
#119848=DIRECTION('ref_axis',(0.,1.,0.));
#119849=DIRECTION('center_axis',(-1.,0.,0.));
#119850=DIRECTION('ref_axis',(0.,0.,1.));
#119851=DIRECTION('center_axis',(0.,0.,1.));
#119852=DIRECTION('ref_axis',(0.,1.,0.));
#119853=DIRECTION('center_axis',(0.,0.,-1.));
#119854=DIRECTION('ref_axis',(0.,1.,0.));
#119855=DIRECTION('center_axis',(0.,1.23467863058847E-16,-1.));
#119856=DIRECTION('ref_axis',(0.,1.,0.));
#119857=DIRECTION('center_axis',(0.,1.,0.));
#119858=DIRECTION('ref_axis',(0.,0.,1.));
#119859=DIRECTION('center_axis',(0.,0.,-1.));
#119860=DIRECTION('ref_axis',(0.,1.,0.));
#119861=DIRECTION('center_axis',(0.,0.,1.));
#119862=DIRECTION('ref_axis',(0.,1.,0.));
#119863=DIRECTION('center_axis',(1.,0.,-1.5273745825629E-32));
#119864=DIRECTION('ref_axis',(0.,1.,0.));
#119865=DIRECTION('center_axis',(-1.,0.,0.));
#119866=DIRECTION('ref_axis',(0.,0.,1.));
#119867=DIRECTION('',(1.,-1.23706245878324E-16,-1.52737458256291E-32));
#119868=DIRECTION('',(-1.,1.23706245878324E-16,1.52737458256291E-32));
#119869=DIRECTION('center_axis',(0.,-1.,0.));
#119870=DIRECTION('ref_axis',(0.,0.,-1.));
#119871=DIRECTION('center_axis',(0.,1.,0.));
#119872=DIRECTION('ref_axis',(0.,0.,1.));
#119873=DIRECTION('',(0.,-1.,-1.23467863058847E-16));
#119874=DIRECTION('',(0.,1.,1.23467863058847E-16));
#119875=DIRECTION('center_axis',(0.,1.23467863058847E-16,-1.));
#119876=DIRECTION('ref_axis',(0.,1.,0.));
#119877=DIRECTION('center_axis',(0.,0.,-1.));
#119878=DIRECTION('ref_axis',(0.,1.,0.));
#119879=DIRECTION('center_axis',(0.,0.,1.));
#119880=DIRECTION('ref_axis',(0.,1.,0.));
#119881=DIRECTION('center_axis',(0.,1.23467863058847E-16,-1.));
#119882=DIRECTION('ref_axis',(0.,1.,0.));
#119883=DIRECTION('center_axis',(-1.,0.,0.));
#119884=DIRECTION('ref_axis',(0.,0.,1.));
#119885=DIRECTION('center_axis',(0.,0.,-1.));
#119886=DIRECTION('ref_axis',(0.,1.,0.));
#119887=DIRECTION('center_axis',(0.,1.,0.));
#119888=DIRECTION('ref_axis',(0.,0.,1.));
#119889=DIRECTION('center_axis',(0.,0.,1.));
#119890=DIRECTION('ref_axis',(0.,1.,0.));
#119891=DIRECTION('center_axis',(7.82779334765923E-17,1.,0.));
#119892=DIRECTION('ref_axis',(0.,0.,1.));
#119893=DIRECTION('center_axis',(-4.57774250604992E-15,1.,1.20466908053943E-16));
#119894=DIRECTION('ref_axis',(-1.,-4.57774250604992E-15,-3.50324616081204E-46));
#119895=DIRECTION('',(-7.82779334765923E-17,-1.,-1.23467863058847E-16));
#119896=DIRECTION('',(7.82779334765923E-17,1.,1.23467863058847E-16));
#119897=DIRECTION('center_axis',(-1.,0.,-1.5273745825629E-32));
#119898=DIRECTION('ref_axis',(0.,-1.,0.));
#119899=DIRECTION('center_axis',(-1.,0.,0.));
#119900=DIRECTION('ref_axis',(0.,0.,1.));
#119901=DIRECTION('',(1.,1.23706245878324E-16,1.52737458256291E-32));
#119902=DIRECTION('',(-1.,-1.23706245878324E-16,-1.52737458256291E-32));
#119903=DIRECTION('center_axis',(0.,1.23467863058847E-16,-1.));
#119904=DIRECTION('ref_axis',(0.,1.,0.));
#119905=DIRECTION('center_axis',(-1.,0.,0.));
#119906=DIRECTION('ref_axis',(0.,0.,1.));
#119907=DIRECTION('center_axis',(0.,0.,1.));
#119908=DIRECTION('ref_axis',(0.,1.,0.));
#119909=DIRECTION('center_axis',(0.,0.,-1.));
#119910=DIRECTION('ref_axis',(0.,1.,0.));
#119911=DIRECTION('center_axis',(0.,1.23467863058847E-16,-1.));
#119912=DIRECTION('ref_axis',(0.,1.,0.));
#119913=DIRECTION('center_axis',(0.,1.,0.));
#119914=DIRECTION('ref_axis',(0.,0.,1.));
#119915=DIRECTION('center_axis',(0.,0.,-1.));
#119916=DIRECTION('ref_axis',(0.,1.,0.));
#119917=DIRECTION('center_axis',(0.,0.,1.));
#119918=DIRECTION('ref_axis',(0.,1.,0.));
#119919=DIRECTION('center_axis',(1.,0.,4.58212374768871E-32));
#119920=DIRECTION('ref_axis',(0.,1.,0.));
#119921=DIRECTION('center_axis',(-1.,0.,0.));
#119922=DIRECTION('ref_axis',(0.,0.,1.));
#119923=DIRECTION('',(1.,3.71118737634973E-16,4.58212374768871E-32));
#119924=DIRECTION('',(-1.,-3.71118737634973E-16,-4.58212374768871E-32));
#119925=DIRECTION('center_axis',(0.,-1.,0.));
#119926=DIRECTION('ref_axis',(0.,0.,-1.));
#119927=DIRECTION('center_axis',(0.,1.,1.20466908053943E-16));
#119928=DIRECTION('ref_axis',(0.,-1.20466908053943E-16,1.));
#119929=DIRECTION('',(0.,-1.,-1.23467863058847E-16));
#119930=DIRECTION('',(0.,1.,1.23467863058847E-16));
#119931=DIRECTION('center_axis',(0.,1.23467863058847E-16,-1.));
#119932=DIRECTION('ref_axis',(0.,1.,0.));
#119933=DIRECTION('center_axis',(0.,0.,-1.));
#119934=DIRECTION('ref_axis',(0.,1.,0.));
#119935=DIRECTION('center_axis',(0.,0.,1.));
#119936=DIRECTION('ref_axis',(0.,1.,0.));
#119937=DIRECTION('center_axis',(0.,1.23467863058847E-16,-1.));
#119938=DIRECTION('ref_axis',(0.,1.,0.));
#119939=DIRECTION('center_axis',(-1.,0.,0.));
#119940=DIRECTION('ref_axis',(0.,0.,1.));
#119941=DIRECTION('center_axis',(0.,0.,-1.));
#119942=DIRECTION('ref_axis',(0.,1.,0.));
#119943=DIRECTION('center_axis',(0.,1.,0.));
#119944=DIRECTION('ref_axis',(0.,0.,1.));
#119945=DIRECTION('center_axis',(0.,0.,1.));
#119946=DIRECTION('ref_axis',(0.,1.,0.));
#119947=DIRECTION('center_axis',(0.,1.,0.));
#119948=DIRECTION('ref_axis',(0.,0.,1.));
#119949=DIRECTION('center_axis',(-3.61400724161836E-16,1.,1.20466908053943E-16));
#119950=DIRECTION('ref_axis',(-1.,-3.61400724161836E-16,1.09476442525376E-47));
#119951=DIRECTION('',(0.,-1.,-1.23467863058847E-16));
#119952=DIRECTION('',(0.,1.,1.23467863058847E-16));
#119953=DIRECTION('center_axis',(-1.,0.,-1.5273745825629E-32));
#119954=DIRECTION('ref_axis',(0.,-1.,0.));
#119955=DIRECTION('center_axis',(-1.,0.,0.));
#119956=DIRECTION('ref_axis',(0.,0.,1.));
#119957=DIRECTION('',(1.,1.23706245878324E-16,1.52737458256291E-32));
#119958=DIRECTION('',(-1.,-1.23706245878324E-16,-1.52737458256291E-32));
#119959=DIRECTION('center_axis',(0.,1.23467863058847E-16,-1.));
#119960=DIRECTION('ref_axis',(0.,1.,0.));
#119961=DIRECTION('center_axis',(-1.,0.,0.));
#119962=DIRECTION('ref_axis',(0.,0.,1.));
#119963=DIRECTION('center_axis',(0.,0.,1.));
#119964=DIRECTION('ref_axis',(0.,1.,0.));
#119965=DIRECTION('center_axis',(0.,0.,-1.));
#119966=DIRECTION('ref_axis',(0.,1.,0.));
#119967=DIRECTION('center_axis',(0.,1.23467863058847E-16,-1.));
#119968=DIRECTION('ref_axis',(0.,1.,0.));
#119969=DIRECTION('center_axis',(-0.0294983404866172,0.999564829267485,
0.));
#119970=DIRECTION('ref_axis',(-0.999564829267485,-0.0294983404866172,0.));
#119971=DIRECTION('center_axis',(0.,0.,-1.));
#119972=DIRECTION('ref_axis',(0.,1.,0.));
#119973=DIRECTION('center_axis',(0.,0.,1.));
#119974=DIRECTION('ref_axis',(0.,1.,0.));
#119975=DIRECTION('center_axis',(1.,0.,4.58212374768871E-32));
#119976=DIRECTION('ref_axis',(0.,1.,0.));
#119977=DIRECTION('center_axis',(-1.,0.,0.));
#119978=DIRECTION('ref_axis',(0.,0.,1.));
#119979=DIRECTION('',(1.,3.71118737634973E-16,4.58212374768871E-32));
#119980=DIRECTION('',(-1.,-3.71118737634973E-16,-4.58212374768871E-32));
#119981=DIRECTION('center_axis',(0.,1.23467863058847E-16,-1.));
#119982=DIRECTION('ref_axis',(0.,1.,1.25697703075927E-16));
#119983=DIRECTION('center_axis',(-0.0175200318846342,0.999846512462169,
1.20448417884836E-16));
#119984=DIRECTION('ref_axis',(-0.999846512462169,-0.0175200318846342,1.51017636338582E-32));
#119985=DIRECTION('center_axis',(0.,1.22914743790472E-16,-1.));
#119986=DIRECTION('ref_axis',(0.,1.,1.22914743790472E-16));
#119987=DIRECTION('center_axis',(1.11644282221188E-31,-1.22833149346405E-16,
1.));
#119988=DIRECTION('ref_axis',(1.75897069864052E-13,1.,1.22833149346405E-16));
#119989=DIRECTION('center_axis',(0.,1.23467863058847E-16,-1.));
#119990=DIRECTION('ref_axis',(0.,1.,0.));
#119991=DIRECTION('center_axis',(0.,0.,-1.));
#119992=DIRECTION('ref_axis',(0.,1.,0.));
#119993=DIRECTION('center_axis',(0.,0.,1.));
#119994=DIRECTION('ref_axis',(0.,1.,0.));
#119995=DIRECTION('center_axis',(0.,1.23467863058847E-16,-1.));
#119996=DIRECTION('ref_axis',(0.,1.,0.));
#119997=DIRECTION('center_axis',(-1.,0.,0.));
#119998=DIRECTION('ref_axis',(0.,0.,1.));
#119999=DIRECTION('center_axis',(0.,0.,-1.));
#120000=DIRECTION('ref_axis',(0.,1.,0.));
#120001=DIRECTION('center_axis',(0.,1.,0.));
#120002=DIRECTION('ref_axis',(0.,0.,1.));
#120003=DIRECTION('center_axis',(0.,0.,1.));
#120004=DIRECTION('ref_axis',(0.,1.,0.));
#120005=DIRECTION('center_axis',(0.,1.,0.));
#120006=DIRECTION('ref_axis',(0.,0.,1.));
#120007=DIRECTION('center_axis',(0.,1.,0.));
#120008=DIRECTION('ref_axis',(0.,0.,1.));
#120009=DIRECTION('',(0.,-1.,-1.23467863058847E-16));
#120010=DIRECTION('',(0.,1.,1.23467863058847E-16));
#120011=DIRECTION('center_axis',(-1.,0.,5.88789495496639E-32));
#120012=DIRECTION('ref_axis',(0.,-1.,0.));
#120013=DIRECTION('center_axis',(-1.,0.,0.));
#120014=DIRECTION('ref_axis',(0.,0.,1.));
#120015=DIRECTION('',(1.,-4.76876719908896E-16,-5.88789495496639E-32));
#120016=DIRECTION('',(-1.,4.76876719908896E-16,5.88789495496639E-32));
#120017=DIRECTION('center_axis',(0.,1.23467863058847E-16,-1.));
#120018=DIRECTION('ref_axis',(0.,1.,0.));
#120019=DIRECTION('center_axis',(-1.,0.,0.));
#120020=DIRECTION('ref_axis',(0.,0.,1.));
#120021=DIRECTION('center_axis',(0.,0.,1.));
#120022=DIRECTION('ref_axis',(0.,1.,0.));
#120023=DIRECTION('center_axis',(0.,0.,-1.));
#120024=DIRECTION('ref_axis',(0.,1.,0.));
#120025=DIRECTION('center_axis',(0.,1.23467863058847E-16,-1.));
#120026=DIRECTION('ref_axis',(0.,1.,0.));
#120027=DIRECTION('center_axis',(-0.646912564190485,0.762564183719962,0.));
#120028=DIRECTION('ref_axis',(-0.762564183719962,-0.646912564190485,0.));
#120029=DIRECTION('center_axis',(0.,0.,-1.));
#120030=DIRECTION('ref_axis',(0.,1.,0.));
#120031=DIRECTION('center_axis',(0.,0.,1.));
#120032=DIRECTION('ref_axis',(0.,1.,0.));
#120033=DIRECTION('center_axis',(1.,0.,-1.5273745825629E-32));
#120034=DIRECTION('ref_axis',(0.,1.,0.));
#120035=DIRECTION('center_axis',(-1.,0.,0.));
#120036=DIRECTION('ref_axis',(0.,0.,1.));
#120037=DIRECTION('',(1.,-1.23706245878324E-16,-1.52737458256291E-32));
#120038=DIRECTION('',(-1.,1.23706245878324E-16,1.52737458256291E-32));
#120039=DIRECTION('center_axis',(0.,1.23467863058847E-16,-1.));
#120040=DIRECTION('ref_axis',(0.,1.,0.));
#120041=DIRECTION('center_axis',(-0.55837318130784,0.829589892896582,0.));
#120042=DIRECTION('ref_axis',(-0.829589892896582,-0.55837318130784,0.));
#120043=DIRECTION('center_axis',(0.,0.,-1.));
#120044=DIRECTION('ref_axis',(0.,1.,0.));
#120045=DIRECTION('center_axis',(-6.57968948972152E-31,-3.50636292785903E-45,
1.));
#120046=DIRECTION('ref_axis',(-5.32907051820075E-15,1.,0.));
#120047=DIRECTION('center_axis',(0.,1.23467863058847E-16,-1.));
#120048=DIRECTION('ref_axis',(0.,1.,0.));
#120049=DIRECTION('center_axis',(0.0331928226750539,-0.999448966442441,
0.));
#120050=DIRECTION('ref_axis',(0.99944896644244,0.0331928226750539,0.));
#120051=DIRECTION('center_axis',(0.,0.,1.));
#120052=DIRECTION('ref_axis',(0.,1.,0.));
#120053=DIRECTION('center_axis',(0.,0.,-1.));
#120054=DIRECTION('ref_axis',(0.,1.,0.));
#120055=DIRECTION('center_axis',(0.,1.23467863058847E-16,-1.));
#120056=DIRECTION('ref_axis',(0.,1.,0.));
#120057=DIRECTION('center_axis',(-0.03879684915621,0.999247118832749,0.));
#120058=DIRECTION('ref_axis',(-0.999247118832749,-0.03879684915621,0.));
#120059=DIRECTION('center_axis',(0.,0.,-1.));
#120060=DIRECTION('ref_axis',(0.,1.,0.));
#120061=DIRECTION('center_axis',(-1.18169710663102E-30,-1.13098908268507E-44,
1.));
#120062=DIRECTION('ref_axis',(-9.57088814332033E-15,1.,-2.7381267222589E-59));
#120063=DIRECTION('center_axis',(0.,1.23467863058847E-16,-1.));
#120064=DIRECTION('ref_axis',(0.,1.,1.25697703075927E-16));
#120065=DIRECTION('center_axis',(0.,1.22914743790472E-16,-1.));
#120066=DIRECTION('ref_axis',(0.,1.,1.22914743790472E-16));
#120067=DIRECTION('center_axis',(1.18920911416235E-31,-1.22833149346405E-16,
1.));
#120068=DIRECTION('ref_axis',(1.87361497136383E-13,1.,1.22833149346405E-16));
#120069=DIRECTION('center_axis',(0.,1.23467863058847E-16,-1.));
#120070=DIRECTION('ref_axis',(0.,1.,0.));
#120071=DIRECTION('center_axis',(-1.,0.,0.));
#120072=DIRECTION('ref_axis',(0.,0.,1.));
#120073=DIRECTION('center_axis',(0.,0.,-1.));
#120074=DIRECTION('ref_axis',(0.,1.,0.));
#120075=DIRECTION('center_axis',(0.,1.,9.63735264431547E-16));
#120076=DIRECTION('ref_axis',(0.,-9.63735264431547E-16,1.));
#120077=DIRECTION('center_axis',(0.,0.,1.));
#120078=DIRECTION('ref_axis',(0.,1.,0.));
#120079=DIRECTION('center_axis',(0.,1.,0.));
#120080=DIRECTION('ref_axis',(0.,0.,1.));
#120081=DIRECTION('center_axis',(-3.85494105772624E-15,1.,0.));
#120082=DIRECTION('ref_axis',(-1.,-3.85494105772625E-15,0.));
#120083=DIRECTION('',(0.,-1.,-1.23467863058847E-16));
#120084=DIRECTION('',(0.,1.,1.23467863058847E-16));
#120085=DIRECTION('center_axis',(-1.,0.,4.58212374768871E-32));
#120086=DIRECTION('ref_axis',(0.,-1.,0.));
#120087=DIRECTION('center_axis',(-1.,0.,0.));
#120088=DIRECTION('ref_axis',(0.,0.,1.));
#120089=DIRECTION('',(1.,-3.71118737634973E-16,-4.58212374768871E-32));
#120090=DIRECTION('',(-1.,3.71118737634973E-16,4.58212374768871E-32));
#120091=DIRECTION('center_axis',(0.,1.23467863058847E-16,-1.));
#120092=DIRECTION('ref_axis',(0.,1.,0.));
#120093=DIRECTION('center_axis',(-1.,0.,0.));
#120094=DIRECTION('ref_axis',(0.,0.,1.));
#120095=DIRECTION('center_axis',(0.,0.,1.));
#120096=DIRECTION('ref_axis',(0.,1.,0.));
#120097=DIRECTION('center_axis',(0.,0.,-1.));
#120098=DIRECTION('ref_axis',(0.,1.,0.));
#120099=DIRECTION('center_axis',(0.,1.23467863058847E-16,-1.));
#120100=DIRECTION('ref_axis',(0.,1.,0.));
#120101=DIRECTION('center_axis',(-0.0138255496962061,0.999904422520272,
0.));
#120102=DIRECTION('ref_axis',(-0.999904422520272,-0.0138255496962061,0.));
#120103=DIRECTION('center_axis',(0.,0.,-1.));
#120104=DIRECTION('ref_axis',(0.,1.,0.));
#120105=DIRECTION('center_axis',(0.,0.,1.));
#120106=DIRECTION('ref_axis',(0.,1.,0.));
#120107=DIRECTION('center_axis',(1.,0.,4.58212374768871E-32));
#120108=DIRECTION('ref_axis',(0.,1.,0.));
#120109=DIRECTION('center_axis',(-1.,0.,0.));
#120110=DIRECTION('ref_axis',(0.,0.,1.));
#120111=DIRECTION('',(1.,3.71118737634973E-16,4.58212374768871E-32));
#120112=DIRECTION('',(-1.,-3.71118737634973E-16,-4.58212374768871E-32));
#120113=DIRECTION('center_axis',(0.,1.23467863058847E-16,-1.));
#120114=DIRECTION('ref_axis',(0.,1.,1.25697703075927E-16));
#120115=DIRECTION('center_axis',(-0.00184724109421639,0.999998293848714,
0.));
#120116=DIRECTION('ref_axis',(-0.999998293848714,-0.00184724109421639,0.));
#120117=DIRECTION('center_axis',(0.,1.22914743790472E-16,-1.));
#120118=DIRECTION('ref_axis',(0.,1.,1.22914743790472E-16));
#120119=DIRECTION('center_axis',(5.51984300367294E-32,-1.22833149346405E-16,
1.));
#120120=DIRECTION('ref_axis',(8.69658697372547E-14,1.,1.22833149346405E-16));
#120121=DIRECTION('center_axis',(0.,1.23467863058847E-16,-1.));
#120122=DIRECTION('ref_axis',(0.,1.,0.));
#120123=DIRECTION('center_axis',(0.,0.,-1.));
#120124=DIRECTION('ref_axis',(0.,1.,0.));
#120125=DIRECTION('center_axis',(0.,0.,1.));
#120126=DIRECTION('ref_axis',(0.,1.,0.));
#120127=DIRECTION('center_axis',(0.,1.23467863058847E-16,-1.));
#120128=DIRECTION('ref_axis',(0.,1.,0.));
#120129=DIRECTION('center_axis',(-1.,0.,0.));
#120130=DIRECTION('ref_axis',(0.,0.,1.));
#120131=DIRECTION('center_axis',(0.,0.,-1.));
#120132=DIRECTION('ref_axis',(0.,1.,0.));
#120133=DIRECTION('center_axis',(0.,1.,9.63735264431547E-16));
#120134=DIRECTION('ref_axis',(0.,-9.63735264431547E-16,1.));
#120135=DIRECTION('center_axis',(0.,0.,1.));
#120136=DIRECTION('ref_axis',(0.,1.,0.));
#120137=DIRECTION('center_axis',(7.82779334765923E-17,1.,0.));
#120138=DIRECTION('ref_axis',(0.,0.,1.));
#120139=DIRECTION('center_axis',(-3.85494105772624E-15,1.,0.));
#120140=DIRECTION('ref_axis',(-1.,-3.85494105772625E-15,0.));
#120141=DIRECTION('',(-7.82779334765923E-17,-1.,-1.23467863058847E-16));
#120142=DIRECTION('',(7.82779334765923E-17,1.,1.23467863058847E-16));
#120143=DIRECTION('center_axis',(-1.,0.,4.58212374768871E-32));
#120144=DIRECTION('ref_axis',(0.,-1.,0.));
#120145=DIRECTION('center_axis',(-1.,0.,0.));
#120146=DIRECTION('ref_axis',(0.,0.,1.));
#120147=DIRECTION('',(1.,-3.71118737634973E-16,-4.58212374768871E-32));
#120148=DIRECTION('',(-1.,3.71118737634973E-16,4.58212374768871E-32));
#120149=DIRECTION('center_axis',(0.,1.23467863058847E-16,-1.));
#120150=DIRECTION('ref_axis',(0.,1.,0.));
#120151=DIRECTION('center_axis',(-1.,0.,0.));
#120152=DIRECTION('ref_axis',(0.,0.,1.));
#120153=DIRECTION('center_axis',(0.,0.,1.));
#120154=DIRECTION('ref_axis',(0.,1.,0.));
#120155=DIRECTION('center_axis',(0.,0.,-1.));
#120156=DIRECTION('ref_axis',(0.,1.,0.));
#120157=DIRECTION('center_axis',(0.,1.23467863058847E-16,-1.));
#120158=DIRECTION('ref_axis',(0.,1.,0.));
#120159=DIRECTION('center_axis',(0.,1.,0.));
#120160=DIRECTION('ref_axis',(0.,0.,1.));
#120161=DIRECTION('center_axis',(0.,0.,-1.));
#120162=DIRECTION('ref_axis',(0.,1.,0.));
#120163=DIRECTION('center_axis',(0.,0.,1.));
#120164=DIRECTION('ref_axis',(0.,1.,0.));
#120165=DIRECTION('center_axis',(1.,0.,4.58212374768871E-32));
#120166=DIRECTION('ref_axis',(0.,1.,0.));
#120167=DIRECTION('center_axis',(-1.,0.,0.));
#120168=DIRECTION('ref_axis',(0.,0.,1.));
#120169=DIRECTION('',(1.,3.71118737634973E-16,4.58212374768871E-32));
#120170=DIRECTION('',(-1.,-3.71118737634973E-16,-4.58212374768871E-32));
#120171=DIRECTION('center_axis',(0.,-1.,0.));
#120172=DIRECTION('ref_axis',(0.,0.,-1.));
#120173=DIRECTION('center_axis',(0.,1.,0.));
#120174=DIRECTION('ref_axis',(0.,0.,1.));
#120175=DIRECTION('',(0.,-1.,-1.23467863058847E-16));
#120176=DIRECTION('',(0.,1.,1.23467863058847E-16));
#120177=DIRECTION('center_axis',(0.,1.23467863058847E-16,-1.));
#120178=DIRECTION('ref_axis',(0.,1.,0.));
#120179=DIRECTION('center_axis',(0.,0.,-1.));
#120180=DIRECTION('ref_axis',(0.,1.,0.));
#120181=DIRECTION('center_axis',(0.,0.,1.));
#120182=DIRECTION('ref_axis',(0.,1.,0.));
#120183=DIRECTION('center_axis',(0.,1.23467863058847E-16,-1.));
#120184=DIRECTION('ref_axis',(0.,1.,0.));
#120185=DIRECTION('center_axis',(0.0972343474872435,-0.995261514210577,
0.));
#120186=DIRECTION('ref_axis',(0.995261514210577,0.0972343474872435,0.));
#120187=DIRECTION('center_axis',(0.,0.,-1.));
#120188=DIRECTION('ref_axis',(0.,1.,0.));
#120189=DIRECTION('center_axis',(-1.,0.,0.));
#120190=DIRECTION('ref_axis',(0.,0.,1.));
#120191=DIRECTION('center_axis',(1.78485500480727E-31,-2.58019156504489E-46,
1.));
#120192=DIRECTION('ref_axis',(1.44560289664734E-15,1.,-3.88938454866321E-62));
#120193=DIRECTION('center_axis',(1.,0.,4.58212374768871E-32));
#120194=DIRECTION('ref_axis',(0.,1.,0.));
#120195=DIRECTION('center_axis',(-1.,0.,0.));
#120196=DIRECTION('ref_axis',(0.,0.,1.));
#120197=DIRECTION('',(1.,3.71118737634973E-16,4.58212374768871E-32));
#120198=DIRECTION('',(-1.,-3.71118737634973E-16,-4.58212374768871E-32));
#120199=DIRECTION('center_axis',(0.,1.23467863058847E-16,-1.));
#120200=DIRECTION('ref_axis',(0.,1.,0.));
#120201=DIRECTION('center_axis',(0.359814015251205,-0.933024048151389,0.));
#120202=DIRECTION('ref_axis',(0.933024048151389,0.359814015251205,0.));
#120203=DIRECTION('center_axis',(-9.86953423458227E-31,-7.88931658768281E-45,
1.));
#120204=DIRECTION('ref_axis',(-7.99360577730113E-15,1.,-2.48920611114446E-60));
#120205=DIRECTION('center_axis',(0.,0.,-1.));
#120206=DIRECTION('ref_axis',(0.,1.,0.));
#120207=DIRECTION('center_axis',(0.,1.23467863058847E-16,-1.));
#120208=DIRECTION('ref_axis',(0.,1.,0.));
#120209=DIRECTION('center_axis',(0.,-1.,0.));
#120210=DIRECTION('ref_axis',(0.,0.,-1.));
#120211=DIRECTION('center_axis',(0.,0.,1.));
#120212=DIRECTION('ref_axis',(0.,1.,0.));
#120213=DIRECTION('center_axis',(0.,0.,-1.));
#120214=DIRECTION('ref_axis',(0.,1.,0.));
#120215=DIRECTION('center_axis',(0.,1.23467863058847E-16,-1.));
#120216=DIRECTION('ref_axis',(0.,1.,0.));
#120217=DIRECTION('center_axis',(0.,-1.,0.));
#120218=DIRECTION('ref_axis',(0.,0.,-1.));
#120219=DIRECTION('center_axis',(0.,0.,-1.));
#120220=DIRECTION('ref_axis',(0.,1.,0.));
#120221=DIRECTION('center_axis',(0.,0.,1.));
#120222=DIRECTION('ref_axis',(0.,1.,0.));
#120223=DIRECTION('center_axis',(7.82779334765923E-17,-1.,0.));
#120224=DIRECTION('ref_axis',(0.,0.,-1.));
#120225=DIRECTION('center_axis',(0.,-1.,0.));
#120226=DIRECTION('ref_axis',(0.,0.,-1.));
#120227=DIRECTION('',(-7.82779334765923E-17,1.,1.23467863058847E-16));
#120228=DIRECTION('',(7.82779334765923E-17,-1.,-1.23467863058847E-16));
#120229=DIRECTION('center_axis',(5.87084501074442E-17,1.,0.));
#120230=DIRECTION('ref_axis',(0.,0.,1.));
#120231=DIRECTION('center_axis',(0.,-1.,0.));
#120232=DIRECTION('ref_axis',(0.,0.,-1.));
#120233=DIRECTION('',(5.87084501074442E-17,1.,1.23467863058847E-16));
#120234=DIRECTION('',(-5.87084501074442E-17,-1.,-1.23467863058847E-16));
#120235=DIRECTION('center_axis',(0.,1.23467863058847E-16,-1.));
#120236=DIRECTION('ref_axis',(0.,1.,0.));
#120237=DIRECTION('center_axis',(1.,0.,0.));
#120238=DIRECTION('ref_axis',(0.,0.,-1.));
#120239=DIRECTION('center_axis',(3.56971000961454E-31,-1.03207662601795E-45,
1.));
#120240=DIRECTION('ref_axis',(2.89120579329468E-15,1.,-2.1780553472514E-60));
#120241=DIRECTION('center_axis',(0.,0.,-1.));
#120242=DIRECTION('ref_axis',(0.,1.,0.));
#120243=DIRECTION('center_axis',(0.,1.23467863058847E-16,-1.));
#120244=DIRECTION('ref_axis',(0.,1.,0.));
#120245=DIRECTION('center_axis',(-1.,0.,0.));
#120246=DIRECTION('ref_axis',(0.,0.,1.));
#120247=DIRECTION('center_axis',(0.,0.,-1.));
#120248=DIRECTION('ref_axis',(0.,1.,0.));
#120249=DIRECTION('center_axis',(0.,0.,1.));
#120250=DIRECTION('ref_axis',(0.,1.,0.));
#120251=DIRECTION('center_axis',(-1.,0.,4.58212374768871E-32));
#120252=DIRECTION('ref_axis',(0.,-1.,0.));
#120253=DIRECTION('',(1.,-3.71118737634973E-16,-4.58212374768871E-32));
#120254=DIRECTION('',(-1.,3.71118737634973E-16,4.58212374768871E-32));
#120255=DIRECTION('center_axis',(0.,1.23467863058847E-16,-1.));
#120256=DIRECTION('ref_axis',(0.,1.,0.));
#120257=DIRECTION('center_axis',(7.70988211545246E-15,-1.,0.));
#120258=DIRECTION('ref_axis',(1.,7.70988211545246E-15,0.));
#120259=DIRECTION('center_axis',(0.,0.,-1.));
#120260=DIRECTION('ref_axis',(0.,1.,0.));
#120261=DIRECTION('center_axis',(-1.,0.,0.));
#120262=DIRECTION('ref_axis',(0.,0.,1.));
#120263=DIRECTION('center_axis',(1.78485500480727E-31,-2.58019156504489E-46,
1.));
#120264=DIRECTION('ref_axis',(1.44560289664734E-15,1.,-3.88938454866321E-62));
#120265=DIRECTION('center_axis',(1.,0.,4.07299888683441E-32));
#120266=DIRECTION('ref_axis',(0.,1.,0.));
#120267=DIRECTION('center_axis',(-1.,0.,0.));
#120268=DIRECTION('ref_axis',(0.,0.,1.));
#120269=DIRECTION('',(1.,3.29883322342198E-16,4.07299888683441E-32));
#120270=DIRECTION('',(-1.,-3.29883322342198E-16,-4.07299888683441E-32));
#120271=DIRECTION('center_axis',(5.87084501074442E-17,1.,0.));
#120272=DIRECTION('ref_axis',(0.,0.,1.));
#120273=DIRECTION('center_axis',(0.,-1.,0.));
#120274=DIRECTION('ref_axis',(0.,0.,-1.));
#120275=DIRECTION('',(5.87084501074442E-17,1.,1.23467863058847E-16));
#120276=DIRECTION('',(-5.87084501074442E-17,-1.,-1.23467863058847E-16));
#120277=DIRECTION('center_axis',(0.,1.23467863058847E-16,-1.));
#120278=DIRECTION('ref_axis',(0.,1.,0.));
#120279=DIRECTION('center_axis',(0.,-1.,0.));
#120280=DIRECTION('ref_axis',(0.,0.,-1.));
#120281=DIRECTION('center_axis',(0.,0.,1.));
#120282=DIRECTION('ref_axis',(0.,1.,0.));
#120283=DIRECTION('center_axis',(0.,0.,-1.));
#120284=DIRECTION('ref_axis',(0.,1.,0.));
#120285=DIRECTION('center_axis',(0.,1.23467863058847E-16,-1.));
#120286=DIRECTION('ref_axis',(0.,1.,0.));
#120287=DIRECTION('center_axis',(-0.359814015251208,-0.933024048151388,
0.));
#120288=DIRECTION('ref_axis',(0.933024048151388,-0.359814015251207,0.));
#120289=DIRECTION('center_axis',(0.,0.,-1.));
#120290=DIRECTION('ref_axis',(0.,1.,0.));
#120291=DIRECTION('center_axis',(0.,0.,1.));
#120292=DIRECTION('ref_axis',(0.,1.,0.));
#120293=DIRECTION('center_axis',(7.82779334765923E-17,-1.,0.));
#120294=DIRECTION('ref_axis',(0.,0.,-1.));
#120295=DIRECTION('center_axis',(-3.85494105772624E-15,-1.,0.));
#120296=DIRECTION('ref_axis',(1.,-3.85494105772625E-15,0.));
#120297=DIRECTION('',(-7.82779334765923E-17,1.,1.23467863058847E-16));
#120298=DIRECTION('',(7.82779334765923E-17,-1.,-1.23467863058847E-16));
#120299=DIRECTION('center_axis',(0.,1.23467863058847E-16,-1.));
#120300=DIRECTION('ref_axis',(0.,1.,0.));
#120301=DIRECTION('center_axis',(-0.0972343474872435,-0.995261514210577,
0.));
#120302=DIRECTION('ref_axis',(0.995261514210577,-0.0972343474872435,0.));
#120303=DIRECTION('center_axis',(-8.77291931962869E-31,-6.2335340939716E-45,
1.));
#120304=DIRECTION('ref_axis',(-7.105427357601E-15,1.,-3.73380916671668E-60));
#120305=DIRECTION('center_axis',(0.,0.,-1.));
#120306=DIRECTION('ref_axis',(0.,1.,0.));
#120307=DIRECTION('center_axis',(0.,1.23467863058847E-16,-1.));
#120308=DIRECTION('ref_axis',(0.,1.,0.));
#120309=DIRECTION('center_axis',(1.,0.,0.));
#120310=DIRECTION('ref_axis',(0.,0.,-1.));
#120311=DIRECTION('center_axis',(0.,0.,1.));
#120312=DIRECTION('ref_axis',(0.,1.,0.));
#120313=DIRECTION('center_axis',(0.,0.,-1.));
#120314=DIRECTION('ref_axis',(0.,1.,0.));
#120315=DIRECTION('center_axis',(0.,1.23467863058847E-16,-1.));
#120316=DIRECTION('ref_axis',(0.,1.,0.));
#120317=DIRECTION('center_axis',(-1.,0.,0.));
#120318=DIRECTION('ref_axis',(0.,0.,1.));
#120319=DIRECTION('center_axis',(0.,0.,-1.));
#120320=DIRECTION('ref_axis',(0.,1.,0.));
#120321=DIRECTION('center_axis',(0.,0.,1.));
#120322=DIRECTION('ref_axis',(0.,1.,0.));
#120323=DIRECTION('center_axis',(-1.,0.,4.58212374768871E-32));
#120324=DIRECTION('ref_axis',(0.,-1.,0.));
#120325=DIRECTION('',(1.,-3.71118737634973E-16,-4.58212374768871E-32));
#120326=DIRECTION('',(-1.,3.71118737634973E-16,4.58212374768871E-32));
#120327=DIRECTION('center_axis',(0.,1.23467863058847E-16,-1.));
#120328=DIRECTION('ref_axis',(0.,1.,0.));
#120329=DIRECTION('center_axis',(0.,-1.,0.));
#120330=DIRECTION('ref_axis',(0.,0.,-1.));
#120331=DIRECTION('center_axis',(0.,0.,-1.));
#120332=DIRECTION('ref_axis',(0.,1.,0.));
#120333=DIRECTION('center_axis',(-1.,0.,0.));
#120334=DIRECTION('ref_axis',(0.,0.,1.));
#120335=DIRECTION('center_axis',(0.,0.,1.));
#120336=DIRECTION('ref_axis',(0.,1.,0.));
#120337=DIRECTION('center_axis',(1.,0.,4.07299888683441E-32));
#120338=DIRECTION('ref_axis',(0.,1.,0.));
#120339=DIRECTION('center_axis',(-1.,0.,0.));
#120340=DIRECTION('ref_axis',(0.,0.,1.));
#120341=DIRECTION('',(1.,3.29883322342198E-16,4.07299888683441E-32));
#120342=DIRECTION('',(-1.,-3.29883322342198E-16,-4.07299888683441E-32));
#120343=DIRECTION('center_axis',(7.82779334765923E-17,1.,0.));
#120344=DIRECTION('ref_axis',(0.,0.,1.));
#120345=DIRECTION('center_axis',(0.,-1.,0.));
#120346=DIRECTION('ref_axis',(0.,0.,-1.));
#120347=DIRECTION('',(7.82779334765923E-17,1.,1.23467863058847E-16));
#120348=DIRECTION('',(-7.82779334765923E-17,-1.,-1.23467863058847E-16));
#120349=DIRECTION('center_axis',(0.,1.23467863058847E-16,-1.));
#120350=DIRECTION('ref_axis',(0.,1.,0.));
#120351=DIRECTION('center_axis',(0.,-1.,0.));
#120352=DIRECTION('ref_axis',(0.,0.,-1.));
#120353=DIRECTION('center_axis',(0.,0.,1.));
#120354=DIRECTION('ref_axis',(0.,1.,0.));
#120355=DIRECTION('center_axis',(0.,0.,-1.));
#120356=DIRECTION('ref_axis',(0.,1.,0.));
#120357=DIRECTION('center_axis',(0.,1.23467863058847E-16,-1.));
#120358=DIRECTION('ref_axis',(0.,1.,0.));
#120359=DIRECTION('center_axis',(-1.,0.,0.));
#120360=DIRECTION('ref_axis',(0.,0.,1.));
#120361=DIRECTION('center_axis',(0.,0.,-1.));
#120362=DIRECTION('ref_axis',(0.,1.,0.));
#120363=DIRECTION('center_axis',(0.,0.,1.));
#120364=DIRECTION('ref_axis',(0.,1.,0.));
#120365=DIRECTION('center_axis',(0.,-1.,0.));
#120366=DIRECTION('ref_axis',(0.,0.,-1.));
#120367=DIRECTION('center_axis',(-3.85494105772624E-15,-1.,0.));
#120368=DIRECTION('ref_axis',(1.,-3.85494105772625E-15,0.));
#120369=DIRECTION('',(0.,1.,1.23467863058847E-16));
#120370=DIRECTION('',(0.,-1.,-1.23467863058847E-16));
#120371=DIRECTION('center_axis',(-1.,0.,4.58212374768871E-32));
#120372=DIRECTION('ref_axis',(0.,-1.,0.));
#120373=DIRECTION('center_axis',(-1.,0.,0.));
#120374=DIRECTION('ref_axis',(0.,0.,1.));
#120375=DIRECTION('',(1.,-3.71118737634973E-16,-4.58212374768871E-32));
#120376=DIRECTION('',(-1.,3.71118737634973E-16,4.58212374768871E-32));
#120377=DIRECTION('center_axis',(0.,1.23467863058847E-16,-1.));
#120378=DIRECTION('ref_axis',(0.,1.,0.));
#120379=DIRECTION('center_axis',(0.,0.,-1.));
#120380=DIRECTION('ref_axis',(0.,1.,0.));
#120381=DIRECTION('center_axis',(0.,0.,1.));
#120382=DIRECTION('ref_axis',(0.,1.,0.));
#120383=DIRECTION('center_axis',(0.,1.23467863058847E-16,-1.));
#120384=DIRECTION('ref_axis',(0.,1.,0.));
#120385=DIRECTION('center_axis',(0.,-1.,0.));
#120386=DIRECTION('ref_axis',(0.,0.,-1.));
#120387=DIRECTION('center_axis',(0.,0.,-1.));
#120388=DIRECTION('ref_axis',(0.,1.,0.));
#120389=DIRECTION('center_axis',(-1.,0.,0.));
#120390=DIRECTION('ref_axis',(0.,0.,1.));
#120391=DIRECTION('center_axis',(0.,0.,1.));
#120392=DIRECTION('ref_axis',(0.,1.,0.));
#120393=DIRECTION('center_axis',(1.,0.,4.07299888683441E-32));
#120394=DIRECTION('ref_axis',(0.,1.,0.));
#120395=DIRECTION('center_axis',(-1.,0.,0.));
#120396=DIRECTION('ref_axis',(0.,0.,1.));
#120397=DIRECTION('',(1.,3.29883322342198E-16,4.07299888683441E-32));
#120398=DIRECTION('',(-1.,-3.29883322342198E-16,-4.07299888683441E-32));
#120399=DIRECTION('center_axis',(0.,1.,0.));
#120400=DIRECTION('ref_axis',(0.,0.,1.));
#120401=DIRECTION('center_axis',(0.,-1.,0.));
#120402=DIRECTION('ref_axis',(0.,0.,-1.));
#120403=DIRECTION('',(0.,1.,1.23467863058847E-16));
#120404=DIRECTION('',(0.,-1.,-1.23467863058847E-16));
#120405=DIRECTION('center_axis',(0.,1.23467863058847E-16,-1.));
#120406=DIRECTION('ref_axis',(0.,1.,0.));
#120407=DIRECTION('center_axis',(-0.0138255496962003,-0.999904422520272,
3.41098746684905E-15));
#120408=DIRECTION('ref_axis',(0.999904422520272,-0.0138255496962003,-3.38006024551251E-32));
#120409=DIRECTION('center_axis',(0.,0.,1.));
#120410=DIRECTION('ref_axis',(0.,1.,0.));
#120411=DIRECTION('center_axis',(0.,0.,-1.));
#120412=DIRECTION('ref_axis',(0.,1.,0.));
#120413=DIRECTION('center_axis',(0.,1.23467863058847E-16,-1.));
#120414=DIRECTION('ref_axis',(0.,1.,0.));
#120415=DIRECTION('center_axis',(-1.,0.,0.));
#120416=DIRECTION('ref_axis',(0.,0.,1.));
#120417=DIRECTION('center_axis',(0.,0.,-1.));
#120418=DIRECTION('ref_axis',(0.,1.,0.));
#120419=DIRECTION('center_axis',(0.,0.,1.));
#120420=DIRECTION('ref_axis',(0.,1.,0.));
#120421=DIRECTION('center_axis',(0.,1.23467863058847E-16,-1.));
#120422=DIRECTION('ref_axis',(0.,1.,1.25697703075927E-16));
#120423=DIRECTION('center_axis',(-0.00184724109421639,-0.999998293848714,
0.));
#120424=DIRECTION('ref_axis',(0.999998293848714,-0.00184724109421639,0.));
#120425=DIRECTION('center_axis',(0.,-1.22833149346405E-16,1.));
#120426=DIRECTION('ref_axis',(0.,1.,1.22833149346405E-16));
#120427=DIRECTION('center_axis',(0.,1.22914743790472E-16,-1.));
#120428=DIRECTION('ref_axis',(0.,1.,1.22914743790472E-16));
#120429=DIRECTION('center_axis',(-1.,0.,4.58212374768871E-32));
#120430=DIRECTION('ref_axis',(0.,-1.,0.));
#120431=DIRECTION('center_axis',(-1.,0.,0.));
#120432=DIRECTION('ref_axis',(0.,0.,1.));
#120433=DIRECTION('',(1.,-3.71118737634973E-16,-4.58212374768871E-32));
#120434=DIRECTION('',(-1.,3.71118737634973E-16,4.58212374768871E-32));
#120435=DIRECTION('center_axis',(0.,1.23467863058847E-16,-1.));
#120436=DIRECTION('ref_axis',(0.,1.,0.));
#120437=DIRECTION('center_axis',(0.,0.,-1.));
#120438=DIRECTION('ref_axis',(0.,1.,0.));
#120439=DIRECTION('center_axis',(0.,0.,1.));
#120440=DIRECTION('ref_axis',(0.,1.,0.));
#120441=DIRECTION('center_axis',(0.,1.23467863058847E-16,-1.));
#120442=DIRECTION('ref_axis',(0.,1.,0.));
#120443=DIRECTION('center_axis',(0.,1.,0.));
#120444=DIRECTION('ref_axis',(0.,0.,1.));
#120445=DIRECTION('center_axis',(0.,0.,-1.));
#120446=DIRECTION('ref_axis',(0.,1.,0.));
#120447=DIRECTION('center_axis',(1.,0.,0.));
#120448=DIRECTION('ref_axis',(0.,0.,-1.));
#120449=DIRECTION('center_axis',(0.,0.,1.));
#120450=DIRECTION('ref_axis',(0.,1.,0.));
#120451=DIRECTION('center_axis',(-1.,0.,4.07299888683441E-32));
#120452=DIRECTION('ref_axis',(0.,-1.,0.));
#120453=DIRECTION('center_axis',(1.,0.,0.));
#120454=DIRECTION('ref_axis',(0.,0.,-1.));
#120455=DIRECTION('',(-1.,3.29883322342198E-16,4.07299888683441E-32));
#120456=DIRECTION('',(1.,-3.29883322342198E-16,-4.07299888683441E-32));
#120457=DIRECTION('center_axis',(0.,-1.,0.));
#120458=DIRECTION('ref_axis',(0.,0.,-1.));
#120459=DIRECTION('center_axis',(0.,1.,0.));
#120460=DIRECTION('ref_axis',(0.,0.,1.));
#120461=DIRECTION('',(0.,-1.,-1.23467863058847E-16));
#120462=DIRECTION('',(0.,1.,1.23467863058847E-16));
#120463=DIRECTION('center_axis',(0.,1.23467863058847E-16,-1.));
#120464=DIRECTION('ref_axis',(0.,1.,0.));
#120465=DIRECTION('center_axis',(0.,1.,0.));
#120466=DIRECTION('ref_axis',(0.,0.,1.));
#120467=DIRECTION('center_axis',(0.,0.,1.));
#120468=DIRECTION('ref_axis',(0.,1.,0.));
#120469=DIRECTION('center_axis',(0.,0.,-1.));
#120470=DIRECTION('ref_axis',(0.,1.,0.));
#120471=DIRECTION('center_axis',(0.,1.23467863058847E-16,-1.));
#120472=DIRECTION('ref_axis',(0.,1.,0.));
#120473=DIRECTION('center_axis',(1.,0.,0.));
#120474=DIRECTION('ref_axis',(0.,0.,-1.));
#120475=DIRECTION('center_axis',(0.,0.,-1.));
#120476=DIRECTION('ref_axis',(0.,1.,0.));
#120477=DIRECTION('center_axis',(0.,0.,1.));
#120478=DIRECTION('ref_axis',(0.,1.,0.));
#120479=DIRECTION('center_axis',(7.82779334765923E-17,1.,0.));
#120480=DIRECTION('ref_axis',(0.,0.,1.));
#120481=DIRECTION('center_axis',(1.5419764230905E-14,1.,0.));
#120482=DIRECTION('ref_axis',(-1.,1.5419764230905E-14,0.));
#120483=DIRECTION('',(-7.82779334765923E-17,-1.,-1.23467863058847E-16));
#120484=DIRECTION('',(7.82779334765923E-17,1.,1.23467863058847E-16));
#120485=DIRECTION('center_axis',(1.,0.,4.07299888683445E-32));
#120486=DIRECTION('ref_axis',(0.,1.,0.));
#120487=DIRECTION('center_axis',(1.,0.,0.));
#120488=DIRECTION('ref_axis',(0.,0.,-1.));
#120489=DIRECTION('',(-1.,-3.29883322342202E-16,-4.07299888683446E-32));
#120490=DIRECTION('',(1.,3.29883322342202E-16,4.07299888683446E-32));
#120491=DIRECTION('center_axis',(0.,1.23467863058847E-16,-1.));
#120492=DIRECTION('ref_axis',(0.,1.,0.));
#120493=DIRECTION('center_axis',(0.,0.,-1.));
#120494=DIRECTION('ref_axis',(0.,1.,0.));
#120495=DIRECTION('center_axis',(0.,0.,1.));
#120496=DIRECTION('ref_axis',(0.,1.,0.));
#120497=DIRECTION('center_axis',(0.,1.23467863058847E-16,-1.));
#120498=DIRECTION('ref_axis',(0.,1.,0.));
#120499=DIRECTION('center_axis',(0.,1.,0.));
#120500=DIRECTION('ref_axis',(0.,0.,1.));
#120501=DIRECTION('center_axis',(0.,0.,-1.));
#120502=DIRECTION('ref_axis',(0.,1.,0.));
#120503=DIRECTION('center_axis',(1.,0.,0.));
#120504=DIRECTION('ref_axis',(0.,0.,-1.));
#120505=DIRECTION('center_axis',(0.,0.,1.));
#120506=DIRECTION('ref_axis',(0.,1.,0.));
#120507=DIRECTION('center_axis',(-1.,0.,4.07299888683441E-32));
#120508=DIRECTION('ref_axis',(0.,-1.,0.));
#120509=DIRECTION('center_axis',(1.,0.,0.));
#120510=DIRECTION('ref_axis',(0.,0.,-1.));
#120511=DIRECTION('',(-1.,3.29883322342198E-16,4.07299888683441E-32));
#120512=DIRECTION('',(1.,-3.29883322342198E-16,-4.07299888683441E-32));
#120513=DIRECTION('center_axis',(7.82779334765923E-17,-1.,0.));
#120514=DIRECTION('ref_axis',(0.,0.,-1.));
#120515=DIRECTION('center_axis',(0.,1.,0.));
#120516=DIRECTION('ref_axis',(0.,0.,1.));
#120517=DIRECTION('',(7.82779334765923E-17,-1.,-1.23467863058847E-16));
#120518=DIRECTION('',(-7.82779334765923E-17,1.,1.23467863058847E-16));
#120519=DIRECTION('center_axis',(0.,1.23467863058847E-16,-1.));
#120520=DIRECTION('ref_axis',(0.,1.,0.));
#120521=DIRECTION('center_axis',(0.,1.,0.));
#120522=DIRECTION('ref_axis',(0.,0.,1.));
#120523=DIRECTION('center_axis',(0.,0.,1.));
#120524=DIRECTION('ref_axis',(0.,1.,0.));
#120525=DIRECTION('center_axis',(0.,0.,-1.));
#120526=DIRECTION('ref_axis',(0.,1.,0.));
#120527=DIRECTION('center_axis',(0.,1.23467863058847E-16,-1.));
#120528=DIRECTION('ref_axis',(0.,1.,0.));
#120529=DIRECTION('center_axis',(1.,0.,0.));
#120530=DIRECTION('ref_axis',(0.,0.,-1.));
#120531=DIRECTION('center_axis',(0.,0.,-1.));
#120532=DIRECTION('ref_axis',(0.,1.,0.));
#120533=DIRECTION('center_axis',(0.,0.,1.));
#120534=DIRECTION('ref_axis',(0.,1.,0.));
#120535=DIRECTION('center_axis',(5.87084501074442E-17,1.,0.));
#120536=DIRECTION('ref_axis',(0.,0.,1.));
#120537=DIRECTION('center_axis',(1.5419764230905E-14,1.,5.94422822341731E-29));
#120538=DIRECTION('ref_axis',(-1.,1.5419764230905E-14,1.59309191113245E-57));
#120539=DIRECTION('',(-5.87084501074442E-17,-1.,-1.23467863058847E-16));
#120540=DIRECTION('',(5.87084501074442E-17,1.,1.23467863058847E-16));
#120541=DIRECTION('center_axis',(1.,0.,4.07299888683445E-32));
#120542=DIRECTION('ref_axis',(0.,1.,0.));
#120543=DIRECTION('center_axis',(1.,0.,0.));
#120544=DIRECTION('ref_axis',(0.,0.,-1.));
#120545=DIRECTION('',(-1.,-3.29883322342202E-16,-4.07299888683446E-32));
#120546=DIRECTION('',(1.,3.29883322342202E-16,4.07299888683446E-32));
#120547=DIRECTION('center_axis',(0.,1.23467863058847E-16,-1.));
#120548=DIRECTION('ref_axis',(0.,1.,0.));
#120549=DIRECTION('center_axis',(0.,0.,-1.));
#120550=DIRECTION('ref_axis',(0.,1.,0.));
#120551=DIRECTION('center_axis',(0.,0.,1.));
#120552=DIRECTION('ref_axis',(0.,1.,0.));
#120553=DIRECTION('center_axis',(0.,1.23467863058847E-16,-1.));
#120554=DIRECTION('ref_axis',(0.,1.,0.));
#120555=DIRECTION('center_axis',(0.,-1.,0.));
#120556=DIRECTION('ref_axis',(0.,0.,-1.));
#120557=DIRECTION('center_axis',(0.,0.,-1.));
#120558=DIRECTION('ref_axis',(0.,1.,0.));
#120559=DIRECTION('center_axis',(-1.,-4.81867632215781E-16,-7.43028527927166E-30));
#120560=DIRECTION('ref_axis',(4.81867632215781E-16,-1.,1.36218908067985E-60));
#120561=DIRECTION('center_axis',(0.,0.,1.));
#120562=DIRECTION('ref_axis',(0.,1.,0.));
#120563=DIRECTION('center_axis',(1.,0.,4.07299888683445E-32));
#120564=DIRECTION('ref_axis',(0.,1.,0.));
#120565=DIRECTION('center_axis',(-1.,0.,0.));
#120566=DIRECTION('ref_axis',(0.,0.,1.));
#120567=DIRECTION('',(1.,3.29883322342202E-16,4.07299888683446E-32));
#120568=DIRECTION('',(-1.,-3.29883322342202E-16,-4.07299888683446E-32));
#120569=DIRECTION('center_axis',(6.11546355285877E-17,1.,0.));
#120570=DIRECTION('ref_axis',(0.,0.,1.));
#120571=DIRECTION('center_axis',(0.,-1.,0.));
#120572=DIRECTION('ref_axis',(0.,0.,-1.));
#120573=DIRECTION('',(6.11546355285877E-17,1.,1.23467863058847E-16));
#120574=DIRECTION('',(-6.11546355285877E-17,-1.,-1.23467863058847E-16));
#120575=DIRECTION('center_axis',(0.,1.23467863058847E-16,-1.));
#120576=DIRECTION('ref_axis',(0.,1.,0.));
#120577=DIRECTION('center_axis',(0.,-1.,0.));
#120578=DIRECTION('ref_axis',(0.,0.,-1.));
#120579=DIRECTION('center_axis',(0.,0.,1.));
#120580=DIRECTION('ref_axis',(0.,1.,0.));
#120581=DIRECTION('center_axis',(0.,0.,-1.));
#120582=DIRECTION('ref_axis',(0.,1.,0.));
#120583=DIRECTION('center_axis',(0.,1.23467863058847E-16,-1.));
#120584=DIRECTION('ref_axis',(0.,1.,0.));
#120585=DIRECTION('center_axis',(-0.995922166025996,-0.0902166238455435,
0.));
#120586=DIRECTION('ref_axis',(0.0902166238455435,-0.995922166025996,0.));
#120587=DIRECTION('center_axis',(0.,0.,-1.));
#120588=DIRECTION('ref_axis',(0.,1.,0.));
#120589=DIRECTION('center_axis',(1.11553437800454E-31,-1.00788733009566E-46,
1.));
#120590=DIRECTION('ref_axis',(9.03501810404587E-16,1.,1.16681536459896E-61));
#120591=DIRECTION('center_axis',(0.,-1.,-1.23467863058847E-16));
#120592=DIRECTION('ref_axis',(1.,0.,0.));
#120593=DIRECTION('center_axis',(0.,-1.,0.));
#120594=DIRECTION('ref_axis',(0.,0.,-1.));
#120595=DIRECTION('',(3.13111733906369E-16,1.,1.23467863058847E-16));
#120596=DIRECTION('',(-3.13111733906369E-16,-1.,-1.23467863058847E-16));
#120597=DIRECTION('center_axis',(0.,1.23467863058847E-16,-1.));
#120598=DIRECTION('ref_axis',(0.,1.,0.));
#120599=DIRECTION('center_axis',(-0.913440670994019,-0.406971916198153,
0.));
#120600=DIRECTION('ref_axis',(0.406971916198153,-0.913440670994019,0.));
#120601=DIRECTION('center_axis',(0.,0.,1.));
#120602=DIRECTION('ref_axis',(0.,1.,0.));
#120603=DIRECTION('center_axis',(0.,0.,-1.));
#120604=DIRECTION('ref_axis',(0.,1.,0.));
#120605=DIRECTION('center_axis',(0.,1.23467863058847E-16,-1.));
#120606=DIRECTION('ref_axis',(0.,1.,0.));
#120607=DIRECTION('center_axis',(0.,0.,1.));
#120608=DIRECTION('ref_axis',(0.,1.,0.));
#120609=DIRECTION('center_axis',(0.,0.,-1.));
#120610=DIRECTION('ref_axis',(0.,1.,0.));
#120611=DIRECTION('center_axis',(0.99836765577839,0.0571141304368842,0.));
#120612=DIRECTION('ref_axis',(-0.0571141304368842,0.99836765577839,0.));
#120613=DIRECTION('center_axis',(0.,1.23467863058847E-16,-1.));
#120614=DIRECTION('ref_axis',(0.,1.,0.));
#120615=DIRECTION('center_axis',(0.,0.,1.));
#120616=DIRECTION('ref_axis',(0.,1.,0.));
#120617=DIRECTION('center_axis',(0.,0.,-1.));
#120618=DIRECTION('ref_axis',(0.,1.,0.));
#120619=DIRECTION('center_axis',(0.,1.23467863058847E-16,-1.));
#120620=DIRECTION('ref_axis',(0.,1.,0.));
#120621=DIRECTION('center_axis',(0.,-1.,0.));
#120622=DIRECTION('ref_axis',(0.,0.,-1.));
#120623=DIRECTION('center_axis',(0.,0.,-1.));
#120624=DIRECTION('ref_axis',(0.,1.,0.));
#120625=DIRECTION('center_axis',(-1.,0.,0.));
#120626=DIRECTION('ref_axis',(0.,0.,1.));
#120627=DIRECTION('center_axis',(0.,0.,1.));
#120628=DIRECTION('ref_axis',(0.,1.,0.));
#120629=DIRECTION('center_axis',(1.,0.,4.07299888683445E-32));
#120630=DIRECTION('ref_axis',(0.,1.,0.));
#120631=DIRECTION('center_axis',(-1.,0.,0.));
#120632=DIRECTION('ref_axis',(0.,0.,1.));
#120633=DIRECTION('',(1.,3.29883322342202E-16,4.07299888683446E-32));
#120634=DIRECTION('',(-1.,-3.29883322342202E-16,-4.07299888683446E-32));
#120635=DIRECTION('center_axis',(0.,1.,0.));
#120636=DIRECTION('ref_axis',(0.,0.,1.));
#120637=DIRECTION('center_axis',(0.,-1.,0.));
#120638=DIRECTION('ref_axis',(0.,0.,-1.));
#120639=DIRECTION('',(0.,1.,1.23467863058847E-16));
#120640=DIRECTION('',(0.,-1.,-1.23467863058847E-16));
#120641=DIRECTION('center_axis',(0.,1.23467863058847E-16,-1.));
#120642=DIRECTION('ref_axis',(0.,1.,0.));
#120643=DIRECTION('center_axis',(-0.0294983404866249,-0.999564829267484,
0.));
#120644=DIRECTION('ref_axis',(0.999564829267484,-0.0294983404866249,0.));
#120645=DIRECTION('center_axis',(0.,0.,1.));
#120646=DIRECTION('ref_axis',(0.,1.,0.));
#120647=DIRECTION('center_axis',(0.,0.,-1.));
#120648=DIRECTION('ref_axis',(0.,1.,0.));
#120649=DIRECTION('center_axis',(0.,1.23467863058847E-16,-1.));
#120650=DIRECTION('ref_axis',(0.,1.,0.));
#120651=DIRECTION('center_axis',(-1.,0.,0.));
#120652=DIRECTION('ref_axis',(0.,0.,1.));
#120653=DIRECTION('center_axis',(0.,0.,-1.));
#120654=DIRECTION('ref_axis',(0.,1.,0.));
#120655=DIRECTION('center_axis',(0.,0.,1.));
#120656=DIRECTION('ref_axis',(0.,1.,0.));
#120657=DIRECTION('center_axis',(0.,1.23467863058847E-16,-1.));
#120658=DIRECTION('ref_axis',(0.,1.,1.25697703075927E-16));
#120659=DIRECTION('center_axis',(-0.0175200318846409,-0.999846512462168,
-7.7086987446295E-15));
#120660=DIRECTION('ref_axis',(0.999846512462168,-0.0175200318846409,1.3995963210887E-31));
#120661=DIRECTION('center_axis',(-1.09981052690886E-31,-1.22833149346405E-16,
1.));
#120662=DIRECTION('ref_axis',(-1.73276629344662E-13,1.,1.22833149346405E-16));
#120663=DIRECTION('center_axis',(0.,1.22914743790472E-16,-1.));
#120664=DIRECTION('ref_axis',(0.,1.,1.22914743790472E-16));
#120665=DIRECTION('center_axis',(-1.,0.,4.07299888683441E-32));
#120666=DIRECTION('ref_axis',(0.,-1.,0.));
#120667=DIRECTION('center_axis',(-1.,0.,0.));
#120668=DIRECTION('ref_axis',(0.,0.,1.));
#120669=DIRECTION('',(1.,-3.29883322342198E-16,-4.07299888683441E-32));
#120670=DIRECTION('',(-1.,3.29883322342198E-16,4.07299888683441E-32));
#120671=DIRECTION('center_axis',(0.,1.23467863058847E-16,-1.));
#120672=DIRECTION('ref_axis',(0.,1.,0.));
#120673=DIRECTION('center_axis',(0.,0.,-1.));
#120674=DIRECTION('ref_axis',(0.,1.,0.));
#120675=DIRECTION('center_axis',(0.,0.,1.));
#120676=DIRECTION('ref_axis',(0.,1.,0.));
#120677=DIRECTION('center_axis',(0.,1.23467863058847E-16,-1.));
#120678=DIRECTION('ref_axis',(0.,1.,0.));
#120679=DIRECTION('center_axis',(-1.5419764230905E-14,-1.,0.));
#120680=DIRECTION('ref_axis',(1.,-1.5419764230905E-14,0.));
#120681=DIRECTION('center_axis',(0.,0.,-1.));
#120682=DIRECTION('ref_axis',(0.,1.,0.));
#120683=DIRECTION('center_axis',(-1.,0.,0.));
#120684=DIRECTION('ref_axis',(0.,0.,1.));
#120685=DIRECTION('center_axis',(0.,0.,1.));
#120686=DIRECTION('ref_axis',(0.,1.,0.));
#120687=DIRECTION('center_axis',(1.,0.,7.06547394595967E-32));
#120688=DIRECTION('ref_axis',(0.,1.,0.));
#120689=DIRECTION('center_axis',(-1.,0.,0.));
#120690=DIRECTION('ref_axis',(0.,0.,1.));
#120691=DIRECTION('',(1.,5.72252063890675E-16,7.06547394595967E-32));
#120692=DIRECTION('',(-1.,-5.72252063890675E-16,-7.06547394595967E-32));
#120693=DIRECTION('center_axis',(0.,1.,0.));
#120694=DIRECTION('ref_axis',(0.,0.,1.));
#120695=DIRECTION('center_axis',(0.,-1.,0.));
#120696=DIRECTION('ref_axis',(0.,0.,-1.));
#120697=DIRECTION('',(0.,1.,1.23467863058847E-16));
#120698=DIRECTION('',(0.,-1.,-1.23467863058847E-16));
#120699=DIRECTION('center_axis',(0.,1.23467863058847E-16,-1.));
#120700=DIRECTION('ref_axis',(0.,1.,0.));
#120701=DIRECTION('center_axis',(-0.64691256419049,-0.762564183719958,0.));
#120702=DIRECTION('ref_axis',(0.762564183719958,-0.64691256419049,0.));
#120703=DIRECTION('center_axis',(0.,0.,1.));
#120704=DIRECTION('ref_axis',(0.,1.,0.));
#120705=DIRECTION('center_axis',(0.,0.,-1.));
#120706=DIRECTION('ref_axis',(0.,1.,0.));
#120707=DIRECTION('center_axis',(0.,1.23467863058847E-16,-1.));
#120708=DIRECTION('ref_axis',(0.,1.,0.));
#120709=DIRECTION('center_axis',(-1.,0.,0.));
#120710=DIRECTION('ref_axis',(0.,0.,1.));
#120711=DIRECTION('center_axis',(0.,0.,-1.));
#120712=DIRECTION('ref_axis',(0.,1.,0.));
#120713=DIRECTION('center_axis',(0.,0.,1.));
#120714=DIRECTION('ref_axis',(0.,1.,0.));
#120715=DIRECTION('center_axis',(0.,1.23467863058847E-16,-1.));
#120716=DIRECTION('ref_axis',(0.,1.,0.));
#120717=DIRECTION('center_axis',(-0.55837318130784,-0.829589892896582,0.));
#120718=DIRECTION('ref_axis',(0.829589892896582,-0.55837318130784,0.));
#120719=DIRECTION('center_axis',(0.,0.,1.));
#120720=DIRECTION('ref_axis',(0.,1.,0.));
#120721=DIRECTION('center_axis',(0.,0.,-1.));
#120722=DIRECTION('ref_axis',(0.,1.,0.));
#120723=DIRECTION('center_axis',(-1.,0.,4.07299888683445E-32));
#120724=DIRECTION('ref_axis',(0.,-1.,0.));
#120725=DIRECTION('center_axis',(-1.,0.,0.));
#120726=DIRECTION('ref_axis',(0.,0.,1.));
#120727=DIRECTION('',(1.,-3.29883322342202E-16,-4.07299888683446E-32));
#120728=DIRECTION('',(-1.,3.29883322342202E-16,4.07299888683446E-32));
#120729=DIRECTION('center_axis',(0.,1.23467863058847E-16,-1.));
#120730=DIRECTION('ref_axis',(0.,1.,0.));
#120731=DIRECTION('center_axis',(-0.03879684915621,-0.999247118832749,-5.83634271056011E-15));
#120732=DIRECTION('ref_axis',(0.999247118832749,-0.03879684915621,-4.4574149748685E-34));
#120733=DIRECTION('center_axis',(0.,0.,1.));
#120734=DIRECTION('ref_axis',(0.,1.,0.));
#120735=DIRECTION('center_axis',(0.,0.,-1.));
#120736=DIRECTION('ref_axis',(0.,1.,0.));
#120737=DIRECTION('center_axis',(0.,1.23467863058847E-16,-1.));
#120738=DIRECTION('ref_axis',(0.,1.,0.));
#120739=DIRECTION('center_axis',(0.0331928226750423,0.999448966442441,0.));
#120740=DIRECTION('ref_axis',(-0.999448966442441,0.0331928226750423,0.));
#120741=DIRECTION('center_axis',(0.,0.,-1.));
#120742=DIRECTION('ref_axis',(0.,1.,0.));
#120743=DIRECTION('center_axis',(0.,0.,1.));
#120744=DIRECTION('ref_axis',(0.,1.,0.));
#120745=DIRECTION('center_axis',(0.,1.23467863058847E-16,-1.));
#120746=DIRECTION('ref_axis',(0.,1.,1.25697703075927E-16));
#120747=DIRECTION('center_axis',(0.,1.22914743790472E-16,-1.));
#120748=DIRECTION('ref_axis',(0.,1.,1.22914743790472E-16));
#120749=DIRECTION('center_axis',(-1.17257681885938E-31,-1.22833149346405E-16,
1.));
#120750=DIRECTION('ref_axis',(-1.84741056616993E-13,1.,1.22833149346405E-16));
#120751=DIRECTION('center_axis',(0.,1.23467863058847E-16,-1.));
#120752=DIRECTION('ref_axis',(0.,1.,0.));
#120753=DIRECTION('center_axis',(0.,-1.,0.));
#120754=DIRECTION('ref_axis',(0.,0.,-1.));
#120755=DIRECTION('center_axis',(0.,0.,-1.));
#120756=DIRECTION('ref_axis',(0.,1.,0.));
#120757=DIRECTION('center_axis',(-1.,0.,0.));
#120758=DIRECTION('ref_axis',(0.,0.,1.));
#120759=DIRECTION('center_axis',(0.,0.,1.));
#120760=DIRECTION('ref_axis',(0.,1.,0.));
#120761=DIRECTION('center_axis',(1.,0.,7.06547394595967E-32));
#120762=DIRECTION('ref_axis',(0.,1.,0.));
#120763=DIRECTION('center_axis',(-1.,0.,0.));
#120764=DIRECTION('ref_axis',(0.,0.,1.));
#120765=DIRECTION('',(1.,5.72252063890675E-16,7.06547394595967E-32));
#120766=DIRECTION('',(-1.,-5.72252063890675E-16,-7.06547394595967E-32));
#120767=DIRECTION('center_axis',(7.82779334765923E-17,1.,0.));
#120768=DIRECTION('ref_axis',(0.,0.,1.));
#120769=DIRECTION('center_axis',(0.,-1.,0.));
#120770=DIRECTION('ref_axis',(0.,0.,-1.));
#120771=DIRECTION('',(7.82779334765923E-17,1.,1.23467863058847E-16));
#120772=DIRECTION('',(-7.82779334765923E-17,-1.,-1.23467863058847E-16));
#120773=DIRECTION('center_axis',(0.,1.23467863058847E-16,-1.));
#120774=DIRECTION('ref_axis',(0.,1.,0.));
#120775=DIRECTION('center_axis',(0.,-1.,0.));
#120776=DIRECTION('ref_axis',(0.,0.,-1.));
#120777=DIRECTION('center_axis',(0.,0.,1.));
#120778=DIRECTION('ref_axis',(0.,1.,0.));
#120779=DIRECTION('center_axis',(0.,0.,-1.));
#120780=DIRECTION('ref_axis',(0.,1.,0.));
#120781=DIRECTION('center_axis',(0.,1.23467863058847E-16,-1.));
#120782=DIRECTION('ref_axis',(0.,1.,0.));
#120783=DIRECTION('center_axis',(-1.,0.,0.));
#120784=DIRECTION('ref_axis',(0.,0.,1.));
#120785=DIRECTION('center_axis',(0.,0.,-1.));
#120786=DIRECTION('ref_axis',(0.,1.,0.));
#120787=DIRECTION('center_axis',(0.,0.,1.));
#120788=DIRECTION('ref_axis',(0.,1.,0.));
#120789=DIRECTION('center_axis',(0.,-1.,0.));
#120790=DIRECTION('ref_axis',(0.,0.,-1.));
#120791=DIRECTION('center_axis',(1.5419764230905E-14,-1.,0.));
#120792=DIRECTION('ref_axis',(1.,1.5419764230905E-14,0.));
#120793=DIRECTION('',(0.,1.,1.23467863058847E-16));
#120794=DIRECTION('',(0.,-1.,-1.23467863058847E-16));
#120795=DIRECTION('center_axis',(-1.,0.,4.07299888683445E-32));
#120796=DIRECTION('ref_axis',(0.,-1.,0.));
#120797=DIRECTION('center_axis',(-1.,0.,0.));
#120798=DIRECTION('ref_axis',(0.,0.,1.));
#120799=DIRECTION('',(1.,-3.29883322342202E-16,-4.07299888683446E-32));
#120800=DIRECTION('',(-1.,3.29883322342202E-16,4.07299888683446E-32));
#120801=DIRECTION('center_axis',(0.,1.23467863058847E-16,-1.));
#120802=DIRECTION('ref_axis',(0.,1.,0.));
#120803=DIRECTION('center_axis',(0.,0.,-1.));
#120804=DIRECTION('ref_axis',(0.,1.,0.));
#120805=DIRECTION('center_axis',(0.,0.,1.));
#120806=DIRECTION('ref_axis',(0.,1.,0.));
#120807=DIRECTION('center_axis',(0.,1.23467863058847E-16,-1.));
#120808=DIRECTION('ref_axis',(0.,1.,0.));
#120809=DIRECTION('center_axis',(-1.5419764230905E-14,1.,0.));
#120810=DIRECTION('ref_axis',(-1.,-1.5419764230905E-14,0.));
#120811=DIRECTION('center_axis',(0.,0.,-1.));
#120812=DIRECTION('ref_axis',(0.,1.,0.));
#120813=DIRECTION('center_axis',(1.,0.,0.));
#120814=DIRECTION('ref_axis',(0.,0.,-1.));
#120815=DIRECTION('center_axis',(0.,0.,1.));
#120816=DIRECTION('ref_axis',(0.,1.,0.));
#120817=DIRECTION('center_axis',(-1.,0.,-2.35515798198655E-32));
#120818=DIRECTION('ref_axis',(0.,-1.,0.));
#120819=DIRECTION('center_axis',(1.,0.,0.));
#120820=DIRECTION('ref_axis',(0.,0.,-1.));
#120821=DIRECTION('',(-1.,-1.90750687963558E-16,-2.35515798198656E-32));
#120822=DIRECTION('',(1.,1.90750687963558E-16,2.35515798198656E-32));
#120823=DIRECTION('center_axis',(0.,-1.,0.));
#120824=DIRECTION('ref_axis',(0.,0.,-1.));
#120825=DIRECTION('center_axis',(0.,1.,0.));
#120826=DIRECTION('ref_axis',(0.,0.,1.));
#120827=DIRECTION('',(0.,-1.,-1.23467863058847E-16));
#120828=DIRECTION('',(0.,1.,1.23467863058847E-16));
#120829=DIRECTION('center_axis',(0.,1.23467863058847E-16,-1.));
#120830=DIRECTION('ref_axis',(0.,1.,0.));
#120831=DIRECTION('center_axis',(0.,1.,0.));
#120832=DIRECTION('ref_axis',(0.,0.,1.));
#120833=DIRECTION('center_axis',(0.,0.,1.));
#120834=DIRECTION('ref_axis',(0.,1.,0.));
#120835=DIRECTION('center_axis',(0.,0.,-1.));
#120836=DIRECTION('ref_axis',(0.,1.,0.));
#120837=DIRECTION('center_axis',(0.,1.23467863058847E-16,-1.));
#120838=DIRECTION('ref_axis',(0.,1.,0.));
#120839=DIRECTION('center_axis',(0.787431540449696,0.616402116402125,0.));
#120840=DIRECTION('ref_axis',(-0.616402116402125,0.787431540449696,0.));
#120841=DIRECTION('center_axis',(0.,0.,-1.));
#120842=DIRECTION('ref_axis',(0.,1.,0.));
#120843=DIRECTION('center_axis',(0.,0.,1.));
#120844=DIRECTION('ref_axis',(0.,1.,0.));
#120845=DIRECTION('center_axis',(7.82779334765923E-17,1.,0.));
#120846=DIRECTION('ref_axis',(0.,0.,1.));
#120847=DIRECTION('center_axis',(0.,1.,0.));
#120848=DIRECTION('ref_axis',(0.,0.,1.));
#120849=DIRECTION('',(-7.82779334765923E-17,-1.,-1.23467863058847E-16));
#120850=DIRECTION('',(7.82779334765923E-17,1.,1.23467863058847E-16));
#120851=DIRECTION('center_axis',(0.,1.23467863058847E-16,-1.));
#120852=DIRECTION('ref_axis',(0.,1.,0.));
#120853=DIRECTION('center_axis',(0.873059908686793,0.487612957009766,0.));
#120854=DIRECTION('ref_axis',(-0.487612957009766,0.873059908686793,0.));
#120855=DIRECTION('center_axis',(0.,0.,-1.));
#120856=DIRECTION('ref_axis',(0.,1.,0.));
#120857=DIRECTION('center_axis',(0.,0.,1.));
#120858=DIRECTION('ref_axis',(0.,1.,0.));
#120859=DIRECTION('center_axis',(0.,1.23467863058847E-16,-1.));
#120860=DIRECTION('ref_axis',(-0.695782815675815,-0.718252235228151,0.));
#120861=DIRECTION('center_axis',(-0.99949512518498,-0.0317725468205174,
0.));
#120862=DIRECTION('ref_axis',(0.0317725468205174,-0.99949512518498,0.));
#120863=DIRECTION('center_axis',(0.,0.,1.));
#120864=DIRECTION('ref_axis',(0.,1.,0.));
#120865=DIRECTION('center_axis',(0.,0.,-1.));
#120866=DIRECTION('ref_axis',(0.,1.,0.));
#120867=DIRECTION('center_axis',(0.,1.23467863058847E-16,-1.));
#120868=DIRECTION('ref_axis',(0.,1.,0.));
#120869=DIRECTION('center_axis',(0.999425898115847,0.0338802918425069,0.));
#120870=DIRECTION('ref_axis',(-0.0338802918425069,0.999425898115847,0.));
#120871=DIRECTION('center_axis',(0.,0.,-1.));
#120872=DIRECTION('ref_axis',(0.,1.,0.));
#120873=DIRECTION('center_axis',(0.,0.,1.));
#120874=DIRECTION('ref_axis',(0.,1.,0.));
#120875=DIRECTION('center_axis',(0.,1.23467863058847E-16,-1.));
#120876=DIRECTION('ref_axis',(0.,1.,1.25697703075927E-16));
#120877=DIRECTION('center_axis',(0.,1.22914743790472E-16,-1.));
#120878=DIRECTION('ref_axis',(0.,1.,1.22914743790472E-16));
#120879=DIRECTION('center_axis',(0.,-1.22833149346405E-16,1.));
#120880=DIRECTION('ref_axis',(0.,1.,1.22833149346405E-16));
#120881=DIRECTION('center_axis',(0.,1.23467863058847E-16,-1.));
#120882=DIRECTION('ref_axis',(0.,1.,0.));
#120883=DIRECTION('center_axis',(-1.5419764230905E-14,1.,0.));
#120884=DIRECTION('ref_axis',(-1.,-1.5419764230905E-14,0.));
#120885=DIRECTION('center_axis',(0.,0.,-1.));
#120886=DIRECTION('ref_axis',(0.,1.,0.));
#120887=DIRECTION('center_axis',(1.,0.,0.));
#120888=DIRECTION('ref_axis',(0.,0.,-1.));
#120889=DIRECTION('center_axis',(0.,0.,1.));
#120890=DIRECTION('ref_axis',(0.,1.,0.));
#120891=DIRECTION('center_axis',(-1.,0.,-2.35515798198655E-32));
#120892=DIRECTION('ref_axis',(0.,-1.,0.));
#120893=DIRECTION('center_axis',(1.,0.,0.));
#120894=DIRECTION('ref_axis',(0.,0.,-1.));
#120895=DIRECTION('',(-1.,-1.90750687963558E-16,-2.35515798198656E-32));
#120896=DIRECTION('',(1.,1.90750687963558E-16,2.35515798198656E-32));
#120897=DIRECTION('center_axis',(7.82779334765923E-17,-1.,0.));
#120898=DIRECTION('ref_axis',(0.,0.,-1.));
#120899=DIRECTION('center_axis',(0.,1.,0.));
#120900=DIRECTION('ref_axis',(0.,0.,1.));
#120901=DIRECTION('',(7.82779334765923E-17,-1.,-1.23467863058847E-16));
#120902=DIRECTION('',(-7.82779334765923E-17,1.,1.23467863058847E-16));
#120903=DIRECTION('center_axis',(0.,1.23467863058847E-16,-1.));
#120904=DIRECTION('ref_axis',(0.,1.,0.));
#120905=DIRECTION('center_axis',(0.,1.,0.));
#120906=DIRECTION('ref_axis',(0.,0.,1.));
#120907=DIRECTION('center_axis',(0.,0.,1.));
#120908=DIRECTION('ref_axis',(0.,1.,0.));
#120909=DIRECTION('center_axis',(0.,0.,-1.));
#120910=DIRECTION('ref_axis',(0.,1.,0.));
#120911=DIRECTION('center_axis',(0.,1.23467863058847E-16,-1.));
#120912=DIRECTION('ref_axis',(0.,1.,0.));
#120913=DIRECTION('center_axis',(0.99960573342019,0.0280780646320843,0.));
#120914=DIRECTION('ref_axis',(-0.0280780646320843,0.99960573342019,0.));
#120915=DIRECTION('center_axis',(0.,0.,-1.));
#120916=DIRECTION('ref_axis',(0.,1.,0.));
#120917=DIRECTION('center_axis',(0.,0.,1.));
#120918=DIRECTION('ref_axis',(0.,1.,0.));
#120919=DIRECTION('center_axis',(5.87084501074442E-17,1.,0.));
#120920=DIRECTION('ref_axis',(0.,0.,1.));
#120921=DIRECTION('center_axis',(0.,1.,0.));
#120922=DIRECTION('ref_axis',(0.,0.,1.));
#120923=DIRECTION('',(-5.87084501074442E-17,-1.,-1.23467863058847E-16));
#120924=DIRECTION('',(5.87084501074442E-17,1.,1.23467863058847E-16));
#120925=DIRECTION('center_axis',(0.,1.23467863058847E-16,-1.));
#120926=DIRECTION('ref_axis',(0.,1.,1.25697703075927E-16));
#120927=DIRECTION('center_axis',(0.999858703750256,0.0168098939573669,0.));
#120928=DIRECTION('ref_axis',(-0.0168098939573669,0.999858703750256,0.));
#120929=DIRECTION('center_axis',(0.,1.22914743790472E-16,-1.));
#120930=DIRECTION('ref_axis',(0.,1.,1.22914743790472E-16));
#120931=DIRECTION('center_axis',(0.,-1.22833149346405E-16,1.));
#120932=DIRECTION('ref_axis',(0.,1.,1.22833149346405E-16));
#120933=DIRECTION('center_axis',(0.,1.23467863058847E-16,-1.));
#120934=DIRECTION('ref_axis',(-0.701138397908224,-0.713025207814344,0.));
#120935=DIRECTION('center_axis',(0.,0.,-1.));
#120936=DIRECTION('ref_axis',(0.,1.,0.));
#120937=DIRECTION('center_axis',(0.,0.,1.));
#120938=DIRECTION('ref_axis',(0.,1.,0.));
#120939=DIRECTION('center_axis',(0.,1.23467863058847E-16,-1.));
#120940=DIRECTION('ref_axis',(0.,1.,0.));
#120941=DIRECTION('center_axis',(-1.5419764230905E-14,-1.,0.));
#120942=DIRECTION('ref_axis',(1.,-1.5419764230905E-14,0.));
#120943=DIRECTION('center_axis',(0.,0.,-1.));
#120944=DIRECTION('ref_axis',(0.,1.,0.));
#120945=DIRECTION('center_axis',(-1.,0.,0.));
#120946=DIRECTION('ref_axis',(0.,0.,1.));
#120947=DIRECTION('center_axis',(0.,0.,1.));
#120948=DIRECTION('ref_axis',(0.,1.,0.));
#120949=DIRECTION('center_axis',(1.,0.,7.06547394595967E-32));
#120950=DIRECTION('ref_axis',(0.,1.,0.));
#120951=DIRECTION('center_axis',(-1.,0.,0.));
#120952=DIRECTION('ref_axis',(0.,0.,1.));
#120953=DIRECTION('',(1.,5.72252063890675E-16,7.06547394595967E-32));
#120954=DIRECTION('',(-1.,-5.72252063890675E-16,-7.06547394595967E-32));
#120955=DIRECTION('center_axis',(5.87084501074442E-17,1.,0.));
#120956=DIRECTION('ref_axis',(0.,0.,1.));
#120957=DIRECTION('center_axis',(0.,-1.,0.));
#120958=DIRECTION('ref_axis',(0.,0.,-1.));
#120959=DIRECTION('',(5.87084501074442E-17,1.,1.23467863058847E-16));
#120960=DIRECTION('',(-5.87084501074442E-17,-1.,-1.23467863058847E-16));
#120961=DIRECTION('center_axis',(0.,1.23467863058847E-16,-1.));
#120962=DIRECTION('ref_axis',(0.,1.,0.));
#120963=DIRECTION('center_axis',(0.,-1.,0.));
#120964=DIRECTION('ref_axis',(0.,0.,-1.));
#120965=DIRECTION('center_axis',(0.,0.,1.));
#120966=DIRECTION('ref_axis',(0.,1.,0.));
#120967=DIRECTION('center_axis',(0.,0.,-1.));
#120968=DIRECTION('ref_axis',(0.,1.,0.));
#120969=DIRECTION('center_axis',(0.,1.23467863058847E-16,-1.));
#120970=DIRECTION('ref_axis',(0.,1.,0.));
#120971=DIRECTION('center_axis',(-1.,0.,0.));
#120972=DIRECTION('ref_axis',(0.,0.,1.));
#120973=DIRECTION('center_axis',(0.,0.,-1.));
#120974=DIRECTION('ref_axis',(0.,1.,0.));
#120975=DIRECTION('center_axis',(0.,0.,1.));
#120976=DIRECTION('ref_axis',(0.,1.,0.));
#120977=DIRECTION('center_axis',(7.82779334765923E-17,-1.,0.));
#120978=DIRECTION('ref_axis',(0.,0.,-1.));
#120979=DIRECTION('center_axis',(1.5419764230905E-14,-1.,0.));
#120980=DIRECTION('ref_axis',(1.,1.5419764230905E-14,0.));
#120981=DIRECTION('',(-7.82779334765923E-17,1.,1.23467863058847E-16));
#120982=DIRECTION('',(7.82779334765923E-17,-1.,-1.23467863058847E-16));
#120983=DIRECTION('center_axis',(-1.,0.,4.07299888683445E-32));
#120984=DIRECTION('ref_axis',(0.,-1.,0.));
#120985=DIRECTION('center_axis',(-1.,0.,0.));
#120986=DIRECTION('ref_axis',(0.,0.,1.));
#120987=DIRECTION('',(1.,-3.29883322342202E-16,-4.07299888683446E-32));
#120988=DIRECTION('',(-1.,3.29883322342202E-16,4.07299888683446E-32));
#120989=DIRECTION('center_axis',(0.,1.23467863058847E-16,-1.));
#120990=DIRECTION('ref_axis',(0.,1.,0.));
#120991=DIRECTION('center_axis',(0.,0.,-1.));
#120992=DIRECTION('ref_axis',(0.,1.,0.));
#120993=DIRECTION('center_axis',(0.,0.,1.));
#120994=DIRECTION('ref_axis',(0.,1.,0.));
#120995=DIRECTION('center_axis',(0.,1.23467863058847E-16,-1.));
#120996=DIRECTION('ref_axis',(0.,1.,0.));
#120997=DIRECTION('center_axis',(0.,1.,0.));
#120998=DIRECTION('ref_axis',(0.,0.,1.));
#120999=DIRECTION('center_axis',(0.,0.,-1.));
#121000=DIRECTION('ref_axis',(0.,1.,0.));
#121001=DIRECTION('center_axis',(1.,0.,0.));
#121002=DIRECTION('ref_axis',(0.,0.,-1.));
#121003=DIRECTION('center_axis',(0.,0.,1.));
#121004=DIRECTION('ref_axis',(0.,1.,0.));
#121005=DIRECTION('center_axis',(-1.,0.,-2.35515798198655E-32));
#121006=DIRECTION('ref_axis',(0.,-1.,0.));
#121007=DIRECTION('center_axis',(1.,4.81867632215781E-16,0.));
#121008=DIRECTION('ref_axis',(-4.81867632215781E-16,1.,0.));
#121009=DIRECTION('',(-1.,-1.90750687963558E-16,-2.35515798198656E-32));
#121010=DIRECTION('',(1.,1.90750687963558E-16,2.35515798198656E-32));
#121011=DIRECTION('center_axis',(0.,-1.,-1.23467863058847E-16));
#121012=DIRECTION('ref_axis',(1.,0.,0.));
#121013=DIRECTION('center_axis',(0.,1.,0.));
#121014=DIRECTION('ref_axis',(0.,0.,1.));
#121015=DIRECTION('',(-3.13111733906369E-16,-1.,-1.23467863058847E-16));
#121016=DIRECTION('',(3.13111733906369E-16,1.,1.23467863058847E-16));
#121017=DIRECTION('center_axis',(0.,1.23467863058847E-16,-1.));
#121018=DIRECTION('ref_axis',(0.,1.,0.));
#121019=DIRECTION('center_axis',(0.,1.,0.));
#121020=DIRECTION('ref_axis',(0.,0.,1.));
#121021=DIRECTION('center_axis',(0.,0.,1.));
#121022=DIRECTION('ref_axis',(0.,1.,0.));
#121023=DIRECTION('center_axis',(0.,0.,-1.));
#121024=DIRECTION('ref_axis',(0.,1.,0.));
#121025=DIRECTION('center_axis',(0.,1.23467863058847E-16,-1.));
#121026=DIRECTION('ref_axis',(0.,1.,0.));
#121027=DIRECTION('center_axis',(0.999913989288144,0.0131154117689341,0.));
#121028=DIRECTION('ref_axis',(-0.0131154117689341,0.999913989288144,0.));
#121029=DIRECTION('center_axis',(0.,0.,-1.));
#121030=DIRECTION('ref_axis',(0.,1.,0.));
#121031=DIRECTION('center_axis',(0.,0.,1.));
#121032=DIRECTION('ref_axis',(0.,1.,0.));
#121033=DIRECTION('center_axis',(6.11546355285877E-17,1.,0.));
#121034=DIRECTION('ref_axis',(0.,0.,1.));
#121035=DIRECTION('center_axis',(0.,1.,0.));
#121036=DIRECTION('ref_axis',(0.,0.,1.));
#121037=DIRECTION('',(-6.11546355285877E-17,-1.,-1.23467863058847E-16));
#121038=DIRECTION('',(6.11546355285877E-17,1.,1.23467863058847E-16));
#121039=DIRECTION('center_axis',(0.,1.23467863058847E-16,-1.));
#121040=DIRECTION('ref_axis',(0.,1.,1.25697703075927E-16));
#121041=DIRECTION('center_axis',(0.999998293848715,0.00184724109421639,
0.));
#121042=DIRECTION('ref_axis',(-0.00184724109421639,0.999998293848714,0.));
#121043=DIRECTION('center_axis',(0.,1.22914743790472E-16,-1.));
#121044=DIRECTION('ref_axis',(0.,1.,1.22914743790472E-16));
#121045=DIRECTION('center_axis',(0.,-1.22833149346405E-16,1.));
#121046=DIRECTION('ref_axis',(0.,1.,1.22833149346405E-16));
#121047=DIRECTION('center_axis',(0.,1.23467863058847E-16,-1.));
#121048=DIRECTION('ref_axis',(-0.706453380948024,-0.707759578209371,0.));
#121049=DIRECTION('center_axis',(0.,0.,-1.));
#121050=DIRECTION('ref_axis',(0.,1.,0.));
#121051=DIRECTION('center_axis',(0.,0.,1.));
#121052=DIRECTION('ref_axis',(0.,1.,0.));
#121053=DIRECTION('center_axis',(0.,1.23467863058847E-16,-1.));
#121054=DIRECTION('ref_axis',(0.,1.,0.));
#121055=DIRECTION('center_axis',(0.,-1.,0.));
#121056=DIRECTION('ref_axis',(0.,0.,-1.));
#121057=DIRECTION('center_axis',(0.,0.,-1.));
#121058=DIRECTION('ref_axis',(0.,1.,0.));
#121059=DIRECTION('center_axis',(-1.,-4.81867632215781E-16,7.43028527927166E-30));
#121060=DIRECTION('ref_axis',(4.81867632215781E-16,-1.,-1.36218908067985E-60));
#121061=DIRECTION('center_axis',(0.,0.,1.));
#121062=DIRECTION('ref_axis',(0.,1.,0.));
#121063=DIRECTION('center_axis',(1.,0.,7.06547394595967E-32));
#121064=DIRECTION('ref_axis',(0.,1.,0.));
#121065=DIRECTION('center_axis',(-1.,0.,0.));
#121066=DIRECTION('ref_axis',(0.,0.,1.));
#121067=DIRECTION('',(1.,5.72252063890675E-16,7.06547394595967E-32));
#121068=DIRECTION('',(-1.,-5.72252063890675E-16,-7.06547394595967E-32));
#121069=DIRECTION('center_axis',(6.11546355285877E-17,1.,0.));
#121070=DIRECTION('ref_axis',(0.,0.,1.));
#121071=DIRECTION('center_axis',(0.,-1.,0.));
#121072=DIRECTION('ref_axis',(0.,0.,-1.));
#121073=DIRECTION('',(6.11546355285877E-17,1.,1.23467863058847E-16));
#121074=DIRECTION('',(-6.11546355285877E-17,-1.,-1.23467863058847E-16));
#121075=DIRECTION('center_axis',(0.,1.23467863058847E-16,-1.));
#121076=DIRECTION('ref_axis',(0.,1.,0.));
#121077=DIRECTION('center_axis',(0.,-1.,0.));
#121078=DIRECTION('ref_axis',(0.,0.,-1.));
#121079=DIRECTION('center_axis',(1.78485500480727E-31,-2.58019156504489E-46,
1.));
#121080=DIRECTION('ref_axis',(1.44560289664734E-15,1.,-3.88938454866321E-62));
#121081=DIRECTION('center_axis',(0.,0.,-1.));
#121082=DIRECTION('ref_axis',(0.,1.,0.));
#121083=DIRECTION('center_axis',(0.,1.23467863058847E-16,-1.));
#121084=DIRECTION('ref_axis',(0.,1.,0.));
#121085=DIRECTION('center_axis',(-1.,4.81867632215781E-16,0.));
#121086=DIRECTION('ref_axis',(-4.81867632215781E-16,-1.,0.));
#121087=DIRECTION('center_axis',(0.,0.,-1.));
#121088=DIRECTION('ref_axis',(0.,1.,0.));
#121089=DIRECTION('center_axis',(0.,0.,1.));
#121090=DIRECTION('ref_axis',(0.,1.,0.));
#121091=DIRECTION('center_axis',(0.,-1.,-1.23467863058847E-16));
#121092=DIRECTION('ref_axis',(1.,0.,0.));
#121093=DIRECTION('center_axis',(0.,-1.,0.));
#121094=DIRECTION('ref_axis',(0.,0.,-1.));
#121095=DIRECTION('',(3.13111733906369E-16,1.,1.23467863058847E-16));
#121096=DIRECTION('',(-3.13111733906369E-16,-1.,-1.23467863058847E-16));
#121097=DIRECTION('center_axis',(-1.,0.,4.07299888683445E-32));
#121098=DIRECTION('ref_axis',(0.,-1.,0.));
#121099=DIRECTION('center_axis',(-1.,0.,0.));
#121100=DIRECTION('ref_axis',(0.,0.,1.));
#121101=DIRECTION('',(1.,-3.29883322342202E-16,-4.07299888683446E-32));
#121102=DIRECTION('',(-1.,3.29883322342202E-16,4.07299888683446E-32));
#121103=DIRECTION('center_axis',(0.,1.23467863058847E-16,-1.));
#121104=DIRECTION('ref_axis',(0.,1.,0.));
#121105=DIRECTION('center_axis',(0.,0.,-1.));
#121106=DIRECTION('ref_axis',(0.,1.,0.));
#121107=DIRECTION('center_axis',(0.,0.,1.));
#121108=DIRECTION('ref_axis',(0.,1.,0.));
#121109=DIRECTION('center_axis',(0.,1.23467863058847E-16,-1.));
#121110=DIRECTION('ref_axis',(0.,1.,0.));
#121111=DIRECTION('center_axis',(0.699822617100543,0.714316669688274,0.));
#121112=DIRECTION('ref_axis',(-0.714316669688274,0.699822617100543,0.));
#121113=DIRECTION('center_axis',(0.,0.,-1.));
#121114=DIRECTION('ref_axis',(0.,1.,0.));
#121115=DIRECTION('center_axis',(1.,0.,0.));
#121116=DIRECTION('ref_axis',(0.,0.,-1.));
#121117=DIRECTION('center_axis',(0.,0.,1.));
#121118=DIRECTION('ref_axis',(0.,1.,0.));
#121119=DIRECTION('center_axis',(-1.,0.,-2.35515798198655E-32));
#121120=DIRECTION('ref_axis',(0.,-1.,0.));
#121121=DIRECTION('center_axis',(1.,0.,0.));
#121122=DIRECTION('ref_axis',(0.,0.,-1.));
#121123=DIRECTION('',(-1.,-1.90750687963558E-16,-2.35515798198656E-32));
#121124=DIRECTION('',(1.,1.90750687963558E-16,2.35515798198656E-32));
#121125=DIRECTION('center_axis',(0.,1.23467863058847E-16,-1.));
#121126=DIRECTION('ref_axis',(0.,1.,0.));
#121127=DIRECTION('center_axis',(0.74298130529014,0.669312169312168,0.));
#121128=DIRECTION('ref_axis',(-0.669312169312168,0.742981305290139,0.));
#121129=DIRECTION('center_axis',(0.,0.,-1.));
#121130=DIRECTION('ref_axis',(0.,1.,0.));
#121131=DIRECTION('center_axis',(0.,0.,1.));
#121132=DIRECTION('ref_axis',(0.,1.,0.));
#121133=DIRECTION('center_axis',(0.,1.23467863058847E-16,-1.));
#121134=DIRECTION('ref_axis',(0.,1.,0.));
#121135=DIRECTION('center_axis',(0.,1.,0.));
#121136=DIRECTION('ref_axis',(0.,0.,1.));
#121137=DIRECTION('center_axis',(0.,0.,1.));
#121138=DIRECTION('ref_axis',(0.,1.,0.));
#121139=DIRECTION('center_axis',(0.,0.,-1.));
#121140=DIRECTION('ref_axis',(0.,1.,0.));
#121141=DIRECTION('center_axis',(0.,1.23467863058847E-16,-1.));
#121142=DIRECTION('ref_axis',(-0.406625030395211,-0.913595142640379,0.));
#121143=DIRECTION('center_axis',(0.,-1.,0.));
#121144=DIRECTION('ref_axis',(0.,0.,-1.));
#121145=DIRECTION('center_axis',(0.,0.,-1.));
#121146=DIRECTION('ref_axis',(0.,1.,0.));
#121147=DIRECTION('center_axis',(0.,0.,1.));
#121148=DIRECTION('ref_axis',(0.,1.,0.));
#121149=DIRECTION('center_axis',(0.,1.,0.));
#121150=DIRECTION('ref_axis',(0.,0.,1.));
#121151=DIRECTION('',(0.,1.,1.23467863058847E-16));
#121152=DIRECTION('',(0.,-1.,-1.23467863058847E-16));
#121153=DIRECTION('center_axis',(0.,1.23467863058847E-16,-1.));
#121154=DIRECTION('ref_axis',(0.,1.,0.));
#121155=DIRECTION('center_axis',(7.13942001922908E-31,-4.12830650407183E-45,
1.));
#121156=DIRECTION('ref_axis',(5.78241158658936E-15,1.,0.));
#121157=DIRECTION('center_axis',(-0.742981305290128,0.669312169312181,0.));
#121158=DIRECTION('ref_axis',(-0.669312169312181,-0.742981305290128,0.));
#121159=DIRECTION('center_axis',(0.,0.,-1.));
#121160=DIRECTION('ref_axis',(0.,1.,0.));
#121161=DIRECTION('center_axis',(0.,1.,0.));
#121162=DIRECTION('ref_axis',(0.,0.,1.));
#121163=DIRECTION('center_axis',(0.,1.,0.));
#121164=DIRECTION('ref_axis',(0.,0.,1.));
#121165=DIRECTION('center_axis',(0.,1.,0.));
#121166=DIRECTION('ref_axis',(0.,0.,1.));
#121167=DIRECTION('',(0.,-1.,-1.23467863058847E-16));
#121168=DIRECTION('',(0.,1.,1.23467863058847E-16));
#121169=DIRECTION('center_axis',(0.,1.23467863058847E-16,-1.));
#121170=DIRECTION('ref_axis',(0.,1.,0.));
#121171=DIRECTION('center_axis',(-0.699822617100527,0.714316669688289,0.));
#121172=DIRECTION('ref_axis',(-0.714316669688289,-0.699822617100527,0.));
#121173=DIRECTION('center_axis',(0.,0.,-1.));
#121174=DIRECTION('ref_axis',(0.,1.,0.));
#121175=DIRECTION('center_axis',(-1.20627640644894E-30,-1.17852753964151E-44,
1.));
#121176=DIRECTION('ref_axis',(-9.76996261670138E-15,1.,-4.97841222228891E-60));
#121177=DIRECTION('center_axis',(0.,1.23467863058847E-16,-1.));
#121178=DIRECTION('ref_axis',(0.,1.,0.));
#121179=DIRECTION('center_axis',(-1.,0.,0.));
#121180=DIRECTION('ref_axis',(0.,0.,1.));
#121181=DIRECTION('center_axis',(0.,0.,1.));
#121182=DIRECTION('ref_axis',(0.,1.,0.));
#121183=DIRECTION('center_axis',(0.,0.,-1.));
#121184=DIRECTION('ref_axis',(0.,1.,0.));
#121185=DIRECTION('center_axis',(0.,1.23467863058847E-16,-1.));
#121186=DIRECTION('ref_axis',(0.,1.,0.));
#121187=DIRECTION('center_axis',(1.,0.,0.));
#121188=DIRECTION('ref_axis',(0.,0.,-1.));
#121189=DIRECTION('center_axis',(0.,0.,-1.));
#121190=DIRECTION('ref_axis',(0.,1.,0.));
#121191=DIRECTION('center_axis',(0.,0.,1.));
#121192=DIRECTION('ref_axis',(0.,1.,0.));
#121193=DIRECTION('center_axis',(1.,0.,-1.17757899099328E-32));
#121194=DIRECTION('ref_axis',(0.,1.,0.));
#121195=DIRECTION('',(-1.,9.53753439817791E-17,1.17757899099328E-32));
#121196=DIRECTION('',(1.,-9.53753439817791E-17,-1.17757899099328E-32));
#121197=DIRECTION('center_axis',(0.,1.23467863058847E-16,-1.));
#121198=DIRECTION('ref_axis',(0.,1.,0.));
#121199=DIRECTION('center_axis',(0.,0.,-1.));
#121200=DIRECTION('ref_axis',(0.,1.,0.));
#121201=DIRECTION('center_axis',(-1.,1.22464679914735E-16,1.51204523292581E-32));
#121202=DIRECTION('ref_axis',(-1.22464679914735E-16,-1.,0.));
#121203=DIRECTION('center_axis',(0.,0.,1.));
#121204=DIRECTION('ref_axis',(0.,1.,0.));
#121205=DIRECTION('center_axis',(0.,1.23467863058847E-16,-1.));
#121206=DIRECTION('ref_axis',(0.,1.,0.));
#121207=DIRECTION('center_axis',(0.,0.,-1.));
#121208=DIRECTION('ref_axis',(0.,1.,0.));
#121209=DIRECTION('center_axis',(-1.,1.22464679914735E-16,1.51204523292581E-32));
#121210=DIRECTION('ref_axis',(-1.22464679914735E-16,-1.,0.));
#121211=DIRECTION('center_axis',(0.,0.,1.));
#121212=DIRECTION('ref_axis',(0.,1.,0.));
#121213=DIRECTION('center_axis',(0.,1.23467863058847E-16,-1.));
#121214=DIRECTION('ref_axis',(1.22464679914735E-16,-1.,-1.24777965780772E-16));
#121215=DIRECTION('center_axis',(-0.999425898115847,-0.0338802918424838,
7.7054558576033E-15));
#121216=DIRECTION('ref_axis',(0.0338802918424838,-0.999425898115847,2.67737997453887E-33));
#121217=DIRECTION('center_axis',(3.13384100142148E-32,-1.21933779888604E-16,
1.));
#121218=DIRECTION('ref_axis',(2.04281036531029E-14,1.,1.21933779888604E-16));
#121219=DIRECTION('center_axis',(0.,1.22014183466588E-16,-1.));
#121220=DIRECTION('ref_axis',(0.,1.,1.22014183466588E-16));
#121221=DIRECTION('center_axis',(0.,1.23467863058847E-16,-1.));
#121222=DIRECTION('ref_axis',(0.,1.,0.));
#121223=DIRECTION('center_axis',(-0.87305990868679,-0.487612957009772,0.));
#121224=DIRECTION('ref_axis',(0.487612957009772,-0.87305990868679,0.));
#121225=DIRECTION('center_axis',(0.,0.,1.));
#121226=DIRECTION('ref_axis',(0.,1.,0.));
#121227=DIRECTION('center_axis',(0.,0.,-1.));
#121228=DIRECTION('ref_axis',(0.,1.,0.));
#121229=DIRECTION('center_axis',(0.,1.23467863058847E-16,-1.));
#121230=DIRECTION('ref_axis',(0.,1.,0.));
#121231=DIRECTION('center_axis',(-0.55837318130784,-0.829589892896582,0.));
#121232=DIRECTION('ref_axis',(0.829589892896582,-0.55837318130784,0.));
#121233=DIRECTION('center_axis',(4.38645965981435E-31,-1.5583835234929E-45,
1.));
#121234=DIRECTION('ref_axis',(3.5527136788005E-15,1.,-1.24460305557223E-60));
#121235=DIRECTION('center_axis',(0.,0.,-1.));
#121236=DIRECTION('ref_axis',(0.,1.,0.));
#121237=DIRECTION('center_axis',(0.,1.23467863058847E-16,-1.));
#121238=DIRECTION('ref_axis',(0.,1.,0.));
#121239=DIRECTION('center_axis',(-0.03879684915621,-0.999247118832749,-5.83634271056011E-15));
#121240=DIRECTION('ref_axis',(0.999247118832749,-0.03879684915621,-4.4574149748685E-34));
#121241=DIRECTION('center_axis',(6.64132094812011E-31,-3.57235825122499E-45,
1.));
#121242=DIRECTION('ref_axis',(5.37898752240871E-15,1.,2.61366641670168E-59));
#121243=DIRECTION('center_axis',(0.,0.,-1.));
#121244=DIRECTION('ref_axis',(0.,1.,0.));
#121245=DIRECTION('center_axis',(0.,1.23467863058847E-16,-1.));
#121246=DIRECTION('ref_axis',(0.,1.,1.24777965780772E-16));
#121247=DIRECTION('center_axis',(0.0387968491562139,-0.999247118832749,
0.));
#121248=DIRECTION('ref_axis',(0.999247118832749,0.0387968491562139,0.));
#121249=DIRECTION('center_axis',(4.09030343683335E-32,-1.21933779888604E-16,
1.));
#121250=DIRECTION('ref_axis',(2.66628532023081E-14,1.,1.21933779888604E-16));
#121251=DIRECTION('center_axis',(0.,1.22014183466588E-16,-1.));
#121252=DIRECTION('ref_axis',(0.,1.,1.22014183466588E-16));
#121253=DIRECTION('center_axis',(0.,1.23467863058847E-16,-1.));
#121254=DIRECTION('ref_axis',(0.,1.,0.));
#121255=DIRECTION('center_axis',(0.55837318130784,-0.829589892896582,0.));
#121256=DIRECTION('ref_axis',(0.829589892896582,0.55837318130784,0.));
#121257=DIRECTION('center_axis',(-1.32826418962402E-31,-1.42894330048999E-46,
1.));
#121258=DIRECTION('ref_axis',(-1.07579750448174E-15,1.,9.14005368935855E-61));
#121259=DIRECTION('center_axis',(0.,0.,-1.));
#121260=DIRECTION('ref_axis',(0.,1.,0.));
#121261=DIRECTION('center_axis',(0.,1.23467863058847E-16,-1.));
#121262=DIRECTION('ref_axis',(0.,1.,0.));
#121263=DIRECTION('center_axis',(0.848949186868297,-0.528474481991002,-8.14895191435076E-15));
#121264=DIRECTION('ref_axis',(0.528474481991002,0.848949186868297,-1.25969070483717E-30));
#121265=DIRECTION('center_axis',(-1.53526088093502E-30,-1.90901981627881E-44,
1.));
#121266=DIRECTION('ref_axis',(-1.24344978758017E-14,1.,2.98704733337335E-59));
#121267=DIRECTION('center_axis',(0.,0.,-1.));
#121268=DIRECTION('ref_axis',(0.,1.,0.));
#121269=DIRECTION('center_axis',(0.,1.23467863058847E-16,-1.));
#121270=DIRECTION('ref_axis',(0.,1.,0.));
#121271=DIRECTION('center_axis',(0.992522955047552,-0.122058116090968,0.));
#121272=DIRECTION('ref_axis',(0.122058116090968,0.992522955047552,0.));
#121273=DIRECTION('center_axis',(-1.32826418962402E-31,-1.42894330048999E-46,
1.));
#121274=DIRECTION('ref_axis',(-1.07579750448174E-15,1.,5.05619991326218E-61));
#121275=DIRECTION('center_axis',(0.,0.,-1.));
#121276=DIRECTION('ref_axis',(0.,1.,0.));
#121277=DIRECTION('center_axis',(0.,1.23467863058847E-16,-1.));
#121278=DIRECTION('ref_axis',(0.,1.,1.35086937000622E-16));
#121279=DIRECTION('center_axis',(1.70695598787294E-31,-1.32203597548532E-16,
1.));
#121280=DIRECTION('ref_axis',(-1.95399252334027E-14,1.,1.32203597548532E-16));
#121281=DIRECTION('center_axis',(0.,1.32487572930867E-16,-1.));
#121282=DIRECTION('ref_axis',(0.,1.,1.32487572930867E-16));
#121283=DIRECTION('center_axis',(0.,1.23467863058847E-16,-1.));
#121284=DIRECTION('ref_axis',(1.22464679914735E-16,-1.,-1.25162611019057E-16));
#121285=DIRECTION('center_axis',(-0.999425898115848,-0.0338802918424761,
0.));
#121286=DIRECTION('ref_axis',(0.0338802918424761,-0.999425898115848,0.));
#121287=DIRECTION('center_axis',(2.53053284261581E-32,-1.22229112323298E-16,
1.));
#121288=DIRECTION('ref_axis',(2.04281036531029E-14,1.,1.22229112323298E-16));
#121289=DIRECTION('center_axis',(0.,1.22309905988566E-16,-1.));
#121290=DIRECTION('ref_axis',(0.,1.,1.22309905988566E-16));
#121291=DIRECTION('center_axis',(0.,1.23467863058847E-16,-1.));
#121292=DIRECTION('ref_axis',(0.,1.,0.));
#121293=DIRECTION('center_axis',(-0.87305990868679,-0.487612957009772,0.));
#121294=DIRECTION('ref_axis',(0.487612957009772,-0.87305990868679,0.));
#121295=DIRECTION('center_axis',(-4.46213751201822E-31,-1.61261972815309E-45,
1.));
#121296=DIRECTION('ref_axis',(-3.61400724161835E-15,1.,1.6490990486332E-59));
#121297=DIRECTION('center_axis',(0.,0.,-1.));
#121298=DIRECTION('ref_axis',(0.,1.,0.));
#121299=DIRECTION('center_axis',(0.,1.23467863058847E-16,-1.));
#121300=DIRECTION('ref_axis',(0.,1.,0.));
#121301=DIRECTION('center_axis',(-0.55837318130784,-0.829589892896582,0.));
#121302=DIRECTION('ref_axis',(0.829589892896582,-0.55837318130784,0.));
#121303=DIRECTION('center_axis',(4.38645965981435E-31,-1.5583835234929E-45,
1.));
#121304=DIRECTION('ref_axis',(3.5527136788005E-15,1.,-1.24460305557223E-60));
#121305=DIRECTION('center_axis',(0.,0.,-1.));
#121306=DIRECTION('ref_axis',(0.,1.,0.));
#121307=DIRECTION('center_axis',(0.,1.23467863058847E-16,-1.));
#121308=DIRECTION('ref_axis',(0.,1.,0.));
#121309=DIRECTION('center_axis',(-0.0387968491561946,-0.99924711883275,
0.));
#121310=DIRECTION('ref_axis',(0.99924711883275,-0.0387968491561946,0.));
#121311=DIRECTION('center_axis',(-8.92427502403635E-31,-6.45047891261223E-45,
1.));
#121312=DIRECTION('ref_axis',(-7.2280144832367E-15,1.,3.73380916671669E-60));
#121313=DIRECTION('center_axis',(0.,0.,-1.));
#121314=DIRECTION('ref_axis',(0.,1.,0.));
#121315=DIRECTION('center_axis',(0.,1.23467863058847E-16,-1.));
#121316=DIRECTION('ref_axis',(0.,1.,1.25162611019057E-16));
#121317=DIRECTION('center_axis',(0.0387968491562177,-0.999247118832749,
0.));
#121318=DIRECTION('ref_axis',(0.999247118832749,0.0387968491562177,0.));
#121319=DIRECTION('center_axis',(3.29067448743359E-32,-1.22229112323298E-16,
1.));
#121320=DIRECTION('ref_axis',(2.65644604115968E-14,1.,1.22229112323298E-16));
#121321=DIRECTION('center_axis',(0.,1.22309905988566E-16,-1.));
#121322=DIRECTION('ref_axis',(0.,1.,1.22309905988566E-16));
#121323=DIRECTION('center_axis',(0.,1.23467863058847E-16,-1.));
#121324=DIRECTION('ref_axis',(0.,1.,0.));
#121325=DIRECTION('center_axis',(0.55837318130784,-0.829589892896582,0.));
#121326=DIRECTION('ref_axis',(0.829589892896582,0.55837318130784,0.));
#121327=DIRECTION('center_axis',(0.,0.,1.));
#121328=DIRECTION('ref_axis',(0.,1.,0.));
#121329=DIRECTION('center_axis',(0.,0.,-1.));
#121330=DIRECTION('ref_axis',(0.,1.,0.));
#121331=DIRECTION('center_axis',(0.,1.23467863058847E-16,-1.));
#121332=DIRECTION('ref_axis',(0.,1.,0.));
#121333=DIRECTION('center_axis',(0.848949186868305,-0.528474481990989,0.));
#121334=DIRECTION('ref_axis',(0.528474481990989,0.848949186868305,0.));
#121335=DIRECTION('center_axis',(-1.53526088093502E-30,-1.90901981627881E-44,
1.));
#121336=DIRECTION('ref_axis',(-1.24344978758017E-14,1.,3.23596794448779E-59));
#121337=DIRECTION('center_axis',(0.,0.,-1.));
#121338=DIRECTION('ref_axis',(0.,1.,0.));
#121339=DIRECTION('center_axis',(0.,1.23467863058847E-16,-1.));
#121340=DIRECTION('ref_axis',(0.,1.,0.));
#121341=DIRECTION('center_axis',(0.992522955047553,-0.12205811609096,0.));
#121342=DIRECTION('ref_axis',(0.12205811609096,0.992522955047552,0.));
#121343=DIRECTION('center_axis',(1.42788400384582E-30,-1.65132260162873E-44,
1.));
#121344=DIRECTION('ref_axis',(1.15648231731787E-14,1.,-2.48920611114446E-60));
#121345=DIRECTION('center_axis',(0.,0.,-1.));
#121346=DIRECTION('ref_axis',(0.,1.,0.));
#121347=DIRECTION('center_axis',(0.,1.23467863058847E-16,-1.));
#121348=DIRECTION('ref_axis',(0.,1.,1.36448859403292E-16));
#121349=DIRECTION('center_axis',(-1.91158623550752E-31,-1.33250839261027E-16,
1.));
#121350=DIRECTION('ref_axis',(1.95399252334028E-14,1.,1.33250839261027E-16));
#121351=DIRECTION('center_axis',(0.,1.33539336354386E-16,-1.));
#121352=DIRECTION('ref_axis',(0.,1.,1.33539336354386E-16));
#121353=DIRECTION('center_axis',(0.,1.23467863058847E-16,-1.));
#121354=DIRECTION('ref_axis',(0.,1.,0.));
#121355=DIRECTION('center_axis',(-0.689680595319751,-0.724113717892013,
0.));
#121356=DIRECTION('ref_axis',(0.724113717892013,-0.689680595319751,0.));
#121357=DIRECTION('center_axis',(0.,0.,-1.));
#121358=DIRECTION('ref_axis',(0.,1.,0.));
#121359=DIRECTION('center_axis',(0.,0.,1.));
#121360=DIRECTION('ref_axis',(0.,1.,0.));
#121361=DIRECTION('center_axis',(-0.68968059531976,-0.724113717892004,-8.94047733597239E-17));
#121362=DIRECTION('ref_axis',(0.724113717892004,-0.68968059531976,2.34589631629098E-32));
#121363=DIRECTION('center_axis',(-0.689680595319751,-0.724113717892013,
0.));
#121364=DIRECTION('ref_axis',(0.724113717892013,-0.689680595319751,0.));
#121365=DIRECTION('',(0.689680595319752,0.724113717892012,8.94047733597238E-17));
#121366=DIRECTION('',(-0.689680595319752,-0.724113717892012,-8.94047733597238E-17));
#121367=DIRECTION('center_axis',(0.,1.23467863058847E-16,-1.));
#121368=DIRECTION('ref_axis',(0.,1.,0.));
#121369=DIRECTION('center_axis',(1.78485500480727E-31,-2.58019156504489E-46,
1.));
#121370=DIRECTION('ref_axis',(1.44560289664734E-15,1.,-3.88938454866321E-62));
#121371=DIRECTION('center_axis',(-0.635568809204586,0.772044227208691,0.));
#121372=DIRECTION('ref_axis',(-0.772044227208691,-0.635568809204586,0.));
#121373=DIRECTION('center_axis',(0.,0.,-1.));
#121374=DIRECTION('ref_axis',(0.,1.,0.));
#121375=DIRECTION('center_axis',(0.,1.23467863058847E-16,-1.));
#121376=DIRECTION('ref_axis',(0.,1.,0.));
#121377=DIRECTION('center_axis',(-0.120708341042265,0.992688015643799,0.));
#121378=DIRECTION('ref_axis',(-0.992688015643799,-0.120708341042265,0.));
#121379=DIRECTION('center_axis',(0.,0.,-1.));
#121380=DIRECTION('ref_axis',(0.,1.,0.));
#121381=DIRECTION('center_axis',(-2.19322982990717E-31,-3.89595880873225E-46,
1.));
#121382=DIRECTION('ref_axis',(-1.77635683940025E-15,1.,7.77876909732643E-62));
#121383=DIRECTION('center_axis',(0.,1.23467863058847E-16,-1.));
#121384=DIRECTION('ref_axis',(0.,1.,0.));
#121385=DIRECTION('center_axis',(1.,0.,0.));
#121386=DIRECTION('ref_axis',(0.,0.,-1.));
#121387=DIRECTION('center_axis',(0.,0.,-1.));
#121388=DIRECTION('ref_axis',(0.,1.,0.));
#121389=DIRECTION('center_axis',(0.,0.,1.));
#121390=DIRECTION('ref_axis',(0.,1.,0.));
#121391=DIRECTION('center_axis',(1.,0.,4.58212374768871E-32));
#121392=DIRECTION('ref_axis',(0.,1.,0.));
#121393=DIRECTION('center_axis',(1.,0.,0.));
#121394=DIRECTION('ref_axis',(0.,0.,-1.));
#121395=DIRECTION('',(-1.,-3.71118737634973E-16,-4.58212374768871E-32));
#121396=DIRECTION('',(1.,3.71118737634973E-16,4.58212374768871E-32));
#121397=DIRECTION('center_axis',(0.,1.23467863058847E-16,-1.));
#121398=DIRECTION('ref_axis',(0.,1.,0.));
#121399=DIRECTION('center_axis',(0.,0.,-1.));
#121400=DIRECTION('ref_axis',(0.,1.,0.));
#121401=DIRECTION('center_axis',(0.,0.,1.));
#121402=DIRECTION('ref_axis',(0.,1.,0.));
#121403=DIRECTION('center_axis',(0.,1.23467863058847E-16,-1.));
#121404=DIRECTION('ref_axis',(0.,1.,0.));
#121405=DIRECTION('center_axis',(-1.,0.,0.));
#121406=DIRECTION('ref_axis',(0.,0.,1.));
#121407=DIRECTION('center_axis',(0.,0.,-1.));
#121408=DIRECTION('ref_axis',(0.,1.,0.));
#121409=DIRECTION('center_axis',(0.,0.,1.));
#121410=DIRECTION('ref_axis',(0.,1.,0.));
#121411=DIRECTION('center_axis',(-1.,0.,4.58212374768871E-32));
#121412=DIRECTION('ref_axis',(0.,-1.,0.));
#121413=DIRECTION('center_axis',(-1.,0.,0.));
#121414=DIRECTION('ref_axis',(0.,0.,1.));
#121415=DIRECTION('',(1.,-3.71118737634973E-16,-4.58212374768871E-32));
#121416=DIRECTION('',(-1.,3.71118737634973E-16,4.58212374768871E-32));
#121417=DIRECTION('center_axis',(0.,1.23467863058847E-16,-1.));
#121418=DIRECTION('ref_axis',(0.,1.,0.));
#121419=DIRECTION('center_axis',(0.120708341042269,0.992688015643799,0.));
#121420=DIRECTION('ref_axis',(-0.992688015643799,0.120708341042269,0.));
#121421=DIRECTION('center_axis',(0.,0.,-1.));
#121422=DIRECTION('ref_axis',(0.,1.,0.));
#121423=DIRECTION('center_axis',(1.78485500480727E-31,-2.58019156504489E-46,
1.));
#121424=DIRECTION('ref_axis',(1.44560289664734E-15,1.,-3.88938454866321E-62));
#121425=DIRECTION('center_axis',(0.,1.23467863058847E-16,-1.));
#121426=DIRECTION('ref_axis',(0.,1.,0.));
#121427=DIRECTION('center_axis',(0.635568809204587,0.77204422720869,0.));
#121428=DIRECTION('ref_axis',(-0.77204422720869,0.635568809204587,0.));
#121429=DIRECTION('center_axis',(0.,0.,-1.));
#121430=DIRECTION('ref_axis',(0.,1.,0.));
#121431=DIRECTION('center_axis',(6.57968948972152E-31,-3.50636292785902E-45,
1.));
#121432=DIRECTION('ref_axis',(5.32907051820075E-15,1.,-4.3561106945028E-60));
#121433=DIRECTION('center_axis',(0.,1.23467863058847E-16,-1.));
#121434=DIRECTION('ref_axis',(0.0361435302645206,-0.999346609150208,0.));
#121435=DIRECTION('center_axis',(0.689680595319753,-0.724113717892011,0.));
#121436=DIRECTION('ref_axis',(0.724113717892011,0.689680595319753,0.));
#121437=DIRECTION('center_axis',(0.,0.,-1.));
#121438=DIRECTION('ref_axis',(0.,1.,0.));
#121439=DIRECTION('center_axis',(1.78485500480727E-31,-2.58019156504489E-46,
1.));
#121440=DIRECTION('ref_axis',(1.44560289664734E-15,1.,-3.88938454866321E-62));
#121441=DIRECTION('center_axis',(0.689680595319751,-0.724113717892013,-8.9404773359724E-17));
#121442=DIRECTION('ref_axis',(0.724113717892013,0.689680595319751,4.19197973383322E-33));
#121443=DIRECTION('center_axis',(0.689680595319753,-0.724113717892011,0.));
#121444=DIRECTION('ref_axis',(0.724113717892011,0.689680595319753,0.));
#121445=DIRECTION('',(-0.689680595319751,0.724113717892013,8.9404773359724E-17));
#121446=DIRECTION('',(0.689680595319751,-0.724113717892013,-8.9404773359724E-17));
#121447=DIRECTION('center_axis',(0.,1.23467863058847E-16,-1.));
#121448=DIRECTION('ref_axis',(0.,1.,0.));
#121449=DIRECTION('center_axis',(0.,0.,-1.));
#121450=DIRECTION('ref_axis',(0.,1.,0.));
#121451=DIRECTION('center_axis',(-8.92427502403635E-32,-6.45047891261222E-47,
1.));
#121452=DIRECTION('ref_axis',(-7.2280144832367E-16,1.,-6.80642296016062E-62));
#121453=DIRECTION('center_axis',(0.,1.23467863058847E-16,-1.));
#121454=DIRECTION('ref_axis',(0.,1.,0.));
#121455=DIRECTION('center_axis',(1.92747052886312E-15,-1.,0.));
#121456=DIRECTION('ref_axis',(1.,1.92747052886312E-15,0.));
#121457=DIRECTION('center_axis',(0.,0.,-1.));
#121458=DIRECTION('ref_axis',(0.,1.,0.));
#121459=DIRECTION('center_axis',(0.,0.,1.));
#121460=DIRECTION('ref_axis',(0.,1.,0.));
#121461=DIRECTION('center_axis',(6.11546355285877E-17,1.,0.));
#121462=DIRECTION('ref_axis',(0.,0.,1.));
#121463=DIRECTION('center_axis',(0.,-1.,0.));
#121464=DIRECTION('ref_axis',(0.,0.,-1.));
#121465=DIRECTION('',(6.11546355285877E-17,1.,1.23467863058847E-16));
#121466=DIRECTION('',(-6.11546355285877E-17,-1.,-1.23467863058847E-16));
#121467=DIRECTION('center_axis',(0.,1.23467863058847E-16,-1.));
#121468=DIRECTION('ref_axis',(0.,1.,0.));
#121469=DIRECTION('center_axis',(-2.63266113209072E-30,-5.61352927370078E-44,
1.));
#121470=DIRECTION('ref_axis',(-2.13226427255483E-14,1.,-2.98704733337335E-59));
#121471=DIRECTION('center_axis',(-0.992688015643799,0.120708341042267,1.45413606216828E-17));
#121472=DIRECTION('ref_axis',(-0.120708341042267,-0.992688015643799,-1.06337197076866E-33));
#121473=DIRECTION('center_axis',(0.,0.,-1.));
#121474=DIRECTION('ref_axis',(0.,1.,0.));
#121475=DIRECTION('center_axis',(0.,1.23467863058847E-16,-1.));
#121476=DIRECTION('ref_axis',(0.,1.,0.));
#121477=DIRECTION('center_axis',(-0.802069210224766,0.597231095983306,0.));
#121478=DIRECTION('ref_axis',(-0.597231095983306,-0.802069210224766,0.));
#121479=DIRECTION('center_axis',(0.,0.,-1.));
#121480=DIRECTION('ref_axis',(0.,1.,0.));
#121481=DIRECTION('center_axis',(8.77291931962869E-31,-6.2335340939716E-45,
1.));
#121482=DIRECTION('ref_axis',(7.105427357601E-15,1.,-4.97841222228891E-60));
#121483=DIRECTION('center_axis',(0.,1.23467863058847E-16,-1.));
#121484=DIRECTION('ref_axis',(0.,1.,0.));
#121485=DIRECTION('center_axis',(0.689680595319753,0.724113717892012,0.));
#121486=DIRECTION('ref_axis',(-0.724113717892012,0.689680595319752,0.));
#121487=DIRECTION('center_axis',(0.,0.,-1.));
#121488=DIRECTION('ref_axis',(0.,1.,0.));
#121489=DIRECTION('center_axis',(0.,0.,1.));
#121490=DIRECTION('ref_axis',(0.,1.,0.));
#121491=DIRECTION('center_axis',(0.68968059531976,0.724113717892004,8.94047733597239E-17));
#121492=DIRECTION('ref_axis',(-0.724113717892004,0.68968059531976,-2.34589631629098E-32));
#121493=DIRECTION('center_axis',(0.689680595319752,0.724113717892012,0.));
#121494=DIRECTION('ref_axis',(-0.724113717892012,0.689680595319752,0.));
#121495=DIRECTION('',(-0.689680595319752,-0.724113717892012,-8.94047733597238E-17));
#121496=DIRECTION('',(0.689680595319752,0.724113717892012,8.94047733597238E-17));
#121497=DIRECTION('center_axis',(0.,1.23467863058847E-16,-1.));
#121498=DIRECTION('ref_axis',(0.0950205176920742,-0.995475314218052,0.));
#121499=DIRECTION('center_axis',(0.,0.,-1.));
#121500=DIRECTION('ref_axis',(0.,1.,0.));
#121501=DIRECTION('center_axis',(0.,0.,1.));
#121502=DIRECTION('ref_axis',(0.,1.,0.));
#121503=DIRECTION('center_axis',(0.,1.23467863058847E-16,-1.));
#121504=DIRECTION('ref_axis',(0.,1.,0.));
#121505=DIRECTION('center_axis',(-1.60636950432654E-30,-2.08995516768636E-44,
1.));
#121506=DIRECTION('ref_axis',(-1.30104260698261E-14,1.,2.24028550003001E-59));
#121507=DIRECTION('center_axis',(-0.689680595319753,0.724113717892011,0.));
#121508=DIRECTION('ref_axis',(-0.724113717892011,-0.689680595319753,0.));
#121509=DIRECTION('center_axis',(0.,0.,-1.));
#121510=DIRECTION('ref_axis',(0.,1.,0.));
#121511=DIRECTION('center_axis',(-0.689680595319751,0.724113717892013,8.9404773359724E-17));
#121512=DIRECTION('ref_axis',(-0.724113717892013,-0.689680595319751,-4.19197973383322E-33));
#121513=DIRECTION('center_axis',(-0.689680595319752,0.724113717892012,0.));
#121514=DIRECTION('ref_axis',(-0.724113717892012,-0.689680595319752,0.));
#121515=DIRECTION('',(0.689680595319751,-0.724113717892013,-8.9404773359724E-17));
#121516=DIRECTION('',(-0.689680595319751,0.724113717892013,8.9404773359724E-17));
#121517=DIRECTION('center_axis',(0.,1.23467863058847E-16,-1.));
#121518=DIRECTION('ref_axis',(0.,1.,0.));
#121519=DIRECTION('center_axis',(0.802069210224767,0.597231095983305,0.));
#121520=DIRECTION('ref_axis',(-0.597231095983305,0.802069210224766,0.));
#121521=DIRECTION('center_axis',(0.,0.,-1.));
#121522=DIRECTION('ref_axis',(0.,1.,0.));
#121523=DIRECTION('center_axis',(0.,0.,1.));
#121524=DIRECTION('ref_axis',(0.,1.,0.));
#121525=DIRECTION('center_axis',(0.,1.23467863058847E-16,-1.));
#121526=DIRECTION('ref_axis',(0.,1.,0.));
#121527=DIRECTION('center_axis',(0.992688015643799,0.120708341042267,0.));
#121528=DIRECTION('ref_axis',(-0.120708341042267,0.992688015643799,0.));
#121529=DIRECTION('center_axis',(0.,0.,-1.));
#121530=DIRECTION('ref_axis',(0.,1.,0.));
#121531=DIRECTION('center_axis',(0.,0.,1.));
#121532=DIRECTION('ref_axis',(0.,1.,0.));
#121533=DIRECTION('center_axis',(0.,1.23467863058847E-16,-1.));
#121534=DIRECTION('ref_axis',(-0.663057938251906,-0.748568080084325,0.));
#121535=DIRECTION('center_axis',(0.,-1.,0.));
#121536=DIRECTION('ref_axis',(0.,0.,-1.));
#121537=DIRECTION('center_axis',(0.,0.,-1.));
#121538=DIRECTION('ref_axis',(0.,1.,0.));
#121539=DIRECTION('center_axis',(0.,0.,1.));
#121540=DIRECTION('ref_axis',(0.,1.,0.));
#121541=DIRECTION('center_axis',(6.11546355285877E-17,1.,0.));
#121542=DIRECTION('ref_axis',(0.,0.,1.));
#121543=DIRECTION('center_axis',(0.,-1.,0.));
#121544=DIRECTION('ref_axis',(0.,0.,-1.));
#121545=DIRECTION('',(6.11546355285877E-17,1.,1.23467863058847E-16));
#121546=DIRECTION('',(-6.11546355285877E-17,-1.,-1.23467863058847E-16));
#121547=DIRECTION('center_axis',(0.,1.23467863058847E-16,-1.));
#121548=DIRECTION('ref_axis',(0.,1.,0.));
#121549=DIRECTION('center_axis',(0.,0.,-1.));
#121550=DIRECTION('ref_axis',(0.,1.,0.));
#121551=DIRECTION('center_axis',(-2.23106875600908E-31,-4.03154932038264E-46,
1.));
#121552=DIRECTION('ref_axis',(-1.80700362080917E-15,1.,2.33363072919793E-61));
#121553=DIRECTION('center_axis',(0.,-1.23467863058847E-16,1.));
#121554=DIRECTION('ref_axis',(1.22464679914735E-16,1.,1.21161349753609E-16));
#121555=DIRECTION('center_axis',(1.55777898081371E-32,1.19083105035399E-16,
-1.));
#121556=DIRECTION('ref_axis',(3.5527136788005E-15,-1.,-1.19083105035399E-16));
#121557=DIRECTION('center_axis',(0.,-1.18321745853506E-16,1.));
#121558=DIRECTION('ref_axis',(0.,1.,1.18321745853506E-16));
#121559=DIRECTION('center_axis',(-0.982297019165463,0.187330099393146,5.41061232187394E-15));
#121560=DIRECTION('ref_axis',(-0.187330099393146,-0.982297019165463,5.34128931770042E-31));
#121561=DIRECTION('center_axis',(0.,-1.23467863058847E-16,1.));
#121562=DIRECTION('ref_axis',(0.,-1.,0.));
#121563=DIRECTION('center_axis',(-0.777162624242383,0.6292998136665,1.36800580655942E-15));
#121564=DIRECTION('ref_axis',(-0.6292998136665,-0.777162624242383,-6.36525986617897E-32));
#121565=DIRECTION('center_axis',(0.,0.,-1.));
#121566=DIRECTION('ref_axis',(0.,-1.,0.));
#121567=DIRECTION('center_axis',(-7.93261518924905E-31,-5.09657996678154E-45,
1.));
#121568=DIRECTION('ref_axis',(-6.42484205421795E-15,1.,4.3561106945028E-60));
#121569=DIRECTION('center_axis',(0.,-1.23467863058847E-16,1.));
#121570=DIRECTION('ref_axis',(0.,-1.,0.));
#121571=DIRECTION('center_axis',(-0.6350303583426,0.772487180465326,0.));
#121572=DIRECTION('ref_axis',(-0.772487180465326,-0.6350303583426,0.));
#121573=DIRECTION('center_axis',(0.,0.,-1.));
#121574=DIRECTION('ref_axis',(0.,-1.,0.));
#121575=DIRECTION('center_axis',(-3.28984474486076E-31,-8.76590731964757E-46,
1.));
#121576=DIRECTION('ref_axis',(-2.66453525910037E-15,1.,-6.22301527786114E-61));
#121577=DIRECTION('center_axis',(0.,-1.23467863058847E-16,1.));
#121578=DIRECTION('ref_axis',(0.,-1.,0.));
#121579=DIRECTION('center_axis',(-0.0394959395290685,0.999219730970479,
-7.30821690739571E-16));
#121580=DIRECTION('ref_axis',(-0.999219730970479,-0.0394959395290685,1.49001220711228E-32));
#121581=DIRECTION('center_axis',(-4.09907119868247E-31,1.3608711024552E-45,
-1.));
#121582=DIRECTION('ref_axis',(-3.31994990204759E-15,-1.,-9.33452291679171E-61));
#121583=DIRECTION('center_axis',(-1.22040233680755E-31,-1.206291116398E-46,
1.));
#121584=DIRECTION('ref_axis',(-9.88437239110456E-16,1.,0.));
#121585=DIRECTION('center_axis',(0.,-1.23467863058847E-16,1.));
#121586=DIRECTION('ref_axis',(0.,-1.,-1.32864206562206E-16));
#121587=DIRECTION('center_axis',(0.0394959395290708,0.999219730970479,0.));
#121588=DIRECTION('ref_axis',(-0.999219730970479,0.0394959395290708,0.));
#121589=DIRECTION('center_axis',(0.,1.29932421951445E-16,-1.));
#121590=DIRECTION('ref_axis',(0.,-1.,-1.29932421951445E-16));
#121591=DIRECTION('center_axis',(2.45193654393607E-31,-1.29750229435012E-16,
1.));
#121592=DIRECTION('ref_axis',(-3.90288690140516E-14,1.,1.29750229435012E-16));
#121593=DIRECTION('center_axis',(0.,-1.23467863058847E-16,1.));
#121594=DIRECTION('ref_axis',(0.,-1.,0.));
#121595=DIRECTION('center_axis',(0.6350303583426,0.772487180465326,-1.66587444809586E-15));
#121596=DIRECTION('ref_axis',(-0.772487180465326,0.6350303583426,9.8727026228538E-31));
#121597=DIRECTION('center_axis',(3.41589266556873E-31,9.45049376705E-46,
-1.));
#121598=DIRECTION('ref_axis',(2.766624918373E-15,-1.,6.22301527786114E-61));
#121599=DIRECTION('center_axis',(1.22040233680755E-31,-1.20629111639801E-46,
1.));
#121600=DIRECTION('ref_axis',(9.88437239110458E-16,1.,-1.75022304689845E-61));
#121601=DIRECTION('center_axis',(0.,-1.23467863058847E-16,1.));
#121602=DIRECTION('ref_axis',(0.,-1.,0.));
#121603=DIRECTION('center_axis',(0.77428749071043,0.632834008037926,3.58179916610815E-15));
#121604=DIRECTION('ref_axis',(-0.632834008037926,0.77428749071043,7.75406439997931E-31));
#121605=DIRECTION('center_axis',(-3.28984474486076E-31,8.76590731964757E-46,
-1.));
#121606=DIRECTION('ref_axis',(-2.66453525910038E-15,-1.,4.66726145839586E-61));
#121607=DIRECTION('center_axis',(-1.09661491495359E-30,-9.73989702183063E-45,
1.));
#121608=DIRECTION('ref_axis',(-8.88178419700125E-15,1.,-2.48920611114446E-60));
#121609=DIRECTION('center_axis',(0.,-1.23467863058847E-16,1.));
#121610=DIRECTION('ref_axis',(0.,-1.,0.));
#121611=DIRECTION('center_axis',(0.999225121087074,0.0393593367388569,-7.28294031357568E-16));
#121612=DIRECTION('ref_axis',(-0.0393593367388569,0.999225121087074,-1.34329260515414E-32));
#121613=DIRECTION('center_axis',(6.83178533113742E-31,3.78019750681997E-45,
-1.));
#121614=DIRECTION('ref_axis',(5.53324983674598E-15,-1.,5.60071375007503E-60));
#121615=DIRECTION('center_axis',(-2.4408046736151E-31,-4.82516446559199E-46,
1.));
#121616=DIRECTION('ref_axis',(-1.97687447822091E-15,1.,-3.11150763893057E-61));
#121617=DIRECTION('center_axis',(0.,-1.23467863058847E-16,1.));
#121618=DIRECTION('ref_axis',(0.,-1.,-1.32864206562206E-16));
#121619=DIRECTION('center_axis',(1.26316997428288E-31,1.29932421951445E-16,
-1.));
#121620=DIRECTION('ref_axis',(-1.95399252334027E-14,-1.,-1.29932421951445E-16));
#121621=DIRECTION('center_axis',(-2.23194489598359E-31,-1.29750229435012E-16,
1.));
#121622=DIRECTION('ref_axis',(3.5527136788005E-14,1.,1.29750229435012E-16));
#121623=DIRECTION('center_axis',(-0.994526788819783,-0.10448189469861,-1.81517644375859E-14));
#121624=DIRECTION('ref_axis',(0.10448189469861,-0.994526788819783,-2.86631910367634E-30));
#121625=DIRECTION('center_axis',(-0.993679318607912,0.112256009954549,1.48651952901285E-13));
#121626=DIRECTION('ref_axis',(-0.112256009954549,-0.993679318607912,-2.2981091857326E-29));
#121627=DIRECTION('center_axis',(0.173003591922937,0.223692887116409,0.959182594418439));
#121628=DIRECTION('ref_axis',(0.884537270739863,0.393052221940888,-0.251204632718837));
#121629=DIRECTION('center_axis',(-0.991556456479175,0.129675724846491,-3.15431192506052E-12));
#121630=DIRECTION('ref_axis',(-0.129675724846491,-0.991556456479175,7.41046500628616E-29));
#121631=DIRECTION('center_axis',(-2.53853736684027E-13,-2.16212897560618E-12,
-1.));
#121632=DIRECTION('ref_axis',(0.129669785749073,0.991557233176073,-2.1767505907557E-12));
#121633=DIRECTION('center_axis',(0.000137331807541708,0.00219823298717573,
0.999997574452913));
#121634=DIRECTION('ref_axis',(0.11217860466933,0.993685625182725,-0.00219976354633589));
#121635=DIRECTION('center_axis',(-0.858927270467749,0.512097592307192,-1.49780811271862E-14));
#121636=DIRECTION('ref_axis',(-0.512097592307192,-0.858927270467749,-6.01293732495529E-30));
#121637=DIRECTION('center_axis',(-0.536899969302814,0.843645910890723,1.46316605705353E-12));
#121638=DIRECTION('ref_axis',(-0.843645910890723,-0.536899969302814,1.20303121328766E-28));
#121639=DIRECTION('center_axis',(-0.040766102180794,0.99916871694073,1.55671748522919E-15));
#121640=DIRECTION('ref_axis',(-0.99916871694073,-0.040766102180794,-1.4838474346331E-32));
#121641=DIRECTION('center_axis',(-0.0297586090124609,0.999557114521048,
-7.26582357398889E-15));
#121642=DIRECTION('ref_axis',(-0.999557114521048,-0.0297586090124609,1.68195404251657E-31));
#121643=DIRECTION('center_axis',(0.,0.,-1.));
#121644=DIRECTION('ref_axis',(0.999557147327688,0.0297575070551087,0.));
#121645=DIRECTION('center_axis',(-0.0210932860527463,-5.46714727619952E-5,
0.999777510396452));
#121646=DIRECTION('ref_axis',(0.998923256585619,0.0413287487753403,0.0210775230292068));
#121647=DIRECTION('center_axis',(0.233238585379144,0.972419540265587,-4.54398481782876E-15));
#121648=DIRECTION('ref_axis',(-0.972419540265587,0.233238585379145,-6.30780798053809E-30));
#121649=DIRECTION('center_axis',(-0.229570335512527,0.973292073867175,1.03212124729447E-14));
#121650=DIRECTION('ref_axis',(-0.973292073867175,-0.229570335512527,2.98849951310675E-30));
#121651=DIRECTION('center_axis',(0.0298379862379757,0.999554748164033,8.0054834066732E-15));
#121652=DIRECTION('ref_axis',(-0.999554748164032,0.0298379862379757,9.39450193490723E-31));
#121653=DIRECTION('center_axis',(0.0407665603815583,0.999168698246025,4.49007546874249E-14));
#121654=DIRECTION('ref_axis',(-0.999168698246025,0.0407665603815583,1.08335075317432E-30));
#121655=DIRECTION('center_axis',(-1.70507880518925E-12,5.55629427464142E-14,
-1.));
#121656=DIRECTION('ref_axis',(0.999168739570264,-0.040765547531825,-1.70593188493018E-12));
#121657=DIRECTION('center_axis',(-0.0206791468565618,-0.000130026885512925,
0.999786155124332));
#121658=DIRECTION('ref_axis',(0.9993253707471,-0.0303600651974135,0.0206656677215903));
#121659=DIRECTION('center_axis',(0.536601093577061,0.843836042351772,-2.84249428416013E-15));
#121660=DIRECTION('ref_axis',(-0.843836042351772,0.536601093577061,2.98189956073675E-31));
#121661=DIRECTION('center_axis',(0.882960425292266,0.469447427693135,-5.17032777304292E-14));
#121662=DIRECTION('ref_axis',(-0.469447427693135,0.882960425292266,-2.22396706740103E-29));
#121663=DIRECTION('center_axis',(0.999360062311266,0.0357696219888033,1.64961351615811E-15));
#121664=DIRECTION('ref_axis',(-0.0357696219888033,0.999360062311266,4.316049615934E-32));
#121665=DIRECTION('center_axis',(0.999556853338411,0.0297673805400138,1.82491045181999E-14));
#121666=DIRECTION('ref_axis',(-0.0297673805400138,0.999556853338411,-8.47827291376735E-32));
#121667=DIRECTION('center_axis',(0.,0.,-1.));
#121668=DIRECTION('ref_axis',(0.0297644531369321,-0.999556940513875,0.));
#121669=DIRECTION('center_axis',(1.57626159414375E-5,0.0233282309877023,
0.999727859665081));
#121670=DIRECTION('ref_axis',(0.0363487305279994,-0.999067219538478,0.023312242119934));
#121671=DIRECTION('center_axis',(0.972436723729276,-0.233166932352493,0.));
#121672=DIRECTION('ref_axis',(0.233166932352493,0.972436723729276,0.));
#121673=DIRECTION('center_axis',(0.0068520731291586,-0.00565696608596777,
-0.999960523135056));
#121674=DIRECTION('ref_axis',(0.755063620042167,-0.655591356155534,0.00888275987323359));
#121675=DIRECTION('center_axis',(-0.635093426738814,-0.772416788158568,
-0.00535207286497078));
#121676=DIRECTION('ref_axis',(0.77242785121363,-0.635102522959478,9.38368926324323E-20));
#121677=DIRECTION('center_axis',(-0.563237659270021,-0.823253026831934,
0.0708363818393295));
#121678=DIRECTION('ref_axis',(0.825326289137892,-0.564656104596307,-9.62895252096333E-18));
#121679=DIRECTION('center_axis',(-0.341333328819756,0.277129686002563,0.898159615977553));
#121680=DIRECTION('ref_axis',(0.751460582051474,-0.493539243236486,0.437865286370611));
#121681=DIRECTION('center_axis',(0.509059682279704,-0.413543807234115,-0.754877314121705));
#121682=DIRECTION('ref_axis',(0.798913102792373,0.55338237641331,0.235596688562935));
#121683=DIRECTION('center_axis',(-0.0353652067153621,-0.980391286708013,
0.193861360515669));
#121684=DIRECTION('ref_axis',(-3.63487303375728E-18,-0.193982705344839,
-0.981004949032928));
#121685=DIRECTION('center_axis',(-0.0385934612262193,-0.999254003953662,
0.00140724310442582));
#121686=DIRECTION('ref_axis',(0.999254993383049,-0.0385934994402315,-2.19294060248386E-20));
#121687=DIRECTION('center_axis',(0.0362455094603874,7.24243967428071E-6,
0.999342915615808));
#121688=DIRECTION('ref_axis',(0.99884239871172,-0.0316458184758586,-0.036227126698248));
#121689=DIRECTION('center_axis',(0.0149227809046296,0.000160750066432761,
-0.999888636183795));
#121690=DIRECTION('ref_axis',(0.999085030892015,-0.0400869256955743,0.0149043428496258));
#121691=DIRECTION('center_axis',(-0.803581860357368,-0.445034265274962,
0.395222337976698));
#121692=DIRECTION('ref_axis',(0.439140785392348,-0.891532545451671,-0.111018426423077));
#121693=DIRECTION('center_axis',(-0.469907551033905,0.216399115636686,-0.855779361887735));
#121694=DIRECTION('ref_axis',(0.876549208984677,-2.3138118535155E-14,-0.481312252314792));
#121695=DIRECTION('center_axis',(-0.460561989867266,0.543327519921019,-0.701910150650338));
#121696=DIRECTION('ref_axis',(-1.68332661555862E-16,0.790771035553874,0.612112056186654));
#121697=DIRECTION('center_axis',(0.488505761670049,0.207277391256933,0.847583744469469));
#121698=DIRECTION('ref_axis',(0.866400038259138,1.13916389737517E-16,-0.499350551921758));
#121699=DIRECTION('center_axis',(-0.485723325571869,-0.464849177451359,
-0.740262178703059));
#121700=DIRECTION('ref_axis',(-0.836086106459356,-1.21161241824207E-16,
0.548598234216658));
#121701=DIRECTION('center_axis',(0.015774878482318,2.06992946781092E-6,
-0.999875568860738));
#121702=DIRECTION('ref_axis',(0.99934939359657,0.0324376701882913,0.0157666442505599));
#121703=DIRECTION('center_axis',(0.0387718059368437,-0.999247421633299,
-0.00115647031964687));
#121704=DIRECTION('ref_axis',(0.999248089842511,0.0387718318640339,-1.43119761272989E-20));
#121705=DIRECTION('center_axis',(0.0366457249192154,0.000264295716704561,
0.999328284895869));
#121706=DIRECTION('ref_axis',(0.998575905634023,0.0387881617069405,-0.0366283933388643));
#121707=DIRECTION('center_axis',(0.0362051861961663,-0.986513040328005,
-0.159628336316885));
#121708=DIRECTION('ref_axis',(3.13261606677306E-17,0.159733060933468,-0.987160244967769));
#121709=DIRECTION('center_axis',(0.586558422242651,-0.80833932738343,-0.0503661503543409));
#121710=DIRECTION('ref_axis',(0.809366559200372,0.587303816476745,6.0201141129801E-17));
#121711=DIRECTION('center_axis',(0.635108704314869,-0.772391525947514,0.00694725470670599));
#121712=DIRECTION('ref_axis',(0.772410166108943,0.635124031423434,-3.90764897276796E-18));
#121713=DIRECTION('center_axis',(-0.367164830643458,-0.297433524522046,
0.88131906006222));
#121714=DIRECTION('ref_axis',(0.67960514144709,0.561137496245174,0.472505621158498));
#121715=DIRECTION('center_axis',(0.533623207901549,0.432878874093675,-0.726541225500833));
#121716=DIRECTION('ref_axis',(0.613440310257391,0.393261638389221,0.684862226672446));
#121717=DIRECTION('center_axis',(0.00304815896002169,0.0038938690271396,
-0.99998777318073));
#121718=DIRECTION('ref_axis',(-0.641245941557608,0.767334721447853,0.00103329397685693));
#121719=DIRECTION('center_axis',(0.119709524432718,-0.500158371272784,0.857619515522967));
#121720=DIRECTION('ref_axis',(5.19703601812987E-17,-0.863831361964004,-0.503781081510029));
#121721=DIRECTION('center_axis',(-0.998342751080717,-0.0344241690564106,
0.0461164607202445));
#121722=DIRECTION('ref_axis',(0.0536635038266924,-0.267462686432825,0.962072730994481));
#121723=DIRECTION('center_axis',(-0.501099625553759,0.466384922602348,-0.728961088974634));
#121724=DIRECTION('ref_axis',(-0.824074180962238,-2.20209609654532E-16,
0.566481901097834));
#121725=DIRECTION('center_axis',(-0.254850132245688,-0.841789549666582,
-0.475858975082417));
#121726=DIRECTION('ref_axis',(-0.487493661504454,0.536841701873146,-0.688586172619612));
#121727=DIRECTION('center_axis',(-0.0894444115370802,-0.865796085393033,
-0.492338131534503));
#121728=DIRECTION('ref_axis',(0.983291176009294,-0.155450632474041,0.0947288976272861));
#121729=DIRECTION('center_axis',(-4.00197585461019E-5,-0.0159615005705134,
-0.999872606334405));
#121730=DIRECTION('ref_axis',(0.0321201706221352,-0.999356707583681,0.0159519793978996));
#121731=DIRECTION('center_axis',(-0.999263201609641,-0.0383614667420372,
-0.00120489761000603));
#121732=DIRECTION('ref_axis',(0.0383614945882391,-0.999263926964722,2.87536200646804E-20));
#121733=DIRECTION('center_axis',(-2.30441962568634E-5,-0.0307840994537002,
0.999526057033927));
#121734=DIRECTION('ref_axis',(0.0383802756232838,-0.998789639512621,-0.0307605338921488));
#121735=DIRECTION('center_axis',(-0.974363720155827,-0.0344964635874725,
-0.222318093829667));
#121736=DIRECTION('ref_axis',(-0.222450491940089,1.26241972147447E-18,0.974943987434977));
#121737=DIRECTION('center_axis',(-0.836810598831192,-0.541308500745221,
-0.0820556439542334));
#121738=DIRECTION('ref_axis',(0.543140105176027,-0.839642082169167,1.69471490770742E-17));
#121739=DIRECTION('center_axis',(-0.774120577489127,-0.632943886852024,
0.0109255482495788));
#121740=DIRECTION('ref_axis',(0.632981666732123,-0.774166784085331,5.39501067277511E-19));
#121741=DIRECTION('center_axis',(-0.26668203931152,0.334936975495388,0.903713401668167));
#121742=DIRECTION('ref_axis',(0.574033930782738,-0.698011739529375,0.428094216019436));
#121743=DIRECTION('center_axis',(0.0101770580641384,-0.0115323051715096,
-0.999881709717));
#121744=DIRECTION('ref_axis',(0.775808985621547,0.630967538505684,0.000619016109577773));
#121745=DIRECTION('center_axis',(-4.45320928885371E-8,0.998303409681459,
0.0582263017748053));
#121746=DIRECTION('ref_axis',(0.,-0.0582263017748052,0.99830340968146));
#121747=DIRECTION('center_axis',(-8.12532577157186E-9,0.998207006171548,
0.0598562680931181));
#121748=DIRECTION('ref_axis',(0.999311726713681,-0.00222038745151431,0.0370289445175939));
#121749=DIRECTION('center_axis',(-0.99999635393917,0.000157155077313813,
-0.00269581354111146));
#121750=DIRECTION('ref_axis',(-0.00269581357440168,1.24619272072387E-21,
0.999996366287984));
#121751=DIRECTION('center_axis',(-2.33119191152438E-9,-0.986382708044219,
-0.164466267882973));
#121752=DIRECTION('ref_axis',(0.999999030863823,-0.000228975224915186,0.00137325953914107));
#121753=DIRECTION('center_axis',(0.244344449131117,0.492606745559265,0.835245104390514));
#121754=DIRECTION('ref_axis',(4.32889927015855E-17,-0.86135403585069,0.508005142615435));
#121755=DIRECTION('center_axis',(0.330813257101916,-0.830741130674896,0.447696060660149));
#121756=DIRECTION('ref_axis',(0.932375699002072,0.214461635172499,-0.291001310906903));
#121757=DIRECTION('center_axis',(0.000178107895792883,0.00455637129950124,
0.999989603825039));
#121758=DIRECTION('ref_axis',(0.986443060931718,-0.16410289554268,0.000572026372399929));
#121759=DIRECTION('center_axis',(-0.982994797178248,0.183632204703407,-0.000664918236953841));
#121760=DIRECTION('ref_axis',(-0.183632245296812,-0.982995014477312,5.7655403569157E-20));
#121761=DIRECTION('center_axis',(-0.433391148275503,-0.470797811534069,
-0.768453989026781));
#121762=DIRECTION('ref_axis',(-8.06979081629128E-16,0.852695228537141,-0.522408697506075));
#121763=DIRECTION('center_axis',(-0.96720597488598,0.18129103740974,-0.177893681449798));
#121764=DIRECTION('ref_axis',(-0.184229551589837,-0.982883244501099,1.61805378326746E-17));
#121765=DIRECTION('center_axis',(-0.831503844166329,0.548952032819844,-0.0851646804701234));
#121766=DIRECTION('ref_axis',(-0.550953708881667,-0.834535805504794,3.15287181374443E-17));
#121767=DIRECTION('center_axis',(-0.777065025633406,0.629380269512156,0.00710086516978589));
#121768=DIRECTION('ref_axis',(-0.62939613750826,-0.777084617071837,1.0927692862107E-18));
#121769=DIRECTION('center_axis',(-0.295452400444952,-0.370381022938362,
0.880639413675341));
#121770=DIRECTION('ref_axis',(0.467331061476171,0.747944548358106,0.471360405168853));
#121771=DIRECTION('center_axis',(0.,0.,-1.));
#121772=DIRECTION('ref_axis',(0.,1.,0.));
#121773=DIRECTION('center_axis',(0.,0.,-1.));
#121774=DIRECTION('ref_axis',(0.,1.,0.));
#121775=DIRECTION('',(-3.82498197630791E-33,-1.23467863058847E-16,1.));
#121776=DIRECTION('',(0.,1.23467863058847E-16,-1.));
#121777=DIRECTION('center_axis',(0.,0.,-1.));
#121778=DIRECTION('ref_axis',(0.,1.,0.));
#121779=DIRECTION('',(0.,-1.23467863058847E-16,1.));
#121780=DIRECTION('',(0.,1.23467863058847E-16,-1.));
#121781=DIRECTION('center_axis',(0.,0.,-1.));
#121782=DIRECTION('ref_axis',(0.,1.,0.));
#121783=DIRECTION('center_axis',(0.,0.,-1.));
#121784=DIRECTION('ref_axis',(0.,1.,0.));
#121785=DIRECTION('',(0.,-1.23467863058847E-16,1.));
#121786=DIRECTION('',(0.,1.23467863058847E-16,-1.));
#121787=DIRECTION('center_axis',(0.,0.,-1.));
#121788=DIRECTION('ref_axis',(0.,1.,0.));
#121789=DIRECTION('center_axis',(0.,0.,-1.));
#121790=DIRECTION('ref_axis',(0.,1.,0.));
#121791=DIRECTION('',(0.,-1.23467863058847E-16,1.));
#121792=DIRECTION('',(0.,1.23467863058847E-16,-1.));
#121793=DIRECTION('center_axis',(0.,0.,-1.));
#121794=DIRECTION('ref_axis',(0.,1.,0.));
#121795=DIRECTION('center_axis',(0.,0.,-1.));
#121796=DIRECTION('ref_axis',(0.,1.,0.));
#121797=DIRECTION('',(0.,-1.23467863058847E-16,1.));
#121798=DIRECTION('',(0.,1.23467863058847E-16,-1.));
#121799=DIRECTION('center_axis',(0.,0.,-1.));
#121800=DIRECTION('ref_axis',(0.,1.,0.));
#121801=DIRECTION('center_axis',(0.,0.,-1.));
#121802=DIRECTION('ref_axis',(0.,1.,0.));
#121803=DIRECTION('',(0.,-1.23467863058847E-16,1.));
#121804=DIRECTION('',(0.,1.23467863058847E-16,-1.));
#121805=DIRECTION('center_axis',(0.,0.,-1.));
#121806=DIRECTION('ref_axis',(0.,1.,0.));
#121807=DIRECTION('center_axis',(0.,0.,-1.));
#121808=DIRECTION('ref_axis',(0.,1.,0.));
#121809=DIRECTION('',(0.,-1.23467863058847E-16,1.));
#121810=DIRECTION('',(1.27503726478586E-32,1.23467863058847E-16,-1.));
#121811=DIRECTION('center_axis',(0.,0.,-1.));
#121812=DIRECTION('ref_axis',(0.,1.,0.));
#121813=DIRECTION('center_axis',(0.,0.,-1.));
#121814=DIRECTION('ref_axis',(0.0950205176920726,-0.995475314218053,0.));
#121815=DIRECTION('',(0.,-1.23467863058847E-16,1.));
#121816=DIRECTION('',(0.,1.23467863058847E-16,-1.));
#121817=DIRECTION('center_axis',(0.,0.,-1.));
#121818=DIRECTION('ref_axis',(0.,1.,0.));
#121819=DIRECTION('center_axis',(0.,0.,-1.));
#121820=DIRECTION('ref_axis',(0.,1.,0.));
#121821=DIRECTION('',(0.,-1.23467863058847E-16,1.));
#121822=DIRECTION('',(0.,1.23467863058847E-16,-1.));
#121823=DIRECTION('center_axis',(0.,0.,-1.));
#121824=DIRECTION('ref_axis',(0.,1.,0.));
#121825=DIRECTION('center_axis',(0.,0.,-1.));
#121826=DIRECTION('ref_axis',(0.,1.,0.));
#121827=DIRECTION('center_axis',(0.,0.,-1.));
#121828=DIRECTION('ref_axis',(0.,1.,0.));
#121829=DIRECTION('',(0.,-1.23467863058847E-16,1.));
#121830=DIRECTION('',(0.,1.23467863058847E-16,-1.));
#121831=DIRECTION('center_axis',(0.,0.,-1.));
#121832=DIRECTION('ref_axis',(0.,1.,0.));
#121833=DIRECTION('',(0.,-1.23467863058847E-16,1.));
#121834=DIRECTION('',(0.,1.23467863058847E-16,-1.));
#121835=DIRECTION('center_axis',(0.,0.,-1.));
#121836=DIRECTION('ref_axis',(0.,1.,0.));
#121837=DIRECTION('center_axis',(1.3684555315672E-48,0.,1.));
#121838=DIRECTION('ref_axis',(0.,-1.,0.));
#121839=DIRECTION('',(0.,-1.23467863058847E-16,1.));
#121840=DIRECTION('',(-1.3684555315672E-48,1.23467863058847E-16,-1.));
#121841=DIRECTION('center_axis',(0.,0.,-1.));
#121842=DIRECTION('ref_axis',(0.,1.,0.));
#121843=DIRECTION('center_axis',(0.,0.,-1.));
#121844=DIRECTION('ref_axis',(0.,1.,0.));
#121845=DIRECTION('',(0.,-1.23467863058847E-16,1.));
#121846=DIRECTION('',(0.,1.23467863058847E-16,-1.));
#121847=DIRECTION('center_axis',(0.,0.,-1.));
#121848=DIRECTION('ref_axis',(0.,1.,0.));
#121849=DIRECTION('center_axis',(0.,0.,1.));
#121850=DIRECTION('ref_axis',(0.,-1.,0.));
#121851=DIRECTION('',(0.,-1.23467863058847E-16,1.));
#121852=DIRECTION('',(0.,1.23467863058847E-16,-1.));
#121853=DIRECTION('center_axis',(0.,0.,-1.));
#121854=DIRECTION('ref_axis',(0.,1.,0.));
#121855=DIRECTION('center_axis',(0.,0.,-1.));
#121856=DIRECTION('ref_axis',(0.,1.,0.));
#121857=DIRECTION('',(0.,-1.23467863058847E-16,1.));
#121858=DIRECTION('',(0.,1.23467863058847E-16,-1.));
#121859=DIRECTION('center_axis',(0.,0.,-1.));
#121860=DIRECTION('ref_axis',(0.,1.,0.));
#121861=DIRECTION('center_axis',(0.,0.,-1.));
#121862=DIRECTION('ref_axis',(0.,1.,0.));
#121863=DIRECTION('',(0.,-1.23467863058847E-16,1.));
#121864=DIRECTION('',(0.,1.23467863058847E-16,-1.));
#121865=DIRECTION('center_axis',(0.,0.,-1.));
#121866=DIRECTION('ref_axis',(0.,1.,0.));
#121867=DIRECTION('center_axis',(0.,0.,1.));
#121868=DIRECTION('ref_axis',(0.,-1.,0.));
#121869=DIRECTION('',(0.,-1.23467863058847E-16,1.));
#121870=DIRECTION('',(0.,1.23467863058847E-16,-1.));
#121871=DIRECTION('center_axis',(0.,0.,-1.));
#121872=DIRECTION('ref_axis',(0.,1.,0.));
#121873=DIRECTION('center_axis',(-1.3684555315672E-48,0.,-1.));
#121874=DIRECTION('ref_axis',(0.,1.,0.));
#121875=DIRECTION('',(1.3684555315672E-48,-1.23467863058847E-16,1.));
#121876=DIRECTION('',(0.,1.23467863058847E-16,-1.));
#121877=DIRECTION('center_axis',(0.,0.,-1.));
#121878=DIRECTION('ref_axis',(0.,1.,0.));
#121879=DIRECTION('center_axis',(0.,0.,-1.));
#121880=DIRECTION('ref_axis',(0.686617021913642,-0.727019301819726,0.));
#121881=DIRECTION('',(0.,-1.23467863058847E-16,1.));
#121882=DIRECTION('',(0.,1.23467863058847E-16,-1.));
#121883=DIRECTION('center_axis',(0.,0.,-1.));
#121884=DIRECTION('ref_axis',(0.,1.,0.));
#121885=DIRECTION('center_axis',(0.,0.,1.));
#121886=DIRECTION('ref_axis',(0.,-1.,0.));
#121887=DIRECTION('',(0.,-1.23467863058847E-16,1.));
#121888=DIRECTION('',(0.,1.23467863058847E-16,-1.));
#121889=DIRECTION('center_axis',(0.,0.,-1.));
#121890=DIRECTION('ref_axis',(0.,1.,0.));
#121891=DIRECTION('center_axis',(0.,0.,-1.));
#121892=DIRECTION('ref_axis',(0.,1.,0.));
#121893=DIRECTION('',(0.,-1.23467863058847E-16,1.));
#121894=DIRECTION('',(0.,1.23467863058847E-16,-1.));
#121895=DIRECTION('center_axis',(0.,0.,-1.));
#121896=DIRECTION('ref_axis',(0.,1.,0.));
#121897=DIRECTION('center_axis',(0.,0.,-1.));
#121898=DIRECTION('ref_axis',(0.,1.,0.));
#121899=DIRECTION('',(0.,-1.23467863058847E-16,1.));
#121900=DIRECTION('',(0.,1.23467863058847E-16,-1.));
#121901=DIRECTION('center_axis',(0.,0.,-1.));
#121902=DIRECTION('ref_axis',(0.,1.,0.));
#121903=DIRECTION('center_axis',(0.,0.,-1.));
#121904=DIRECTION('ref_axis',(0.,1.,0.));
#121905=DIRECTION('',(0.,-1.23467863058847E-16,1.));
#121906=DIRECTION('',(0.,1.23467863058847E-16,-1.));
#121907=DIRECTION('center_axis',(0.,0.,-1.));
#121908=DIRECTION('ref_axis',(0.,1.,0.));
#121909=DIRECTION('center_axis',(0.,0.,1.));
#121910=DIRECTION('ref_axis',(0.,-1.,0.));
#121911=DIRECTION('',(0.,-1.23467863058847E-16,1.));
#121912=DIRECTION('',(0.,1.23467863058847E-16,-1.));
#121913=DIRECTION('center_axis',(0.,0.,-1.));
#121914=DIRECTION('ref_axis',(0.,1.,0.));
#121915=DIRECTION('center_axis',(0.,0.,-1.));
#121916=DIRECTION('ref_axis',(0.,1.,0.));
#121917=DIRECTION('',(0.,-1.23467863058847E-16,1.));
#121918=DIRECTION('',(0.,1.23467863058847E-16,-1.));
#121919=DIRECTION('center_axis',(0.,0.,-1.));
#121920=DIRECTION('ref_axis',(0.,1.,0.));
#121921=DIRECTION('center_axis',(0.,0.,1.));
#121922=DIRECTION('ref_axis',(0.,-1.,0.));
#121923=DIRECTION('',(0.,-1.23467863058847E-16,1.));
#121924=DIRECTION('',(0.,1.23467863058847E-16,-1.));
#121925=DIRECTION('center_axis',(0.,0.,-1.));
#121926=DIRECTION('ref_axis',(0.,1.,0.));
#121927=DIRECTION('center_axis',(0.,0.,-1.));
#121928=DIRECTION('ref_axis',(0.,1.,0.));
#121929=DIRECTION('',(0.,-1.23467863058847E-16,1.));
#121930=DIRECTION('',(0.,1.23467863058847E-16,-1.));
#121931=DIRECTION('center_axis',(0.,0.,-1.));
#121932=DIRECTION('ref_axis',(0.,1.,0.));
#121933=DIRECTION('center_axis',(0.,0.,-1.));
#121934=DIRECTION('ref_axis',(0.,1.,0.));
#121935=DIRECTION('center_axis',(0.,0.,-1.));
#121936=DIRECTION('ref_axis',(0.,1.,0.));
#121937=DIRECTION('',(0.,-1.23467863058847E-16,1.));
#121938=DIRECTION('',(0.,1.23467863058847E-16,-1.));
#121939=DIRECTION('center_axis',(0.,0.,1.));
#121940=DIRECTION('ref_axis',(0.,-1.,0.));
#121941=DIRECTION('',(0.,-1.23467863058847E-16,1.));
#121942=DIRECTION('',(0.,1.23467863058847E-16,-1.));
#121943=DIRECTION('center_axis',(0.,0.,-1.));
#121944=DIRECTION('ref_axis',(0.,1.,0.));
#121945=DIRECTION('center_axis',(0.,0.,-1.));
#121946=DIRECTION('ref_axis',(0.,1.,0.));
#121947=DIRECTION('',(0.,-1.23467863058847E-16,1.));
#121948=DIRECTION('',(0.,1.23467863058847E-16,-1.));
#121949=DIRECTION('center_axis',(0.,0.,-1.));
#121950=DIRECTION('ref_axis',(0.,1.,0.));
#121951=DIRECTION('center_axis',(0.,0.,1.));
#121952=DIRECTION('ref_axis',(0.,-1.,0.));
#121953=DIRECTION('',(0.,-1.23467863058847E-16,1.));
#121954=DIRECTION('',(0.,1.23467863058847E-16,-1.));
#121955=DIRECTION('center_axis',(0.,0.,-1.));
#121956=DIRECTION('ref_axis',(0.,1.,0.));
#121957=DIRECTION('center_axis',(0.,0.,-1.));
#121958=DIRECTION('ref_axis',(0.,1.,0.));
#121959=DIRECTION('',(0.,-1.23467863058847E-16,1.));
#121960=DIRECTION('',(0.,1.23467863058847E-16,-1.));
#121961=DIRECTION('center_axis',(0.,0.,-1.));
#121962=DIRECTION('ref_axis',(0.,1.,0.));
#121963=DIRECTION('center_axis',(0.,0.,1.));
#121964=DIRECTION('ref_axis',(0.,-1.,0.));
#121965=DIRECTION('',(0.,-1.23467863058847E-16,1.));
#121966=DIRECTION('',(0.,1.23467863058847E-16,-1.));
#121967=DIRECTION('center_axis',(0.,0.,-1.));
#121968=DIRECTION('ref_axis',(0.,1.,0.));
#121969=DIRECTION('center_axis',(0.,0.,-1.));
#121970=DIRECTION('ref_axis',(0.,1.,0.));
#121971=DIRECTION('',(0.,-1.23467863058847E-16,1.));
#121972=DIRECTION('',(0.,1.23467863058847E-16,-1.));
#121973=DIRECTION('center_axis',(0.,0.,-1.));
#121974=DIRECTION('ref_axis',(0.,1.,0.));
#121975=DIRECTION('center_axis',(0.,0.,1.));
#121976=DIRECTION('ref_axis',(0.,-1.,0.));
#121977=DIRECTION('',(0.,-1.23467863058847E-16,1.));
#121978=DIRECTION('',(0.,1.23467863058847E-16,-1.));
#121979=DIRECTION('center_axis',(0.,0.,-1.));
#121980=DIRECTION('ref_axis',(0.,1.,0.));
#121981=DIRECTION('center_axis',(0.,0.,-1.));
#121982=DIRECTION('ref_axis',(0.,1.,0.));
#121983=DIRECTION('',(0.,-1.23467863058847E-16,1.));
#121984=DIRECTION('',(0.,1.23467863058847E-16,-1.));
#121985=DIRECTION('center_axis',(0.,0.,-1.));
#121986=DIRECTION('ref_axis',(0.,1.,0.));
#121987=DIRECTION('center_axis',(0.,0.,1.));
#121988=DIRECTION('ref_axis',(0.,-1.,0.));
#121989=DIRECTION('',(0.,-1.23467863058847E-16,1.));
#121990=DIRECTION('',(0.,1.23467863058847E-16,-1.));
#121991=DIRECTION('center_axis',(0.,0.,-1.));
#121992=DIRECTION('ref_axis',(0.,1.,0.));
#121993=DIRECTION('center_axis',(0.,0.,-1.));
#121994=DIRECTION('ref_axis',(0.,1.,0.));
#121995=DIRECTION('',(0.,-1.23467863058847E-16,1.));
#121996=DIRECTION('',(0.,1.23467863058847E-16,-1.));
#121997=DIRECTION('center_axis',(0.,0.,-1.));
#121998=DIRECTION('ref_axis',(0.,1.,0.));
#121999=DIRECTION('center_axis',(0.,0.,-1.));
#122000=DIRECTION('ref_axis',(-0.695782815675815,-0.718252235228151,0.));
#122001=DIRECTION('',(0.,-1.23467863058847E-16,1.));
#122002=DIRECTION('',(0.,1.23467863058847E-16,-1.));
#122003=DIRECTION('center_axis',(0.,0.,-1.));
#122004=DIRECTION('ref_axis',(0.,1.,0.));
#122005=DIRECTION('center_axis',(0.,0.,-1.));
#122006=DIRECTION('ref_axis',(0.,1.,0.));
#122007=DIRECTION('',(0.,-1.23467863058847E-16,1.));
#122008=DIRECTION('',(0.,1.23467863058847E-16,-1.));
#122009=DIRECTION('center_axis',(0.,0.,-1.));
#122010=DIRECTION('ref_axis',(0.,1.,0.));
#122011=DIRECTION('center_axis',(0.,0.,1.));
#122012=DIRECTION('ref_axis',(0.,-1.,0.));
#122013=DIRECTION('',(0.,-1.23467863058847E-16,1.));
#122014=DIRECTION('',(0.,1.23467863058847E-16,-1.));
#122015=DIRECTION('center_axis',(0.,0.,-1.));
#122016=DIRECTION('ref_axis',(0.,1.,0.));
#122017=DIRECTION('center_axis',(0.,0.,-1.));
#122018=DIRECTION('ref_axis',(0.,1.,0.));
#122019=DIRECTION('',(0.,-1.23467863058847E-16,1.));
#122020=DIRECTION('',(0.,1.23467863058847E-16,-1.));
#122021=DIRECTION('center_axis',(0.,0.,-1.));
#122022=DIRECTION('ref_axis',(0.,1.,0.));
#122023=DIRECTION('center_axis',(0.,0.,-1.));
#122024=DIRECTION('ref_axis',(0.,1.,0.));
#122025=DIRECTION('',(0.,-1.23467863058847E-16,1.));
#122026=DIRECTION('',(0.,1.23467863058847E-16,-1.));
#122027=DIRECTION('center_axis',(0.,0.,-1.));
#122028=DIRECTION('ref_axis',(0.,1.,0.));
#122029=DIRECTION('center_axis',(0.,0.,-1.));
#122030=DIRECTION('ref_axis',(0.,1.,0.));
#122031=DIRECTION('',(0.,-1.23467863058847E-16,1.));
#122032=DIRECTION('',(0.,1.23467863058847E-16,-1.));
#122033=DIRECTION('center_axis',(0.,0.,-1.));
#122034=DIRECTION('ref_axis',(0.,1.,0.));
#122035=DIRECTION('center_axis',(0.,0.,1.));
#122036=DIRECTION('ref_axis',(0.,-1.,0.));
#122037=DIRECTION('',(0.,-1.23467863058847E-16,1.));
#122038=DIRECTION('',(0.,1.23467863058847E-16,-1.));
#122039=DIRECTION('center_axis',(0.,0.,-1.));
#122040=DIRECTION('ref_axis',(0.,1.,0.));
#122041=DIRECTION('center_axis',(0.,0.,-1.));
#122042=DIRECTION('ref_axis',(0.,1.,0.));
#122043=DIRECTION('',(0.,-1.23467863058847E-16,1.));
#122044=DIRECTION('',(0.,1.23467863058847E-16,-1.));
#122045=DIRECTION('center_axis',(0.,0.,-1.));
#122046=DIRECTION('ref_axis',(0.,1.,0.));
#122047=DIRECTION('center_axis',(0.,0.,1.));
#122048=DIRECTION('ref_axis',(0.,-1.,0.));
#122049=DIRECTION('',(0.,-1.23467863058847E-16,1.));
#122050=DIRECTION('',(0.,1.23467863058847E-16,-1.));
#122051=DIRECTION('center_axis',(0.,0.,-1.));
#122052=DIRECTION('ref_axis',(0.,1.,0.));
#122053=DIRECTION('center_axis',(0.,0.,-1.));
#122054=DIRECTION('ref_axis',(0.,1.,0.));
#122055=DIRECTION('',(0.,-1.23467863058847E-16,1.));
#122056=DIRECTION('',(0.,1.23467863058847E-16,-1.));
#122057=DIRECTION('center_axis',(0.,0.,-1.));
#122058=DIRECTION('ref_axis',(0.,1.,0.));
#122059=DIRECTION('center_axis',(0.,0.,1.));
#122060=DIRECTION('ref_axis',(0.,-1.,0.));
#122061=DIRECTION('',(0.,-1.23467863058847E-16,1.));
#122062=DIRECTION('',(0.,1.23467863058847E-16,-1.));
#122063=DIRECTION('center_axis',(0.,0.,-1.));
#122064=DIRECTION('ref_axis',(0.,1.,0.));
#122065=DIRECTION('center_axis',(0.,0.,-1.));
#122066=DIRECTION('ref_axis',(0.,1.,0.));
#122067=DIRECTION('',(0.,-1.23467863058847E-16,1.));
#122068=DIRECTION('',(0.,1.23467863058847E-16,-1.));
#122069=DIRECTION('center_axis',(0.,0.,-1.));
#122070=DIRECTION('ref_axis',(0.,1.,0.));
#122071=DIRECTION('center_axis',(0.,0.,1.));
#122072=DIRECTION('ref_axis',(0.,-1.,0.));
#122073=DIRECTION('',(0.,-1.23467863058847E-16,1.));
#122074=DIRECTION('',(0.,1.23467863058847E-16,-1.));
#122075=DIRECTION('center_axis',(0.,0.,-1.));
#122076=DIRECTION('ref_axis',(0.,1.,0.));
#122077=DIRECTION('center_axis',(0.,0.,-1.));
#122078=DIRECTION('ref_axis',(0.,1.,0.));
#122079=DIRECTION('',(0.,-1.23467863058847E-16,1.));
#122080=DIRECTION('',(0.,1.23467863058847E-16,-1.));
#122081=DIRECTION('center_axis',(0.,0.,-1.));
#122082=DIRECTION('ref_axis',(0.,1.,0.));
#122083=DIRECTION('center_axis',(0.,0.,1.));
#122084=DIRECTION('ref_axis',(0.,-1.,0.));
#122085=DIRECTION('',(0.,-1.23467863058847E-16,1.));
#122086=DIRECTION('',(0.,1.23467863058847E-16,-1.));
#122087=DIRECTION('center_axis',(0.,0.,-1.));
#122088=DIRECTION('ref_axis',(0.,1.,0.));
#122089=DIRECTION('center_axis',(0.,0.,-1.));
#122090=DIRECTION('ref_axis',(0.,1.,0.));
#122091=DIRECTION('',(0.,-1.23467863058847E-16,1.));
#122092=DIRECTION('',(0.,1.23467863058847E-16,-1.));
#122093=DIRECTION('center_axis',(0.,0.,-1.));
#122094=DIRECTION('ref_axis',(0.,1.,0.));
#122095=DIRECTION('center_axis',(0.,0.,1.));
#122096=DIRECTION('ref_axis',(0.,-1.,0.));
#122097=DIRECTION('',(0.,-1.23467863058847E-16,1.));
#122098=DIRECTION('',(0.,1.23467863058847E-16,-1.));
#122099=DIRECTION('center_axis',(0.,0.,-1.));
#122100=DIRECTION('ref_axis',(0.,1.,0.));
#122101=DIRECTION('center_axis',(0.,0.,-1.));
#122102=DIRECTION('ref_axis',(0.,1.,0.));
#122103=DIRECTION('',(0.,-1.23467863058847E-16,1.));
#122104=DIRECTION('',(0.,1.23467863058847E-16,-1.));
#122105=DIRECTION('center_axis',(0.,0.,-1.));
#122106=DIRECTION('ref_axis',(0.,1.,0.));
#122107=DIRECTION('center_axis',(0.,0.,-1.));
#122108=DIRECTION('ref_axis',(0.,1.,0.));
#122109=DIRECTION('',(0.,-1.23467863058847E-16,1.));
#122110=DIRECTION('',(0.,1.23467863058847E-16,-1.));
#122111=DIRECTION('center_axis',(0.,0.,-1.));
#122112=DIRECTION('ref_axis',(0.,1.,0.));
#122113=DIRECTION('center_axis',(0.,0.,-1.));
#122114=DIRECTION('ref_axis',(-0.406625030395207,-0.91359514264038,0.));
#122115=DIRECTION('',(0.,-1.23467863058847E-16,1.));
#122116=DIRECTION('',(0.,1.23467863058847E-16,-1.));
#122117=DIRECTION('center_axis',(0.,0.,-1.));
#122118=DIRECTION('ref_axis',(0.,1.,0.));
#122119=DIRECTION('center_axis',(0.,0.,-1.));
#122120=DIRECTION('ref_axis',(0.,1.,0.));
#122121=DIRECTION('',(0.,-1.23467863058847E-16,1.));
#122122=DIRECTION('',(0.,1.23467863058847E-16,-1.));
#122123=DIRECTION('center_axis',(0.,0.,-1.));
#122124=DIRECTION('ref_axis',(0.,1.,0.));
#122125=DIRECTION('center_axis',(0.,0.,-1.));
#122126=DIRECTION('ref_axis',(0.,1.,0.));
#122127=DIRECTION('',(0.,-1.23467863058847E-16,1.));
#122128=DIRECTION('',(0.,1.23467863058847E-16,-1.));
#122129=DIRECTION('center_axis',(0.,0.,-1.));
#122130=DIRECTION('ref_axis',(0.,1.,0.));
#122131=DIRECTION('center_axis',(0.,0.,1.));
#122132=DIRECTION('ref_axis',(0.,-1.,0.));
#122133=DIRECTION('',(0.,-1.23467863058847E-16,1.));
#122134=DIRECTION('',(0.,1.23467863058847E-16,-1.));
#122135=DIRECTION('center_axis',(0.,0.,-1.));
#122136=DIRECTION('ref_axis',(0.,1.,0.));
#122137=DIRECTION('center_axis',(0.,0.,-1.));
#122138=DIRECTION('ref_axis',(0.,1.,0.));
#122139=DIRECTION('',(0.,-1.23467863058847E-16,1.));
#122140=DIRECTION('',(0.,1.23467863058847E-16,-1.));
#122141=DIRECTION('center_axis',(0.,0.,-1.));
#122142=DIRECTION('ref_axis',(0.,1.,0.));
#122143=DIRECTION('center_axis',(0.,0.,1.));
#122144=DIRECTION('ref_axis',(0.,-1.,0.));
#122145=DIRECTION('',(0.,-1.23467863058847E-16,1.));
#122146=DIRECTION('',(0.,1.23467863058847E-16,-1.));
#122147=DIRECTION('center_axis',(0.,0.,-1.));
#122148=DIRECTION('ref_axis',(0.,1.,0.));
#122149=DIRECTION('center_axis',(0.,0.,-1.));
#122150=DIRECTION('ref_axis',(0.,1.,0.));
#122151=DIRECTION('',(0.,-1.23467863058847E-16,1.));
#122152=DIRECTION('',(0.,1.23467863058847E-16,-1.));
#122153=DIRECTION('center_axis',(0.,0.,-1.));
#122154=DIRECTION('ref_axis',(0.,1.,0.));
#122155=DIRECTION('center_axis',(0.,0.,1.));
#122156=DIRECTION('ref_axis',(0.,-1.,0.));
#122157=DIRECTION('',(0.,-1.23467863058847E-16,1.));
#122158=DIRECTION('',(0.,1.23467863058847E-16,-1.));
#122159=DIRECTION('center_axis',(0.,0.,-1.));
#122160=DIRECTION('ref_axis',(0.,1.,0.));
#122161=DIRECTION('center_axis',(0.,0.,-1.));
#122162=DIRECTION('ref_axis',(0.,1.,0.));
#122163=DIRECTION('',(0.,-1.23467863058847E-16,1.));
#122164=DIRECTION('',(0.,1.23467863058847E-16,-1.));
#122165=DIRECTION('center_axis',(0.,0.,-1.));
#122166=DIRECTION('ref_axis',(0.,1.,0.));
#122167=DIRECTION('center_axis',(0.,0.,-1.));
#122168=DIRECTION('ref_axis',(0.,1.,0.));
#122169=DIRECTION('',(0.,-1.23467863058847E-16,1.));
#122170=DIRECTION('',(0.,1.23467863058847E-16,-1.));
#122171=DIRECTION('center_axis',(0.,0.,-1.));
#122172=DIRECTION('ref_axis',(0.,1.,0.));
#122173=DIRECTION('center_axis',(0.,0.,-1.));
#122174=DIRECTION('ref_axis',(0.,1.,0.));
#122175=DIRECTION('',(0.,-1.23467863058847E-16,1.));
#122176=DIRECTION('',(0.,1.23467863058847E-16,-1.));
#122177=DIRECTION('center_axis',(0.,0.,-1.));
#122178=DIRECTION('ref_axis',(0.,1.,0.));
#122179=DIRECTION('center_axis',(0.,0.,1.));
#122180=DIRECTION('ref_axis',(0.,-1.,0.));
#122181=DIRECTION('',(0.,-1.23467863058847E-16,1.));
#122182=DIRECTION('',(0.,1.23467863058847E-16,-1.));
#122183=DIRECTION('center_axis',(0.,0.,-1.));
#122184=DIRECTION('ref_axis',(0.,1.,0.));
#122185=DIRECTION('center_axis',(0.,0.,-1.));
#122186=DIRECTION('ref_axis',(0.,1.,0.));
#122187=DIRECTION('',(0.,-1.23467863058847E-16,1.));
#122188=DIRECTION('',(0.,1.23467863058847E-16,-1.));
#122189=DIRECTION('center_axis',(0.,0.,-1.));
#122190=DIRECTION('ref_axis',(0.,1.,0.));
#122191=DIRECTION('center_axis',(0.,0.,-1.));
#122192=DIRECTION('ref_axis',(0.,1.,0.));
#122193=DIRECTION('',(0.,-1.23467863058847E-16,1.));
#122194=DIRECTION('',(0.,1.23467863058847E-16,-1.));
#122195=DIRECTION('center_axis',(0.,0.,-1.));
#122196=DIRECTION('ref_axis',(0.,1.,0.));
#122197=DIRECTION('center_axis',(0.,0.,-1.));
#122198=DIRECTION('ref_axis',(0.,1.,0.));
#122199=DIRECTION('',(0.,-1.23467863058847E-16,1.));
#122200=DIRECTION('',(0.,1.23467863058847E-16,-1.));
#122201=DIRECTION('center_axis',(0.,0.,-1.));
#122202=DIRECTION('ref_axis',(0.,1.,0.));
#122203=DIRECTION('center_axis',(0.,0.,1.));
#122204=DIRECTION('ref_axis',(0.,-1.,0.));
#122205=DIRECTION('',(0.,-1.23467863058847E-16,1.));
#122206=DIRECTION('',(0.,1.23467863058847E-16,-1.));
#122207=DIRECTION('center_axis',(0.,0.,-1.));
#122208=DIRECTION('ref_axis',(0.,1.,0.));
#122209=DIRECTION('center_axis',(0.,0.,-1.));
#122210=DIRECTION('ref_axis',(0.,1.,0.));
#122211=DIRECTION('',(0.,-1.23467863058847E-16,1.));
#122212=DIRECTION('',(0.,1.23467863058847E-16,-1.));
#122213=DIRECTION('center_axis',(0.,0.,-1.));
#122214=DIRECTION('ref_axis',(0.,1.,0.));
#122215=DIRECTION('center_axis',(0.,0.,-1.));
#122216=DIRECTION('ref_axis',(0.,1.,0.));
#122217=DIRECTION('',(0.,-1.23467863058847E-16,1.));
#122218=DIRECTION('',(0.,1.23467863058847E-16,-1.));
#122219=DIRECTION('center_axis',(0.,0.,-1.));
#122220=DIRECTION('ref_axis',(0.,1.,0.));
#122221=DIRECTION('center_axis',(0.,0.,-1.));
#122222=DIRECTION('ref_axis',(0.,1.,0.));
#122223=DIRECTION('',(0.,-1.23467863058847E-16,1.));
#122224=DIRECTION('',(0.,1.23467863058847E-16,-1.));
#122225=DIRECTION('center_axis',(0.,0.,-1.));
#122226=DIRECTION('ref_axis',(0.,1.,0.));
#122227=DIRECTION('center_axis',(0.,0.,1.));
#122228=DIRECTION('ref_axis',(0.,-1.,0.));
#122229=DIRECTION('',(0.,-1.23467863058847E-16,1.));
#122230=DIRECTION('',(0.,1.23467863058847E-16,-1.));
#122231=DIRECTION('center_axis',(0.,0.,-1.));
#122232=DIRECTION('ref_axis',(0.,1.,0.));
#122233=DIRECTION('center_axis',(0.,0.,-1.));
#122234=DIRECTION('ref_axis',(0.,1.,0.));
#122235=DIRECTION('',(0.,-1.23467863058847E-16,1.));
#122236=DIRECTION('',(0.,1.23467863058847E-16,-1.));
#122237=DIRECTION('center_axis',(0.,0.,-1.));
#122238=DIRECTION('ref_axis',(0.,1.,0.));
#122239=DIRECTION('center_axis',(0.,0.,-1.));
#122240=DIRECTION('ref_axis',(0.,1.,0.));
#122241=DIRECTION('',(0.,-1.23467863058847E-16,1.));
#122242=DIRECTION('',(0.,1.23467863058847E-16,-1.));
#122243=DIRECTION('center_axis',(0.,0.,-1.));
#122244=DIRECTION('ref_axis',(0.,1.,0.));
#122245=DIRECTION('center_axis',(0.,0.,-1.));
#122246=DIRECTION('ref_axis',(0.,1.,0.));
#122247=DIRECTION('',(0.,-1.23467863058847E-16,1.));
#122248=DIRECTION('',(0.,1.23467863058847E-16,-1.));
#122249=DIRECTION('center_axis',(0.,0.,-1.));
#122250=DIRECTION('ref_axis',(0.,1.,0.));
#122251=DIRECTION('center_axis',(0.,0.,1.));
#122252=DIRECTION('ref_axis',(0.,-1.,0.));
#122253=DIRECTION('',(0.,-1.23467863058847E-16,1.));
#122254=DIRECTION('',(0.,1.23467863058847E-16,-1.));
#122255=DIRECTION('center_axis',(0.,0.,-1.));
#122256=DIRECTION('ref_axis',(0.,1.,0.));
#122257=DIRECTION('center_axis',(0.,0.,-1.));
#122258=DIRECTION('ref_axis',(0.,1.,0.));
#122259=DIRECTION('',(0.,-1.23467863058847E-16,1.));
#122260=DIRECTION('',(0.,1.23467863058847E-16,-1.));
#122261=DIRECTION('center_axis',(0.,0.,-1.));
#122262=DIRECTION('ref_axis',(0.,1.,0.));
#122263=DIRECTION('center_axis',(0.,0.,-1.));
#122264=DIRECTION('ref_axis',(0.,1.,0.));
#122265=DIRECTION('',(0.,-1.23467863058847E-16,1.));
#122266=DIRECTION('',(0.,1.23467863058847E-16,-1.));
#122267=DIRECTION('center_axis',(0.,0.,-1.));
#122268=DIRECTION('ref_axis',(0.,1.,0.));
#122269=DIRECTION('center_axis',(0.,0.,-1.));
#122270=DIRECTION('ref_axis',(0.,1.,0.));
#122271=DIRECTION('',(0.,-1.23467863058847E-16,1.));
#122272=DIRECTION('',(0.,1.23467863058847E-16,-1.));
#122273=DIRECTION('center_axis',(0.,0.,-1.));
#122274=DIRECTION('ref_axis',(0.,1.,0.));
#122275=DIRECTION('center_axis',(0.,0.,-1.));
#122276=DIRECTION('ref_axis',(0.,1.,0.));
#122277=DIRECTION('',(0.,-1.23467863058847E-16,1.));
#122278=DIRECTION('',(0.,1.23467863058847E-16,-1.));
#122279=DIRECTION('center_axis',(0.,0.,-1.));
#122280=DIRECTION('ref_axis',(0.,1.,0.));
#122281=DIRECTION('center_axis',(0.,0.,-1.));
#122282=DIRECTION('ref_axis',(0.,1.,0.));
#122283=DIRECTION('center_axis',(0.,0.,-1.));
#122284=DIRECTION('ref_axis',(0.,1.,0.));
#122285=DIRECTION('',(0.,-1.23467863058847E-16,1.));
#122286=DIRECTION('',(0.,1.23467863058847E-16,-1.));
#122287=DIRECTION('center_axis',(0.,0.,1.));
#122288=DIRECTION('ref_axis',(0.,-1.,0.));
#122289=DIRECTION('',(0.,-1.23467863058847E-16,1.));
#122290=DIRECTION('',(0.,1.23467863058847E-16,-1.));
#122291=DIRECTION('center_axis',(0.,0.,-1.));
#122292=DIRECTION('ref_axis',(0.,1.,0.));
#122293=DIRECTION('center_axis',(0.,0.,-1.));
#122294=DIRECTION('ref_axis',(0.,1.,0.));
#122295=DIRECTION('',(0.,-1.23467863058847E-16,1.));
#122296=DIRECTION('',(0.,1.23467863058847E-16,-1.));
#122297=DIRECTION('center_axis',(0.,0.,-1.));
#122298=DIRECTION('ref_axis',(0.,1.,0.));
#122299=DIRECTION('center_axis',(0.,0.,1.));
#122300=DIRECTION('ref_axis',(0.,-1.,0.));
#122301=DIRECTION('',(0.,-1.23467863058847E-16,1.));
#122302=DIRECTION('',(0.,1.23467863058847E-16,-1.));
#122303=DIRECTION('center_axis',(0.,0.,-1.));
#122304=DIRECTION('ref_axis',(0.,1.,0.));
#122305=DIRECTION('center_axis',(-1.3684555315672E-48,0.,-1.));
#122306=DIRECTION('ref_axis',(0.,1.,0.));
#122307=DIRECTION('',(1.3684555315672E-48,-1.23467863058847E-16,1.));
#122308=DIRECTION('',(0.,1.23467863058847E-16,-1.));
#122309=DIRECTION('center_axis',(0.,0.,-1.));
#122310=DIRECTION('ref_axis',(0.,1.,0.));
#122311=DIRECTION('center_axis',(0.,0.,-1.));
#122312=DIRECTION('ref_axis',(-0.701138397908223,-0.713025207814346,0.));
#122313=DIRECTION('',(0.,-1.23467863058847E-16,1.));
#122314=DIRECTION('',(-1.3684555315672E-48,1.23467863058847E-16,-1.));
#122315=DIRECTION('center_axis',(0.,0.,-1.));
#122316=DIRECTION('ref_axis',(0.,1.,0.));
#122317=DIRECTION('center_axis',(0.,0.,1.));
#122318=DIRECTION('ref_axis',(0.,-1.,0.));
#122319=DIRECTION('',(0.,-1.23467863058847E-16,1.));
#122320=DIRECTION('',(0.,1.23467863058847E-16,-1.));
#122321=DIRECTION('center_axis',(0.,0.,-1.));
#122322=DIRECTION('ref_axis',(0.,1.,0.));
#122323=DIRECTION('center_axis',(-1.3684555315672E-48,0.,-1.));
#122324=DIRECTION('ref_axis',(0.,1.,0.));
#122325=DIRECTION('',(1.3684555315672E-48,-1.23467863058847E-16,1.));
#122326=DIRECTION('',(0.,1.23467863058847E-16,-1.));
#122327=DIRECTION('center_axis',(0.,0.,-1.));
#122328=DIRECTION('ref_axis',(0.,1.,0.));
#122329=DIRECTION('center_axis',(1.3684555315672E-48,0.,1.));
#122330=DIRECTION('ref_axis',(0.,-1.,0.));
#122331=DIRECTION('',(0.,-1.23467863058847E-16,1.));
#122332=DIRECTION('',(-1.3684555315672E-48,1.23467863058847E-16,-1.));
#122333=DIRECTION('center_axis',(0.,0.,-1.));
#122334=DIRECTION('ref_axis',(0.,1.,0.));
#122335=DIRECTION('center_axis',(0.,0.,-1.));
#122336=DIRECTION('ref_axis',(0.,1.,0.));
#122337=DIRECTION('',(0.,-1.23467863058847E-16,1.));
#122338=DIRECTION('',(0.,1.23467863058847E-16,-1.));
#122339=DIRECTION('center_axis',(0.,0.,-1.));
#122340=DIRECTION('ref_axis',(0.,1.,0.));
#122341=DIRECTION('center_axis',(0.,0.,1.));
#122342=DIRECTION('ref_axis',(0.,-1.,0.));
#122343=DIRECTION('',(0.,-1.23467863058847E-16,1.));
#122344=DIRECTION('',(0.,1.23467863058847E-16,-1.));
#122345=DIRECTION('center_axis',(0.,0.,-1.));
#122346=DIRECTION('ref_axis',(0.,1.,0.));
#122347=DIRECTION('center_axis',(-1.3684555315672E-48,0.,-1.));
#122348=DIRECTION('ref_axis',(0.,1.,0.));
#122349=DIRECTION('',(1.3684555315672E-48,-1.23467863058847E-16,1.));
#122350=DIRECTION('',(0.,1.23467863058847E-16,-1.));
#122351=DIRECTION('center_axis',(0.,0.,-1.));
#122352=DIRECTION('ref_axis',(0.,1.,0.));
#122353=DIRECTION('center_axis',(1.3684555315672E-48,0.,1.));
#122354=DIRECTION('ref_axis',(0.,-1.,0.));
#122355=DIRECTION('',(0.,-1.23467863058847E-16,1.));
#122356=DIRECTION('',(-1.3684555315672E-48,1.23467863058847E-16,-1.));
#122357=DIRECTION('center_axis',(0.,0.,-1.));
#122358=DIRECTION('ref_axis',(0.,1.,0.));
#122359=DIRECTION('center_axis',(0.,0.,-1.));
#122360=DIRECTION('ref_axis',(0.,1.,0.));
#122361=DIRECTION('',(0.,-1.23467863058847E-16,1.));
#122362=DIRECTION('',(0.,1.23467863058847E-16,-1.));
#122363=DIRECTION('center_axis',(0.,0.,-1.));
#122364=DIRECTION('ref_axis',(0.,1.,0.));
#122365=DIRECTION('center_axis',(0.,0.,1.));
#122366=DIRECTION('ref_axis',(0.,-1.,0.));
#122367=DIRECTION('',(0.,-1.23467863058847E-16,1.));
#122368=DIRECTION('',(0.,1.23467863058847E-16,-1.));
#122369=DIRECTION('center_axis',(0.,0.,-1.));
#122370=DIRECTION('ref_axis',(0.,1.,0.));
#122371=DIRECTION('center_axis',(-1.3684555315672E-48,0.,-1.));
#122372=DIRECTION('ref_axis',(0.,1.,0.));
#122373=DIRECTION('',(1.3684555315672E-48,-1.23467863058847E-16,1.));
#122374=DIRECTION('',(0.,1.23467863058847E-16,-1.));
#122375=DIRECTION('center_axis',(0.,0.,-1.));
#122376=DIRECTION('ref_axis',(0.,1.,0.));
#122377=DIRECTION('center_axis',(1.3684555315672E-48,0.,1.));
#122378=DIRECTION('ref_axis',(0.,-1.,0.));
#122379=DIRECTION('',(0.,-1.23467863058847E-16,1.));
#122380=DIRECTION('',(-1.3684555315672E-48,1.23467863058847E-16,-1.));
#122381=DIRECTION('center_axis',(0.,0.,-1.));
#122382=DIRECTION('ref_axis',(0.,1.,0.));
#122383=DIRECTION('center_axis',(0.,0.,-1.));
#122384=DIRECTION('ref_axis',(0.,1.,0.));
#122385=DIRECTION('',(0.,-1.23467863058847E-16,1.));
#122386=DIRECTION('',(0.,1.23467863058847E-16,-1.));
#122387=DIRECTION('center_axis',(0.,0.,-1.));
#122388=DIRECTION('ref_axis',(0.,1.,0.));
#122389=DIRECTION('center_axis',(0.,0.,-1.));
#122390=DIRECTION('ref_axis',(0.,1.,0.));
#122391=DIRECTION('',(0.,-1.23467863058847E-16,1.));
#122392=DIRECTION('',(0.,1.23467863058847E-16,-1.));
#122393=DIRECTION('center_axis',(0.,0.,-1.));
#122394=DIRECTION('ref_axis',(0.,1.,0.));
#122395=DIRECTION('center_axis',(0.,0.,1.));
#122396=DIRECTION('ref_axis',(0.,-1.,0.));
#122397=DIRECTION('',(0.,-1.23467863058847E-16,1.));
#122398=DIRECTION('',(0.,1.23467863058847E-16,-1.));
#122399=DIRECTION('center_axis',(0.,0.,-1.));
#122400=DIRECTION('ref_axis',(0.,1.,0.));
#122401=DIRECTION('center_axis',(-1.3684555315672E-48,0.,-1.));
#122402=DIRECTION('ref_axis',(0.,1.,0.));
#122403=DIRECTION('',(1.3684555315672E-48,-1.23467863058847E-16,1.));
#122404=DIRECTION('',(0.,1.23467863058847E-16,-1.));
#122405=DIRECTION('center_axis',(0.,0.,-1.));
#122406=DIRECTION('ref_axis',(0.,1.,0.));
#122407=DIRECTION('center_axis',(1.3684555315672E-48,0.,1.));
#122408=DIRECTION('ref_axis',(0.,-1.,0.));
#122409=DIRECTION('',(0.,-1.23467863058847E-16,1.));
#122410=DIRECTION('',(-1.3684555315672E-48,1.23467863058847E-16,-1.));
#122411=DIRECTION('center_axis',(0.,0.,-1.));
#122412=DIRECTION('ref_axis',(0.,1.,0.));
#122413=DIRECTION('center_axis',(0.,0.,-1.));
#122414=DIRECTION('ref_axis',(0.,1.,0.));
#122415=DIRECTION('',(0.,-1.23467863058847E-16,1.));
#122416=DIRECTION('',(0.,1.23467863058847E-16,-1.));
#122417=DIRECTION('center_axis',(0.,0.,-1.));
#122418=DIRECTION('ref_axis',(0.,1.,0.));
#122419=DIRECTION('center_axis',(0.,0.,-1.));
#122420=DIRECTION('ref_axis',(0.,1.,0.));
#122421=DIRECTION('',(0.,-1.23467863058847E-16,1.));
#122422=DIRECTION('',(0.,1.23467863058847E-16,-1.));
#122423=DIRECTION('center_axis',(0.,0.,-1.));
#122424=DIRECTION('ref_axis',(0.,1.,0.));
#122425=DIRECTION('center_axis',(0.,0.,-1.));
#122426=DIRECTION('ref_axis',(0.,1.,0.));
#122427=DIRECTION('center_axis',(0.,0.,-1.));
#122428=DIRECTION('ref_axis',(0.,1.,0.));
#122429=DIRECTION('',(1.3684555315672E-48,-1.23467863058847E-16,1.));
#122430=DIRECTION('',(0.,1.23467863058847E-16,-1.));
#122431=DIRECTION('center_axis',(1.3684555315672E-48,0.,1.));
#122432=DIRECTION('ref_axis',(0.,-1.,0.));
#122433=DIRECTION('',(1.3684555315672E-48,-1.23467863058847E-16,1.));
#122434=DIRECTION('',(-1.3684555315672E-48,1.23467863058847E-16,-1.));
#122435=DIRECTION('center_axis',(0.,0.,-1.));
#122436=DIRECTION('ref_axis',(0.,1.,0.));
#122437=DIRECTION('center_axis',(0.,0.,-1.));
#122438=DIRECTION('ref_axis',(0.,1.,0.));
#122439=DIRECTION('',(0.,-1.23467863058847E-16,1.));
#122440=DIRECTION('',(0.,1.23467863058847E-16,-1.));
#122441=DIRECTION('center_axis',(0.,0.,-1.));
#122442=DIRECTION('ref_axis',(0.,1.,0.));
#122443=DIRECTION('center_axis',(0.,0.,1.));
#122444=DIRECTION('ref_axis',(0.,-1.,0.));
#122445=DIRECTION('',(0.,-1.23467863058847E-16,1.));
#122446=DIRECTION('',(0.,1.23467863058847E-16,-1.));
#122447=DIRECTION('center_axis',(0.,0.,-1.));
#122448=DIRECTION('ref_axis',(0.,1.,0.));
#122449=DIRECTION('center_axis',(0.,0.,-1.));
#122450=DIRECTION('ref_axis',(0.,1.,0.));
#122451=DIRECTION('',(0.,-1.23467863058847E-16,1.));
#122452=DIRECTION('',(0.,1.23467863058847E-16,-1.));
#122453=DIRECTION('center_axis',(0.,0.,-1.));
#122454=DIRECTION('ref_axis',(0.,1.,0.));
#122455=DIRECTION('center_axis',(0.,0.,-1.));
#122456=DIRECTION('ref_axis',(-0.706453380948025,-0.707759578209369,0.));
#122457=DIRECTION('',(0.,-1.23467863058847E-16,1.));
#122458=DIRECTION('',(0.,1.23467863058847E-16,-1.));
#122459=DIRECTION('center_axis',(0.,0.,-1.));
#122460=DIRECTION('ref_axis',(0.,1.,0.));
#122461=DIRECTION('center_axis',(0.,0.,1.));
#122462=DIRECTION('ref_axis',(0.,-1.,0.));
#122463=DIRECTION('',(0.,-1.23467863058847E-16,1.));
#122464=DIRECTION('',(0.,1.23467863058847E-16,-1.));
#122465=DIRECTION('center_axis',(0.,0.,-1.));
#122466=DIRECTION('ref_axis',(0.,1.,0.));
#122467=DIRECTION('center_axis',(0.,0.,-1.));
#122468=DIRECTION('ref_axis',(0.,1.,0.));
#122469=DIRECTION('',(0.,-1.23467863058847E-16,1.));
#122470=DIRECTION('',(0.,1.23467863058847E-16,-1.));
#122471=DIRECTION('center_axis',(0.,0.,-1.));
#122472=DIRECTION('ref_axis',(0.,1.,0.));
#122473=DIRECTION('center_axis',(0.,0.,1.));
#122474=DIRECTION('ref_axis',(0.,-1.,0.));
#122475=DIRECTION('',(0.,-1.23467863058847E-16,1.));
#122476=DIRECTION('',(0.,1.23467863058847E-16,-1.));
#122477=DIRECTION('center_axis',(0.,0.,-1.));
#122478=DIRECTION('ref_axis',(0.,1.,0.));
#122479=DIRECTION('center_axis',(0.,0.,-1.));
#122480=DIRECTION('ref_axis',(0.,1.,0.));
#122481=DIRECTION('',(0.,-1.23467863058847E-16,1.));
#122482=DIRECTION('',(0.,1.23467863058847E-16,-1.));
#122483=DIRECTION('center_axis',(0.,0.,-1.));
#122484=DIRECTION('ref_axis',(0.,1.,0.));
#122485=DIRECTION('center_axis',(0.,0.,-1.));
#122486=DIRECTION('ref_axis',(0.,1.,0.));
#122487=DIRECTION('',(0.,-1.23467863058847E-16,1.));
#122488=DIRECTION('',(0.,1.23467863058847E-16,-1.));
#122489=DIRECTION('center_axis',(0.,0.,-1.));
#122490=DIRECTION('ref_axis',(0.,1.,0.));
#122491=DIRECTION('center_axis',(0.,0.,1.));
#122492=DIRECTION('ref_axis',(0.,-1.,0.));
#122493=DIRECTION('',(0.,-1.23467863058847E-16,1.));
#122494=DIRECTION('',(0.,1.23467863058847E-16,-1.));
#122495=DIRECTION('center_axis',(0.,0.,-1.));
#122496=DIRECTION('ref_axis',(0.,1.,0.));
#122497=DIRECTION('center_axis',(0.,0.,-1.));
#122498=DIRECTION('ref_axis',(0.,1.,0.));
#122499=DIRECTION('',(0.,-1.23467863058847E-16,1.));
#122500=DIRECTION('',(0.,1.23467863058847E-16,-1.));
#122501=DIRECTION('center_axis',(0.,0.,-1.));
#122502=DIRECTION('ref_axis',(0.,1.,0.));
#122503=DIRECTION('center_axis',(0.,0.,1.));
#122504=DIRECTION('ref_axis',(0.,-1.,0.));
#122505=DIRECTION('',(0.,-1.23467863058847E-16,1.));
#122506=DIRECTION('',(0.,1.23467863058847E-16,-1.));
#122507=DIRECTION('center_axis',(0.,0.,-1.));
#122508=DIRECTION('ref_axis',(0.,1.,0.));
#122509=DIRECTION('center_axis',(0.,0.,-1.));
#122510=DIRECTION('ref_axis',(0.,1.,0.));
#122511=DIRECTION('',(0.,-1.23467863058847E-16,1.));
#122512=DIRECTION('',(0.,1.23467863058847E-16,-1.));
#122513=DIRECTION('center_axis',(0.,0.,-1.));
#122514=DIRECTION('ref_axis',(0.,1.,0.));
#122515=DIRECTION('center_axis',(0.,0.,-1.));
#122516=DIRECTION('ref_axis',(0.,1.,0.));
#122517=DIRECTION('',(0.,-1.23467863058847E-16,1.));
#122518=DIRECTION('',(0.,1.23467863058847E-16,-1.));
#122519=DIRECTION('center_axis',(0.,0.,-1.));
#122520=DIRECTION('ref_axis',(0.,1.,0.));
#122521=DIRECTION('center_axis',(0.,0.,-1.));
#122522=DIRECTION('ref_axis',(0.,1.,0.));
#122523=DIRECTION('center_axis',(0.,0.,-1.));
#122524=DIRECTION('ref_axis',(0.,1.,0.));
#122525=DIRECTION('',(0.,-1.23467863058847E-16,1.));
#122526=DIRECTION('',(0.,1.23467863058847E-16,-1.));
#122527=DIRECTION('center_axis',(0.,0.,1.));
#122528=DIRECTION('ref_axis',(0.,-1.,0.));
#122529=DIRECTION('',(0.,-1.23467863058847E-16,1.));
#122530=DIRECTION('',(0.,1.23467863058847E-16,-1.));
#122531=DIRECTION('center_axis',(0.,0.,-1.));
#122532=DIRECTION('ref_axis',(0.,1.,0.));
#122533=DIRECTION('center_axis',(0.,0.,-1.));
#122534=DIRECTION('ref_axis',(0.0361435302645155,-0.999346609150208,0.));
#122535=DIRECTION('',(0.,-1.23467863058847E-16,1.));
#122536=DIRECTION('',(-1.27503726478586E-32,1.23467863058847E-16,-1.));
#122537=DIRECTION('center_axis',(0.,0.,-1.));
#122538=DIRECTION('ref_axis',(0.,1.,0.));
#122539=DIRECTION('center_axis',(0.,0.,-1.));
#122540=DIRECTION('ref_axis',(0.,1.,0.));
#122541=DIRECTION('',(0.,-1.23467863058847E-16,1.));
#122542=DIRECTION('',(0.,1.23467863058847E-16,-1.));
#122543=DIRECTION('center_axis',(0.,0.,-1.));
#122544=DIRECTION('ref_axis',(0.,1.,0.));
#122545=DIRECTION('center_axis',(0.,0.,-1.));
#122546=DIRECTION('ref_axis',(0.,1.,0.));
#122547=DIRECTION('',(0.,-1.23467863058847E-16,1.));
#122548=DIRECTION('',(0.,1.23467863058847E-16,-1.));
#122549=DIRECTION('center_axis',(0.,0.,-1.));
#122550=DIRECTION('ref_axis',(0.,1.,0.));
#122551=DIRECTION('center_axis',(0.,0.,-1.));
#122552=DIRECTION('ref_axis',(0.,1.,0.));
#122553=DIRECTION('center_axis',(0.,0.,-1.));
#122554=DIRECTION('ref_axis',(0.,1.,0.));
#122555=DIRECTION('',(0.,-1.23467863058847E-16,1.));
#122556=DIRECTION('',(0.,1.23467863058847E-16,-1.));
#122557=DIRECTION('center_axis',(0.,0.,-1.));
#122558=DIRECTION('ref_axis',(-0.663057938251906,-0.748568080084324,0.));
#122559=DIRECTION('',(0.,-1.23467863058847E-16,1.));
#122560=DIRECTION('',(0.,1.23467863058847E-16,-1.));
#122561=DIRECTION('center_axis',(0.,0.,-1.));
#122562=DIRECTION('ref_axis',(0.,1.,0.));
#122563=DIRECTION('center_axis',(0.,0.,-1.));
#122564=DIRECTION('ref_axis',(0.,1.,0.));
#122565=DIRECTION('center_axis',(0.,0.,-1.));
#122566=DIRECTION('ref_axis',(0.,1.,0.));
#122567=DIRECTION('',(0.,-1.23467863058847E-16,1.));
#122568=DIRECTION('',(0.,1.23467863058847E-16,-1.));
#122569=DIRECTION('center_axis',(0.,0.,-1.));
#122570=DIRECTION('ref_axis',(0.,1.,0.));
#122571=DIRECTION('',(3.82498197630791E-33,-1.23467863058847E-16,1.));
#122572=DIRECTION('',(0.,1.23467863058847E-16,-1.));
#122573=DIRECTION('center_axis',(0.,0.,-1.));
#122574=DIRECTION('ref_axis',(0.,1.,0.));
#122575=DIRECTION('center_axis',(0.,0.,-1.));
#122576=DIRECTION('ref_axis',(0.,1.,0.));
#122577=DIRECTION('',(0.,-1.23467863058847E-16,1.));
#122578=DIRECTION('',(-1.3684555315672E-48,1.23467863058847E-16,-1.));
#122579=DIRECTION('center_axis',(0.,0.,-1.));
#122580=DIRECTION('ref_axis',(0.,1.,0.));
#122581=DIRECTION('center_axis',(0.,0.,-1.));
#122582=DIRECTION('ref_axis',(0.,1.,0.));
#122583=DIRECTION('',(1.3684555315672E-48,-1.23467863058847E-16,1.));
#122584=DIRECTION('',(0.,1.23467863058847E-16,-1.));
#122585=DIRECTION('center_axis',(0.,0.,-1.));
#122586=DIRECTION('ref_axis',(0.,1.,0.));
#122587=DIRECTION('center_axis',(0.,0.,-1.));
#122588=DIRECTION('ref_axis',(0.,1.,0.));
#122589=DIRECTION('',(0.,-1.23467863058847E-16,1.));
#122590=DIRECTION('center_axis',(0.,0.,-1.));
#122591=DIRECTION('ref_axis',(0.,1.,0.));
#122592=DIRECTION('center_axis',(0.,0.,-1.));
#122593=DIRECTION('ref_axis',(0.,1.,0.));
#122594=DIRECTION('',(0.,1.23467863058847E-16,-1.));
#122595=DIRECTION('center_axis',(0.,0.,-1.));
#122596=DIRECTION('ref_axis',(0.,1.,0.));
#122597=DIRECTION('center_axis',(0.,1.23467863058847E-16,-1.));
#122598=DIRECTION('ref_axis',(-1.,0.,0.));
#122599=DIRECTION('center_axis',(0.,0.,-1.));
#122600=DIRECTION('ref_axis',(0.,1.,0.));
#122601=DIRECTION('center_axis',(0.,0.,-1.));
#122602=DIRECTION('ref_axis',(0.,1.,0.));
#122603=DIRECTION('',(0.,0.,-1.));
#122604=DIRECTION('center_axis',(0.,1.23467863058847E-16,-1.));
#122605=DIRECTION('ref_axis',(-1.,0.,0.));
#122606=DIRECTION('center_axis',(0.,0.,-1.));
#122607=DIRECTION('ref_axis',(0.,1.,0.));
#122608=DIRECTION('center_axis',(0.,0.,1.));
#122609=DIRECTION('ref_axis',(0.,1.,0.));
#122610=DIRECTION('center_axis',(0.,0.,-1.));
#122611=DIRECTION('ref_axis',(0.,1.,0.));
#122612=DIRECTION('center_axis',(-5.48307457476793E-31,-2.43497425545765E-45,
1.));
#122613=DIRECTION('ref_axis',(-4.44089209850063E-15,1.,-3.42265840282363E-60));
#122614=DIRECTION('center_axis',(0.,0.,-1.));
#122615=DIRECTION('ref_axis',(0.,1.,0.));
#122616=DIRECTION('',(0.,0.,1.));
#122617=DIRECTION('center_axis',(0.,0.,-1.));
#122618=DIRECTION('ref_axis',(0.,1.,0.));
#122619=DIRECTION('center_axis',(0.,0.,-1.));
#122620=DIRECTION('ref_axis',(0.,1.,0.));
#122621=DIRECTION('center_axis',(0.,0.,1.));
#122622=DIRECTION('ref_axis',(0.,1.,0.));
#122623=DIRECTION('center_axis',(0.,0.,-1.));
#122624=DIRECTION('ref_axis',(0.,1.,0.));
#122625=DIRECTION('center_axis',(0.,0.,1.));
#122626=DIRECTION('ref_axis',(0.,1.,0.));
#122627=DIRECTION('center_axis',(-6.57968948972152E-31,3.50636292785902E-45,
-1.));
#122628=DIRECTION('ref_axis',(5.32907051820075E-15,1.,-4.97841222228891E-60));
#122629=DIRECTION('center_axis',(0.,0.,1.));
#122630=DIRECTION('ref_axis',(0.,1.,0.));
#122631=DIRECTION('center_axis',(7.6763044046751E-31,4.77254954069701E-45,
-1.));
#122632=DIRECTION('ref_axis',(-6.21724893790088E-15,1.,-2.48920611114446E-60));
#122633=DIRECTION('center_axis',(0.,0.,-1.));
#122634=DIRECTION('ref_axis',(0.,1.,0.));
#122635=DIRECTION('center_axis',(7.6763044046751E-31,-4.77254954069701E-45,
1.));
#122636=DIRECTION('ref_axis',(6.21724893790088E-15,1.,-2.48920611114446E-60));
#122637=DIRECTION('center_axis',(0.,0.,-1.));
#122638=DIRECTION('ref_axis',(0.,1.,0.));
#122639=DIRECTION('center_axis',(-6.57968948972152E-31,-3.50636292785902E-45,
1.));
#122640=DIRECTION('ref_axis',(-5.32907051820075E-15,1.,-4.97841222228891E-60));
#122641=DIRECTION('center_axis',(0.,0.,-1.));
#122642=DIRECTION('ref_axis',(0.,1.,0.));
#122643=DIRECTION('center_axis',(0.,0.,1.));
#122644=DIRECTION('ref_axis',(0.,1.,0.));
#122645=DIRECTION('center_axis',(0.,0.,-1.));
#122646=DIRECTION('ref_axis',(0.,1.,0.));
#122647=DIRECTION('center_axis',(0.,0.,1.));
#122648=DIRECTION('ref_axis',(0.,1.,0.));
#122649=DIRECTION('center_axis',(0.,0.,-1.));
#122650=DIRECTION('ref_axis',(0.,1.,0.));
#122651=DIRECTION('center_axis',(0.,0.,-1.));
#122652=DIRECTION('ref_axis',(0.,1.,0.));
#122653=DIRECTION('center_axis',(0.,0.,1.));
#122654=DIRECTION('ref_axis',(0.,1.,0.));
#122655=DIRECTION('center_axis',(0.724113717892013,0.689680595319751,8.51533892972834E-17));
#122656=DIRECTION('ref_axis',(-4.33608168928332E-33,1.23467863058847E-16,
-1.));
#122657=DIRECTION('',(-0.689680595319751,0.724113717892013,8.9404773359724E-17));
#122658=DIRECTION('center_axis',(-0.724113717892013,-0.689680595319751,
-8.51533892972834E-17));
#122659=DIRECTION('ref_axis',(-0.689680595319751,0.724113717892013,-2.49214163614276E-33));
#122660=DIRECTION('',(0.689680595319751,-0.724113717892013,-8.9404773359724E-17));
#122661=DIRECTION('center_axis',(0.,0.,-1.));
#122662=DIRECTION('ref_axis',(0.,1.,0.));
#122663=DIRECTION('center_axis',(2.19322982990717E-31,-3.89595880873225E-46,
1.));
#122664=DIRECTION('ref_axis',(1.77635683940025E-15,1.,7.77876909732643E-62));
#122665=DIRECTION('center_axis',(0.,0.,-1.));
#122666=DIRECTION('ref_axis',(0.,1.,0.));
#122667=DIRECTION('center_axis',(-4.38645965981435E-31,-1.5583835234929E-45,
1.));
#122668=DIRECTION('ref_axis',(-3.5527136788005E-15,1.,-9.33452291679171E-61));
#122669=DIRECTION('center_axis',(0.,0.,-1.));
#122670=DIRECTION('ref_axis',(0.,1.,0.));
#122671=DIRECTION('center_axis',(7.6763044046751E-31,-4.77254954069701E-45,
1.));
#122672=DIRECTION('ref_axis',(6.21724893790088E-15,1.,-1.86690458335834E-60));
#122673=DIRECTION('center_axis',(-0.724113717892013,0.689680595319752,8.51533892972836E-17));
#122674=DIRECTION('ref_axis',(1.17596707800504E-16,1.43114502276974E-33,
1.));
#122675=DIRECTION('',(-0.689680595319752,-0.724113717892012,-8.94047733597238E-17));
#122676=DIRECTION('center_axis',(0.724113717892013,-0.689680595319752,-8.51533892972834E-17));
#122677=DIRECTION('ref_axis',(-1.94663562866425E-33,1.23467863058847E-16,
-1.));
#122678=DIRECTION('',(0.689680595319752,0.724113717892012,8.94047733597238E-17));
#122679=DIRECTION('center_axis',(0.,0.,-1.));
#122680=DIRECTION('ref_axis',(0.,1.,0.));
#122681=DIRECTION('center_axis',(-1.09661491495359E-31,-9.73989702183063E-47,
1.));
#122682=DIRECTION('ref_axis',(-8.88178419700125E-16,1.,0.));
#122683=DIRECTION('center_axis',(0.,0.,-1.));
#122684=DIRECTION('ref_axis',(0.,1.,0.));
#122685=DIRECTION('center_axis',(-9.86953423458227E-31,-7.88931658768281E-45,
1.));
#122686=DIRECTION('ref_axis',(-7.99360577730113E-15,1.,-2.48920611114446E-60));
#122687=DIRECTION('center_axis',(1.,0.,0.));
#122688=DIRECTION('ref_axis',(0.,1.,0.));
#122689=DIRECTION('',(0.,1.,0.));
#122690=DIRECTION('center_axis',(-1.,0.,0.));
#122691=DIRECTION('ref_axis',(0.,0.,1.));
#122692=DIRECTION('',(0.,-1.,0.));
#122693=DIRECTION('center_axis',(-1.,0.,0.));
#122694=DIRECTION('ref_axis',(0.,0.,1.));
#122695=DIRECTION('',(0.,-1.,0.));
#122696=DIRECTION('center_axis',(1.,0.,0.));
#122697=DIRECTION('ref_axis',(0.,1.,0.));
#122698=DIRECTION('',(0.,1.,0.));
#122699=DIRECTION('center_axis',(-1.,0.,0.));
#122700=DIRECTION('ref_axis',(0.,0.,1.));
#122701=DIRECTION('',(0.,-1.,0.));
#122702=DIRECTION('center_axis',(1.,0.,0.));
#122703=DIRECTION('ref_axis',(0.,1.,0.));
#122704=DIRECTION('',(0.,1.,0.));
#122705=DIRECTION('center_axis',(-1.,0.,0.));
#122706=DIRECTION('ref_axis',(0.,0.,1.));
#122707=DIRECTION('',(0.,-1.,0.));
#122708=DIRECTION('center_axis',(1.,0.,0.));
#122709=DIRECTION('ref_axis',(0.,1.,0.));
#122710=DIRECTION('',(0.,1.,0.));
#122711=DIRECTION('center_axis',(-1.,0.,0.));
#122712=DIRECTION('ref_axis',(0.,0.,1.));
#122713=DIRECTION('',(0.,-1.,0.));
#122714=DIRECTION('center_axis',(1.,0.,0.));
#122715=DIRECTION('ref_axis',(0.,1.,0.));
#122716=DIRECTION('',(0.,1.,0.));
#122717=DIRECTION('center_axis',(-1.,0.,0.));
#122718=DIRECTION('ref_axis',(0.,0.,1.));
#122719=DIRECTION('',(0.,-1.,0.));
#122720=DIRECTION('center_axis',(1.,0.,0.));
#122721=DIRECTION('ref_axis',(0.,1.,0.));
#122722=DIRECTION('',(0.,1.,0.));
#122723=DIRECTION('center_axis',(-1.,0.,0.));
#122724=DIRECTION('ref_axis',(0.,0.,1.));
#122725=DIRECTION('',(0.,-1.,0.));
#122726=DIRECTION('center_axis',(1.,0.,0.));
#122727=DIRECTION('ref_axis',(0.,1.,0.));
#122728=DIRECTION('',(0.,1.,0.));
#122729=DIRECTION('center_axis',(-1.,0.,0.));
#122730=DIRECTION('ref_axis',(0.,0.,1.));
#122731=DIRECTION('',(0.,-1.,0.));
#122732=DIRECTION('center_axis',(1.,0.,0.));
#122733=DIRECTION('ref_axis',(0.,1.,0.));
#122734=DIRECTION('',(0.,1.,0.));
#122735=DIRECTION('center_axis',(1.,7.82779334765923E-17,9.66480917101747E-33));
#122736=DIRECTION('ref_axis',(-7.82779334765923E-17,1.,1.39213059235047E-65));
#122737=DIRECTION('',(-7.82779334765923E-17,1.,0.));
#122738=DIRECTION('center_axis',(-1.,7.82779334765923E-17,9.66480917101747E-33));
#122739=DIRECTION('ref_axis',(9.66480917101747E-33,0.,1.));
#122740=DIRECTION('',(-7.82779334765923E-17,-1.,0.));
#122741=DIRECTION('center_axis',(-1.,7.82779334765923E-17,9.66480917101747E-33));
#122742=DIRECTION('ref_axis',(9.66480917101747E-33,0.,1.));
#122743=DIRECTION('',(-7.82779334765923E-17,-1.,0.));
#122744=DIRECTION('center_axis',(1.,7.82779334765923E-17,9.66480917101747E-33));
#122745=DIRECTION('ref_axis',(-7.82779334765923E-17,1.,1.39213059235047E-65));
#122746=DIRECTION('',(-7.82779334765923E-17,1.,0.));
#122747=DIRECTION('center_axis',(-1.,7.82779334765923E-17,9.66480917101747E-33));
#122748=DIRECTION('ref_axis',(9.66480917101747E-33,0.,1.));
#122749=DIRECTION('',(-7.82779334765923E-17,-1.,0.));
#122750=DIRECTION('center_axis',(1.,7.82779334765923E-17,9.66480917101747E-33));
#122751=DIRECTION('ref_axis',(-7.82779334765923E-17,1.,1.39213059235047E-65));
#122752=DIRECTION('',(-7.82779334765923E-17,1.,0.));
#122753=DIRECTION('center_axis',(-1.,7.82779334765923E-17,9.66480917101747E-33));
#122754=DIRECTION('ref_axis',(9.66480917101747E-33,0.,1.));
#122755=DIRECTION('',(-7.82779334765923E-17,-1.,0.));
#122756=DIRECTION('center_axis',(1.,7.82779334765923E-17,9.66480917101747E-33));
#122757=DIRECTION('ref_axis',(-7.82779334765923E-17,1.,1.39213059235047E-65));
#122758=DIRECTION('',(-7.82779334765923E-17,1.,0.));
#122759=DIRECTION('center_axis',(-1.,7.82779334765923E-17,9.66480917101747E-33));
#122760=DIRECTION('ref_axis',(9.66480917101747E-33,0.,1.));
#122761=DIRECTION('',(-7.82779334765923E-17,-1.,0.));
#122762=DIRECTION('center_axis',(1.,7.82779334765923E-17,9.66480917101747E-33));
#122763=DIRECTION('ref_axis',(-7.82779334765923E-17,1.,1.39213059235047E-65));
#122764=DIRECTION('',(-7.82779334765923E-17,1.,0.));
#122765=DIRECTION('center_axis',(-1.,7.82779334765923E-17,9.66480917101747E-33));
#122766=DIRECTION('ref_axis',(9.66480917101747E-33,0.,1.));
#122767=DIRECTION('',(-7.82779334765923E-17,-1.,0.));
#122768=DIRECTION('center_axis',(1.,7.82779334765923E-17,9.66480917101747E-33));
#122769=DIRECTION('ref_axis',(-7.82779334765923E-17,1.,1.39213059235047E-65));
#122770=DIRECTION('',(-7.82779334765923E-17,1.,0.));
#122771=DIRECTION('center_axis',(-1.,7.82779334765923E-17,9.66480917101747E-33));
#122772=DIRECTION('ref_axis',(9.66480917101747E-33,0.,1.));
#122773=DIRECTION('',(-7.82779334765923E-17,-1.,0.));
#122774=DIRECTION('center_axis',(1.,7.82779334765923E-17,9.66480917101747E-33));
#122775=DIRECTION('ref_axis',(-7.82779334765923E-17,1.,1.39213059235047E-65));
#122776=DIRECTION('',(-7.82779334765923E-17,1.,0.));
#122777=DIRECTION('center_axis',(-1.,7.82779334765923E-17,9.66480917101747E-33));
#122778=DIRECTION('ref_axis',(9.66480917101747E-33,0.,1.));
#122779=DIRECTION('',(-7.82779334765923E-17,-1.,0.));
#122780=DIRECTION('center_axis',(1.,7.82779334765923E-17,9.66480917101747E-33));
#122781=DIRECTION('ref_axis',(-7.82779334765923E-17,1.,1.39213059235047E-65));
#122782=DIRECTION('',(-7.82779334765923E-17,1.,0.));
#122783=DIRECTION('center_axis',(0.,-1.,-1.23467863058847E-16));
#122784=DIRECTION('ref_axis',(0.,1.23467863058847E-16,-1.));
#122785=DIRECTION('',(0.,-1.23467863058847E-16,1.));
#122786=DIRECTION('',(-1.,0.,0.));
#122787=DIRECTION('',(0.,-1.23467863058847E-16,1.));
#122788=DIRECTION('',(1.,0.,0.));
#122789=DIRECTION('center_axis',(-1.,7.82779334765923E-17,9.66480917101747E-33));
#122790=DIRECTION('ref_axis',(9.66480917101747E-33,0.,1.));
#122791=DIRECTION('',(0.,-1.23467863058847E-16,1.));
#122792=DIRECTION('',(7.82779334765923E-17,1.,1.23467863058847E-16));
#122793=DIRECTION('',(-7.82779334765923E-17,-1.,0.));
#122794=DIRECTION('center_axis',(1.,7.82779334765923E-17,9.66480917101747E-33));
#122795=DIRECTION('ref_axis',(-7.82779334765923E-17,1.,1.39213059235047E-65));
#122796=DIRECTION('',(7.82779334765923E-17,-1.,-1.23467863058847E-16));
#122797=DIRECTION('',(0.,1.23467863058847E-16,-1.));
#122798=DIRECTION('',(-7.82779334765923E-17,1.,0.));
#122799=DIRECTION('center_axis',(1.,-3.13111733906369E-16,-3.86592366840699E-32));
#122800=DIRECTION('ref_axis',(-3.13111733906369E-16,-1.,-9.91259258008946E-64));
#122801=DIRECTION('',(3.13111733906369E-16,1.,0.));
#122802=DIRECTION('center_axis',(-1.,5.87084501074442E-17,7.2486068782631E-33));
#122803=DIRECTION('ref_axis',(7.2486068782631E-33,0.,1.));
#122804=DIRECTION('',(-5.87084501074442E-17,-1.,0.));
#122805=DIRECTION('center_axis',(-1.,5.87084501074442E-17,7.2486068782631E-33));
#122806=DIRECTION('ref_axis',(7.2486068782631E-33,0.,1.));
#122807=DIRECTION('',(-5.87084501074442E-17,-1.,0.));
#122808=DIRECTION('center_axis',(1.,-3.13111733906369E-16,-3.86592366840699E-32));
#122809=DIRECTION('ref_axis',(-3.13111733906369E-16,-1.,-9.91259258008946E-64));
#122810=DIRECTION('',(3.13111733906369E-16,1.,0.));
#122811=DIRECTION('center_axis',(-1.,5.87084501074442E-17,7.2486068782631E-33));
#122812=DIRECTION('ref_axis',(7.2486068782631E-33,0.,1.));
#122813=DIRECTION('',(-5.87084501074442E-17,-1.,0.));
#122814=DIRECTION('center_axis',(1.,-3.13111733906369E-16,-3.86592366840699E-32));
#122815=DIRECTION('ref_axis',(-3.13111733906369E-16,-1.,-9.91259258008946E-64));
#122816=DIRECTION('',(3.13111733906369E-16,1.,0.));
#122817=DIRECTION('center_axis',(-1.,5.87084501074442E-17,7.2486068782631E-33));
#122818=DIRECTION('ref_axis',(7.2486068782631E-33,0.,1.));
#122819=DIRECTION('',(-5.87084501074442E-17,-1.,0.));
#122820=DIRECTION('center_axis',(1.,-3.13111733906369E-16,-3.86592366840699E-32));
#122821=DIRECTION('ref_axis',(-3.13111733906369E-16,-1.,-9.91259258008946E-64));
#122822=DIRECTION('',(3.13111733906369E-16,1.,0.));
#122823=DIRECTION('center_axis',(-1.,5.87084501074442E-17,7.2486068782631E-33));
#122824=DIRECTION('ref_axis',(7.2486068782631E-33,0.,1.));
#122825=DIRECTION('',(-5.87084501074442E-17,-1.,0.));
#122826=DIRECTION('center_axis',(-1.,5.87084501074442E-17,7.2486068782631E-33));
#122827=DIRECTION('ref_axis',(7.2486068782631E-33,0.,1.));
#122828=DIRECTION('',(-5.87084501074442E-17,-1.,0.));
#122829=DIRECTION('center_axis',(-1.,5.87084501074442E-17,7.2486068782631E-33));
#122830=DIRECTION('ref_axis',(7.2486068782631E-33,0.,1.));
#122831=DIRECTION('',(-5.87084501074442E-17,-1.,0.));
#122832=DIRECTION('center_axis',(1.,-3.13111733906369E-16,-3.86592366840699E-32));
#122833=DIRECTION('ref_axis',(-3.13111733906369E-16,-1.,-9.91259258008946E-64));
#122834=DIRECTION('',(3.13111733906369E-16,1.,0.));
#122835=DIRECTION('center_axis',(-1.,5.87084501074442E-17,7.2486068782631E-33));
#122836=DIRECTION('ref_axis',(7.2486068782631E-33,0.,1.));
#122837=DIRECTION('',(-5.87084501074442E-17,-1.,0.));
#122838=DIRECTION('center_axis',(1.,-3.13111733906369E-16,-3.86592366840699E-32));
#122839=DIRECTION('ref_axis',(-3.13111733906369E-16,-1.,-9.91259258008946E-64));
#122840=DIRECTION('',(3.13111733906369E-16,1.,0.));
#122841=DIRECTION('center_axis',(-1.,6.11546355285877E-17,7.5506321648574E-33));
#122842=DIRECTION('ref_axis',(7.5506321648574E-33,0.,1.));
#122843=DIRECTION('',(-6.11546355285877E-17,-1.,0.));
#122844=DIRECTION('center_axis',(-1.,6.11546355285877E-17,7.5506321648574E-33));
#122845=DIRECTION('ref_axis',(7.5506321648574E-33,0.,1.));
#122846=DIRECTION('',(-6.11546355285877E-17,-1.,0.));
#122847=DIRECTION('center_axis',(-1.,6.11546355285877E-17,7.5506321648574E-33));
#122848=DIRECTION('ref_axis',(7.5506321648574E-33,0.,1.));
#122849=DIRECTION('',(-6.11546355285877E-17,-1.,0.));
#122850=DIRECTION('center_axis',(-1.,6.11546355285877E-17,7.5506321648574E-33));
#122851=DIRECTION('ref_axis',(7.5506321648574E-33,0.,1.));
#122852=DIRECTION('',(-6.11546355285877E-17,-1.,0.));
#122853=DIRECTION('center_axis',(-1.,6.11546355285877E-17,7.5506321648574E-33));
#122854=DIRECTION('ref_axis',(7.5506321648574E-33,0.,1.));
#122855=DIRECTION('',(-6.11546355285877E-17,-1.,0.));
#122856=DIRECTION('center_axis',(-1.,6.11546355285877E-17,7.5506321648574E-33));
#122857=DIRECTION('ref_axis',(7.5506321648574E-33,0.,1.));
#122858=DIRECTION('',(-6.11546355285877E-17,-1.,0.));
#122859=DIRECTION('center_axis',(-1.,6.11546355285877E-17,7.5506321648574E-33));
#122860=DIRECTION('ref_axis',(7.5506321648574E-33,0.,1.));
#122861=DIRECTION('',(-6.11546355285877E-17,-1.,0.));
#122862=DIRECTION('center_axis',(-1.,6.11546355285877E-17,7.5506321648574E-33));
#122863=DIRECTION('ref_axis',(7.5506321648574E-33,0.,1.));
#122864=DIRECTION('',(-6.11546355285877E-17,-1.,0.));
#122865=DIRECTION('center_axis',(0.,1.23467863058847E-16,-1.));
#122866=DIRECTION('ref_axis',(-1.,0.,0.));
#122867=DIRECTION('center_axis',(0.,1.34087697701688E-16,-1.));
#122868=DIRECTION('ref_axis',(0.,1.,1.34087697701688E-16));
#122869=DIRECTION('center_axis',(0.,1.22462808028055E-16,-1.));
#122870=DIRECTION('ref_axis',(0.,1.,1.22462808028055E-16));
#122871=DIRECTION('center_axis',(0.,0.,-1.));
#122872=DIRECTION('ref_axis',(0.,1.,0.));
#122873=DIRECTION('center_axis',(0.,0.,-1.));
#122874=DIRECTION('ref_axis',(0.,1.,0.));
#122875=DIRECTION('center_axis',(0.,0.,-1.));
#122876=DIRECTION('ref_axis',(0.,1.,0.));
#122877=DIRECTION('center_axis',(0.,1.22462808028055E-16,-1.));
#122878=DIRECTION('ref_axis',(0.,1.,1.22462808028055E-16));
#122879=DIRECTION('center_axis',(0.,0.,-1.));
#122880=DIRECTION('ref_axis',(0.,1.,0.));
#122881=DIRECTION('center_axis',(0.,0.,-1.));
#122882=DIRECTION('ref_axis',(0.,1.,0.));
#122883=DIRECTION('center_axis',(0.,0.,-1.));
#122884=DIRECTION('ref_axis',(0.,1.,0.));
#122885=DIRECTION('center_axis',(0.,1.34087697701688E-16,-1.));
#122886=DIRECTION('ref_axis',(0.,1.,1.34087697701688E-16));
#122887=DIRECTION('center_axis',(0.,1.22914743790472E-16,-1.));
#122888=DIRECTION('ref_axis',(0.,1.,1.22914743790472E-16));
#122889=DIRECTION('',(-1.,-1.90750687963558E-16,0.));
#122890=DIRECTION('',(-1.,4.76876719908896E-16,0.));
#122891=DIRECTION('',(1.,-1.23706245878324E-16,0.));
#122892=DIRECTION('',(-1.,-1.23706245878324E-16,0.));
#122893=DIRECTION('',(1.,3.71118737634973E-16,0.));
#122894=DIRECTION('',(-1.,3.29883322342198E-16,0.));
#122895=DIRECTION('',(1.,3.29883322342202E-16,0.));
#122896=DIRECTION('',(1.,5.72252063890675E-16,0.));
#122897=DIRECTION('',(-1.,3.29883322342202E-16,0.));
#122898=DIRECTION('center_axis',(0.,1.35726946151947E-16,-1.));
#122899=DIRECTION('ref_axis',(0.,1.,1.35726946151947E-16));
#122900=DIRECTION('',(1.,-9.53753439817791E-17,0.));
#122901=DIRECTION('center_axis',(0.,1.35726946151947E-16,-1.));
#122902=DIRECTION('ref_axis',(0.,1.,1.35726946151947E-16));
#122903=DIRECTION('',(1.,-9.53753439817791E-17,0.));
#122904=DIRECTION('',(1.,5.72252063890675E-16,0.));
#122905=DIRECTION('',(-1.,3.29883322342202E-16,0.));
#122906=DIRECTION('',(-1.,4.76876719908896E-16,0.));
#122907=DIRECTION('',(1.,-1.23706245878324E-16,0.));
#122908=DIRECTION('center_axis',(0.,1.22914743790472E-16,-1.));
#122909=DIRECTION('ref_axis',(0.,1.,1.22914743790472E-16));
#122910=DIRECTION('',(-1.,-1.90750687963558E-16,0.));
#122911=DIRECTION('',(1.,-9.53753439817791E-17,0.));
#122912=DIRECTION('center_axis',(0.,1.35726946151947E-16,-1.));
#122913=DIRECTION('ref_axis',(0.,1.,1.35726946151947E-16));
#122914=DIRECTION('center_axis',(0.,0.,-1.));
#122915=DIRECTION('ref_axis',(0.,1.,0.));
#122916=DIRECTION('center_axis',(0.,0.,-1.));
#122917=DIRECTION('ref_axis',(0.,1.,0.));
#122918=DIRECTION('',(1.,-1.23706245878324E-16,0.));
#122919=DIRECTION('',(-1.,4.76876719908896E-16,0.));
#122920=DIRECTION('center_axis',(0.,0.,-1.));
#122921=DIRECTION('ref_axis',(0.,1.,0.));
#122922=DIRECTION('center_axis',(0.,0.,-1.));
#122923=DIRECTION('ref_axis',(0.,1.,0.));
#122924=DIRECTION('center_axis',(0.,1.22914743790472E-16,-1.));
#122925=DIRECTION('ref_axis',(0.,1.,1.22914743790472E-16));
#122926=DIRECTION('',(1.,3.71118737634973E-16,0.));
#122927=DIRECTION('',(-1.,-1.23706245878324E-16,0.));
#122928=DIRECTION('center_axis',(0.,1.22914743790472E-16,-1.));
#122929=DIRECTION('ref_axis',(0.,1.,1.22914743790472E-16));
#122930=DIRECTION('',(1.,3.71118737634973E-16,0.));
#122931=DIRECTION('',(-1.,3.71118737634973E-16,0.));
#122932=DIRECTION('center_axis',(0.,1.22914743790472E-16,-1.));
#122933=DIRECTION('ref_axis',(0.,1.,1.22914743790472E-16));
#122934=DIRECTION('',(1.,3.29883322342198E-16,0.));
#122935=DIRECTION('',(-1.,3.71118737634973E-16,0.));
#122936=DIRECTION('center_axis',(0.,1.22914743790472E-16,-1.));
#122937=DIRECTION('ref_axis',(0.,1.,1.22914743790472E-16));
#122938=DIRECTION('',(1.,3.29883322342202E-16,0.));
#122939=DIRECTION('',(-1.,3.29883322342198E-16,0.));
#122940=DIRECTION('center_axis',(0.,1.22914743790472E-16,-1.));
#122941=DIRECTION('ref_axis',(0.,1.,1.22914743790472E-16));
#122942=DIRECTION('',(1.,5.72252063890675E-16,0.));
#122943=DIRECTION('',(-1.,3.29883322342202E-16,0.));
#122944=DIRECTION('',(-1.,-1.90750687963558E-16,0.));
#122945=DIRECTION('center_axis',(0.,0.,-1.));
#122946=DIRECTION('ref_axis',(0.,1.,0.));
#122947=DIRECTION('',(-1.,3.29883322342198E-16,0.));
#122948=DIRECTION('',(1.,3.29883322342202E-16,0.));
#122949=DIRECTION('',(-1.,3.71118737634973E-16,0.));
#122950=DIRECTION('',(1.,3.29883322342198E-16,0.));
#122951=DIRECTION('',(-1.,3.71118737634973E-16,0.));
#122952=DIRECTION('',(1.,3.71118737634973E-16,0.));
#122953=DIRECTION('',(1.,5.72252063890675E-16,0.));
#122954=DIRECTION('',(-1.,3.29883322342202E-16,0.));
#122955=DIRECTION('center_axis',(0.,1.22914743790472E-16,-1.));
#122956=DIRECTION('ref_axis',(0.,1.,1.22914743790472E-16));
#122957=DIRECTION('center_axis',(0.,0.,-1.));
#122958=DIRECTION('ref_axis',(0.,1.,0.));
#122959=DIRECTION('center_axis',(0.,0.,-1.));
#122960=DIRECTION('ref_axis',(0.,1.,0.));
#122961=DIRECTION('',(-1.,-1.90750687963558E-16,0.));
#122962=DIRECTION('center_axis',(0.,0.,-1.));
#122963=DIRECTION('ref_axis',(0.,1.,0.));
#122964=DIRECTION('center_axis',(0.,0.,-1.));
#122965=DIRECTION('ref_axis',(0.,1.,0.));
#122966=DIRECTION('center_axis',(0.,1.22914743790472E-16,-1.));
#122967=DIRECTION('ref_axis',(0.,1.,1.22914743790472E-16));
#122968=DIRECTION('',(-1.,-1.23706245878324E-16,0.));
#122969=DIRECTION('',(1.,3.71118737634973E-16,0.));
#122970=DIRECTION('',(-1.,4.76876719908896E-16,0.));
#122971=DIRECTION('',(1.,-1.23706245878324E-16,0.));
#122972=DIRECTION('',(1.,-9.53753439817791E-17,0.));
#122973=DIRECTION('center_axis',(0.,0.,-1.));
#122974=DIRECTION('ref_axis',(0.,1.,0.));
#122975=DIRECTION('',(1.,3.71118737634973E-16,0.));
#122976=DIRECTION('',(-1.,3.71118737634973E-16,0.));
#122977=DIRECTION('',(1.,3.29883322342202E-16,0.));
#122978=DIRECTION('',(-1.,3.71118737634973E-16,0.));
#122979=DIRECTION('',(-1.,-1.23706245878324E-16,0.));
#122980=DIRECTION('',(1.,3.71118737634973E-16,0.));
#122981=DIRECTION('',(-1.,3.71118737634973E-16,0.));
#122982=DIRECTION('',(1.,3.29883322342198E-16,0.));
#122983=DIRECTION('center_axis',(0.,0.,-1.));
#122984=DIRECTION('ref_axis',(0.,1.,0.));
#122985=DIRECTION('',(0.,1.23467863058847E-16,-1.));
#122986=DIRECTION('',(0.,1.23467863058847E-16,-1.));
#122987=DIRECTION('center_axis',(0.,0.,-1.));
#122988=DIRECTION('ref_axis',(0.,1.,0.));
#122989=DIRECTION('center_axis',(0.,0.,-1.));
#122990=DIRECTION('ref_axis',(0.,1.,0.));
#122991=DIRECTION('center_axis',(-2.19322982990717E-31,-3.89595880873225E-46,
1.));
#122992=DIRECTION('ref_axis',(-1.77635683940025E-15,1.,1.55575381946529E-61));
#122993=DIRECTION('',(0.,1.23467863058847E-16,-1.));
#122994=DIRECTION('center_axis',(0.,0.,-1.));
#122995=DIRECTION('ref_axis',(0.,1.,0.));
#122996=DIRECTION('',(0.,1.23467863058847E-16,-1.));
#122997=DIRECTION('center_axis',(0.,0.,-1.));
#122998=DIRECTION('ref_axis',(0.,1.,0.));
#122999=DIRECTION('center_axis',(0.,1.22462808028055E-16,-1.));
#123000=DIRECTION('ref_axis',(0.,1.,1.22462808028055E-16));
#123001=DIRECTION('',(0.,1.23467863058847E-16,-1.));
#123002=DIRECTION('center_axis',(0.,1.22462808028055E-16,-1.));
#123003=DIRECTION('ref_axis',(0.,1.,1.22462808028055E-16));
#123004=DIRECTION('center_axis',(0.,0.,-1.));
#123005=DIRECTION('ref_axis',(0.,1.,0.));
#123006=DIRECTION('',(0.,1.23467863058847E-16,-1.));
#123007=DIRECTION('center_axis',(0.,0.,-1.));
#123008=DIRECTION('ref_axis',(0.,1.,0.));
#123009=DIRECTION('center_axis',(0.,0.,-1.));
#123010=DIRECTION('ref_axis',(0.,1.,0.));
#123011=DIRECTION('center_axis',(4.38645965981435E-31,-1.5583835234929E-45,
1.));
#123012=DIRECTION('ref_axis',(3.5527136788005E-15,1.,-9.33452291679171E-61));
#123013=DIRECTION('',(0.,1.23467863058847E-16,-1.));
#123014=DIRECTION('center_axis',(0.,0.,-1.));
#123015=DIRECTION('ref_axis',(0.,1.,0.));
#123016=DIRECTION('',(0.,1.23467863058847E-16,-1.));
#123017=DIRECTION('center_axis',(0.,0.,-1.));
#123018=DIRECTION('ref_axis',(0.,1.,0.));
#123019=DIRECTION('center_axis',(0.,1.22462808028055E-16,-1.));
#123020=DIRECTION('ref_axis',(1.22464679914735E-16,-1.,-1.22462808028055E-16));
#123021=DIRECTION('center_axis',(0.,1.22462808028055E-16,-1.));
#123022=DIRECTION('ref_axis',(0.,1.,1.22462808028055E-16));
#123023=DIRECTION('center_axis',(0.,-1.23467863058847E-16,1.));
#123024=DIRECTION('ref_axis',(0.,-1.,-1.23467863058847E-16));
#123025=DIRECTION('',(0.700366780446485,-0.713783141330072,-8.81292791474553E-17));
#123026=DIRECTION('',(-0.700366780446451,0.713783141330105,8.81292791474594E-17));
#123027=DIRECTION('center_axis',(0.,0.,-1.));
#123028=DIRECTION('ref_axis',(0.,-1.,0.));
#123029=DIRECTION('center_axis',(-0.713783141330072,-0.700366780446485,
-8.64727897391325E-17));
#123030=DIRECTION('ref_axis',(-0.700366780446485,0.713783141330072,-1.3612391051092E-33));
#123031=DIRECTION('',(-0.507302896983364,0.517020784572389,-0.689444181230387));
#123032=DIRECTION('',(-0.0133576962200374,0.0136135788205688,-0.999818104668739));
#123033=DIRECTION('center_axis',(0.,1.23467863058847E-16,-1.));
#123034=DIRECTION('ref_axis',(-1.,0.,0.));
#123035=DIRECTION('center_axis',(-7.1617481931302E-31,-4.1541690210802E-45,
1.));
#123036=DIRECTION('ref_axis',(-5.80049578546342E-15,1.,-2.48920611114446E-60));
#123037=DIRECTION('',(0.70592193778968,0.708289642552581,8.74510085926821E-17));
#123038=DIRECTION('center_axis',(0.708289642552581,-0.70592193778968,-8.71586731452524E-17));
#123039=DIRECTION('ref_axis',(9.155251692876E-34,1.23467863058847E-16,-1.));
#123040=DIRECTION('',(-0.0134621338381862,-0.0135072866467963,-0.999818145544461));
#123041=DIRECTION('center_axis',(0.966292363511968,0.257447214431338,3.17864574162902E-17));
#123042=DIRECTION('ref_axis',(-3.29101538697003E-33,1.23467863058847E-16,
-1.));
#123043=DIRECTION('',(0.257447214431338,-0.966292363511968,-1.19306053212906E-16));
#123044=DIRECTION('',(0.,1.23467863058847E-16,-1.));
#123045=DIRECTION('center_axis',(-0.260190353924911,-0.965557341499939,
-1.19215301615779E-16));
#123046=DIRECTION('ref_axis',(-0.965557341499939,0.260190353924911,3.58038858923534E-33));
#123047=DIRECTION('',(0.,1.23467863058847E-16,-1.));
#123048=DIRECTION('',(-0.965557341499939,0.260190353924911,3.21251469876339E-17));
#123049=DIRECTION('center_axis',(0.,0.,-1.));
#123050=DIRECTION('ref_axis',(0.,1.,0.));
#123051=DIRECTION('center_axis',(0.,0.,1.));
#123052=DIRECTION('ref_axis',(0.,-1.,0.));
#123053=DIRECTION('center_axis',(-4.93476711729114E-30,1.97232914692071E-43,
-1.));
#123054=DIRECTION('ref_axis',(-3.99680288865056E-14,-1.,0.));
#123055=DIRECTION('center_axis',(0.966876318092686,-0.255245343760725,-3.15145971498576E-17));
#123056=DIRECTION('ref_axis',(-1.08811059507331E-34,1.23467863058847E-16,
-1.));
#123057=DIRECTION('',(0.,1.23467863058847E-16,-1.));
#123058=DIRECTION('',(-0.255245343760725,-0.966876318092686,-1.1937815283711E-16));
#123059=DIRECTION('center_axis',(-0.262389207151869,0.964962125666191,1.19141811588728E-16));
#123060=DIRECTION('ref_axis',(4.54065214350716E-16,4.72048517437092E-33,
1.));
#123061=DIRECTION('',(0.964962125666191,0.262389207151869,3.23966346967465E-17));
#123062=DIRECTION('',(0.,1.23467863058847E-16,-1.));
#123063=DIRECTION('center_axis',(0.,0.,-1.));
#123064=DIRECTION('ref_axis',(0.,1.,0.));
#123065=DIRECTION('center_axis',(0.,0.,1.));
#123066=DIRECTION('ref_axis',(0.,-1.,0.));
#123067=DIRECTION('center_axis',(0.,0.,-1.));
#123068=DIRECTION('ref_axis',(0.,1.,0.));
#123069=DIRECTION('center_axis',(0.,0.,-1.));
#123070=DIRECTION('ref_axis',(0.,1.,0.));
#123071=DIRECTION('center_axis',(0.,0.,-1.));
#123072=DIRECTION('ref_axis',(0.,1.,0.));
#123073=DIRECTION('',(0.,1.23467863058847E-16,-1.));
#123074=DIRECTION('center_axis',(0.,0.,-1.));
#123075=DIRECTION('ref_axis',(0.,1.,0.));
#123076=DIRECTION('',(0.,1.23467863058847E-16,-1.));
#123077=DIRECTION('center_axis',(0.,1.21568833848598E-16,-1.));
#123078=DIRECTION('ref_axis',(1.01064309961486E-15,-1.,-1.21568833848598E-16));
#123079=DIRECTION('center_axis',(0.,1.21568833848598E-16,-1.));
#123080=DIRECTION('ref_axis',(0.,1.,1.21568833848598E-16));
#123081=DIRECTION('center_axis',(0.,1.21568833848598E-16,-1.));
#123082=DIRECTION('ref_axis',(0.,1.,1.21568833848598E-16));
#123083=DIRECTION('center_axis',(0.,1.30925187718918E-16,-1.));
#123084=DIRECTION('ref_axis',(0.,1.,1.30925187718918E-16));
#123085=DIRECTION('center_axis',(0.,1.30925187718918E-16,-1.));
#123086=DIRECTION('ref_axis',(0.,1.,1.30925187718918E-16));
#123087=DIRECTION('',(0.,1.23467863058847E-16,-1.));
#123088=DIRECTION('center_axis',(0.,1.30925187718918E-16,-1.));
#123089=DIRECTION('ref_axis',(0.,1.,1.30925187718918E-16));
#123090=DIRECTION('center_axis',(0.,1.30925187718918E-16,-1.));
#123091=DIRECTION('ref_axis',(0.,1.,1.30925187718918E-16));
#123092=DIRECTION('center_axis',(0.,1.30925187718918E-16,-1.));
#123093=DIRECTION('ref_axis',(0.,1.,1.30925187718918E-16));
#123094=DIRECTION('center_axis',(0.,0.,-1.));
#123095=DIRECTION('ref_axis',(0.,1.,0.));
#123096=DIRECTION('center_axis',(0.,0.,-1.));
#123097=DIRECTION('ref_axis',(0.,1.,0.));
#123098=DIRECTION('center_axis',(0.,0.,-1.));
#123099=DIRECTION('ref_axis',(0.,1.,0.));
#123100=DIRECTION('',(0.,1.23467863058847E-16,-1.));
#123101=DIRECTION('center_axis',(0.,0.,-1.));
#123102=DIRECTION('ref_axis',(0.,1.,0.));
#123103=DIRECTION('center_axis',(0.,0.,-1.));
#123104=DIRECTION('ref_axis',(0.,1.,0.));
#123105=DIRECTION('center_axis',(0.,0.,-1.));
#123106=DIRECTION('ref_axis',(0.,1.,0.));
#123107=DIRECTION('',(0.,1.23467863058847E-16,-1.));
#123108=DIRECTION('center_axis',(0.,0.,-1.));
#123109=DIRECTION('ref_axis',(0.,1.,0.));
#123110=DIRECTION('center_axis',(0.,0.,-1.));
#123111=DIRECTION('ref_axis',(0.,1.,0.));
#123112=DIRECTION('center_axis',(0.,0.,-1.));
#123113=DIRECTION('ref_axis',(0.,1.,0.));
#123114=DIRECTION('',(0.,1.23467863058847E-16,-1.));
#123115=DIRECTION('center_axis',(0.,1.21568833848598E-16,-1.));
#123116=DIRECTION('ref_axis',(0.,1.,1.21568833848598E-16));
#123117=DIRECTION('center_axis',(0.,1.21568833848598E-16,-1.));
#123118=DIRECTION('ref_axis',(0.,1.,1.21568833848598E-16));
#123119=DIRECTION('center_axis',(0.,1.21568833848598E-16,-1.));
#123120=DIRECTION('ref_axis',(0.,1.,1.21568833848598E-16));
#123121=DIRECTION('center_axis',(0.,0.,-1.));
#123122=DIRECTION('ref_axis',(0.,1.,0.));
#123123=DIRECTION('center_axis',(0.,0.,-1.));
#123124=DIRECTION('ref_axis',(0.,1.,0.));
#123125=DIRECTION('',(0.,1.23467863058847E-16,-1.));
#123126=DIRECTION('center_axis',(0.,0.,-1.));
#123127=DIRECTION('ref_axis',(0.,1.,0.));
#123128=DIRECTION('',(0.,1.23467863058847E-16,-1.));
#123129=DIRECTION('center_axis',(0.,0.,-1.));
#123130=DIRECTION('ref_axis',(0.,1.,0.));
#123131=DIRECTION('center_axis',(0.,0.,-1.));
#123132=DIRECTION('ref_axis',(0.,1.,0.));
#123133=DIRECTION('center_axis',(0.,0.,-1.));
#123134=DIRECTION('ref_axis',(0.,1.,0.));
#123135=DIRECTION('center_axis',(0.,0.,1.));
#123136=DIRECTION('ref_axis',(0.,1.,0.));
#123137=DIRECTION('center_axis',(9.45862666529894E-32,7.24606518465966E-47,
-1.));
#123138=DIRECTION('ref_axis',(7.66080049574581E-16,-1.,2.91703841149741E-62));
#123139=DIRECTION('',(0.0110444763156131,-0.0135131799871829,0.999847695156391));
#123140=DIRECTION('',(0.000686915141868458,-0.0174388829355556,0.999847695156391));
#123141=DIRECTION('center_axis',(0.,0.,1.));
#123142=DIRECTION('ref_axis',(0.,1.,0.));
#123143=DIRECTION('center_axis',(4.38645965981435E-31,1.5583835234929E-45,
-1.));
#123144=DIRECTION('ref_axis',(3.5527136788005E-15,-1.,1.24460305557223E-60));
#123145=DIRECTION('',(0.013481760241072,-0.011082807913809,0.999847695156391));
#123146=DIRECTION('center_axis',(0.,0.,1.));
#123147=DIRECTION('ref_axis',(0.,1.,0.));
#123148=DIRECTION('center_axis',(1.89172533305981E-31,2.89842607386392E-46,
-1.));
#123149=DIRECTION('ref_axis',(1.53216009914918E-15,-1.,7.38983064246011E-61));
#123150=DIRECTION('',(0.0174387888650499,-0.000689299189283617,0.999847695156391));
#123151=DIRECTION('center_axis',(-0.49830877570858,0.40695051295028,0.765558387101415));
#123152=DIRECTION('ref_axis',(0.616776838376874,-0.454175066156573,0.642892946705359));
#123153=DIRECTION('center_axis',(0.,0.,1.));
#123154=DIRECTION('ref_axis',(0.,1.,0.));
#123155=DIRECTION('center_axis',(-6.62103866570927E-31,3.55057194048325E-45,
-1.));
#123156=DIRECTION('ref_axis',(-5.36256034702207E-15,-1.,-1.86690458335834E-60));
#123157=DIRECTION('',(0.0134817602410721,0.0110828079138087,0.999847695156391));
#123158=DIRECTION('center_axis',(0.524694312992163,0.428071664074771,-0.735833220458236));
#123159=DIRECTION('ref_axis',(0.586317116694794,0.444960261363177,0.67693618936966));
#123160=DIRECTION('',(0.0174387888650499,0.000689299189283565,0.999847695156391));
#123161=DIRECTION('center_axis',(0.,0.,1.));
#123162=DIRECTION('ref_axis',(0.,1.,0.));
#123163=DIRECTION('center_axis',(1.09661491495359E-30,9.73989702183064E-45,
-1.));
#123164=DIRECTION('ref_axis',(8.88178419700126E-15,-1.,3.73380916671668E-60));
#123165=DIRECTION('',(0.0109827961190146,0.0135633579861438,0.999847695156391));
#123166=DIRECTION('center_axis',(0.,0.,1.));
#123167=DIRECTION('ref_axis',(0.,1.,0.));
#123168=DIRECTION('center_axis',(0.,0.,-1.));
#123169=DIRECTION('ref_axis',(0.,-1.,0.));
#123170=DIRECTION('',(0.003269361032546,0.0171434468206077,0.999847695156391));
#123171=DIRECTION('center_axis',(-0.424375096187792,-0.528257078927607,
0.735425207820941));
#123172=DIRECTION('ref_axis',(0.426055759035728,0.600170551540012,0.676957752933407));
#123173=DIRECTION('center_axis',(0.,-1.30362731016209E-16,1.));
#123174=DIRECTION('ref_axis',(-1.22464679914735E-16,-1.,-1.30362731016209E-16));
#123175=DIRECTION('center_axis',(0.,1.30357480714758E-16,-1.));
#123176=DIRECTION('ref_axis',(0.,-1.,-1.30357480714758E-16));
#123177=DIRECTION('center_axis',(0.,-1.23467863058847E-16,1.));
#123178=DIRECTION('ref_axis',(0.,-1.,-1.23467863058847E-16));
#123179=DIRECTION('center_axis',(2.75730074378449E-32,1.19587307245642E-16,
-1.));
#123180=DIRECTION('ref_axis',(7.105427357601E-15,-1.,-1.19587307245642E-16));
#123181=DIRECTION('center_axis',(0.,1.30052077910778E-16,-1.));
#123182=DIRECTION('ref_axis',(0.,-1.,-1.30052077910778E-16));
#123183=DIRECTION('center_axis',(9.63646068259673E-31,7.52109676045604E-45,
-1.));
#123184=DIRECTION('ref_axis',(7.80483313135807E-15,-1.,-3.73380916671668E-60));
#123185=DIRECTION('center_axis',(7.6763044046751E-31,4.77254954069701E-45,
-1.));
#123186=DIRECTION('ref_axis',(6.21724893790088E-15,-1.,1.86690458335834E-60));
#123187=DIRECTION('center_axis',(2.22379861906079E-31,4.00531780142632E-46,
-1.));
#123188=DIRECTION('ref_axis',(1.80111533800572E-15,-1.,8.55664600705907E-61));
#123189=DIRECTION('center_axis',(2.57572279529701E-31,1.30052077910778E-16,
-1.));
#123190=DIRECTION('ref_axis',(-3.91196650355621E-14,-1.,-1.30052077910778E-16));
#123191=DIRECTION('center_axis',(-2.96506482541439E-31,7.12056498031345E-46,
-1.));
#123192=DIRECTION('ref_axis',(-2.40148711734095E-15,-1.,1.0890276736257E-60));
#123193=DIRECTION('center_axis',(0.,0.,-1.));
#123194=DIRECTION('ref_axis',(0.,-1.,0.));
#123195=DIRECTION('center_axis',(0.,0.,-1.));
#123196=DIRECTION('ref_axis',(0.,-1.,0.));
#123197=DIRECTION('center_axis',(1.83206263248512E-32,1.20889464124791E-16,
-1.));
#123198=DIRECTION('ref_axis',(7.105427357601E-15,-1.,-1.20889464124791E-16));
#123199=DIRECTION('center_axis',(0.,1.30357480714758E-16,-1.));
#123200=DIRECTION('ref_axis',(0.,-1.,-1.30357480714758E-16));
#123201=DIRECTION('center_axis',(0.,-1.30002649721837E-16,1.));
#123202=DIRECTION('ref_axis',(0.,1.,1.30002649721837E-16));
#123203=DIRECTION('center_axis',(0.,1.30002742469137E-16,-1.));
#123204=DIRECTION('ref_axis',(0.,-1.,-1.30002742469137E-16));
#123205=DIRECTION('',(0.0174387888650499,0.000689299189283565,0.999847695156391));
#123206=DIRECTION('',(0.0174387888650499,-0.000689299189283839,0.999847695156391));
#123207=DIRECTION('center_axis',(0.,0.,1.));
#123208=DIRECTION('ref_axis',(0.,1.,0.));
#123209=DIRECTION('center_axis',(2.14851878863042E-31,3.73873238811768E-46,
-1.));
#123210=DIRECTION('ref_axis',(1.74014414391086E-15,-1.,-5.4451383681285E-61));
#123211=DIRECTION('',(0.013481760241072,0.0110828079138088,0.999847695156391));
#123212=DIRECTION('center_axis',(0.,0.,1.));
#123213=DIRECTION('ref_axis',(0.,1.,0.));
#123214=DIRECTION('center_axis',(0.,0.,-1.));
#123215=DIRECTION('ref_axis',(0.,-1.,0.));
#123216=DIRECTION('',(0.0109827961190146,0.0135633579861438,0.999847695156391));
#123217=DIRECTION('center_axis',(0.,0.,1.));
#123218=DIRECTION('ref_axis',(0.,1.,0.));
#123219=DIRECTION('center_axis',(-3.58086464771735E-31,1.03853677447713E-45,
-1.));
#123220=DIRECTION('ref_axis',(-2.90024023985143E-15,-1.,1.55575381946529E-61));
#123221=DIRECTION('',(0.0032693610325459,0.0171434468206077,0.999847695156391));
#123222=DIRECTION('center_axis',(0.,-1.19378624347407E-16,1.));
#123223=DIRECTION('ref_axis',(0.,1.,1.19378624347407E-16));
#123224=DIRECTION('center_axis',(2.90530101061278E-32,1.19379015387349E-16,
-1.));
#123225=DIRECTION('ref_axis',(7.105427357601E-15,-1.,-1.19379015387349E-16));
#123226=DIRECTION('center_axis',(0.,-1.30002649721837E-16,1.));
#123227=DIRECTION('ref_axis',(-1.22464679914735E-16,-1.,-1.30002649721837E-16));
#123228=DIRECTION('center_axis',(0.,1.30002742469137E-16,-1.));
#123229=DIRECTION('ref_axis',(0.,-1.,-1.30002742469137E-16));
#123230=DIRECTION('',(0.000686915141868465,-0.0174388829355556,0.999847695156391));
#123231=DIRECTION('center_axis',(0.,0.,1.));
#123232=DIRECTION('ref_axis',(0.,1.,0.));
#123233=DIRECTION('center_axis',(-2.14851878863041E-31,3.73873238811767E-46,
-1.));
#123234=DIRECTION('ref_axis',(-1.74014414391086E-15,-1.,-6.22301527786114E-61));
#123235=DIRECTION('',(0.0110444763156131,-0.0135131799871829,0.999847695156391));
#123236=DIRECTION('center_axis',(0.,0.,1.));
#123237=DIRECTION('ref_axis',(0.,1.,0.));
#123238=DIRECTION('center_axis',(1.09661491495359E-30,9.73989702183063E-45,
-1.));
#123239=DIRECTION('ref_axis',(8.88178419700125E-15,-1.,2.48920611114446E-60));
#123240=DIRECTION('',(0.013481760241072,-0.011082807913809,0.999847695156391));
#123241=DIRECTION('center_axis',(0.,0.,1.));
#123242=DIRECTION('ref_axis',(0.,-1.,0.));
#123243=DIRECTION('center_axis',(-2.14851878863042E-31,3.73873238811769E-46,
-1.));
#123244=DIRECTION('ref_axis',(-1.74014414391087E-15,-1.,2.33363072919793E-61));
#123245=DIRECTION('center_axis',(0.,-1.30362731016209E-16,1.));
#123246=DIRECTION('ref_axis',(0.,1.,1.30362731016209E-16));
#123247=DIRECTION('center_axis',(9.64691113863996E-8,8.44900850580662E-7,
-0.999999999999639));
#123248=DIRECTION('ref_axis',(0.131285471389481,0.991344604565596,8.5025289246305E-7));
#123249=DIRECTION('center_axis',(0.,-1.20912044068284E-16,1.));
#123250=DIRECTION('ref_axis',(0.,1.,1.20912044068284E-16));
#123251=DIRECTION('center_axis',(0.,1.23467863058847E-16,-1.));
#123252=DIRECTION('ref_axis',(-1.,0.,0.));
#123253=DIRECTION('center_axis',(0.,1.21568833848598E-16,-1.));
#123254=DIRECTION('ref_axis',(0.,1.,1.21568833848598E-16));
#123255=DIRECTION('center_axis',(0.,1.21568833848598E-16,-1.));
#123256=DIRECTION('ref_axis',(0.,1.,1.21568833848598E-16));
#123257=DIRECTION('center_axis',(2.34984018715753E-7,-7.16719780920963E-6,
-0.999999999974288));
#123258=DIRECTION('ref_axis',(0.0297033272169244,-0.999558758803514,7.17101515365848E-6));
#123259=DIRECTION('center_axis',(0.,1.23467863058847E-16,-1.));
#123260=DIRECTION('ref_axis',(-1.,0.,0.));
#123261=DIRECTION('center_axis',(0.,0.,-1.));
#123262=DIRECTION('ref_axis',(0.,1.,0.));
#123263=DIRECTION('center_axis',(0.,-1.23467863058847E-16,1.));
#123264=DIRECTION('ref_axis',(0.,-1.,-1.23467863058847E-16));
#123265=DIRECTION('center_axis',(0.,0.,-1.));
#123266=DIRECTION('ref_axis',(0.,1.,0.));
#123267=DIRECTION('center_axis',(0.,1.23467863058847E-16,-1.));
#123268=DIRECTION('ref_axis',(-1.,0.,0.));
#123269=DIRECTION('center_axis',(0.,1.23467863058847E-16,-1.));
#123270=DIRECTION('ref_axis',(-1.,0.,0.));
#123271=DIRECTION('center_axis',(0.,1.23467863058847E-16,-1.));
#123272=DIRECTION('ref_axis',(-1.,0.,0.));
#123273=DIRECTION('center_axis',(0.,1.23467863058847E-16,-1.));
#123274=DIRECTION('ref_axis',(-1.,0.,0.));
#123275=DIRECTION('center_axis',(0.,1.21568833848598E-16,-1.));
#123276=DIRECTION('ref_axis',(0.,1.,1.21568833848598E-16));
#123277=DIRECTION('center_axis',(0.,1.23467863058847E-16,-1.));
#123278=DIRECTION('ref_axis',(-1.,0.,0.));
#123279=DIRECTION('center_axis',(0.,1.21568833848598E-16,-1.));
#123280=DIRECTION('ref_axis',(0.,1.,1.21568833848598E-16));
#123281=DIRECTION('center_axis',(0.,1.23467863058847E-16,-1.));
#123282=DIRECTION('ref_axis',(-1.,0.,0.));
#123283=DIRECTION('center_axis',(0.,1.21568833848598E-16,-1.));
#123284=DIRECTION('ref_axis',(0.,1.,1.21568833848598E-16));
#123285=DIRECTION('center_axis',(0.,1.23467863058847E-16,-1.));
#123286=DIRECTION('ref_axis',(-1.,0.,0.));
#123287=DIRECTION('center_axis',(0.,1.23467863058847E-16,-1.));
#123288=DIRECTION('ref_axis',(-1.,0.,0.));
#123289=DIRECTION('center_axis',(0.,1.21568833848598E-16,-1.));
#123290=DIRECTION('ref_axis',(0.,1.,1.21568833848598E-16));
#123291=DIRECTION('center_axis',(0.,1.23467863058847E-16,-1.));
#123292=DIRECTION('ref_axis',(-1.,0.,0.));
#123293=DIRECTION('',(-0.7059219377897,-0.708289642552561,-8.74510085926797E-17));
#123294=DIRECTION('center_axis',(7.1617481931302E-31,-4.1541690210802E-45,
1.));
#123295=DIRECTION('ref_axis',(5.80049578546342E-15,1.,-2.48920611114446E-60));
#123296=DIRECTION('center_axis',(0.,1.21568833848598E-16,-1.));
#123297=DIRECTION('ref_axis',(0.,1.,1.21568833848598E-16));
#123298=DIRECTION('center_axis',(0.,1.21568833848598E-16,-1.));
#123299=DIRECTION('ref_axis',(0.,1.,1.21568833848598E-16));
#123300=DIRECTION('center_axis',(0.,1.21568833848598E-16,-1.));
#123301=DIRECTION('ref_axis',(0.,1.,1.21568833848598E-16));
#123302=DIRECTION('center_axis',(0.,1.21568833848598E-16,-1.));
#123303=DIRECTION('ref_axis',(0.,1.,1.21568833848598E-16));
#123304=DIRECTION('center_axis',(0.,1.21568833848598E-16,-1.));
#123305=DIRECTION('ref_axis',(0.,1.,1.21568833848598E-16));
#123306=DIRECTION('center_axis',(0.,1.21568833848598E-16,-1.));
#123307=DIRECTION('ref_axis',(0.,1.,1.21568833848598E-16));
#123308=DIRECTION('center_axis',(0.,1.21568833848598E-16,-1.));
#123309=DIRECTION('ref_axis',(0.,1.,1.21568833848598E-16));
#123310=DIRECTION('center_axis',(0.,1.21568833848598E-16,-1.));
#123311=DIRECTION('ref_axis',(0.,1.,1.21568833848598E-16));
#123312=DIRECTION('center_axis',(0.,1.21568833848598E-16,-1.));
#123313=DIRECTION('ref_axis',(0.,1.,1.21568833848598E-16));
#123314=DIRECTION('center_axis',(0.,1.21568833848598E-16,-1.));
#123315=DIRECTION('ref_axis',(0.,1.,1.21568833848598E-16));
#123316=DIRECTION('center_axis',(0.713783141330105,0.700366780446451,8.64727897391283E-17));
#123317=DIRECTION('ref_axis',(-6.33941656186775E-33,1.23467863058847E-16,
-1.));
#123318=DIRECTION('',(0.0133579710326364,-0.0136138588975274,0.999818097183587));
#123319=DIRECTION('center_axis',(0.,0.,-1.));
#123320=DIRECTION('ref_axis',(-0.705510697508481,-0.708699270284015,0.));
#123321=DIRECTION('',(0.0134623247494151,0.0135074781986352,0.999818140386068));
#123322=DIRECTION('center_axis',(-0.708289642552561,0.7059219377897,8.71586731452547E-17));
#123323=DIRECTION('ref_axis',(1.23055128733987E-16,2.43647158576037E-33,
1.));
#123324=DIRECTION('center_axis',(0.,0.,-1.));
#123325=DIRECTION('ref_axis',(0.,1.,0.));
#123326=DIRECTION('center_axis',(0.,0.,-1.));
#123327=DIRECTION('ref_axis',(0.,1.,0.));
#123328=DIRECTION('',(0.,1.23467863058847E-16,-1.));
#123329=DIRECTION('',(0.,1.23467863058847E-16,-1.));
#123330=DIRECTION('center_axis',(0.,0.,-1.));
#123331=DIRECTION('ref_axis',(0.,1.,0.));
#123332=DIRECTION('',(0.,1.23467863058847E-16,-1.));
#123333=DIRECTION('center_axis',(0.,0.,-1.));
#123334=DIRECTION('ref_axis',(0.,1.,0.));
#123335=DIRECTION('',(0.,1.23467863058847E-16,-1.));
#123336=DIRECTION('center_axis',(0.,1.22914743790472E-16,-1.));
#123337=DIRECTION('ref_axis',(0.,1.,1.22914743790472E-16));
#123338=DIRECTION('center_axis',(0.,0.,-1.));
#123339=DIRECTION('ref_axis',(0.,1.,0.));
#123340=DIRECTION('',(0.,1.23467863058847E-16,-1.));
#123341=DIRECTION('',(0.,1.23467863058847E-16,-1.));
#123342=DIRECTION('center_axis',(0.,0.,-1.));
#123343=DIRECTION('ref_axis',(0.,1.,0.));
#123344=DIRECTION('center_axis',(0.,0.,-1.));
#123345=DIRECTION('ref_axis',(0.,1.,0.));
#123346=DIRECTION('',(0.,1.23467863058847E-16,-1.));
#123347=DIRECTION('',(0.,1.23467863058847E-16,-1.));
#123348=DIRECTION('center_axis',(0.,1.23467863058847E-16,-1.));
#123349=DIRECTION('ref_axis',(-1.,0.,0.));
#123350=DIRECTION('center_axis',(0.,0.,-1.));
#123351=DIRECTION('ref_axis',(0.,1.,0.));
#123352=DIRECTION('center_axis',(0.,0.,-1.));
#123353=DIRECTION('ref_axis',(0.,1.,0.));
#123354=DIRECTION('',(-2.13730336808358E-18,-0.0174524064372818,-0.999847695156391));
#123355=DIRECTION('center_axis',(0.,1.23467863058847E-16,-1.));
#123356=DIRECTION('ref_axis',(-1.,0.,0.));
#123357=DIRECTION('center_axis',(0.,0.,-1.));
#123358=DIRECTION('ref_axis',(0.,1.,0.));
#123359=DIRECTION('center_axis',(0.,0.,-1.));
#123360=DIRECTION('ref_axis',(0.,1.,0.));
#123361=DIRECTION('',(-2.13730336808358E-18,-0.0174524064372818,-0.999847695156391));
#123362=DIRECTION('center_axis',(0.,-1.23467863058847E-16,1.));
#123363=DIRECTION('ref_axis',(0.,-1.,-1.23467863058847E-16));
#123364=DIRECTION('center_axis',(-0.713783141330072,-0.700366780446485,
-8.64727897391325E-17));
#123365=DIRECTION('ref_axis',(-0.700366780446485,0.713783141330072,-1.3612391051092E-33));
#123366=DIRECTION('center_axis',(0.713783141330105,0.700366780446451,8.64727897391283E-17));
#123367=DIRECTION('ref_axis',(-6.33941656186775E-33,1.23467863058847E-16,
-1.));
#123368=DIRECTION('center_axis',(0.,0.,1.));
#123369=DIRECTION('ref_axis',(0.,-1.,0.));
#123370=DIRECTION('center_axis',(0.,1.23467863058847E-16,-1.));
#123371=DIRECTION('ref_axis',(-1.,0.,0.));
#123372=DIRECTION('center_axis',(0.708289642552581,-0.70592193778968,-8.71586731452524E-17));
#123373=DIRECTION('ref_axis',(9.155251692876E-34,1.23467863058847E-16,-1.));
#123374=DIRECTION('center_axis',(-0.708289642552561,0.7059219377897,8.71586731452547E-17));
#123375=DIRECTION('ref_axis',(1.23055128733987E-16,2.43647158576037E-33,
1.));
#123376=DIRECTION('center_axis',(0.,0.,1.));
#123377=DIRECTION('ref_axis',(0.,-1.,0.));
#123378=DIRECTION('center_axis',(0.966292363511968,0.257447214431338,3.17864574162902E-17));
#123379=DIRECTION('ref_axis',(-3.29101538697003E-33,1.23467863058847E-16,
-1.));
#123380=DIRECTION('center_axis',(-0.260190353924911,-0.965557341499939,
-1.19215301615779E-16));
#123381=DIRECTION('ref_axis',(-0.965557341499939,0.260190353924911,3.58038858923534E-33));
#123382=DIRECTION('center_axis',(0.,0.,-1.));
#123383=DIRECTION('ref_axis',(0.,1.,0.));
#123384=DIRECTION('center_axis',(0.966876318092686,-0.255245343760725,-3.15145971498576E-17));
#123385=DIRECTION('ref_axis',(-1.08811059507331E-34,1.23467863058847E-16,
-1.));
#123386=DIRECTION('center_axis',(-0.262389207151869,0.964962125666191,1.19141811588728E-16));
#123387=DIRECTION('ref_axis',(4.54065214350716E-16,4.72048517437092E-33,
1.));
#123388=DIRECTION('center_axis',(0.,0.,-1.));
#123389=DIRECTION('ref_axis',(0.,1.,0.));
#123390=DIRECTION('center_axis',(0.,1.23467863058847E-16,-1.));
#123391=DIRECTION('ref_axis',(-1.,0.,0.));
#123392=DIRECTION('center_axis',(0.,0.,-1.));
#123393=DIRECTION('ref_axis',(0.,1.,0.));
#123394=DIRECTION('',(0.,1.23467863058847E-16,-1.));
#123395=DIRECTION('',(0.,1.23467863058847E-16,-1.));
#123396=DIRECTION('center_axis',(0.,0.,-1.));
#123397=DIRECTION('ref_axis',(0.,1.,0.));
#123398=DIRECTION('center_axis',(0.,0.,-1.));
#123399=DIRECTION('ref_axis',(0.,1.,0.));
#123400=DIRECTION('',(0.,1.23467863058847E-16,-1.));
#123401=DIRECTION('center_axis',(0.,0.,-1.));
#123402=DIRECTION('ref_axis',(0.,1.,0.));
#123403=DIRECTION('center_axis',(0.,1.22229112323298E-16,-1.));
#123404=DIRECTION('ref_axis',(0.,1.,1.22229112323298E-16));
#123405=DIRECTION('',(0.,1.23467863058847E-16,-1.));
#123406=DIRECTION('center_axis',(0.,1.22229112323298E-16,-1.));
#123407=DIRECTION('ref_axis',(0.,1.,1.22229112323298E-16));
#123408=DIRECTION('center_axis',(0.,0.,-1.));
#123409=DIRECTION('ref_axis',(0.,1.,0.));
#123410=DIRECTION('',(0.,1.23467863058847E-16,-1.));
#123411=DIRECTION('center_axis',(0.,0.,-1.));
#123412=DIRECTION('ref_axis',(0.,1.,0.));
#123413=DIRECTION('center_axis',(0.,0.,-1.));
#123414=DIRECTION('ref_axis',(0.,1.,0.));
#123415=DIRECTION('',(0.,1.23467863058847E-16,-1.));
#123416=DIRECTION('center_axis',(0.,0.,-1.));
#123417=DIRECTION('ref_axis',(0.,1.,0.));
#123418=DIRECTION('center_axis',(0.,0.,-1.));
#123419=DIRECTION('ref_axis',(0.,1.,0.));
#123420=DIRECTION('',(0.,1.23467863058847E-16,-1.));
#123421=DIRECTION('center_axis',(0.,0.,-1.));
#123422=DIRECTION('ref_axis',(0.,1.,0.));
#123423=DIRECTION('center_axis',(0.,1.22229112323298E-16,-1.));
#123424=DIRECTION('ref_axis',(1.22464679914735E-16,-1.,-1.22229112323298E-16));
#123425=DIRECTION('center_axis',(0.,1.22229112323298E-16,-1.));
#123426=DIRECTION('ref_axis',(0.,1.,1.22229112323298E-16));
#123427=DIRECTION('center_axis',(0.,1.33250839261027E-16,-1.));
#123428=DIRECTION('ref_axis',(0.,1.,1.33250839261027E-16));
#123429=DIRECTION('center_axis',(0.,1.33250839261027E-16,-1.));
#123430=DIRECTION('ref_axis',(0.,-1.,-1.33250839261027E-16));
#123431=DIRECTION('',(0.,1.23467863058847E-16,-1.));
#123432=DIRECTION('center_axis',(0.,0.,-1.));
#123433=DIRECTION('ref_axis',(0.,1.,0.));
#123434=DIRECTION('center_axis',(0.,0.,-1.));
#123435=DIRECTION('ref_axis',(0.,1.,0.));
#123436=DIRECTION('center_axis',(0.,1.23467863058847E-16,-1.));
#123437=DIRECTION('ref_axis',(-1.,0.,0.));
#123438=DIRECTION('center_axis',(0.,1.22014183466588E-16,-1.));
#123439=DIRECTION('ref_axis',(0.,1.,1.22014183466588E-16));
#123440=DIRECTION('center_axis',(0.,1.32487572930867E-16,-1.));
#123441=DIRECTION('ref_axis',(0.,-1.,-1.32487572930867E-16));
#123442=DIRECTION('center_axis',(0.,0.,-1.));
#123443=DIRECTION('ref_axis',(0.,1.,0.));
#123444=DIRECTION('center_axis',(0.,0.,-1.));
#123445=DIRECTION('ref_axis',(0.,1.,0.));
#123446=DIRECTION('center_axis',(0.,0.,-1.));
#123447=DIRECTION('ref_axis',(0.,1.,0.));
#123448=DIRECTION('center_axis',(0.,1.22014183466588E-16,-1.));
#123449=DIRECTION('ref_axis',(0.,1.,1.22014183466588E-16));
#123450=DIRECTION('center_axis',(0.,0.,-1.));
#123451=DIRECTION('ref_axis',(0.,1.,0.));
#123452=DIRECTION('center_axis',(0.,0.,-1.));
#123453=DIRECTION('ref_axis',(0.,1.,0.));
#123454=DIRECTION('center_axis',(0.,0.,-1.));
#123455=DIRECTION('ref_axis',(0.,1.,0.));
#123456=DIRECTION('center_axis',(0.,0.,-1.));
#123457=DIRECTION('ref_axis',(0.,1.,0.));
#123458=DIRECTION('',(0.,1.23467863058847E-16,-1.));
#123459=DIRECTION('',(0.,1.23467863058847E-16,-1.));
#123460=DIRECTION('center_axis',(0.,1.22014183466588E-16,-1.));
#123461=DIRECTION('ref_axis',(1.22464679914735E-16,-1.,-1.22014183466588E-16));
#123462=DIRECTION('center_axis',(0.,1.32487572930867E-16,-1.));
#123463=DIRECTION('ref_axis',(0.,1.,1.32487572930867E-16));
#123464=DIRECTION('',(0.,1.23467863058847E-16,-1.));
#123465=DIRECTION('center_axis',(0.,0.,-1.));
#123466=DIRECTION('ref_axis',(0.,1.,0.));
#123467=DIRECTION('',(0.,1.23467863058847E-16,-1.));
#123468=DIRECTION('center_axis',(0.,0.,-1.));
#123469=DIRECTION('ref_axis',(0.,1.,0.));
#123470=DIRECTION('',(0.,1.23467863058847E-16,-1.));
#123471=DIRECTION('center_axis',(0.,0.,-1.));
#123472=DIRECTION('ref_axis',(0.,1.,0.));
#123473=DIRECTION('',(0.,1.23467863058847E-16,-1.));
#123474=DIRECTION('center_axis',(0.,1.22014183466588E-16,-1.));
#123475=DIRECTION('ref_axis',(0.,1.,1.22014183466588E-16));
#123476=DIRECTION('',(0.,1.23467863058847E-16,-1.));
#123477=DIRECTION('center_axis',(0.,0.,-1.));
#123478=DIRECTION('ref_axis',(0.,1.,0.));
#123479=DIRECTION('',(0.,1.23467863058847E-16,-1.));
#123480=DIRECTION('center_axis',(0.,0.,-1.));
#123481=DIRECTION('ref_axis',(0.,1.,0.));
#123482=DIRECTION('',(0.459549353210719,-0.545727376107149,0.700711083779054));
#123483=DIRECTION('',(0.595667475496749,-0.42912133257888,0.678995685230073));
#123484=DIRECTION('',(0.580626046021037,0.392567954055243,0.713276801901518));
#123485=DIRECTION('',(-0.484796374610729,-0.46748816331627,-0.739207205270264));
#123486=DIRECTION('center_axis',(0.,0.,1.));
#123487=DIRECTION('ref_axis',(0.,1.,0.));
#123488=DIRECTION('',(0.0110444763156131,-0.0135131799871829,0.999847695156391));
#123489=DIRECTION('',(0.000686915141868466,-0.0174388829355556,0.999847695156391));
#123490=DIRECTION('center_axis',(0.,0.,1.));
#123491=DIRECTION('ref_axis',(0.,1.,0.));
#123492=DIRECTION('',(0.013481760241072,-0.011082807913809,0.999847695156391));
#123493=DIRECTION('center_axis',(0.,0.,1.));
#123494=DIRECTION('ref_axis',(0.,1.,0.));
#123495=DIRECTION('',(0.0174387888650499,-0.000689299189283616,0.999847695156391));
#123496=DIRECTION('center_axis',(0.,0.,1.));
#123497=DIRECTION('ref_axis',(0.,1.,0.));
#123498=DIRECTION('',(0.0134817602410721,0.0110828079138087,0.999847695156391));
#123499=DIRECTION('',(0.0174387888650499,0.000689299189283565,0.999847695156391));
#123500=DIRECTION('center_axis',(0.,0.,1.));
#123501=DIRECTION('ref_axis',(0.,1.,0.));
#123502=DIRECTION('',(0.0109827961190146,0.0135633579861438,0.999847695156391));
#123503=DIRECTION('center_axis',(0.,0.,1.));
#123504=DIRECTION('ref_axis',(0.,1.,0.));
#123505=DIRECTION('',(0.00326936103254579,0.0171434468206077,0.999847695156391));
#123506=DIRECTION('center_axis',(0.,-1.30057350048735E-16,1.));
#123507=DIRECTION('ref_axis',(1.22464679914735E-16,-1.,-1.30057350048735E-16));
#123508=DIRECTION('center_axis',(0.,-1.23467863058847E-16,1.));
#123509=DIRECTION('ref_axis',(0.,-1.,-1.23467863058847E-16));
#123510=DIRECTION('center_axis',(0.,1.18108832406932E-16,-1.));
#123511=DIRECTION('ref_axis',(0.,1.,1.18108832406932E-16));
#123512=DIRECTION('center_axis',(0.,1.29698951474901E-16,-1.));
#123513=DIRECTION('ref_axis',(0.,1.,1.29698951474901E-16));
#123514=DIRECTION('center_axis',(0.,0.,-1.));
#123515=DIRECTION('ref_axis',(0.,1.,0.));
#123516=DIRECTION('center_axis',(0.,0.,-1.));
#123517=DIRECTION('ref_axis',(0.,1.,0.));
#123518=DIRECTION('center_axis',(0.,0.,-1.));
#123519=DIRECTION('ref_axis',(0.,-1.,0.));
#123520=DIRECTION('center_axis',(0.,1.29698951474901E-16,-1.));
#123521=DIRECTION('ref_axis',(0.,1.,1.29698951474901E-16));
#123522=DIRECTION('center_axis',(0.,0.,-1.));
#123523=DIRECTION('ref_axis',(0.,1.,0.));
#123524=DIRECTION('center_axis',(0.,0.,-1.));
#123525=DIRECTION('ref_axis',(0.,1.,0.));
#123526=DIRECTION('center_axis',(0.,0.,-1.));
#123527=DIRECTION('ref_axis',(0.,1.,0.));
#123528=DIRECTION('center_axis',(0.,-1.23467863058847E-16,1.));
#123529=DIRECTION('ref_axis',(0.,-1.,-1.23467863058847E-16));
#123530=DIRECTION('center_axis',(0.,-1.29698951474901E-16,1.));
#123531=DIRECTION('ref_axis',(0.,1.,1.29698951474901E-16));
#123532=DIRECTION('',(0.0174387888650499,-0.000689299189283839,0.999847695156391));
#123533=DIRECTION('',(0.0174387888650499,0.000689299189283565,0.999847695156391));
#123534=DIRECTION('center_axis',(0.,0.,1.));
#123535=DIRECTION('ref_axis',(0.,1.,0.));
#123536=DIRECTION('',(0.0134817602410721,0.0110828079138088,0.999847695156391));
#123537=DIRECTION('center_axis',(0.,0.,1.));
#123538=DIRECTION('ref_axis',(0.,1.,0.));
#123539=DIRECTION('',(0.0109827961190146,0.0135633579861438,0.999847695156391));
#123540=DIRECTION('center_axis',(0.,0.,1.));
#123541=DIRECTION('ref_axis',(0.,1.,0.));
#123542=DIRECTION('',(0.0032693610325459,0.0171434468206077,0.999847695156391));
#123543=DIRECTION('center_axis',(0.,-1.18108832406932E-16,1.));
#123544=DIRECTION('ref_axis',(0.,1.,1.18108832406932E-16));
#123545=DIRECTION('center_axis',(0.,-1.29698951474901E-16,1.));
#123546=DIRECTION('ref_axis',(-1.22464679914735E-16,-1.,-1.29698951474901E-16));
#123547=DIRECTION('',(0.000686915141868473,-0.0174388829355556,0.999847695156391));
#123548=DIRECTION('center_axis',(0.,0.,1.));
#123549=DIRECTION('ref_axis',(0.,1.,0.));
#123550=DIRECTION('',(0.0110444763156131,-0.0135131799871829,0.999847695156391));
#123551=DIRECTION('center_axis',(0.,0.,1.));
#123552=DIRECTION('ref_axis',(0.,1.,0.));
#123553=DIRECTION('',(0.013481760241072,-0.011082807913809,0.999847695156391));
#123554=DIRECTION('center_axis',(0.,0.,1.));
#123555=DIRECTION('ref_axis',(0.,-1.,0.));
#123556=DIRECTION('center_axis',(0.,-1.30057350048735E-16,1.));
#123557=DIRECTION('ref_axis',(0.,1.,1.30057350048735E-16));
#123558=DIRECTION('center_axis',(0.,-1.1960959958765E-16,1.));
#123559=DIRECTION('ref_axis',(0.,1.,1.1960959958765E-16));
#123560=DIRECTION('center_axis',(0.,1.23467863058847E-16,-1.));
#123561=DIRECTION('ref_axis',(-1.,0.,0.));
#123562=DIRECTION('center_axis',(0.,1.23467863058847E-16,-1.));
#123563=DIRECTION('ref_axis',(-1.,0.,0.));
#123564=DIRECTION('center_axis',(0.,-1.23467863058847E-16,1.));
#123565=DIRECTION('ref_axis',(0.,-1.,-1.23467863058847E-16));
#123566=DIRECTION('center_axis',(0.,1.22914743790472E-16,-1.));
#123567=DIRECTION('ref_axis',(0.,1.,1.22914743790472E-16));
#123568=DIRECTION('center_axis',(0.,1.22914743790472E-16,-1.));
#123569=DIRECTION('ref_axis',(0.,1.,1.22914743790472E-16));
#123570=DIRECTION('center_axis',(0.,1.22914743790472E-16,-1.));
#123571=DIRECTION('ref_axis',(0.,1.,1.22914743790472E-16));
#123572=DIRECTION('center_axis',(0.,1.22914743790472E-16,-1.));
#123573=DIRECTION('ref_axis',(0.,1.,1.22914743790472E-16));
#123574=DIRECTION('center_axis',(0.,1.22914743790472E-16,-1.));
#123575=DIRECTION('ref_axis',(0.,1.,1.22914743790472E-16));
#123576=DIRECTION('center_axis',(-3.29883322342201E-16,1.,1.23467863058847E-16));
#123577=DIRECTION('ref_axis',(1.,3.29883322342202E-16,0.));
#123578=DIRECTION('center_axis',(-3.29883322342201E-16,-1.,-1.23467863058847E-16));
#123579=DIRECTION('ref_axis',(-1.,3.29883322342202E-16,0.));
#123580=DIRECTION('center_axis',(-3.71118737634973E-16,1.,1.23467863058847E-16));
#123581=DIRECTION('ref_axis',(1.,3.71118737634973E-16,0.));
#123582=DIRECTION('center_axis',(-3.71118737634973E-16,-1.,-1.23467863058847E-16));
#123583=DIRECTION('ref_axis',(-1.,3.71118737634973E-16,0.));
#123584=DIRECTION('center_axis',(-5.72252063890675E-16,1.,1.23467863058847E-16));
#123585=DIRECTION('ref_axis',(1.,5.72252063890675E-16,0.));
#123586=DIRECTION('center_axis',(1.90750687963558E-16,-1.,-1.23467863058847E-16));
#123587=DIRECTION('ref_axis',(-2.39311615755447E-50,1.23467863058847E-16,
-1.));
#123588=DIRECTION('center_axis',(1.23706245878324E-16,-1.,-1.23467863058847E-16));
#123589=DIRECTION('ref_axis',(9.34199996189111E-49,1.23467863058847E-16,
-1.));
#123590=DIRECTION('center_axis',(1.23706245878324E-16,1.,1.23467863058847E-16));
#123591=DIRECTION('ref_axis',(1.,-1.23706245878324E-16,0.));
#123592=DIRECTION('center_axis',(-4.76876719908896E-16,-1.,-1.23467863058847E-16));
#123593=DIRECTION('ref_axis',(-1.,4.76876719908896E-16,0.));
#123594=DIRECTION('center_axis',(9.53753439817791E-17,1.,1.23467863058847E-16));
#123595=DIRECTION('ref_axis',(-4.60419424770999E-49,1.23467863058847E-16,
-1.));
#123596=DIRECTION('center_axis',(0.,1.35726946151947E-16,-1.));
#123597=DIRECTION('ref_axis',(0.,1.,1.35726946151947E-16));
#123598=DIRECTION('center_axis',(0.,1.22914743790472E-16,-1.));
#123599=DIRECTION('ref_axis',(0.,1.,1.22914743790472E-16));
#123600=DIRECTION('center_axis',(0.,1.34087697701688E-16,-1.));
#123601=DIRECTION('ref_axis',(0.,1.,1.34087697701688E-16));
#123602=DIRECTION('center_axis',(0.,-1.34087697701688E-16,1.));
#123603=DIRECTION('ref_axis',(0.,1.,1.34087697701688E-16));
#123604=DIRECTION('center_axis',(0.,1.34087697701688E-16,-1.));
#123605=DIRECTION('ref_axis',(0.,1.,1.34087697701688E-16));
#123606=DIRECTION('center_axis',(1.86759697420978E-30,-1.34087697701688E-16,
1.));
#123607=DIRECTION('ref_axis',(-1.75859327100625E-13,1.,1.34087697701688E-16));
#123608=DIRECTION('center_axis',(0.,1.23467863058847E-16,-1.));
#123609=DIRECTION('ref_axis',(-1.,0.,0.));
#123610=DIRECTION('center_axis',(-3.29883322342201E-16,1.,1.23467863058847E-16));
#123611=DIRECTION('ref_axis',(1.,3.29883322342202E-16,0.));
#123612=DIRECTION('center_axis',(-3.29883322342201E-16,-1.,-1.23467863058847E-16));
#123613=DIRECTION('ref_axis',(-1.,3.29883322342202E-16,0.));
#123614=DIRECTION('center_axis',(-3.29883322342198E-16,1.,1.23467863058847E-16));
#123615=DIRECTION('ref_axis',(1.,3.29883322342198E-16,0.));
#123616=DIRECTION('center_axis',(-3.29883322342198E-16,-1.,-1.23467863058847E-16));
#123617=DIRECTION('ref_axis',(-1.,3.29883322342198E-16,0.));
#123618=DIRECTION('center_axis',(-3.71118737634973E-16,1.,1.23467863058847E-16));
#123619=DIRECTION('ref_axis',(1.,3.71118737634973E-16,0.));
#123620=DIRECTION('center_axis',(-3.71118737634973E-16,-1.,-1.23467863058847E-16));
#123621=DIRECTION('ref_axis',(-1.,3.71118737634973E-16,0.));
#123622=DIRECTION('center_axis',(-3.71118737634973E-16,1.,1.23467863058847E-16));
#123623=DIRECTION('ref_axis',(1.,3.71118737634973E-16,0.));
#123624=DIRECTION('center_axis',(-3.71118737634973E-16,-1.,-1.23467863058847E-16));
#123625=DIRECTION('ref_axis',(-1.,3.71118737634973E-16,0.));
#123626=DIRECTION('center_axis',(-5.72252063890675E-16,1.,1.23467863058847E-16));
#123627=DIRECTION('ref_axis',(1.,5.72252063890675E-16,0.));
#123628=DIRECTION('center_axis',(1.90750687963558E-16,-1.,-1.23467863058847E-16));
#123629=DIRECTION('ref_axis',(-2.39311615755447E-50,1.23467863058847E-16,
-1.));
#123630=DIRECTION('center_axis',(1.23706245878324E-16,-1.,-1.23467863058847E-16));
#123631=DIRECTION('ref_axis',(9.34199996189111E-49,1.23467863058847E-16,
-1.));
#123632=DIRECTION('center_axis',(1.23706245878324E-16,1.,1.23467863058847E-16));
#123633=DIRECTION('ref_axis',(1.,-1.23706245878324E-16,0.));
#123634=DIRECTION('center_axis',(-4.76876719908896E-16,-1.,-1.23467863058847E-16));
#123635=DIRECTION('ref_axis',(-1.,4.76876719908896E-16,0.));
#123636=DIRECTION('center_axis',(9.53753439817791E-17,1.,1.23467863058847E-16));
#123637=DIRECTION('ref_axis',(-4.60419424770999E-49,1.23467863058847E-16,
-1.));
#123638=DIRECTION('center_axis',(0.,1.35726946151947E-16,-1.));
#123639=DIRECTION('ref_axis',(0.,1.,1.35726946151947E-16));
#123640=DIRECTION('center_axis',(0.,1.35726946151947E-16,-1.));
#123641=DIRECTION('ref_axis',(0.,1.,1.35726946151947E-16));
#123642=DIRECTION('center_axis',(0.,1.22914743790472E-16,-1.));
#123643=DIRECTION('ref_axis',(0.,1.,1.22914743790472E-16));
#123644=DIRECTION('center_axis',(0.,1.22914743790472E-16,-1.));
#123645=DIRECTION('ref_axis',(0.,1.,1.22914743790472E-16));
#123646=DIRECTION('center_axis',(0.,0.,-1.));
#123647=DIRECTION('ref_axis',(0.,1.,0.));
#123648=DIRECTION('center_axis',(0.,0.,-1.));
#123649=DIRECTION('ref_axis',(0.,1.,0.));
#123650=DIRECTION('center_axis',(0.,0.,-1.));
#123651=DIRECTION('ref_axis',(0.,1.,0.));
#123652=DIRECTION('center_axis',(0.,0.,-1.));
#123653=DIRECTION('ref_axis',(0.,1.,0.));
#123654=DIRECTION('center_axis',(-3.29883322342201E-16,1.,1.23467863058847E-16));
#123655=DIRECTION('ref_axis',(1.,3.29883322342202E-16,0.));
#123656=DIRECTION('center_axis',(-3.29883322342201E-16,1.,1.23467863058847E-16));
#123657=DIRECTION('ref_axis',(1.,3.29883322342202E-16,0.));
#123658=DIRECTION('center_axis',(-3.29883322342201E-16,-1.,-1.23467863058847E-16));
#123659=DIRECTION('ref_axis',(-1.,3.29883322342202E-16,0.));
#123660=DIRECTION('center_axis',(-3.29883322342201E-16,-1.,-1.23467863058847E-16));
#123661=DIRECTION('ref_axis',(-1.,3.29883322342202E-16,0.));
#123662=DIRECTION('center_axis',(-3.29883322342198E-16,1.,1.23467863058847E-16));
#123663=DIRECTION('ref_axis',(1.,3.29883322342198E-16,0.));
#123664=DIRECTION('center_axis',(-3.29883322342198E-16,1.,1.23467863058847E-16));
#123665=DIRECTION('ref_axis',(1.,3.29883322342198E-16,0.));
#123666=DIRECTION('center_axis',(-3.29883322342198E-16,-1.,-1.23467863058847E-16));
#123667=DIRECTION('ref_axis',(-1.,3.29883322342198E-16,0.));
#123668=DIRECTION('center_axis',(-3.29883322342198E-16,-1.,-1.23467863058847E-16));
#123669=DIRECTION('ref_axis',(-1.,3.29883322342198E-16,0.));
#123670=DIRECTION('center_axis',(-3.71118737634973E-16,1.,1.23467863058847E-16));
#123671=DIRECTION('ref_axis',(1.,3.71118737634973E-16,0.));
#123672=DIRECTION('center_axis',(-3.71118737634973E-16,1.,1.23467863058847E-16));
#123673=DIRECTION('ref_axis',(1.,3.71118737634973E-16,0.));
#123674=DIRECTION('center_axis',(-3.71118737634973E-16,-1.,-1.23467863058847E-16));
#123675=DIRECTION('ref_axis',(-1.,3.71118737634973E-16,0.));
#123676=DIRECTION('center_axis',(-3.71118737634973E-16,-1.,-1.23467863058847E-16));
#123677=DIRECTION('ref_axis',(-1.,3.71118737634973E-16,0.));
#123678=DIRECTION('center_axis',(-3.71118737634973E-16,1.,1.23467863058847E-16));
#123679=DIRECTION('ref_axis',(1.,3.71118737634973E-16,0.));
#123680=DIRECTION('center_axis',(-3.71118737634973E-16,1.,1.23467863058847E-16));
#123681=DIRECTION('ref_axis',(1.,3.71118737634973E-16,0.));
#123682=DIRECTION('center_axis',(-3.71118737634973E-16,-1.,-1.23467863058847E-16));
#123683=DIRECTION('ref_axis',(-1.,3.71118737634973E-16,0.));
#123684=DIRECTION('center_axis',(-3.71118737634973E-16,-1.,-1.23467863058847E-16));
#123685=DIRECTION('ref_axis',(-1.,3.71118737634973E-16,0.));
#123686=DIRECTION('center_axis',(-5.72252063890675E-16,1.,1.23467863058847E-16));
#123687=DIRECTION('ref_axis',(1.,5.72252063890675E-16,0.));
#123688=DIRECTION('center_axis',(-5.72252063890675E-16,1.,1.23467863058847E-16));
#123689=DIRECTION('ref_axis',(1.,5.72252063890675E-16,0.));
#123690=DIRECTION('center_axis',(1.90750687963558E-16,-1.,-1.23467863058847E-16));
#123691=DIRECTION('ref_axis',(-2.39311615755447E-50,1.23467863058847E-16,
-1.));
#123692=DIRECTION('center_axis',(1.90750687963558E-16,-1.,-1.23467863058847E-16));
#123693=DIRECTION('ref_axis',(-2.39311615755447E-50,1.23467863058847E-16,
-1.));
#123694=DIRECTION('center_axis',(1.23706245878324E-16,-1.,-1.23467863058847E-16));
#123695=DIRECTION('ref_axis',(9.34199996189111E-49,1.23467863058847E-16,
-1.));
#123696=DIRECTION('center_axis',(1.23706245878324E-16,-1.,-1.23467863058847E-16));
#123697=DIRECTION('ref_axis',(9.34199996189111E-49,1.23467863058847E-16,
-1.));
#123698=DIRECTION('center_axis',(1.23706245878324E-16,1.,1.23467863058847E-16));
#123699=DIRECTION('ref_axis',(1.,-1.23706245878324E-16,0.));
#123700=DIRECTION('center_axis',(1.23706245878324E-16,1.,1.23467863058847E-16));
#123701=DIRECTION('ref_axis',(1.,-1.23706245878324E-16,0.));
#123702=DIRECTION('center_axis',(-4.76876719908896E-16,-1.,-1.23467863058847E-16));
#123703=DIRECTION('ref_axis',(-1.,4.76876719908896E-16,0.));
#123704=DIRECTION('center_axis',(-4.76876719908896E-16,-1.,-1.23467863058847E-16));
#123705=DIRECTION('ref_axis',(-1.,4.76876719908896E-16,0.));
#123706=DIRECTION('center_axis',(9.53753439817791E-17,1.,1.23467863058847E-16));
#123707=DIRECTION('ref_axis',(-4.60419424770999E-49,1.23467863058847E-16,
-1.));
#123708=DIRECTION('center_axis',(9.53753439817791E-17,1.,1.23467863058847E-16));
#123709=DIRECTION('ref_axis',(-4.60419424770999E-49,1.23467863058847E-16,
-1.));
#123710=DIRECTION('center_axis',(0.,1.23467863058847E-16,-1.));
#123711=DIRECTION('ref_axis',(0.705921937789673,-0.708289642552588,0.));
#123712=DIRECTION('center_axis',(0.5,0.866025403784438,1.0692630595994E-16));
#123713=DIRECTION('ref_axis',(2.13852611919879E-16,-5.48307457472744E-35,
-1.));
#123714=DIRECTION('',(0.,1.23467863058847E-16,-1.));
#123715=DIRECTION('',(0.,1.23467863058847E-16,-1.));
#123716=DIRECTION('center_axis',(1.,0.,0.));
#123717=DIRECTION('ref_axis',(0.,1.,0.));
#123718=DIRECTION('',(0.,1.23467863058847E-16,-1.));
#123719=DIRECTION('center_axis',(0.5,-0.866025403784439,-1.0692630595994E-16));
#123720=DIRECTION('ref_axis',(4.1166144903646E-33,1.23467863058847E-16,
-1.));
#123721=DIRECTION('',(0.,1.23467863058847E-16,-1.));
#123722=DIRECTION('center_axis',(-0.5,-0.866025403784439,-1.0692630595994E-16));
#123723=DIRECTION('ref_axis',(-0.866025403784439,0.5,-7.83367607530638E-34));
#123724=DIRECTION('',(0.,1.23467863058847E-16,-1.));
#123725=DIRECTION('center_axis',(-1.,0.,0.));
#123726=DIRECTION('ref_axis',(0.,0.,1.));
#123727=DIRECTION('',(0.,1.23467863058847E-16,-1.));
#123728=DIRECTION('center_axis',(-0.5,0.866025403784439,1.0692630595994E-16));
#123729=DIRECTION('ref_axis',(2.1385261191988E-16,4.09037363277686E-33,
1.));
#123730=DIRECTION('center_axis',(0.,0.,-1.));
#123731=DIRECTION('ref_axis',(0.,1.,0.));
#123732=DIRECTION('',(-1.06057523872491E-16,-0.866025403784439,-0.5));
#123733=DIRECTION('center_axis',(0.,0.,-1.));
#123734=DIRECTION('ref_axis',(0.,1.,0.));
#123735=DIRECTION('center_axis',(0.,0.,1.));
#123736=DIRECTION('ref_axis',(0.,1.,0.));
#123737=DIRECTION('center_axis',(0.,0.,-1.));
#123738=DIRECTION('ref_axis',(0.,1.,0.));
#123739=DIRECTION('center_axis',(0.,0.,1.));
#123740=DIRECTION('ref_axis',(0.,1.,0.));
#123741=DIRECTION('center_axis',(0.,0.,-1.));
#123742=DIRECTION('ref_axis',(0.,1.,0.));
#123743=DIRECTION('center_axis',(0.,0.,1.));
#123744=DIRECTION('ref_axis',(0.,1.,0.));
#123745=DIRECTION('center_axis',(0.,0.,-1.));
#123746=DIRECTION('ref_axis',(0.,1.,0.));
#123747=DIRECTION('center_axis',(0.,0.,1.));
#123748=DIRECTION('ref_axis',(0.,1.,0.));
#123749=DIRECTION('center_axis',(0.,0.,-1.));
#123750=DIRECTION('ref_axis',(0.,1.,0.));
#123751=DIRECTION('center_axis',(0.,0.,1.));
#123752=DIRECTION('ref_axis',(0.,1.,0.));
#123753=DIRECTION('center_axis',(0.,0.,-1.));
#123754=DIRECTION('ref_axis',(0.,1.,0.));
#123755=DIRECTION('center_axis',(0.,0.,1.));
#123756=DIRECTION('ref_axis',(0.,1.,0.));
#123757=DIRECTION('center_axis',(0.,1.23467863058847E-16,-1.));
#123758=DIRECTION('ref_axis',(0.,1.,0.));
#123759=DIRECTION('center_axis',(0.,0.,1.));
#123760=DIRECTION('ref_axis',(0.,1.,0.));
#123761=DIRECTION('center_axis',(-1.,0.,0.));
#123762=DIRECTION('ref_axis',(0.,-1.,0.));
#123763=DIRECTION('center_axis',(0.,0.,-1.));
#123764=DIRECTION('ref_axis',(0.,1.,0.));
#123765=DIRECTION('center_axis',(0.,0.,-1.));
#123766=DIRECTION('ref_axis',(0.,1.,0.));
#123767=DIRECTION('center_axis',(0.,1.23467863058847E-16,-1.));
#123768=DIRECTION('ref_axis',(-1.,0.,0.));
#123769=DIRECTION('center_axis',(0.,0.,1.));
#123770=DIRECTION('ref_axis',(0.,1.,0.));
#123771=DIRECTION('center_axis',(0.,1.23467863058847E-16,-1.));
#123772=DIRECTION('ref_axis',(-1.,0.,0.));
#123773=DIRECTION('center_axis',(0.,0.,1.));
#123774=DIRECTION('ref_axis',(0.,-1.,0.));
#123775=DIRECTION('',(0.,0.,-1.));
#123776=DIRECTION('center_axis',(1.51575151553259E-16,1.51575151553259E-16,
-1.));
#123777=DIRECTION('ref_axis',(-1.,-2.17577274266937E-49,-1.51575151553259E-16));
#123778=DIRECTION('center_axis',(1.51575151553259E-16,4.20705558038691E-31,
-1.));
#123779=DIRECTION('ref_axis',(2.77555756156289E-15,-1.,-1.66404192638572E-45));
#123780=DIRECTION('center_axis',(1.51575151553259E-16,4.20705558038691E-31,
-1.));
#123781=DIRECTION('ref_axis',(2.77555756156289E-15,-1.,-1.66404192638572E-45));
#123782=DIRECTION('center_axis',(1.51575151553259E-16,4.20705558038691E-31,
-1.));
#123783=DIRECTION('ref_axis',(2.77555756156289E-15,-1.,-1.66404192638572E-45));
#123784=DIRECTION('center_axis',(1.51575151553259E-16,4.20705558038691E-31,
-1.));
#123785=DIRECTION('ref_axis',(2.77555756156289E-15,-1.,-1.66404192638572E-45));
#123786=DIRECTION('center_axis',(1.51575151553259E-16,4.20705558038691E-31,
-1.));
#123787=DIRECTION('ref_axis',(2.77555756156289E-15,-1.,-1.66404192638572E-45));
#123788=DIRECTION('center_axis',(1.51575151553259E-16,4.20705558038691E-31,
-1.));
#123789=DIRECTION('ref_axis',(2.77555756156289E-15,-1.,-1.66404192638572E-45));
#123790=DIRECTION('center_axis',(-1.51575151553259E-16,-4.20705558038691E-31,
1.));
#123791=DIRECTION('ref_axis',(2.77555756156289E-15,-1.,-1.66404192638572E-45));
#123792=DIRECTION('center_axis',(-1.51575151553259E-16,-4.20705558038691E-31,
1.));
#123793=DIRECTION('ref_axis',(2.77555756156289E-15,-1.,-1.66404192638572E-45));
#123794=DIRECTION('center_axis',(-1.51575151553259E-16,-4.20705558038691E-31,
1.));
#123795=DIRECTION('ref_axis',(2.77555756156289E-15,-1.,-1.66404192638572E-45));
#123796=DIRECTION('center_axis',(-1.51575151553259E-16,-4.20705558038691E-31,
1.));
#123797=DIRECTION('ref_axis',(2.77555756156289E-15,-1.,-1.66404192638572E-45));
#123798=DIRECTION('center_axis',(-1.51575151553259E-16,-4.20705558038691E-31,
1.));
#123799=DIRECTION('ref_axis',(2.77555756156289E-15,-1.,-1.66404192638572E-45));
#123800=DIRECTION('center_axis',(-1.51575151553259E-16,-4.20705558038691E-31,
1.));
#123801=DIRECTION('ref_axis',(2.77555756156289E-15,-1.,-1.66404192638572E-45));
#123802=DIRECTION('center_axis',(1.51575151553259E-16,1.51575151553259E-16,
-1.));
#123803=DIRECTION('ref_axis',(-1.,-2.17577274266937E-49,-1.51575151553259E-16));
#123804=DIRECTION('center_axis',(1.51575151553259E-16,4.20705558038691E-31,
-1.));
#123805=DIRECTION('ref_axis',(2.77555756156289E-15,-1.,-1.66404192638572E-45));
#123806=DIRECTION('center_axis',(-1.51575151553259E-16,-8.41411116077385E-31,
1.));
#123807=DIRECTION('ref_axis',(5.55111512312578E-15,-1.,-3.67840846885265E-45));
#123808=DIRECTION('center_axis',(-1.51575151553259E-16,-8.41411116077385E-31,
1.));
#123809=DIRECTION('ref_axis',(5.55111512312578E-15,-1.,-3.67840846885265E-45));
#123810=DIRECTION('center_axis',(-1.51575151553259E-16,0.,1.));
#123811=DIRECTION('ref_axis',(0.,-1.,0.));
#123812=DIRECTION('center_axis',(-1.51575151553259E-16,-4.20705558038691E-31,
1.));
#123813=DIRECTION('ref_axis',(2.77555756156289E-15,-1.,-1.66404192638572E-45));
#123814=DIRECTION('center_axis',(-1.51575151553258E-16,4.20705558038689E-31,
1.));
#123815=DIRECTION('ref_axis',(-2.77555756156289E-15,-1.,7.00649232162409E-46));
#123816=DIRECTION('center_axis',(1.51575151553259E-16,4.20705558038691E-31,
-1.));
#123817=DIRECTION('ref_axis',(2.77555756156289E-15,-1.,-1.66404192638572E-45));
#123818=DIRECTION('center_axis',(1.51575151553259E-16,4.20705558038691E-31,
-1.));
#123819=DIRECTION('ref_axis',(2.77555756156289E-15,-1.,-1.66404192638572E-45));
#123820=DIRECTION('center_axis',(1.51575151553259E-16,4.20705558038691E-31,
-1.));
#123821=DIRECTION('ref_axis',(2.77555756156289E-15,-1.,-1.66404192638572E-45));
#123822=DIRECTION('center_axis',(1.51575151553259E-16,4.20705558038691E-31,
-1.));
#123823=DIRECTION('ref_axis',(2.77555756156289E-15,-1.,-1.66404192638572E-45));
#123824=DIRECTION('center_axis',(1.51575151553259E-16,4.20705558038691E-31,
-1.));
#123825=DIRECTION('ref_axis',(2.77555756156289E-15,-1.,-1.66404192638572E-45));
#123826=DIRECTION('center_axis',(1.51575151553259E-16,4.20705558038691E-31,
-1.));
#123827=DIRECTION('ref_axis',(2.77555756156289E-15,-1.,-1.66404192638572E-45));
#123828=DIRECTION('center_axis',(-3.49148133884314E-15,1.,1.51575151553259E-16));
#123829=DIRECTION('ref_axis',(1.,3.49148133884314E-15,0.));
#123830=DIRECTION('',(3.95893176803294E-18,-1.51575151553259E-16,1.));
#123831=DIRECTION('',(3.95893176803294E-18,-1.51575151553259E-16,1.));
#123832=DIRECTION('center_axis',(-0.866025403784439,0.499999999999999,7.92161112595944E-17));
#123833=DIRECTION('ref_axis',(9.14708863197643E-17,-1.05181136389903E-33,
1.));
#123834=DIRECTION('',(3.95893176803294E-18,-1.51575151553259E-16,1.));
#123835=DIRECTION('center_axis',(-0.866025403784438,-0.500000000000001,
-7.23590402936645E-17));
#123836=DIRECTION('ref_axis',(-0.500000000000001,0.866025403784438,-2.57334411451296E-33));
#123837=DIRECTION('',(3.95893176803294E-18,-1.51575151553259E-16,1.));
#123838=DIRECTION('center_axis',(3.64171279871685E-15,-1.,-1.51575151553259E-16));
#123839=DIRECTION('ref_axis',(5.87651897213004E-48,1.51575151553259E-16,
-1.));
#123840=DIRECTION('',(3.95893176803294E-18,-1.51575151553259E-16,1.));
#123841=DIRECTION('center_axis',(0.866025403784439,-0.499999999999999,-7.92161112595951E-17));
#123842=DIRECTION('ref_axis',(8.15047850955652E-33,1.5843222251919E-16,
-1.));
#123843=DIRECTION('',(3.95893176803294E-18,-1.51575151553259E-16,1.));
#123844=DIRECTION('center_axis',(0.866025403784438,0.500000000000001,7.23590402936639E-17));
#123845=DIRECTION('ref_axis',(-3.44176788548726E-33,1.44718080587327E-16,
-1.));
#123846=DIRECTION('center_axis',(0.,0.,-1.));
#123847=DIRECTION('ref_axis',(0.,-1.,0.));
#123848=DIRECTION('center_axis',(0.,0.,-1.));
#123849=DIRECTION('ref_axis',(-1.,0.,0.));
#123850=DIRECTION('center_axis',(0.,0.,-1.));
#123851=DIRECTION('ref_axis',(-1.,0.,0.));
#123852=DIRECTION('center_axis',(0.,0.,-1.));
#123853=DIRECTION('ref_axis',(-1.,0.,0.));
#123854=DIRECTION('center_axis',(0.,0.,-1.));
#123855=DIRECTION('ref_axis',(-1.,0.,0.));
#123856=DIRECTION('center_axis',(0.,0.,-1.));
#123857=DIRECTION('ref_axis',(-1.,0.,0.));
#123858=DIRECTION('center_axis',(0.,0.,-1.));
#123859=DIRECTION('ref_axis',(-1.,0.,0.));
#123860=DIRECTION('center_axis',(0.,0.,1.));
#123861=DIRECTION('ref_axis',(-1.,0.,0.));
#123862=DIRECTION('center_axis',(0.,0.,1.));
#123863=DIRECTION('ref_axis',(-1.,0.,0.));
#123864=DIRECTION('center_axis',(0.,0.,1.));
#123865=DIRECTION('ref_axis',(-1.,0.,0.));
#123866=DIRECTION('center_axis',(0.,0.,1.));
#123867=DIRECTION('ref_axis',(-1.,0.,0.));
#123868=DIRECTION('center_axis',(0.,0.,1.));
#123869=DIRECTION('ref_axis',(-1.,0.,0.));
#123870=DIRECTION('center_axis',(0.,0.,1.));
#123871=DIRECTION('ref_axis',(-1.,0.,0.));
#123872=DIRECTION('center_axis',(0.,0.,-1.));
#123873=DIRECTION('ref_axis',(0.,-1.,0.));
#123874=DIRECTION('center_axis',(0.,0.,-1.));
#123875=DIRECTION('ref_axis',(-1.,0.,0.));
#123876=DIRECTION('center_axis',(0.,0.,1.));
#123877=DIRECTION('ref_axis',(-1.,0.,0.));
#123878=DIRECTION('center_axis',(0.,0.,1.));
#123879=DIRECTION('ref_axis',(-1.,-1.38777878078145E-15,0.));
#123880=DIRECTION('center_axis',(0.,0.,1.));
#123881=DIRECTION('ref_axis',(-1.,1.38777878078145E-15,0.));
#123882=DIRECTION('center_axis',(0.,0.,1.));
#123883=DIRECTION('ref_axis',(-1.,-1.38777878078145E-15,0.));
#123884=DIRECTION('center_axis',(0.,0.,1.));
#123885=DIRECTION('ref_axis',(-1.,4.16333634234434E-15,0.));
#123886=DIRECTION('center_axis',(0.,0.,-1.));
#123887=DIRECTION('ref_axis',(-1.,0.,0.));
#123888=DIRECTION('center_axis',(0.,0.,-1.));
#123889=DIRECTION('ref_axis',(-1.,0.,0.));
#123890=DIRECTION('center_axis',(0.,0.,-1.));
#123891=DIRECTION('ref_axis',(-1.,0.,0.));
#123892=DIRECTION('center_axis',(0.,0.,-1.));
#123893=DIRECTION('ref_axis',(-1.,0.,0.));
#123894=DIRECTION('center_axis',(0.,0.,-1.));
#123895=DIRECTION('ref_axis',(-1.,0.,0.));
#123896=DIRECTION('center_axis',(0.,0.,-1.));
#123897=DIRECTION('ref_axis',(-1.,0.,0.));
#123898=DIRECTION('center_axis',(1.,0.,0.));
#123899=DIRECTION('ref_axis',(0.,1.,0.));
#123900=DIRECTION('',(0.,-1.55534083321291E-16,1.));
#123901=DIRECTION('',(0.,-1.55534083321291E-16,1.));
#123902=DIRECTION('center_axis',(0.5,0.866025403784439,1.34696467310564E-16));
#123903=DIRECTION('ref_axis',(2.69392934621129E-16,1.24972477443329E-33,
-1.));
#123904=DIRECTION('',(0.,-1.55534083321291E-16,1.));
#123905=DIRECTION('center_axis',(-0.5,0.866025403784438,1.34696467310564E-16));
#123906=DIRECTION('ref_axis',(2.69392934621128E-16,-2.09027289648572E-32,
1.));
#123907=DIRECTION('',(0.,-1.55534083321291E-16,1.));
#123908=DIRECTION('center_axis',(-1.,-1.50231459873716E-16,-2.33661123974778E-32));
#123909=DIRECTION('ref_axis',(-1.50231459873716E-16,1.,-1.23954453046792E-64));
#123910=DIRECTION('',(0.,-1.55534083321291E-16,1.));
#123911=DIRECTION('center_axis',(-0.5,-0.866025403784439,-1.34696467310564E-16));
#123912=DIRECTION('ref_axis',(-0.866025403784439,0.5,-3.71223821158428E-33));
#123913=DIRECTION('',(0.,-1.55534083321291E-16,1.));
#123914=DIRECTION('center_axis',(0.5,-0.866025403784438,-1.34696467310564E-16));
#123915=DIRECTION('ref_axis',(4.44087077315589E-33,1.55534083321292E-16,
-1.));
#123916=DIRECTION('center_axis',(-0.5,0.866025403784438,1.0692630595994E-16));
#123917=DIRECTION('ref_axis',(2.13852611919879E-16,5.48307457472744E-35,
1.));
#123918=DIRECTION('',(0.,1.23467863058847E-16,-1.));
#123919=DIRECTION('',(0.,1.23467863058847E-16,-1.));
#123920=DIRECTION('center_axis',(-1.,0.,0.));
#123921=DIRECTION('ref_axis',(0.,0.,1.));
#123922=DIRECTION('',(0.,1.23467863058847E-16,-1.));
#123923=DIRECTION('center_axis',(-0.5,-0.866025403784439,-1.0692630595994E-16));
#123924=DIRECTION('ref_axis',(-0.866025403784439,0.5,-9.26929360883051E-34));
#123925=DIRECTION('',(0.,1.23467863058847E-16,-1.));
#123926=DIRECTION('center_axis',(0.5,-0.866025403784439,-1.0692630595994E-16));
#123927=DIRECTION('ref_axis',(-4.5474696259435E-34,1.23467863058847E-16,
-1.));
#123928=DIRECTION('',(0.,1.23467863058847E-16,-1.));
#123929=DIRECTION('center_axis',(1.,0.,0.));
#123930=DIRECTION('ref_axis',(0.,1.,0.));
#123931=DIRECTION('',(0.,1.23467863058847E-16,-1.));
#123932=DIRECTION('center_axis',(0.5,0.866025403784439,1.0692630595994E-16));
#123933=DIRECTION('ref_axis',(2.1385261191988E-16,-4.09037363277686E-33,
-1.));
#123934=DIRECTION('center_axis',(0.,0.,-1.));
#123935=DIRECTION('ref_axis',(0.,1.,0.));
#123936=DIRECTION('',(-1.06057523872491E-16,-0.866025403784439,-0.5));
#123937=DIRECTION('center_axis',(0.,0.,-1.));
#123938=DIRECTION('ref_axis',(0.,1.,0.));
#123939=DIRECTION('center_axis',(0.,0.,-1.));
#123940=DIRECTION('ref_axis',(0.,1.,0.));
#123941=DIRECTION('center_axis',(0.,0.,-1.));
#123942=DIRECTION('ref_axis',(0.,1.,0.));
#123943=DIRECTION('center_axis',(0.,0.,-1.));
#123944=DIRECTION('ref_axis',(0.,1.,0.));
#123945=DIRECTION('center_axis',(0.,0.,-1.));
#123946=DIRECTION('ref_axis',(0.,1.,0.));
#123947=DIRECTION('center_axis',(0.,0.,-1.));
#123948=DIRECTION('ref_axis',(0.,1.,0.));
#123949=DIRECTION('center_axis',(0.,0.,-1.));
#123950=DIRECTION('ref_axis',(0.,1.,0.));
#123951=DIRECTION('center_axis',(0.,0.,-1.));
#123952=DIRECTION('ref_axis',(0.,1.,0.));
#123953=DIRECTION('center_axis',(0.,0.,-1.));
#123954=DIRECTION('ref_axis',(0.,1.,0.));
#123955=DIRECTION('center_axis',(0.,0.,-1.));
#123956=DIRECTION('ref_axis',(0.,1.,0.));
#123957=DIRECTION('center_axis',(0.,0.,-1.));
#123958=DIRECTION('ref_axis',(0.,1.,0.));
#123959=DIRECTION('center_axis',(0.,0.,-1.));
#123960=DIRECTION('ref_axis',(0.,1.,0.));
#123961=DIRECTION('center_axis',(0.,1.23467863058847E-16,-1.));
#123962=DIRECTION('ref_axis',(0.,1.,0.));
#123963=DIRECTION('center_axis',(0.,0.,-1.));
#123964=DIRECTION('ref_axis',(0.,1.,0.));
#123965=DIRECTION('center_axis',(-1.,0.,0.));
#123966=DIRECTION('ref_axis',(0.,-1.,0.));
#123967=DIRECTION('center_axis',(0.,0.,1.));
#123968=DIRECTION('ref_axis',(0.,1.,0.));
#123969=DIRECTION('center_axis',(0.,0.,1.));
#123970=DIRECTION('ref_axis',(0.,1.,0.));
#123971=DIRECTION('center_axis',(0.,1.23467863058847E-16,-1.));
#123972=DIRECTION('ref_axis',(-1.,0.,0.));
#123973=DIRECTION('center_axis',(0.,0.,-1.));
#123974=DIRECTION('ref_axis',(0.,1.,0.));
#123975=DIRECTION('center_axis',(0.,1.23467863058847E-16,-1.));
#123976=DIRECTION('ref_axis',(-1.,0.,0.));
#123977=DIRECTION('center_axis',(0.,0.,1.));
#123978=DIRECTION('ref_axis',(0.,-1.,0.));
#123979=DIRECTION('',(0.,0.,-1.));
#123980=DIRECTION('center_axis',(0.,0.,-1.));
#123981=DIRECTION('ref_axis',(1.,0.,0.));
#123982=DIRECTION('center_axis',(1.,0.,0.));
#123983=DIRECTION('ref_axis',(0.,0.,1.));
#123984=DIRECTION('center_axis',(0.0436193873653361,0.,0.999048221581858));
#123985=DIRECTION('ref_axis',(-0.999048221581858,0.,0.0436193873653362));
#123986=DIRECTION('center_axis',(0.0436193873653361,0.,-0.999048221581858));
#123987=DIRECTION('ref_axis',(0.999048221581858,0.,0.0436193873653362));
#123988=DIRECTION('center_axis',(-1.,0.,0.));
#123989=DIRECTION('ref_axis',(0.,0.,1.));
#123990=DIRECTION('center_axis',(-1.,0.,0.));
#123991=DIRECTION('ref_axis',(0.,0.,1.));
#123992=DIRECTION('center_axis',(-1.,0.,0.));
#123993=DIRECTION('ref_axis',(0.,0.,1.));
#123994=DIRECTION('center_axis',(0.,-1.,0.));
#123995=DIRECTION('ref_axis',(0.,0.,-1.));
#123996=DIRECTION('center_axis',(-1.,0.,0.));
#123997=DIRECTION('ref_axis',(0.,0.,1.));
#123998=DIRECTION('center_axis',(-1.,0.,0.));
#123999=DIRECTION('ref_axis',(0.,0.,1.));
#124000=DIRECTION('center_axis',(0.,-1.,0.));
#124001=DIRECTION('ref_axis',(0.,0.,-1.));
#124002=DIRECTION('center_axis',(1.,0.,0.));
#124003=DIRECTION('ref_axis',(0.,0.,1.));
#124004=DIRECTION('center_axis',(1.,0.,0.));
#124005=DIRECTION('ref_axis',(0.,0.,1.));
#124006=DIRECTION('center_axis',(-1.,0.,0.));
#124007=DIRECTION('ref_axis',(0.,0.,1.));
#124008=DIRECTION('center_axis',(-1.,0.,0.));
#124009=DIRECTION('ref_axis',(0.,0.,1.));
#124010=DIRECTION('',(0.,1.,0.));
#124011=DIRECTION('center_axis',(-1.,0.,0.));
#124012=DIRECTION('ref_axis',(0.,0.,1.));
#124013=DIRECTION('',(0.,-1.,0.));
#124014=DIRECTION('center_axis',(-0.0436193873653361,0.,-0.999048221581858));
#124015=DIRECTION('ref_axis',(-0.999048221581858,0.,0.0436193873653361));
#124016=DIRECTION('',(-0.999048221581858,-8.07120802883996E-16,0.0436193873653362));
#124017=DIRECTION('',(-0.999048221581858,0.,0.0436193873653362));
#124018=DIRECTION('center_axis',(1.,0.,0.));
#124019=DIRECTION('ref_axis',(0.,0.,1.));
#124020=DIRECTION('',(-0.999048221581858,0.,-0.0436193873653362));
#124021=DIRECTION('center_axis',(-0.0436193873653361,0.,0.999048221581858));
#124022=DIRECTION('ref_axis',(0.,1.,0.));
#124023=DIRECTION('',(-0.999048221581858,0.,-0.0436193873653362));
#124024=DIRECTION('center_axis',(1.,0.,0.));
#124025=DIRECTION('ref_axis',(0.,0.,1.));
#124026=DIRECTION('center_axis',(-1.,0.,0.));
#124027=DIRECTION('ref_axis',(0.,0.,1.));
#124028=DIRECTION('center_axis',(-1.,0.,0.));
#124029=DIRECTION('ref_axis',(0.,0.,1.));
#124030=DIRECTION('center_axis',(1.,0.,0.));
#124031=DIRECTION('ref_axis',(0.,0.,-1.));
#124032=DIRECTION('center_axis',(-1.,0.,0.));
#124033=DIRECTION('ref_axis',(0.,0.,1.));
#124034=DIRECTION('',(-1.,0.,0.));
#124035=DIRECTION('center_axis',(1.,0.,0.));
#124036=DIRECTION('ref_axis',(0.,0.,-1.));
#124037=DIRECTION('',(-1.,0.,0.));
#124038=DIRECTION('center_axis',(-1.,0.,0.));
#124039=DIRECTION('ref_axis',(0.,0.,1.));
#124040=DIRECTION('center_axis',(0.,0.,-1.));
#124041=DIRECTION('ref_axis',(1.,0.,0.));
#124042=DIRECTION('center_axis',(0.,0.,1.));
#124043=DIRECTION('ref_axis',(-1.,0.,0.));
#124044=DIRECTION('',(0.707106781186552,-8.65956056235499E-17,0.707106781186543));
#124045=DIRECTION('center_axis',(0.,0.,-1.));
#124046=DIRECTION('ref_axis',(-1.,0.,0.));
#124047=DIRECTION('center_axis',(0.,0.,1.));
#124048=DIRECTION('ref_axis',(1.,0.,0.));
#124049=DIRECTION('center_axis',(0.,0.,-1.));
#124050=DIRECTION('ref_axis',(1.,0.,0.));
#124051=DIRECTION('center_axis',(0.,0.,-1.));
#124052=DIRECTION('ref_axis',(-1.,0.,0.));
#124053=DIRECTION('',(0.,0.,1.));
#124054=DIRECTION('center_axis',(0.,1.23467863058847E-16,-1.));
#124055=DIRECTION('ref_axis',(-1.,0.,0.));
#124056=DIRECTION('center_axis',(0.,0.,1.));
#124057=DIRECTION('ref_axis',(0.,1.,0.));
#124058=DIRECTION('center_axis',(0.,0.,-1.));
#124059=DIRECTION('ref_axis',(1.,0.,0.));
#124060=DIRECTION('center_axis',(0.,0.,-1.));
#124061=DIRECTION('ref_axis',(-1.,0.,0.));
#124062=DIRECTION('',(0.,0.,1.));
#124063=DIRECTION('center_axis',(0.,0.,1.));
#124064=DIRECTION('ref_axis',(1.,0.,0.));
#124065=DIRECTION('center_axis',(0.,1.,0.));
#124066=DIRECTION('ref_axis',(0.,0.,1.));
#124067=DIRECTION('center_axis',(1.,0.,0.));
#124068=DIRECTION('ref_axis',(0.,0.,-1.));
#124069=DIRECTION('center_axis',(0.,-1.,0.));
#124070=DIRECTION('ref_axis',(0.,0.,1.));
#124071=DIRECTION('center_axis',(0.,0.,1.));
#124072=DIRECTION('ref_axis',(1.,0.,0.));
#124073=DIRECTION('center_axis',(0.,1.,0.));
#124074=DIRECTION('ref_axis',(0.,0.,1.));
#124075=DIRECTION('center_axis',(0.,0.,-1.));
#124076=DIRECTION('ref_axis',(-1.,0.,0.));
#124077=DIRECTION('center_axis',(0.,0.,1.));
#124078=DIRECTION('ref_axis',(1.,0.,0.));
#124079=DIRECTION('',(0.,0.,-1.));
#124080=DIRECTION('',(0.,0.,1.));
#124081=DIRECTION('center_axis',(1.,0.,0.));
#124082=DIRECTION('ref_axis',(0.,0.,-1.));
#124083=DIRECTION('center_axis',(1.,0.,0.));
#124084=DIRECTION('ref_axis',(0.,0.,-1.));
#124085=DIRECTION('',(-1.,0.,0.));
#124086=DIRECTION('',(1.,0.,0.));
#124087=DIRECTION('center_axis',(0.,1.,0.));
#124088=DIRECTION('ref_axis',(0.,0.,1.));
#124089=DIRECTION('center_axis',(1.,0.,0.));
#124090=DIRECTION('ref_axis',(0.,0.,-1.));
#124091=DIRECTION('center_axis',(0.,1.,0.));
#124092=DIRECTION('ref_axis',(0.,0.,1.));
#124093=DIRECTION('center_axis',(0.,-1.,0.));
#124094=DIRECTION('ref_axis',(0.,0.,1.));
#124095=DIRECTION('center_axis',(0.,1.,0.));
#124096=DIRECTION('ref_axis',(0.,0.,1.));
#124097=DIRECTION('center_axis',(0.,0.,1.));
#124098=DIRECTION('ref_axis',(1.,0.,0.));
#124099=DIRECTION('center_axis',(0.,-1.,0.));
#124100=DIRECTION('ref_axis',(0.,0.,1.));
#124101=DIRECTION('center_axis',(0.,1.,0.));
#124102=DIRECTION('ref_axis',(0.,0.,1.));
#124103=DIRECTION('center_axis',(-1.,0.,0.));
#124104=DIRECTION('ref_axis',(0.,0.,1.));
#124105=DIRECTION('center_axis',(1.,0.,0.));
#124106=DIRECTION('ref_axis',(0.,0.,-1.));
#124107=DIRECTION('',(-1.,0.,0.));
#124108=DIRECTION('',(1.,0.,0.));
#124109=DIRECTION('center_axis',(0.,0.,-1.));
#124110=DIRECTION('ref_axis',(-1.,0.,0.));
#124111=DIRECTION('center_axis',(0.,0.,1.));
#124112=DIRECTION('ref_axis',(1.,0.,0.));
#124113=DIRECTION('',(0.,0.,-1.));
#124114=DIRECTION('',(0.,0.,1.));
#124115=DIRECTION('center_axis',(0.,1.,0.));
#124116=DIRECTION('ref_axis',(0.,0.,1.));
#124117=DIRECTION('center_axis',(0.,-1.,0.));
#124118=DIRECTION('ref_axis',(0.,0.,1.));
#124119=DIRECTION('center_axis',(0.,1.,0.));
#124120=DIRECTION('ref_axis',(0.,0.,1.));
#124121=DIRECTION('center_axis',(1.,0.,0.));
#124122=DIRECTION('ref_axis',(0.,1.,0.));
#124123=DIRECTION('',(0.,-1.,0.));
#124124=DIRECTION('',(0.,-1.,0.));
#124125=DIRECTION('',(0.,3.03450170724806E-16,1.));
#124126=DIRECTION('center_axis',(0.,-1.,0.));
#124127=DIRECTION('ref_axis',(0.,0.,-1.));
#124128=DIRECTION('',(0.,-1.,0.));
#124129=DIRECTION('center_axis',(0.,1.,0.));
#124130=DIRECTION('ref_axis',(0.,0.,-1.));
#124131=DIRECTION('center_axis',(0.,-1.,0.));
#124132=DIRECTION('ref_axis',(0.,0.,-1.));
#124133=DIRECTION('',(0.,-1.,0.));
#124134=DIRECTION('center_axis',(0.,1.,0.));
#124135=DIRECTION('ref_axis',(0.,0.,-1.));
#124136=DIRECTION('center_axis',(1.,0.,0.));
#124137=DIRECTION('ref_axis',(0.,1.,0.));
#124138=DIRECTION('',(0.,-1.,0.));
#124139=DIRECTION('',(0.,0.,1.));
#124140=DIRECTION('',(0.,1.,0.));
#124141=DIRECTION('',(0.,0.,-1.));
#124142=DIRECTION('center_axis',(-1.,0.,0.));
#124143=DIRECTION('ref_axis',(0.,0.,1.));
#124144=DIRECTION('center_axis',(-1.,0.,0.));
#124145=DIRECTION('ref_axis',(0.,0.,1.));
#124146=DIRECTION('center_axis',(0.,1.,0.));
#124147=DIRECTION('ref_axis',(0.,0.,1.));
#124148=DIRECTION('center_axis',(0.,0.,1.));
#124149=DIRECTION('ref_axis',(1.,0.,0.));
#124150=DIRECTION('center_axis',(0.,1.,0.));
#124151=DIRECTION('ref_axis',(5.20417042793042E-15,0.,1.));
#124152=DIRECTION('center_axis',(1.,0.,0.));
#124153=DIRECTION('ref_axis',(0.,0.,-1.));
#124154=DIRECTION('center_axis',(0.,-1.,0.));
#124155=DIRECTION('ref_axis',(0.,0.,1.));
#124156=DIRECTION('center_axis',(0.,0.,1.));
#124157=DIRECTION('ref_axis',(-1.,0.,0.));
#124158=DIRECTION('center_axis',(0.,0.,1.));
#124159=DIRECTION('ref_axis',(1.,0.,0.));
#124160=DIRECTION('',(0.,0.,-1.));
#124161=DIRECTION('center_axis',(0.,1.,0.));
#124162=DIRECTION('ref_axis',(0.,0.,1.));
#124163=DIRECTION('center_axis',(-1.,0.,0.));
#124164=DIRECTION('ref_axis',(0.,0.,1.));
#124165=DIRECTION('center_axis',(0.,1.,0.));
#124166=DIRECTION('ref_axis',(0.,0.,1.));
#124167=DIRECTION('center_axis',(0.,-1.,0.));
#124168=DIRECTION('ref_axis',(0.,0.,1.));
#124169=DIRECTION('center_axis',(0.,-1.,0.));
#124170=DIRECTION('ref_axis',(0.,0.,-1.));
#124171=DIRECTION('',(0.,-1.,0.));
#124172=DIRECTION('center_axis',(0.,-1.,0.));
#124173=DIRECTION('ref_axis',(0.,0.,-1.));
#124174=DIRECTION('center_axis',(0.,-1.,0.));
#124175=DIRECTION('ref_axis',(0.,0.,-1.));
#124176=DIRECTION('center_axis',(1.,0.,0.));
#124177=DIRECTION('ref_axis',(0.,0.,-1.));
#124178=DIRECTION('center_axis',(0.,1.,0.));
#124179=DIRECTION('ref_axis',(0.,0.,-1.));
#124180=DIRECTION('center_axis',(0.,0.,-1.));
#124181=DIRECTION('ref_axis',(-1.,0.,0.));
#124182=DIRECTION('center_axis',(0.,-1.,0.));
#124183=DIRECTION('ref_axis',(0.,0.,-1.));
#124184=DIRECTION('center_axis',(0.,0.,-1.));
#124185=DIRECTION('ref_axis',(-1.,0.,0.));
#124186=DIRECTION('center_axis',(0.,1.,0.));
#124187=DIRECTION('ref_axis',(0.,0.,-1.));
#124188=DIRECTION('center_axis',(-1.,0.,0.));
#124189=DIRECTION('ref_axis',(0.,0.,1.));
#124190=DIRECTION('center_axis',(0.,-1.,0.));
#124191=DIRECTION('ref_axis',(0.,0.,-1.));
#124192=DIRECTION('center_axis',(0.,0.,1.));
#124193=DIRECTION('ref_axis',(-1.,0.,0.));
#124194=DIRECTION('',(0.,0.,1.));
#124195=DIRECTION('center_axis',(0.,-1.,0.));
#124196=DIRECTION('ref_axis',(0.,0.,-1.));
#124197=DIRECTION('',(0.,1.,0.));
#124198=DIRECTION('center_axis',(0.,-1.,0.));
#124199=DIRECTION('ref_axis',(0.,0.,-1.));
#124200=DIRECTION('',(0.,1.,0.));
#124201=DIRECTION('center_axis',(0.,1.,0.));
#124202=DIRECTION('ref_axis',(0.,0.,-1.));
#124203=DIRECTION('',(0.,-1.,0.));
#124204=DIRECTION('center_axis',(0.,-1.,0.));
#124205=DIRECTION('ref_axis',(-5.20417042793042E-15,0.,1.));
#124206=DIRECTION('center_axis',(0.,0.,1.));
#124207=DIRECTION('ref_axis',(1.,0.,0.));
#124208=DIRECTION('center_axis',(0.,0.,1.));
#124209=DIRECTION('ref_axis',(1.,0.,0.));
#124210=DIRECTION('',(0.,0.,-1.));
#124211=DIRECTION('center_axis',(0.,0.,1.));
#124212=DIRECTION('ref_axis',(1.,0.,0.));
#124213=DIRECTION('',(0.,0.,1.));
#124214=DIRECTION('center_axis',(0.,-1.,0.));
#124215=DIRECTION('ref_axis',(0.,0.,-1.));
#124216=DIRECTION('center_axis',(-1.,0.,0.));
#124217=DIRECTION('ref_axis',(0.,0.,1.));
#124218=DIRECTION('center_axis',(0.,-1.,0.));
#124219=DIRECTION('ref_axis',(0.,0.,-1.));
#124220=DIRECTION('center_axis',(0.,-1.,0.));
#124221=DIRECTION('ref_axis',(0.,0.,-1.));
#124222=DIRECTION('center_axis',(1.,0.,0.));
#124223=DIRECTION('ref_axis',(0.,0.,-1.));
#124224=DIRECTION('center_axis',(0.,1.,0.));
#124225=DIRECTION('ref_axis',(0.,0.,-1.));
#124226=DIRECTION('center_axis',(0.,-1.,0.));
#124227=DIRECTION('ref_axis',(0.,0.,-1.));
#124228=DIRECTION('center_axis',(0.,-1.,0.));
#124229=DIRECTION('ref_axis',(0.,0.,-1.));
#124230=DIRECTION('',(0.,1.,0.));
#124231=DIRECTION('',(0.,-1.,0.));
#124232=DIRECTION('center_axis',(0.,-1.,0.));
#124233=DIRECTION('ref_axis',(0.,0.,1.));
#124234=DIRECTION('center_axis',(0.,1.,0.));
#124235=DIRECTION('ref_axis',(0.,0.,1.));
#124236=DIRECTION('center_axis',(-1.,0.,0.));
#124237=DIRECTION('ref_axis',(0.,0.,1.));
#124238=DIRECTION('center_axis',(0.,1.,0.));
#124239=DIRECTION('ref_axis',(0.,0.,1.));
#124240=DIRECTION('center_axis',(0.,0.,-1.));
#124241=DIRECTION('ref_axis',(-1.,0.,0.));
#124242=DIRECTION('center_axis',(0.,0.,1.));
#124243=DIRECTION('ref_axis',(1.,0.,0.));
#124244=DIRECTION('',(0.,0.,-1.));
#124245=DIRECTION('center_axis',(0.,0.,-1.));
#124246=DIRECTION('ref_axis',(-1.,0.,0.));
#124247=DIRECTION('',(0.,0.,1.));
#124248=DIRECTION('center_axis',(0.,1.,0.));
#124249=DIRECTION('ref_axis',(0.,0.,1.));
#124250=DIRECTION('center_axis',(0.,1.,0.));
#124251=DIRECTION('ref_axis',(0.,0.,1.));
#124252=DIRECTION('center_axis',(1.,0.,0.));
#124253=DIRECTION('ref_axis',(0.,0.,-1.));
#124254=DIRECTION('center_axis',(-1.,0.,0.));
#124255=DIRECTION('ref_axis',(0.,0.,1.));
#124256=DIRECTION('center_axis',(-1.,0.,0.));
#124257=DIRECTION('ref_axis',(0.,0.,1.));
#124258=DIRECTION('center_axis',(-1.,0.,0.));
#124259=DIRECTION('ref_axis',(0.,0.,1.));
#124260=DIRECTION('center_axis',(0.,-1.,0.));
#124261=DIRECTION('ref_axis',(0.,0.,-1.));
#124262=DIRECTION('',(0.,-1.,0.));
#124263=DIRECTION('',(0.,-1.,0.));
#124264=DIRECTION('center_axis',(0.,-1.,0.));
#124265=DIRECTION('ref_axis',(0.,0.,-1.));
#124266=DIRECTION('center_axis',(0.,-1.,0.));
#124267=DIRECTION('ref_axis',(0.,0.,-1.));
#124268=DIRECTION('',(0.,-1.,0.));
#124269=DIRECTION('',(0.,-1.,0.));
#124270=DIRECTION('center_axis',(0.,-1.,0.));
#124271=DIRECTION('ref_axis',(0.,0.,-1.));
#124272=DIRECTION('center_axis',(-1.,0.,0.));
#124273=DIRECTION('ref_axis',(0.,0.,1.));
#124274=DIRECTION('',(1.,0.,0.));
#124275=DIRECTION('',(-1.,0.,0.));
#124276=DIRECTION('center_axis',(0.,0.,-1.));
#124277=DIRECTION('ref_axis',(0.,-1.,0.));
#124278=DIRECTION('',(1.,0.,0.));
#124279=DIRECTION('center_axis',(-1.,0.,0.));
#124280=DIRECTION('ref_axis',(0.,0.,1.));
#124281=DIRECTION('',(-1.,0.,0.));
#124282=DIRECTION('center_axis',(0.,-1.,0.));
#124283=DIRECTION('ref_axis',(0.,0.,-1.));
#124284=DIRECTION('',(1.,0.,0.));
#124285=DIRECTION('center_axis',(1.,0.,0.));
#124286=DIRECTION('ref_axis',(0.,0.,-1.));
#124287=DIRECTION('',(-1.,0.,0.));
#124288=DIRECTION('center_axis',(0.,0.,1.));
#124289=DIRECTION('ref_axis',(1.,0.,0.));
#124290=DIRECTION('',(1.,0.,0.));
#124291=DIRECTION('center_axis',(1.,0.,0.));
#124292=DIRECTION('ref_axis',(0.,0.,-1.));
#124293=DIRECTION('',(-1.,0.,0.));
#124294=DIRECTION('center_axis',(0.,1.,0.));
#124295=DIRECTION('ref_axis',(1.,0.,0.));
#124296=DIRECTION('center_axis',(0.,0.,1.));
#124297=DIRECTION('ref_axis',(1.,0.,0.));
#124298=DIRECTION('',(1.,0.,0.));
#124299=DIRECTION('center_axis',(0.,0.,-1.));
#124300=DIRECTION('ref_axis',(0.,-1.,0.));
#124301=DIRECTION('',(-1.,0.,0.));
#124302=DIRECTION('center_axis',(-1.,0.,0.));
#124303=DIRECTION('ref_axis',(0.,0.,1.));
#124304=DIRECTION('',(-1.,0.,0.));
#124305=DIRECTION('center_axis',(-1.,0.,0.));
#124306=DIRECTION('ref_axis',(0.,0.,1.));
#124307=DIRECTION('',(-1.,0.,0.));
#124308=DIRECTION('center_axis',(-1.,0.,0.));
#124309=DIRECTION('ref_axis',(0.,0.,1.));
#124310=DIRECTION('',(0.,3.03450170724806E-16,1.));
#124311=DIRECTION('center_axis',(0.,-1.,3.03450170724806E-16));
#124312=DIRECTION('ref_axis',(-1.,0.,0.));
#124313=DIRECTION('center_axis',(0.,0.,-1.));
#124314=DIRECTION('ref_axis',(1.,0.,0.));
#124315=DIRECTION('center_axis',(1.,0.,0.));
#124316=DIRECTION('ref_axis',(0.,0.,1.));
#124317=DIRECTION('center_axis',(0.0436193873653361,0.,0.999048221581858));
#124318=DIRECTION('ref_axis',(-0.999048221581858,0.,0.0436193873653362));
#124319=DIRECTION('center_axis',(0.0436193873653361,0.,-0.999048221581858));
#124320=DIRECTION('ref_axis',(0.999048221581858,0.,0.0436193873653362));
#124321=DIRECTION('center_axis',(-1.,0.,0.));
#124322=DIRECTION('ref_axis',(0.,0.,1.));
#124323=DIRECTION('center_axis',(-1.,0.,0.));
#124324=DIRECTION('ref_axis',(0.,0.,1.));
#124325=DIRECTION('center_axis',(-1.,0.,0.));
#124326=DIRECTION('ref_axis',(0.,0.,1.));
#124327=DIRECTION('center_axis',(0.,-1.,0.));
#124328=DIRECTION('ref_axis',(0.,0.,-1.));
#124329=DIRECTION('center_axis',(-1.,0.,0.));
#124330=DIRECTION('ref_axis',(0.,0.,1.));
#124331=DIRECTION('center_axis',(-1.,0.,0.));
#124332=DIRECTION('ref_axis',(0.,0.,1.));
#124333=DIRECTION('center_axis',(0.,-1.,0.));
#124334=DIRECTION('ref_axis',(0.,0.,-1.));
#124335=DIRECTION('center_axis',(1.,0.,0.));
#124336=DIRECTION('ref_axis',(0.,0.,1.));
#124337=DIRECTION('center_axis',(1.,0.,0.));
#124338=DIRECTION('ref_axis',(0.,0.,1.));
#124339=DIRECTION('center_axis',(-1.,0.,0.));
#124340=DIRECTION('ref_axis',(0.,0.,1.));
#124341=DIRECTION('center_axis',(-1.,0.,0.));
#124342=DIRECTION('ref_axis',(0.,0.,1.));
#124343=DIRECTION('',(0.,1.,0.));
#124344=DIRECTION('center_axis',(-1.,0.,0.));
#124345=DIRECTION('ref_axis',(0.,0.,1.));
#124346=DIRECTION('',(0.,-1.,0.));
#124347=DIRECTION('center_axis',(-0.0436193873653361,0.,-0.999048221581858));
#124348=DIRECTION('ref_axis',(-0.999048221581858,0.,0.0436193873653361));
#124349=DIRECTION('',(-0.999048221581858,-8.07120802883996E-16,0.0436193873653362));
#124350=DIRECTION('',(-0.999048221581858,0.,0.0436193873653362));
#124351=DIRECTION('center_axis',(1.,0.,0.));
#124352=DIRECTION('ref_axis',(0.,0.,1.));
#124353=DIRECTION('',(-0.999048221581858,0.,-0.0436193873653362));
#124354=DIRECTION('center_axis',(-0.0436193873653361,0.,0.999048221581858));
#124355=DIRECTION('ref_axis',(0.,1.,0.));
#124356=DIRECTION('',(-0.999048221581858,0.,-0.0436193873653362));
#124357=DIRECTION('center_axis',(1.,0.,0.));
#124358=DIRECTION('ref_axis',(0.,0.,1.));
#124359=DIRECTION('center_axis',(-1.,0.,0.));
#124360=DIRECTION('ref_axis',(0.,0.,1.));
#124361=DIRECTION('center_axis',(-1.,0.,0.));
#124362=DIRECTION('ref_axis',(0.,0.,1.));
#124363=DIRECTION('center_axis',(1.,0.,0.));
#124364=DIRECTION('ref_axis',(0.,0.,-1.));
#124365=DIRECTION('center_axis',(-1.,0.,0.));
#124366=DIRECTION('ref_axis',(0.,0.,1.));
#124367=DIRECTION('',(-1.,0.,0.));
#124368=DIRECTION('center_axis',(1.,0.,0.));
#124369=DIRECTION('ref_axis',(0.,0.,-1.));
#124370=DIRECTION('',(-1.,0.,0.));
#124371=DIRECTION('center_axis',(-1.,0.,0.));
#124372=DIRECTION('ref_axis',(0.,0.,1.));
#124373=DIRECTION('center_axis',(-0.707106781186548,-0.707106781186548,
-8.73049632275228E-17));
#124374=DIRECTION('ref_axis',(0.707106781186548,-0.707106781186548,1.64082548650651E-34));
#124375=DIRECTION('center_axis',(0.707106781186548,0.707106781186548,0.));
#124376=DIRECTION('ref_axis',(-0.707106781186548,0.707106781186548,0.));
#124377=DIRECTION('',(-0.707106781186549,-0.707106781186546,-8.73049632275229E-17));
#124378=DIRECTION('',(0.707106781186549,0.707106781186546,8.73049632275229E-17));
#124379=DIRECTION('center_axis',(0.,-1.23467863058847E-16,1.));
#124380=DIRECTION('ref_axis',(0.,-1.,0.));
#124381=DIRECTION('center_axis',(1.,0.,-1.38777878078144E-14));
#124382=DIRECTION('ref_axis',(-1.38777878078144E-14,0.,-1.));
#124383=DIRECTION('center_axis',(-1.19942256323048E-29,1.16517322770923E-42,
-1.));
#124384=DIRECTION('ref_axis',(-9.71445146547011E-14,-1.,-7.96545955566226E-58));
#124385=DIRECTION('center_axis',(0.,0.,1.));
#124386=DIRECTION('ref_axis',(0.,-1.,0.));
#124387=DIRECTION('center_axis',(-1.,0.,-8.56730402307488E-31));
#124388=DIRECTION('ref_axis',(0.,-1.,0.));
#124389=DIRECTION('center_axis',(1.,0.,0.));
#124390=DIRECTION('ref_axis',(0.,0.,-1.));
#124391=DIRECTION('',(-1.,-6.93889390390722E-15,-8.56730402307488E-31));
#124392=DIRECTION('',(1.,6.93889390390722E-15,8.56730402307488E-31));
#124393=DIRECTION('center_axis',(0.,-1.23467863058847E-16,1.));
#124394=DIRECTION('ref_axis',(0.,-1.,0.));
#124395=DIRECTION('center_axis',(0.,-1.,0.));
#124396=DIRECTION('ref_axis',(0.,0.,-1.));
#124397=DIRECTION('center_axis',(0.,0.,-1.));
#124398=DIRECTION('ref_axis',(0.,-1.,0.));
#124399=DIRECTION('center_axis',(0.,0.,1.));
#124400=DIRECTION('ref_axis',(0.,-1.,0.));
#124401=DIRECTION('center_axis',(0.,1.,0.));
#124402=DIRECTION('ref_axis',(0.,0.,1.));
#124403=DIRECTION('',(0.,1.,1.23467863058847E-16));
#124404=DIRECTION('',(0.,-1.,-1.23467863058847E-16));
#124405=DIRECTION('center_axis',(0.,1.,0.));
#124406=DIRECTION('ref_axis',(0.,0.,1.));
#124407=DIRECTION('center_axis',(0.,-1.,0.));
#124408=DIRECTION('ref_axis',(0.,0.,-1.));
#124409=DIRECTION('',(0.,1.,1.23467863058847E-16));
#124410=DIRECTION('center_axis',(0.,-1.,0.));
#124411=DIRECTION('ref_axis',(0.,0.,1.));
#124412=DIRECTION('',(0.,-1.,-1.23467863058847E-16));
#124413=DIRECTION('center_axis',(0.,-1.23467863058847E-16,1.));
#124414=DIRECTION('ref_axis',(0.,-1.,0.));
#124415=DIRECTION('center_axis',(-1.,2.77555756156289E-14,0.));
#124416=DIRECTION('ref_axis',(-2.77555756156289E-14,-1.,0.));
#124417=DIRECTION('center_axis',(0.,0.,-1.));
#124418=DIRECTION('ref_axis',(0.,-1.,0.));
#124419=DIRECTION('center_axis',(0.,0.,1.));
#124420=DIRECTION('ref_axis',(0.,-1.,0.));
#124421=DIRECTION('center_axis',(1.,-2.77555756156289E-14,-3.42692160922995E-30));
#124422=DIRECTION('ref_axis',(2.77555756156289E-14,1.,-4.38683821655986E-59));
#124423=DIRECTION('center_axis',(-1.,2.77555756156289E-14,0.));
#124424=DIRECTION('ref_axis',(-2.77555756156289E-14,-1.,0.));
#124425=DIRECTION('',(1.,-2.77555756156289E-14,-3.42692160922995E-30));
#124426=DIRECTION('',(-1.,2.77555756156289E-14,3.42692160922995E-30));
#124427=DIRECTION('center_axis',(0.,-1.23467863058847E-16,1.));
#124428=DIRECTION('ref_axis',(0.,-1.,0.));
#124429=DIRECTION('center_axis',(-0.707106781186548,0.707106781186548,0.));
#124430=DIRECTION('ref_axis',(-0.707106781186548,-0.707106781186548,0.));
#124431=DIRECTION('center_axis',(0.,0.,-1.));
#124432=DIRECTION('ref_axis',(0.,-1.,0.));
#124433=DIRECTION('center_axis',(0.,0.,1.));
#124434=DIRECTION('ref_axis',(0.,-1.,0.));
#124435=DIRECTION('center_axis',(0.707106781186548,-0.707106781186548,-8.73049632275231E-17));
#124436=DIRECTION('ref_axis',(0.707106781186548,0.707106781186548,-4.20650685500144E-34));
#124437=DIRECTION('',(0.707106781186546,-0.707106781186549,-8.73049632275233E-17));
#124438=DIRECTION('',(-0.707106781186546,0.707106781186549,8.73049632275232E-17));
#124439=DIRECTION('center_axis',(0.,0.,-1.));
#124440=DIRECTION('ref_axis',(-1.,0.,0.));
#124441=DIRECTION('center_axis',(0.,0.,-1.));
#124442=DIRECTION('ref_axis',(-1.,0.,0.));
#124443=DIRECTION('',(1.03377769602066E-32,0.,1.));
#124444=DIRECTION('center_axis',(0.,0.,-1.));
#124445=DIRECTION('ref_axis',(0.,-1.,0.));
#124446=DIRECTION('',(-1.03377769602066E-32,-1.51929083932157E-64,-1.));
#124447=DIRECTION('center_axis',(0.,1.,0.));
#124448=DIRECTION('ref_axis',(0.,0.,1.));
#124449=DIRECTION('center_axis',(1.,0.,0.));
#124450=DIRECTION('ref_axis',(0.,0.,-1.));
#124451=DIRECTION('center_axis',(0.,-1.,0.));
#124452=DIRECTION('ref_axis',(0.,0.,1.));
#124453=DIRECTION('center_axis',(0.,1.,0.));
#124454=DIRECTION('ref_axis',(0.,0.,1.));
#124455=DIRECTION('center_axis',(1.,0.,0.));
#124456=DIRECTION('ref_axis',(0.,0.,-1.));
#124457=DIRECTION('center_axis',(1.,0.,0.));
#124458=DIRECTION('ref_axis',(0.,0.,-1.));
#124459=DIRECTION('',(-1.,0.,0.));
#124460=DIRECTION('',(1.,0.,0.));
#124461=DIRECTION('center_axis',(0.,-1.23467863058847E-16,1.));
#124462=DIRECTION('ref_axis',(0.,-1.,0.));
#124463=DIRECTION('center_axis',(0.139173100960066,0.99026806874157,0.));
#124464=DIRECTION('ref_axis',(-0.99026806874157,0.139173100960066,0.));
#124465=DIRECTION('center_axis',(0.,0.,1.));
#124466=DIRECTION('ref_axis',(0.,-1.,0.));
#124467=DIRECTION('center_axis',(0.,0.,-1.));
#124468=DIRECTION('ref_axis',(0.,-1.,0.));
#124469=DIRECTION('center_axis',(-0.139173100960066,-0.99026806874157,-1.22266282302934E-16));
#124470=DIRECTION('ref_axis',(0.99026806874157,-0.139173100960066,-1.22723965167578E-33));
#124471=DIRECTION('center_axis',(0.139173100960066,0.99026806874157,0.));
#124472=DIRECTION('ref_axis',(-0.99026806874157,0.139173100960066,0.));
#124473=DIRECTION('',(-0.139173100960065,-0.99026806874157,-1.22266282302933E-16));
#124474=DIRECTION('',(0.139173100960065,0.99026806874157,1.22266282302933E-16));
#124475=DIRECTION('center_axis',(0.,-1.23467863058847E-16,1.));
#124476=DIRECTION('ref_axis',(0.,-1.,0.));
#124477=DIRECTION('center_axis',(-1.,0.,0.));
#124478=DIRECTION('ref_axis',(0.,0.,1.));
#124479=DIRECTION('center_axis',(0.,0.,1.));
#124480=DIRECTION('ref_axis',(0.,-1.,0.));
#124481=DIRECTION('center_axis',(0.,0.,-1.));
#124482=DIRECTION('ref_axis',(0.,-1.,0.));
#124483=DIRECTION('center_axis',(-1.,0.,0.));
#124484=DIRECTION('ref_axis',(0.,0.,1.));
#124485=DIRECTION('center_axis',(-1.,0.,0.));
#124486=DIRECTION('ref_axis',(0.,0.,1.));
#124487=DIRECTION('',(1.,0.,0.));
#124488=DIRECTION('',(-1.,0.,0.));
#124489=DIRECTION('center_axis',(0.,-1.,0.));
#124490=DIRECTION('ref_axis',(0.,0.,-1.));
#124491=DIRECTION('center_axis',(0.,0.,1.));
#124492=DIRECTION('ref_axis',(1.,0.,0.));
#124493=DIRECTION('center_axis',(0.,1.,0.));
#124494=DIRECTION('ref_axis',(0.,0.,-1.));
#124495=DIRECTION('center_axis',(0.,-1.,0.));
#124496=DIRECTION('ref_axis',(0.,0.,-1.));
#124497=DIRECTION('center_axis',(0.,0.,1.));
#124498=DIRECTION('ref_axis',(1.,0.,0.));
#124499=DIRECTION('center_axis',(0.,0.,-1.));
#124500=DIRECTION('ref_axis',(0.,-1.,0.));
#124501=DIRECTION('',(-1.03377769602066E-32,0.,-1.));
#124502=DIRECTION('',(1.03377769602066E-32,1.51929083932157E-64,1.));
#124503=DIRECTION('center_axis',(1.3684555315672E-48,0.,1.));
#124504=DIRECTION('ref_axis',(0.,-1.,0.));
#124505=DIRECTION('center_axis',(0.,0.,-1.));
#124506=DIRECTION('ref_axis',(0.,-1.,0.));
#124507=DIRECTION('',(-1.3684555315672E-48,1.23467863058847E-16,-1.));
#124508=DIRECTION('center_axis',(0.,0.,-1.));
#124509=DIRECTION('ref_axis',(-1.,0.,0.));
#124510=DIRECTION('',(1.3684555315672E-48,-1.23467863058847E-16,1.));
#124511=DIRECTION('center_axis',(0.,1.,1.23467863058847E-16));
#124512=DIRECTION('ref_axis',(0.,0.,1.));
#124513=DIRECTION('center_axis',(1.,0.,0.));
#124514=DIRECTION('ref_axis',(0.,0.,-1.));
#124515=DIRECTION('center_axis',(0.,-1.,0.));
#124516=DIRECTION('ref_axis',(0.,0.,1.));
#124517=DIRECTION('center_axis',(0.,1.,0.));
#124518=DIRECTION('ref_axis',(0.,0.,1.));
#124519=DIRECTION('center_axis',(1.,0.,0.));
#124520=DIRECTION('ref_axis',(0.,0.,-1.));
#124521=DIRECTION('center_axis',(1.,0.,0.));
#124522=DIRECTION('ref_axis',(0.,0.,-1.));
#124523=DIRECTION('',(-1.,0.,0.));
#124524=DIRECTION('',(1.,0.,0.));
#124525=DIRECTION('center_axis',(0.,-1.23467863058847E-16,1.));
#124526=DIRECTION('ref_axis',(0.,-1.,0.));
#124527=DIRECTION('center_axis',(-0.707106781186548,0.707106781186548,0.));
#124528=DIRECTION('ref_axis',(-0.707106781186548,-0.707106781186548,0.));
#124529=DIRECTION('center_axis',(0.,0.,1.));
#124530=DIRECTION('ref_axis',(0.,-1.,0.));
#124531=DIRECTION('center_axis',(0.,0.,-1.));
#124532=DIRECTION('ref_axis',(0.,-1.,0.));
#124533=DIRECTION('center_axis',(-0.707106781186548,0.707106781186548,8.73049632275231E-17));
#124534=DIRECTION('ref_axis',(-0.707106781186548,-0.707106781186548,8.65064369663437E-31));
#124535=DIRECTION('',(0.707106781186546,-0.707106781186549,-8.73049632275232E-17));
#124536=DIRECTION('',(-0.707106781186546,0.707106781186549,8.73049632275232E-17));
#124537=DIRECTION('center_axis',(0.,0.,-1.));
#124538=DIRECTION('ref_axis',(-1.,0.,0.));
#124539=DIRECTION('center_axis',(0.,0.,-1.));
#124540=DIRECTION('ref_axis',(-1.,0.,0.));
#124541=DIRECTION('',(1.03377769602066E-32,0.,1.));
#124542=DIRECTION('center_axis',(0.,0.,-1.));
#124543=DIRECTION('ref_axis',(0.,-1.,0.));
#124544=DIRECTION('',(-1.03377769602066E-32,-1.51929083932157E-64,-1.));
#124545=DIRECTION('center_axis',(0.,1.,0.));
#124546=DIRECTION('ref_axis',(0.,0.,1.));
#124547=DIRECTION('center_axis',(1.,0.,0.));
#124548=DIRECTION('ref_axis',(0.,0.,-1.));
#124549=DIRECTION('center_axis',(0.,-1.,0.));
#124550=DIRECTION('ref_axis',(0.,0.,1.));
#124551=DIRECTION('center_axis',(0.,1.,0.));
#124552=DIRECTION('ref_axis',(0.,0.,1.));
#124553=DIRECTION('center_axis',(1.,0.,0.));
#124554=DIRECTION('ref_axis',(0.,0.,-1.));
#124555=DIRECTION('center_axis',(1.,0.,0.));
#124556=DIRECTION('ref_axis',(0.,0.,-1.));
#124557=DIRECTION('',(-1.,0.,0.));
#124558=DIRECTION('',(1.,0.,0.));
#124559=DIRECTION('center_axis',(0.,-1.23467863058847E-16,1.));
#124560=DIRECTION('ref_axis',(0.,-1.,0.));
#124561=DIRECTION('center_axis',(0.272177601648339,0.962247033334454,0.));
#124562=DIRECTION('ref_axis',(-0.962247033334454,0.272177601648339,0.));
#124563=DIRECTION('center_axis',(0.,0.,1.));
#124564=DIRECTION('ref_axis',(0.,-1.,0.));
#124565=DIRECTION('center_axis',(0.,0.,-1.));
#124566=DIRECTION('ref_axis',(0.,-1.,0.));
#124567=DIRECTION('center_axis',(0.,-1.23467863058847E-16,1.));
#124568=DIRECTION('ref_axis',(0.,-1.,0.));
#124569=DIRECTION('center_axis',(0.139173100960066,0.99026806874157,0.));
#124570=DIRECTION('ref_axis',(-0.99026806874157,0.139173100960066,0.));
#124571=DIRECTION('center_axis',(0.,0.,1.));
#124572=DIRECTION('ref_axis',(0.,-1.,0.));
#124573=DIRECTION('center_axis',(0.,0.,-1.));
#124574=DIRECTION('ref_axis',(0.,-1.,0.));
#124575=DIRECTION('center_axis',(-0.139173100960066,-0.99026806874157,-1.22266282302934E-16));
#124576=DIRECTION('ref_axis',(0.99026806874157,-0.139173100960066,-1.22723965167578E-33));
#124577=DIRECTION('center_axis',(0.139173100960066,0.99026806874157,0.));
#124578=DIRECTION('ref_axis',(-0.99026806874157,0.139173100960066,0.));
#124579=DIRECTION('',(-0.139173100960065,-0.99026806874157,-1.22266282302933E-16));
#124580=DIRECTION('',(0.139173100960065,0.99026806874157,1.22266282302933E-16));
#124581=DIRECTION('center_axis',(0.,-1.23467863058847E-16,1.));
#124582=DIRECTION('ref_axis',(0.,-1.,0.));
#124583=DIRECTION('center_axis',(-1.,0.,0.));
#124584=DIRECTION('ref_axis',(0.,0.,1.));
#124585=DIRECTION('center_axis',(0.,0.,1.));
#124586=DIRECTION('ref_axis',(0.,-1.,0.));
#124587=DIRECTION('center_axis',(0.,0.,-1.));
#124588=DIRECTION('ref_axis',(0.,-1.,0.));
#124589=DIRECTION('center_axis',(-1.,0.,0.));
#124590=DIRECTION('ref_axis',(0.,0.,1.));
#124591=DIRECTION('center_axis',(-1.,0.,0.));
#124592=DIRECTION('ref_axis',(0.,0.,1.));
#124593=DIRECTION('',(1.,0.,0.));
#124594=DIRECTION('',(-1.,0.,0.));
#124595=DIRECTION('center_axis',(0.,-1.,0.));
#124596=DIRECTION('ref_axis',(0.,0.,-1.));
#124597=DIRECTION('center_axis',(0.,0.,1.));
#124598=DIRECTION('ref_axis',(1.,0.,0.));
#124599=DIRECTION('center_axis',(0.,1.,0.));
#124600=DIRECTION('ref_axis',(0.,0.,-1.));
#124601=DIRECTION('center_axis',(0.,-1.,0.));
#124602=DIRECTION('ref_axis',(0.,0.,-1.));
#124603=DIRECTION('center_axis',(0.,0.,1.));
#124604=DIRECTION('ref_axis',(1.,0.,0.));
#124605=DIRECTION('center_axis',(0.,0.,-1.));
#124606=DIRECTION('ref_axis',(0.,-1.,0.));
#124607=DIRECTION('',(-1.03377769602066E-32,0.,-1.));
#124608=DIRECTION('',(1.03377769602066E-32,1.51929083932157E-64,1.));
#124609=DIRECTION('center_axis',(0.,-2.74330011127376E-48,-1.));
#124610=DIRECTION('ref_axis',(-1.,0.,0.));
#124611=DIRECTION('center_axis',(0.,0.,-1.));
#124612=DIRECTION('ref_axis',(-1.,0.,0.));
#124613=DIRECTION('',(1.03377769602066E-32,2.74330011127376E-48,1.));
#124614=DIRECTION('center_axis',(0.,0.,-1.));
#124615=DIRECTION('ref_axis',(0.,-1.,0.));
#124616=DIRECTION('',(-1.03377769602066E-32,-2.74330011127376E-48,-1.));
#124617=DIRECTION('center_axis',(-2.65366540778891E-16,1.,0.));
#124618=DIRECTION('ref_axis',(-1.,0.,0.));
#124619=DIRECTION('center_axis',(1.,0.,0.));
#124620=DIRECTION('ref_axis',(0.,0.,-1.));
#124621=DIRECTION('center_axis',(0.,-1.,0.));
#124622=DIRECTION('ref_axis',(-1.,0.,0.));
#124623=DIRECTION('center_axis',(0.,1.,0.));
#124624=DIRECTION('ref_axis',(-1.,0.,0.));
#124625=DIRECTION('center_axis',(1.,0.,3.27642397172882E-32));
#124626=DIRECTION('ref_axis',(0.,1.,0.));
#124627=DIRECTION('center_axis',(1.,0.,0.));
#124628=DIRECTION('ref_axis',(0.,0.,-1.));
#124629=DIRECTION('',(-1.,-2.65366540778891E-16,-3.27642397172882E-32));
#124630=DIRECTION('',(1.,2.65366540778891E-16,3.27642397172882E-32));
#124631=DIRECTION('center_axis',(0.,-1.23467863058847E-16,1.));
#124632=DIRECTION('ref_axis',(0.,-1.,0.));
#124633=DIRECTION('center_axis',(0.299364406779191,0.954138853602421,0.));
#124634=DIRECTION('ref_axis',(-0.954138853602421,0.299364406779191,0.));
#124635=DIRECTION('center_axis',(0.,0.,1.));
#124636=DIRECTION('ref_axis',(0.,-1.,0.));
#124637=DIRECTION('center_axis',(0.,0.,-1.));
#124638=DIRECTION('ref_axis',(0.,-1.,0.));
#124639=DIRECTION('center_axis',(0.,-1.23467863058847E-16,1.));
#124640=DIRECTION('ref_axis',(0.,-1.,0.));
#124641=DIRECTION('center_axis',(0.395127118643591,0.918626452978801,0.));
#124642=DIRECTION('ref_axis',(-0.918626452978801,0.395127118643591,0.));
#124643=DIRECTION('center_axis',(-2.74153728738396E-30,6.08743563864414E-44,
-1.));
#124644=DIRECTION('ref_axis',(-2.22044604925031E-14,-1.,9.95682444457782E-59));
#124645=DIRECTION('center_axis',(0.,0.,1.));
#124646=DIRECTION('ref_axis',(0.,-1.,0.));
#124647=DIRECTION('center_axis',(0.,-1.23467863058847E-16,1.));
#124648=DIRECTION('ref_axis',(0.,-1.,0.));
#124649=DIRECTION('center_axis',(-1.,0.,0.));
#124650=DIRECTION('ref_axis',(0.,0.,1.));
#124651=DIRECTION('center_axis',(0.,0.,1.));
#124652=DIRECTION('ref_axis',(0.,-1.,0.));
#124653=DIRECTION('center_axis',(0.,0.,-1.));
#124654=DIRECTION('ref_axis',(0.,-1.,0.));
#124655=DIRECTION('center_axis',(-1.,0.,0.));
#124656=DIRECTION('ref_axis',(0.,0.,1.));
#124657=DIRECTION('center_axis',(-1.,0.,0.));
#124658=DIRECTION('ref_axis',(0.,0.,1.));
#124659=DIRECTION('',(1.,0.,0.));
#124660=DIRECTION('',(-1.,0.,0.));
#124661=DIRECTION('center_axis',(0.,-1.,0.));
#124662=DIRECTION('ref_axis',(0.,0.,-1.));
#124663=DIRECTION('center_axis',(0.,0.,1.));
#124664=DIRECTION('ref_axis',(1.,0.,0.));
#124665=DIRECTION('center_axis',(0.,1.,0.));
#124666=DIRECTION('ref_axis',(0.,0.,-1.));
#124667=DIRECTION('center_axis',(0.,-1.,0.));
#124668=DIRECTION('ref_axis',(0.,0.,-1.));
#124669=DIRECTION('center_axis',(0.,0.,1.));
#124670=DIRECTION('ref_axis',(1.,0.,0.));
#124671=DIRECTION('center_axis',(0.,0.,-1.));
#124672=DIRECTION('ref_axis',(0.,-1.,0.));
#124673=DIRECTION('',(-1.03377769602066E-32,0.,-1.));
#124674=DIRECTION('',(1.03377769602066E-32,1.51929083932157E-64,1.));
#124675=DIRECTION('center_axis',(0.,0.,-1.));
#124676=DIRECTION('ref_axis',(-1.,0.,0.));
#124677=DIRECTION('center_axis',(0.,0.,-1.));
#124678=DIRECTION('ref_axis',(-1.,0.,0.));
#124679=DIRECTION('',(1.03377769602066E-32,0.,1.));
#124680=DIRECTION('center_axis',(0.,0.,-1.));
#124681=DIRECTION('ref_axis',(0.,-1.,0.));
#124682=DIRECTION('',(-1.03377769602066E-32,-1.51929083932157E-64,-1.));
#124683=DIRECTION('center_axis',(0.,1.,0.));
#124684=DIRECTION('ref_axis',(0.,0.,1.));
#124685=DIRECTION('center_axis',(1.,0.,0.));
#124686=DIRECTION('ref_axis',(0.,0.,-1.));
#124687=DIRECTION('center_axis',(0.,-1.,0.));
#124688=DIRECTION('ref_axis',(0.,0.,1.));
#124689=DIRECTION('center_axis',(0.,1.,0.));
#124690=DIRECTION('ref_axis',(0.,0.,1.));
#124691=DIRECTION('center_axis',(1.,0.,0.));
#124692=DIRECTION('ref_axis',(0.,0.,-1.));
#124693=DIRECTION('center_axis',(1.,0.,0.));
#124694=DIRECTION('ref_axis',(0.,0.,-1.));
#124695=DIRECTION('',(-1.,0.,0.));
#124696=DIRECTION('',(1.,0.,0.));
#124697=DIRECTION('center_axis',(0.,-1.23467863058847E-16,1.));
#124698=DIRECTION('ref_axis',(0.,-1.,0.));
#124699=DIRECTION('center_axis',(0.161228813558844,0.986917053089269,0.));
#124700=DIRECTION('ref_axis',(-0.986917053089269,0.161228813558844,0.));
#124701=DIRECTION('center_axis',(0.,0.,1.));
#124702=DIRECTION('ref_axis',(0.,-1.,0.));
#124703=DIRECTION('center_axis',(8.56730402307488E-31,5.94476136586342E-45,
-1.));
#124704=DIRECTION('ref_axis',(6.93889390390722E-15,-1.,-9.95682444457783E-60));
#124705=DIRECTION('center_axis',(0.,-1.23467863058847E-16,1.));
#124706=DIRECTION('ref_axis',(0.,-1.,0.));
#124707=DIRECTION('center_axis',(0.256991525423251,0.966413656702258,0.));
#124708=DIRECTION('ref_axis',(-0.966413656702259,0.256991525423251,0.));
#124709=DIRECTION('center_axis',(-4.16713667682363E-30,1.40644112995234E-43,
-1.));
#124710=DIRECTION('ref_axis',(-3.37507799486048E-14,-1.,3.98272977783113E-59));
#124711=DIRECTION('center_axis',(0.,0.,1.));
#124712=DIRECTION('ref_axis',(0.,-1.,0.));
#124713=DIRECTION('center_axis',(0.,-1.23467863058847E-16,1.));
#124714=DIRECTION('ref_axis',(0.,-1.,0.));
#124715=DIRECTION('center_axis',(-1.,0.,0.));
#124716=DIRECTION('ref_axis',(0.,0.,1.));
#124717=DIRECTION('center_axis',(0.,0.,1.));
#124718=DIRECTION('ref_axis',(0.,-1.,0.));
#124719=DIRECTION('center_axis',(0.,0.,-1.));
#124720=DIRECTION('ref_axis',(0.,-1.,0.));
#124721=DIRECTION('center_axis',(-1.,0.,-3.39012271766808E-32));
#124722=DIRECTION('ref_axis',(0.,-1.,0.));
#124723=DIRECTION('center_axis',(-1.,0.,0.));
#124724=DIRECTION('ref_axis',(0.,0.,1.));
#124725=DIRECTION('',(1.,2.74575313258015E-16,3.39012271766808E-32));
#124726=DIRECTION('',(-1.,-2.74575313258015E-16,-3.39012271766808E-32));
#124727=DIRECTION('center_axis',(2.74575313258015E-16,-1.,0.));
#124728=DIRECTION('ref_axis',(1.,0.,0.));
#124729=DIRECTION('center_axis',(0.,0.,1.));
#124730=DIRECTION('ref_axis',(1.,0.,0.));
#124731=DIRECTION('center_axis',(0.,1.,0.));
#124732=DIRECTION('ref_axis',(1.,0.,0.));
#124733=DIRECTION('center_axis',(0.,-1.,0.));
#124734=DIRECTION('ref_axis',(1.,0.,0.));
#124735=DIRECTION('center_axis',(0.,2.83849834724024E-48,1.));
#124736=DIRECTION('ref_axis',(1.,0.,0.));
#124737=DIRECTION('center_axis',(0.,0.,-1.));
#124738=DIRECTION('ref_axis',(0.,-1.,0.));
#124739=DIRECTION('',(-1.03377769602066E-32,-2.83849834724023E-48,-1.));
#124740=DIRECTION('',(1.03377769602066E-32,2.83849834724023E-48,1.));
#124741=DIRECTION('center_axis',(0.,0.,-1.));
#124742=DIRECTION('ref_axis',(-1.,0.,0.));
#124743=DIRECTION('center_axis',(0.,0.,-1.));
#124744=DIRECTION('ref_axis',(-1.,0.,0.));
#124745=DIRECTION('',(1.03377769602066E-32,0.,1.));
#124746=DIRECTION('center_axis',(0.,0.,-1.));
#124747=DIRECTION('ref_axis',(0.,-1.,0.));
#124748=DIRECTION('',(-1.03377769602066E-32,-1.51929083932157E-64,-1.));
#124749=DIRECTION('center_axis',(0.,1.,0.));
#124750=DIRECTION('ref_axis',(0.,0.,1.));
#124751=DIRECTION('center_axis',(1.,0.,0.));
#124752=DIRECTION('ref_axis',(0.,0.,-1.));
#124753=DIRECTION('center_axis',(0.,-1.,0.));
#124754=DIRECTION('ref_axis',(0.,0.,1.));
#124755=DIRECTION('center_axis',(0.,1.,0.));
#124756=DIRECTION('ref_axis',(0.,0.,1.));
#124757=DIRECTION('center_axis',(1.,0.,0.));
#124758=DIRECTION('ref_axis',(0.,0.,-1.));
#124759=DIRECTION('center_axis',(1.,0.,0.));
#124760=DIRECTION('ref_axis',(0.,0.,-1.));
#124761=DIRECTION('',(-1.,0.,0.));
#124762=DIRECTION('',(1.,0.,0.));
#124763=DIRECTION('center_axis',(0.,-1.23467863058847E-16,1.));
#124764=DIRECTION('ref_axis',(0.,-1.,0.));
#124765=DIRECTION('center_axis',(0.0230932203385063,0.999733316027028,0.));
#124766=DIRECTION('ref_axis',(-0.999733316027028,0.0230932203385063,0.));
#124767=DIRECTION('center_axis',(0.,0.,1.));
#124768=DIRECTION('ref_axis',(0.,-1.,0.));
#124769=DIRECTION('center_axis',(0.,0.,-1.));
#124770=DIRECTION('ref_axis',(0.,-1.,0.));
#124771=DIRECTION('center_axis',(0.,-1.23467863058847E-16,1.));
#124772=DIRECTION('ref_axis',(0.,-1.,0.));
#124773=DIRECTION('center_axis',(0.118855932202914,0.99291151034731,0.));
#124774=DIRECTION('ref_axis',(-0.99291151034731,0.118855932202914,0.));
#124775=DIRECTION('center_axis',(-1.3159378979443E-30,1.40254517114361E-44,
-1.));
#124776=DIRECTION('ref_axis',(-1.06581410364015E-14,-1.,-2.48920611114446E-60));
#124777=DIRECTION('center_axis',(0.,0.,1.));
#124778=DIRECTION('ref_axis',(0.,-1.,0.));
#124779=DIRECTION('center_axis',(0.,-1.23467863058847E-16,1.));
#124780=DIRECTION('ref_axis',(0.,-1.,0.));
#124781=DIRECTION('center_axis',(-1.,0.,0.));
#124782=DIRECTION('ref_axis',(0.,0.,1.));
#124783=DIRECTION('center_axis',(0.,0.,1.));
#124784=DIRECTION('ref_axis',(0.,-1.,0.));
#124785=DIRECTION('center_axis',(0.,0.,-1.));
#124786=DIRECTION('ref_axis',(0.,-1.,0.));
#124787=DIRECTION('center_axis',(-1.,0.,0.));
#124788=DIRECTION('ref_axis',(0.,0.,1.));
#124789=DIRECTION('center_axis',(-1.,0.,0.));
#124790=DIRECTION('ref_axis',(0.,0.,1.));
#124791=DIRECTION('',(1.,0.,0.));
#124792=DIRECTION('',(-1.,0.,0.));
#124793=DIRECTION('center_axis',(0.,-1.,0.));
#124794=DIRECTION('ref_axis',(0.,0.,-1.));
#124795=DIRECTION('center_axis',(0.,0.,1.));
#124796=DIRECTION('ref_axis',(1.,0.,0.));
#124797=DIRECTION('center_axis',(0.,1.,0.));
#124798=DIRECTION('ref_axis',(0.,0.,-1.));
#124799=DIRECTION('center_axis',(0.,-1.,0.));
#124800=DIRECTION('ref_axis',(0.,0.,-1.));
#124801=DIRECTION('center_axis',(0.,0.,1.));
#124802=DIRECTION('ref_axis',(1.,0.,0.));
#124803=DIRECTION('center_axis',(0.,0.,-1.));
#124804=DIRECTION('ref_axis',(0.,-1.,0.));
#124805=DIRECTION('',(-1.03377769602066E-32,0.,-1.));
#124806=DIRECTION('',(1.03377769602066E-32,1.51929083932157E-64,1.));
#124807=DIRECTION('center_axis',(0.,-1.63688369328374E-48,-1.));
#124808=DIRECTION('ref_axis',(-1.,0.,0.));
#124809=DIRECTION('center_axis',(0.,0.,-1.));
#124810=DIRECTION('ref_axis',(-1.,0.,0.));
#124811=DIRECTION('',(1.03377769602066E-32,1.63688369328374E-48,1.));
#124812=DIRECTION('center_axis',(0.,0.,-1.));
#124813=DIRECTION('ref_axis',(0.,-1.,0.));
#124814=DIRECTION('',(-1.03377769602066E-32,-1.63688369328374E-48,-1.));
#124815=DIRECTION('center_axis',(-1.58340008648341E-16,1.,0.));
#124816=DIRECTION('ref_axis',(-1.,0.,0.));
#124817=DIRECTION('center_axis',(1.,0.,0.));
#124818=DIRECTION('ref_axis',(0.,0.,-1.));
#124819=DIRECTION('center_axis',(0.,-1.,0.));
#124820=DIRECTION('ref_axis',(-1.,0.,0.));
#124821=DIRECTION('center_axis',(-2.89120579329468E-16,1.,0.));
#124822=DIRECTION('ref_axis',(-1.,-2.89120579329468E-16,0.));
#124823=DIRECTION('center_axis',(1.,0.,1.95499025045301E-32));
#124824=DIRECTION('ref_axis',(0.,1.,0.));
#124825=DIRECTION('center_axis',(1.,0.,0.));
#124826=DIRECTION('ref_axis',(0.,0.,-1.));
#124827=DIRECTION('',(-1.,-1.58340008648341E-16,-1.95499025045301E-32));
#124828=DIRECTION('',(1.,1.58340008648341E-16,1.95499025045301E-32));
#124829=DIRECTION('center_axis',(0.,-1.23467863058847E-16,1.));
#124830=DIRECTION('ref_axis',(0.,-1.,0.));
#124831=DIRECTION('center_axis',(-0.115042372881831,0.993360585307127,0.));
#124832=DIRECTION('ref_axis',(-0.993360585307127,-0.115042372881831,0.));
#124833=DIRECTION('center_axis',(0.,0.,1.));
#124834=DIRECTION('ref_axis',(0.,-1.,0.));
#124835=DIRECTION('center_axis',(0.,0.,-1.));
#124836=DIRECTION('ref_axis',(0.,-1.,0.));
#124837=DIRECTION('center_axis',(0.,-1.23467863058847E-16,1.));
#124838=DIRECTION('ref_axis',(0.,-1.,0.));
#124839=DIRECTION('center_axis',(-0.0192796610174253,0.99981413006171,0.));
#124840=DIRECTION('ref_axis',(-0.99981413006171,-0.0192796610174253,0.));
#124841=DIRECTION('center_axis',(0.,0.,-1.));
#124842=DIRECTION('ref_axis',(0.,-1.,0.));
#124843=DIRECTION('center_axis',(0.,0.,1.));
#124844=DIRECTION('ref_axis',(0.,-1.,0.));
#124845=DIRECTION('center_axis',(0.,-1.23467863058847E-16,1.));
#124846=DIRECTION('ref_axis',(0.,-1.,0.));
#124847=DIRECTION('center_axis',(-1.,0.,0.));
#124848=DIRECTION('ref_axis',(0.,0.,1.));
#124849=DIRECTION('center_axis',(0.,0.,1.));
#124850=DIRECTION('ref_axis',(0.,-1.,0.));
#124851=DIRECTION('center_axis',(0.,0.,-1.));
#124852=DIRECTION('ref_axis',(0.,-1.,0.));
#124853=DIRECTION('center_axis',(-1.,0.,0.));
#124854=DIRECTION('ref_axis',(0.,0.,1.));
#124855=DIRECTION('center_axis',(-1.,0.,0.));
#124856=DIRECTION('ref_axis',(0.,0.,1.));
#124857=DIRECTION('',(1.,0.,0.));
#124858=DIRECTION('',(-1.,0.,0.));
#124859=DIRECTION('center_axis',(0.,-1.,0.));
#124860=DIRECTION('ref_axis',(0.,0.,-1.));
#124861=DIRECTION('center_axis',(0.,0.,1.));
#124862=DIRECTION('ref_axis',(1.,0.,0.));
#124863=DIRECTION('center_axis',(0.,1.,0.));
#124864=DIRECTION('ref_axis',(0.,0.,-1.));
#124865=DIRECTION('center_axis',(0.,-1.,0.));
#124866=DIRECTION('ref_axis',(0.,0.,-1.));
#124867=DIRECTION('center_axis',(0.,0.,1.));
#124868=DIRECTION('ref_axis',(1.,0.,0.));
#124869=DIRECTION('center_axis',(0.,0.,-1.));
#124870=DIRECTION('ref_axis',(0.,-1.,0.));
#124871=DIRECTION('',(-1.03377769602066E-32,0.,-1.));
#124872=DIRECTION('',(1.03377769602066E-32,1.51929083932157E-64,1.));
#124873=DIRECTION('center_axis',(0.,0.,-1.));
#124874=DIRECTION('ref_axis',(-1.,0.,0.));
#124875=DIRECTION('center_axis',(0.,0.,-1.));
#124876=DIRECTION('ref_axis',(-1.,0.,0.));
#124877=DIRECTION('',(1.03377769602066E-32,0.,1.));
#124878=DIRECTION('center_axis',(0.,0.,-1.));
#124879=DIRECTION('ref_axis',(0.,-1.,0.));
#124880=DIRECTION('',(-1.03377769602066E-32,-1.51929083932157E-64,-1.));
#124881=DIRECTION('center_axis',(0.,1.,0.));
#124882=DIRECTION('ref_axis',(0.,0.,1.));
#124883=DIRECTION('center_axis',(1.,0.,0.));
#124884=DIRECTION('ref_axis',(0.,0.,-1.));
#124885=DIRECTION('center_axis',(0.,-1.,0.));
#124886=DIRECTION('ref_axis',(0.,0.,1.));
#124887=DIRECTION('center_axis',(0.,1.,0.));
#124888=DIRECTION('ref_axis',(0.,0.,1.));
#124889=DIRECTION('center_axis',(1.,0.,0.));
#124890=DIRECTION('ref_axis',(0.,0.,-1.));
#124891=DIRECTION('center_axis',(1.,0.,0.));
#124892=DIRECTION('ref_axis',(0.,0.,-1.));
#124893=DIRECTION('',(-1.,0.,0.));
#124894=DIRECTION('',(1.,0.,0.));
#124895=DIRECTION('center_axis',(0.,-1.23467863058847E-16,1.));
#124896=DIRECTION('ref_axis',(0.,-1.,0.));
#124897=DIRECTION('center_axis',(-0.25317796610217,0.967419721465491,0.));
#124898=DIRECTION('ref_axis',(-0.967419721465491,-0.25317796610217,0.));
#124899=DIRECTION('center_axis',(0.,0.,1.));
#124900=DIRECTION('ref_axis',(0.,-1.,0.));
#124901=DIRECTION('center_axis',(0.,0.,-1.));
#124902=DIRECTION('ref_axis',(0.,-1.,0.));
#124903=DIRECTION('center_axis',(0.,-1.23467863058847E-16,1.));
#124904=DIRECTION('ref_axis',(0.,-1.,0.));
#124905=DIRECTION('center_axis',(-0.157415254237766,0.98753249958331,0.));
#124906=DIRECTION('ref_axis',(-0.98753249958331,-0.157415254237765,0.));
#124907=DIRECTION('center_axis',(-3.72849071084219E-30,1.12593209572362E-43,
-1.));
#124908=DIRECTION('ref_axis',(-3.01980662698043E-14,-1.,1.99136488891557E-59));
#124909=DIRECTION('center_axis',(0.,0.,1.));
#124910=DIRECTION('ref_axis',(0.,-1.,0.));
#124911=DIRECTION('center_axis',(0.,-1.23467863058847E-16,1.));
#124912=DIRECTION('ref_axis',(0.,-1.,0.));
#124913=DIRECTION('center_axis',(-1.,0.,0.));
#124914=DIRECTION('ref_axis',(0.,0.,1.));
#124915=DIRECTION('center_axis',(0.,0.,1.));
#124916=DIRECTION('ref_axis',(0.,-1.,0.));
#124917=DIRECTION('center_axis',(0.,0.,-1.));
#124918=DIRECTION('ref_axis',(0.,-1.,0.));
#124919=DIRECTION('center_axis',(-1.,0.,0.));
#124920=DIRECTION('ref_axis',(0.,0.,1.));
#124921=DIRECTION('center_axis',(-1.,0.,0.));
#124922=DIRECTION('ref_axis',(0.,0.,1.));
#124923=DIRECTION('',(1.,0.,0.));
#124924=DIRECTION('',(-1.,0.,0.));
#124925=DIRECTION('center_axis',(0.,-1.,0.));
#124926=DIRECTION('ref_axis',(0.,0.,-1.));
#124927=DIRECTION('center_axis',(0.,0.,1.));
#124928=DIRECTION('ref_axis',(1.,0.,0.));
#124929=DIRECTION('center_axis',(0.,1.,0.));
#124930=DIRECTION('ref_axis',(0.,0.,-1.));
#124931=DIRECTION('center_axis',(0.,-1.,0.));
#124932=DIRECTION('ref_axis',(0.,0.,-1.));
#124933=DIRECTION('center_axis',(0.,0.,1.));
#124934=DIRECTION('ref_axis',(1.,0.,0.));
#124935=DIRECTION('center_axis',(0.,0.,-1.));
#124936=DIRECTION('ref_axis',(0.,-1.,0.));
#124937=DIRECTION('',(-1.03377769602066E-32,0.,-1.));
#124938=DIRECTION('',(1.03377769602066E-32,0.,1.));
#124939=DIRECTION('center_axis',(0.,1.15951658690774E-48,-1.));
#124940=DIRECTION('ref_axis',(-1.,0.,0.));
#124941=DIRECTION('center_axis',(0.,0.,-1.));
#124942=DIRECTION('ref_axis',(-1.,0.,0.));
#124943=DIRECTION('',(1.03377769602066E-32,-1.15951658690774E-48,1.));
#124944=DIRECTION('center_axis',(0.,0.,-1.));
#124945=DIRECTION('ref_axis',(0.,-1.,0.));
#124946=DIRECTION('',(-1.03377769602066E-32,1.15951658690774E-48,-1.));
#124947=DIRECTION('center_axis',(1.12163049306547E-16,1.,0.));
#124948=DIRECTION('ref_axis',(-1.,0.,0.));
#124949=DIRECTION('center_axis',(1.,0.,0.));
#124950=DIRECTION('ref_axis',(0.,0.,-1.));
#124951=DIRECTION('center_axis',(0.,-1.,0.));
#124952=DIRECTION('ref_axis',(-1.,0.,0.));
#124953=DIRECTION('center_axis',(0.,1.,0.));
#124954=DIRECTION('ref_axis',(-1.,0.,0.));
#124955=DIRECTION('center_axis',(1.,0.,-1.38485320120435E-32));
#124956=DIRECTION('ref_axis',(0.,1.,0.));
#124957=DIRECTION('center_axis',(1.,0.,0.));
#124958=DIRECTION('ref_axis',(0.,0.,-1.));
#124959=DIRECTION('',(-1.,1.12163049306547E-16,1.38485320120435E-32));
#124960=DIRECTION('',(1.,-1.12163049306547E-16,-1.38485320120435E-32));
#124961=DIRECTION('center_axis',(0.,-1.23467863058847E-16,1.));
#124962=DIRECTION('ref_axis',(0.,-1.,0.));
#124963=DIRECTION('center_axis',(-0.391313559322503,0.920257408712559,0.));
#124964=DIRECTION('ref_axis',(-0.920257408712559,-0.391313559322503,0.));
#124965=DIRECTION('center_axis',(0.,0.,1.));
#124966=DIRECTION('ref_axis',(0.,-1.,0.));
#124967=DIRECTION('center_axis',(0.,0.,-1.));
#124968=DIRECTION('ref_axis',(0.,-1.,0.));
#124969=DIRECTION('center_axis',(0.,-1.23467863058847E-16,1.));
#124970=DIRECTION('ref_axis',(0.,-1.,0.));
#124971=DIRECTION('center_axis',(-0.295550847458105,0.955327010278049,0.));
#124972=DIRECTION('ref_axis',(-0.955327010278049,-0.295550847458105,0.));
#124973=DIRECTION('center_axis',(2.30289132140253E-30,4.29529458662731E-44,
-1.));
#124974=DIRECTION('ref_axis',(1.86517468137027E-14,-1.,3.48488855560224E-59));
#124975=DIRECTION('center_axis',(0.,0.,1.));
#124976=DIRECTION('ref_axis',(0.,-1.,0.));
#124977=DIRECTION('center_axis',(0.,-1.23467863058847E-16,1.));
#124978=DIRECTION('ref_axis',(0.,-1.,0.));
#124979=DIRECTION('center_axis',(-1.,0.,0.));
#124980=DIRECTION('ref_axis',(0.,0.,1.));
#124981=DIRECTION('center_axis',(0.,0.,1.));
#124982=DIRECTION('ref_axis',(0.,-1.,0.));
#124983=DIRECTION('center_axis',(0.,0.,-1.));
#124984=DIRECTION('ref_axis',(0.,-1.,0.));
#124985=DIRECTION('center_axis',(-1.,0.,1.64684708935465E-32));
#124986=DIRECTION('ref_axis',(0.,-1.,0.));
#124987=DIRECTION('center_axis',(-1.,0.,0.));
#124988=DIRECTION('ref_axis',(0.,0.,1.));
#124989=DIRECTION('',(1.,-1.33382651044161E-16,-1.64684708935465E-32));
#124990=DIRECTION('',(-1.,1.33382651044161E-16,1.64684708935465E-32));
#124991=DIRECTION('center_axis',(-1.33382651044161E-16,-1.,0.));
#124992=DIRECTION('ref_axis',(1.,-1.48029736616688E-16,0.));
#124993=DIRECTION('center_axis',(0.,0.,1.));
#124994=DIRECTION('ref_axis',(1.,0.,0.));
#124995=DIRECTION('center_axis',(0.,1.,0.));
#124996=DIRECTION('ref_axis',(1.,0.,0.));
#124997=DIRECTION('center_axis',(-1.44560289664734E-16,-1.,0.));
#124998=DIRECTION('ref_axis',(1.,-1.44560289664734E-16,0.));
#124999=DIRECTION('center_axis',(0.,-1.37888009685561E-48,1.));
#125000=DIRECTION('ref_axis',(1.,0.,0.));
#125001=DIRECTION('center_axis',(0.,0.,-1.));
#125002=DIRECTION('ref_axis',(0.,-1.,0.));
#125003=DIRECTION('',(-1.03377769602066E-32,1.37888009685561E-48,-1.));
#125004=DIRECTION('',(1.03377769602066E-32,-1.37888009685561E-48,1.));
#125005=DIRECTION('center_axis',(0.,0.,-1.));
#125006=DIRECTION('ref_axis',(-1.,0.,0.));
#125007=DIRECTION('center_axis',(0.,0.,-1.));
#125008=DIRECTION('ref_axis',(-1.,0.,0.));
#125009=DIRECTION('',(1.03377769602066E-32,0.,1.));
#125010=DIRECTION('center_axis',(0.,0.,-1.));
#125011=DIRECTION('ref_axis',(0.,-1.,0.));
#125012=DIRECTION('',(-1.03377769602066E-32,-1.51929083932157E-64,-1.));
#125013=DIRECTION('center_axis',(0.,1.,0.));
#125014=DIRECTION('ref_axis',(0.,0.,1.));
#125015=DIRECTION('center_axis',(1.,0.,0.));
#125016=DIRECTION('ref_axis',(0.,0.,-1.));
#125017=DIRECTION('center_axis',(0.,-1.,0.));
#125018=DIRECTION('ref_axis',(0.,0.,1.));
#125019=DIRECTION('center_axis',(0.,1.,0.));
#125020=DIRECTION('ref_axis',(0.,0.,1.));
#125021=DIRECTION('center_axis',(1.,0.,0.));
#125022=DIRECTION('ref_axis',(0.,0.,-1.));
#125023=DIRECTION('center_axis',(1.,0.,0.));
#125024=DIRECTION('ref_axis',(0.,0.,-1.));
#125025=DIRECTION('',(-1.,0.,0.));
#125026=DIRECTION('',(1.,0.,0.));
#125027=DIRECTION('center_axis',(0.,-1.23467863058847E-16,1.));
#125028=DIRECTION('ref_axis',(0.,-1.,0.));
#125029=DIRECTION('center_axis',(-0.139173100960066,0.99026806874157,0.));
#125030=DIRECTION('ref_axis',(-0.99026806874157,-0.139173100960066,0.));
#125031=DIRECTION('center_axis',(0.,0.,1.));
#125032=DIRECTION('ref_axis',(0.,-1.,0.));
#125033=DIRECTION('center_axis',(0.,0.,-1.));
#125034=DIRECTION('ref_axis',(0.,-1.,0.));
#125035=DIRECTION('center_axis',(0.139173100960066,-0.99026806874157,-1.22266282302933E-16));
#125036=DIRECTION('ref_axis',(0.99026806874157,0.139173100960066,9.57340194962255E-34));
#125037=DIRECTION('center_axis',(-0.139173100960066,0.99026806874157,0.));
#125038=DIRECTION('ref_axis',(-0.99026806874157,-0.139173100960066,0.));
#125039=DIRECTION('',(0.139173100960067,-0.99026806874157,-1.22266282302933E-16));
#125040=DIRECTION('',(-0.139173100960067,0.99026806874157,1.22266282302933E-16));
#125041=DIRECTION('center_axis',(0.,-1.23467863058847E-16,1.));
#125042=DIRECTION('ref_axis',(0.,-1.,0.));
#125043=DIRECTION('center_axis',(-0.322177601635812,0.94667924504776,0.));
#125044=DIRECTION('ref_axis',(-0.94667924504776,-0.322177601635812,0.));
#125045=DIRECTION('center_axis',(0.,0.,1.));
#125046=DIRECTION('ref_axis',(0.,-1.,0.));
#125047=DIRECTION('center_axis',(6.23076656223628E-31,3.14433659020876E-45,
-1.));
#125048=DIRECTION('ref_axis',(5.04646829375071E-15,-1.,-4.3561106945028E-60));
#125049=DIRECTION('center_axis',(0.,-1.23467863058847E-16,1.));
#125050=DIRECTION('ref_axis',(0.,-1.,0.));
#125051=DIRECTION('center_axis',(-1.,0.,0.));
#125052=DIRECTION('ref_axis',(0.,0.,1.));
#125053=DIRECTION('center_axis',(0.,0.,1.));
#125054=DIRECTION('ref_axis',(0.,-1.,0.));
#125055=DIRECTION('center_axis',(0.,0.,-1.));
#125056=DIRECTION('ref_axis',(0.,-1.,0.));
#125057=DIRECTION('center_axis',(-1.,0.,0.));
#125058=DIRECTION('ref_axis',(0.,0.,1.));
#125059=DIRECTION('center_axis',(-1.,0.,0.));
#125060=DIRECTION('ref_axis',(0.,0.,1.));
#125061=DIRECTION('',(1.,0.,0.));
#125062=DIRECTION('',(-1.,0.,0.));
#125063=DIRECTION('center_axis',(0.,-1.,0.));
#125064=DIRECTION('ref_axis',(0.,0.,-1.));
#125065=DIRECTION('center_axis',(0.,0.,1.));
#125066=DIRECTION('ref_axis',(1.,0.,0.));
#125067=DIRECTION('center_axis',(0.,1.,0.));
#125068=DIRECTION('ref_axis',(0.,0.,-1.));
#125069=DIRECTION('center_axis',(0.,-1.,0.));
#125070=DIRECTION('ref_axis',(0.,0.,-1.));
#125071=DIRECTION('center_axis',(0.,0.,1.));
#125072=DIRECTION('ref_axis',(1.,0.,0.));
#125073=DIRECTION('center_axis',(0.,0.,-1.));
#125074=DIRECTION('ref_axis',(0.,-1.,0.));
#125075=DIRECTION('',(-1.03377769602066E-32,0.,-1.));
#125076=DIRECTION('',(1.03377769602066E-32,1.51929083932157E-64,1.));
#125077=DIRECTION('center_axis',(0.,0.,-1.));
#125078=DIRECTION('ref_axis',(-1.,0.,0.));
#125079=DIRECTION('center_axis',(0.,0.,-1.));
#125080=DIRECTION('ref_axis',(-1.,0.,0.));
#125081=DIRECTION('',(1.03377769602066E-32,0.,1.));
#125082=DIRECTION('center_axis',(0.,0.,-1.));
#125083=DIRECTION('ref_axis',(0.,-1.,0.));
#125084=DIRECTION('',(-1.03377769602066E-32,-1.51929083932157E-64,-1.));
#125085=DIRECTION('center_axis',(0.,1.,0.));
#125086=DIRECTION('ref_axis',(0.,0.,1.));
#125087=DIRECTION('center_axis',(1.,0.,0.));
#125088=DIRECTION('ref_axis',(0.,0.,-1.));
#125089=DIRECTION('center_axis',(0.,-1.,0.));
#125090=DIRECTION('ref_axis',(0.,0.,1.));
#125091=DIRECTION('center_axis',(0.,1.,0.));
#125092=DIRECTION('ref_axis',(0.,0.,1.));
#125093=DIRECTION('center_axis',(1.,0.,0.));
#125094=DIRECTION('ref_axis',(0.,0.,-1.));
#125095=DIRECTION('center_axis',(1.,0.,0.));
#125096=DIRECTION('ref_axis',(0.,0.,-1.));
#125097=DIRECTION('',(-1.,0.,0.));
#125098=DIRECTION('',(1.,0.,0.));
#125099=DIRECTION('center_axis',(0.,-1.23467863058847E-16,1.));
#125100=DIRECTION('ref_axis',(0.,-1.,0.));
#125101=DIRECTION('center_axis',(-0.139173100960066,0.99026806874157,0.));
#125102=DIRECTION('ref_axis',(-0.99026806874157,-0.139173100960066,0.));
#125103=DIRECTION('center_axis',(0.,0.,1.));
#125104=DIRECTION('ref_axis',(0.,-1.,0.));
#125105=DIRECTION('center_axis',(0.,0.,-1.));
#125106=DIRECTION('ref_axis',(0.,-1.,0.));
#125107=DIRECTION('center_axis',(0.139173100960066,-0.99026806874157,-1.22266282302933E-16));
#125108=DIRECTION('ref_axis',(0.99026806874157,0.139173100960066,9.57340194962255E-34));
#125109=DIRECTION('center_axis',(-0.139173100960066,0.99026806874157,0.));
#125110=DIRECTION('ref_axis',(-0.99026806874157,-0.139173100960066,0.));
#125111=DIRECTION('',(0.139173100960067,-0.99026806874157,-1.22266282302933E-16));
#125112=DIRECTION('',(-0.139173100960067,0.99026806874157,1.22266282302933E-16));
#125113=DIRECTION('center_axis',(0.,-1.23467863058847E-16,1.));
#125114=DIRECTION('ref_axis',(0.,-1.,0.));
#125115=DIRECTION('center_axis',(-1.,0.,0.));
#125116=DIRECTION('ref_axis',(0.,0.,1.));
#125117=DIRECTION('center_axis',(0.,0.,1.));
#125118=DIRECTION('ref_axis',(0.,-1.,0.));
#125119=DIRECTION('center_axis',(0.,0.,-1.));
#125120=DIRECTION('ref_axis',(0.,-1.,0.));
#125121=DIRECTION('center_axis',(-1.,0.,-2.45282604044407E-32));
#125122=DIRECTION('ref_axis',(0.,-1.,0.));
#125123=DIRECTION('center_axis',(-1.,0.,0.));
#125124=DIRECTION('ref_axis',(0.,0.,1.));
#125125=DIRECTION('',(1.,1.98661091208406E-16,2.45282604044407E-32));
#125126=DIRECTION('',(-1.,-1.98661091208406E-16,-2.45282604044407E-32));
#125127=DIRECTION('center_axis',(1.98661091208406E-16,-1.,0.));
#125128=DIRECTION('ref_axis',(1.,0.,0.));
#125129=DIRECTION('center_axis',(0.,0.,1.));
#125130=DIRECTION('ref_axis',(1.,0.,0.));
#125131=DIRECTION('center_axis',(0.,1.,0.));
#125132=DIRECTION('ref_axis',(1.,0.,0.));
#125133=DIRECTION('center_axis',(0.,-1.,0.));
#125134=DIRECTION('ref_axis',(1.,0.,0.));
#125135=DIRECTION('center_axis',(0.,2.05371405158377E-48,1.));
#125136=DIRECTION('ref_axis',(1.,0.,0.));
#125137=DIRECTION('center_axis',(0.,0.,-1.));
#125138=DIRECTION('ref_axis',(0.,-1.,0.));
#125139=DIRECTION('',(-1.03377769602066E-32,-2.05371405158378E-48,-1.));
#125140=DIRECTION('',(1.03377769602066E-32,2.05371405158377E-48,1.));
#125141=DIRECTION('center_axis',(0.707106781186548,0.707106781186548,8.73049632275229E-17));
#125142=DIRECTION('ref_axis',(-0.707106781186548,0.707106781186548,3.00811589707026E-33));
#125143=DIRECTION('',(0.707106781186548,0.707106781186547,8.7304963227523E-17));
#125144=DIRECTION('center_axis',(0.707106781186537,0.707106781186558,0.));
#125145=DIRECTION('ref_axis',(-0.707106781186558,0.707106781186537,0.));
#125146=DIRECTION('',(-0.707106781186548,-0.707106781186547,-8.7304963227523E-17));
#125147=DIRECTION('center_axis',(0.,-1.23467863058847E-16,1.));
#125148=DIRECTION('ref_axis',(0.,-1.,0.));
#125149=DIRECTION('center_axis',(-1.,0.,0.));
#125150=DIRECTION('ref_axis',(0.,0.,1.));
#125151=DIRECTION('center_axis',(0.,0.,1.));
#125152=DIRECTION('ref_axis',(0.,-1.,0.));
#125153=DIRECTION('center_axis',(0.,0.,-1.));
#125154=DIRECTION('ref_axis',(0.,-1.,0.));
#125155=DIRECTION('center_axis',(-1.,0.,0.));
#125156=DIRECTION('ref_axis',(0.,0.,1.));
#125157=DIRECTION('center_axis',(-1.,0.,0.));
#125158=DIRECTION('ref_axis',(0.,0.,1.));
#125159=DIRECTION('',(1.,0.,0.));
#125160=DIRECTION('',(-1.,0.,0.));
#125161=DIRECTION('center_axis',(0.,-1.,-1.23467863058847E-16));
#125162=DIRECTION('ref_axis',(0.,0.,-1.));
#125163=DIRECTION('center_axis',(0.,0.,1.));
#125164=DIRECTION('ref_axis',(1.,0.,0.));
#125165=DIRECTION('center_axis',(0.,1.,0.));
#125166=DIRECTION('ref_axis',(0.,0.,-1.));
#125167=DIRECTION('center_axis',(0.,-1.,0.));
#125168=DIRECTION('ref_axis',(0.,0.,-1.));
#125169=DIRECTION('center_axis',(1.3684555315672E-48,0.,1.));
#125170=DIRECTION('ref_axis',(0.,-1.,0.));
#125171=DIRECTION('center_axis',(0.,0.,-1.));
#125172=DIRECTION('ref_axis',(0.,-1.,0.));
#125173=DIRECTION('',(-1.3684555315672E-48,1.23467863058847E-16,-1.));
#125174=DIRECTION('',(1.3684555315672E-48,-1.23467863058847E-16,1.));
#125175=DIRECTION('center_axis',(1.74315279842105E-32,0.,-1.));
#125176=DIRECTION('ref_axis',(0.,1.,0.));
#125177=DIRECTION('',(1.74315279842105E-32,1.23467863058847E-16,-1.));
#125178=DIRECTION('',(-2.46519032881566E-32,-1.23467863058847E-16,1.));
#125179=DIRECTION('center_axis',(0.,0.,1.));
#125180=DIRECTION('ref_axis',(0.,-1.,0.));
#125181=DIRECTION('center_axis',(0.,0.,-1.));
#125182=DIRECTION('ref_axis',(0.,1.,0.));
#125183=DIRECTION('',(3.61018765197304E-33,1.23467863058847E-16,-1.));
#125184=DIRECTION('',(0.,-1.23467863058847E-16,1.));
#125185=DIRECTION('center_axis',(0.,0.,1.));
#125186=DIRECTION('ref_axis',(0.,-1.,0.));
#125187=DIRECTION('center_axis',(-5.10557634013221E-33,0.,-1.));
#125188=DIRECTION('ref_axis',(0.,1.,0.));
#125189=DIRECTION('',(-8.71576399210524E-33,1.23467863058847E-16,-1.));
#125190=DIRECTION('',(5.10557634013221E-33,-1.23467863058847E-16,1.));
#125191=DIRECTION('center_axis',(0.,0.,1.));
#125192=DIRECTION('ref_axis',(0.,-1.,0.));
#125193=DIRECTION('center_axis',(-1.74315279842107E-32,0.,-1.));
#125194=DIRECTION('ref_axis',(0.,1.,0.));
#125195=DIRECTION('',(-1.74315279842107E-32,1.23467863058847E-16,-1.));
#125196=DIRECTION('',(2.46519032881566E-32,-1.23467863058847E-16,1.));
#125197=DIRECTION('center_axis',(0.,0.,1.));
#125198=DIRECTION('ref_axis',(0.,-1.,0.));
#125199=DIRECTION('center_axis',(0.,0.,-1.));
#125200=DIRECTION('ref_axis',(0.,1.,0.));
#125201=DIRECTION('',(0.,1.23467863058847E-16,-1.));
#125202=DIRECTION('',(0.,-1.23467863058847E-16,1.));
#125203=DIRECTION('center_axis',(0.,0.,1.));
#125204=DIRECTION('ref_axis',(0.,-1.,0.));
#125205=DIRECTION('center_axis',(0.,0.,1.));
#125206=DIRECTION('ref_axis',(-0.754709580222749,0.656059028990534,0.));
#125207=DIRECTION('',(1.73522765332111E-17,0.,-1.));
#125208=DIRECTION('',(-1.73522765332111E-17,-7.66623374189429E-34,1.));
#125209=DIRECTION('center_axis',(0.,0.,1.));
#125210=DIRECTION('ref_axis',(0.,-1.,0.));
#125211=DIRECTION('center_axis',(0.,0.,1.));
#125212=DIRECTION('ref_axis',(-0.754709580222751,0.656059028990531,0.));
#125213=DIRECTION('',(1.73522765332111E-17,0.,-1.));
#125214=DIRECTION('',(-1.73522765332111E-17,-7.66623374189429E-34,1.));
#125215=DIRECTION('center_axis',(0.,0.,1.));
#125216=DIRECTION('ref_axis',(0.,-1.,0.));
#125217=DIRECTION('center_axis',(0.,0.,1.));
#125218=DIRECTION('ref_axis',(0.,-1.,0.));
#125219=DIRECTION('',(-1.38485320120435E-32,1.55329357889012E-48,-1.));
#125220=DIRECTION('',(0.,-1.23467863058847E-16,1.));
#125221=DIRECTION('center_axis',(0.,0.,1.));
#125222=DIRECTION('ref_axis',(0.,-1.,0.));
#125223=DIRECTION('center_axis',(0.,0.,1.));
#125224=DIRECTION('ref_axis',(0.,-1.,0.));
#125225=DIRECTION('',(0.,0.,-1.));
#125226=DIRECTION('',(0.,-1.23467863058847E-16,1.));
#125227=DIRECTION('center_axis',(0.,0.,1.));
#125228=DIRECTION('ref_axis',(0.,-1.,0.));
#125229=DIRECTION('center_axis',(0.,0.,1.));
#125230=DIRECTION('ref_axis',(0.,-1.,0.));
#125231=DIRECTION('',(1.95499025045301E-32,3.09553173164152E-48,-1.));
#125232=DIRECTION('',(0.,-1.23467863058847E-16,1.));
#125233=DIRECTION('center_axis',(0.,0.,1.));
#125234=DIRECTION('ref_axis',(0.,-1.,0.));
#125235=DIRECTION('center_axis',(0.,0.,1.));
#125236=DIRECTION('ref_axis',(0.,-1.,0.));
#125237=DIRECTION('',(0.,0.,-1.));
#125238=DIRECTION('',(0.,-1.23467863058847E-16,1.));
#125239=DIRECTION('center_axis',(0.,0.,1.));
#125240=DIRECTION('ref_axis',(0.,-1.,0.));
#125241=DIRECTION('center_axis',(0.,0.,1.));
#125242=DIRECTION('ref_axis',(0.,-1.,0.));
#125243=DIRECTION('',(0.,1.23467863058847E-16,-1.));
#125244=DIRECTION('',(0.,0.,1.));
#125245=DIRECTION('center_axis',(0.,0.,1.));
#125246=DIRECTION('ref_axis',(0.,-1.,0.));
#125247=DIRECTION('center_axis',(0.,0.,1.));
#125248=DIRECTION('ref_axis',(0.,-1.,0.));
#125249=DIRECTION('',(0.,1.23467863058847E-16,-1.));
#125250=DIRECTION('',(0.,0.,1.));
#125251=DIRECTION('center_axis',(0.,0.,1.));
#125252=DIRECTION('ref_axis',(0.,-1.,0.));
#125253=DIRECTION('center_axis',(0.,0.,1.));
#125254=DIRECTION('ref_axis',(0.,-1.,0.));
#125255=DIRECTION('',(0.,1.23467863058847E-16,-1.));
#125256=DIRECTION('',(1.64684708935465E-32,-2.19660830642484E-48,1.));
#125257=DIRECTION('center_axis',(0.,0.,1.));
#125258=DIRECTION('ref_axis',(0.,-1.,0.));
#125259=DIRECTION('center_axis',(0.,0.,1.));
#125260=DIRECTION('ref_axis',(0.,-1.,0.));
#125261=DIRECTION('',(0.,1.23467863058847E-16,-1.));
#125262=DIRECTION('',(0.,0.,1.));
#125263=DIRECTION('center_axis',(0.,0.,1.));
#125264=DIRECTION('ref_axis',(0.,-1.,0.));
#125265=DIRECTION('center_axis',(0.,-3.44722219103775E-33,1.));
#125266=DIRECTION('ref_axis',(1.,0.,0.));
#125267=DIRECTION('',(1.73522765332111E-17,4.28072011692203E-33,-1.));
#125268=DIRECTION('',(-1.73522765332111E-17,-3.44722219103775E-33,1.));
#125269=DIRECTION('center_axis',(0.,0.,1.));
#125270=DIRECTION('ref_axis',(0.,-1.,0.));
#125271=DIRECTION('center_axis',(0.,0.,1.));
#125272=DIRECTION('ref_axis',(0.,-1.,0.));
#125273=DIRECTION('',(0.,1.23467863058847E-16,-1.));
#125274=DIRECTION('',(0.,0.,1.));
#125275=DIRECTION('center_axis',(0.,0.,1.));
#125276=DIRECTION('ref_axis',(0.,-1.,0.));
#125277=DIRECTION('center_axis',(0.,0.,1.));
#125278=DIRECTION('ref_axis',(0.,-1.,0.));
#125279=DIRECTION('',(0.,0.,-1.));
#125280=DIRECTION('',(0.,-1.23467863058847E-16,1.));
#125281=DIRECTION('center_axis',(0.,0.,1.));
#125282=DIRECTION('ref_axis',(0.,-1.,0.));
#125283=DIRECTION('center_axis',(0.,0.,1.));
#125284=DIRECTION('ref_axis',(0.,-1.,0.));
#125285=DIRECTION('',(0.,1.23467863058847E-16,-1.));
#125286=DIRECTION('',(-3.39012271766808E-32,-9.30844007186829E-48,1.));
#125287=DIRECTION('center_axis',(0.,0.,1.));
#125288=DIRECTION('ref_axis',(0.,-1.,0.));
#125289=DIRECTION('center_axis',(0.,0.,1.));
#125290=DIRECTION('ref_axis',(0.,-1.,0.));
#125291=DIRECTION('',(3.27642397172882E-32,8.69453295502712E-48,-1.));
#125292=DIRECTION('',(0.,-1.23467863058847E-16,1.));
#125293=DIRECTION('center_axis',(0.,0.,1.));
#125294=DIRECTION('ref_axis',(0.,-1.,0.));
#125295=DIRECTION('center_axis',(0.,0.,1.));
#125296=DIRECTION('ref_axis',(0.,-1.,0.));
#125297=DIRECTION('',(0.,0.,-1.));
#125298=DIRECTION('',(0.,-1.23467863058847E-16,1.));
#125299=DIRECTION('center_axis',(0.,0.,1.));
#125300=DIRECTION('ref_axis',(0.,-1.,0.));
#125301=DIRECTION('center_axis',(0.,0.,1.));
#125302=DIRECTION('ref_axis',(0.,-1.,0.));
#125303=DIRECTION('',(0.,1.23467863058847E-16,-1.));
#125304=DIRECTION('',(0.,0.,1.));
#125305=DIRECTION('center_axis',(0.,0.,1.));
#125306=DIRECTION('ref_axis',(0.,-1.,0.));
#125307=DIRECTION('center_axis',(0.,-4.33074883140017E-34,1.));
#125308=DIRECTION('ref_axis',(-0.754709580222784,-0.656059028990493,-2.84122687313011E-34));
#125309=DIRECTION('',(-1.73522765332109E-17,0.,-1.));
#125310=DIRECTION('',(1.73522765332109E-17,0.,1.));
#125311=DIRECTION('center_axis',(0.,0.,1.));
#125312=DIRECTION('ref_axis',(0.,-1.,0.));
#125313=DIRECTION('center_axis',(0.,-1.72738015942773E-49,1.));
#125314=DIRECTION('ref_axis',(1.,0.,0.));
#125315=DIRECTION('',(-1.73522765332109E-17,0.,-1.));
#125316=DIRECTION('',(1.73522765332109E-17,3.85185988877447E-34,1.));
#125317=DIRECTION('center_axis',(0.,0.,1.));
#125318=DIRECTION('ref_axis',(0.,-1.,0.));
#125319=DIRECTION('center_axis',(0.,-4.33074883140017E-34,1.));
#125320=DIRECTION('ref_axis',(-0.754709580222761,-0.656059028990519,-2.84122687313022E-34));
#125321=DIRECTION('',(-1.73522765332109E-17,0.,-1.));
#125322=DIRECTION('',(1.73522765332109E-17,0.,1.));
#125323=DIRECTION('center_axis',(0.,0.,1.));
#125324=DIRECTION('ref_axis',(0.,-1.,0.));
#125325=DIRECTION('center_axis',(0.,0.,-1.));
#125326=DIRECTION('ref_axis',(0.,1.,0.));
#125327=DIRECTION('',(0.,1.23467863058847E-16,-1.));
#125328=DIRECTION('',(0.,-1.23467863058847E-16,1.));
#125329=DIRECTION('center_axis',(0.,0.,1.));
#125330=DIRECTION('ref_axis',(0.,-1.,0.));
#125331=DIRECTION('center_axis',(0.,-1.23467863058847E-16,1.));
#125332=DIRECTION('ref_axis',(0.,-1.,-1.23467863058847E-16));
#125333=DIRECTION('center_axis',(0.,0.,-1.));
#125334=DIRECTION('ref_axis',(0.,-1.,0.));
#125335=DIRECTION('center_axis',(0.,1.19636298170419E-16,-1.));
#125336=DIRECTION('ref_axis',(0.,1.,1.19636298170419E-16));
#125337=DIRECTION('',(1.23138919323476E-16,1.,0.));
#125338=DIRECTION('',(-1.,0.,0.));
#125339=DIRECTION('center_axis',(0.,0.,-1.));
#125340=DIRECTION('ref_axis',(0.,-1.,0.));
#125341=DIRECTION('',(8.37284837049414E-17,1.,1.23467863058847E-16));
#125342=DIRECTION('',(8.37284837049414E-17,1.,1.23467863058847E-16));
#125343=DIRECTION('',(8.37284837049414E-17,1.,1.23467863058847E-16));
#125344=DIRECTION('',(8.37284837049414E-17,1.,1.23467863058847E-16));
#125345=DIRECTION('',(8.37284837049414E-17,1.,1.23467863058847E-16));
#125346=DIRECTION('',(8.37284837049414E-17,1.,1.23467863058847E-16));
#125347=DIRECTION('',(8.37284837049414E-17,1.,1.23467863058847E-16));
#125348=DIRECTION('',(8.37284837049414E-17,1.,1.23467863058847E-16));
#125349=DIRECTION('',(8.37284837049414E-17,1.,1.23467863058847E-16));
#125350=DIRECTION('',(8.37284837049414E-17,1.,1.23467863058847E-16));
#125351=DIRECTION('',(8.37284837049414E-17,1.,1.23467863058847E-16));
#125352=DIRECTION('center_axis',(0.,1.,1.23467863058847E-16));
#125353=DIRECTION('ref_axis',(0.,1.23467863058847E-16,-1.));
#125354=DIRECTION('',(-1.,0.,0.));
#125355=DIRECTION('center_axis',(0.,-1.19636298170419E-16,1.));
#125356=DIRECTION('ref_axis',(0.,-1.,-1.19636298170419E-16));
#125357=DIRECTION('',(0.,-1.23467863058847E-16,1.));
#125358=DIRECTION('center_axis',(0.,1.19636298170419E-16,-1.));
#125359=DIRECTION('ref_axis',(0.,1.,1.19636298170419E-16));
#125360=DIRECTION('',(0.,-1.23467863058847E-16,1.));
#125361=DIRECTION('center_axis',(-1.,0.,0.));
#125362=DIRECTION('ref_axis',(0.,0.,1.));
#125363=DIRECTION('',(0.,-1.,0.));
#125364=DIRECTION('center_axis',(2.77555756156289E-14,1.,1.23467863058847E-16));
#125365=DIRECTION('ref_axis',(1.,-2.77555756156289E-14,0.));
#125366=DIRECTION('',(-1.,2.77555756156289E-14,0.));
#125367=DIRECTION('center_axis',(-1.,0.,0.));
#125368=DIRECTION('ref_axis',(0.,0.,1.));
#125369=DIRECTION('',(0.,-1.23467863058847E-16,1.));
#125370=DIRECTION('',(0.,-1.,0.));
#125371=DIRECTION('center_axis',(0.,-1.,0.));
#125372=DIRECTION('ref_axis',(0.,0.,-1.));
#125373=DIRECTION('',(1.,0.,0.));
#125374=DIRECTION('center_axis',(0.,1.,0.));
#125375=DIRECTION('ref_axis',(1.,0.,0.));
#125376=DIRECTION('',(-1.,0.,0.));
#125377=DIRECTION('center_axis',(0.,-1.,0.));
#125378=DIRECTION('ref_axis',(0.,0.,-1.));
#125379=DIRECTION('',(1.,0.,0.));
#125380=DIRECTION('center_axis',(0.,1.,0.));
#125381=DIRECTION('ref_axis',(1.,0.,0.));
#125382=DIRECTION('',(-1.,0.,0.));
#125383=DIRECTION('center_axis',(-1.33382651044161E-16,-1.,0.));
#125384=DIRECTION('ref_axis',(-1.,1.33382651044161E-16,0.));
#125385=DIRECTION('',(1.,-1.33382651044161E-16,-1.64684708935465E-32));
#125386=DIRECTION('center_axis',(1.12163049306547E-16,1.,0.));
#125387=DIRECTION('ref_axis',(1.,-1.12163049306547E-16,0.));
#125388=DIRECTION('',(-1.,1.12163049306547E-16,1.38485320120435E-32));
#125389=DIRECTION('center_axis',(0.,1.,0.));
#125390=DIRECTION('ref_axis',(1.,0.,0.));
#125391=DIRECTION('',(-1.,0.,0.));
#125392=DIRECTION('center_axis',(0.,-1.,0.));
#125393=DIRECTION('ref_axis',(0.,0.,-1.));
#125394=DIRECTION('',(1.,0.,0.));
#125395=DIRECTION('center_axis',(0.,-1.,0.));
#125396=DIRECTION('ref_axis',(0.,0.,-1.));
#125397=DIRECTION('',(1.,0.,0.));
#125398=DIRECTION('center_axis',(-1.58340008648341E-16,1.,0.));
#125399=DIRECTION('ref_axis',(1.,1.58340008648341E-16,0.));
#125400=DIRECTION('',(-1.,-1.58340008648341E-16,-1.95499025045301E-32));
#125401=DIRECTION('center_axis',(-1.,8.37284837049414E-17,1.03377769602066E-32));
#125402=DIRECTION('ref_axis',(1.03377769602066E-32,0.,1.));
#125403=DIRECTION('',(-8.37284837049414E-17,-1.,0.));
#125404=DIRECTION('',(-8.37284837049414E-17,-1.,-1.23467863058847E-16));
#125405=DIRECTION('center_axis',(8.37284837049414E-17,1.,0.));
#125406=DIRECTION('ref_axis',(0.,0.,1.));
#125407=DIRECTION('center_axis',(0.,0.,1.));
#125408=DIRECTION('ref_axis',(0.,-1.,0.));
#125409=DIRECTION('center_axis',(0.,0.,-1.));
#125410=DIRECTION('ref_axis',(0.,-1.,0.));
#125411=DIRECTION('center_axis',(0.,-1.,0.));
#125412=DIRECTION('ref_axis',(0.,0.,-1.));
#125413=DIRECTION('',(1.,0.,0.));
#125414=DIRECTION('center_axis',(0.,1.,0.));
#125415=DIRECTION('ref_axis',(1.,0.,0.));
#125416=DIRECTION('',(-1.,0.,0.));
#125417=DIRECTION('center_axis',(-1.,8.37284837049414E-17,1.03377769602066E-32));
#125418=DIRECTION('ref_axis',(1.03377769602066E-32,0.,1.));
#125419=DIRECTION('',(-8.37284837049414E-17,-1.,0.));
#125420=DIRECTION('',(-8.37284837049414E-17,-1.,-1.23467863058847E-16));
#125421=DIRECTION('center_axis',(8.37284837049414E-17,1.,0.));
#125422=DIRECTION('ref_axis',(0.,0.,1.));
#125423=DIRECTION('center_axis',(0.,0.,1.));
#125424=DIRECTION('ref_axis',(0.,-1.,0.));
#125425=DIRECTION('center_axis',(-1.3159378979443E-30,1.40254517114361E-44,
-1.));
#125426=DIRECTION('ref_axis',(-1.06581410364015E-14,-1.,-2.48920611114446E-60));
#125427=DIRECTION('center_axis',(2.74575313258015E-16,-1.,0.));
#125428=DIRECTION('ref_axis',(0.,0.,-1.));
#125429=DIRECTION('',(1.,2.74575313258015E-16,3.39012271766808E-32));
#125430=DIRECTION('center_axis',(0.,1.,0.));
#125431=DIRECTION('ref_axis',(1.,0.,0.));
#125432=DIRECTION('',(-1.,0.,0.));
#125433=DIRECTION('center_axis',(-1.,8.37284837049414E-17,1.03377769602066E-32));
#125434=DIRECTION('ref_axis',(1.03377769602066E-32,0.,1.));
#125435=DIRECTION('',(-8.37284837049414E-17,-1.,0.));
#125436=DIRECTION('',(-8.37284837049414E-17,-1.,-1.23467863058847E-16));
#125437=DIRECTION('center_axis',(8.37284837049414E-17,1.,0.));
#125438=DIRECTION('ref_axis',(0.,0.,1.));
#125439=DIRECTION('center_axis',(0.,0.,1.));
#125440=DIRECTION('ref_axis',(0.,-1.,0.));
#125441=DIRECTION('center_axis',(-4.16713667682363E-30,1.40644112995234E-43,
-1.));
#125442=DIRECTION('ref_axis',(-3.37507799486048E-14,-1.,7.96545955566226E-59));
#125443=DIRECTION('center_axis',(0.,-1.,0.));
#125444=DIRECTION('ref_axis',(0.,0.,-1.));
#125445=DIRECTION('',(1.,0.,0.));
#125446=DIRECTION('center_axis',(-2.65366540778891E-16,1.,0.));
#125447=DIRECTION('ref_axis',(1.,2.65366540778891E-16,0.));
#125448=DIRECTION('',(-1.,-2.65366540778891E-16,-3.27642397172882E-32));
#125449=DIRECTION('center_axis',(-1.,8.37284837049414E-17,1.03377769602066E-32));
#125450=DIRECTION('ref_axis',(1.03377769602066E-32,0.,1.));
#125451=DIRECTION('',(-8.37284837049414E-17,-1.,0.));
#125452=DIRECTION('',(-8.37284837049414E-17,-1.,-1.23467863058847E-16));
#125453=DIRECTION('center_axis',(8.37284837049414E-17,1.,0.));
#125454=DIRECTION('ref_axis',(0.,0.,1.));
#125455=DIRECTION('center_axis',(0.,0.,1.));
#125456=DIRECTION('ref_axis',(0.,-1.,0.));
#125457=DIRECTION('center_axis',(-2.74153728738396E-30,6.08743563864414E-44,
-1.));
#125458=DIRECTION('ref_axis',(-2.22044604925031E-14,-1.,9.95682444457782E-59));
#125459=DIRECTION('center_axis',(1.98661091208406E-16,-1.,0.));
#125460=DIRECTION('ref_axis',(0.,0.,-1.));
#125461=DIRECTION('',(1.,1.98661091208406E-16,2.45282604044407E-32));
#125462=DIRECTION('center_axis',(0.,1.,0.));
#125463=DIRECTION('ref_axis',(1.,0.,0.));
#125464=DIRECTION('',(-1.,0.,0.));
#125465=DIRECTION('center_axis',(-1.,8.37284837049414E-17,1.03377769602066E-32));
#125466=DIRECTION('ref_axis',(1.03377769602066E-32,0.,1.));
#125467=DIRECTION('',(-8.37284837049414E-17,-1.,0.));
#125468=DIRECTION('',(-8.37284837049414E-17,-1.,-1.23467863058847E-16));
#125469=DIRECTION('center_axis',(8.37284837049414E-17,1.,0.));
#125470=DIRECTION('ref_axis',(0.,0.,1.));
#125471=DIRECTION('center_axis',(0.99026806874157,0.139173100960067,1.71834053708127E-17));
#125472=DIRECTION('ref_axis',(1.48746998541713E-33,1.23467863058847E-16,
-1.));
#125473=DIRECTION('',(0.139173100960066,-0.99026806874157,-1.22266282302933E-16));
#125474=DIRECTION('center_axis',(0.,0.,1.));
#125475=DIRECTION('ref_axis',(0.,-1.,0.));
#125476=DIRECTION('',(-3.79382742684518E-34,-1.23467863058847E-16,1.));
#125477=DIRECTION('center_axis',(0.,0.,1.));
#125478=DIRECTION('ref_axis',(0.,-1.,0.));
#125479=DIRECTION('center_axis',(0.99026806874157,-0.139173100960065,-1.71834053708124E-17));
#125480=DIRECTION('ref_axis',(2.50622989185404E-33,1.23467863058847E-16,
-1.));
#125481=DIRECTION('',(-0.139173100960064,-0.99026806874157,-1.22266282302934E-16));
#125482=DIRECTION('center_axis',(0.,0.,1.));
#125483=DIRECTION('ref_axis',(0.,-1.,0.));
#125484=DIRECTION('',(3.05149908249585E-33,1.23467863058847E-16,-1.));
#125485=DIRECTION('center_axis',(0.,0.,1.));
#125486=DIRECTION('ref_axis',(0.,-1.,0.));
#125487=DIRECTION('center_axis',(0.,-1.,0.));
#125488=DIRECTION('ref_axis',(0.,0.,-1.));
#125489=DIRECTION('',(1.,0.,0.));
#125490=DIRECTION('center_axis',(0.,-1.23467863058847E-16,1.));
#125491=DIRECTION('ref_axis',(0.,-1.,-1.23467863058847E-16));
#125492=DIRECTION('',(1.,0.,0.));
#125493=DIRECTION('',(-8.37284837049414E-17,-1.,0.));
#125494=DIRECTION('',(0.139173100960067,-0.99026806874157,-1.22266282302933E-16));
#125495=DIRECTION('',(-8.37284837049414E-17,-1.,0.));
#125496=DIRECTION('center_axis',(2.30289132140253E-30,4.29529458662731E-44,
-1.));
#125497=DIRECTION('ref_axis',(1.86517468137027E-14,-1.,3.48488855560224E-59));
#125498=DIRECTION('',(-8.37284837049414E-17,-1.,0.));
#125499=DIRECTION('center_axis',(-3.72849071084219E-30,1.12593209572362E-43,
-1.));
#125500=DIRECTION('ref_axis',(-3.01980662698043E-14,-1.,1.99136488891557E-59));
#125501=DIRECTION('',(-8.37284837049414E-17,-1.,0.));
#125502=DIRECTION('',(-1.,0.,0.));
#125503=DIRECTION('',(-8.37284837049414E-17,-1.,0.));
#125504=DIRECTION('',(-0.139173100960064,-0.99026806874157,-1.22266282302933E-16));
#125505=DIRECTION('',(-8.37284837049414E-17,-1.,0.));
#125506=DIRECTION('',(0.707106781186546,-0.707106781186549,0.));
#125507=DIRECTION('center_axis',(0.,0.,-1.));
#125508=DIRECTION('ref_axis',(0.,-1.,0.));
#125509=DIRECTION('',(-0.707106781186546,0.707106781186549,0.));
#125510=DIRECTION('',(-1.,0.,0.));
#125511=DIRECTION('',(1.23138919323476E-16,1.,0.));
#125512=DIRECTION('',(1.,6.93889390390722E-15,0.));
#125513=DIRECTION('',(0.707106781186549,0.707106781186546,0.));
#125514=DIRECTION('center_axis',(0.,0.,-1.));
#125515=DIRECTION('ref_axis',(0.,-1.,0.));
#125516=DIRECTION('',(-0.707106781186548,-0.707106781186547,0.));
#125517=DIRECTION('center_axis',(0.99026806874157,0.139173100960067,1.71834053708127E-17));
#125518=DIRECTION('ref_axis',(1.48746998541713E-33,1.23467863058847E-16,
-1.));
#125519=DIRECTION('center_axis',(0.,1.,0.));
#125520=DIRECTION('ref_axis',(1.,0.,0.));
#125521=DIRECTION('center_axis',(8.37284837049414E-17,1.,0.));
#125522=DIRECTION('ref_axis',(0.,0.,1.));
#125523=DIRECTION('',(-8.37284837049414E-17,-1.,-1.23467863058847E-16));
#125524=DIRECTION('center_axis',(-1.,8.37284837049414E-17,1.03377769602066E-32));
#125525=DIRECTION('ref_axis',(1.03377769602066E-32,0.,1.));
#125526=DIRECTION('center_axis',(8.37284837049414E-17,1.,0.));
#125527=DIRECTION('ref_axis',(0.,0.,1.));
#125528=DIRECTION('',(-8.37284837049414E-17,-1.,-1.23467863058847E-16));
#125529=DIRECTION('center_axis',(-1.,8.37284837049414E-17,1.03377769602066E-32));
#125530=DIRECTION('ref_axis',(1.03377769602066E-32,0.,1.));
#125531=DIRECTION('center_axis',(8.37284837049414E-17,1.,0.));
#125532=DIRECTION('ref_axis',(0.,0.,1.));
#125533=DIRECTION('',(-8.37284837049414E-17,-1.,-1.23467863058847E-16));
#125534=DIRECTION('center_axis',(-1.,8.37284837049414E-17,1.03377769602066E-32));
#125535=DIRECTION('ref_axis',(1.03377769602066E-32,0.,1.));
#125536=DIRECTION('center_axis',(8.37284837049414E-17,1.,0.));
#125537=DIRECTION('ref_axis',(0.,0.,1.));
#125538=DIRECTION('',(-8.37284837049414E-17,-1.,-1.23467863058847E-16));
#125539=DIRECTION('center_axis',(-1.,8.37284837049414E-17,1.03377769602066E-32));
#125540=DIRECTION('ref_axis',(1.03377769602066E-32,0.,1.));
#125541=DIRECTION('center_axis',(0.,0.,1.));
#125542=DIRECTION('ref_axis',(0.,-1.,0.));
#125543=DIRECTION('center_axis',(8.37284837049414E-17,1.,0.));
#125544=DIRECTION('ref_axis',(0.,0.,1.));
#125545=DIRECTION('',(-8.37284837049414E-17,-1.,-1.23467863058847E-16));
#125546=DIRECTION('center_axis',(-1.,8.37284837049414E-17,1.03377769602066E-32));
#125547=DIRECTION('ref_axis',(1.03377769602066E-32,0.,1.));
#125548=DIRECTION('center_axis',(0.,0.,1.));
#125549=DIRECTION('ref_axis',(0.,-1.,0.));
#125550=DIRECTION('center_axis',(0.99026806874157,-0.139173100960065,-1.71834053708124E-17));
#125551=DIRECTION('ref_axis',(2.50622989185404E-33,1.23467863058847E-16,
-1.));
#125552=DIRECTION('center_axis',(8.37284837049414E-17,1.,0.));
#125553=DIRECTION('ref_axis',(0.,0.,1.));
#125554=DIRECTION('',(-8.37284837049414E-17,-1.,-1.23467863058847E-16));
#125555=DIRECTION('center_axis',(-1.,8.37284837049414E-17,1.03377769602066E-32));
#125556=DIRECTION('ref_axis',(1.03377769602066E-32,0.,1.));
#125557=DIRECTION('center_axis',(0.707106781186549,0.707106781186546,8.73049632275228E-17));
#125558=DIRECTION('ref_axis',(-1.37111453708203E-33,1.23467863058847E-16,
-1.));
#125559=DIRECTION('',(0.,-1.23467863058847E-16,1.));
#125560=DIRECTION('center_axis',(0.,1.,1.23467863058847E-16));
#125561=DIRECTION('ref_axis',(0.,1.23467863058847E-16,-1.));
#125562=DIRECTION('',(0.,-1.23467863058847E-16,1.));
#125563=DIRECTION('center_axis',(-1.,0.,0.));
#125564=DIRECTION('ref_axis',(0.,0.,1.));
#125565=DIRECTION('center_axis',(6.93889390390722E-15,-1.,-1.23467863058847E-16));
#125566=DIRECTION('ref_axis',(1.7439285617587E-47,1.23467863058847E-16,
-1.));
#125567=DIRECTION('center_axis',(0.707106781186546,-0.707106781186549,-8.73049632275232E-17));
#125568=DIRECTION('ref_axis',(6.2670764807642E-34,1.23467863058847E-16,
-1.));
#125569=DIRECTION('',(0.,-1.23467863058847E-16,1.));
#125570=DIRECTION('center_axis',(0.,0.,1.));
#125571=DIRECTION('ref_axis',(0.,-1.,0.));
#125572=DIRECTION('',(0.,-1.23467863058847E-16,1.));
#125573=DIRECTION('center_axis',(-0.707106781186547,0.707106781186548,8.73049632275232E-17));
#125574=DIRECTION('ref_axis',(1.23467863058848E-16,-3.38443013258907E-33,
1.));
#125575=DIRECTION('center_axis',(0.,-1.,-1.23467863058847E-16));
#125576=DIRECTION('ref_axis',(0.,1.23467863058847E-16,-1.));
#125577=DIRECTION('center_axis',(-0.707106781186549,-0.707106781186546,
-8.73049632275229E-17));
#125578=DIRECTION('ref_axis',(-0.707106781186546,0.707106781186549,-5.88012513992254E-33));
#125579=DIRECTION('',(0.,-1.23467863058847E-16,1.));
#125580=DIRECTION('center_axis',(0.,0.,1.));
#125581=DIRECTION('ref_axis',(0.,-1.,0.));
#125582=DIRECTION('center_axis',(-1.51575151553259E-16,1.51575151553257E-16,
-1.));
#125583=DIRECTION('ref_axis',(-1.,-7.79357634404829E-50,1.51575151553259E-16));
#125584=DIRECTION('center_axis',(-1.51575151553257E-16,-1.68282223215474E-30,
-1.));
#125585=DIRECTION('ref_axis',(-1.11022302462516E-14,1.,-5.25486924121806E-45));
#125586=DIRECTION('center_axis',(-1.51575151553257E-16,-1.68282223215474E-30,
-1.));
#125587=DIRECTION('ref_axis',(-1.11022302462516E-14,1.,-5.25486924121806E-45));
#125588=DIRECTION('center_axis',(-1.51575151553257E-16,-1.68282223215474E-30,
-1.));
#125589=DIRECTION('ref_axis',(-1.11022302462516E-14,1.,-5.25486924121806E-45));
#125590=DIRECTION('center_axis',(-1.51575151553257E-16,-1.68282223215474E-30,
-1.));
#125591=DIRECTION('ref_axis',(-1.11022302462516E-14,1.,-5.25486924121806E-45));
#125592=DIRECTION('center_axis',(-1.51575151553257E-16,-1.68282223215474E-30,
-1.));
#125593=DIRECTION('ref_axis',(-1.11022302462516E-14,1.,-5.25486924121806E-45));
#125594=DIRECTION('center_axis',(-1.51575151553257E-16,-1.68282223215474E-30,
-1.));
#125595=DIRECTION('ref_axis',(-1.11022302462516E-14,1.,-5.25486924121806E-45));
#125596=DIRECTION('center_axis',(1.51575151553257E-16,1.68282223215474E-30,
1.));
#125597=DIRECTION('ref_axis',(-1.11022302462516E-14,1.,-5.25486924121806E-45));
#125598=DIRECTION('center_axis',(1.51575151553257E-16,1.68282223215474E-30,
1.));
#125599=DIRECTION('ref_axis',(-1.11022302462516E-14,1.,-5.25486924121806E-45));
#125600=DIRECTION('center_axis',(1.51575151553257E-16,1.68282223215474E-30,
1.));
#125601=DIRECTION('ref_axis',(-1.11022302462516E-14,1.,-5.25486924121806E-45));
#125602=DIRECTION('center_axis',(1.51575151553257E-16,1.68282223215474E-30,
1.));
#125603=DIRECTION('ref_axis',(-1.11022302462516E-14,1.,-5.25486924121806E-45));
#125604=DIRECTION('center_axis',(1.51575151553257E-16,1.68282223215474E-30,
1.));
#125605=DIRECTION('ref_axis',(-1.11022302462516E-14,1.,-5.25486924121806E-45));
#125606=DIRECTION('center_axis',(1.51575151553257E-16,1.68282223215474E-30,
1.));
#125607=DIRECTION('ref_axis',(-1.11022302462516E-14,1.,-5.25486924121806E-45));
#125608=DIRECTION('center_axis',(-1.51575151553259E-16,1.51575151553257E-16,
-1.));
#125609=DIRECTION('ref_axis',(-1.,-7.79357634404829E-50,1.51575151553259E-16));
#125610=DIRECTION('center_axis',(-1.51575151553257E-16,-1.68282223215474E-30,
-1.));
#125611=DIRECTION('ref_axis',(-1.11022302462516E-14,1.,-5.25486924121806E-45));
#125612=DIRECTION('center_axis',(1.51575151553257E-16,1.68282223215474E-30,
1.));
#125613=DIRECTION('ref_axis',(-1.11022302462516E-14,1.,-5.25486924121806E-45));
#125614=DIRECTION('center_axis',(1.51575151553256E-16,2.10352779019342E-30,
1.));
#125615=DIRECTION('ref_axis',(-1.38777878078145E-14,1.,-8.0574661698677E-45));
#125616=DIRECTION('center_axis',(1.51575151553257E-16,1.26211667411606E-30,
1.));
#125617=DIRECTION('ref_axis',(-8.32667268468868E-15,1.,-4.55422000905566E-45));
#125618=DIRECTION('center_axis',(1.51575151553258E-16,8.41411116077375E-31,
1.));
#125619=DIRECTION('ref_axis',(-5.55111512312578E-15,1.,-2.10194769648723E-45));
#125620=DIRECTION('center_axis',(1.51575151553256E-16,2.94493890627077E-30,
1.));
#125621=DIRECTION('ref_axis',(-1.94289029309402E-14,1.,-3.50324616081204E-45));
#125622=DIRECTION('center_axis',(-1.51575151553257E-16,-1.68282223215474E-30,
-1.));
#125623=DIRECTION('ref_axis',(-1.11022302462516E-14,1.,-5.25486924121806E-45));
#125624=DIRECTION('center_axis',(-1.51575151553257E-16,-1.68282223215474E-30,
-1.));
#125625=DIRECTION('ref_axis',(-1.11022302462516E-14,1.,-5.25486924121806E-45));
#125626=DIRECTION('center_axis',(-1.51575151553257E-16,-1.68282223215474E-30,
-1.));
#125627=DIRECTION('ref_axis',(-1.11022302462516E-14,1.,-5.25486924121806E-45));
#125628=DIRECTION('center_axis',(-1.51575151553257E-16,-1.68282223215474E-30,
-1.));
#125629=DIRECTION('ref_axis',(-1.11022302462516E-14,1.,-5.25486924121806E-45));
#125630=DIRECTION('center_axis',(-1.51575151553257E-16,-1.68282223215474E-30,
-1.));
#125631=DIRECTION('ref_axis',(-1.11022302462516E-14,1.,-5.25486924121806E-45));
#125632=DIRECTION('center_axis',(-1.51575151553257E-16,-1.68282223215474E-30,
-1.));
#125633=DIRECTION('ref_axis',(-1.11022302462516E-14,1.,-5.25486924121806E-45));
#125634=DIRECTION('center_axis',(1.04744440165294E-14,-1.,-1.51575151553259E-16));
#125635=DIRECTION('ref_axis',(1.25902247940101E-46,1.51575151553259E-16,
-1.));
#125636=DIRECTION('',(-3.95893176803294E-18,-1.51575151553259E-16,1.));
#125637=DIRECTION('',(-3.95893176803294E-18,-1.51575151553259E-16,1.));
#125638=DIRECTION('center_axis',(0.866025403784444,-0.49999999999999,-7.23590402936621E-17));
#125639=DIRECTION('ref_axis',(-3.6604109175554E-33,1.44718080587327E-16,
-1.));
#125640=DIRECTION('',(-3.95893176803294E-18,-1.51575151553259E-16,1.));
#125641=DIRECTION('center_axis',(0.866025403784433,0.50000000000001,7.92161112595966E-17));
#125642=DIRECTION('ref_axis',(-8.33872958215071E-33,1.5843222251919E-16,
-1.));
#125643=DIRECTION('',(-3.95893176803294E-18,-1.51575151553259E-16,1.));
#125644=DIRECTION('center_axis',(-1.06246754764031E-14,1.,1.51575151553259E-16));
#125645=DIRECTION('ref_axis',(1.,1.06246754764031E-14,0.));
#125646=DIRECTION('',(-3.95893176803294E-18,-1.51575151553259E-16,1.));
#125647=DIRECTION('center_axis',(-0.866025403784444,0.499999999999991,7.23590402936622E-17));
#125648=DIRECTION('ref_axis',(8.35530227836972E-17,-4.07346201807404E-33,
1.));
#125649=DIRECTION('',(-3.95893176803294E-18,-1.51575151553259E-16,1.));
#125650=DIRECTION('center_axis',(-0.866025403784432,-0.500000000000011,
-7.92161112595969E-17));
#125651=DIRECTION('ref_axis',(-0.500000000000011,0.866025403784432,1.10736588620036E-33));
#125652=DIRECTION('center_axis',(0.,3.03150303106518E-16,-1.));
#125653=DIRECTION('ref_axis',(-1.,0.,0.));
#125654=DIRECTION('center_axis',(0.,3.03150303106518E-16,-1.));
#125655=DIRECTION('ref_axis',(1.,0.,0.));
#125656=DIRECTION('center_axis',(0.,3.03150303106518E-16,-1.));
#125657=DIRECTION('ref_axis',(1.,0.,0.));
#125658=DIRECTION('center_axis',(0.,3.03150303106518E-16,-1.));
#125659=DIRECTION('ref_axis',(1.,0.,0.));
#125660=DIRECTION('center_axis',(0.,3.03150303106518E-16,-1.));
#125661=DIRECTION('ref_axis',(1.,0.,0.));
#125662=DIRECTION('center_axis',(0.,3.03150303106518E-16,-1.));
#125663=DIRECTION('ref_axis',(1.,0.,0.));
#125664=DIRECTION('center_axis',(0.,3.03150303106518E-16,-1.));
#125665=DIRECTION('ref_axis',(1.,0.,0.));
#125666=DIRECTION('center_axis',(0.,-3.03150303106518E-16,1.));
#125667=DIRECTION('ref_axis',(1.,0.,0.));
#125668=DIRECTION('center_axis',(0.,-3.03150303106518E-16,1.));
#125669=DIRECTION('ref_axis',(1.,0.,0.));
#125670=DIRECTION('center_axis',(0.,-3.03150303106518E-16,1.));
#125671=DIRECTION('ref_axis',(1.,0.,0.));
#125672=DIRECTION('center_axis',(0.,-3.03150303106518E-16,1.));
#125673=DIRECTION('ref_axis',(1.,0.,0.));
#125674=DIRECTION('center_axis',(0.,-3.03150303106518E-16,1.));
#125675=DIRECTION('ref_axis',(1.,0.,0.));
#125676=DIRECTION('center_axis',(0.,-3.03150303106518E-16,1.));
#125677=DIRECTION('ref_axis',(1.,0.,0.));
#125678=DIRECTION('center_axis',(0.,3.03150303106518E-16,-1.));
#125679=DIRECTION('ref_axis',(-1.,0.,0.));
#125680=DIRECTION('center_axis',(0.,3.03150303106518E-16,-1.));
#125681=DIRECTION('ref_axis',(1.,0.,0.));
#125682=DIRECTION('center_axis',(0.,-3.03150303106518E-16,1.));
#125683=DIRECTION('ref_axis',(1.,0.,0.));
#125684=DIRECTION('center_axis',(-8.4141111607738E-31,-3.03150303106518E-16,
1.));
#125685=DIRECTION('ref_axis',(1.,-2.77555756156289E-15,2.83543986140725E-45));
#125686=DIRECTION('center_axis',(-8.4141111607738E-31,-3.03150303106518E-16,
1.));
#125687=DIRECTION('ref_axis',(1.,-2.77555756156289E-15,2.83543986140725E-45));
#125688=DIRECTION('center_axis',(8.4141111607738E-31,-3.03150303106518E-16,
1.));
#125689=DIRECTION('ref_axis',(1.,2.77555756156289E-15,-2.83543986140725E-45));
#125690=DIRECTION('center_axis',(-1.68282223215476E-30,-3.03150303106518E-16,
1.));
#125691=DIRECTION('ref_axis',(1.,-5.55111512312578E-15,5.67087972281449E-45));
#125692=DIRECTION('center_axis',(0.,3.03150303106518E-16,-1.));
#125693=DIRECTION('ref_axis',(1.,0.,0.));
#125694=DIRECTION('center_axis',(0.,3.03150303106518E-16,-1.));
#125695=DIRECTION('ref_axis',(1.,0.,0.));
#125696=DIRECTION('center_axis',(0.,3.03150303106518E-16,-1.));
#125697=DIRECTION('ref_axis',(1.,0.,0.));
#125698=DIRECTION('center_axis',(0.,3.03150303106518E-16,-1.));
#125699=DIRECTION('ref_axis',(1.,0.,0.));
#125700=DIRECTION('center_axis',(0.,3.03150303106518E-16,-1.));
#125701=DIRECTION('ref_axis',(1.,0.,0.));
#125702=DIRECTION('center_axis',(0.,3.03150303106518E-16,-1.));
#125703=DIRECTION('ref_axis',(1.,0.,0.));
#125704=DIRECTION('center_axis',(-1.,0.,0.));
#125705=DIRECTION('ref_axis',(0.,0.,1.));
#125706=DIRECTION('',(0.,-1.47616219785226E-16,1.));
#125707=DIRECTION('',(0.,-1.47616219785226E-16,1.));
#125708=DIRECTION('center_axis',(-0.5,-0.866025403784439,-1.27839396344633E-16));
#125709=DIRECTION('ref_axis',(-0.866025403784439,0.5,-4.56072208893389E-33));
#125710=DIRECTION('',(0.,-1.47616219785226E-16,1.));
#125711=DIRECTION('center_axis',(0.5,-0.866025403784438,-1.27839396344633E-16));
#125712=DIRECTION('ref_axis',(-5.60121745056272E-33,1.47616219785226E-16,
-1.));
#125713=DIRECTION('',(0.,-1.47616219785226E-16,1.));
#125714=DIRECTION('center_axis',(1.,1.50231459873716E-16,2.21766001993738E-32));
#125715=DIRECTION('ref_axis',(-1.50231459873716E-16,1.,5.05166336074856E-65));
#125716=DIRECTION('',(0.,-1.47616219785226E-16,1.));
#125717=DIRECTION('center_axis',(0.5,0.866025403784439,1.27839396344633E-16));
#125718=DIRECTION('ref_axis',(2.55678792689265E-16,1.22570872579745E-32,
-1.));
#125719=DIRECTION('',(0.,-1.47616219785226E-16,1.));
#125720=DIRECTION('center_axis',(-0.5,0.866025403784438,1.27839396344632E-16));
#125721=DIRECTION('ref_axis',(2.55678792689264E-16,1.21193584857665E-32,
1.));
#125722=DIRECTION('center_axis',(0.5,0.866025403784438,1.0692630595994E-16));
#125723=DIRECTION('ref_axis',(2.13852611919879E-16,-5.48307457472744E-35,
-1.));
#125724=DIRECTION('',(0.,1.23467863058847E-16,-1.));
#125725=DIRECTION('',(0.,1.23467863058847E-16,-1.));
#125726=DIRECTION('center_axis',(1.,0.,0.));
#125727=DIRECTION('ref_axis',(0.,1.,0.));
#125728=DIRECTION('',(0.,1.23467863058847E-16,-1.));
#125729=DIRECTION('center_axis',(0.5,-0.866025403784439,-1.0692630595994E-16));
#125730=DIRECTION('ref_axis',(4.1166144903646E-33,1.23467863058847E-16,
-1.));
#125731=DIRECTION('',(0.,1.23467863058847E-16,-1.));
#125732=DIRECTION('center_axis',(-0.5,-0.866025403784439,-1.0692630595994E-16));
#125733=DIRECTION('ref_axis',(-0.866025403784439,0.5,-7.83367607530638E-34));
#125734=DIRECTION('',(0.,1.23467863058847E-16,-1.));
#125735=DIRECTION('center_axis',(-1.,0.,0.));
#125736=DIRECTION('ref_axis',(0.,0.,1.));
#125737=DIRECTION('',(0.,1.23467863058847E-16,-1.));
#125738=DIRECTION('center_axis',(-0.5,0.866025403784439,1.0692630595994E-16));
#125739=DIRECTION('ref_axis',(2.1385261191988E-16,4.09037363277686E-33,
1.));
#125740=DIRECTION('center_axis',(0.,0.,-1.));
#125741=DIRECTION('ref_axis',(0.,1.,0.));
#125742=DIRECTION('',(-1.06057523872491E-16,-0.866025403784439,-0.5));
#125743=DIRECTION('center_axis',(0.,0.,-1.));
#125744=DIRECTION('ref_axis',(0.,1.,0.));
#125745=DIRECTION('center_axis',(0.,0.,1.));
#125746=DIRECTION('ref_axis',(0.,1.,0.));
#125747=DIRECTION('center_axis',(0.,0.,-1.));
#125748=DIRECTION('ref_axis',(0.,1.,0.));
#125749=DIRECTION('center_axis',(0.,0.,1.));
#125750=DIRECTION('ref_axis',(0.,1.,0.));
#125751=DIRECTION('center_axis',(0.,0.,-1.));
#125752=DIRECTION('ref_axis',(0.,1.,0.));
#125753=DIRECTION('center_axis',(0.,0.,1.));
#125754=DIRECTION('ref_axis',(0.,1.,0.));
#125755=DIRECTION('center_axis',(0.,0.,-1.));
#125756=DIRECTION('ref_axis',(0.,1.,0.));
#125757=DIRECTION('center_axis',(0.,0.,1.));
#125758=DIRECTION('ref_axis',(0.,1.,0.));
#125759=DIRECTION('center_axis',(0.,0.,-1.));
#125760=DIRECTION('ref_axis',(0.,1.,0.));
#125761=DIRECTION('center_axis',(0.,0.,1.));
#125762=DIRECTION('ref_axis',(0.,1.,0.));
#125763=DIRECTION('center_axis',(0.,0.,-1.));
#125764=DIRECTION('ref_axis',(0.,1.,0.));
#125765=DIRECTION('center_axis',(0.,0.,1.));
#125766=DIRECTION('ref_axis',(0.,1.,0.));
#125767=DIRECTION('center_axis',(0.,1.23467863058847E-16,-1.));
#125768=DIRECTION('ref_axis',(0.,1.,0.));
#125769=DIRECTION('center_axis',(0.,0.,1.));
#125770=DIRECTION('ref_axis',(0.,1.,0.));
#125771=DIRECTION('center_axis',(-1.,0.,0.));
#125772=DIRECTION('ref_axis',(0.,-1.,0.));
#125773=DIRECTION('center_axis',(0.,0.,-1.));
#125774=DIRECTION('ref_axis',(0.,1.,0.));
#125775=DIRECTION('center_axis',(0.,0.,-1.));
#125776=DIRECTION('ref_axis',(0.,1.,0.));
#125777=DIRECTION('center_axis',(0.,1.23467863058847E-16,-1.));
#125778=DIRECTION('ref_axis',(-1.,0.,0.));
#125779=DIRECTION('center_axis',(0.,0.,1.));
#125780=DIRECTION('ref_axis',(0.,1.,0.));
#125781=DIRECTION('center_axis',(0.,1.23467863058847E-16,-1.));
#125782=DIRECTION('ref_axis',(-1.,0.,0.));
#125783=DIRECTION('center_axis',(0.,0.,1.));
#125784=DIRECTION('ref_axis',(0.,-1.,0.));
#125785=DIRECTION('',(0.,0.,-1.));
#125786=DIRECTION('center_axis',(0.,0.581981048437469,0.813202348287082));
#125787=DIRECTION('ref_axis',(0.,-0.813202348287082,0.581981048437469));
#125788=DIRECTION('center_axis',(-4.57440509151562E-13,-3.7199169624361E-13,
1.));
#125789=DIRECTION('ref_axis',(1.53744223053601E-12,-1.,-3.71991696242907E-13));
#125790=DIRECTION('center_axis',(6.93710496602244E-15,-1.,3.73149770104689E-14));
#125791=DIRECTION('ref_axis',(-7.99856117158489E-13,-3.73149770104744E-14,
-1.));
#125792=DIRECTION('',(0.,-0.581981048437474,-0.813202348287079));
#125793=DIRECTION('center_axis',(0.,-0.581981048437448,0.813202348287097));
#125794=DIRECTION('ref_axis',(0.,-0.813202348287097,-0.581981048437448));
#125795=DIRECTION('',(0.,0.581981048437457,-0.813202348287091));
#125796=DIRECTION('center_axis',(-2.04313070362676E-13,-1.,-2.05422270127779E-14));
#125797=DIRECTION('ref_axis',(-1.51334794436645E-12,2.05422270130871E-14,
-1.));
#125798=DIRECTION('center_axis',(0.,-0.581981048437448,0.813202348287097));
#125799=DIRECTION('ref_axis',(0.,-0.813202348287097,-0.581981048437448));
#125800=DIRECTION('center_axis',(0.,0.,-1.));
#125801=DIRECTION('ref_axis',(-1.,0.,0.));
#125802=DIRECTION('center_axis',(0.,-1.,0.));
#125803=DIRECTION('ref_axis',(-4.85369761888787E-14,0.,1.));
#125804=DIRECTION('center_axis',(-1.,2.31296463463574E-14,0.));
#125805=DIRECTION('ref_axis',(-2.31296463463574E-14,-1.,0.));
#125806=DIRECTION('center_axis',(0.,-1.,0.));
#125807=DIRECTION('ref_axis',(0.,0.,1.));
#125808=DIRECTION('center_axis',(1.,0.,0.));
#125809=DIRECTION('ref_axis',(0.,0.,1.));
#125810=DIRECTION('',(-1.,0.,0.));
#125811=DIRECTION('center_axis',(-1.,-9.25185853854296E-15,0.));
#125812=DIRECTION('ref_axis',(9.25185853854296E-15,-1.,0.));
#125813=DIRECTION('',(1.,0.,0.));
#125814=DIRECTION('center_axis',(0.,0.,-1.));
#125815=DIRECTION('ref_axis',(-1.,0.,0.));
#125816=DIRECTION('center_axis',(0.,-1.,0.));
#125817=DIRECTION('ref_axis',(0.,0.,1.));
#125818=DIRECTION('center_axis',(0.79173164804714,0.610869051008938,0.));
#125819=DIRECTION('ref_axis',(0.610869051008938,-0.79173164804714,0.));
#125820=DIRECTION('center_axis',(1.,0.,0.));
#125821=DIRECTION('ref_axis',(0.,0.,1.));
#125822=DIRECTION('center_axis',(0.,0.598310875192794,0.801264061733729));
#125823=DIRECTION('ref_axis',(0.,-0.801264061733729,0.598310875192794));
#125824=DIRECTION('center_axis',(0.,0.,-1.));
#125825=DIRECTION('ref_axis',(-1.,0.,0.));
#125826=DIRECTION('center_axis',(-1.,0.,0.));
#125827=DIRECTION('ref_axis',(0.,0.,1.));
#125828=DIRECTION('center_axis',(0.,0.,-1.));
#125829=DIRECTION('ref_axis',(-1.,0.,0.));
#125830=DIRECTION('center_axis',(-1.8733679913752E-13,0.0769742127966581,
0.997033083986853));
#125831=DIRECTION('ref_axis',(5.10679254440911E-30,0.997033083986853,-0.0769742127966581));
#125832=DIRECTION('center_axis',(0.,-1.,0.));
#125833=DIRECTION('ref_axis',(9.86527759356758E-14,0.,1.));
#125834=DIRECTION('center_axis',(1.,0.,0.));
#125835=DIRECTION('ref_axis',(0.,0.,1.));
#125836=DIRECTION('center_axis',(1.,0.,0.));
#125837=DIRECTION('ref_axis',(0.,2.66826051581462E-14,1.));
#125838=DIRECTION('center_axis',(1.,0.,0.));
#125839=DIRECTION('ref_axis',(0.,0.,1.));
#125840=DIRECTION('center_axis',(2.95998963611366E-29,-0.0769742127965279,
0.997033083986863));
#125841=DIRECTION('ref_axis',(1.85037170770858E-14,-0.997033083986863,-0.0769742127965279));
#125842=DIRECTION('center_axis',(1.,0.,0.));
#125843=DIRECTION('ref_axis',(0.,2.66826051581462E-14,1.));
#125844=DIRECTION('center_axis',(0.,0.,-1.));
#125845=DIRECTION('ref_axis',(-1.,0.,0.));
#125846=DIRECTION('center_axis',(2.36831436293266E-13,-0.598310875192877,
0.801264061733667));
#125847=DIRECTION('ref_axis',(4.05016586084113E-29,0.801264061733667,0.598310875192877));
#125848=DIRECTION('center_axis',(0.,-1.,0.));
#125849=DIRECTION('ref_axis',(0.,0.,1.));
#125850=DIRECTION('center_axis',(1.,0.,0.));
#125851=DIRECTION('ref_axis',(0.,0.,1.));
#125852=DIRECTION('center_axis',(0.,0.,1.));
#125853=DIRECTION('ref_axis',(1.,0.,0.));
#125854=DIRECTION('center_axis',(-1.,0.,0.));
#125855=DIRECTION('ref_axis',(0.,0.,1.));
#125856=DIRECTION('center_axis',(0.,0.,1.));
#125857=DIRECTION('ref_axis',(-1.,0.,0.));
#125858=DIRECTION('center_axis',(1.,0.,0.));
#125859=DIRECTION('ref_axis',(0.,0.,-1.));
#125860=DIRECTION('center_axis',(0.,0.,-1.));
#125861=DIRECTION('ref_axis',(-1.,0.,0.));
#125862=DIRECTION('center_axis',(0.,0.,-1.));
#125863=DIRECTION('ref_axis',(1.,0.,0.));
#125864=DIRECTION('center_axis',(1.,0.,-9.25185853854296E-15));
#125865=DIRECTION('ref_axis',(-9.25185853854296E-15,0.,-1.));
#125866=DIRECTION('center_axis',(0.,0.,1.));
#125867=DIRECTION('ref_axis',(1.,0.,0.));
#125868=DIRECTION('center_axis',(0.,0.581981048437445,0.813202348287099));
#125869=DIRECTION('ref_axis',(0.,-0.813202348287099,0.581981048437445));
#125870=DIRECTION('center_axis',(6.06486161256154E-14,-1.,-1.46202248832107E-14));
#125871=DIRECTION('ref_axis',(7.25749190859778E-12,1.46202248836508E-14,
-1.));
#125872=DIRECTION('',(0.,-0.581981048437472,-0.81320234828708));
#125873=DIRECTION('center_axis',(1.71540190931773E-13,1.39496886091321E-13,
-1.));
#125874=DIRECTION('ref_axis',(1.40059985610807E-12,1.,1.39496886091562E-13));
#125875=DIRECTION('',(0.,0.581981048437472,0.81320234828708));
#125876=DIRECTION('center_axis',(0.,-0.581981048437456,0.813202348287091));
#125877=DIRECTION('ref_axis',(0.,-0.813202348287091,-0.581981048437456));
#125878=DIRECTION('center_axis',(8.57700954657943E-14,-1.,4.99165700837713E-14));
#125879=DIRECTION('ref_axis',(-3.54373217756707E-13,-4.99165700838017E-14,
-1.));
#125880=DIRECTION('',(0.,-0.581981048437457,0.813202348287091));
#125881=DIRECTION('',(0.,0.581981048437457,-0.813202348287091));
#125882=DIRECTION('center_axis',(-1.,0.,0.));
#125883=DIRECTION('ref_axis',(0.,0.,1.));
#125884=DIRECTION('',(0.,0.,-1.));
#125885=DIRECTION('',(0.,1.,0.));
#125886=DIRECTION('center_axis',(-1.,0.,0.));
#125887=DIRECTION('ref_axis',(0.,0.,1.));
#125888=DIRECTION('',(0.,0.,-1.));
#125889=DIRECTION('',(0.,1.,0.));
#125890=DIRECTION('center_axis',(1.,0.,0.));
#125891=DIRECTION('ref_axis',(0.,1.,0.));
#125892=DIRECTION('',(0.,0.,1.));
#125893=DIRECTION('',(0.,0.,1.));
#125894=DIRECTION('',(0.,-1.,0.));
#125895=DIRECTION('',(0.,3.03450170724806E-16,1.));
#125896=DIRECTION('',(0.,-1.,0.));
#125897=DIRECTION('',(0.,0.,1.));
#125898=DIRECTION('center_axis',(0.,0.581981048437469,0.813202348287082));
#125899=DIRECTION('ref_axis',(0.,-0.813202348287082,0.581981048437469));
#125900=DIRECTION('',(0.,-0.581981048437474,-0.813202348287079));
#125901=DIRECTION('center_axis',(1.64603085965779E-13,-1.,1.37148117178086E-13));
#125902=DIRECTION('ref_axis',(6.31098224630747E-13,-1.37148117177982E-13,
-1.));
#125903=DIRECTION('center_axis',(-4.57440509151577E-13,3.71991696243625E-13,
-1.));
#125904=DIRECTION('ref_axis',(1.52275222876736E-12,1.,3.71991696242928E-13));
#125905=DIRECTION('center_axis',(0.,-0.581981048437448,0.813202348287097));
#125906=DIRECTION('ref_axis',(0.,-0.813202348287097,-0.581981048437448));
#125907=DIRECTION('center_axis',(0.,0.581981048437448,-0.813202348287097));
#125908=DIRECTION('ref_axis',(0.,-0.813202348287097,-0.581981048437448));
#125909=DIRECTION('center_axis',(2.04313070362666E-13,-1.,-2.05422270127758E-14));
#125910=DIRECTION('ref_axis',(7.96460775263604E-12,2.05422270144031E-14,
-1.));
#125911=DIRECTION('',(0.,0.581981048437457,-0.813202348287091));
#125912=DIRECTION('center_axis',(0.,0.,-1.));
#125913=DIRECTION('ref_axis',(1.,0.,0.));
#125914=DIRECTION('center_axis',(-1.,-2.31296463463574E-14,0.));
#125915=DIRECTION('ref_axis',(2.31296463463574E-14,-1.,0.));
#125916=DIRECTION('center_axis',(0.,-1.,0.));
#125917=DIRECTION('ref_axis',(-1.61789920629596E-14,0.,1.));
#125918=DIRECTION('center_axis',(0.,1.,0.));
#125919=DIRECTION('ref_axis',(0.,0.,1.));
#125920=DIRECTION('center_axis',(-1.,0.,0.));
#125921=DIRECTION('ref_axis',(0.,0.,1.));
#125922=DIRECTION('center_axis',(-1.,9.25185853854296E-15,0.));
#125923=DIRECTION('ref_axis',(-9.25185853854296E-15,-1.,0.));
#125924=DIRECTION('',(-1.,0.,0.));
#125925=DIRECTION('',(-1.,0.,0.));
#125926=DIRECTION('center_axis',(0.,0.,-1.));
#125927=DIRECTION('ref_axis',(1.,0.,0.));
#125928=DIRECTION('center_axis',(0.79173164804714,-0.610869051008938,0.));
#125929=DIRECTION('ref_axis',(-0.610869051008938,-0.79173164804714,0.));
#125930=DIRECTION('center_axis',(0.,-1.,0.));
#125931=DIRECTION('ref_axis',(1.29431936503677E-13,0.,1.));
#125932=DIRECTION('center_axis',(-1.,0.,0.));
#125933=DIRECTION('ref_axis',(0.,0.,1.));
#125934=DIRECTION('center_axis',(0.,0.,1.));
#125935=DIRECTION('ref_axis',(1.,0.,0.));
#125936=DIRECTION('center_axis',(0.,-0.598310875192794,-0.801264061733729));
#125937=DIRECTION('ref_axis',(0.,-0.801264061733729,0.598310875192794));
#125938=DIRECTION('center_axis',(-1.,0.,0.));
#125939=DIRECTION('ref_axis',(0.,0.,1.));
#125940=DIRECTION('center_axis',(0.,0.,-1.));
#125941=DIRECTION('ref_axis',(1.,0.,0.));
#125942=DIRECTION('center_axis',(0.,-1.,0.));
#125943=DIRECTION('ref_axis',(2.30189810516577E-13,0.,1.));
#125944=DIRECTION('center_axis',(-1.8733679913752E-13,-0.0769742127966581,
-0.997033083986853));
#125945=DIRECTION('ref_axis',(-5.10679254440911E-30,0.997033083986853,-0.0769742127966581));
#125946=DIRECTION('center_axis',(-1.,0.,0.));
#125947=DIRECTION('ref_axis',(0.,0.,1.));
#125948=DIRECTION('center_axis',(1.,0.,0.));
#125949=DIRECTION('ref_axis',(0.,2.66826051581462E-14,1.));
#125950=DIRECTION('center_axis',(-1.,0.,0.));
#125951=DIRECTION('ref_axis',(0.,0.,1.));
#125952=DIRECTION('center_axis',(1.,0.,0.));
#125953=DIRECTION('ref_axis',(0.,2.66826051581462E-14,1.));
#125954=DIRECTION('center_axis',(2.95998963611366E-29,0.0769742127965279,
-0.997033083986863));
#125955=DIRECTION('ref_axis',(-1.85037170770858E-14,-0.997033083986863,
-0.0769742127965279));
#125956=DIRECTION('center_axis',(0.,0.,-1.));
#125957=DIRECTION('ref_axis',(1.,0.,0.));
#125958=DIRECTION('center_axis',(0.,-1.,0.));
#125959=DIRECTION('ref_axis',(-2.19228390968164E-14,0.,1.));
#125960=DIRECTION('center_axis',(2.36831436293266E-13,0.598310875192877,
-0.801264061733667));
#125961=DIRECTION('ref_axis',(-4.05016586084113E-29,0.801264061733667,0.598310875192877));
#125962=DIRECTION('center_axis',(-1.,0.,0.));
#125963=DIRECTION('ref_axis',(0.,0.,1.));
#125964=DIRECTION('center_axis',(0.,0.,-1.));
#125965=DIRECTION('ref_axis',(-1.,0.,0.));
#125966=DIRECTION('center_axis',(-1.,0.,0.));
#125967=DIRECTION('ref_axis',(0.,0.,1.));
#125968=DIRECTION('center_axis',(0.,0.,1.));
#125969=DIRECTION('ref_axis',(1.,0.,0.));
#125970=DIRECTION('center_axis',(0.,0.,1.));
#125971=DIRECTION('ref_axis',(1.,0.,0.));
#125972=DIRECTION('center_axis',(1.,0.,0.));
#125973=DIRECTION('ref_axis',(0.,0.,-1.));
#125974=DIRECTION('center_axis',(0.,0.,-1.));
#125975=DIRECTION('ref_axis',(-1.,0.,0.));
#125976=DIRECTION('center_axis',(1.,0.,9.25185853854296E-15));
#125977=DIRECTION('ref_axis',(9.25185853854296E-15,0.,-1.));
#125978=DIRECTION('center_axis',(0.,0.,-1.));
#125979=DIRECTION('ref_axis',(-1.,0.,0.));
#125980=DIRECTION('center_axis',(0.,0.581981048437445,0.813202348287099));
#125981=DIRECTION('ref_axis',(0.,-0.813202348287099,0.581981048437445));
#125982=DIRECTION('center_axis',(-6.06486161256147E-14,-1.,-1.46202248832103E-14));
#125983=DIRECTION('ref_axis',(-6.92803770888931E-12,1.46202248836305E-14,
-1.));
#125984=DIRECTION('',(0.,0.581981048437472,0.81320234828708));
#125985=DIRECTION('center_axis',(1.71540190931776E-13,-1.39496886091324E-13,
1.));
#125986=DIRECTION('ref_axis',(1.4629488977046E-12,-1.,-1.39496886091575E-13));
#125987=DIRECTION('',(0.,-0.581981048437472,-0.81320234828708));
#125988=DIRECTION('center_axis',(0.,-0.581981048437456,0.813202348287091));
#125989=DIRECTION('ref_axis',(0.,-0.813202348287091,-0.581981048437456));
#125990=DIRECTION('center_axis',(-8.5770095465791E-14,-1.,4.99165700837693E-14));
#125991=DIRECTION('ref_axis',(8.1434249535045E-13,-4.99165700838392E-14,
-1.));
#125992=DIRECTION('',(0.,0.581981048437457,-0.813202348287091));
#125993=DIRECTION('',(0.,-0.581981048437457,0.813202348287091));
#125994=DIRECTION('center_axis',(1.,0.,0.));
#125995=DIRECTION('ref_axis',(0.,1.,0.));
#125996=DIRECTION('',(0.,0.,1.));
#125997=DIRECTION('',(0.,1.,0.));
#125998=DIRECTION('center_axis',(1.,0.,0.));
#125999=DIRECTION('ref_axis',(0.,1.,0.));
#126000=DIRECTION('',(0.,0.,1.));
#126001=DIRECTION('',(0.,1.,0.));
#126002=DIRECTION('center_axis',(0.,0.81320234828708,-0.581981048437472));
#126003=DIRECTION('ref_axis',(-1.,0.,0.));
#126004=DIRECTION('',(1.,0.,0.));
#126005=DIRECTION('',(-1.,0.,0.));
#126006=DIRECTION('center_axis',(0.,0.813202348287091,0.581981048437457));
#126007=DIRECTION('ref_axis',(1.,0.,0.));
#126008=DIRECTION('',(-1.,0.,0.));
#126009=DIRECTION('',(1.,0.,0.));
#126010=DIRECTION('center_axis',(-1.,0.,0.));
#126011=DIRECTION('ref_axis',(0.,0.,1.));
#126012=DIRECTION('',(0.,0.,-1.));
#126013=DIRECTION('',(0.,0.,1.));
#126014=DIRECTION('',(0.,-1.,0.));
#126015=DIRECTION('',(0.,3.03450170724806E-16,1.));
#126016=DIRECTION('',(0.,-1.,0.));
#126017=DIRECTION('',(0.,0.,1.));
#126018=DIRECTION('center_axis',(0.,-1.,0.));
#126019=DIRECTION('ref_axis',(0.,0.,-1.));
#126020=DIRECTION('center_axis',(0.,-1.,0.));
#126021=DIRECTION('ref_axis',(0.,0.,1.));
#126022=DIRECTION('',(0.,-1.,0.));
#126023=DIRECTION('center_axis',(1.,0.,0.));
#126024=DIRECTION('ref_axis',(0.,0.,-1.));
#126025=DIRECTION('center_axis',(0.,0.,-1.));
#126026=DIRECTION('ref_axis',(1.,0.,0.));
#126027=DIRECTION('center_axis',(0.,0.,-1.));
#126028=DIRECTION('ref_axis',(-1.,0.,0.));
#126029=DIRECTION('',(0.,0.,-1.));
#126030=DIRECTION('center_axis',(0.,1.,0.));
#126031=DIRECTION('ref_axis',(0.,0.,1.));
#126032=DIRECTION('center_axis',(1.,0.,0.));
#126033=DIRECTION('ref_axis',(0.,0.,-1.));
#126034=DIRECTION('center_axis',(0.,1.,0.));
#126035=DIRECTION('ref_axis',(0.,0.,1.));
#126036=DIRECTION('center_axis',(0.,-1.,0.));
#126037=DIRECTION('ref_axis',(0.,0.,1.));
#126038=DIRECTION('center_axis',(1.,0.,0.));
#126039=DIRECTION('ref_axis',(0.,0.,1.));
#126040=DIRECTION('',(-1.,0.,0.));
#126041=DIRECTION('',(1.,0.,0.));
#126042=DIRECTION('center_axis',(0.,0.,1.));
#126043=DIRECTION('ref_axis',(-1.,0.,0.));
#126044=DIRECTION('center_axis',(0.,0.,1.));
#126045=DIRECTION('ref_axis',(1.,0.,0.));
#126046=DIRECTION('',(0.,0.,-1.));
#126047=DIRECTION('center_axis',(0.,-1.,0.));
#126048=DIRECTION('ref_axis',(0.,0.,-1.));
#126049=DIRECTION('center_axis',(1.,0.,0.));
#126050=DIRECTION('ref_axis',(0.,0.,-1.));
#126051=DIRECTION('center_axis',(0.,-1.,0.));
#126052=DIRECTION('ref_axis',(0.,0.,-1.));
#126053=DIRECTION('center_axis',(0.,1.,0.));
#126054=DIRECTION('ref_axis',(0.,0.,-1.));
#126055=DIRECTION('center_axis',(1.,0.,0.));
#126056=DIRECTION('ref_axis',(0.,0.,1.));
#126057=DIRECTION('',(-1.,0.,0.));
#126058=DIRECTION('',(1.,0.,0.));
#126059=DIRECTION('center_axis',(0.,-1.,0.));
#126060=DIRECTION('ref_axis',(0.,0.,-1.));
#126061=DIRECTION('center_axis',(0.,1.,0.));
#126062=DIRECTION('ref_axis',(0.,0.,-1.));
#126063=DIRECTION('',(0.,-1.,0.));
#126064=DIRECTION('center_axis',(0.,-1.,0.));
#126065=DIRECTION('ref_axis',(0.,0.,-1.));
#126066=DIRECTION('center_axis',(0.,1.,0.));
#126067=DIRECTION('ref_axis',(0.,0.,-1.));
#126068=DIRECTION('',(0.,-1.,0.));
#126069=DIRECTION('center_axis',(0.,-1.,3.03450170724806E-16));
#126070=DIRECTION('ref_axis',(-1.,0.,0.));
#126071=DIRECTION('',(1.,0.,0.));
#126072=DIRECTION('center_axis',(0.,-1.,0.));
#126073=DIRECTION('ref_axis',(0.,0.,-1.));
#126074=DIRECTION('center_axis',(0.,-1.,0.));
#126075=DIRECTION('ref_axis',(0.,0.,-1.));
#126076=DIRECTION('',(-1.,0.,0.));
#126077=DIRECTION('center_axis',(0.,-1.,0.));
#126078=DIRECTION('ref_axis',(0.,0.,-1.));
#126079=DIRECTION('center_axis',(0.,1.,0.));
#126080=DIRECTION('ref_axis',(0.,0.,1.));
#126081=DIRECTION('',(0.,-1.,0.));
#126082=DIRECTION('center_axis',(1.,0.,0.));
#126083=DIRECTION('ref_axis',(0.,0.,-1.));
#126084=DIRECTION('center_axis',(-1.,0.,0.));
#126085=DIRECTION('ref_axis',(0.,0.,1.));
#126086=DIRECTION('',(-1.,0.,0.));
#126087=DIRECTION('center_axis',(0.,0.,-1.));
#126088=DIRECTION('ref_axis',(-1.,0.,0.));
#126089=DIRECTION('center_axis',(0.,0.,1.));
#126090=DIRECTION('ref_axis',(1.,0.,0.));
#126091=DIRECTION('',(0.,0.,-1.));
#126092=DIRECTION('center_axis',(0.,1.,0.));
#126093=DIRECTION('ref_axis',(0.,0.,1.));
#126094=DIRECTION('center_axis',(1.,0.,0.));
#126095=DIRECTION('ref_axis',(0.,0.,-1.));
#126096=DIRECTION('center_axis',(0.,1.,0.));
#126097=DIRECTION('ref_axis',(0.,0.,1.));
#126098=DIRECTION('center_axis',(0.,-1.,0.));
#126099=DIRECTION('ref_axis',(0.,0.,1.));
#126100=DIRECTION('center_axis',(-1.,0.,0.));
#126101=DIRECTION('ref_axis',(0.,0.,1.));
#126102=DIRECTION('',(-1.,0.,0.));
#126103=DIRECTION('',(1.,0.,0.));
#126104=DIRECTION('center_axis',(0.,0.,1.));
#126105=DIRECTION('ref_axis',(1.,0.,0.));
#126106=DIRECTION('center_axis',(0.,0.,-1.));
#126107=DIRECTION('ref_axis',(-1.,0.,0.));
#126108=DIRECTION('',(0.,0.,-1.));
#126109=DIRECTION('center_axis',(0.,-1.,0.));
#126110=DIRECTION('ref_axis',(0.,0.,-1.));
#126111=DIRECTION('center_axis',(1.,0.,0.));
#126112=DIRECTION('ref_axis',(0.,0.,-1.));
#126113=DIRECTION('center_axis',(0.,-1.,0.));
#126114=DIRECTION('ref_axis',(0.,0.,-1.));
#126115=DIRECTION('center_axis',(0.,1.,0.));
#126116=DIRECTION('ref_axis',(0.,0.,-1.));
#126117=DIRECTION('center_axis',(-1.,0.,0.));
#126118=DIRECTION('ref_axis',(0.,0.,1.));
#126119=DIRECTION('',(-1.,0.,0.));
#126120=DIRECTION('',(1.,0.,0.));
#126121=DIRECTION('center_axis',(0.,1.,0.));
#126122=DIRECTION('ref_axis',(1.,0.,0.));
#126123=DIRECTION('',(1.,0.,0.));
#126124=DIRECTION('',(-1.,0.,0.));
#126125=DIRECTION('center_axis',(0.,0.,1.));
#126126=DIRECTION('ref_axis',(1.,0.,0.));
#126127=DIRECTION('',(0.,-1.,0.));
#126128=DIRECTION('center_axis',(0.,0.,-1.));
#126129=DIRECTION('ref_axis',(0.,-1.,0.));
#126130=DIRECTION('',(0.,-1.,0.));
#126131=DIRECTION('center_axis',(0.,-1.,0.));
#126132=DIRECTION('ref_axis',(0.,0.,-1.));
#126133=DIRECTION('center_axis',(0.,-1.,0.));
#126134=DIRECTION('ref_axis',(0.,0.,-1.));
#126135=DIRECTION('center_axis',(0.,0.,-1.));
#126136=DIRECTION('ref_axis',(0.,1.,0.));
#126137=DIRECTION('',(0.,0.,-1.));
#126138=DIRECTION('center_axis',(0.,0.,1.));
#126139=DIRECTION('ref_axis',(-1.,0.,0.));
#126140=DIRECTION('center_axis',(0.,0.,-1.));
#126141=DIRECTION('ref_axis',(0.,1.,0.));
#126142=DIRECTION('',(0.,0.,-1.));
#126143=DIRECTION('center_axis',(0.,0.,-1.));
#126144=DIRECTION('ref_axis',(0.,1.,0.));
#126145=DIRECTION('',(0.,0.,-1.));
#126146=DIRECTION('center_axis',(0.,0.,-1.));
#126147=DIRECTION('ref_axis',(0.,1.,0.));
#126148=DIRECTION('',(0.,0.,-1.));
#126149=DIRECTION('center_axis',(0.,0.,-1.));
#126150=DIRECTION('ref_axis',(0.,1.,0.));
#126151=DIRECTION('',(0.,0.,-1.));
#126152=DIRECTION('center_axis',(0.,0.,-1.));
#126153=DIRECTION('ref_axis',(0.,1.,0.));
#126154=DIRECTION('',(0.,0.,-1.));
#126155=DIRECTION('center_axis',(0.,0.,-1.));
#126156=DIRECTION('ref_axis',(0.,1.,0.));
#126157=DIRECTION('',(0.,0.,-1.));
#126158=DIRECTION('center_axis',(0.,0.,-1.));
#126159=DIRECTION('ref_axis',(0.,1.,0.));
#126160=DIRECTION('',(0.,0.,-1.));
#126161=DIRECTION('center_axis',(0.,0.,-1.));
#126162=DIRECTION('ref_axis',(0.,1.,0.));
#126163=DIRECTION('',(0.,0.,-1.));
#126164=DIRECTION('center_axis',(0.,0.,-1.));
#126165=DIRECTION('ref_axis',(0.,1.,0.));
#126166=DIRECTION('',(0.,0.,-1.));
#126167=DIRECTION('center_axis',(0.,0.,-1.));
#126168=DIRECTION('ref_axis',(0.,1.,0.));
#126169=DIRECTION('',(0.,0.,-1.));
#126170=DIRECTION('center_axis',(0.,0.,-1.));
#126171=DIRECTION('ref_axis',(0.,1.,0.));
#126172=DIRECTION('',(0.,0.,-1.));
#126173=DIRECTION('center_axis',(0.,0.,-1.));
#126174=DIRECTION('ref_axis',(0.,1.,0.));
#126175=DIRECTION('',(0.,0.,-1.));
#126176=DIRECTION('center_axis',(0.,0.,-1.));
#126177=DIRECTION('ref_axis',(0.,1.,0.));
#126178=DIRECTION('',(0.,0.,-1.));
#126179=DIRECTION('center_axis',(0.,0.,-1.));
#126180=DIRECTION('ref_axis',(0.,1.,0.));
#126181=DIRECTION('',(0.,0.,-1.));
#126182=DIRECTION('center_axis',(0.,0.,-1.));
#126183=DIRECTION('ref_axis',(0.,1.,0.));
#126184=DIRECTION('',(0.,0.,-1.));
#126185=DIRECTION('center_axis',(0.,0.,-1.));
#126186=DIRECTION('ref_axis',(0.,1.,0.));
#126187=DIRECTION('',(0.,0.,-1.));
#126188=DIRECTION('center_axis',(0.,0.,-1.));
#126189=DIRECTION('ref_axis',(0.,1.,0.));
#126190=DIRECTION('',(0.,0.,-1.));
#126191=DIRECTION('center_axis',(0.,0.,-1.));
#126192=DIRECTION('ref_axis',(0.,1.,0.));
#126193=DIRECTION('',(0.,0.,-1.));
#126194=DIRECTION('center_axis',(0.,0.,-1.));
#126195=DIRECTION('ref_axis',(0.,1.,0.));
#126196=DIRECTION('',(0.,0.,-1.));
#126197=DIRECTION('center_axis',(0.,0.,-1.));
#126198=DIRECTION('ref_axis',(1.,0.,0.));
#126199=DIRECTION('center_axis',(0.,0.,-1.));
#126200=DIRECTION('ref_axis',(0.,1.,0.));
#126201=DIRECTION('',(0.,0.,-1.));
#126202=DIRECTION('center_axis',(0.,0.,-1.));
#126203=DIRECTION('ref_axis',(0.,1.,0.));
#126204=DIRECTION('',(0.,0.,-1.));
#126205=DIRECTION('center_axis',(0.,0.,-1.));
#126206=DIRECTION('ref_axis',(0.,1.,0.));
#126207=DIRECTION('',(0.,0.,-1.));
#126208=DIRECTION('center_axis',(0.,0.,-1.));
#126209=DIRECTION('ref_axis',(0.,1.,0.));
#126210=DIRECTION('',(0.,0.,-1.));
#126211=DIRECTION('center_axis',(0.,0.,-1.));
#126212=DIRECTION('ref_axis',(0.,1.,0.));
#126213=DIRECTION('',(0.,0.,-1.));
#126214=DIRECTION('center_axis',(0.,0.,-1.));
#126215=DIRECTION('ref_axis',(0.,1.,0.));
#126216=DIRECTION('',(0.,0.,-1.));
#126217=DIRECTION('center_axis',(0.,0.,-1.));
#126218=DIRECTION('ref_axis',(0.,1.,0.));
#126219=DIRECTION('',(0.,0.,-1.));
#126220=DIRECTION('center_axis',(0.,0.,-1.));
#126221=DIRECTION('ref_axis',(0.,1.,0.));
#126222=DIRECTION('',(0.,0.,-1.));
#126223=DIRECTION('center_axis',(0.,0.,-1.));
#126224=DIRECTION('ref_axis',(0.,1.,0.));
#126225=DIRECTION('',(0.,0.,-1.));
#126226=DIRECTION('center_axis',(0.,0.,-1.));
#126227=DIRECTION('ref_axis',(0.,1.,0.));
#126228=DIRECTION('',(0.,0.,-1.));
#126229=DIRECTION('center_axis',(0.,0.,-1.));
#126230=DIRECTION('ref_axis',(0.,1.,0.));
#126231=DIRECTION('',(0.,0.,-1.));
#126232=DIRECTION('center_axis',(0.,0.,-1.));
#126233=DIRECTION('ref_axis',(0.,1.,0.));
#126234=DIRECTION('',(0.,0.,-1.));
#126235=DIRECTION('center_axis',(0.,0.,-1.));
#126236=DIRECTION('ref_axis',(0.,1.,0.));
#126237=DIRECTION('',(0.,0.,-1.));
#126238=DIRECTION('center_axis',(0.,0.,-1.));
#126239=DIRECTION('ref_axis',(0.,1.,0.));
#126240=DIRECTION('',(0.,0.,-1.));
#126241=DIRECTION('center_axis',(0.,0.,-1.));
#126242=DIRECTION('ref_axis',(0.,1.,0.));
#126243=DIRECTION('',(0.,0.,-1.));
#126244=DIRECTION('center_axis',(0.,0.,-1.));
#126245=DIRECTION('ref_axis',(0.,1.,0.));
#126246=DIRECTION('',(0.,0.,-1.));
#126247=DIRECTION('center_axis',(0.,0.,-1.));
#126248=DIRECTION('ref_axis',(0.,1.,0.));
#126249=DIRECTION('',(0.,0.,-1.));
#126250=DIRECTION('center_axis',(0.,0.,-1.));
#126251=DIRECTION('ref_axis',(0.,1.,0.));
#126252=DIRECTION('',(0.,0.,-1.));
#126253=DIRECTION('center_axis',(0.,0.,1.));
#126254=DIRECTION('ref_axis',(1.,-1.06448650818115E-14,0.));
#126255=DIRECTION('',(0.,0.,1.));
#126256=DIRECTION('center_axis',(0.,0.,1.));
#126257=DIRECTION('ref_axis',(1.,-1.06448650818115E-14,0.));
#126258=DIRECTION('',(0.,0.,1.));
#126259=DIRECTION('center_axis',(0.,0.,1.));
#126260=DIRECTION('ref_axis',(1.,-1.06448650818115E-14,0.));
#126261=DIRECTION('',(0.,0.,1.));
#126262=DIRECTION('center_axis',(0.,0.,1.));
#126263=DIRECTION('ref_axis',(1.,-1.06448650818115E-14,0.));
#126264=DIRECTION('',(0.,0.,1.));
#126265=DIRECTION('center_axis',(0.,0.,1.));
#126266=DIRECTION('ref_axis',(1.,-1.06448650818115E-14,0.));
#126267=DIRECTION('',(0.,0.,1.));
#126268=DIRECTION('center_axis',(0.,0.,1.));
#126269=DIRECTION('ref_axis',(1.,-1.06448650818115E-14,0.));
#126270=DIRECTION('',(0.,0.,1.));
#126271=DIRECTION('center_axis',(0.,0.,1.));
#126272=DIRECTION('ref_axis',(1.,-1.06448650818115E-14,0.));
#126273=DIRECTION('',(0.,0.,1.));
#126274=DIRECTION('center_axis',(0.,0.,1.));
#126275=DIRECTION('ref_axis',(1.,-1.06448650818115E-14,0.));
#126276=DIRECTION('',(0.,0.,1.));
#126277=DIRECTION('center_axis',(0.,0.,1.));
#126278=DIRECTION('ref_axis',(1.,-1.06448650818115E-14,0.));
#126279=DIRECTION('',(0.,0.,1.));
#126280=DIRECTION('center_axis',(0.,0.,1.));
#126281=DIRECTION('ref_axis',(1.,-1.06448650818115E-14,0.));
#126282=DIRECTION('',(0.,0.,1.));
#126283=DIRECTION('center_axis',(0.,0.,1.));
#126284=DIRECTION('ref_axis',(1.,-1.06448650818115E-14,0.));
#126285=DIRECTION('',(0.,0.,1.));
#126286=DIRECTION('center_axis',(0.,0.,1.));
#126287=DIRECTION('ref_axis',(1.,-1.06448650818115E-14,0.));
#126288=DIRECTION('',(0.,0.,1.));
#126289=DIRECTION('center_axis',(0.,0.,1.));
#126290=DIRECTION('ref_axis',(1.,-1.06448650818115E-14,0.));
#126291=DIRECTION('',(0.,0.,1.));
#126292=DIRECTION('center_axis',(0.,0.,1.));
#126293=DIRECTION('ref_axis',(1.,-1.06448650818115E-14,0.));
#126294=DIRECTION('',(0.,0.,1.));
#126295=DIRECTION('center_axis',(0.,0.,1.));
#126296=DIRECTION('ref_axis',(1.,-1.06448650818115E-14,0.));
#126297=DIRECTION('',(0.,0.,1.));
#126298=DIRECTION('center_axis',(0.,0.,1.));
#126299=DIRECTION('ref_axis',(1.,-1.06448650818115E-14,0.));
#126300=DIRECTION('',(0.,0.,1.));
#126301=DIRECTION('center_axis',(0.,0.,1.));
#126302=DIRECTION('ref_axis',(1.,-1.06448650818115E-14,0.));
#126303=DIRECTION('',(0.,0.,1.));
#126304=DIRECTION('center_axis',(0.,0.,1.));
#126305=DIRECTION('ref_axis',(1.,-1.06448650818115E-14,0.));
#126306=DIRECTION('',(0.,0.,1.));
#126307=DIRECTION('center_axis',(0.,0.,1.));
#126308=DIRECTION('ref_axis',(1.,-1.06448650818115E-14,0.));
#126309=DIRECTION('',(0.,0.,1.));
#126310=DIRECTION('center_axis',(0.,0.,1.));
#126311=DIRECTION('ref_axis',(1.,-1.06448650818115E-14,0.));
#126312=DIRECTION('center_axis',(0.,0.,-1.));
#126313=DIRECTION('ref_axis',(0.,1.,0.));
#126314=DIRECTION('',(0.,0.,-1.));
#126315=DIRECTION('center_axis',(0.,0.,1.));
#126316=DIRECTION('ref_axis',(-1.,0.,0.));
#126317=DIRECTION('center_axis',(0.,0.,-1.));
#126318=DIRECTION('ref_axis',(0.,1.,0.));
#126319=DIRECTION('',(0.,0.,-1.));
#126320=DIRECTION('center_axis',(0.,0.,-1.));
#126321=DIRECTION('ref_axis',(0.,1.,0.));
#126322=DIRECTION('',(0.,0.,-1.));
#126323=DIRECTION('center_axis',(0.,0.,-1.));
#126324=DIRECTION('ref_axis',(0.,1.,0.));
#126325=DIRECTION('',(0.,0.,-1.));
#126326=DIRECTION('center_axis',(0.,0.,-1.));
#126327=DIRECTION('ref_axis',(0.,1.,0.));
#126328=DIRECTION('',(0.,0.,-1.));
#126329=DIRECTION('center_axis',(0.,0.,-1.));
#126330=DIRECTION('ref_axis',(0.,1.,0.));
#126331=DIRECTION('',(0.,0.,-1.));
#126332=DIRECTION('center_axis',(0.,0.,-1.));
#126333=DIRECTION('ref_axis',(0.,1.,0.));
#126334=DIRECTION('',(0.,0.,-1.));
#126335=DIRECTION('center_axis',(0.,0.,-1.));
#126336=DIRECTION('ref_axis',(0.,1.,0.));
#126337=DIRECTION('',(0.,0.,-1.));
#126338=DIRECTION('center_axis',(0.,0.,-1.));
#126339=DIRECTION('ref_axis',(0.,1.,0.));
#126340=DIRECTION('',(0.,0.,-1.));
#126341=DIRECTION('center_axis',(0.,0.,-1.));
#126342=DIRECTION('ref_axis',(0.,1.,0.));
#126343=DIRECTION('',(0.,0.,-1.));
#126344=DIRECTION('center_axis',(0.,0.,-1.));
#126345=DIRECTION('ref_axis',(0.,1.,0.));
#126346=DIRECTION('',(0.,0.,-1.));
#126347=DIRECTION('center_axis',(0.,0.,-1.));
#126348=DIRECTION('ref_axis',(0.,1.,0.));
#126349=DIRECTION('',(0.,0.,-1.));
#126350=DIRECTION('center_axis',(0.,0.,-1.));
#126351=DIRECTION('ref_axis',(0.,1.,0.));
#126352=DIRECTION('',(0.,0.,-1.));
#126353=DIRECTION('center_axis',(0.,0.,-1.));
#126354=DIRECTION('ref_axis',(0.,1.,0.));
#126355=DIRECTION('',(0.,0.,-1.));
#126356=DIRECTION('center_axis',(0.,0.,-1.));
#126357=DIRECTION('ref_axis',(0.,1.,0.));
#126358=DIRECTION('',(0.,0.,-1.));
#126359=DIRECTION('center_axis',(0.,0.,-1.));
#126360=DIRECTION('ref_axis',(0.,1.,0.));
#126361=DIRECTION('',(0.,0.,-1.));
#126362=DIRECTION('center_axis',(0.,0.,-1.));
#126363=DIRECTION('ref_axis',(0.,1.,0.));
#126364=DIRECTION('',(0.,0.,-1.));
#126365=DIRECTION('center_axis',(0.,0.,-1.));
#126366=DIRECTION('ref_axis',(0.,1.,0.));
#126367=DIRECTION('',(0.,0.,-1.));
#126368=DIRECTION('center_axis',(0.18797044408042,-0.201600124387681,0.961261932045101));
#126369=DIRECTION('ref_axis',(-0.567481399358022,-0.82110585529472,-0.0612375357390118));
#126370=DIRECTION('center_axis',(0.,0.,1.));
#126371=DIRECTION('ref_axis',(-3.72570277863391E-14,-1.,0.));
#126372=DIRECTION('',(0.,0.,1.));
#126373=DIRECTION('center_axis',(0.,0.,1.));
#126374=DIRECTION('ref_axis',(-3.72570277863391E-14,-1.,0.));
#126375=DIRECTION('',(0.,0.,1.));
#126376=DIRECTION('center_axis',(0.,0.,1.));
#126377=DIRECTION('ref_axis',(-3.72570277863391E-14,-1.,0.));
#126378=DIRECTION('',(0.,0.,1.));
#126379=DIRECTION('center_axis',(0.,0.,1.));
#126380=DIRECTION('ref_axis',(-3.72570277863391E-14,-1.,0.));
#126381=DIRECTION('',(0.,0.,1.));
#126382=DIRECTION('center_axis',(0.,0.,1.));
#126383=DIRECTION('ref_axis',(-3.72570277863391E-14,-1.,0.));
#126384=DIRECTION('',(0.,0.,1.));
#126385=DIRECTION('center_axis',(0.,0.,1.));
#126386=DIRECTION('ref_axis',(-3.72570277863391E-14,-1.,0.));
#126387=DIRECTION('',(0.,0.,1.));
#126388=DIRECTION('center_axis',(0.,0.,1.));
#126389=DIRECTION('ref_axis',(-3.72570277863391E-14,-1.,0.));
#126390=DIRECTION('',(0.,0.,1.));
#126391=DIRECTION('center_axis',(0.,0.,1.));
#126392=DIRECTION('ref_axis',(-3.72570277863391E-14,-1.,0.));
#126393=DIRECTION('',(0.,0.,1.));
#126394=DIRECTION('center_axis',(0.,0.,1.));
#126395=DIRECTION('ref_axis',(-3.72570277863391E-14,-1.,0.));
#126396=DIRECTION('',(0.,0.,1.));
#126397=DIRECTION('center_axis',(0.,0.,1.));
#126398=DIRECTION('ref_axis',(-3.72570277863391E-14,-1.,0.));
#126399=DIRECTION('',(0.,0.,1.));
#126400=DIRECTION('center_axis',(0.,0.,1.));
#126401=DIRECTION('ref_axis',(-3.72570277863391E-14,-1.,0.));
#126402=DIRECTION('',(0.,0.,1.));
#126403=DIRECTION('center_axis',(0.,0.,1.));
#126404=DIRECTION('ref_axis',(-3.72570277863391E-14,-1.,0.));
#126405=DIRECTION('',(0.,0.,1.));
#126406=DIRECTION('center_axis',(0.,0.,1.));
#126407=DIRECTION('ref_axis',(-3.72570277863391E-14,-1.,0.));
#126408=DIRECTION('',(0.,0.,1.));
#126409=DIRECTION('center_axis',(0.,0.,1.));
#126410=DIRECTION('ref_axis',(-3.72570277863391E-14,-1.,0.));
#126411=DIRECTION('',(0.,0.,1.));
#126412=DIRECTION('center_axis',(0.,0.,1.));
#126413=DIRECTION('ref_axis',(-3.72570277863391E-14,-1.,0.));
#126414=DIRECTION('',(0.,0.,1.));
#126415=DIRECTION('center_axis',(0.,0.,1.));
#126416=DIRECTION('ref_axis',(-3.72570277863391E-14,-1.,0.));
#126417=DIRECTION('',(0.,0.,1.));
#126418=DIRECTION('center_axis',(0.,0.,1.));
#126419=DIRECTION('ref_axis',(-3.72570277863391E-14,-1.,0.));
#126420=DIRECTION('',(0.,0.,1.));
#126421=DIRECTION('center_axis',(0.,0.,1.));
#126422=DIRECTION('ref_axis',(-3.72570277863391E-14,-1.,0.));
#126423=DIRECTION('',(0.,0.,1.));
#126424=DIRECTION('center_axis',(0.,0.,1.));
#126425=DIRECTION('ref_axis',(-3.72570277863391E-14,-1.,0.));
#126426=DIRECTION('',(0.,0.,1.));
#126427=DIRECTION('center_axis',(0.,0.,1.));
#126428=DIRECTION('ref_axis',(-3.72570277863391E-14,-1.,0.));
#126429=DIRECTION('center_axis',(0.,0.,-1.));
#126430=DIRECTION('ref_axis',(0.,1.,0.));
#126431=DIRECTION('',(0.,0.,-1.));
#126432=DIRECTION('center_axis',(0.,0.,-1.));
#126433=DIRECTION('ref_axis',(1.,0.,0.));
#126434=DIRECTION('center_axis',(0.,0.,-1.));
#126435=DIRECTION('ref_axis',(0.,1.,0.));
#126436=DIRECTION('',(0.,0.,-1.));
#126437=DIRECTION('center_axis',(0.,0.,-1.));
#126438=DIRECTION('ref_axis',(0.,1.,0.));
#126439=DIRECTION('',(0.,0.,-1.));
#126440=DIRECTION('center_axis',(0.,0.,-1.));
#126441=DIRECTION('ref_axis',(0.,1.,0.));
#126442=DIRECTION('',(0.,0.,-1.));
#126443=DIRECTION('center_axis',(0.,0.,-1.));
#126444=DIRECTION('ref_axis',(0.,1.,0.));
#126445=DIRECTION('',(0.,0.,-1.));
#126446=DIRECTION('center_axis',(0.,0.,-1.));
#126447=DIRECTION('ref_axis',(0.,1.,0.));
#126448=DIRECTION('',(0.,0.,-1.));
#126449=DIRECTION('center_axis',(0.,0.,-1.));
#126450=DIRECTION('ref_axis',(0.,1.,0.));
#126451=DIRECTION('',(0.,0.,-1.));
#126452=DIRECTION('center_axis',(0.,0.,-1.));
#126453=DIRECTION('ref_axis',(0.,1.,0.));
#126454=DIRECTION('',(0.,0.,-1.));
#126455=DIRECTION('center_axis',(0.,0.,-1.));
#126456=DIRECTION('ref_axis',(0.,1.,0.));
#126457=DIRECTION('',(0.,0.,-1.));
#126458=DIRECTION('center_axis',(0.,0.,-1.));
#126459=DIRECTION('ref_axis',(0.,1.,0.));
#126460=DIRECTION('',(0.,0.,-1.));
#126461=DIRECTION('center_axis',(0.,0.,-1.));
#126462=DIRECTION('ref_axis',(0.,1.,0.));
#126463=DIRECTION('',(0.,0.,-1.));
#126464=DIRECTION('center_axis',(0.,0.,-1.));
#126465=DIRECTION('ref_axis',(0.,1.,0.));
#126466=DIRECTION('',(0.,0.,-1.));
#126467=DIRECTION('center_axis',(0.,0.,-1.));
#126468=DIRECTION('ref_axis',(0.,1.,0.));
#126469=DIRECTION('',(0.,0.,-1.));
#126470=DIRECTION('center_axis',(0.,0.,-1.));
#126471=DIRECTION('ref_axis',(0.,1.,0.));
#126472=DIRECTION('',(0.,0.,-1.));
#126473=DIRECTION('center_axis',(0.,0.,-1.));
#126474=DIRECTION('ref_axis',(0.,1.,0.));
#126475=DIRECTION('',(0.,0.,-1.));
#126476=DIRECTION('center_axis',(0.,0.,-1.));
#126477=DIRECTION('ref_axis',(0.,1.,0.));
#126478=DIRECTION('',(0.,0.,-1.));
#126479=DIRECTION('center_axis',(0.,0.,-1.));
#126480=DIRECTION('ref_axis',(0.,1.,0.));
#126481=DIRECTION('',(0.,0.,-1.));
#126482=DIRECTION('center_axis',(0.,0.,-1.));
#126483=DIRECTION('ref_axis',(0.,1.,0.));
#126484=DIRECTION('',(0.,0.,-1.));
#126485=DIRECTION('center_axis',(0.,0.,-1.));
#126486=DIRECTION('ref_axis',(0.,1.,0.));
#126487=DIRECTION('',(0.,0.,-1.));
#126488=DIRECTION('center_axis',(0.,0.,1.));
#126489=DIRECTION('ref_axis',(-1.,-2.66121627045289E-15,0.));
#126490=DIRECTION('',(0.,0.,1.));
#126491=DIRECTION('center_axis',(0.,0.,1.));
#126492=DIRECTION('ref_axis',(-1.,-2.66121627045289E-15,0.));
#126493=DIRECTION('',(0.,0.,1.));
#126494=DIRECTION('center_axis',(0.,0.,1.));
#126495=DIRECTION('ref_axis',(-1.,-2.66121627045289E-15,0.));
#126496=DIRECTION('',(0.,0.,1.));
#126497=DIRECTION('center_axis',(0.,0.,1.));
#126498=DIRECTION('ref_axis',(-1.,-2.66121627045289E-15,0.));
#126499=DIRECTION('',(0.,0.,1.));
#126500=DIRECTION('center_axis',(0.,0.,1.));
#126501=DIRECTION('ref_axis',(-1.,-2.66121627045289E-15,0.));
#126502=DIRECTION('',(0.,0.,1.));
#126503=DIRECTION('center_axis',(0.,0.,1.));
#126504=DIRECTION('ref_axis',(-1.,-2.66121627045289E-15,0.));
#126505=DIRECTION('',(0.,0.,1.));
#126506=DIRECTION('center_axis',(0.,0.,1.));
#126507=DIRECTION('ref_axis',(-1.,-2.66121627045289E-15,0.));
#126508=DIRECTION('',(0.,0.,1.));
#126509=DIRECTION('center_axis',(0.,0.,1.));
#126510=DIRECTION('ref_axis',(-1.,-2.66121627045289E-15,0.));
#126511=DIRECTION('',(0.,0.,1.));
#126512=DIRECTION('center_axis',(0.,0.,1.));
#126513=DIRECTION('ref_axis',(-1.,-2.66121627045289E-15,0.));
#126514=DIRECTION('',(0.,0.,1.));
#126515=DIRECTION('center_axis',(0.,0.,1.));
#126516=DIRECTION('ref_axis',(-1.,-2.66121627045289E-15,0.));
#126517=DIRECTION('',(0.,0.,1.));
#126518=DIRECTION('center_axis',(0.,0.,1.));
#126519=DIRECTION('ref_axis',(-1.,-2.66121627045289E-15,0.));
#126520=DIRECTION('',(0.,0.,1.));
#126521=DIRECTION('center_axis',(0.,0.,1.));
#126522=DIRECTION('ref_axis',(-1.,-2.66121627045289E-15,0.));
#126523=DIRECTION('',(0.,0.,1.));
#126524=DIRECTION('center_axis',(0.,0.,1.));
#126525=DIRECTION('ref_axis',(-1.,-2.66121627045289E-15,0.));
#126526=DIRECTION('',(0.,0.,1.));
#126527=DIRECTION('center_axis',(0.,0.,1.));
#126528=DIRECTION('ref_axis',(-1.,-2.66121627045289E-15,0.));
#126529=DIRECTION('',(0.,0.,1.));
#126530=DIRECTION('center_axis',(0.,0.,1.));
#126531=DIRECTION('ref_axis',(-1.,-2.66121627045289E-15,0.));
#126532=DIRECTION('',(0.,0.,1.));
#126533=DIRECTION('center_axis',(0.,0.,1.));
#126534=DIRECTION('ref_axis',(-1.,-2.66121627045289E-15,0.));
#126535=DIRECTION('',(0.,0.,1.));
#126536=DIRECTION('center_axis',(0.,0.,1.));
#126537=DIRECTION('ref_axis',(-1.,-2.66121627045289E-15,0.));
#126538=DIRECTION('',(0.,0.,1.));
#126539=DIRECTION('center_axis',(0.,0.,1.));
#126540=DIRECTION('ref_axis',(-1.,-2.66121627045289E-15,0.));
#126541=DIRECTION('',(0.,0.,1.));
#126542=DIRECTION('center_axis',(0.,0.,1.));
#126543=DIRECTION('ref_axis',(-1.,-2.66121627045289E-15,0.));
#126544=DIRECTION('',(0.,0.,1.));
#126545=DIRECTION('center_axis',(0.,0.,1.));
#126546=DIRECTION('ref_axis',(-1.,-2.66121627045289E-15,0.));
#126547=DIRECTION('center_axis',(0.,0.,1.));
#126548=DIRECTION('ref_axis',(-1.59672976227174E-14,1.,0.));
#126549=DIRECTION('',(0.,0.,1.));
#126550=DIRECTION('center_axis',(0.,0.,1.));
#126551=DIRECTION('ref_axis',(-1.59672976227174E-14,1.,0.));
#126552=DIRECTION('',(0.,0.,1.));
#126553=DIRECTION('center_axis',(0.,0.,1.));
#126554=DIRECTION('ref_axis',(-1.59672976227174E-14,1.,0.));
#126555=DIRECTION('',(0.,0.,1.));
#126556=DIRECTION('center_axis',(0.,0.,1.));
#126557=DIRECTION('ref_axis',(-1.59672976227174E-14,1.,0.));
#126558=DIRECTION('',(0.,0.,1.));
#126559=DIRECTION('center_axis',(0.,0.,1.));
#126560=DIRECTION('ref_axis',(-1.59672976227174E-14,1.,0.));
#126561=DIRECTION('',(0.,0.,1.));
#126562=DIRECTION('center_axis',(0.,0.,1.));
#126563=DIRECTION('ref_axis',(-1.59672976227174E-14,1.,0.));
#126564=DIRECTION('',(0.,0.,1.));
#126565=DIRECTION('center_axis',(0.,0.,1.));
#126566=DIRECTION('ref_axis',(-1.59672976227174E-14,1.,0.));
#126567=DIRECTION('',(0.,0.,1.));
#126568=DIRECTION('center_axis',(0.,0.,1.));
#126569=DIRECTION('ref_axis',(-1.59672976227174E-14,1.,0.));
#126570=DIRECTION('',(0.,0.,1.));
#126571=DIRECTION('center_axis',(0.,0.,1.));
#126572=DIRECTION('ref_axis',(-1.59672976227174E-14,1.,0.));
#126573=DIRECTION('',(0.,0.,1.));
#126574=DIRECTION('center_axis',(0.,0.,1.));
#126575=DIRECTION('ref_axis',(-1.59672976227174E-14,1.,0.));
#126576=DIRECTION('',(0.,0.,1.));
#126577=DIRECTION('center_axis',(0.,0.,1.));
#126578=DIRECTION('ref_axis',(-1.59672976227174E-14,1.,0.));
#126579=DIRECTION('',(0.,0.,1.));
#126580=DIRECTION('center_axis',(0.,0.,1.));
#126581=DIRECTION('ref_axis',(-1.59672976227174E-14,1.,0.));
#126582=DIRECTION('',(0.,0.,1.));
#126583=DIRECTION('center_axis',(0.,0.,1.));
#126584=DIRECTION('ref_axis',(-1.59672976227174E-14,1.,0.));
#126585=DIRECTION('',(0.,0.,1.));
#126586=DIRECTION('center_axis',(0.,0.,1.));
#126587=DIRECTION('ref_axis',(-1.59672976227174E-14,1.,0.));
#126588=DIRECTION('',(0.,0.,1.));
#126589=DIRECTION('center_axis',(0.,0.,1.));
#126590=DIRECTION('ref_axis',(-1.59672976227174E-14,1.,0.));
#126591=DIRECTION('',(0.,0.,1.));
#126592=DIRECTION('center_axis',(0.,0.,1.));
#126593=DIRECTION('ref_axis',(-1.59672976227174E-14,1.,0.));
#126594=DIRECTION('',(0.,0.,1.));
#126595=DIRECTION('center_axis',(0.,0.,1.));
#126596=DIRECTION('ref_axis',(-1.59672976227174E-14,1.,0.));
#126597=DIRECTION('',(0.,0.,1.));
#126598=DIRECTION('center_axis',(0.,0.,1.));
#126599=DIRECTION('ref_axis',(-1.59672976227174E-14,1.,0.));
#126600=DIRECTION('',(0.,0.,1.));
#126601=DIRECTION('center_axis',(0.,0.,1.));
#126602=DIRECTION('ref_axis',(-1.59672976227174E-14,1.,0.));
#126603=DIRECTION('',(0.,0.,1.));
#126604=DIRECTION('center_axis',(0.,0.,1.));
#126605=DIRECTION('ref_axis',(-1.59672976227174E-14,1.,0.));
#126606=DIRECTION('center_axis',(0.,-1.,0.));
#126607=DIRECTION('ref_axis',(0.,0.,-1.));
#126608=DIRECTION('',(-1.,0.,0.));
#126609=DIRECTION('',(0.,0.,1.));
#126610=DIRECTION('',(-1.,0.,0.));
#126611=DIRECTION('',(1.23917670974841E-16,0.,1.));
#126612=DIRECTION('',(-1.,0.,0.));
#126613=DIRECTION('',(0.,0.,-1.));
#126614=DIRECTION('',(-1.,0.,0.));
#126615=DIRECTION('',(0.,0.,-1.));
#126616=DIRECTION('center_axis',(-1.,0.,0.));
#126617=DIRECTION('ref_axis',(0.,0.,1.));
#126618=DIRECTION('',(0.,0.,-1.));
#126619=DIRECTION('center_axis',(1.,0.,0.));
#126620=DIRECTION('ref_axis',(0.,0.,1.));
#126621=DIRECTION('',(0.,1.,0.));
#126622=DIRECTION('',(0.,1.,0.));
#126623=DIRECTION('center_axis',(1.,0.,0.));
#126624=DIRECTION('ref_axis',(0.,0.,1.));
#126625=DIRECTION('center_axis',(0.,1.,0.));
#126626=DIRECTION('ref_axis',(0.,0.,1.));
#126627=DIRECTION('',(1.,0.,0.));
#126628=DIRECTION('',(-1.,0.,0.));
#126629=DIRECTION('',(0.,0.,-1.));
#126630=DIRECTION('',(1.,0.,0.));
#126631=DIRECTION('center_axis',(1.,0.,0.));
#126632=DIRECTION('ref_axis',(0.,0.,-1.));
#126633=DIRECTION('',(0.,1.,0.));
#126634=DIRECTION('',(0.,0.,-1.));
#126635=DIRECTION('',(0.,-1.,0.));
#126636=DIRECTION('',(0.,0.,1.));
#126637=DIRECTION('center_axis',(1.,0.,-1.23917670974841E-16));
#126638=DIRECTION('ref_axis',(-1.23917670974841E-16,0.,-1.));
#126639=DIRECTION('',(-2.06949078009218E-16,-1.,0.));
#126640=DIRECTION('',(1.23917670974841E-16,0.,1.));
#126641=DIRECTION('',(0.,-1.,0.));
#126642=DIRECTION('center_axis',(-1.,0.,0.));
#126643=DIRECTION('ref_axis',(0.,0.,1.));
#126644=DIRECTION('',(0.,1.,0.));
#126645=DIRECTION('',(0.,-1.,0.));
#126646=DIRECTION('',(0.,0.,-1.));
#126647=DIRECTION('center_axis',(0.,1.,0.));
#126648=DIRECTION('ref_axis',(1.,0.,0.));
#126649=DIRECTION('',(-1.,0.,0.));
#126650=DIRECTION('',(-1.,0.,0.));
#126651=DIRECTION('center_axis',(0.,0.,-1.));
#126652=DIRECTION('ref_axis',(-1.,0.,0.));
#126653=DIRECTION('',(-1.,0.,0.));
#126654=DIRECTION('center_axis',(0.,0.,-1.));
#126655=DIRECTION('ref_axis',(0.,-1.,0.));
#126656=DIRECTION('',(-1.,0.,0.));
#126657=DIRECTION('',(0.,1.,0.));
#126658=DIRECTION('center_axis',(-5.2588194754836E-31,1.51575151553259E-16,
-1.));
#126659=DIRECTION('ref_axis',(-1.,-3.46944695195361E-15,-1.08106823316757E-45));
#126660=DIRECTION('',(0.,1.,0.));
#126661=DIRECTION('center_axis',(-1.57764584264508E-30,1.51575151553259E-16,
-1.));
#126662=DIRECTION('ref_axis',(1.,1.04083408558608E-14,2.98046123744179E-45));
#126663=DIRECTION('center_axis',(0.,0.,-1.));
#126664=DIRECTION('ref_axis',(0.,1.,0.));
#126665=DIRECTION('',(-0.38268343236509,0.923879532511287,1.43936534571762E-16));
#126666=DIRECTION('',(0.923879532511287,0.38268343236509,5.95203168551499E-17));
#126667=DIRECTION('center_axis',(5.37437186243472E-32,-1.25279059425027E-16,
1.));
#126668=DIRECTION('ref_axis',(1.77635683940025E-15,1.,1.25279059425027E-16));
#126669=DIRECTION('',(-0.923879532511287,-0.38268343236509,-5.95203168551499E-17));
#126670=DIRECTION('',(-0.38268343236509,0.923879532511287,1.43936534571762E-16));
#126671=DIRECTION('center_axis',(1.93192743997308E-15,8.00230547157578E-16,
1.));
#126672=DIRECTION('ref_axis',(0.92387953251129,0.382683432365083,-2.09110319255771E-15));
#126673=DIRECTION('center_axis',(0.,0.,-1.));
#126674=DIRECTION('ref_axis',(0.,-1.,0.));
#126675=DIRECTION('center_axis',(0.,0.,-1.));
#126676=DIRECTION('ref_axis',(-1.,0.,0.));
#126677=DIRECTION('center_axis',(0.,0.,-1.));
#126678=DIRECTION('ref_axis',(-1.,0.,0.));
#126679=DIRECTION('center_axis',(0.,0.,1.));
#126680=DIRECTION('ref_axis',(0.,-1.,0.));
#126681=DIRECTION('',(0.,0.,1.));
#126682=DIRECTION('center_axis',(0.,0.,-1.));
#126683=DIRECTION('ref_axis',(0.,1.,0.));
#126684=DIRECTION('center_axis',(0.,0.,1.));
#126685=DIRECTION('ref_axis',(0.,-1.,0.));
#126686=DIRECTION('',(0.,0.,-1.));
#126687=DIRECTION('center_axis',(0.,0.,-1.));
#126688=DIRECTION('ref_axis',(-1.,0.,0.));
#126689=DIRECTION('center_axis',(-1.51575151553259E-16,1.51575151553257E-16,
-1.));
#126690=DIRECTION('ref_axis',(-1.,-7.79357634404829E-50,1.51575151553259E-16));
#126691=DIRECTION('center_axis',(-1.51575151553257E-16,-1.75293982516118E-30,
-1.));
#126692=DIRECTION('ref_axis',(-1.15648231731787E-14,1.,2.10194769648723E-45));
#126693=DIRECTION('center_axis',(-1.51575151553257E-16,-1.40235186012895E-30,
-1.));
#126694=DIRECTION('ref_axis',(-9.25185853854297E-15,1.,-3.50324616081204E-46));
#126695=DIRECTION('center_axis',(1.57764584264508E-30,-1.51575151553259E-16,
1.));
#126696=DIRECTION('ref_axis',(-1.,-1.04083408558608E-14,-2.98046123744179E-45));
#126697=DIRECTION('',(1.57764584264508E-30,-1.51575151553259E-16,1.));
#126698=DIRECTION('center_axis',(-1.57764584264508E-30,1.51575151553259E-16,
-1.));
#126699=DIRECTION('ref_axis',(1.,1.04083408558608E-14,2.98046123744179E-45));
#126700=DIRECTION('center_axis',(1.57764584264509E-30,-1.51575151553259E-16,
1.));
#126701=DIRECTION('ref_axis',(-1.,-1.04083408558608E-14,1.09360074820117E-47));
#126702=DIRECTION('',(-1.57764584264509E-30,1.51575151553259E-16,-1.));
#126703=DIRECTION('center_axis',(0.,0.,-1.));
#126704=DIRECTION('ref_axis',(-1.,0.,0.));
#126705=DIRECTION('center_axis',(1.51575151553259E-16,1.51575151553259E-16,
-1.));
#126706=DIRECTION('ref_axis',(-1.,-2.17577274266937E-49,-1.51575151553259E-16));
#126707=DIRECTION('center_axis',(1.51575151553259E-16,7.01175930064484E-31,
-1.));
#126708=DIRECTION('ref_axis',(4.62592926927148E-15,-1.,1.75162308040602E-46));
#126709=DIRECTION('center_axis',(1.51575151553259E-16,7.01175930064484E-31,
-1.));
#126710=DIRECTION('ref_axis',(4.62592926927148E-15,-1.,8.75811540203011E-47));
#126711=DIRECTION('center_axis',(5.2588194754836E-31,-1.51575151553259E-16,
1.));
#126712=DIRECTION('ref_axis',(1.,3.46944695195361E-15,1.08106823316757E-45));
#126713=DIRECTION('',(5.2588194754836E-31,-1.51575151553259E-16,1.));
#126714=DIRECTION('center_axis',(-5.2588194754836E-31,1.51575151553259E-16,
-1.));
#126715=DIRECTION('ref_axis',(-1.,-3.46944695195361E-15,-1.08106823316757E-45));
#126716=DIRECTION('center_axis',(5.25881947548361E-31,-1.51575151553259E-16,
1.));
#126717=DIRECTION('ref_axis',(1.,3.46944695195362E-15,6.8773879687219E-46));
#126718=DIRECTION('',(-5.25881947548361E-31,1.51575151553259E-16,-1.));
#126719=DIRECTION('center_axis',(0.,0.,-1.));
#126720=DIRECTION('ref_axis',(-1.,0.,0.));
#126721=DIRECTION('center_axis',(0.,3.03150303106518E-16,-1.));
#126722=DIRECTION('ref_axis',(-1.,0.,0.));
#126723=DIRECTION('center_axis',(0.,3.03150303106518E-16,-1.));
#126724=DIRECTION('ref_axis',(1.,0.,0.));
#126725=DIRECTION('center_axis',(0.,3.03150303106518E-16,-1.));
#126726=DIRECTION('ref_axis',(1.,0.,0.));
#126727=DIRECTION('center_axis',(0.,0.,1.));
#126728=DIRECTION('ref_axis',(0.,1.,0.));
#126729=DIRECTION('',(0.,0.,1.));
#126730=DIRECTION('center_axis',(0.,0.,-1.));
#126731=DIRECTION('ref_axis',(0.,-1.,0.));
#126732=DIRECTION('center_axis',(0.,0.,1.));
#126733=DIRECTION('ref_axis',(0.,1.,0.));
#126734=DIRECTION('center_axis',(0.,0.,-1.));
#126735=DIRECTION('ref_axis',(0.,-1.,0.));
#126736=DIRECTION('',(0.,0.,-1.));
#126737=DIRECTION('center_axis',(0.,0.,-1.));
#126738=DIRECTION('ref_axis',(0.,-1.,0.));
#126739=DIRECTION('center_axis',(0.,0.,-1.));
#126740=DIRECTION('ref_axis',(-1.,0.,0.));
#126741=DIRECTION('center_axis',(-0.868162779195992,-0.359604797490499,
-0.342020143325665));
#126742=DIRECTION('ref_axis',(0.315985410125154,0.130885442385879,-0.939692620785909));
#126743=DIRECTION('center_axis',(-0.868162779195992,-0.359604797490498,
-0.342020143325665));
#126744=DIRECTION('ref_axis',(0.38268343236509,-0.923879532511287,1.23981593187411E-17));
#126745=DIRECTION('center_axis',(-0.868162779195992,-0.359604797490498,
-0.342020143325665));
#126746=DIRECTION('ref_axis',(0.38268343236509,-0.923879532511287,1.23981593187411E-17));
#126747=DIRECTION('center_axis',(0.868162779195992,0.359604797490499,0.342020143325665));
#126748=DIRECTION('ref_axis',(0.38268343236509,-0.923879532511287,1.71567912920634E-16));
#126749=DIRECTION('center_axis',(-0.868162779195992,-0.359604797490499,
-0.342020143325665));
#126750=DIRECTION('ref_axis',(0.382683432365091,-0.923879532511286,0.));
#126751=DIRECTION('center_axis',(-0.868162779195992,-0.359604797490499,
-0.342020143325665));
#126752=DIRECTION('ref_axis',(0.382683432365091,-0.923879532511286,-1.45911995829617E-16));
#126753=DIRECTION('center_axis',(0.315985410125159,0.130885442385866,-0.93969262078591));
#126754=DIRECTION('ref_axis',(-0.38268343236509,0.923879532511287,0.));
#126755=DIRECTION('center_axis',(0.868162779195992,0.359604797490499,0.342020143325665));
#126756=DIRECTION('ref_axis',(0.382683432365091,-0.923879532511287,-1.04982926230618E-18));
#126757=DIRECTION('center_axis',(0.868162779195992,0.359604797490499,0.342020143325665));
#126758=DIRECTION('ref_axis',(0.382683432365091,-0.923879532511287,-1.04982926230618E-18));
#126759=DIRECTION('center_axis',(-0.868162779195992,-0.359604797490499,
-0.342020143325665));
#126760=DIRECTION('ref_axis',(0.382683432365091,-0.923879532511286,0.));
#126761=DIRECTION('center_axis',(-0.868162779195992,-0.359604797490499,
-0.342020143325665));
#126762=DIRECTION('ref_axis',(-0.382683432365091,0.923879532511286,1.1958072337233E-16));
#126763=DIRECTION('center_axis',(-0.868162779195992,-0.359604797490499,
-0.342020143325665));
#126764=DIRECTION('ref_axis',(-0.382683432365091,0.923879532511286,1.1958072337233E-16));
#126765=DIRECTION('center_axis',(0.315985410125158,0.130885442385866,-0.93969262078591));
#126766=DIRECTION('ref_axis',(-0.382683432365091,0.923879532511286,0.));
#126767=DIRECTION('center_axis',(0.868162779195992,0.359604797490499,0.342020143325665));
#126768=DIRECTION('ref_axis',(0.382683432365091,-0.923879532511286,-1.88969662411402E-16));
#126769=DIRECTION('center_axis',(0.868162779195992,0.359604797490499,0.342020143325665));
#126770=DIRECTION('ref_axis',(0.382683432365091,-0.923879532511286,-1.88969662411402E-16));
#126771=DIRECTION('center_axis',(-0.489406279098172,0.734660423998332,0.469846310392955));
#126772=DIRECTION('ref_axis',(0.692544317692113,6.99668119051868E-17,0.721375330900888));
#126773=DIRECTION('',(-0.868162779195992,-0.359604797490499,-0.342020143325665));
#126774=DIRECTION('',(-0.868162779195992,-0.359604797490499,-0.342020143325665));
#126775=DIRECTION('center_axis',(-0.315985410125159,-0.130885442385866,
0.93969262078591));
#126776=DIRECTION('ref_axis',(-0.382683432365091,0.923879532511286,-9.25792640816383E-18));
#126777=DIRECTION('',(-0.868162779195992,-0.359604797490499,-0.342020143325665));
#126778=DIRECTION('center_axis',(0.173420868973012,-0.865545866384198,0.469846310392956));
#126779=DIRECTION('ref_axis',(-0.980512713657042,-0.196455639666833,-1.27106818020157E-17));
#126780=DIRECTION('',(-0.868162779195992,-0.359604797490499,-0.342020143325665));
#126781=DIRECTION('center_axis',(0.489406279098172,-0.734660423998332,-0.469846310392956));
#126782=DIRECTION('ref_axis',(2.69783883395398E-17,0.538780036928174,-0.842446480085041));
#126783=DIRECTION('',(-0.868162779195992,-0.359604797490499,-0.342020143325665));
#126784=DIRECTION('center_axis',(0.315985410125159,0.130885442385866,-0.93969262078591));
#126785=DIRECTION('ref_axis',(4.33389766930712E-18,-0.990438688967689,-0.137953627701358));
#126786=DIRECTION('',(-0.868162779195992,-0.359604797490499,-0.342020143325665));
#126787=DIRECTION('center_axis',(-0.173420868973013,0.865545866384198,-0.469846310392955));
#126788=DIRECTION('ref_axis',(-0.938135943967436,-1.39985742631978E-17,
0.346267166558321));
#126789=DIRECTION('center_axis',(-0.868162779195992,-0.359604797490499,
-0.342020143325665));
#126790=DIRECTION('ref_axis',(0.38268343236509,-0.923879532511287,1.84142372121514E-16));
#126791=DIRECTION('',(-0.765494963633587,0.620300746446016,-0.171010071662833));
#126792=DIRECTION('center_axis',(-0.868162779195992,-0.359604797490499,
-0.342020143325665));
#126793=DIRECTION('ref_axis',(0.38268343236509,-0.923879532511287,4.70737048728512E-17));
#126794=DIRECTION('center_axis',(-0.868162779195992,-0.359604797490499,
-0.342020143325665));
#126795=DIRECTION('ref_axis',(0.38268343236509,-0.923879532511287,4.70737048728512E-17));
#126796=DIRECTION('center_axis',(-0.868162779195992,-0.359604797490499,
-0.342020143325665));
#126797=DIRECTION('ref_axis',(0.38268343236509,-0.923879532511287,4.70737048728512E-17));
#126798=DIRECTION('center_axis',(-0.868162779195992,-0.359604797490499,
-0.342020143325665));
#126799=DIRECTION('ref_axis',(0.38268343236509,-0.923879532511287,4.70737048728512E-17));
#126800=DIRECTION('center_axis',(-0.868162779195992,-0.359604797490499,
-0.342020143325665));
#126801=DIRECTION('ref_axis',(0.38268343236509,-0.923879532511287,4.70737048728512E-17));
#126802=DIRECTION('center_axis',(-0.868162779195992,-0.359604797490499,
-0.342020143325665));
#126803=DIRECTION('ref_axis',(0.38268343236509,-0.923879532511287,4.70737048728512E-17));
#126804=DIRECTION('center_axis',(-0.868162779195992,-0.359604797490499,
-0.342020143325665));
#126805=DIRECTION('ref_axis',(0.38268343236509,-0.923879532511287,4.70737048728512E-17));
#126806=DIRECTION('center_axis',(-0.868162779195992,-0.359604797490499,
-0.342020143325665));
#126807=DIRECTION('ref_axis',(0.38268343236509,-0.923879532511287,4.70737048728512E-17));
#126808=DIRECTION('center_axis',(-0.868162779195992,-0.359604797490499,
-0.342020143325665));
#126809=DIRECTION('ref_axis',(0.38268343236509,-0.923879532511287,4.70737048728512E-17));
#126810=DIRECTION('center_axis',(-0.868162779195992,-0.359604797490499,
-0.342020143325665));
#126811=DIRECTION('ref_axis',(0.38268343236509,-0.923879532511287,4.70737048728512E-17));
#126812=DIRECTION('center_axis',(-0.868162779195992,-0.359604797490499,
-0.342020143325665));
#126813=DIRECTION('ref_axis',(0.38268343236509,-0.923879532511287,4.70737048728512E-17));
#126814=DIRECTION('center_axis',(-0.868162779195992,-0.359604797490499,
-0.342020143325665));
#126815=DIRECTION('ref_axis',(0.38268343236509,-0.923879532511287,4.70737048728512E-17));
#126816=DIRECTION('center_axis',(0.868162779195992,0.3596047974905,0.342020143325665));
#126817=DIRECTION('ref_axis',(-0.382683432365091,0.923879532511286,1.50485916215286E-17));
#126818=DIRECTION('',(-0.884481838416343,0.399002491585443,-0.241844762647972));
#126819=DIRECTION('center_axis',(-0.868162779195992,-0.359604797490499,
-0.342020143325665));
#126820=DIRECTION('ref_axis',(-0.38268343236509,0.923879532511287,-1.64291196909507E-17));
#126821=DIRECTION('center_axis',(0.868162779195992,0.359604797490499,0.342020143325665));
#126822=DIRECTION('ref_axis',(-0.382683432365091,0.923879532511286,1.45911995829617E-16));
#126823=DIRECTION('',(-0.868162779195992,-0.359604797490499,-0.342020143325665));
#126824=DIRECTION('center_axis',(0.207767103126159,0.124142226786913,-0.970268796976874));
#126825=DIRECTION('ref_axis',(0.558629433047175,-0.829307248729054,0.0135145750520801));
#126826=DIRECTION('center_axis',(-0.382637984861907,0.923898340295368,-0.000171290056814656));
#126827=DIRECTION('ref_axis',(0.892345806659134,0.369618341309029,0.259039076407058));
#126828=DIRECTION('center_axis',(0.803015285854003,0.544766314634934,0.241652877334176));
#126829=DIRECTION('ref_axis',(-0.561404803271713,0.827541326377994,1.44349153113304E-16));
#126830=DIRECTION('center_axis',(0.0669619156029896,-0.957600006962959,
0.280211221265884));
#126831=DIRECTION('ref_axis',(4.52485696084786E-18,-0.280841561131646,-0.959754144320898));
#126832=DIRECTION('center_axis',(0.0693609655093104,-0.991908018991874,
0.106336909505741));
#126833=DIRECTION('ref_axis',(3.26002624601434E-19,-0.106593626600315,-0.994302669597237));
#126834=DIRECTION('center_axis',(0.997564050259817,0.0697564737442329,5.27888523360413E-13));
#126835=DIRECTION('ref_axis',(0.0681007776048493,-0.973886492346363,-0.216581125943402));
#126836=DIRECTION('center_axis',(-0.997974582307943,-0.063160693020796,
0.00758023247798644));
#126837=DIRECTION('ref_axis',(0.0591504890733341,-0.96518844253331,-0.254779296730542));
#126838=DIRECTION('center_axis',(0.424778659972963,-0.88724503879059,0.179886995564043));
#126839=DIRECTION('ref_axis',(0.901958432317943,0.431822864575925,-3.94566691152879E-17));
#126840=DIRECTION('center_axis',(0.240037971429266,-0.880321972893445,-0.409163776882944));
#126841=DIRECTION('ref_axis',(-3.13002221110141E-17,0.421486569103856,-0.906834644279243));
#126842=DIRECTION('center_axis',(-0.877516698994613,0.406924946271124,0.253725306360719));
#126843=DIRECTION('ref_axis',(-0.420691523302729,-0.907203749011891,-9.67787277356546E-18));
#126844=DIRECTION('center_axis',(-0.489478788704461,0.506750770244223,0.709657785320009));
#126845=DIRECTION('ref_axis',(4.89383052204965E-17,-0.813813546305325,0.581126072251065));
#126846=DIRECTION('',(-0.489348180803406,0.50550620705824,0.710634809568169));
#126847=DIRECTION('',(-0.0114108069061362,0.703450190767272,-0.710652955102024));
#126848=DIRECTION('center_axis',(-0.0122131352712882,0.704440676751092,
-0.709657785320015));
#126849=DIRECTION('ref_axis',(1.46094887112304E-18,0.709710717758151,0.704493220051982));
#126850=DIRECTION('center_axis',(0.332758619521767,0.908237397405967,-0.253725306359464));
#126851=DIRECTION('ref_axis',(-0.938963751759069,0.344016093929534,5.28665875370305E-17));
#126852=DIRECTION('',(-0.796920821694072,-0.55369873650563,-0.241526216263399));
#126853=DIRECTION('center_axis',(0.315985410124948,0.130885442386372,-0.93969262078591));
#126854=DIRECTION('ref_axis',(-0.947846471025676,1.41403886388541E-17,-0.31872726172101));
#126855=DIRECTION('center_axis',(0.868162779110503,0.359604797646558,0.342020143378583));
#126856=DIRECTION('ref_axis',(-0.305572312858413,-0.155701183571717,0.93935227846039));
#126857=DIRECTION('center_axis',(0.31598541012516,0.130885442385866,-0.939692620785909));
#126858=DIRECTION('ref_axis',(-0.947846471025611,1.76887230820116E-17,-0.318727261721202));
#126859=DIRECTION('center_axis',(0.315985410125156,0.130885442385873,-0.93969262078591));
#126860=DIRECTION('ref_axis',(-0.947846471025612,-3.00392539194327E-17,
-0.318727261721199));
#126861=DIRECTION('',(-0.315985410125159,-0.130885442385866,0.93969262078591));
#126862=DIRECTION('',(0.315985410125159,0.130885442385866,-0.93969262078591));
#126863=DIRECTION('center_axis',(0.315985410125156,0.130885442385873,-0.93969262078591));
#126864=DIRECTION('ref_axis',(-0.947846471025612,-3.00392539194327E-17,
-0.318727261721199));
#126865=DIRECTION('center_axis',(0.315985410126442,0.130885442386398,-0.939692620785404));
#126866=DIRECTION('ref_axis',(-0.947846471025169,5.20709087205665E-17,-0.318727261722518));
#126867=DIRECTION('center_axis',(0.868162779214872,0.359604797427702,0.342020143343766));
#126868=DIRECTION('ref_axis',(-0.32168655692517,-0.117021230958172,0.939587031944707));
#126869=DIRECTION('center_axis',(-0.315985410125157,-0.130885442385866,
0.93969262078591));
#126870=DIRECTION('ref_axis',(0.947846471025612,-2.96658686303126E-17,0.318727261721199));
#126871=DIRECTION('center_axis',(0.315985410125168,0.130885442385872,-0.939692620785906));
#126872=DIRECTION('ref_axis',(-0.947846471025608,-1.83411763673086E-17,
-0.318727261721211));
#126873=DIRECTION('',(-0.315985410125159,-0.130885442385866,0.93969262078591));
#126874=DIRECTION('',(0.315985410125159,0.130885442385866,-0.93969262078591));
#126875=DIRECTION('center_axis',(-0.483641379709625,0.875232579647714,0.00767771813624582));
#126876=DIRECTION('ref_axis',(-0.583254653729399,-0.328814087806622,0.742761943399699));
#126877=DIRECTION('center_axis',(0.382683432364578,-0.923879532511499,2.29641113224045E-12));
#126878=DIRECTION('ref_axis',(-0.336984534075557,-0.139583564321541,0.931105714924559));
#126879=DIRECTION('center_axis',(0.897231051697274,0.371645270195287,0.238445450809354));
#126880=DIRECTION('ref_axis',(-0.38268343236509,0.923879532511287,-5.599049694823E-17));
#126881=DIRECTION('center_axis',(0.89730838161834,0.371677301297369,0.238104288028965));
#126882=DIRECTION('ref_axis',(-0.38268343236509,0.923879532511287,1.43867310709335E-17));
#126883=DIRECTION('center_axis',(-0.333396134868013,0.924692779654905,-0.183821327677601));
#126884=DIRECTION('ref_axis',(-0.288398744889462,0.0856014296512129,0.953676338800461));
#126885=DIRECTION('center_axis',(0.382683432406618,-0.923879532494085,-1.8240588452439E-10));
#126886=DIRECTION('ref_axis',(-0.220298531052334,-0.0912506395364631,0.97115491967058));
#126887=DIRECTION('center_axis',(0.382683432365091,-0.923879532511286,0.));
#126888=DIRECTION('ref_axis',(-0.923879532511287,-0.382683432365088,0.));
#126889=DIRECTION('center_axis',(0.,0.,1.));
#126890=DIRECTION('ref_axis',(1.,0.,0.));
#126891=DIRECTION('center_axis',(0.207956138914421,-0.978138151943684,-1.20768627396809E-16));
#126892=DIRECTION('ref_axis',(-0.978138151943684,-0.207956138914421,-6.93889390390724E-15));
#126893=DIRECTION('center_axis',(0.,0.,-1.));
#126894=DIRECTION('ref_axis',(0.,1.,0.));
#126895=DIRECTION('center_axis',(0.,0.,1.));
#126896=DIRECTION('ref_axis',(1.,0.,0.));
#126897=DIRECTION('',(0.,-1.23467863058847E-16,1.));
#126898=DIRECTION('',(-5.72527083528863E-17,2.61688128046977E-16,-1.));
#126899=DIRECTION('center_axis',(-0.923879532511287,-0.38268343236509,7.73840192406943E-15));
#126900=DIRECTION('ref_axis',(0.38268343236509,-0.923879532511287,1.1683584407418E-30));
#126901=DIRECTION('center_axis',(-0.923879532511287,-0.38268343236509,-5.95203168551499E-17));
#126902=DIRECTION('ref_axis',(0.38268343236509,-0.923879532511287,-2.30223036877952E-33));
#126903=DIRECTION('',(0.923879532511287,0.38268343236509,5.95203168551499E-17));
#126904=DIRECTION('center_axis',(-0.382683432316632,0.923879532531359,-2.13765135084401E-10));
#126905=DIRECTION('ref_axis',(-0.219984261016821,-0.0911204641832574,0.971238377491289));
#126906=DIRECTION('center_axis',(0.418112262482855,-0.889598787804806,-0.183837245131902));
#126907=DIRECTION('ref_axis',(-0.143722924471232,-0.264610116560947,0.953585448292411));
#126908=DIRECTION('center_axis',(0.897308381618341,0.371677301297376,0.238104288028952));
#126909=DIRECTION('ref_axis',(-0.382683432365096,0.923879532511284,6.65294430386245E-16));
#126910=DIRECTION('center_axis',(0.382683432365091,-0.923879532511286,0.));
#126911=DIRECTION('ref_axis',(-0.923879532511286,-0.382683432365091,0.));
#126912=DIRECTION('center_axis',(-0.5446009241609,0.838695316192414,1.03551918447742E-16));
#126913=DIRECTION('ref_axis',(-0.838695316192414,-0.5446009241609,4.64565385920393E-32));
#126914=DIRECTION('center_axis',(3.84325181751198E-15,-6.93889390390722E-15,
1.));
#126915=DIRECTION('ref_axis',(5.60519385729927E-45,-1.,-6.93889390390722E-15));
#126916=DIRECTION('center_axis',(0.,0.,-1.));
#126917=DIRECTION('ref_axis',(0.,1.,0.));
#126918=DIRECTION('center_axis',(0.,0.,1.));
#126919=DIRECTION('ref_axis',(1.,0.,0.));
#126920=DIRECTION('',(5.72527083528863E-17,-2.61688128046977E-16,1.));
#126921=DIRECTION('',(0.,1.23467863058847E-16,-1.));
#126922=DIRECTION('center_axis',(-0.923879532511287,-0.38268343236509,0.));
#126923=DIRECTION('ref_axis',(0.38268343236509,-0.923879532511287,0.));
#126924=DIRECTION('center_axis',(0.923879532511287,0.38268343236509,5.95203168551498E-17));
#126925=DIRECTION('ref_axis',(-0.38268343236509,0.923879532511287,-1.86999513136017E-32));
#126926=DIRECTION('',(-0.923879532511287,-0.38268343236509,-5.95203168551499E-17));
#126927=DIRECTION('center_axis',(-0.38268343236509,0.923879532511287,-2.16840434497101E-16));
#126928=DIRECTION('ref_axis',(-5.66631362003227E-16,-2.40839253845808E-32,
1.));
#126929=DIRECTION('center_axis',(0.868162779195992,0.359604797490499,0.342020143325665));
#126930=DIRECTION('ref_axis',(-0.382683432365091,0.923879532511286,9.04008445983594E-17));
#126931=DIRECTION('center_axis',(-0.868162779195992,-0.359604797490499,
-0.342020143325665));
#126932=DIRECTION('ref_axis',(0.38268343236509,-0.923879532511287,-1.25544037310089E-16));
#126933=DIRECTION('center_axis',(-0.38268343236509,0.923879532511287,2.63677968348474E-16));
#126934=DIRECTION('ref_axis',(6.89023736195924E-16,-2.65450765404649E-32,
1.));
#126935=DIRECTION('center_axis',(-0.38268343236509,0.923879532511287,2.63677968348474E-16));
#126936=DIRECTION('ref_axis',(6.89023736195924E-16,-2.65450765404649E-32,
1.));
#126937=DIRECTION('center_axis',(0.868162779195992,0.359604797490499,0.342020143325665));
#126938=DIRECTION('ref_axis',(2.46876234589468E-17,0.689168323296269,-0.724601284959535));
#126939=DIRECTION('center_axis',(0.,0.,-1.));
#126940=DIRECTION('ref_axis',(0.,1.,0.));
#126941=DIRECTION('',(0.,1.23467863058847E-16,-1.));
#126942=DIRECTION('center_axis',(1.42788400384581E-31,1.65132260162873E-46,
-1.));
#126943=DIRECTION('ref_axis',(-1.15648231731787E-15,1.,-3.88938454866321E-62));
#126944=DIRECTION('',(0.,-1.23467863058847E-16,1.));
#126945=DIRECTION('center_axis',(0.,0.,-1.));
#126946=DIRECTION('ref_axis',(0.,1.,0.));
#126947=DIRECTION('',(0.,1.23467863058847E-16,-1.));
#126948=DIRECTION('center_axis',(0.,0.,-1.));
#126949=DIRECTION('ref_axis',(0.,1.,0.));
#126950=DIRECTION('',(0.,-1.23467863058847E-16,1.));
#126951=DIRECTION('center_axis',(0.,0.,-1.));
#126952=DIRECTION('ref_axis',(0.,1.,0.));
#126953=DIRECTION('',(0.,1.23467863058847E-16,-1.));
#126954=DIRECTION('center_axis',(4.28365201153745E-31,1.48619034146585E-45,
-1.));
#126955=DIRECTION('ref_axis',(-3.46944695195361E-15,1.,-6.22301527786114E-61));
#126956=DIRECTION('',(0.,-1.23467863058847E-16,1.));
#126957=DIRECTION('center_axis',(0.901958432317944,0.431822864575923,-2.31577870403057E-15));
#126958=DIRECTION('ref_axis',(-0.431822864575923,0.901958432317944,-1.23890881716737E-31));
#126959=DIRECTION('center_axis',(0.992770886529525,0.0694213030853436,0.0979114372140112));
#126960=DIRECTION('ref_axis',(0.0981482265735623,2.06880671420837E-18,-0.995171807086829));
#126961=DIRECTION('center_axis',(0.,0.,-1.));
#126962=DIRECTION('ref_axis',(0.,1.,0.));
#126963=DIRECTION('',(0.,1.23467863058847E-16,-1.));
#126964=DIRECTION('center_axis',(0.,0.,1.));
#126965=DIRECTION('ref_axis',(0.,1.,0.));
#126966=DIRECTION('',(0.,-1.23467863058847E-16,1.));
#126967=DIRECTION('center_axis',(0.,0.,-1.));
#126968=DIRECTION('ref_axis',(0.,1.,0.));
#126969=DIRECTION('',(0.,1.23467863058847E-16,-1.));
#126970=DIRECTION('center_axis',(0.,0.,1.));
#126971=DIRECTION('ref_axis',(0.,1.,0.));
#126972=DIRECTION('',(0.,-1.23467863058847E-16,1.));
#126973=DIRECTION('center_axis',(-0.0697564737441281,0.997564050259824,
1.23167101549909E-16));
#126974=DIRECTION('ref_axis',(1.76567270303392E-15,-9.8268693212801E-33,
1.));
#126975=DIRECTION('',(0.997564050259824,0.0697564737441281,8.61268274770809E-18));
#126976=DIRECTION('center_axis',(0.98660590693345,0.0689902057164932,0.147814532165213));
#126977=DIRECTION('ref_axis',(0.148167565509255,-4.52088703569399E-18,-0.988962270529599));
#126978=DIRECTION('center_axis',(0.747470084264675,0.664295471254592,-6.06224791631038E-16));
#126979=DIRECTION('ref_axis',(-0.664295471254592,0.747470084264675,9.59955536918487E-32));
#126980=DIRECTION('center_axis',(0.,0.,-1.));
#126981=DIRECTION('ref_axis',(0.,1.,0.));
#126982=DIRECTION('center_axis',(1.10148875902005E-31,1.02798428206033E-16,
-1.));
#126983=DIRECTION('ref_axis',(-5.32907051820075E-15,1.,1.02798428206033E-16));
#126984=DIRECTION('center_axis',(0.,-1.02798428206033E-16,1.));
#126985=DIRECTION('ref_axis',(0.,-1.,-1.02798428206033E-16));
#126986=DIRECTION('center_axis',(0.664295471254592,0.747470084264675,-2.95837698315952E-15));
#126987=DIRECTION('ref_axis',(-0.747470084264675,0.664295471254592,-5.32960101812494E-31));
#126988=DIRECTION('center_axis',(0.0689902057164909,0.986605906933449,-0.14781453216522));
#126989=DIRECTION('ref_axis',(4.37731061835132E-18,-0.148167565509262,-0.988962270529598));
#126990=DIRECTION('center_axis',(-0.997564050259824,0.0697564737441242,
8.61268274770762E-18));
#126991=DIRECTION('ref_axis',(8.63371404118299E-18,-2.27387344266631E-35,
1.));
#126992=DIRECTION('',(0.0697564737441243,0.997564050259824,1.23167101549909E-16));
#126993=DIRECTION('center_axis',(0.0694213030853413,0.992770886529525,-0.0979114372140151));
#126994=DIRECTION('ref_axis',(-3.30612675079287E-17,-0.0981482265735662,
-0.995171807086829));
#126995=DIRECTION('center_axis',(0.431822864575922,0.901958432317945,1.52768647491022E-15));
#126996=DIRECTION('ref_axis',(-0.901958432317945,0.431822864575922,-1.17097176385396E-30));
#126997=DIRECTION('center_axis',(0.,0.,-1.));
#126998=DIRECTION('ref_axis',(0.,1.,0.));
#126999=DIRECTION('',(0.,1.23467863058847E-16,-1.));
#127000=DIRECTION('center_axis',(0.,0.,1.));
#127001=DIRECTION('ref_axis',(0.,1.,0.));
#127002=DIRECTION('',(0.,-1.23467863058847E-16,1.));
#127003=DIRECTION('center_axis',(0.,0.,-1.));
#127004=DIRECTION('ref_axis',(0.,1.,0.));
#127005=DIRECTION('',(-1.53699078067169E-33,1.23467863058847E-16,-1.));
#127006=DIRECTION('center_axis',(0.,0.,1.));
#127007=DIRECTION('ref_axis',(0.,1.,0.));
#127008=DIRECTION('',(0.,-1.23467863058847E-16,1.));
#127009=DIRECTION('center_axis',(-0.997564050259824,-0.069756473744129,
-8.6126827477082E-18));
#127010=DIRECTION('ref_axis',(-0.069756473744129,0.997564050259824,-8.38175983410215E-37));
#127011=DIRECTION('',(1.53699078067169E-33,-1.23467863058847E-16,1.));
#127012=DIRECTION('',(-0.069756473744129,0.997564050259824,1.23167101549909E-16));
#127013=DIRECTION('center_axis',(-0.0689902057164932,0.98660590693345,0.147814532165213));
#127014=DIRECTION('ref_axis',(5.43774297173137E-18,0.148167565509255,-0.988962270529599));
#127015=DIRECTION('center_axis',(-0.664295471254594,0.747470084264672,2.08541328321077E-15));
#127016=DIRECTION('ref_axis',(-0.747470084264672,-0.664295471254594,-8.18696566210924E-31));
#127017=DIRECTION('center_axis',(0.,0.,-1.));
#127018=DIRECTION('ref_axis',(0.,1.,0.));
#127019=DIRECTION('center_axis',(0.,1.02798428206033E-16,-1.));
#127020=DIRECTION('ref_axis',(0.,1.,1.02798428206033E-16));
#127021=DIRECTION('center_axis',(0.,-1.02798428206033E-16,1.));
#127022=DIRECTION('ref_axis',(0.,-1.,-1.02798428206033E-16));
#127023=DIRECTION('center_axis',(-0.747470084264675,0.664295471254592,1.01845764994016E-15));
#127024=DIRECTION('ref_axis',(-0.664295471254592,-0.747470084264675,3.38786561065658E-30));
#127025=DIRECTION('center_axis',(-0.986605906933449,0.068990205716489,-0.147814532165218));
#127026=DIRECTION('ref_axis',(-0.14816756550926,4.04951997064162E-18,0.988962270529599));
#127027=DIRECTION('center_axis',(-0.0697564737441252,-0.997564050259824,
-1.23167101549909E-16));
#127028=DIRECTION('ref_axis',(-0.997564050259824,0.0697564737441252,1.56258158132391E-34));
#127029=DIRECTION('',(-0.997564050259824,0.0697564737441252,8.61268274770774E-18));
#127030=DIRECTION('center_axis',(-0.992770886529525,0.0694213030853416,
-0.0979114372140158));
#127031=DIRECTION('ref_axis',(-0.0981482265735668,2.47795101036114E-18,
0.995171807086829));
#127032=DIRECTION('center_axis',(-0.901958432317947,0.431822864575918,-5.06803925803546E-15));
#127033=DIRECTION('ref_axis',(-0.431822864575917,-0.901958432317947,6.66597837156041E-31));
#127034=DIRECTION('center_axis',(0.,-1.23467863058847E-16,1.));
#127035=DIRECTION('ref_axis',(0.,-1.,-1.05265590482978E-16));
#127036=DIRECTION('center_axis',(0.,1.04559862480377E-16,-1.));
#127037=DIRECTION('ref_axis',(0.,-1.,-1.04559862480377E-16));
#127038=DIRECTION('center_axis',(0.,-1.23467863058847E-16,1.));
#127039=DIRECTION('ref_axis',(0.,-1.,-1.05265590482978E-16));
#127040=DIRECTION('center_axis',(0.,1.04559862480377E-16,-1.));
#127041=DIRECTION('ref_axis',(0.,-1.,-1.04559862480377E-16));
#127042=DIRECTION('center_axis',(0.,0.,-1.));
#127043=DIRECTION('ref_axis',(0.,1.,0.));
#127044=DIRECTION('',(0.,1.23467863058847E-16,-1.));
#127045=DIRECTION('',(0.,-1.23467863058847E-16,1.));
#127046=DIRECTION('center_axis',(1.42788400384581E-31,-1.65132260162873E-46,
1.));
#127047=DIRECTION('ref_axis',(1.15648231731787E-15,1.,-3.88938454866321E-62));
#127048=DIRECTION('center_axis',(0.,0.,-1.));
#127049=DIRECTION('ref_axis',(0.,1.,0.));
#127050=DIRECTION('',(0.,1.23467863058847E-16,-1.));
#127051=DIRECTION('',(-1.53699078067169E-33,-1.23467863058847E-16,1.));
#127052=DIRECTION('center_axis',(0.,0.,1.));
#127053=DIRECTION('ref_axis',(0.,1.,0.));
#127054=DIRECTION('center_axis',(0.,0.,-1.));
#127055=DIRECTION('ref_axis',(0.,1.,0.));
#127056=DIRECTION('',(0.,1.23467863058847E-16,-1.));
#127057=DIRECTION('',(0.,-1.23467863058847E-16,1.));
#127058=DIRECTION('center_axis',(0.,0.,1.));
#127059=DIRECTION('ref_axis',(0.,1.,0.));
#127060=DIRECTION('center_axis',(0.,0.,-1.));
#127061=DIRECTION('ref_axis',(0.,1.,0.));
#127062=DIRECTION('',(0.,1.23467863058847E-16,-1.));
#127063=DIRECTION('',(0.,-1.23467863058847E-16,1.));
#127064=DIRECTION('center_axis',(4.28365201153745E-31,-1.48619034146585E-45,
1.));
#127065=DIRECTION('ref_axis',(3.46944695195361E-15,1.,-6.22301527786114E-61));
#127066=DIRECTION('center_axis',(0.,1.18842113532929E-16,-1.));
#127067=DIRECTION('ref_axis',(0.,1.,1.18842113532929E-16));
#127068=DIRECTION('center_axis',(0.,1.18842113532929E-16,-1.));
#127069=DIRECTION('ref_axis',(0.,-1.,-1.18842113532929E-16));
#127070=DIRECTION('center_axis',(0.,-1.18842113532929E-16,1.));
#127071=DIRECTION('ref_axis',(0.,1.,1.18842113532929E-16));
#127072=DIRECTION('center_axis',(0.901958432317944,-0.431822864575923,2.31577870403057E-15));
#127073=DIRECTION('ref_axis',(0.431822864575923,0.901958432317944,-1.23890881716737E-31));
#127074=DIRECTION('center_axis',(0.992770886529525,-0.0694213030853436,
-0.0979114372140112));
#127075=DIRECTION('ref_axis',(-0.0981482265735623,2.06880671420837E-18,
-0.995171807086829));
#127076=DIRECTION('center_axis',(0.,0.,-1.));
#127077=DIRECTION('ref_axis',(0.,1.,0.));
#127078=DIRECTION('',(0.,1.23467863058847E-16,-1.));
#127079=DIRECTION('',(0.,-1.23467863058847E-16,1.));
#127080=DIRECTION('center_axis',(0.,0.,-1.));
#127081=DIRECTION('ref_axis',(0.,1.,0.));
#127082=DIRECTION('center_axis',(0.,0.,-1.));
#127083=DIRECTION('ref_axis',(0.,1.,0.));
#127084=DIRECTION('',(0.,1.23467863058847E-16,-1.));
#127085=DIRECTION('',(0.,-1.23467863058847E-16,1.));
#127086=DIRECTION('center_axis',(0.,0.,-1.));
#127087=DIRECTION('ref_axis',(0.,1.,0.));
#127088=DIRECTION('center_axis',(0.0697564737441281,0.997564050259824,1.23167101549909E-16));
#127089=DIRECTION('ref_axis',(1.76567270303392E-15,9.8268693212801E-33,
-1.));
#127090=DIRECTION('',(-0.997564050259824,0.0697564737441281,8.61268274770809E-18));
#127091=DIRECTION('center_axis',(0.98660590693345,-0.0689902057164932,-0.147814532165213));
#127092=DIRECTION('ref_axis',(-0.148167565509255,-4.52088703569399E-18,
-0.988962270529599));
#127093=DIRECTION('center_axis',(0.747470084264675,-0.664295471254592,6.06224791631038E-16));
#127094=DIRECTION('ref_axis',(0.664295471254592,0.747470084264675,9.59955536918487E-32));
#127095=DIRECTION('center_axis',(0.,0.,-1.));
#127096=DIRECTION('ref_axis',(0.,1.,0.));
#127097=DIRECTION('center_axis',(0.,1.02798428206033E-16,-1.));
#127098=DIRECTION('ref_axis',(0.,-1.,-1.02798428206033E-16));
#127099=DIRECTION('center_axis',(1.10148875902005E-31,-1.02798428206033E-16,
1.));
#127100=DIRECTION('ref_axis',(5.32907051820075E-15,1.,1.02798428206033E-16));
#127101=DIRECTION('center_axis',(0.664295471254592,-0.747470084264675,2.95837698315952E-15));
#127102=DIRECTION('ref_axis',(0.747470084264675,0.664295471254592,-5.32960101812494E-31));
#127103=DIRECTION('center_axis',(0.0689902057164909,-0.986605906933449,
0.14781453216522));
#127104=DIRECTION('ref_axis',(-4.37731061835132E-18,-0.148167565509262,
-0.988962270529598));
#127105=DIRECTION('center_axis',(0.997564050259824,0.0697564737441242,8.61268274770761E-18));
#127106=DIRECTION('ref_axis',(-6.56745262755161E-34,1.23467863058847E-16,
-1.));
#127107=DIRECTION('',(-0.0697564737441243,0.997564050259824,1.23167101549909E-16));
#127108=DIRECTION('center_axis',(0.0694213030853413,-0.992770886529525,
0.0979114372140151));
#127109=DIRECTION('ref_axis',(3.30612675079287E-17,-0.0981482265735662,
-0.995171807086829));
#127110=DIRECTION('center_axis',(0.431822864575922,-0.901958432317945,-1.52768647491022E-15));
#127111=DIRECTION('ref_axis',(0.901958432317945,0.431822864575922,-1.17097176385396E-30));
#127112=DIRECTION('center_axis',(0.,1.18842113532929E-16,-1.));
#127113=DIRECTION('ref_axis',(0.,1.,1.18842113532929E-16));
#127114=DIRECTION('center_axis',(0.,-1.18842113532929E-16,1.));
#127115=DIRECTION('ref_axis',(0.,1.,1.18842113532929E-16));
#127116=DIRECTION('center_axis',(8.21698180771796E-33,1.18842113532929E-16,
-1.));
#127117=DIRECTION('ref_axis',(1.77635683940025E-15,-1.,-1.18842113532929E-16));
#127118=DIRECTION('center_axis',(-0.431822864575923,-0.901958432317944,
1.69742941656691E-16));
#127119=DIRECTION('ref_axis',(0.901958432317944,-0.431822864575923,7.92903681942359E-33));
#127120=DIRECTION('center_axis',(-0.0694213030853481,-0.992770886529524,
-0.0979114372140207));
#127121=DIRECTION('ref_axis',(-3.05094293527062E-18,0.0981482265735718,
-0.995171807086828));
#127122=DIRECTION('center_axis',(0.,0.,-1.));
#127123=DIRECTION('ref_axis',(0.,1.,0.));
#127124=DIRECTION('',(0.,1.23467863058847E-16,-1.));
#127125=DIRECTION('',(0.,-1.23467863058847E-16,1.));
#127126=DIRECTION('center_axis',(0.,0.,-1.));
#127127=DIRECTION('ref_axis',(0.,1.,0.));
#127128=DIRECTION('center_axis',(0.,0.,-1.));
#127129=DIRECTION('ref_axis',(0.,1.,0.));
#127130=DIRECTION('',(1.53699078067169E-33,1.23467863058847E-16,-1.));
#127131=DIRECTION('',(0.,-1.23467863058847E-16,1.));
#127132=DIRECTION('center_axis',(0.,0.,-1.));
#127133=DIRECTION('ref_axis',(0.,1.,0.));
#127134=DIRECTION('center_axis',(0.997564050259824,-0.069756473744129,-8.6126827477082E-18));
#127135=DIRECTION('ref_axis',(-2.43965120172245E-34,1.23467863058847E-16,
-1.));
#127136=DIRECTION('',(0.069756473744129,0.997564050259824,1.23167101549909E-16));
#127137=DIRECTION('center_axis',(-0.0689902057164932,-0.98660590693345,
-0.147814532165213));
#127138=DIRECTION('ref_axis',(-5.43774297173137E-18,0.148167565509255,-0.988962270529599));
#127139=DIRECTION('center_axis',(-0.664295471254594,-0.747470084264672,
-2.08541328321077E-15));
#127140=DIRECTION('ref_axis',(0.747470084264672,-0.664295471254594,-8.18696566210924E-31));
#127141=DIRECTION('center_axis',(0.,0.,-1.));
#127142=DIRECTION('ref_axis',(0.,1.,0.));
#127143=DIRECTION('center_axis',(0.,1.02798428206033E-16,-1.));
#127144=DIRECTION('ref_axis',(0.,-1.,-1.02798428206033E-16));
#127145=DIRECTION('center_axis',(0.,-1.02798428206033E-16,1.));
#127146=DIRECTION('ref_axis',(0.,1.,1.02798428206033E-16));
#127147=DIRECTION('center_axis',(-0.747470084264675,-0.664295471254592,
-1.01845764994016E-15));
#127148=DIRECTION('ref_axis',(0.664295471254592,-0.747470084264675,3.38786561065658E-30));
#127149=DIRECTION('center_axis',(-0.986605906933449,-0.068990205716489,
0.147814532165218));
#127150=DIRECTION('ref_axis',(0.14816756550926,4.04951997064162E-18,0.988962270529599));
#127151=DIRECTION('center_axis',(0.0697564737441252,-0.997564050259824,
-1.23167101549909E-16));
#127152=DIRECTION('ref_axis',(9.67324855439588E-34,1.23467863058847E-16,
-1.));
#127153=DIRECTION('',(0.997564050259824,0.0697564737441252,8.61268274770774E-18));
#127154=DIRECTION('center_axis',(-0.992770886529525,-0.0694213030853416,
0.0979114372140158));
#127155=DIRECTION('ref_axis',(0.0981482265735668,2.47795101036114E-18,0.995171807086829));
#127156=DIRECTION('center_axis',(-0.901958432317947,-0.431822864575918,
5.06803925803546E-15));
#127157=DIRECTION('ref_axis',(0.431822864575917,-0.901958432317947,6.66597837156041E-31));
#127158=DIRECTION('center_axis',(0.,1.18842113532929E-16,-1.));
#127159=DIRECTION('ref_axis',(1.22464679914735E-16,-1.,-1.18842113532929E-16));
#127160=DIRECTION('center_axis',(-8.21698180771796E-33,1.18842113532929E-16,
-1.));
#127161=DIRECTION('ref_axis',(-1.77635683940025E-15,-1.,-1.18842113532929E-16));
#127162=DIRECTION('center_axis',(8.21698180771796E-33,-1.18842113532929E-16,
1.));
#127163=DIRECTION('ref_axis',(1.77635683940025E-15,1.,1.18842113532929E-16));
#127164=DIRECTION('center_axis',(0.,-1.23467863058847E-16,1.));
#127165=DIRECTION('ref_axis',(0.,-1.,-1.21694324257719E-16));
#127166=DIRECTION('center_axis',(0.,-1.21202576459344E-16,1.));
#127167=DIRECTION('ref_axis',(0.,-1.,-1.21202576459344E-16));
#127168=DIRECTION('center_axis',(0.,1.23467863058847E-16,-1.));
#127169=DIRECTION('ref_axis',(0.923879532507622,0.382683432373937,0.));
#127170=DIRECTION('center_axis',(0.,1.26979970650999E-16,-1.));
#127171=DIRECTION('ref_axis',(0.,1.,1.26979970650999E-16));
#127172=DIRECTION('center_axis',(0.,-1.28766298379097E-16,1.));
#127173=DIRECTION('ref_axis',(0.,1.,1.28766298379097E-16));
#127174=DIRECTION('center_axis',(0.,1.55534083321291E-16,-1.));
#127175=DIRECTION('ref_axis',(0.923879532511285,0.382683432365093,6.24515698316632E-17));
#127176=DIRECTION('center_axis',(0.,1.28766298379097E-16,-1.));
#127177=DIRECTION('ref_axis',(0.,1.,1.28766298379097E-16));
#127178=DIRECTION('center_axis',(0.,-1.23467863058847E-16,1.));
#127179=DIRECTION('ref_axis',(1.22464679914735E-16,1.,1.21694324257719E-16));
#127180=DIRECTION('center_axis',(0.,-1.21202576459343E-16,1.));
#127181=DIRECTION('ref_axis',(0.,-1.,-1.21202576459343E-16));
#127182=DIRECTION('center_axis',(0.,-1.23467863058847E-16,1.));
#127183=DIRECTION('ref_axis',(0.,-1.,-1.21694324257719E-16));
#127184=DIRECTION('center_axis',(0.,-1.21202576459343E-16,1.));
#127185=DIRECTION('ref_axis',(0.,-1.,-1.21202576459343E-16));
#127186=DIRECTION('center_axis',(0.,-1.23467863058847E-16,1.));
#127187=DIRECTION('ref_axis',(0.,-1.,-1.05265590482978E-16));
#127188=DIRECTION('center_axis',(0.,-1.04559862480377E-16,1.));
#127189=DIRECTION('ref_axis',(0.,-1.,-1.04559862480377E-16));
#127190=DIRECTION('center_axis',(0.,-1.23467863058847E-16,1.));
#127191=DIRECTION('ref_axis',(0.,-1.,-1.05265590482978E-16));
#127192=DIRECTION('center_axis',(0.,-1.04559862480377E-16,1.));
#127193=DIRECTION('ref_axis',(0.,-1.,-1.04559862480377E-16));
#127194=DIRECTION('center_axis',(0.,0.,-1.));
#127195=DIRECTION('ref_axis',(0.,1.,0.));
#127196=DIRECTION('',(0.,1.23467863058847E-16,-1.));
#127197=DIRECTION('center_axis',(0.,0.,-1.));
#127198=DIRECTION('ref_axis',(0.,1.,0.));
#127199=DIRECTION('center_axis',(0.,1.18842113532929E-16,-1.));
#127200=DIRECTION('ref_axis',(0.,1.,1.18842113532929E-16));
#127201=DIRECTION('center_axis',(1.64339636154359E-32,-1.18842113532929E-16,
1.));
#127202=DIRECTION('ref_axis',(-3.5527136788005E-15,-1.,-1.18842113532929E-16));
#127203=DIRECTION('center_axis',(0.,1.18842113532929E-16,-1.));
#127204=DIRECTION('ref_axis',(0.,1.,1.18842113532929E-16));
#127205=DIRECTION('center_axis',(0.,-1.23467863058847E-16,1.));
#127206=DIRECTION('ref_axis',(0.,-1.,-1.21694324257719E-16));
#127207=DIRECTION('center_axis',(0.,1.21202576459343E-16,-1.));
#127208=DIRECTION('ref_axis',(0.,-1.,-1.21202576459343E-16));
#127209=DIRECTION('center_axis',(0.,0.,-1.));
#127210=DIRECTION('ref_axis',(0.,1.,0.));
#127211=DIRECTION('',(-0.654839500710631,0.0924107866510669,-0.75009697694337));
#127212=DIRECTION('',(0.425886568670936,-0.388175269924452,-0.817276324412236));
#127213=DIRECTION('center_axis',(0.189676565537595,0.200807286409187,0.961092729246685));
#127214=DIRECTION('ref_axis',(-0.938097396016776,0.326004004576076,0.117024205132558));
#127215=DIRECTION('',(0.425886568671724,-0.38817526992251,-0.817276324412748));
#127216=DIRECTION('',(-0.654839500710178,0.0924107866496375,-0.750096976943942));
#127217=DIRECTION('center_axis',(0.200678112292284,0.188576796953589,0.961336094660723));
#127218=DIRECTION('ref_axis',(0.903627963715395,-0.41466272120114,-0.107290870243625));
#127219=DIRECTION('center_axis',(0.,0.,1.));
#127220=DIRECTION('ref_axis',(-1.59672976227174E-14,1.,0.));
#127221=DIRECTION('center_axis',(0.,0.,-1.));
#127222=DIRECTION('ref_axis',(0.535742164068221,-0.844381627961847,0.));
#127223=DIRECTION('',(-0.425886568670953,-0.388175269924826,-0.81727632441205));
#127224=DIRECTION('center_axis',(-0.188086755331098,0.201586350617653,0.961242069259183));
#127225=DIRECTION('ref_axis',(0.629481269533852,-0.726522398490792,0.275533184566283));
#127226=DIRECTION('',(-0.425886568671143,-0.388175269923767,-0.817276324412454));
#127227=DIRECTION('',(0.654839500710178,0.0924107866496375,-0.750096976943942));
#127228=DIRECTION('center_axis',(0.,0.,1.));
#127229=DIRECTION('ref_axis',(-1.,-2.66121627045289E-15,0.));
#127230=DIRECTION('center_axis',(0.,0.,-1.));
#127231=DIRECTION('ref_axis',(0.,1.,0.));
#127232=DIRECTION('center_axis',(0.,0.,-1.));
#127233=DIRECTION('ref_axis',(0.,1.,0.));
#127234=DIRECTION('',(0.435638227654975,-0.396444898338133,-0.808115571677281));
#127235=DIRECTION('center_axis',(-0.201738744861899,-0.187890027474552,
0.96124857159694));
#127236=DIRECTION('ref_axis',(-0.681118454259118,0.732173219627526,0.000166517061419875));
#127237=DIRECTION('',(0.435638227812403,-0.396444898257199,-0.80811557163212));
#127238=DIRECTION('',(-0.141856700036149,0.637752802814605,-0.757065412733252));
#127239=DIRECTION('center_axis',(0.,0.,1.));
#127240=DIRECTION('ref_axis',(-3.72570277863391E-14,-1.,0.));
#127241=DIRECTION('center_axis',(0.,0.,-1.));
#127242=DIRECTION('ref_axis',(0.,1.,0.));
#127243=DIRECTION('center_axis',(0.,0.,-1.));
#127244=DIRECTION('ref_axis',(0.,1.,0.));
#127245=DIRECTION('',(0.141856700036448,0.637752802815158,-0.75706541273273));
#127246=DIRECTION('',(-0.435638227813814,-0.39644489825645,-0.808115571631727));
#127247=DIRECTION('center_axis',(0.200985107811872,-0.189230679181084,0.961143452609711));
#127248=DIRECTION('ref_axis',(0.32607544192224,0.938135929232121,0.116515168364468));
#127249=DIRECTION('',(-0.43563822781117,-0.396444898257902,-0.80811557163244));
#127250=DIRECTION('',(0.141856700036051,0.637752802814614,-0.757065412733263));
#127251=DIRECTION('center_axis',(0.188364697331784,-0.201014679344831,0.961307359530239));
#127252=DIRECTION('ref_axis',(-0.494479298944248,-0.865119964932013,-0.0840099350769745));
#127253=DIRECTION('center_axis',(0.,0.,-1.));
#127254=DIRECTION('ref_axis',(0.,-1.,0.));
#127255=DIRECTION('center_axis',(0.,0.,1.));
#127256=DIRECTION('ref_axis',(1.,-1.06448650818115E-14,0.));
#127257=DIRECTION('center_axis',(0.,0.,-1.));
#127258=DIRECTION('ref_axis',(0.,1.,0.));
#127259=DIRECTION('center_axis',(0.,0.,-1.));
#127260=DIRECTION('ref_axis',(0.,1.,0.));
#127261=DIRECTION('center_axis',(0.,1.18842113532929E-16,-1.));
#127262=DIRECTION('ref_axis',(0.927815008667248,0.373040627401085,4.43329365939947E-17));
#127263=DIRECTION('center_axis',(0.,1.28766298379097E-16,-1.));
#127264=DIRECTION('ref_axis',(0.923879532511286,0.382683432365091,4.92767290366603E-17));
#127265=DIRECTION('',(-0.141856700036947,0.637752802814889,-0.757065412732863));
#127266=DIRECTION('',(0.654839500710788,0.0924107866506205,-0.750096976943288));
#127267=DIRECTION('center_axis',(0.,0.,1.));
#127268=DIRECTION('ref_axis',(1.,0.,0.));
#127269=DIRECTION('center_axis',(0.,0.,1.));
#127270=DIRECTION('ref_axis',(1.,0.,0.));
#127271=DIRECTION('',(0.,-1.,0.));
#127272=DIRECTION('',(1.,0.,0.));
#127273=DIRECTION('center_axis',(-1.,0.,0.));
#127274=DIRECTION('ref_axis',(0.,0.,1.));
#127275=DIRECTION('center_axis',(-1.,-1.73472347597681E-16,0.));
#127276=DIRECTION('ref_axis',(1.73472347597681E-16,-1.,0.));
#127277=DIRECTION('center_axis',(-1.,0.,4.35694038576837E-17));
#127278=DIRECTION('ref_axis',(4.35694038576837E-17,0.,1.));
#127279=DIRECTION('center_axis',(-1.,0.,-2.60208521396521E-16));
#127280=DIRECTION('ref_axis',(-2.60208521396521E-16,0.,1.));
#127281=DIRECTION('center_axis',(-1.,0.,0.));
#127282=DIRECTION('ref_axis',(0.,0.,1.));
#127283=DIRECTION('center_axis',(-1.,0.,0.));
#127284=DIRECTION('ref_axis',(0.,0.,1.));
#127285=DIRECTION('center_axis',(0.,0.,-1.));
#127286=DIRECTION('ref_axis',(-1.,0.,0.));
#127287=DIRECTION('center_axis',(0.,0.,-1.));
#127288=DIRECTION('ref_axis',(-1.,0.,0.));
#127289=DIRECTION('center_axis',(0.,0.,1.));
#127290=DIRECTION('ref_axis',(1.,0.,0.));
#127291=DIRECTION('center_axis',(-1.,0.,0.));
#127292=DIRECTION('ref_axis',(0.,0.,1.));
#127293=DIRECTION('center_axis',(-1.,0.,0.));
#127294=DIRECTION('ref_axis',(0.,0.,1.));
#127295=DIRECTION('center_axis',(1.,0.,0.));
#127296=DIRECTION('ref_axis',(0.,0.,-1.));
#127297=DIRECTION('center_axis',(0.,1.,0.));
#127298=DIRECTION('ref_axis',(0.,0.,-1.));
#127299=DIRECTION('center_axis',(1.,0.,0.));
#127300=DIRECTION('ref_axis',(0.,0.,-1.));
#127301=DIRECTION('center_axis',(0.,1.,0.));
#127302=DIRECTION('ref_axis',(0.,0.,-1.));
#127303=DIRECTION('center_axis',(0.,1.,0.));
#127304=DIRECTION('ref_axis',(0.,0.,1.));
#127305=DIRECTION('center_axis',(5.58059449121998E-15,0.707106781186545,
-0.70710678118655));
#127306=DIRECTION('ref_axis',(1.98375245311818E-13,0.70710678118655,0.707106781186545));
#127307=DIRECTION('center_axis',(0.,1.,0.));
#127308=DIRECTION('ref_axis',(0.,0.,1.));
#127309=DIRECTION('center_axis',(9.84810792568227E-16,0.707106781186547,
0.707106781186548));
#127310=DIRECTION('ref_axis',(-8.25384288032917E-14,-0.707106781186548,
0.707106781186547));
#127311=DIRECTION('center_axis',(0.,0.,-1.));
#127312=DIRECTION('ref_axis',(-1.,0.,0.));
#131308=CARTESIAN_POINT('',(0.,0.,0.));
#131309=CARTESIAN_POINT('Origin',(-44.5079524583208,31.5404524382925,-39.8944822890418));
#131310=CARTESIAN_POINT('',(-46.5079524583208,31.5404524382925,-40.4194822890418));
#131311=CARTESIAN_POINT('Origin',(-44.5079524583208,31.5404524382925,-40.4194822890418));
#131312=CARTESIAN_POINT('',(-45.9829524583208,31.5404524382925,-39.8944822890418));
#131313=CARTESIAN_POINT('',(-45.9829524583208,31.5404524382925,-39.8944822890418));
#131314=CARTESIAN_POINT('Origin',(-44.5079524583208,31.5404524382925,-39.8944822890418));
#131315=CARTESIAN_POINT('Origin',(-44.5079524583208,31.5404524382925,-39.8944822890418));
#131316=CARTESIAN_POINT('Origin',(-44.5079524583208,31.5404524382925,-39.8944822890418));
#131317=CARTESIAN_POINT('',(-46.5079524583208,31.5404524382925,-55.24995));
#131318=CARTESIAN_POINT('Origin',(-44.5079524583208,31.5404524382925,-55.24995));
#131319=CARTESIAN_POINT('',(-46.5079524583208,31.5404524382925,-39.8944822890418));
#131320=CARTESIAN_POINT('Origin',(0.,45.41999998,-55.24995));
#131321=CARTESIAN_POINT('',(-47.0079524583208,31.5404524382925,-55.24995));
#131322=CARTESIAN_POINT('Origin',(-44.5079524583208,31.5404524382925,-55.24995));
#131323=CARTESIAN_POINT('Origin',(-44.5079524583208,31.5404524382925,-48.1788821881345));
#131324=CARTESIAN_POINT('',(-47.0079524583208,31.5404524382925,-179.64995));
#131325=CARTESIAN_POINT('Origin',(-44.5079524583208,31.5404524382925,-179.64995));
#131326=CARTESIAN_POINT('',(-47.0079524583208,31.5404524382925,-48.1788821881345));
#131327=CARTESIAN_POINT('Origin',(-44.5079524583208,31.5404524382925,-179.64995));
#131328=CARTESIAN_POINT('Origin',(44.5079524583208,31.5404524382925,-39.8944822890418));
#131329=CARTESIAN_POINT('',(46.5079524583208,31.5404524382925,-40.4194822890418));
#131330=CARTESIAN_POINT('Origin',(44.5079524583208,31.5404524382925,-40.4194822890418));
#131331=CARTESIAN_POINT('',(45.9829524583208,31.5404524382925,-39.8944822890418));
#131332=CARTESIAN_POINT('',(45.9829524583208,31.5404524382925,-39.8944822890418));
#131333=CARTESIAN_POINT('Origin',(44.5079524583208,31.5404524382925,-39.8944822890418));
#131334=CARTESIAN_POINT('Origin',(44.5079524583208,31.5404524382925,-39.8944822890418));
#131335=CARTESIAN_POINT('Origin',(44.5079524583208,31.5404524382925,-39.8944822890418));
#131336=CARTESIAN_POINT('',(46.5079524583208,31.5404524382925,-55.24995));
#131337=CARTESIAN_POINT('Origin',(44.5079524583208,31.5404524382925,-55.24995));
#131338=CARTESIAN_POINT('',(46.5079524583208,31.5404524382925,-39.8944822890418));
#131339=CARTESIAN_POINT('Origin',(0.,45.41999998,-55.24995));
#131340=CARTESIAN_POINT('',(47.0079524583208,31.5404524382925,-55.24995));
#131341=CARTESIAN_POINT('Origin',(44.5079524583208,31.5404524382925,-55.24995));
#131342=CARTESIAN_POINT('Origin',(44.5079524583208,31.5404524382925,-48.1788821881345));
#131343=CARTESIAN_POINT('',(47.0079524583208,31.5404524382925,-179.64995));
#131344=CARTESIAN_POINT('Origin',(44.5079524583208,31.5404524382925,-179.64995));
#131345=CARTESIAN_POINT('',(47.0079524583208,31.5404524382925,-48.1788821881345));
#131346=CARTESIAN_POINT('Origin',(44.5079524583208,31.5404524382925,-179.64995));
#131347=CARTESIAN_POINT('Origin',(-57.8922230010149,-38.7834964612722,-55.24995));
#131348=CARTESIAN_POINT('',(-52.9112495105562,-38.347717747534,-54.9585476429427));
#131349=CARTESIAN_POINT('',(-52.9112495105562,-38.347717747534,-52.64995));
#131350=CARTESIAN_POINT('',(-52.9112495105562,-38.347717747534,-52.64995));
#131351=CARTESIAN_POINT('',(-53.3256899305366,-36.7471331056238,-52.64995));
#131352=CARTESIAN_POINT('Origin',(-57.8922230010149,-38.7834964612722,-52.64995));
#131353=CARTESIAN_POINT('',(-53.3256899305366,-36.7471331056238,-54.8057004429536));
#131354=CARTESIAN_POINT('',(-53.3256899305366,-36.7471331056238,-55.24995));
#131355=CARTESIAN_POINT('',(-53.1795531264094,-37.1129448598587,-54.74995));
#131356=CARTESIAN_POINT('Ctrl Pts',(-53.1795531264094,-37.1129448598586,
-54.74995));
#131357=CARTESIAN_POINT('Ctrl Pts',(-53.2037450099618,-37.0446989219713,
-54.7499500137454));
#131358=CARTESIAN_POINT('Ctrl Pts',(-53.2291153576388,-36.9778304553028,
-54.7554548649733));
#131359=CARTESIAN_POINT('Ctrl Pts',(-53.2555724802117,-36.9122732840979,
-54.7662993117295));
#131360=CARTESIAN_POINT('Ctrl Pts',(-53.2781697189553,-36.8562803829428,
-54.7755616399256));
#131361=CARTESIAN_POINT('Ctrl Pts',(-53.3015600056389,-36.8012443229211,
-54.7887202323915));
#131362=CARTESIAN_POINT('Ctrl Pts',(-53.3256899305359,-36.7471331056253,
-54.8057004429567));
#131363=CARTESIAN_POINT('',(-53.0181298732915,-37.6685004154142,-54.74995));
#131364=CARTESIAN_POINT('Origin',(-57.8922230010149,-38.7834964612722,-54.74995));
#131365=CARTESIAN_POINT('Ctrl Pts',(-52.9112495105562,-38.347717747534,
-54.9585476429427));
#131366=CARTESIAN_POINT('Ctrl Pts',(-52.9283556128915,-38.1521941031454,
-54.8226237570584));
#131367=CARTESIAN_POINT('Ctrl Pts',(-52.9626456126999,-37.9110442829472,
-54.7499500131212));
#131368=CARTESIAN_POINT('Ctrl Pts',(-53.0181298732915,-37.6685004154142,
-54.74995));
#131369=CARTESIAN_POINT('Origin',(-25.30491873532,-68.8967968514054,-55.24995));
#131370=CARTESIAN_POINT('',(-24.0682702937655,-66.1635386067456,-54.74995));
#131371=CARTESIAN_POINT('',(-24.579016252936,-65.9859437829616,-54.74995));
#131372=CARTESIAN_POINT('Origin',(-25.30491873532,-68.8967968514054,-54.74995));
#131373=CARTESIAN_POINT('',(-24.0682702937655,-66.1635386067456,-52.64995));
#131374=CARTESIAN_POINT('',(-24.0682702937655,-66.1635386067456,-55.24995));
#131375=CARTESIAN_POINT('',(-25.043451507077,-65.9082127571302,-52.64995));
#131376=CARTESIAN_POINT('Origin',(-25.30491873532,-68.8967968514054,-52.64995));
#131377=CARTESIAN_POINT('',(-25.043451507077,-65.9082127571302,-54.8278826162281));
#131378=CARTESIAN_POINT('',(-25.043451507077,-65.9082127571302,-55.24995));
#131379=CARTESIAN_POINT('Ctrl Pts',(-24.579016252936,-65.9859437829616,
-54.74995));
#131380=CARTESIAN_POINT('Ctrl Pts',(-24.7361092859404,-65.946768249212,
-54.749950009163));
#131381=CARTESIAN_POINT('Ctrl Pts',(-24.8931309886626,-65.9213640983868,
-54.7753029040978));
#131382=CARTESIAN_POINT('Ctrl Pts',(-25.043451507077,-65.9082127571302,
-54.8278826162281));
#131383=CARTESIAN_POINT('Origin',(-25.30491873532,-68.8967968514054,-54.74995));
#131384=CARTESIAN_POINT('',(-24.2743783673579,-66.6190816475223,-55.24995));
#131385=CARTESIAN_POINT('Origin',(-24.2743783673579,-66.6190816475223,-54.74995));
#131386=CARTESIAN_POINT('',(-24.7,-66.4710859610356,-55.24995));
#131387=CARTESIAN_POINT('Origin',(-24.7,-66.4710859610356,-54.74995));
#131388=CARTESIAN_POINT('Origin',(-25.30491873532,-68.8967968514054,-55.24995));
#131389=CARTESIAN_POINT('Ctrl Pts',(-24.7,-66.4710859610356,-55.24995));
#131390=CARTESIAN_POINT('Ctrl Pts',(-24.579016252936,-65.9859437829616,
-55.24995));
#131391=CARTESIAN_POINT('Ctrl Pts',(-24.579016252936,-65.9859437829616,
-54.74995));
#131392=CARTESIAN_POINT('Ctrl Pts',(-24.7654791450057,-66.4384278647148,
-55.24995));
#131393=CARTESIAN_POINT('Ctrl Pts',(-24.67310951117,-65.9624790000681,-55.2343403176332));
#131394=CARTESIAN_POINT('Ctrl Pts',(-24.7361092859404,-65.946768249212,
-54.749950009163));
#131395=CARTESIAN_POINT('Ctrl Pts',(-24.8308799729202,-66.4172697443503,
-55.2626259569449));
#131396=CARTESIAN_POINT('Ctrl Pts',(-24.7709452774937,-65.9414368141194,
-55.24317591549));
#131397=CARTESIAN_POINT('Ctrl Pts',(-24.8931309886626,-65.9213640983868,
-54.7753029040978));
#131398=CARTESIAN_POINT('Ctrl Pts',(-24.8935146892254,-66.4063101061761,
-55.2889163081141));
#131399=CARTESIAN_POINT('Ctrl Pts',(-24.8576734148988,-65.9244662341272,
-55.273872259957));
#131400=CARTESIAN_POINT('Ctrl Pts',(-25.043451507077,-65.9082127571302,
-54.8278826162281));
#131401=CARTESIAN_POINT('',(-24.8935146892254,-66.4063101061761,-55.2889163081141));
#131402=CARTESIAN_POINT('Origin',(-25.0870293784509,-66.4063101061761,-54.8278826162281));
#131403=CARTESIAN_POINT('Ctrl Pts',(-24.8935146892254,-66.4063101061761,
-55.2889163081141));
#131404=CARTESIAN_POINT('Ctrl Pts',(-24.870965187297,-66.410255751606,-55.2794513602487));
#131405=CARTESIAN_POINT('Ctrl Pts',(-24.8480399226665,-66.4155232380401,
-55.271770535973));
#131406=CARTESIAN_POINT('Ctrl Pts',(-24.8248933073001,-66.4221732960834,
-55.2657995463271));
#131407=CARTESIAN_POINT('Ctrl Pts',(-24.8005026591807,-66.4291807666419,
-55.2595076412226));
#131408=CARTESIAN_POINT('Ctrl Pts',(-24.7758648518602,-66.4377234172793,
-55.2551132760505));
#131409=CARTESIAN_POINT('Ctrl Pts',(-24.7511183249211,-66.44787230635,-55.2525699472664));
#131410=CARTESIAN_POINT('Ctrl Pts',(-24.7341178138436,-66.4548444484004,
-55.2508227166642));
#131411=CARTESIAN_POINT('Ctrl Pts',(-24.7170650830423,-66.4625746537229,
-55.24995));
#131412=CARTESIAN_POINT('Ctrl Pts',(-24.7,-66.4710859610356,-55.24995));
#131413=CARTESIAN_POINT('Origin',(-42.8449509429986,-61.3393238500942,-52.64995));
#131414=CARTESIAN_POINT('',(-43.1064181712415,-64.3279079443695,-59.64995));
#131415=CARTESIAN_POINT('',(-43.1064181712415,-64.3279079443695,-52.64995));
#131416=CARTESIAN_POINT('',(-43.1064181712415,-64.3279079443695,-52.64995));
#131417=CARTESIAN_POINT('',(-44.9662712865582,-63.4606441936539,-52.64995));
#131418=CARTESIAN_POINT('Origin',(-42.8449509429986,-61.3393238500942,-52.64995));
#131419=CARTESIAN_POINT('',(-44.9662712865582,-63.4606441936539,-59.64995));
#131420=CARTESIAN_POINT('',(-44.9662712865582,-63.4606441936539,-52.64995));
#131421=CARTESIAN_POINT('Origin',(-42.8449509429986,-61.3393238500942,-59.64995));
#131422=CARTESIAN_POINT('Origin',(-44.1941738241591,-64.2327416560529,-52.64995));
#131423=CARTESIAN_POINT('',(-33.8064221286261,-65.1415521689341,-59.64995));
#131424=CARTESIAN_POINT('',(-39.4564221286262,-64.6472412200127,-59.64995));
#131425=CARTESIAN_POINT('',(-44.1941738241591,-64.2327416560529,-59.64995));
#131426=CARTESIAN_POINT('',(-33.8064221286261,-65.1415521689341,-55.74995));
#131427=CARTESIAN_POINT('',(-33.8064221286261,-65.1415521689341,-52.64995));
#131428=CARTESIAN_POINT('',(-32.8064221286262,-65.22904083246,-54.74995));
#131429=CARTESIAN_POINT('Ctrl Pts',(-32.8064221286262,-65.22904083246,-54.74995));
#131430=CARTESIAN_POINT('Ctrl Pts',(-33.0689568200132,-65.2060720231813,
-54.7499500000659));
#131431=CARTESIAN_POINT('Ctrl Pts',(-33.3284088181247,-65.1833729146174,
-54.8577231271255));
#131432=CARTESIAN_POINT('Ctrl Pts',(-33.5135289098127,-65.1671770052039,
-55.0428432188135));
#131433=CARTESIAN_POINT('Ctrl Pts',(-33.6986490015007,-65.1509810957903,
-55.2279633105015));
#131434=CARTESIAN_POINT('Ctrl Pts',(-33.8064221285606,-65.1415521689398,
-55.487415308613));
#131435=CARTESIAN_POINT('Ctrl Pts',(-33.8064221286261,-65.1415521689341,
-55.74995));
#131436=CARTESIAN_POINT('',(-32.3064221286262,-65.2727851642229,-54.74995));
#131437=CARTESIAN_POINT('',(-44.1941738241591,-64.2327416560529,-54.74995));
#131438=CARTESIAN_POINT('',(-31.3064221286262,-65.3602738277489,-55.74995));
#131439=CARTESIAN_POINT('Ctrl Pts',(-31.3064221286262,-65.3602738277489,
-55.74995));
#131440=CARTESIAN_POINT('Ctrl Pts',(-31.3064221286917,-65.3602738277431,
-55.4874153086129));
#131441=CARTESIAN_POINT('Ctrl Pts',(-31.4141952557525,-65.3508449008926,
-55.2279633105016));
#131442=CARTESIAN_POINT('Ctrl Pts',(-31.5993153474396,-65.3346489914791,
-55.0428432188135));
#131443=CARTESIAN_POINT('Ctrl Pts',(-31.7844354391267,-65.3184530820656,
-54.8577231271254));
#131444=CARTESIAN_POINT('Ctrl Pts',(-32.0438874372397,-65.2957539735015,
-54.7499500000659));
#131445=CARTESIAN_POINT('Ctrl Pts',(-32.3064221286262,-65.2727851642229,
-54.74995));
#131446=CARTESIAN_POINT('',(-31.3064221286262,-65.3602738277489,-59.64995));
#131447=CARTESIAN_POINT('',(-31.3064221286262,-65.3602738277489,-52.64995));
#131448=CARTESIAN_POINT('',(-28.7021688185769,-65.588116469328,-59.64995));
#131449=CARTESIAN_POINT('',(-44.1941738241591,-64.2327416560529,-59.64995));
#131450=CARTESIAN_POINT('',(-25.6564221281368,-65.8545847710806,-60.0322609860572));
#131451=CARTESIAN_POINT('Ctrl Pts',(-25.6564221266688,-65.8545847543119,
-60.0322609860537));
#131452=CARTESIAN_POINT('Ctrl Pts',(-25.7808509976504,-65.8436986122352,
-59.9993769765733));
#131453=CARTESIAN_POINT('Ctrl Pts',(-25.9056363008897,-65.8327812988126,
-59.9689324054821));
#131454=CARTESIAN_POINT('Ctrl Pts',(-26.0307566852339,-65.8218346938133,
-59.9407811370796));
#131455=CARTESIAN_POINT('Ctrl Pts',(-26.2520372217489,-65.8024751734605,
-59.8909944631628));
#131456=CARTESIAN_POINT('Ctrl Pts',(-26.474388494988,-65.783021979914,-59.8484921029749));
#131457=CARTESIAN_POINT('Ctrl Pts',(-26.6976513564664,-65.763489017205,
-59.812264924349));
#131458=CARTESIAN_POINT('Ctrl Pts',(-26.7996931166554,-65.7545615230246,
-59.7957073784626));
#131459=CARTESIAN_POINT('Ctrl Pts',(-26.9019251840797,-65.7456173770719,
-59.7804614113619));
#131460=CARTESIAN_POINT('Ctrl Pts',(-27.0043315823481,-65.7366579782249,
-59.7664341473284));
#131461=CARTESIAN_POINT('Ctrl Pts',(-27.0579416473936,-65.7319677053213,
-59.7590908313837));
#131462=CARTESIAN_POINT('Ctrl Pts',(-27.1116030957325,-65.7272729367138,
-59.7520917680714));
#131463=CARTESIAN_POINT('Ctrl Pts',(-27.1653166053581,-65.7225736127227,
-59.7454407818488));
#131464=CARTESIAN_POINT('Ctrl Pts',(-27.466811923079,-65.6961961857093,
-59.7081086242913));
#131465=CARTESIAN_POINT('Ctrl Pts',(-27.7698631240412,-65.6696826439603,
-59.681449712741));
#131466=CARTESIAN_POINT('Ctrl Pts',(-28.0745495814084,-65.6430260356544,
-59.6659440379886));
#131467=CARTESIAN_POINT('Ctrl Pts',(-28.2829846777342,-65.6247903294534,
-59.6553366521582));
#131468=CARTESIAN_POINT('Ctrl Pts',(-28.4921848717831,-65.6064876841949,
-59.6499500008557));
#131469=CARTESIAN_POINT('Ctrl Pts',(-28.7021688185769,-65.588116469328,
-59.64995));
#131470=CARTESIAN_POINT('',(-25.6564221286262,-65.8545847766702,-55.74995));
#131471=CARTESIAN_POINT('',(-25.6564221286262,-65.8545847766702,-52.64995));
#131472=CARTESIAN_POINT('Ctrl Pts',(-25.043451507077,-65.9082127571302,
-54.8278826162281));
#131473=CARTESIAN_POINT('Ctrl Pts',(-25.0742713040834,-65.90551637428,-54.8408189450663));
#131474=CARTESIAN_POINT('Ctrl Pts',(-25.104915072702,-65.9028353919181,
-54.8555499531048));
#131475=CARTESIAN_POINT('Ctrl Pts',(-25.1350929986057,-65.9001951655129,
-54.8720618327809));
#131476=CARTESIAN_POINT('Ctrl Pts',(-25.1657431004607,-65.8975136290646,
-54.8888320639594));
#131477=CARTESIAN_POINT('Ctrl Pts',(-25.1959121242359,-65.8948741814946,
-54.9074392518001));
#131478=CARTESIAN_POINT('Ctrl Pts',(-25.2252929736523,-65.892303690246,
-54.9278152010716));
#131479=CARTESIAN_POINT('Ctrl Pts',(-25.2553889373856,-65.8896706346014,
-54.9486870901588));
#131480=CARTESIAN_POINT('Ctrl Pts',(-25.2846571909018,-65.8871099942175,
-54.9714147499623));
#131481=CARTESIAN_POINT('Ctrl Pts',(-25.3127736146752,-65.8846501258785,
-54.9958704922167));
#131482=CARTESIAN_POINT('Ctrl Pts',(-25.3411372062356,-65.88216863316,-55.0205412216878));
#131483=CARTESIAN_POINT('Ctrl Pts',(-25.3683278367126,-65.8797897612392,
-55.0469701419947));
#131484=CARTESIAN_POINT('Ctrl Pts',(-25.3940301284273,-65.8775411020875,
-55.0749758606088));
#131485=CARTESIAN_POINT('Ctrl Pts',(-25.4197097931075,-65.8752944225448,
-55.1029569243646));
#131486=CARTESIAN_POINT('Ctrl Pts',(-25.4439029560561,-65.873177795052,
-55.1325114406684));
#131487=CARTESIAN_POINT('Ctrl Pts',(-25.4663241567112,-65.871216194172,
-55.1634160027496));
#131488=CARTESIAN_POINT('Ctrl Pts',(-25.4741688835925,-65.8705298695015,
-55.1742288870657));
#131489=CARTESIAN_POINT('Ctrl Pts',(-25.4817970097154,-65.8698624949418,
-55.1852066986187));
#131490=CARTESIAN_POINT('Ctrl Pts',(-25.4891974219829,-65.869215042763,
-55.1963388451498));
#131491=CARTESIAN_POINT('Ctrl Pts',(-25.510338242743,-65.8673654606088,
-55.228140142967));
#131492=CARTESIAN_POINT('Ctrl Pts',(-25.5295950731415,-65.8656807062535,
-55.2611692657123));
#131493=CARTESIAN_POINT('Ctrl Pts',(-25.5468557307134,-65.864170594391,
-55.295083999148));
#131494=CARTESIAN_POINT('Ctrl Pts',(-25.5641515040968,-65.862657410293,
-55.3290677301512));
#131495=CARTESIAN_POINT('Ctrl Pts',(-25.5794427196934,-65.8613196022768,
-55.363939731283));
#131496=CARTESIAN_POINT('Ctrl Pts',(-25.5926659905796,-65.8601627159795,
-55.3993402855053));
#131497=CARTESIAN_POINT('Ctrl Pts',(-25.6056853291763,-65.8590236714457,
-55.4341948843334));
#131498=CARTESIAN_POINT('Ctrl Pts',(-25.6166999804352,-65.8580600143278,
-55.4695609780295));
#131499=CARTESIAN_POINT('Ctrl Pts',(-25.6256992872677,-65.8572726770004,
-55.5050939643816));
#131500=CARTESIAN_POINT('Ctrl Pts',(-25.6345695399044,-65.8564966304521,
-55.5401173913793));
#131501=CARTESIAN_POINT('Ctrl Pts',(-25.641481865841,-65.855891880294,-55.5753022272925));
#131502=CARTESIAN_POINT('Ctrl Pts',(-25.6464749038184,-65.8554550460744,
-55.6103291116175));
#131503=CARTESIAN_POINT('Ctrl Pts',(-25.6513699614093,-65.8550267840279,
-55.6446686493459));
#131504=CARTESIAN_POINT('Ctrl Pts',(-25.6544204578572,-65.8547599001706,
-55.6788558270728));
#131505=CARTESIAN_POINT('Ctrl Pts',(-25.6557087574904,-65.8546471885575,
-55.7126093508298));
#131506=CARTESIAN_POINT('Ctrl Pts',(-25.6561862637138,-65.8546054121762,
-55.7251200410772));
#131507=CARTESIAN_POINT('Ctrl Pts',(-25.6564221286231,-65.8545847766705,
-55.7375713926724));
#131508=CARTESIAN_POINT('Ctrl Pts',(-25.6564221286262,-65.8545847766702,
-55.74995));
#131509=CARTESIAN_POINT('',(-44.1941738241591,-64.2327416560529,-52.64995));
#131510=CARTESIAN_POINT('',(-41.9564221286262,-64.428519561198,-59.64995));
#131511=CARTESIAN_POINT('',(-44.1941738241591,-64.2327416560529,-59.64995));
#131512=CARTESIAN_POINT('',(-41.9564221286262,-64.428519561198,-55.74995));
#131513=CARTESIAN_POINT('',(-41.9564221286262,-64.428519561198,-52.64995));
#131514=CARTESIAN_POINT('',(-40.9564221286262,-64.5160082247239,-54.74995));
#131515=CARTESIAN_POINT('Ctrl Pts',(-40.9564221286262,-64.5160082247239,
-54.74995));
#131516=CARTESIAN_POINT('Ctrl Pts',(-41.2189568200132,-64.4930394154452,
-54.7499500000659));
#131517=CARTESIAN_POINT('Ctrl Pts',(-41.4784088181247,-64.4703403068813,
-54.8577231271255));
#131518=CARTESIAN_POINT('Ctrl Pts',(-41.6635289098127,-64.4541443974678,
-55.0428432188135));
#131519=CARTESIAN_POINT('Ctrl Pts',(-41.8486490015007,-64.4379484880542,
-55.2279633105015));
#131520=CARTESIAN_POINT('Ctrl Pts',(-41.9564221285606,-64.4285195612037,
-55.487415308613));
#131521=CARTESIAN_POINT('Ctrl Pts',(-41.9564221286262,-64.428519561198,
-55.74995));
#131522=CARTESIAN_POINT('',(-40.4564221286262,-64.5597525564868,-54.74995));
#131523=CARTESIAN_POINT('',(-44.1941738241591,-64.2327416560529,-54.74995));
#131524=CARTESIAN_POINT('',(-39.4564221286262,-64.6472412200127,-55.74995));
#131525=CARTESIAN_POINT('Ctrl Pts',(-39.4564221286262,-64.6472412200127,
-55.74995));
#131526=CARTESIAN_POINT('Ctrl Pts',(-39.4564221286917,-64.647241220007,
-55.4874153086129));
#131527=CARTESIAN_POINT('Ctrl Pts',(-39.5641952557525,-64.6378122931564,
-55.2279633105016));
#131528=CARTESIAN_POINT('Ctrl Pts',(-39.7493153474396,-64.6216163837429,
-55.0428432188135));
#131529=CARTESIAN_POINT('Ctrl Pts',(-39.9344354391268,-64.6054204743294,
-54.8577231271254));
#131530=CARTESIAN_POINT('Ctrl Pts',(-40.1938874372398,-64.5827213657654,
-54.7499500000659));
#131531=CARTESIAN_POINT('Ctrl Pts',(-40.4564221286262,-64.5597525564868,
-54.74995));
#131532=CARTESIAN_POINT('',(-39.4564221286262,-64.6472412200127,-52.64995));
#131533=CARTESIAN_POINT('Origin',(-42.8449509429986,-61.3393238500942,-59.64995));
#131534=CARTESIAN_POINT('',(-43.0192624284939,-63.3317132462777,-60.64995));
#131535=CARTESIAN_POINT('Origin',(-43.0192624284939,-63.3317132462777,-59.64995));
#131536=CARTESIAN_POINT('',(-44.2591645053717,-62.7535374124673,-60.64995));
#131537=CARTESIAN_POINT('Origin',(-44.2591645053717,-62.7535374124673,-59.64995));
#131538=CARTESIAN_POINT('Origin',(-42.8449509429986,-61.3393238500942,-60.64995));
#131539=CARTESIAN_POINT('Origin',(-48.3718238300662,-55.8124509630266,-52.64995));
#131540=CARTESIAN_POINT('',(-50.4931441736259,-57.9337713065862,-59.64995));
#131541=CARTESIAN_POINT('',(-50.4931441736259,-57.9337713065862,-52.64995));
#131542=CARTESIAN_POINT('',(-50.4931441736259,-57.9337713065862,-52.64995));
#131543=CARTESIAN_POINT('',(-51.3604079243415,-56.0739181912695,-52.64995));
#131544=CARTESIAN_POINT('Origin',(-48.3718238300662,-55.8124509630266,-52.64995));
#131545=CARTESIAN_POINT('',(-51.3604079243415,-56.0739181912695,-59.64995));
#131546=CARTESIAN_POINT('',(-51.3604079243415,-56.0739181912695,-52.64995));
#131547=CARTESIAN_POINT('Origin',(-48.3718238300662,-55.8124509630266,-59.64995));
#131548=CARTESIAN_POINT('Origin',(-51.265241636025,-57.1616738441871,-52.64995));
#131549=CARTESIAN_POINT('',(-51.265241636025,-57.1616738441871,-52.64995));
#131550=CARTESIAN_POINT('',(-51.265241636025,-57.1616738441871,-59.64995));
#131551=CARTESIAN_POINT('Origin',(-48.3718238300662,-55.8124509630266,-59.64995));
#131552=CARTESIAN_POINT('',(-49.7860373924393,-57.2266645253997,-60.64995));
#131553=CARTESIAN_POINT('Origin',(-49.7860373924393,-57.2266645253997,-59.64995));
#131554=CARTESIAN_POINT('',(-50.3642132262497,-55.9867624485218,-60.64995));
#131555=CARTESIAN_POINT('Origin',(-50.3642132262497,-55.9867624485218,-59.64995));
#131556=CARTESIAN_POINT('Origin',(-48.3718238300662,-55.8124509630266,-60.64995));
#131557=CARTESIAN_POINT('Origin',(-52.9858497431864,-37.4950331867729,-52.64995));
#131558=CARTESIAN_POINT('',(-52.6206164493,-41.6696688386047,-59.64995));
#131559=CARTESIAN_POINT('',(-52.8772422786263,-38.736422148331,-60.0032396521556));
#131560=CARTESIAN_POINT('Ctrl Pts',(-52.6206164493,-41.6696688386047,-59.64995));
#131561=CARTESIAN_POINT('Ctrl Pts',(-52.6471771938443,-41.3660781392638,
-59.649950001162));
#131562=CARTESIAN_POINT('Ctrl Pts',(-52.6736027803766,-41.0640322847433,
-59.6612277190036));
#131563=CARTESIAN_POINT('Ctrl Pts',(-52.6998985433591,-40.7634703219199,
-59.6832689389194));
#131564=CARTESIAN_POINT('Ctrl Pts',(-52.7166476389898,-40.5720272722695,
-59.6973081018229));
#131565=CARTESIAN_POINT('Ctrl Pts',(-52.7333441220444,-40.3811856093979,
-59.715714898338));
#131566=CARTESIAN_POINT('Ctrl Pts',(-52.7499897489645,-40.1909252438875,
-59.7383666003326));
#131567=CARTESIAN_POINT('Ctrl Pts',(-52.7543856861046,-40.1406794579502,
-59.7443486795034));
#131568=CARTESIAN_POINT('Ctrl Pts',(-52.7587779570344,-40.0904755740926,
-59.7506312543479));
#131569=CARTESIAN_POINT('Ctrl Pts',(-52.7631665715902,-40.0403134816151,
-59.7572129455377));
#131570=CARTESIAN_POINT('Ctrl Pts',(-52.7801318002605,-39.8464000361234,
-59.7826560311971));
#131571=CARTESIAN_POINT('Ctrl Pts',(-52.7970456659898,-39.6530737072156,
-59.8124579292866));
#131572=CARTESIAN_POINT('Ctrl Pts',(-52.813898709432,-39.4604424150672,
-59.8472750881764));
#131573=CARTESIAN_POINT('Ctrl Pts',(-52.8286848633261,-39.2914357937844,
-59.8778222039694));
#131574=CARTESIAN_POINT('Ctrl Pts',(-52.8434252414647,-39.1229522134554,
-59.9121898106588));
#131575=CARTESIAN_POINT('Ctrl Pts',(-52.8581158408284,-38.9550379662894,
-59.9506823384324));
#131576=CARTESIAN_POINT('Ctrl Pts',(-52.8645007938114,-38.882057651002,
-59.9674122875614));
#131577=CARTESIAN_POINT('Ctrl Pts',(-52.870876360439,-38.8091846968969,
-59.9849220508822));
#131578=CARTESIAN_POINT('Ctrl Pts',(-52.8772422685109,-38.7364221474456,
-60.003239652154));
#131579=CARTESIAN_POINT('',(-52.3829313330767,-44.3864221486262,-59.64995));
#131580=CARTESIAN_POINT('',(-52.9858497431864,-37.4950331867729,-59.64995));
#131581=CARTESIAN_POINT('',(-52.3829313330767,-44.3864221486262,-55.74995));
#131582=CARTESIAN_POINT('',(-52.3829313330767,-44.3864221486262,-52.64995));
#131583=CARTESIAN_POINT('',(-52.2954426695508,-45.3864221486261,-54.74995));
#131584=CARTESIAN_POINT('Ctrl Pts',(-52.2954426695508,-45.3864221486261,
-54.74995));
#131585=CARTESIAN_POINT('Ctrl Pts',(-52.3184114788294,-45.123887457239,
-54.7499500000658));
#131586=CARTESIAN_POINT('Ctrl Pts',(-52.3411105873933,-44.8644354591276,
-54.8577231271254));
#131587=CARTESIAN_POINT('Ctrl Pts',(-52.3573064968069,-44.6793153674396,
-55.0428432188135));
#131588=CARTESIAN_POINT('Ctrl Pts',(-52.3735024062205,-44.4941952757516,
-55.2279633105015));
#131589=CARTESIAN_POINT('Ctrl Pts',(-52.3829313330709,-44.3864221486917,
-55.4874153086129));
#131590=CARTESIAN_POINT('Ctrl Pts',(-52.3829313330767,-44.3864221486262,
-55.74995));
#131591=CARTESIAN_POINT('',(-52.2516983377878,-45.8864221486262,-54.74995));
#131592=CARTESIAN_POINT('',(-52.9858497431864,-37.4950331867729,-54.74995));
#131593=CARTESIAN_POINT('',(-52.1642096742619,-46.8864221486262,-55.74995));
#131594=CARTESIAN_POINT('Ctrl Pts',(-52.1642096742619,-46.8864221486262,
-55.74995));
#131595=CARTESIAN_POINT('Ctrl Pts',(-52.1642096742676,-46.8864221485606,
-55.487415308613));
#131596=CARTESIAN_POINT('Ctrl Pts',(-52.1736386011181,-46.7786490215007,
-55.2279633105015));
#131597=CARTESIAN_POINT('Ctrl Pts',(-52.1898345105317,-46.5935289298127,
-55.0428432188135));
#131598=CARTESIAN_POINT('Ctrl Pts',(-52.2060304199453,-46.4084088381247,
-54.8577231271255));
#131599=CARTESIAN_POINT('Ctrl Pts',(-52.2287295285091,-46.1489568400132,
-54.7499500000658));
#131600=CARTESIAN_POINT('Ctrl Pts',(-52.2516983377878,-45.8864221486262,
-54.74995));
#131601=CARTESIAN_POINT('',(-52.1642096742619,-46.8864221486262,-59.64995));
#131602=CARTESIAN_POINT('',(-52.1642096742619,-46.8864221486262,-52.64995));
#131603=CARTESIAN_POINT('',(-51.6698987253405,-52.5364221486262,-59.64995));
#131604=CARTESIAN_POINT('',(-52.9858497431864,-37.4950331867729,-59.64995));
#131605=CARTESIAN_POINT('',(-51.6698987253405,-52.5364221486262,-55.74995));
#131606=CARTESIAN_POINT('',(-51.6698987253405,-52.5364221486262,-52.64995));
#131607=CARTESIAN_POINT('',(-51.5824100618146,-53.5364221486262,-54.74995));
#131608=CARTESIAN_POINT('Ctrl Pts',(-51.5824100618146,-53.5364221486262,
-54.74995));
#131609=CARTESIAN_POINT('Ctrl Pts',(-51.6053788710933,-53.2738874572391,
-54.7499500000658));
#131610=CARTESIAN_POINT('Ctrl Pts',(-51.6280779796571,-53.0144354591276,
-54.8577231271254));
#131611=CARTESIAN_POINT('Ctrl Pts',(-51.6442738890707,-52.8293153674396,
-55.0428432188135));
#131612=CARTESIAN_POINT('Ctrl Pts',(-51.6604697984843,-52.6441952757516,
-55.2279633105015));
#131613=CARTESIAN_POINT('Ctrl Pts',(-51.6698987253348,-52.5364221486917,
-55.4874153086129));
#131614=CARTESIAN_POINT('Ctrl Pts',(-51.6698987253405,-52.5364221486262,
-55.74995));
#131615=CARTESIAN_POINT('',(-51.5386657300517,-54.0364221486261,-54.74995));
#131616=CARTESIAN_POINT('',(-52.9858497431864,-37.4950331867729,-54.74995));
#131617=CARTESIAN_POINT('',(-51.4511770665258,-55.0364221486262,-55.74995));
#131618=CARTESIAN_POINT('Ctrl Pts',(-51.4511770665258,-55.0364221486262,
-55.74995));
#131619=CARTESIAN_POINT('Ctrl Pts',(-51.4511770665315,-55.0364221485606,
-55.4874153086129));
#131620=CARTESIAN_POINT('Ctrl Pts',(-51.460605993382,-54.9286490214999,
-55.2279633105015));
#131621=CARTESIAN_POINT('Ctrl Pts',(-51.4768019027956,-54.7435289298127,
-55.0428432188135));
#131622=CARTESIAN_POINT('Ctrl Pts',(-51.4929978122091,-54.5584088381255,
-54.8577231271254));
#131623=CARTESIAN_POINT('Ctrl Pts',(-51.5156969207731,-54.2989568400126,
-54.7499500000658));
#131624=CARTESIAN_POINT('Ctrl Pts',(-51.5386657300517,-54.0364221486262,
-54.74995));
#131625=CARTESIAN_POINT('',(-51.4511770665258,-55.0364221486262,-59.64995));
#131626=CARTESIAN_POINT('',(-51.4511770665258,-55.0364221486262,-52.64995));
#131627=CARTESIAN_POINT('',(-52.9858497431864,-37.4950331867729,-59.64995));
#131628=CARTESIAN_POINT('',(-52.9858497431864,-37.4950331867729,-52.64995));
#131629=CARTESIAN_POINT('',(-52.877242281998,-38.7364221486262,-55.74995));
#131630=CARTESIAN_POINT('Origin',(-52.9541266237314,-37.8576301013502,-55.6904184160493));
#131631=CARTESIAN_POINT('',(-52.877242281998,-38.7364221486262,-52.64995));
#131632=CARTESIAN_POINT('Ctrl Pts',(-1.2393865421354,-71.3418443611208,
-56.1920015047684));
#131633=CARTESIAN_POINT('Ctrl Pts',(-0.749999999999951,-71.3522348691612,
-56.1920015047684));
#131634=CARTESIAN_POINT('Ctrl Pts',(-0.749999999999965,-71.8417317029411,
-56.1920015047684));
#131635=CARTESIAN_POINT('Ctrl Pts',(-1.23938657388158,-71.3418443604468,
-55.8977818815622));
#131636=CARTESIAN_POINT('Ctrl Pts',(-0.817143227758975,-71.350809303989,
-55.9852769982734));
#131637=CARTESIAN_POINT('Ctrl Pts',(-0.749999999999968,-71.7679993860759,
-55.9713019100196));
#131638=CARTESIAN_POINT('Ctrl Pts',(-1.17148444765176,-71.3435038399877,
-55.5953607449048));
#131639=CARTESIAN_POINT('Ctrl Pts',(-0.822125649397247,-71.3503107976076,
-55.7434666115786));
#131640=CARTESIAN_POINT('Ctrl Pts',(-0.715758200751532,-71.705555960146,
-55.7746050694403));
#131641=CARTESIAN_POINT('Ctrl Pts',(-0.911534986295056,-71.3479485504093,
-55.2320500655911));
#131642=CARTESIAN_POINT('Ctrl Pts',(-0.680372527884655,-71.3515033251648,
-55.4569572564689));
#131643=CARTESIAN_POINT('Ctrl Pts',(-0.584670453989408,-71.6422004184537,
-55.5485996630821));
#131644=CARTESIAN_POINT('Ctrl Pts',(-0.802354774810878,-71.3496303532999,
-55.1310699758717));
#131645=CARTESIAN_POINT('Ctrl Pts',(-0.61343369370942,-71.3521282334297,
-55.3772175182816));
#131646=CARTESIAN_POINT('Ctrl Pts',(-0.529612862082923,-71.6265518657637,
-55.4878844649265));
#131647=CARTESIAN_POINT('Ctrl Pts',(-0.543457447472851,-71.3526142995993,
-54.9878205454944));
#131648=CARTESIAN_POINT('Ctrl Pts',(-0.446700352388622,-71.3534136965962,
-55.2655230738672));
#131649=CARTESIAN_POINT('Ctrl Pts',(-0.399055664911118,-71.6054835497946,
-55.4025039623078));
#131650=CARTESIAN_POINT('Ctrl Pts',(-0.399927732415193,-71.3538238656642,
-54.9488753843798));
#131651=CARTESIAN_POINT('Ctrl Pts',(-0.350200382979481,-71.3540360830669,
-55.2347429562386));
#131652=CARTESIAN_POINT('Ctrl Pts',(-0.326675282358978,-71.6004595978917,
-55.3797802668488));
#131653=CARTESIAN_POINT('Ctrl Pts',(-0.24960231081565,-71.3544665017672,
-54.948950578459));
#131654=CARTESIAN_POINT('Ctrl Pts',(-0.249744175924072,-71.3544658952987,
-55.234934426787));
#131655=CARTESIAN_POINT('Ctrl Pts',(-0.250869887203208,-71.6009673739965,
-55.3799259279328));
#131656=CARTESIAN_POINT('',(-0.749999999999963,-71.8417317505524,-56.1920013490171));
#131657=CARTESIAN_POINT('',(-1.2393865421354,-71.3418443611208,-56.1920015047684));
#131658=CARTESIAN_POINT('Origin',(-1.24999999999996,-71.8417317029411,-56.1920015047684));
#131659=CARTESIAN_POINT('',(-0.250869887203081,-71.6009673739936,-55.3799259279326));
#131660=CARTESIAN_POINT('Ctrl Pts',(-0.749999999999961,-71.8417316609121,
-56.1920013789646));
#131661=CARTESIAN_POINT('Ctrl Pts',(-0.749999986987558,-71.7679993623464,
-55.9713018352718));
#131662=CARTESIAN_POINT('Ctrl Pts',(-0.715758184146415,-71.7055559521206,
-55.7746050408118));
#131663=CARTESIAN_POINT('Ctrl Pts',(-0.584670453989408,-71.6422004184537,
-55.5485996630821));
#131664=CARTESIAN_POINT('Ctrl Pts',(-0.529612862082923,-71.6265518657637,
-55.4878844649265));
#131665=CARTESIAN_POINT('Ctrl Pts',(-0.399055664911118,-71.6054835497946,
-55.4025039623078));
#131666=CARTESIAN_POINT('Ctrl Pts',(-0.326675282358978,-71.6004595978917,
-55.3797802668488));
#131667=CARTESIAN_POINT('Ctrl Pts',(-0.250869887203096,-71.6009673739964,
-55.3799259279342));
#131668=CARTESIAN_POINT('',(-0.249602310815417,-71.3544665017672,-54.9489505784606));
#131669=CARTESIAN_POINT('Origin',(-0.251739774406202,-71.8544619329957,
-54.9489505784606));
#131670=CARTESIAN_POINT('Ctrl Pts',(-0.249602310815417,-71.3544665017672,
-54.9489505784606));
#131671=CARTESIAN_POINT('Ctrl Pts',(-0.399927732415193,-71.3538238656642,
-54.9488753843798));
#131672=CARTESIAN_POINT('Ctrl Pts',(-0.543457447472851,-71.3526142995993,
-54.9878205454944));
#131673=CARTESIAN_POINT('Ctrl Pts',(-0.802354774810878,-71.3496303532999,
-55.1310699758717));
#131674=CARTESIAN_POINT('Ctrl Pts',(-0.911534986295056,-71.3479485504093,
-55.2320500655911));
#131675=CARTESIAN_POINT('Ctrl Pts',(-1.17148444765176,-71.3435038399877,
-55.5953607449048));
#131676=CARTESIAN_POINT('Ctrl Pts',(-1.23938657388158,-71.3418443604468,
-55.8977818815622));
#131677=CARTESIAN_POINT('Ctrl Pts',(-1.2393865421354,-71.3418443611208,
-56.1920015047684));
#131678=CARTESIAN_POINT('Origin',(-1.24999999999996,-71.8417317029411,-55.24995));
#131679=CARTESIAN_POINT('',(-0.749999999999965,-71.8417317029411,-60.42825533736));
#131680=CARTESIAN_POINT('',(-1.2393865421354,-71.3418443611208,-60.42825533736));
#131681=CARTESIAN_POINT('Origin',(-1.24999999999996,-71.8417317029411,-60.42825533736));
#131682=CARTESIAN_POINT('',(-0.749999999999965,-71.8417317029411,-55.24995));
#131683=CARTESIAN_POINT('',(-1.2393865421354,-71.3418443611208,-55.24995));
#131684=CARTESIAN_POINT('Origin',(0.,-12.9675000200281,-60.42825533736));
#131685=CARTESIAN_POINT('',(-6.84677576889373,-70.8578246683297,-60.8508735991007));
#131686=CARTESIAN_POINT('',(-1.24035792914739,-71.2481103336038,-60.8508735991007));
#131687=CARTESIAN_POINT('Origin',(0.,-12.9675000200281,-60.8508735991007));
#131688=CARTESIAN_POINT('Origin',(-1.24990493606806,-70.3423238919629,-60.4282489645659));
#131689=CARTESIAN_POINT('',(-6.84141371258755,-70.9528017323285,-60.42825533736));
#131690=CARTESIAN_POINT('Origin',(0.,-12.9675000200281,-60.42825533736));
#131691=CARTESIAN_POINT('Origin',(-6.92387950998942,-69.4954305645409,-60.33066203808));
#131692=CARTESIAN_POINT('Origin',(-6.9,-71.449357516634,-55.24995));
#131693=CARTESIAN_POINT('',(-6.9,-70.949357516634,-56.0666111687498));
#131694=CARTESIAN_POINT('',(-7.40000000638209,-71.4493575166325,-56.0666111687523));
#131695=CARTESIAN_POINT('Origin',(-6.9,-71.449357516634,-56.0666111687498));
#131696=CARTESIAN_POINT('',(-7.4,-71.449357516634,-60.42825533736));
#131697=CARTESIAN_POINT('',(-7.4,-71.449357516634,-55.24995));
#131698=CARTESIAN_POINT('',(-6.9,-70.949357516634,-60.42825533736));
#131699=CARTESIAN_POINT('Origin',(-6.9,-71.449357516634,-60.42825533736));
#131700=CARTESIAN_POINT('Origin',(-6.9,-71.449357516634,-60.42825533736));
#131701=CARTESIAN_POINT('',(-6.84141371258755,-70.9528017323285,-56.0666111687498));
#131702=CARTESIAN_POINT('',(-6.84141371258755,-70.9528017323285,-55.24995));
#131703=CARTESIAN_POINT('Origin',(-6.9,-71.449357516634,-56.0666111687498));
#131704=CARTESIAN_POINT('Ctrl Pts',(-7.86502491569091,-70.8228501557662,
-54.8850140141151));
#131705=CARTESIAN_POINT('Ctrl Pts',(-7.87072047725574,-70.8220758845275,
-55.2299609924928));
#131706=CARTESIAN_POINT('Ctrl Pts',(-7.91618843693208,-71.1413940909409,
-55.352394666395));
#131707=CARTESIAN_POINT('Ctrl Pts',(-7.72241706825884,-70.8422366821738,
-54.8874327557878));
#131708=CARTESIAN_POINT('Ctrl Pts',(-7.77985413280654,-70.8344428879727,
-55.236521459352));
#131709=CARTESIAN_POINT('Ctrl Pts',(-7.844285602846,-71.157562039706,-55.3560236134997));
#131710=CARTESIAN_POINT('Ctrl Pts',(-7.5794821547774,-70.8610938450093,
-54.9239881329105));
#131711=CARTESIAN_POINT('Ctrl Pts',(-7.69016530757976,-70.8464897855799,
-55.2681271844367));
#131712=CARTESIAN_POINT('Ctrl Pts',(-7.77219443565847,-71.177222127411,
-55.3781864762555));
#131713=CARTESIAN_POINT('Ctrl Pts',(-7.32391158111293,-70.8939799308472,
-55.0534925677837));
#131714=CARTESIAN_POINT('Ctrl Pts',(-7.53737924067218,-70.8668804541439,
-55.3692852810369));
#131715=CARTESIAN_POINT('Ctrl Pts',(-7.64331486532417,-71.2207339188645,
-55.4539331018544));
#131716=CARTESIAN_POINT('Ctrl Pts',(-7.20960774580809,-70.9082476913312,
-55.1469663768362));
#131717=CARTESIAN_POINT('Ctrl Pts',(-7.47303212720142,-70.8754018535837,
-55.4405214339084));
#131718=CARTESIAN_POINT('Ctrl Pts',(-7.58567352642291,-71.2449041853563,
-55.5078568245776));
#131719=CARTESIAN_POINT('Ctrl Pts',(-7.02628770602923,-70.9307639518508,
-55.3693141862512));
#131720=CARTESIAN_POINT('Ctrl Pts',(-7.38267219174721,-70.8874980297502,
-55.6027965247728));
#131721=CARTESIAN_POINT('Ctrl Pts',(-7.49322857950783,-71.2966779191941,
-55.6376571876191));
#131722=CARTESIAN_POINT('Ctrl Pts',(-6.95597670016225,-70.9391888126349,
-55.4992549495758));
#131723=CARTESIAN_POINT('Ctrl Pts',(-7.35664509914443,-70.8910885028411,
-55.6963616877968));
#131724=CARTESIAN_POINT('Ctrl Pts',(-7.45777202258463,-71.3246266217341,
-55.7141753031788));
#131725=CARTESIAN_POINT('Ctrl Pts',(-6.86374100295758,-70.950181682438,
-55.7748476118441));
#131726=CARTESIAN_POINT('Ctrl Pts',(-7.34624804767826,-70.8930407983775,
-55.8848711139694));
#131727=CARTESIAN_POINT('Ctrl Pts',(-7.41125924474539,-71.38419243799,-55.8811540356734));
#131728=CARTESIAN_POINT('Ctrl Pts',(-6.84141371299613,-70.9528017322803,
-55.9212771125469));
#131729=CARTESIAN_POINT('Ctrl Pts',(-7.36384050363832,-70.8911630457611,
-55.9819410866112));
#131730=CARTESIAN_POINT('Ctrl Pts',(-7.4,-71.4160375965177,-55.9720928529598));
#131731=CARTESIAN_POINT('Ctrl Pts',(-6.84141371258755,-70.9528017323285,
-56.0666111687498));
#131732=CARTESIAN_POINT('Ctrl Pts',(-7.3999999999998,-70.8868967568689,
-56.06661116875));
#131733=CARTESIAN_POINT('Ctrl Pts',(-7.4,-71.4493575166339,-56.06661116875));
#131734=CARTESIAN_POINT('',(-7.86502491569136,-70.8228501557662,-54.8850140141151));
#131735=CARTESIAN_POINT('Ctrl Pts',(-6.84141371258755,-70.9528017323285,
-56.0666111687498));
#131736=CARTESIAN_POINT('Ctrl Pts',(-6.84141371272281,-70.9528017323125,
-56.0185004951022));
#131737=CARTESIAN_POINT('Ctrl Pts',(-6.84385625486988,-70.9525150960356,
-55.9705185340178));
#131738=CARTESIAN_POINT('Ctrl Pts',(-6.84874395952159,-70.951938515923,
-55.922884915407));
#131739=CARTESIAN_POINT('Ctrl Pts',(-6.85371160739848,-70.9513525052747,
-55.8744722020329));
#131740=CARTESIAN_POINT('Ctrl Pts',(-6.86120476133718,-70.9504670347036,
-55.8264180258316));
#131741=CARTESIAN_POINT('Ctrl Pts',(-6.87128050874744,-70.9492722819139,
-55.7789472465282));
#131742=CARTESIAN_POINT('Ctrl Pts',(-6.88084558986922,-70.9481380824458,
-55.7338824154579));
#131743=CARTESIAN_POINT('Ctrl Pts',(-6.89273836925603,-70.9467251353176,
-55.6893423359324));
#131744=CARTESIAN_POINT('Ctrl Pts',(-6.90705554696955,-70.9450193012212,
-55.645530903299));
#131745=CARTESIAN_POINT('Ctrl Pts',(-6.90781992104138,-70.9449282291272,
-55.6431918722535));
#131746=CARTESIAN_POINT('Ctrl Pts',(-6.90859121688158,-70.9448363208197,
-55.6408549230079));
#131747=CARTESIAN_POINT('Ctrl Pts',(-6.90936945309023,-70.944743573674,
-55.638520088397));
#131748=CARTESIAN_POINT('Ctrl Pts',(-6.90953264041296,-70.9447241256476,
-55.6380305000112));
#131749=CARTESIAN_POINT('Ctrl Pts',(-6.90969612810931,-70.9447046413087,
-55.6375410188016));
#131750=CARTESIAN_POINT('Ctrl Pts',(-6.90985991625218,-70.9446851206452,
-55.6370516451987));
#131751=CARTESIAN_POINT('Ctrl Pts',(-6.93890470840657,-70.9412234926851,
-55.5502703047941));
#131752=CARTESIAN_POINT('Ctrl Pts',(-6.97755496303225,-70.9365992546703,
-55.4665613054832));
#131753=CARTESIAN_POINT('Ctrl Pts',(-7.02515534568038,-70.9308292795787,
-55.3886379526022));
#131754=CARTESIAN_POINT('Ctrl Pts',(-7.05265246384246,-70.9274961616906,
-55.3436242883719));
#131755=CARTESIAN_POINT('Ctrl Pts',(-7.08313672341662,-70.92378064339,-55.3005419198596));
#131756=CARTESIAN_POINT('Ctrl Pts',(-7.11648530834341,-70.9196854249332,
-55.2599212236758));
#131757=CARTESIAN_POINT('Ctrl Pts',(-7.11697272521332,-70.9196255699628,
-55.2593275189465));
#131758=CARTESIAN_POINT('Ctrl Pts',(-7.11746075366589,-70.9195656339149,
-55.2587343401393));
#131759=CARTESIAN_POINT('Ctrl Pts',(-7.11794939330103,-70.9195056167998,
-55.2581416889457));
#131760=CARTESIAN_POINT('Ctrl Pts',(-7.1776695866293,-70.912170489928,-55.1857094887856));
#131761=CARTESIAN_POINT('Ctrl Pts',(-7.24707274855763,-70.9035491680656,
-55.1207030262982));
#131762=CARTESIAN_POINT('Ctrl Pts',(-7.32365993963484,-70.8938669826859,
-55.0662525944787));
#131763=CARTESIAN_POINT('Ctrl Pts',(-7.36395975880774,-70.8887722623481,
-55.0376010337496));
#131764=CARTESIAN_POINT('Ctrl Pts',(-7.406247882039,-70.8833838941671,-55.0118727368965));
#131765=CARTESIAN_POINT('Ctrl Pts',(-7.450155212976,-70.8777352422905,-54.9895263260323));
#131766=CARTESIAN_POINT('Ctrl Pts',(-7.45066930715087,-70.8776691043822,
-54.989264680439));
#131767=CARTESIAN_POINT('Ctrl Pts',(-7.45118359869241,-70.877602933957,
-54.9890035107279));
#131768=CARTESIAN_POINT('Ctrl Pts',(-7.45169808724107,-70.8775367310404,
-54.9887428173532));
#131769=CARTESIAN_POINT('Ctrl Pts',(-7.48702485166255,-70.8729909839197,
-54.9708426066328));
#131770=CARTESIAN_POINT('Ctrl Pts',(-7.52340553096599,-70.8682741670682,
-54.9551443604244));
#131771=CARTESIAN_POINT('Ctrl Pts',(-7.56060369340833,-70.8634146986663,
-54.9417107539087));
#131772=CARTESIAN_POINT('Ctrl Pts',(-7.59755058615547,-70.8585880554651,
-54.9283678899994));
#131773=CARTESIAN_POINT('Ctrl Pts',(-7.63530511490777,-70.8536205390166,
-54.9172587967144));
#131774=CARTESIAN_POINT('Ctrl Pts',(-7.67365359691511,-70.8485368945066,
-54.9084923483496));
#131775=CARTESIAN_POINT('Ctrl Pts',(-7.71043547056378,-70.8436609265346,
-54.9000840260582));
#131776=CARTESIAN_POINT('Ctrl Pts',(-7.74776474509219,-70.8386779998652,
-54.8938307755624));
#131777=CARTESIAN_POINT('Ctrl Pts',(-7.78545391476949,-70.8336090347271,
-54.8898753244176));
#131778=CARTESIAN_POINT('Ctrl Pts',(-7.81182391853939,-70.8300624288733,
-54.887107811562));
#131779=CARTESIAN_POINT('Ctrl Pts',(-7.83837014274923,-70.8264736832847,
-54.8854661001065));
#131780=CARTESIAN_POINT('Ctrl Pts',(-7.86502491569091,-70.8228501557662,
-54.8850140141151));
#131781=CARTESIAN_POINT('',(-7.91618843693321,-71.1413940908982,-55.3523946663788));
#131782=CARTESIAN_POINT('Origin',(-7.93237687386467,-71.3182931027643,-54.8850140141151));
#131783=CARTESIAN_POINT('Ctrl Pts',(-7.91618843693208,-71.1413940909408,
-55.3523946663949));
#131784=CARTESIAN_POINT('Ctrl Pts',(-7.844285602846,-71.157562039706,-55.3560236134997));
#131785=CARTESIAN_POINT('Ctrl Pts',(-7.77219443565847,-71.177222127411,
-55.3781864762555));
#131786=CARTESIAN_POINT('Ctrl Pts',(-7.64331486532417,-71.2207339188645,
-55.4539331018544));
#131787=CARTESIAN_POINT('Ctrl Pts',(-7.58567352642291,-71.2449041853563,
-55.5078568245776));
#131788=CARTESIAN_POINT('Ctrl Pts',(-7.49322857950783,-71.2966779191941,
-55.6376571876191));
#131789=CARTESIAN_POINT('Ctrl Pts',(-7.45777202258463,-71.3246266217341,
-55.7141753031788));
#131790=CARTESIAN_POINT('Ctrl Pts',(-7.41125924474539,-71.38419243799,-55.8811540356734));
#131791=CARTESIAN_POINT('Ctrl Pts',(-7.4,-71.4160375965177,-55.9720928529598));
#131792=CARTESIAN_POINT('Ctrl Pts',(-7.4,-71.449357516634,-56.06661116875));
#131793=CARTESIAN_POINT('Ctrl Pts',(-8.35962920986988,-70.7534564084689,
-54.8763024037297));
#131794=CARTESIAN_POINT('Ctrl Pts',(-8.36589323739404,-70.752550220344,
-55.2292031667489));
#131795=CARTESIAN_POINT('Ctrl Pts',(-8.41560835021369,-71.0814043774777,
-55.3473655916165));
#131796=CARTESIAN_POINT('Ctrl Pts',(-8.19486187074245,-70.7772925435282,
-54.8793138184774));
#131797=CARTESIAN_POINT('Ctrl Pts',(-8.2013544983267,-70.7763714724242,
-55.2294679275358));
#131798=CARTESIAN_POINT('Ctrl Pts',(-8.24918690883785,-71.102010310254,
-55.3491521481271));
#131799=CARTESIAN_POINT('Ctrl Pts',(-8.02999374674379,-70.8004238120746,
-54.8822160506073));
#131800=CARTESIAN_POINT('Ctrl Pts',(-8.03626733023182,-70.7995543826982,
-55.2297202388378));
#131801=CARTESIAN_POINT('Ctrl Pts',(-8.08271475024063,-71.1220068981801,
-55.3508246944299));
#131802=CARTESIAN_POINT('Ctrl Pts',(-7.86502491569137,-70.8228501557662,
-54.8850140141151));
#131803=CARTESIAN_POINT('Ctrl Pts',(-7.87072047725699,-70.8220758845274,
-55.2299609924931));
#131804=CARTESIAN_POINT('Ctrl Pts',(-7.91618843693366,-71.141394090941,
-55.3523946663951));
#131805=CARTESIAN_POINT('',(-8.35962920986979,-70.7534564084689,-54.8763024037297));
#131806=CARTESIAN_POINT('Origin',(-0.0280298706588222,-14.2420762575821,
-46.319218516546));
#131807=CARTESIAN_POINT('',(-8.41560835064733,-71.0814043774055,-55.3473655916053));
#131808=CARTESIAN_POINT('Origin',(-8.4312167004274,-71.248305103724,-54.8763024037297));
#131809=CARTESIAN_POINT('Origin',(-0.0696643368815508,-4.70111132130388,
-43.5213887605807));
#131810=CARTESIAN_POINT('Ctrl Pts',(-9.32018679685842,-70.6063261212332,
-55.8925850873));
#131811=CARTESIAN_POINT('Ctrl Pts',(-8.89999999999995,-70.674270243298,
-55.8925850872999));
#131812=CARTESIAN_POINT('Ctrl Pts',(-8.9,-71.0999148696911,-55.8925850873));
#131813=CARTESIAN_POINT('Ctrl Pts',(-9.32018679646957,-70.606326121296,
-55.7609765242912));
#131814=CARTESIAN_POINT('Ctrl Pts',(-8.92045674363165,-70.670962391591,
-55.8099505084873));
#131815=CARTESIAN_POINT('Ctrl Pts',(-8.9,-71.0753963340341,-55.8158206410579));
#131816=CARTESIAN_POINT('Ctrl Pts',(-9.29866745626329,-70.6098198655576,
-55.6301334688925));
#131817=CARTESIAN_POINT('Ctrl Pts',(-8.92288173642606,-70.6704214883702,
-55.7222104842267));
#131818=CARTESIAN_POINT('Ctrl Pts',(-8.88914819160783,-71.0574685211989,
-55.7424878932553));
#131819=CARTESIAN_POINT('Ctrl Pts',(-9.20823066610786,-70.6243360556297,
-55.3829240249879));
#131820=CARTESIAN_POINT('Ctrl Pts',(-8.88787909971282,-70.6754793338957,
-55.5563944136962));
#131821=CARTESIAN_POINT('Ctrl Pts',(-8.84354256567003,-71.0340357122248,
-55.606998619986));
#131822=CARTESIAN_POINT('Ctrl Pts',(-9.14039822217997,-70.6351795268323,
-55.2697323706429));
#131823=CARTESIAN_POINT('Ctrl Pts',(-8.8515542998134,-70.6809070626089,
-55.4791108159719));
#131824=CARTESIAN_POINT('Ctrl Pts',(-8.80933590722104,-71.0287732217429,
-55.5465658668829));
#131825=CARTESIAN_POINT('Ctrl Pts',(-8.96386239650929,-70.6628838067398,
-55.0780797399289));
#131826=CARTESIAN_POINT('Ctrl Pts',(-8.74741150404566,-70.6964574226719,
-55.3507681953891));
#131827=CARTESIAN_POINT('Ctrl Pts',(-8.72031210976081,-71.028802992332,
-55.4457995958176));
#131828=CARTESIAN_POINT('Ctrl Pts',(-8.85596081453515,-70.679599541712,
-55.0012953993776));
#131829=CARTESIAN_POINT('Ctrl Pts',(-8.67980906181977,-70.7065384951403,
-55.2998814604833));
#131830=CARTESIAN_POINT('Ctrl Pts',(-8.66589931539785,-71.0341559413021,
-55.4063653507056));
#131831=CARTESIAN_POINT('Ctrl Pts',(-8.61934915026951,-70.7154116132197,
-54.8994528680703));
#131832=CARTESIAN_POINT('Ctrl Pts',(-8.53037007175256,-70.7286009969627,
-55.2361886195963));
#131833=CARTESIAN_POINT('Ctrl Pts',(-8.5465803724842,-71.0525391488732,
-55.3555557927532));
#131834=CARTESIAN_POINT('Ctrl Pts',(-8.48994814797731,-70.7346037655486,
-54.8739206038906));
#131835=CARTESIAN_POINT('Ctrl Pts',(-8.44749087161521,-70.7407315090392,
-55.2227831389152));
#131836=CARTESIAN_POINT('Ctrl Pts',(-8.48132333269968,-71.0655965765406,
-55.3439422058852));
#131837=CARTESIAN_POINT('Ctrl Pts',(-8.35962920986983,-70.7534564084689,
-54.8763024037294));
#131838=CARTESIAN_POINT('Ctrl Pts',(-8.36589323739407,-70.7525502203441,
-55.2292031667485));
#131839=CARTESIAN_POINT('Ctrl Pts',(-8.41560835021371,-71.0814043774774,
-55.3473655916161));
#131840=CARTESIAN_POINT('',(-9.32018679685842,-70.6063261212332,-55.8925850873));
#131841=CARTESIAN_POINT('Ctrl Pts',(-8.35962920986984,-70.7534564084689,
-54.8763024037297));
#131842=CARTESIAN_POINT('Ctrl Pts',(-8.42669320976301,-70.7437545672695,
-54.8750766952757));
#131843=CARTESIAN_POINT('Ctrl Pts',(-8.49356141096547,-70.7339558949385,
-54.8812481493055));
#131844=CARTESIAN_POINT('Ctrl Pts',(-8.5587840601874,-70.7242909712569,
-54.894476436547));
#131845=CARTESIAN_POINT('Ctrl Pts',(-8.62027176255611,-70.715179505258,
-54.9069472116299));
#131846=CARTESIAN_POINT('Ctrl Pts',(-8.68029576330479,-70.7061871116828,
-54.9256889700024));
#131847=CARTESIAN_POINT('Ctrl Pts',(-8.73765415640112,-70.6975057024889,
-54.9503761135537));
#131848=CARTESIAN_POINT('Ctrl Pts',(-8.73812533670876,-70.6974343875717,
-54.950578910307));
#131849=CARTESIAN_POINT('Ctrl Pts',(-8.7385963482321,-70.6973630921029,
-54.9507821155763));
#131850=CARTESIAN_POINT('Ctrl Pts',(-8.73906719037139,-70.697291816191,
-54.9509857288994));
#131851=CARTESIAN_POINT('Ctrl Pts',(-8.81806341257093,-70.6853333967876,
-54.9851472492404));
#131852=CARTESIAN_POINT('Ctrl Pts',(-8.89230144999735,-70.6739241189874,
-55.0307996075112));
#131853=CARTESIAN_POINT('Ctrl Pts',(-8.95909820839892,-70.6635530304614,
-55.0858633072379));
#131854=CARTESIAN_POINT('Ctrl Pts',(-8.99202329692719,-70.658440970894,
-55.1130050014095));
#131855=CARTESIAN_POINT('Ctrl Pts',(-9.02314073107063,-70.6535810854988,
-55.1424341547024));
#131856=CARTESIAN_POINT('Ctrl Pts',(-9.05213028602995,-70.6490316704449,
-55.1739060774789));
#131857=CARTESIAN_POINT('Ctrl Pts',(-9.05261593139238,-70.6489554567077,
-55.1744333085235));
#131858=CARTESIAN_POINT('Ctrl Pts',(-9.05310095531286,-70.6488793344915,
-55.1749610621635));
#131859=CARTESIAN_POINT('Ctrl Pts',(-9.05358535746144,-70.6488033038874,
-55.1754893372344));
#131860=CARTESIAN_POINT('Ctrl Pts',(-9.1020755169914,-70.641192404282,-55.2283713125433));
#131861=CARTESIAN_POINT('Ctrl Pts',(-9.14429186553979,-70.6345063768039,
-55.2864243412901));
#131862=CARTESIAN_POINT('Ctrl Pts',(-9.17994788064335,-70.6288295105426,
-55.348502954041));
#131863=CARTESIAN_POINT('Ctrl Pts',(-9.20880098471981,-70.6242357495014,
-55.3987374143254));
#131864=CARTESIAN_POINT('Ctrl Pts',(-9.23335776597293,-70.6203028545583,
-55.4516091557798));
#131865=CARTESIAN_POINT('Ctrl Pts',(-9.25344901950571,-70.6170779672838,
-55.5065287627148));
#131866=CARTESIAN_POINT('Ctrl Pts',(-9.25361952044245,-70.6170505998375,
-55.506994828429));
#131867=CARTESIAN_POINT('Ctrl Pts',(-9.25378968425506,-70.6170232859403,
-55.5074609965585));
#131868=CARTESIAN_POINT('Ctrl Pts',(-9.25395951106862,-70.6169960255762,
-55.5079272667724));
#131869=CARTESIAN_POINT('Ctrl Pts',(-9.26917261736368,-70.6145540388982,
-55.5496958083666));
#131870=CARTESIAN_POINT('Ctrl Pts',(-9.28164780823391,-70.6125470433612,
-55.5921779695173));
#131871=CARTESIAN_POINT('Ctrl Pts',(-9.2915203488035,-70.6109563835461,
-55.6352174890368));
#131872=CARTESIAN_POINT('Ctrl Pts',(-9.30173630321666,-70.609310393029,
-55.6797541274306));
#131873=CARTESIAN_POINT('Ctrl Pts',(-9.30916540444186,-70.6081101941254,
-55.7248883638109));
#131874=CARTESIAN_POINT('Ctrl Pts',(-9.31390296845358,-70.6073438342246,
-55.7704597578367));
#131875=CARTESIAN_POINT('Ctrl Pts',(-9.31810307746837,-70.606664414354,
-55.8108612853708));
#131876=CARTESIAN_POINT('Ctrl Pts',(-9.32018679673735,-70.6063261212527,
-55.8516070077996));
#131877=CARTESIAN_POINT('Ctrl Pts',(-9.32018679685842,-70.6063261212332,
-55.8925850873));
#131878=CARTESIAN_POINT('',(-8.89999999157093,-71.0999148696892,-55.8925850873042));
#131879=CARTESIAN_POINT('Origin',(-9.4,-71.0999148696911,-55.8925850873));
#131880=CARTESIAN_POINT('Ctrl Pts',(-8.9,-71.0999148696911,-55.8925850873));
#131881=CARTESIAN_POINT('Ctrl Pts',(-8.9,-71.0753963340341,-55.8158206410579));
#131882=CARTESIAN_POINT('Ctrl Pts',(-8.88914819160783,-71.0574685211989,
-55.7424878932553));
#131883=CARTESIAN_POINT('Ctrl Pts',(-8.84354256567003,-71.0340357122248,
-55.606998619986));
#131884=CARTESIAN_POINT('Ctrl Pts',(-8.80933590722104,-71.0287732217429,
-55.5465658668829));
#131885=CARTESIAN_POINT('Ctrl Pts',(-8.72031210976081,-71.028802992332,
-55.4457995958176));
#131886=CARTESIAN_POINT('Ctrl Pts',(-8.66589931539785,-71.0341559413021,
-55.4063653507056));
#131887=CARTESIAN_POINT('Ctrl Pts',(-8.5465803724842,-71.0525391488732,
-55.3555557927532));
#131888=CARTESIAN_POINT('Ctrl Pts',(-8.48132333269968,-71.0655965765406,
-55.3439422058852));
#131889=CARTESIAN_POINT('Ctrl Pts',(-8.41560835021378,-71.0814043774777,
-55.3473655916165));
#131890=CARTESIAN_POINT('Origin',(-9.4,-71.0999148696911,-55.24995));
#131891=CARTESIAN_POINT('',(-8.9,-71.0999148696911,-60.4282553373601));
#131892=CARTESIAN_POINT('',(-9.32018679685842,-70.6063261212332,-60.4282553373601));
#131893=CARTESIAN_POINT('Origin',(-9.4,-71.0999148696911,-60.4282553373601));
#131894=CARTESIAN_POINT('',(-8.9,-71.0999148696911,-55.24995));
#131895=CARTESIAN_POINT('',(-9.32018679685842,-70.6063261212332,-55.24995));
#131896=CARTESIAN_POINT('Origin',(0.,-12.9675000200281,-60.42825533736));
#131897=CARTESIAN_POINT('',(-14.9339094669349,-69.3159372152925,-60.8508735991008));
#131898=CARTESIAN_POINT('',(-9.32749162718857,-70.5102313269446,-60.8508735991008));
#131899=CARTESIAN_POINT('Origin',(0.,-12.9675000200281,-60.8508735991007));
#131900=CARTESIAN_POINT('Origin',(-9.4006078237226,-69.5628833426966,-60.4240593941771));
#131901=CARTESIAN_POINT('',(-14.9222139673106,-69.4159516070034,-60.4282553373601));
#131902=CARTESIAN_POINT('Origin',(0.,-12.9675000200281,-60.42825533736));
#131903=CARTESIAN_POINT('Origin',(-15.0817374974215,-68.0546682136643,-60.3659067766217));
#131904=CARTESIAN_POINT('Origin',(-15.05,-69.8993466109593,-55.24995));
#131905=CARTESIAN_POINT('',(-14.9222139673106,-69.4159516070034,-55.74995));
#131906=CARTESIAN_POINT('',(-15.55,-69.8993466109593,-55.74995));
#131907=CARTESIAN_POINT('Origin',(-15.05,-69.8993466109593,-55.74995));
#131908=CARTESIAN_POINT('',(-15.55,-69.8993466109592,-60.4282553373601));
#131909=CARTESIAN_POINT('',(-15.55,-69.8993466109593,-55.24995));
#131910=CARTESIAN_POINT('',(-15.05,-69.3993466109593,-60.4282553373601));
#131911=CARTESIAN_POINT('Origin',(-15.05,-69.8993466109592,-60.4282553373601));
#131912=CARTESIAN_POINT('Origin',(-15.05,-69.8993466109592,-60.4282553373601));
#131913=CARTESIAN_POINT('',(-14.9222139673106,-69.4159516070034,-55.24995));
#131914=CARTESIAN_POINT('Ctrl Pts',(-15.9137232010189,-69.1444843653509,
-54.74995));
#131915=CARTESIAN_POINT('Ctrl Pts',(-15.9137232010189,-69.1444843653508,
-55.24995));
#131916=CARTESIAN_POINT('Ctrl Pts',(-16.05,-69.6255546658887,-55.24995));
#131917=CARTESIAN_POINT('Ctrl Pts',(-15.6596579837658,-69.2164555398362,
-54.7499500371751));
#131918=CARTESIAN_POINT('Ctrl Pts',(-15.771227820187,-69.1848502198413,
-55.2866827527478));
#131919=CARTESIAN_POINT('Ctrl Pts',(-15.9218478003938,-69.698160151404,
-55.24995));
#131920=CARTESIAN_POINT('Ctrl Pts',(-15.40465081614,-69.286534600552,-54.8528648356211));
#131921=CARTESIAN_POINT('Ctrl Pts',(-15.6724279126842,-69.212867833855,
-55.3793785506899));
#131922=CARTESIAN_POINT('Ctrl Pts',(-15.7932840899848,-69.7688213437999,
-55.3014074151129));
#131923=CARTESIAN_POINT('Ctrl Pts',(-15.0344159790517,-69.3864973437867,
-55.2190131651604));
#131924=CARTESIAN_POINT('Ctrl Pts',(-15.5617369148846,-69.2455690283436,
-55.5713612535417));
#131925=CARTESIAN_POINT('Ctrl Pts',(-15.6065814283354,-69.8696401180232,
-55.4844815852779));
#131926=CARTESIAN_POINT('Ctrl Pts',(-14.9222139938746,-69.4159515999812,
-55.4795342126294));
#131927=CARTESIAN_POINT('Ctrl Pts',(-15.5500000039585,-69.2499956362206,
-55.6640902421462));
#131928=CARTESIAN_POINT('Ctrl Pts',(-15.55,-69.8993466038797,-55.6147421042263));
#131929=CARTESIAN_POINT('Ctrl Pts',(-14.9222139673106,-69.4159516070034,
-55.74995));
#131930=CARTESIAN_POINT('Ctrl Pts',(-15.55,-69.2499956375816,-55.74995));
#131931=CARTESIAN_POINT('Ctrl Pts',(-15.55,-69.8993466109593,-55.74995));
#131932=CARTESIAN_POINT('',(-15.913723201019,-69.1444843653509,-54.74995));
#131933=CARTESIAN_POINT('Ctrl Pts',(-14.9222139673106,-69.4159516070034,
-55.74995));
#131934=CARTESIAN_POINT('Ctrl Pts',(-14.9222139938746,-69.4159515999812,
-55.4795342126294));
#131935=CARTESIAN_POINT('Ctrl Pts',(-15.0344159790517,-69.3864973437867,
-55.2190131651604));
#131936=CARTESIAN_POINT('Ctrl Pts',(-15.40465081614,-69.286534600552,-54.8528648356211));
#131937=CARTESIAN_POINT('Ctrl Pts',(-15.6596579837658,-69.2164555398362,
-54.7499500371751));
#131938=CARTESIAN_POINT('Ctrl Pts',(-15.913723201019,-69.1444843653509,
-54.74995));
#131939=CARTESIAN_POINT('',(-16.05,-69.6255546658886,-55.24995));
#131940=CARTESIAN_POINT('Origin',(-16.05,-69.6255546658886,-54.74995));
#131941=CARTESIAN_POINT('Ctrl Pts',(-16.05,-69.6255546658886,-55.24995));
#131942=CARTESIAN_POINT('Ctrl Pts',(-15.9218478003938,-69.698160151404,
-55.24995));
#131943=CARTESIAN_POINT('Ctrl Pts',(-15.7932840899848,-69.7688213437999,
-55.3014074151129));
#131944=CARTESIAN_POINT('Ctrl Pts',(-15.6065814283354,-69.8696401180232,
-55.4844815852779));
#131945=CARTESIAN_POINT('Ctrl Pts',(-15.55,-69.8993466038797,-55.6147421042263));
#131946=CARTESIAN_POINT('Ctrl Pts',(-15.55,-69.8993466109593,-55.74995));
#131947=CARTESIAN_POINT('Origin',(0.,-12.9675000200281,-54.74995));
#131948=CARTESIAN_POINT('',(-16.4094778178732,-69.001678821881,-54.74995));
#131949=CARTESIAN_POINT('Origin',(0.,-12.9675000200281,-54.74995));
#131950=CARTESIAN_POINT('',(-16.55,-69.4815262104643,-55.24995));
#131951=CARTESIAN_POINT('Origin',(-16.55,-69.4815262104644,-54.74995));
#131952=CARTESIAN_POINT('Origin',(0.,-12.9675000200281,-55.24995));
#131953=CARTESIAN_POINT('Ctrl Pts',(-17.4009870515814,-68.7017426890013,
-55.74995));
#131954=CARTESIAN_POINT('Ctrl Pts',(-17.05,-68.8113256105117,-55.74995));
#131955=CARTESIAN_POINT('Ctrl Pts',(-17.05,-69.1790215814778,-55.74995));
#131956=CARTESIAN_POINT('Ctrl Pts',(-17.4009870278268,-68.7017426964178,
-55.6164169522954));
#131957=CARTESIAN_POINT('Ctrl Pts',(-17.0499999824983,-68.8113256158083,
-55.6678220871153));
#131958=CARTESIAN_POINT('Ctrl Pts',(-17.05,-69.179021588958,-55.683183477332));
#131959=CARTESIAN_POINT('Ctrl Pts',(-17.3738309471109,-68.7102398223756,
-55.4822907797671));
#131960=CARTESIAN_POINT('Ctrl Pts',(-17.0296370884236,-68.8175010382642,
-55.5850039716587));
#131961=CARTESIAN_POINT('Ctrl Pts',(-17.0363056762739,-69.1875914802515,
-55.6161203882819));
#131962=CARTESIAN_POINT('Ctrl Pts',(-17.2712219065013,-68.7421173320939,
-55.237857759257));
#131963=CARTESIAN_POINT('Ctrl Pts',(-16.9553391166104,-68.8399176416641,
-55.4404431349053));
#131964=CARTESIAN_POINT('Ctrl Pts',(-16.9845618032129,-69.2197419714937,
-55.4939038812302));
#131965=CARTESIAN_POINT('Ctrl Pts',(-17.1955506950046,-68.7655509085055,
-55.1267370897427));
#131966=CARTESIAN_POINT('Ctrl Pts',(-16.9005894152091,-68.8563914475931,
-55.377823329943));
#131967=CARTESIAN_POINT('Ctrl Pts',(-16.9464021983051,-69.2433762217045,
-55.4383435435979));
#131968=CARTESIAN_POINT('Ctrl Pts',(-17.0112333722604,-68.8220198533602,
-54.9445960314883));
#131969=CARTESIAN_POINT('Ctrl Pts',(-16.7737497934953,-68.8942921521941,
-55.2851829950906));
#131970=CARTESIAN_POINT('Ctrl Pts',(-16.8534543357224,-69.300328736023,
-55.3472730170175));
#131971=CARTESIAN_POINT('Ctrl Pts',(-16.9010650546211,-68.8555068833233,
-54.8720727600904));
#131972=CARTESIAN_POINT('Ctrl Pts',(-16.6998467063121,-68.9162473809411,
-55.2547261014823));
#131973=CARTESIAN_POINT('Ctrl Pts',(-16.7978984661854,-69.3341025322853,
-55.3110113805052));
#131974=CARTESIAN_POINT('Ctrl Pts',(-16.6652454739222,-68.9262786380983,
-54.7753009573657));
#131975=CARTESIAN_POINT('Ctrl Pts',(-16.5521913264397,-68.9598430749121,
-55.2279532590823));
#131976=CARTESIAN_POINT('Ctrl Pts',(-16.6789789583454,-69.4054803385803,
-55.2626254782229));
#131977=CARTESIAN_POINT('Ctrl Pts',(-16.5367871504596,-68.9643965824736,
-54.7499500149468));
#131978=CARTESIAN_POINT('Ctrl Pts',(-16.4764075692004,-68.9820786017848,
-55.2322379892913));
#131979=CARTESIAN_POINT('Ctrl Pts',(-16.6141964540128,-69.4439266482582,
-55.24995));
#131980=CARTESIAN_POINT('Ctrl Pts',(-16.4094778178732,-69.001678821881,
-54.74995));
#131981=CARTESIAN_POINT('Ctrl Pts',(-16.4094778178731,-69.001678821881,
-55.24995));
#131982=CARTESIAN_POINT('Ctrl Pts',(-16.55,-69.4815262104644,-55.24995));
#131983=CARTESIAN_POINT('',(-17.4009870515814,-68.7017426890012,-55.74995));
#131984=CARTESIAN_POINT('Ctrl Pts',(-16.4094778178732,-69.001678821881,
-54.74995));
#131985=CARTESIAN_POINT('Ctrl Pts',(-16.4504095598616,-68.9896920572568,
-54.7499500048056));
#131986=CARTESIAN_POINT('Ctrl Pts',(-16.4912475287742,-68.9776812452657,
-54.7525666780149));
#131987=CARTESIAN_POINT('Ctrl Pts',(-16.5317041745654,-68.965736321318,
-54.757667934043));
#131988=CARTESIAN_POINT('Ctrl Pts',(-16.5749366447117,-68.9529718284177,
-54.7631191990857));
#131989=CARTESIAN_POINT('Ctrl Pts',(-16.6177350648204,-68.9402821612408,
-54.771407370512));
#131990=CARTESIAN_POINT('Ctrl Pts',(-16.659758562013,-68.9277728443736,
-54.7824337221976));
#131991=CARTESIAN_POINT('Ctrl Pts',(-16.7017820592057,-68.9152635275064,
-54.7934600738833));
#131992=CARTESIAN_POINT('Ctrl Pts',(-16.7430322683556,-68.9029340622973,
-54.8072249335998));
#131993=CARTESIAN_POINT('Ctrl Pts',(-16.7831545131606,-68.8908929861314,
-54.8236888710244));
#131994=CARTESIAN_POINT('Ctrl Pts',(-16.7835975596796,-68.890760023559,
-54.8238706726708));
#131995=CARTESIAN_POINT('Ctrl Pts',(-16.7840405080022,-68.8906270844636,
-54.8240528195673));
#131996=CARTESIAN_POINT('Ctrl Pts',(-16.7844833577117,-68.8904941689839,
-54.8242353115275));
#131997=CARTESIAN_POINT('Ctrl Pts',(-16.8581304439988,-68.8683899706622,
-54.8545842106015));
#131998=CARTESIAN_POINT('Ctrl Pts',(-16.9287006566096,-68.8470438209494,
-54.8943416412349));
#131999=CARTESIAN_POINT('Ctrl Pts',(-16.9936792242025,-68.8272773402426,
-54.9420858838156));
#132000=CARTESIAN_POINT('Ctrl Pts',(-17.0324101749564,-68.815495384758,
-54.970544189018));
#132001=CARTESIAN_POINT('Ctrl Pts',(-17.0691551792516,-68.8042744590646,
-55.0018396382534));
#132002=CARTESIAN_POINT('Ctrl Pts',(-17.1033900455892,-68.7937859900155,
-55.0356687800906));
#132003=CARTESIAN_POINT('Ctrl Pts',(-17.103886172442,-68.7936339926019,
-55.0361590272412));
#132004=CARTESIAN_POINT('Ctrl Pts',(-17.1043818163765,-68.7934821358841,
-55.0366498500402));
#132005=CARTESIAN_POINT('Ctrl Pts',(-17.1048769761793,-68.7933304202781,
-55.0371412470353));
#132006=CARTESIAN_POINT('Ctrl Pts',(-17.1669690008271,-68.7743055941548,
-55.0987614233146));
#132007=CARTESIAN_POINT('Ctrl Pts',(-17.2214535479523,-68.7574981762719,
-55.1694239623158));
#132008=CARTESIAN_POINT('Ctrl Pts',(-17.2659841189476,-68.7437133283472,
-55.2463463516028));
#132009=CARTESIAN_POINT('Ctrl Pts',(-17.2871667241188,-68.7371560580403,
-55.2829373174196));
#132010=CARTESIAN_POINT('Ctrl Pts',(-17.3060972390716,-68.7312826257117,
-55.3209455236331));
#132011=CARTESIAN_POINT('Ctrl Pts',(-17.322524151481,-68.7261792841162,
-55.3600753258131));
#132012=CARTESIAN_POINT('Ctrl Pts',(-17.3227235277485,-68.7261173439796,
-55.3605502509672));
#132013=CARTESIAN_POINT('Ctrl Pts',(-17.3229225385083,-68.7260555164805,
-55.3610253536613));
#132014=CARTESIAN_POINT('Ctrl Pts',(-17.3231211835968,-68.7259938016769,
-55.3615006331605));
#132015=CARTESIAN_POINT('Ctrl Pts',(-17.3377397858477,-68.7214521129136,
-55.3964771936486));
#132016=CARTESIAN_POINT('Ctrl Pts',(-17.3503329508714,-68.717534766207,
-55.4322944098896));
#132017=CARTESIAN_POINT('Ctrl Pts',(-17.3608936617493,-68.7142467873541,
-55.4687543689715));
#132018=CARTESIAN_POINT('Ctrl Pts',(-17.3714744037536,-68.7109525719968,
-55.5052834838195));
#132019=CARTESIAN_POINT('Ctrl Pts',(-17.3800152474177,-68.70829001851,-55.5424589028238));
#132020=CARTESIAN_POINT('Ctrl Pts',(-17.3864625050711,-68.7062785938727,
-55.5800999366541));
#132021=CARTESIAN_POINT('Ctrl Pts',(-17.3927323721603,-68.7043225117965,
-55.6167053108928));
#132022=CARTESIAN_POINT('Ctrl Pts',(-17.3970223360455,-68.7029821923561,
-55.6537520599017));
#132023=CARTESIAN_POINT('Ctrl Pts',(-17.399236871165,-68.7022899564979,
-55.6910754862815));
#132024=CARTESIAN_POINT('Ctrl Pts',(-17.4003972743764,-68.7019272290316,
-55.7106327393814));
#132025=CARTESIAN_POINT('Ctrl Pts',(-17.4009870480798,-68.7017426900946,
-55.7302658927369));
#132026=CARTESIAN_POINT('Ctrl Pts',(-17.4009870515814,-68.7017426890013,
-55.74995));
#132027=CARTESIAN_POINT('',(-17.05,-69.1790215814778,-55.74995));
#132028=CARTESIAN_POINT('Origin',(-17.55,-69.1790215814778,-55.74995));
#132029=CARTESIAN_POINT('Ctrl Pts',(-17.05,-69.1790215814778,-55.74995));
#132030=CARTESIAN_POINT('Ctrl Pts',(-17.05,-69.1790215840141,-55.7273117036717));
#132031=CARTESIAN_POINT('Ctrl Pts',(-17.0484581724605,-69.1800068330463,
-55.704632518585));
#132032=CARTESIAN_POINT('Ctrl Pts',(-17.045383935534,-69.1819358319623,
-55.6821653674136));
#132033=CARTESIAN_POINT('Ctrl Pts',(-17.0423062744033,-69.183866979472,
-55.6596731914591));
#132034=CARTESIAN_POINT('Ctrl Pts',(-17.0376928923171,-69.1867439804066,
-55.6373943130373));
#132035=CARTESIAN_POINT('Ctrl Pts',(-17.0316050134448,-69.1905251993378,
-55.6155751101402));
#132036=CARTESIAN_POINT('Ctrl Pts',(-17.0258391557959,-69.1941064089108,
-55.5949100442681));
#132037=CARTESIAN_POINT('Ctrl Pts',(-17.0187512873944,-69.1984987083453,
-55.5746577770516));
#132038=CARTESIAN_POINT('Ctrl Pts',(-17.0104337397434,-69.2036667258726,
-55.555012134756));
#132039=CARTESIAN_POINT('Ctrl Pts',(-17.0013343801787,-69.2093205137066,
-55.5335198908125));
#132040=CARTESIAN_POINT('Ctrl Pts',(-16.9907376252434,-69.2159093376612,
-55.512693370794));
#132041=CARTESIAN_POINT('Ctrl Pts',(-16.9787804466987,-69.2233149929863,
-55.4927587705056));
#132042=CARTESIAN_POINT('Ctrl Pts',(-16.9667872973728,-69.2307429267449,
-55.4727642009576));
#132043=CARTESIAN_POINT('Ctrl Pts',(-16.9534260163454,-69.2389926138138,
-55.4536675252671));
#132044=CARTESIAN_POINT('Ctrl Pts',(-16.9388754710694,-69.2479447794443,
-55.4356637164931));
#132045=CARTESIAN_POINT('Ctrl Pts',(-16.9266858743886,-69.2554443807571,
-55.4205811774192));
#132046=CARTESIAN_POINT('Ctrl Pts',(-16.9136625469686,-69.2634369892112,
-55.4062651589592));
#132047=CARTESIAN_POINT('Ctrl Pts',(-16.8999282670137,-69.2718524788637,
-55.3928082803077));
#132048=CARTESIAN_POINT('Ctrl Pts',(-16.8836819568998,-69.2818071801734,
-55.3768901088086));
#132049=CARTESIAN_POINT('Ctrl Pts',(-16.8663408763305,-69.2924092697525,
-55.3620781535359));
#132050=CARTESIAN_POINT('Ctrl Pts',(-16.8481019051626,-69.3035142485201,
-55.3485334406276));
#132051=CARTESIAN_POINT('Ctrl Pts',(-16.8298276464078,-69.3146407124856,
-55.3349625222809));
#132052=CARTESIAN_POINT('Ctrl Pts',(-16.8106526893114,-69.3262720134373,
-55.3226641848208));
#132053=CARTESIAN_POINT('Ctrl Pts',(-16.7908030911076,-69.3382628119682,
-55.3117561258837));
#132054=CARTESIAN_POINT('Ctrl Pts',(-16.7737921641089,-69.3485388183827,
-55.3024080175557));
#132055=CARTESIAN_POINT('Ctrl Pts',(-16.7562864891711,-69.3590788518886,
-55.2940803227657));
#132056=CARTESIAN_POINT('Ctrl Pts',(-16.7384387122654,-69.3697914354328,
-55.286818429364));
#132057=CARTESIAN_POINT('Ctrl Pts',(-16.7180829214159,-69.3820093778262,
-55.2785360766634));
#132058=CARTESIAN_POINT('Ctrl Pts',(-16.6971109842387,-69.3945504898523,
-55.2715719188538));
#132059=CARTESIAN_POINT('Ctrl Pts',(-16.6757471551705,-69.407270161634,
-55.2660206115904));
#132060=CARTESIAN_POINT('Ctrl Pts',(-16.6543745545499,-69.4199950558536,
-55.2604670250734));
#132061=CARTESIAN_POINT('Ctrl Pts',(-16.6326105138126,-69.4328986564849,
-55.2563277011337));
#132062=CARTESIAN_POINT('Ctrl Pts',(-16.6106950449315,-69.4458361754561,
-55.2536475604324));
#132063=CARTESIAN_POINT('Ctrl Pts',(-16.590527650153,-69.4577417410619,
-55.251181199531));
#132064=CARTESIAN_POINT('Ctrl Pts',(-16.5702326710683,-69.4696760298565,
-55.24995));
#132065=CARTESIAN_POINT('Ctrl Pts',(-16.55,-69.4815262104643,-55.24995));
#132066=CARTESIAN_POINT('Origin',(-17.55,-69.1790215814778,-55.24995));
#132067=CARTESIAN_POINT('',(-17.05,-69.1790215814778,-60.42825533736));
#132068=CARTESIAN_POINT('',(-17.4009870515814,-68.7017426890012,-60.42825533736));
#132069=CARTESIAN_POINT('Origin',(-17.55,-69.1790215814778,-60.42825533736));
#132070=CARTESIAN_POINT('',(-17.05,-69.1790215814778,-55.24995));
#132071=CARTESIAN_POINT('',(-17.4009870515814,-68.7017426890012,-55.24995));
#132072=CARTESIAN_POINT('Origin',(0.,-12.9675000200281,-60.42825533736));
#132073=CARTESIAN_POINT('',(-23.0210431649761,-66.5230748737403,-60.8508735991007));
#132074=CARTESIAN_POINT('',(-17.4146253252297,-68.5993151180197,-60.8508735991007));
#132075=CARTESIAN_POINT('Origin',(0.,-12.9675000200281,-60.8508735991007));
#132076=CARTESIAN_POINT('Origin',(-17.5536315931459,-67.566484588888,-60.418466472047));
#132077=CARTESIAN_POINT('',(-23.0030142220336,-66.6327727106072,-60.42825533736));
#132078=CARTESIAN_POINT('Origin',(0.,-12.9675000200281,-60.42825533736));
#132079=CARTESIAN_POINT('Origin',(-23.206372880927,-65.3976857628708,-60.4139613002479));
#132080=CARTESIAN_POINT('Origin',(-23.2,-67.0923340267327,-55.24995));
#132081=CARTESIAN_POINT('',(-23.0030142220336,-66.6327727106072,-55.74995));
#132082=CARTESIAN_POINT('',(-23.7,-67.0923340267327,-55.74995));
#132083=CARTESIAN_POINT('Origin',(-23.2,-67.0923340267327,-55.74995));
#132084=CARTESIAN_POINT('',(-23.7,-67.0923340267327,-60.42825533736));
#132085=CARTESIAN_POINT('',(-23.7,-67.0923340267327,-55.24995));
#132086=CARTESIAN_POINT('Origin',(-23.2,-67.0923340267327,-60.42825533736));
#132087=CARTESIAN_POINT('',(-23.0030142220336,-66.6327727106072,-55.24995));
#132088=CARTESIAN_POINT('Ctrl Pts',(-23.9945234557419,-66.1968434349636,
-54.74995));
#132089=CARTESIAN_POINT('Ctrl Pts',(-23.9945234557419,-66.1968434349636,
-55.24995));
#132090=CARTESIAN_POINT('Ctrl Pts',(-24.2,-66.6526716808631,-55.24995));
#132091=CARTESIAN_POINT('Ctrl Pts',(-23.8699830688991,-66.2529832826787,
-54.7499500150097));
#132092=CARTESIAN_POINT('Ctrl Pts',(-23.9202432240961,-66.2303271978257,
-55.2764502978682));
#132093=CARTESIAN_POINT('Ctrl Pts',(-24.1371955572435,-66.7092931820382,
-55.24995));
#132094=CARTESIAN_POINT('Ctrl Pts',(-23.7474276190468,-66.3076948875735,
-54.7731313367517));
#132095=CARTESIAN_POINT('Ctrl Pts',(-23.8581370153758,-66.2582349963978,
-55.3179716549212));
#132096=CARTESIAN_POINT('Ctrl Pts',(-24.0753940809144,-66.764472406879,
-55.2615406660682));
#132097=CARTESIAN_POINT('Ctrl Pts',(-23.5121407959317,-66.4118256516783,
-54.867008414748));
#132098=CARTESIAN_POINT('Ctrl Pts',(-23.7601274312421,-66.3025641007665,
-55.4174636561498));
#132099=CARTESIAN_POINT('Ctrl Pts',(-23.9567432347527,-66.8694948932304,
-55.3084792096817));
#132100=CARTESIAN_POINT('Ctrl Pts',(-23.4042122584794,-66.4591215590598,
-54.9358182281615));
#132101=CARTESIAN_POINT('Ctrl Pts',(-23.7282344734586,-66.3172128520127,
-55.4737170925055));
#132102=CARTESIAN_POINT('Ctrl Pts',(-23.902316841733,-66.9171958169871,
-55.3428841126209));
#132103=CARTESIAN_POINT('Ctrl Pts',(-23.2156877780054,-66.5412115519831,
-55.117294361456));
#132104=CARTESIAN_POINT('Ctrl Pts',(-23.6919934707232,-66.3346728811278,
-55.5807863787511));
#132105=CARTESIAN_POINT('Ctrl Pts',(-23.8072473920369,-66.9999887868491,
-55.4336221821879));
#132106=CARTESIAN_POINT('Ctrl Pts',(-23.138673673191,-66.5744522205999,
-55.227252767375));
#132107=CARTESIAN_POINT('Ctrl Pts',(-23.6899497583265,-66.3364476351196,
-55.6278104638636));
#132108=CARTESIAN_POINT('Ctrl Pts',(-23.7684105820677,-67.0335141101085,
-55.4886013829516));
#132109=CARTESIAN_POINT('Ctrl Pts',(-23.0317566828166,-66.6204750325317,
-55.4753103039836));
#132110=CARTESIAN_POINT('Ctrl Pts',(-23.6944387661923,-66.3359499016387,
-55.7013955638849));
#132111=CARTESIAN_POINT('Ctrl Pts',(-23.7144942998795,-67.079931038232,
-55.6126301527277));
#132112=CARTESIAN_POINT('Ctrl Pts',(-23.0030142327697,-66.6327727060053,
-55.6101370134438));
#132113=CARTESIAN_POINT('Ctrl Pts',(-23.6999999982635,-66.3340176139022,
-55.7259208430489));
#132114=CARTESIAN_POINT('Ctrl Pts',(-23.7,-67.0923340220896,-55.6800435061715));
#132115=CARTESIAN_POINT('Ctrl Pts',(-23.0030142220336,-66.6327727106072,
-55.74995));
#132116=CARTESIAN_POINT('Ctrl Pts',(-23.6999999999999,-66.3340176133293,
-55.74995));
#132117=CARTESIAN_POINT('Ctrl Pts',(-23.7,-67.0923340267327,-55.74995));
#132118=CARTESIAN_POINT('',(-23.9945234557419,-66.1968434349636,-54.74995));
#132119=CARTESIAN_POINT('Ctrl Pts',(-23.0030142220336,-66.6327727106072,
-55.74995));
#132120=CARTESIAN_POINT('Ctrl Pts',(-23.0030142252181,-66.6327727092422,
-55.7084794961837));
#132121=CARTESIAN_POINT('Ctrl Pts',(-23.0055473075491,-66.6316889244747,
-55.6672305708314));
#132122=CARTESIAN_POINT('Ctrl Pts',(-23.01056277729,-66.6295393332012,-55.6264611420266));
#132123=CARTESIAN_POINT('Ctrl Pts',(-23.0156442349954,-66.62736146,-55.585155314488));
#132124=CARTESIAN_POINT('Ctrl Pts',(-23.0232736525723,-66.6240896154023,
-55.5443421797599));
#132125=CARTESIAN_POINT('Ctrl Pts',(-23.0333489722998,-66.6197635354293,
-55.5042845968467));
#132126=CARTESIAN_POINT('Ctrl Pts',(-23.0435966387887,-66.6153634542441,
-55.4635417955117));
#132127=CARTESIAN_POINT('Ctrl Pts',(-23.0563743830217,-66.6098728426923,
-55.4235811788329));
#132128=CARTESIAN_POINT('Ctrl Pts',(-23.0715270926203,-66.6033540441774,
-55.3846656949086));
#132129=CARTESIAN_POINT('Ctrl Pts',(-23.075698862771,-66.6015593203436,
-55.3739516735531));
#132130=CARTESIAN_POINT('Ctrl Pts',(-23.08005038839,-66.5996867754406,-55.3633167653533));
#132131=CARTESIAN_POINT('Ctrl Pts',(-23.0845778500673,-66.5977379631867,
-55.3527661917799));
#132132=CARTESIAN_POINT('Ctrl Pts',(-23.084790216786,-66.5976465515099,
-55.3522713028445));
#132133=CARTESIAN_POINT('Ctrl Pts',(-23.0850029782865,-66.5975549687209,
-55.3517765816013));
#132134=CARTESIAN_POINT('Ctrl Pts',(-23.0852161343291,-66.5974632149135,
-55.3512820284305));
#132135=CARTESIAN_POINT('Ctrl Pts',(-23.1225303099355,-66.5814011899271,
-55.2647076876699));
#132136=CARTESIAN_POINT('Ctrl Pts',(-23.171373896406,-66.560332705268,-55.1848774594358));
#132137=CARTESIAN_POINT('Ctrl Pts',(-23.2296539151234,-66.5350590387648,
-55.1136222625269));
#132138=CARTESIAN_POINT('Ctrl Pts',(-23.254282078481,-66.5243788090568,
-55.0835110053899));
#132139=CARTESIAN_POINT('Ctrl Pts',(-23.2805947528025,-66.5129478823944,
-55.0549311560836));
#132140=CARTESIAN_POINT('Ctrl Pts',(-23.3084314920874,-66.5008277482104,
-55.0280211962633));
#132141=CARTESIAN_POINT('Ctrl Pts',(-23.3089371697075,-66.5006075758495,
-55.0275323543663));
#132142=CARTESIAN_POINT('Ctrl Pts',(-23.3094433520675,-66.5003871752661,
-55.0270440618914));
#132143=CARTESIAN_POINT('Ctrl Pts',(-23.3099500382032,-66.5001665468298,
-55.0265563196877));
#132144=CARTESIAN_POINT('Ctrl Pts',(-23.3737418241132,-66.4723894260756,
-54.9651495748562));
#132145=CARTESIAN_POINT('Ctrl Pts',(-23.4438814283319,-66.4417108192545,
-54.913708537172));
#132146=CARTESIAN_POINT('Ctrl Pts',(-23.5191429186309,-66.4085890914567,
-54.8723032868967));
#132147=CARTESIAN_POINT('Ctrl Pts',(-23.5545073851492,-66.3930255910651,
-54.8528474592054));
#132148=CARTESIAN_POINT('Ctrl Pts',(-23.5910022261981,-66.3769228800001,
-54.8356069181204));
#132149=CARTESIAN_POINT('Ctrl Pts',(-23.6284978920678,-66.3603295348338,
-54.8205860088576));
#132150=CARTESIAN_POINT('Ctrl Pts',(-23.6289267193329,-66.360139761465,
-54.8204142189909));
#132151=CARTESIAN_POINT('Ctrl Pts',(-23.6293556721512,-66.359949926291,
-54.8202427216662));
#132152=CARTESIAN_POINT('Ctrl Pts',(-23.629784750377,-66.3597600293637,
-54.8200715168436));
#132153=CARTESIAN_POINT('Ctrl Pts',(-23.6783390158401,-66.3382713933413,
-54.8006980695173));
#132154=CARTESIAN_POINT('Ctrl Pts',(-23.7276801213798,-66.316354158209,
-54.7853871133686));
#132155=CARTESIAN_POINT('Ctrl Pts',(-23.7776797138645,-66.29405966747,-54.7740684617323));
#132156=CARTESIAN_POINT('Ctrl Pts',(-23.8282083296012,-66.2715292887286,
-54.7626300525221));
#132157=CARTESIAN_POINT('Ctrl Pts',(-23.8794098794654,-66.2486134489514,
-54.75526886116));
#132158=CARTESIAN_POINT('Ctrl Pts',(-23.9311587890205,-66.2253609159866,
-54.7519649331453));
#132159=CARTESIAN_POINT('Ctrl Pts',(-23.9521926643966,-66.2159096853276,
-54.7506220176962));
#132160=CARTESIAN_POINT('Ctrl Pts',(-23.97331701039,-66.2064027967322,-54.7499500025558));
#132161=CARTESIAN_POINT('Ctrl Pts',(-23.9945234557419,-66.1968434349636,
-54.74995));
#132162=CARTESIAN_POINT('',(-24.2,-66.6526716808631,-55.24995));
#132163=CARTESIAN_POINT('Origin',(-24.2,-66.6526716808631,-54.74995));
#132164=CARTESIAN_POINT('Ctrl Pts',(-24.2,-66.6526716808631,-55.24995));
#132165=CARTESIAN_POINT('Ctrl Pts',(-24.1371955572435,-66.7092931820382,
-55.24995));
#132166=CARTESIAN_POINT('Ctrl Pts',(-24.0753940809144,-66.764472406879,
-55.2615406660682));
#132167=CARTESIAN_POINT('Ctrl Pts',(-23.9567432347527,-66.8694948932304,
-55.3084792096817));
#132168=CARTESIAN_POINT('Ctrl Pts',(-23.902316841733,-66.9171958169871,
-55.3428841126209));
#132169=CARTESIAN_POINT('Ctrl Pts',(-23.8072473920369,-66.9999887868491,
-55.4336221821879));
#132170=CARTESIAN_POINT('Ctrl Pts',(-23.7684105820677,-67.0335141101085,
-55.4886013829516));
#132171=CARTESIAN_POINT('Ctrl Pts',(-23.7144942998795,-67.079931038232,
-55.6126301527277));
#132172=CARTESIAN_POINT('Ctrl Pts',(-23.7,-67.0923340220896,-55.6800435061715));
#132173=CARTESIAN_POINT('Ctrl Pts',(-23.7,-67.0923340267327,-55.74995));
#132174=CARTESIAN_POINT('Origin',(0.,-12.9675000200281,-54.74995));
#132175=CARTESIAN_POINT('Origin',(0.,-12.9675000200281,-54.74995));
#132176=CARTESIAN_POINT('Origin',(0.,-12.9675000200281,-55.24995));
#132177=CARTESIAN_POINT('Origin',(-25.8159964412441,44.9247229809868,-55.24995));
#132178=CARTESIAN_POINT('',(-25.3802177275058,39.9437494905281,-60.1097730249189));
#132179=CARTESIAN_POINT('',(-25.3802177275058,39.9437494905281,-52.64995));
#132180=CARTESIAN_POINT('',(-25.3802177275058,39.9437494905281,-52.64995));
#132181=CARTESIAN_POINT('',(-23.7796330855957,40.3581899105085,-52.64995));
#132182=CARTESIAN_POINT('Origin',(-25.8159964412441,44.9247229809868,-52.64995));
#132183=CARTESIAN_POINT('',(-23.7796330855957,40.3581899105085,-60.5010370523947));
#132184=CARTESIAN_POINT('',(-23.7796330855957,40.3581899105085,-55.24995));
#132185=CARTESIAN_POINT('Ctrl Pts',(-25.3802177275058,39.9437494905281,
-60.1097730249189));
#132186=CARTESIAN_POINT('Ctrl Pts',(-25.2914736937722,39.9515135874353,
-60.1414728066845));
#132187=CARTESIAN_POINT('Ctrl Pts',(-25.2032163472256,39.9616205609225,
-60.1731437386284));
#132188=CARTESIAN_POINT('Ctrl Pts',(-25.115294687975,39.9740647365747,-60.2040070978231));
#132189=CARTESIAN_POINT('Ctrl Pts',(-25.0249019722788,39.9868586583613,
-60.235737878121));
#132190=CARTESIAN_POINT('Ctrl Pts',(-24.9348634969356,40.0021228222354,
-60.2666150537668));
#132191=CARTESIAN_POINT('Ctrl Pts',(-24.8450231973729,40.0199079019358,
-60.2957923806914));
#132192=CARTESIAN_POINT('Ctrl Pts',(-24.7551828978101,40.0376929816362,
-60.324969707616));
#132193=CARTESIAN_POINT('Ctrl Pts',(-24.6655401952566,40.0579990530801,
-60.3524471858193));
#132194=CARTESIAN_POINT('Ctrl Pts',(-24.5759556726477,40.0809332567916,
-60.3773785712321));
#132195=CARTESIAN_POINT('Ctrl Pts',(-24.4871224941809,40.1036751116563,
-60.402100857463));
#132196=CARTESIAN_POINT('Ctrl Pts',(-24.3980209679472,40.1290938411118,
-60.4240895083655));
#132197=CARTESIAN_POINT('Ctrl Pts',(-24.3090165921686,40.157227649633,-60.442417337988));
#132198=CARTESIAN_POINT('Ctrl Pts',(-24.2201098694864,40.1853305905312,
-60.4607250588316));
#132199=CARTESIAN_POINT('Ctrl Pts',(-24.1313005324118,40.2161427128992,
-60.4753799870885));
#132200=CARTESIAN_POINT('Ctrl Pts',(-24.0429505749462,40.2496498953545,
-60.4854579853069));
#132201=CARTESIAN_POINT('Ctrl Pts',(-23.9546006174805,40.2831570778098,
-60.4955359835253));
#132202=CARTESIAN_POINT('Ctrl Pts',(-23.8667104997529,40.3193593025707,
-60.5010370517052));
#132203=CARTESIAN_POINT('Ctrl Pts',(-23.7796330855957,40.3581899105084,
-60.5010370523947));
#132204=CARTESIAN_POINT('Origin',(0.,-12.9675000200281,-60.5010370523947));
#132205=CARTESIAN_POINT('',(-22.3428990418278,40.7794755973209,-61.0754935261978));
#132206=CARTESIAN_POINT('',(-23.7057274034393,40.1924568448808,-61.0754935261973));
#132207=CARTESIAN_POINT('Origin',(0.,-12.9675000200281,-61.0754935261978));
#132208=CARTESIAN_POINT('Origin',(-23.372360414466,39.4448832964128,-60.5010370523947));
#132209=CARTESIAN_POINT('',(-22.3089577584378,40.9899884313956,-60.5010370523947));
#132210=CARTESIAN_POINT('Origin',(0.,-12.9675000200281,-60.5010370523947));
#132211=CARTESIAN_POINT('Ctrl Pts',(-22.3428990418278,40.7794755973209,
-61.0754935261978));
#132212=CARTESIAN_POINT('Ctrl Pts',(-22.3211558478618,40.913825471773,-60.9106181484486));
#132213=CARTESIAN_POINT('Ctrl Pts',(-22.3089577682091,40.9899884273556,
-60.7079658702078));
#132214=CARTESIAN_POINT('Ctrl Pts',(-22.3089577584378,40.9899884313956,
-60.5010370523947));
#132215=CARTESIAN_POINT('Origin',(-22.5,41.4520521304013,-55.24995));
#132216=CARTESIAN_POINT('',(-22.,41.4520521304013,-55.74995));
#132217=CARTESIAN_POINT('',(-22.3089577584378,40.9899884313956,-55.74995));
#132218=CARTESIAN_POINT('Origin',(-22.5,41.4520521304013,-55.74995));
#132219=CARTESIAN_POINT('',(-22.,41.4520521304013,-60.5010370523947));
#132220=CARTESIAN_POINT('',(-22.,41.4520521304013,-92.34995));
#132221=CARTESIAN_POINT('Origin',(-22.5,41.4520521304013,-60.5010370523947));
#132222=CARTESIAN_POINT('',(-22.3089577584378,40.9899884313956,-55.24995));
#132223=CARTESIAN_POINT('Ctrl Pts',(-21.3174485247294,41.3893444859658,
-54.74995));
#132224=CARTESIAN_POINT('Ctrl Pts',(-21.3174485247294,41.3893444859657,
-55.2499499999999));
#132225=CARTESIAN_POINT('Ctrl Pts',(-21.5,41.8548280612684,-55.24995));
#132226=CARTESIAN_POINT('Ctrl Pts',(-21.5685182080957,41.2908809879478,
-54.7499500358909));
#132227=CARTESIAN_POINT('Ctrl Pts',(-21.4527403558093,41.3362862814715,
-55.2057014819632));
#132228=CARTESIAN_POINT('Ctrl Pts',(-21.6265769007959,41.7555472214248,
-55.24995));
#132229=CARTESIAN_POINT('Ctrl Pts',(-21.8184932751815,41.1905485577301,
-54.8481958669544));
#132230=CARTESIAN_POINT('Ctrl Pts',(-21.6281820015964,41.2670053764725,
-55.2194033701588));
#132231=CARTESIAN_POINT('Ctrl Pts',(-21.7526677202179,41.6543297475467,
-55.2990729306864));
#132232=CARTESIAN_POINT('Ctrl Pts',(-22.1923090650992,41.0384468090859,
-55.2114532855809));
#132233=CARTESIAN_POINT('Ctrl Pts',(-21.9027572404762,41.1571860364011,
-55.4056848867362));
#132234=CARTESIAN_POINT('Ctrl Pts',(-21.9411761916919,41.5009254814558,
-55.4807016455813));
#132235=CARTESIAN_POINT('Ctrl Pts',(-22.3089577352982,40.9899884409628,
-55.4723235737238));
#132236=CARTESIAN_POINT('Ctrl Pts',(-21.9999999817668,41.117728364782,-55.5719557452777));
#132237=CARTESIAN_POINT('Ctrl Pts',(-22.,41.4520521400528,-55.6111367847502));
#132238=CARTESIAN_POINT('Ctrl Pts',(-22.3089577584378,40.9899884313956,
-55.74995));
#132239=CARTESIAN_POINT('Ctrl Pts',(-22.,41.1177283573993,-55.74995));
#132240=CARTESIAN_POINT('Ctrl Pts',(-22.,41.4520521304013,-55.74995));
#132241=CARTESIAN_POINT('',(-21.5,41.8548280612684,-55.24995));
#132242=CARTESIAN_POINT('',(-21.3174485247294,41.3893444859658,-54.74995));
#132243=CARTESIAN_POINT('Origin',(-21.5,41.8548280612684,-54.74995));
#132244=CARTESIAN_POINT('Ctrl Pts',(-21.5,41.8548280612684,-55.24995));
#132245=CARTESIAN_POINT('Ctrl Pts',(-21.6265769007959,41.7555472214248,
-55.24995));
#132246=CARTESIAN_POINT('Ctrl Pts',(-21.7526677202179,41.6543297475467,
-55.2990729306864));
#132247=CARTESIAN_POINT('Ctrl Pts',(-21.9411761916919,41.5009254814558,
-55.4807016455813));
#132248=CARTESIAN_POINT('Ctrl Pts',(-22.,41.4520521400528,-55.6111367847502));
#132249=CARTESIAN_POINT('Ctrl Pts',(-22.,41.4520521304013,-55.74995));
#132250=CARTESIAN_POINT('Ctrl Pts',(-22.3089577584378,40.9899884313956,
-55.74995));
#132251=CARTESIAN_POINT('Ctrl Pts',(-22.3089577352982,40.9899884409628,
-55.4723235737238));
#132252=CARTESIAN_POINT('Ctrl Pts',(-22.1923090650992,41.0384468090859,
-55.2114532855809));
#132253=CARTESIAN_POINT('Ctrl Pts',(-21.8184932751815,41.1905485577301,
-54.8481958669544));
#132254=CARTESIAN_POINT('Ctrl Pts',(-21.5685182080957,41.2908809879478,
-54.7499500358909));
#132255=CARTESIAN_POINT('Ctrl Pts',(-21.3174485247294,41.3893444859658,
-54.74995));
#132256=CARTESIAN_POINT('Origin',(0.,-12.9675000200281,-54.74995));
#132257=CARTESIAN_POINT('',(-21.,42.0482945870964,-55.24995));
#132258=CARTESIAN_POINT('',(-20.8216939078753,41.5811683327377,-54.74995));
#132259=CARTESIAN_POINT('Origin',(-21.,42.0482945870964,-54.74995));
#132260=CARTESIAN_POINT('Origin',(0.,-12.9675000200281,-55.24995));
#132261=CARTESIAN_POINT('Origin',(0.,-12.9675000200281,-54.74995));
#132262=CARTESIAN_POINT('Ctrl Pts',(-19.8301846741669,41.9493820112901,
-55.74995));
#132263=CARTESIAN_POINT('Ctrl Pts',(-20.5,41.7075153736088,-55.7499499999999));
#132264=CARTESIAN_POINT('Ctrl Pts',(-20.5,42.4196614549321,-55.74995));
#132265=CARTESIAN_POINT('Ctrl Pts',(-19.8301846986023,41.9493820024666,
-55.6149487156912));
#132266=CARTESIAN_POINT('Ctrl Pts',(-20.4999999995541,41.7075153734334,
-55.7174757167052));
#132267=CARTESIAN_POINT('Ctrl Pts',(-20.5,42.4196614460347,-55.6824493590803));
#132268=CARTESIAN_POINT('Ctrl Pts',(-19.8580536242861,41.939338788612,-55.4791792828035));
#132269=CARTESIAN_POINT('Ctrl Pts',(-20.4987004734351,41.7075927453749,
-55.6840485748926));
#132270=CARTESIAN_POINT('Ctrl Pts',(-20.514053798786,42.4095322277552,-55.614564639731));
#132271=CARTESIAN_POINT('Ctrl Pts',(-19.9624885940201,41.9014556000366,
-55.2332682431543));
#132272=CARTESIAN_POINT('Ctrl Pts',(-20.5049952302095,41.704035376344,-55.6029041515887));
#132273=CARTESIAN_POINT('Ctrl Pts',(-20.5667184545259,42.3713246265636,
-55.4916091232479));
#132274=CARTESIAN_POINT('Ctrl Pts',(-20.0393490386551,41.8734921844523,
-55.1219509819824));
#132275=CARTESIAN_POINT('Ctrl Pts',(-20.5131880407467,41.7002281457635,
-55.5554275272938));
#132276=CARTESIAN_POINT('Ctrl Pts',(-20.6054777681041,42.3431217478432,
-55.4359504896237));
#132277=CARTESIAN_POINT('Ctrl Pts',(-20.2250038078484,41.8052957533979,
-54.9407461359128));
#132278=CARTESIAN_POINT('Ctrl Pts',(-20.5562936263709,41.682844191329,-55.4545960701533));
#132279=CARTESIAN_POINT('Ctrl Pts',(-20.6991000803093,42.274341317199,-55.3453480693239));
#132280=CARTESIAN_POINT('Ctrl Pts',(-20.3351498160899,41.7645520870248,
-54.8693487992283));
#132281=CARTESIAN_POINT('Ctrl Pts',(-20.5906196334233,41.6694809696074,
-55.401758477076));
#132282=CARTESIAN_POINT('Ctrl Pts',(-20.7546446997872,42.233248744276,-55.3096493999238));
#132283=CARTESIAN_POINT('Ctrl Pts',(-20.569794123189,41.6767990021169,-54.774393519968));
#132284=CARTESIAN_POINT('Ctrl Pts',(-20.6877494411454,41.6322368154735,
-55.3113977742726));
#132285=CARTESIAN_POINT('Ctrl Pts',(-20.8729715384853,42.1447441871192,
-55.2621717596744));
#132286=CARTESIAN_POINT('Ctrl Pts',(-20.6965038706024,41.6289544421905,
-54.7499500128377));
#132287=CARTESIAN_POINT('Ctrl Pts',(-20.7498635250281,41.608586604298,-55.2730231656551));
#132288=CARTESIAN_POINT('Ctrl Pts',(-20.936865425116,42.0964926027484,-55.24995));
#132289=CARTESIAN_POINT('Ctrl Pts',(-20.8216939078753,41.5811683327377,
-54.74995));
#132290=CARTESIAN_POINT('Ctrl Pts',(-20.8216939078753,41.5811683327377,
-55.2499499999999));
#132291=CARTESIAN_POINT('Ctrl Pts',(-21.,42.0482945870964,-55.24995));
#132292=CARTESIAN_POINT('',(-20.5,42.4196614549321,-55.74995));
#132293=CARTESIAN_POINT('',(-19.8301846741669,41.9493820112901,-55.74995));
#132294=CARTESIAN_POINT('Origin',(-20.,42.4196614549321,-55.74995));
#132295=CARTESIAN_POINT('Ctrl Pts',(-20.5,42.4196614549321,-55.74995));
#132296=CARTESIAN_POINT('Ctrl Pts',(-20.5,42.4196614460347,-55.6824493590803));
#132297=CARTESIAN_POINT('Ctrl Pts',(-20.514053798786,42.4095322277552,-55.614564639731));
#132298=CARTESIAN_POINT('Ctrl Pts',(-20.5667184545259,42.3713246265636,
-55.4916091232479));
#132299=CARTESIAN_POINT('Ctrl Pts',(-20.6054777681041,42.3431217478432,
-55.4359504896237));
#132300=CARTESIAN_POINT('Ctrl Pts',(-20.6991000803093,42.274341317199,-55.3453480693239));
#132301=CARTESIAN_POINT('Ctrl Pts',(-20.7546446997872,42.233248744276,-55.3096493999238));
#132302=CARTESIAN_POINT('Ctrl Pts',(-20.8729715384853,42.1447441871192,
-55.2621717596744));
#132303=CARTESIAN_POINT('Ctrl Pts',(-20.936865425116,42.0964926027484,-55.24995));
#132304=CARTESIAN_POINT('Ctrl Pts',(-21.,42.0482945870964,-55.24995));
#132305=CARTESIAN_POINT('Ctrl Pts',(-20.8216939078753,41.5811683327377,
-54.74995));
#132306=CARTESIAN_POINT('Ctrl Pts',(-20.7819408740053,41.5963424062421,
-54.7499500040765));
#132307=CARTESIAN_POINT('Ctrl Pts',(-20.7422583702479,41.6114370651536,
-54.7524107511961));
#132308=CARTESIAN_POINT('Ctrl Pts',(-20.7028910580564,41.6263644244518,
-54.7572302478587));
#132309=CARTESIAN_POINT('Ctrl Pts',(-20.6627696815177,41.6415777110541,
-54.7621420599578));
#132310=CARTESIAN_POINT('Ctrl Pts',(-20.6229744854674,41.6566176734326,
-54.769503891898));
#132311=CARTESIAN_POINT('Ctrl Pts',(-20.5837549178886,41.6713937246249,
-54.7792610196498));
#132312=CARTESIAN_POINT('Ctrl Pts',(-20.5448758646519,41.6860414863519,
-54.7889334335166));
#132313=CARTESIAN_POINT('Ctrl Pts',(-20.5065612917295,41.7004303395792,
-54.8009599654575));
#132314=CARTESIAN_POINT('Ctrl Pts',(-20.4690629498571,41.7144677618963,
-54.8153366743301));
#132315=CARTESIAN_POINT('Ctrl Pts',(-20.4635146440737,41.716544758039,-54.8174638717741));
#132316=CARTESIAN_POINT('Ctrl Pts',(-20.4579842421572,41.7186140458698,
-54.8196426059304));
#132317=CARTESIAN_POINT('Ctrl Pts',(-20.452472600707,41.7206753085659,-54.8218729523577));
#132318=CARTESIAN_POINT('Ctrl Pts',(-20.4520370571492,41.7208381946492,
-54.8220491998562));
#132319=CARTESIAN_POINT('Ctrl Pts',(-20.4516016002718,41.7210010421259,
-54.8222257818663));
#132320=CARTESIAN_POINT('Ctrl Pts',(-20.451166230457,41.7211638508663,-54.8224026982642));
#132321=CARTESIAN_POINT('Ctrl Pts',(-20.3795793872674,41.7479341123136,
-54.851492648923));
#132322=CARTESIAN_POINT('Ctrl Pts',(-20.310713633462,41.7735197491881,-54.8894829736819));
#132323=CARTESIAN_POINT('Ctrl Pts',(-20.246890665183,41.797116806489,-54.9352464330119));
#132324=CARTESIAN_POINT('Ctrl Pts',(-20.2064337192093,41.8120748207916,
-54.9642555789606));
#132325=CARTESIAN_POINT('Ctrl Pts',(-20.1680024696344,41.8262340118398,
-54.9963875370302));
#132326=CARTESIAN_POINT('Ctrl Pts',(-20.1321785809257,41.8393931763607,
-55.0313510893754));
#132327=CARTESIAN_POINT('Ctrl Pts',(-20.1316789419887,41.8395767083895,
-55.0318387291252));
#132328=CARTESIAN_POINT('Ctrl Pts',(-20.1311797709301,41.8397600607401,
-55.0323269633832));
#132329=CARTESIAN_POINT('Ctrl Pts',(-20.1306810690887,41.839943232968,-55.0328157906737));
#132330=CARTESIAN_POINT('Ctrl Pts',(-20.0684907293798,41.8627856252243,
-55.0937747299283));
#132331=CARTESIAN_POINT('Ctrl Pts',(-20.0135863047507,41.8828310295763,
-55.16397742118));
#132332=CARTESIAN_POINT('Ctrl Pts',(-19.9685212499155,41.8992323516681,
-55.2406426510445));
#132333=CARTESIAN_POINT('Ctrl Pts',(-19.9467038340028,41.907172749542,-55.2777587094209));
#132334=CARTESIAN_POINT('Ctrl Pts',(-19.9271921606261,41.9142591786561,
-55.3163901520212));
#132335=CARTESIAN_POINT('Ctrl Pts',(-19.9102738131902,41.9203962134609,
-55.3562250735781));
#132336=CARTESIAN_POINT('Ctrl Pts',(-19.9100688061412,41.9204705786079,
-55.356707770824));
#132337=CARTESIAN_POINT('Ctrl Pts',(-19.9098641753246,41.9205448062603,
-55.3571906629275));
#132338=CARTESIAN_POINT('Ctrl Pts',(-19.9096599209391,41.9206188963538,
-55.3576737490625));
#132339=CARTESIAN_POINT('Ctrl Pts',(-19.8950560556066,41.9259162207946,
-55.3922136432421));
#132340=CARTESIAN_POINT('Ctrl Pts',(-19.8824223932141,41.9304937150683,
-55.4276284386808));
#132341=CARTESIAN_POINT('Ctrl Pts',(-19.8717730238587,41.934349206398,-55.4637108040148));
#132342=CARTESIAN_POINT('Ctrl Pts',(-19.8611060292098,41.9382110787784,
-55.499852887653));
#132343=CARTESIAN_POINT('Ctrl Pts',(-19.8524296011668,41.9413486539406,
-55.5366659074258));
#132344=CARTESIAN_POINT('Ctrl Pts',(-19.8458033807232,41.9437431691666,
-55.5739608322423));
#132345=CARTESIAN_POINT('Ctrl Pts',(-19.8393763220395,41.9460657133694,
-55.6101347978453));
#132346=CARTESIAN_POINT('Ctrl Pts',(-19.8348780094478,41.9476892093277,
-55.6467631869939));
#132347=CARTESIAN_POINT('Ctrl Pts',(-19.832407933269,41.9485802658015,-55.6836754313748));
#132348=CARTESIAN_POINT('Ctrl Pts',(-19.8309355210528,41.9491114244956,
-55.7056788173518));
#132349=CARTESIAN_POINT('Ctrl Pts',(-19.8301846781792,41.9493820098413,
-55.7277830320761));
#132350=CARTESIAN_POINT('Ctrl Pts',(-19.8301846741669,41.9493820112901,
-55.74995));
#132351=CARTESIAN_POINT('Origin',(-20.,42.4196614549321,-55.24995));
#132352=CARTESIAN_POINT('',(-19.8301846741669,41.9493820112901,-60.42825533736));
#132353=CARTESIAN_POINT('',(-19.8301846741669,41.9493820112901,-55.24995));
#132354=CARTESIAN_POINT('',(-20.5,42.4196614549321,-60.42825533736));
#132355=CARTESIAN_POINT('Origin',(-20.,42.4196614549321,-60.42825533736));
#132356=CARTESIAN_POINT('',(-20.5,42.4196614549321,-92.34995));
#132357=CARTESIAN_POINT('Origin',(0.,-12.9675000200281,-60.42825533736));
#132358=CARTESIAN_POINT('',(-13.8920088064511,43.6468101642065,-60.8508735991007));
#132359=CARTESIAN_POINT('',(-19.8457268663587,41.8441333387867,-60.8508735991007));
#132360=CARTESIAN_POINT('Origin',(0.,-12.9675000200281,-60.8508735991007));
#132361=CARTESIAN_POINT('Origin',(-20.0201720011615,40.6653127489884,-60.3953656913166));
#132362=CARTESIAN_POINT('',(-13.8811292719168,43.7459411239336,-60.42825533736));
#132363=CARTESIAN_POINT('Origin',(0.,-12.9675000200281,-60.42825533736));
#132364=CARTESIAN_POINT('Origin',(-14.0020199016113,42.6566962185633,-60.4209701665496));
#132365=CARTESIAN_POINT('Origin',(-14.,44.2316053598056,-55.24995));
#132366=CARTESIAN_POINT('',(-13.5,44.2316053598049,-55.7692503840784));
#132367=CARTESIAN_POINT('',(-13.8811292719168,43.7459411239337,-55.7692503840715));
#132368=CARTESIAN_POINT('Origin',(-14.,44.2316053598044,-55.7692503840718));
#132369=CARTESIAN_POINT('',(-13.5,44.2316053598056,-60.42825533736));
#132370=CARTESIAN_POINT('',(-13.5,44.2316053598056,-92.34995));
#132371=CARTESIAN_POINT('Origin',(-14.,44.2316053598056,-60.42825533736));
#132372=CARTESIAN_POINT('',(-13.8811292719168,43.7459411239336,-55.24995));
#132373=CARTESIAN_POINT('Ctrl Pts',(-12.8921600942007,43.978899026433,-54.7926966592038));
#132374=CARTESIAN_POINT('Ctrl Pts',(-12.9056883239205,43.9758363551094,
-55.2210744412793));
#132375=CARTESIAN_POINT('Ctrl Pts',(-13.0012809038513,44.3884784473357,
-55.2865609247418));
#132376=CARTESIAN_POINT('Ctrl Pts',(-13.0193597758081,43.9501021457404,
-54.7884376491597));
#132377=CARTESIAN_POINT('Ctrl Pts',(-12.9784387965694,43.9593348061506,
-55.2098637836594));
#132378=CARTESIAN_POINT('Ctrl Pts',(-13.0654243459864,44.3636027691474,
-55.2827944545873));
#132379=CARTESIAN_POINT('Ctrl Pts',(-13.1474090807614,43.9206427834081,
-54.8097712354121));
#132380=CARTESIAN_POINT('Ctrl Pts',(-13.0552570243808,43.9418365181403,
-55.2141810151918));
#132381=CARTESIAN_POINT('Ctrl Pts',(-13.1299983077116,44.3395152672781,
-55.2921354075477));
#132382=CARTESIAN_POINT('Ctrl Pts',(-13.3859583749986,43.8649843137035,
-54.9019989045167));
#132383=CARTESIAN_POINT('Ctrl Pts',(-13.2011715416027,43.9084021006501,
-55.25643129776));
#132384=CARTESIAN_POINT('Ctrl Pts',(-13.2502943581078,44.2958064353142,
-55.3361304655099));
#132385=CARTESIAN_POINT('Ctrl Pts',(-13.496053992198,43.8388872267122,-54.9728361666051));
#132386=CARTESIAN_POINT('Ctrl Pts',(-13.2704159548698,43.8924342454859,
-55.2940831522118));
#132387=CARTESIAN_POINT('Ctrl Pts',(-13.3058135696287,44.2762488685004,
-55.3707576859229));
#132388=CARTESIAN_POINT('Ctrl Pts',(-13.6800589131788,43.7948562869374,
-55.1530004401584));
#132389=CARTESIAN_POINT('Ctrl Pts',(-13.3860573147077,43.8656515577332,
-55.3967868701307));
#132390=CARTESIAN_POINT('Ctrl Pts',(-13.3986038888631,44.2453125071312,
-55.4597899571993));
#132391=CARTESIAN_POINT('Ctrl Pts',(-13.7547890917519,43.7767382792428,
-55.2636104102621));
#132392=CARTESIAN_POINT('Ctrl Pts',(-13.4334072964209,43.8546223828157,
-55.46277372953));
#132393=CARTESIAN_POINT('Ctrl Pts',(-13.4362889542451,44.2338103823362,
-55.514828855807));
#132394=CARTESIAN_POINT('Ctrl Pts',(-13.8547672339164,43.7524103115038,
-55.5042410247415));
#132395=CARTESIAN_POINT('Ctrl Pts',(-13.4931806941864,43.8407149886408,
-55.6082533108594));
#132396=CARTESIAN_POINT('Ctrl Pts',(-13.4867061057231,44.2229131048268,
-55.6353022097904));
#132397=CARTESIAN_POINT('Ctrl Pts',(-13.8811292609786,43.7459411266109,
-55.6370500544614));
#132398=CARTESIAN_POINT('Ctrl Pts',(-13.5063795391638,43.8376645208725,
-55.6900657479953));
#132399=CARTESIAN_POINT('Ctrl Pts',(-13.5,44.2234307110675,-55.7021231738993));
#132400=CARTESIAN_POINT('Ctrl Pts',(-13.8811292719168,43.7459411239336,
-55.7692503840715));
#132401=CARTESIAN_POINT('Ctrl Pts',(-13.5,43.83922597116,-55.7692503840715));
#132402=CARTESIAN_POINT('Ctrl Pts',(-13.5,44.2316053598055,-55.7692503840715));
#132403=CARTESIAN_POINT('',(-13.0012809040741,44.3884784473346,-55.2865609247422));
#132404=CARTESIAN_POINT('',(-12.8921600942007,43.978899026433,-54.7926966592038));
#132405=CARTESIAN_POINT('Origin',(-13.0025618077027,44.4665581918916,-54.7926966592038));
#132406=CARTESIAN_POINT('Ctrl Pts',(-13.0012809038513,44.3884784473357,
-55.2865609247418));
#132407=CARTESIAN_POINT('Ctrl Pts',(-13.0654243459864,44.3636027691474,
-55.2827944545873));
#132408=CARTESIAN_POINT('Ctrl Pts',(-13.1299983077116,44.3395152672781,
-55.2921354075477));
#132409=CARTESIAN_POINT('Ctrl Pts',(-13.2502943581078,44.2958064353142,
-55.3361304655099));
#132410=CARTESIAN_POINT('Ctrl Pts',(-13.3058135696287,44.2762488685004,
-55.3707576859229));
#132411=CARTESIAN_POINT('Ctrl Pts',(-13.3986038888631,44.2453125071312,
-55.4597899571993));
#132412=CARTESIAN_POINT('Ctrl Pts',(-13.4362889542451,44.2338103823362,
-55.514828855807));
#132413=CARTESIAN_POINT('Ctrl Pts',(-13.4867061057231,44.2229131048268,
-55.6353022097904));
#132414=CARTESIAN_POINT('Ctrl Pts',(-13.5,44.2234307110675,-55.7021231738993));
#132415=CARTESIAN_POINT('Ctrl Pts',(-13.5,44.2316053598049,-55.7692503840784));
#132416=CARTESIAN_POINT('Ctrl Pts',(-13.8811292719168,43.7459411239336,
-55.7692503840715));
#132417=CARTESIAN_POINT('Ctrl Pts',(-13.8811292682097,43.745941124841,-55.7244458157437));
#132418=CARTESIAN_POINT('Ctrl Pts',(-13.878105549578,43.7466831296689,-55.6797361384662));
#132419=CARTESIAN_POINT('Ctrl Pts',(-13.8722047277525,43.7481272051964,
-55.6355346293342));
#132420=CARTESIAN_POINT('Ctrl Pts',(-13.8662038608383,43.7495957642058,
-55.5905837086734));
#132421=CARTESIAN_POINT('Ctrl Pts',(-13.8572273197946,43.7517904587082,
-55.546156909735));
#132422=CARTESIAN_POINT('Ctrl Pts',(-13.8453776205414,43.7546819864356,
-55.5026858819472));
#132423=CARTESIAN_POINT('Ctrl Pts',(-13.8344632356935,43.7573452815742,
-55.4626460871073));
#132424=CARTESIAN_POINT('Ctrl Pts',(-13.8211106222446,43.7605999346755,
-55.42341623202));
#132425=CARTESIAN_POINT('Ctrl Pts',(-13.8053642538662,43.7644316776827,
-55.3853473456883));
#132426=CARTESIAN_POINT('Ctrl Pts',(-13.8051683359555,43.7644793526174,
-55.3848736887475));
#132427=CARTESIAN_POINT('Ctrl Pts',(-13.8049720511568,43.7645271159922,
-55.3844002212373));
#132428=CARTESIAN_POINT('Ctrl Pts',(-13.8047753996222,43.7645749677634,
-55.3839269439647));
#132429=CARTESIAN_POINT('Ctrl Pts',(-13.7718577708347,43.7725849069894,
-55.3047047522731));
#132430=CARTESIAN_POINT('Ctrl Pts',(-13.728178051491,43.7831849346495,-55.2296008411733));
#132431=CARTESIAN_POINT('Ctrl Pts',(-13.6758172364543,43.7957998172914,
-55.1617614773858));
#132432=CARTESIAN_POINT('Ctrl Pts',(-13.6492141753641,43.8022090852399,
-55.1272941999399));
#132433=CARTESIAN_POINT('Ctrl Pts',(-13.6203708268823,43.8091382966092,
-55.0947027771972));
#132434=CARTESIAN_POINT('Ctrl Pts',(-13.5895638615798,43.8165110245856,
-55.0644031256242));
#132435=CARTESIAN_POINT('Ctrl Pts',(-13.5890610147607,43.8166313659687,
-55.0639085594356));
#132436=CARTESIAN_POINT('Ctrl Pts',(-13.5885576424949,43.8167518260625,
-55.0634146006456));
#132437=CARTESIAN_POINT('Ctrl Pts',(-13.5880537459902,43.8168724045334,
-55.0629212511039));
#132438=CARTESIAN_POINT('Ctrl Pts',(-13.5330913533195,43.8300244728725,
-55.0091092659349));
#132439=CARTESIAN_POINT('Ctrl Pts',(-13.4715943783259,43.8446517471105,
-54.9620890033323));
#132440=CARTESIAN_POINT('Ctrl Pts',(-13.4054646975513,43.8602521578836,
-54.9231113264506));
#132441=CARTESIAN_POINT('Ctrl Pts',(-13.3615129962604,43.8706206427498,
-54.8972056334056));
#132442=CARTESIAN_POINT('Ctrl Pts',(-13.3155161569051,43.881418679702,-54.8748524249685));
#132443=CARTESIAN_POINT('Ctrl Pts',(-13.2680436044718,43.8924962435662,
-54.8564136580933));
#132444=CARTESIAN_POINT('Ctrl Pts',(-13.2675902582944,43.8926020304046,
-54.8562375743555));
#132445=CARTESIAN_POINT('Ctrl Pts',(-13.267136793244,43.89270783907,-54.8560618534164));
#132446=CARTESIAN_POINT('Ctrl Pts',(-13.2666832096553,43.8928136694707,
-54.8558864954404));
#132447=CARTESIAN_POINT('Ctrl Pts',(-13.2297963270863,43.9014201395016,
-54.8416258184039));
#132448=CARTESIAN_POINT('Ctrl Pts',(-13.1921658567097,43.9101602729064,
-54.82976688078));
#132449=CARTESIAN_POINT('Ctrl Pts',(-13.1539812007031,43.9189886853961,
-54.8202850097806));
#132450=CARTESIAN_POINT('Ctrl Pts',(-13.1156262419326,43.9278564724202,
-54.8107608498357));
#132451=CARTESIAN_POINT('Ctrl Pts',(-13.0767111408946,43.9368135671448,
-54.8036348844097));
#132452=CARTESIAN_POINT('Ctrl Pts',(-13.037416426663,43.9458157565233,-54.7989332461647));
#132453=CARTESIAN_POINT('Ctrl Pts',(-12.9988139657374,43.9546593547151,
-54.7943144364803));
#132454=CARTESIAN_POINT('Ctrl Pts',(-12.9598441948041,43.9635466980804,
-54.7920353122774));
#132455=CARTESIAN_POINT('Ctrl Pts',(-12.9206817922385,43.9724341406896,
-54.7921703301218));
#132456=CARTESIAN_POINT('Ctrl Pts',(-12.9111849603394,43.9745893340114,
-54.7922030717742));
#132457=CARTESIAN_POINT('Ctrl Pts',(-12.9016768542622,43.976744516291,-54.7923780107907));
#132458=CARTESIAN_POINT('Ctrl Pts',(-12.8921600942007,43.978899026433,-54.7926966592038));
#132459=CARTESIAN_POINT('Ctrl Pts',(-13.0012809038513,44.3884784473357,
-55.2865609247418));
#132460=CARTESIAN_POINT('Ctrl Pts',(-12.9056883239205,43.9758363551094,
-55.2210744412794));
#132461=CARTESIAN_POINT('Ctrl Pts',(-12.8921600942007,43.978899026433,-54.7926966592038));
#132462=CARTESIAN_POINT('Ctrl Pts',(-12.8359967737338,44.4202801831072,
-55.2911600797832));
#132463=CARTESIAN_POINT('Ctrl Pts',(-12.743502264335,44.012594228669,-55.2216770608656));
#132464=CARTESIAN_POINT('Ctrl Pts',(-12.7296669706488,44.015686029617,-54.798137418056));
#132465=CARTESIAN_POINT('Ctrl Pts',(-12.6706421628547,44.4514812651211,
-55.2954855956284));
#132466=CARTESIAN_POINT('Ctrl Pts',(-12.5803648873612,44.0488388411796,
-55.2222478741758));
#132467=CARTESIAN_POINT('Ctrl Pts',(-12.5670134373343,44.0517782170206,
-54.8033818322122));
#132468=CARTESIAN_POINT('Ctrl Pts',(-12.5052115625551,44.4820814550629,
-55.2995670619066));
#132469=CARTESIAN_POINT('Ctrl Pts',(-12.4164090892806,44.0845209580867,
-55.2227904669344));
#132470=CARTESIAN_POINT('Ctrl Pts',(-12.4042000461459,44.0871753139748,
-54.8084491013774));
#132471=CARTESIAN_POINT('',(-12.5052115622199,44.4820814550383,-55.2995670618994));
#132472=CARTESIAN_POINT('',(-12.4042000461459,44.0871753139748,-54.8084491013776));
#132473=CARTESIAN_POINT('Origin',(-12.5104231251106,44.5757617009068,-54.8084491013774));
#132474=CARTESIAN_POINT('Origin',(-1.07162825033821,-13.9448070428209,-29.8942234462249));
#132475=CARTESIAN_POINT('Origin',(-0.360052490448792,-9.26137067391203,
-40.4793207392782));
#132476=CARTESIAN_POINT('Ctrl Pts',(-11.402356187646,44.2958078622741,-55.9012688372262));
#132477=CARTESIAN_POINT('Ctrl Pts',(-12.,44.1768041254343,-55.9012688372262));
#132478=CARTESIAN_POINT('Ctrl Pts',(-12.,44.7861808691872,-55.9012688372262));
#132479=CARTESIAN_POINT('Ctrl Pts',(-11.4023562275606,44.2958078543263,
-55.6244035357895));
#132480=CARTESIAN_POINT('Ctrl Pts',(-11.9474030636527,44.1872773054367,
-55.780904033187));
#132481=CARTESIAN_POINT('Ctrl Pts',(-12.,44.7411652565669,-55.7461428048454));
#132482=CARTESIAN_POINT('Ctrl Pts',(-11.5065640898974,44.2752649070124,
-55.34818818067));
#132483=CARTESIAN_POINT('Ctrl Pts',(-11.9557714038036,44.1846647896565,
-55.6127743620011));
#132484=CARTESIAN_POINT('Ctrl Pts',(-12.0525501385771,44.690888206552,-55.5962799769554));
#132485=CARTESIAN_POINT('Ctrl Pts',(-11.8731403310981,44.2003553912551,
-54.9432617778679));
#132486=CARTESIAN_POINT('Ctrl Pts',(-12.1135094933846,44.1501114029528,
-55.3471606562964));
#132487=CARTESIAN_POINT('Ctrl Pts',(-12.2374078497883,44.5869769557055,
-55.3765885853276));
#132488=CARTESIAN_POINT('Ctrl Pts',(-12.1323033844902,44.146288095939,-54.8169114178557));
#132489=CARTESIAN_POINT('Ctrl Pts',(-12.2536090925735,44.1199772025877,
-55.2458645392504));
#132490=CARTESIAN_POINT('Ctrl Pts',(-12.3680985162645,44.5329923862803,
-55.3078232766261));
#132491=CARTESIAN_POINT('Ctrl Pts',(-12.4042000461455,44.0871753139749,
-54.8084491013774));
#132492=CARTESIAN_POINT('Ctrl Pts',(-12.4164090892808,44.0845209580867,
-55.2227904669341));
#132493=CARTESIAN_POINT('Ctrl Pts',(-12.5052115625553,44.4820814550625,
-55.2995670619065));
#132494=CARTESIAN_POINT('',(-12.0000000086793,44.7861491811712,-55.9011596426166));
#132495=CARTESIAN_POINT('',(-11.402356187646,44.2958078622741,-55.9012688372262));
#132496=CARTESIAN_POINT('Origin',(-11.5,44.7861808691872,-55.9012688372262));
#132497=CARTESIAN_POINT('Ctrl Pts',(-12.0000000086793,44.7861491811712,
-55.9011596426166));
#132498=CARTESIAN_POINT('Ctrl Pts',(-12.0000246627355,44.7411416626413,
-55.74607247996));
#132499=CARTESIAN_POINT('Ctrl Pts',(-12.0525718259175,44.6908760157775,
-55.596254202959));
#132500=CARTESIAN_POINT('Ctrl Pts',(-12.2374078497883,44.5869769557055,
-55.3765885853276));
#132501=CARTESIAN_POINT('Ctrl Pts',(-12.3680985162645,44.5329923862803,
-55.3078232766261));
#132502=CARTESIAN_POINT('Ctrl Pts',(-12.5052115625557,44.4820814550628,
-55.2995670619079));
#132503=CARTESIAN_POINT('Ctrl Pts',(-12.4042000461459,44.0871753139748,
-54.8084491013776));
#132504=CARTESIAN_POINT('Ctrl Pts',(-12.1323033844902,44.146288095939,-54.8169114178557));
#132505=CARTESIAN_POINT('Ctrl Pts',(-11.8731403310981,44.2003553912551,
-54.9432617778679));
#132506=CARTESIAN_POINT('Ctrl Pts',(-11.5065640898974,44.2752649070124,
-55.34818818067));
#132507=CARTESIAN_POINT('Ctrl Pts',(-11.4023562275606,44.2958078543263,
-55.6244035357895));
#132508=CARTESIAN_POINT('Ctrl Pts',(-11.402356187646,44.2958078622741,-55.9012688372262));
#132509=CARTESIAN_POINT('Origin',(-11.5,44.7861808691872,-55.24995));
#132510=CARTESIAN_POINT('',(-12.,44.7861808691872,-60.42825533736));
#132511=CARTESIAN_POINT('',(-11.402356187646,44.2958078622741,-60.42825533736));
#132512=CARTESIAN_POINT('Origin',(-11.5,44.7861808691872,-60.42825533736));
#132513=CARTESIAN_POINT('',(-12.,44.7861808691872,-92.34995));
#132514=CARTESIAN_POINT('',(-11.402356187646,44.2958078622741,-55.24995));
#132515=CARTESIAN_POINT('Origin',(0.,-12.9675000200281,-60.42825533736));
#132516=CARTESIAN_POINT('',(-5.45757488824865,45.0702713246265,-60.8508735991007));
#132517=CARTESIAN_POINT('',(-11.4112929481563,44.1984900402045,-60.8508735991007));
#132518=CARTESIAN_POINT('Origin',(0.,-12.9675000200281,-60.8508735991007));
#132519=CARTESIAN_POINT('Origin',(-11.5321619114544,42.885355037367,-60.3485867710543));
#132520=CARTESIAN_POINT('',(-5.4533007853959,45.1647773033082,-60.42825533736));
#132521=CARTESIAN_POINT('Origin',(0.,-12.9675000200281,-60.42825533736));
#132522=CARTESIAN_POINT('Origin',(-5.49875184992484,44.1739762304382,-60.4281300090422));
#132523=CARTESIAN_POINT('Origin',(-5.5,45.6625917098448,-55.24995));
#132524=CARTESIAN_POINT('',(-4.9999999999978,45.6625933174098,-56.1488938878456));
#132525=CARTESIAN_POINT('',(-5.4533007853959,45.1647773033082,-56.1488993661993));
#132526=CARTESIAN_POINT('Origin',(-5.5,45.6625917098448,-56.1488993661993));
#132527=CARTESIAN_POINT('',(-5.,45.6625917098448,-60.42825533736));
#132528=CARTESIAN_POINT('',(-5.,45.6625917098448,-92.34995));
#132529=CARTESIAN_POINT('Origin',(-5.5,45.6625917098448,-60.42825533736));
#132530=CARTESIAN_POINT('',(-5.4533007853959,45.1647773033082,-55.24995));
#132531=CARTESIAN_POINT('Ctrl Pts',(-4.40504871546089,45.2535845867532,
-54.9609750843567));
#132532=CARTESIAN_POINT('Ctrl Pts',(-4.4367234185141,45.2509948349534,-55.2414357815079));
#132533=CARTESIAN_POINT('Ctrl Pts',(-4.47139039164496,45.4906548448225,
-55.3863604038317));
#132534=CARTESIAN_POINT('Ctrl Pts',(-4.5746726100032,45.2407903510215,-54.9401638606374));
#132535=CARTESIAN_POINT('Ctrl Pts',(-4.55013513142196,45.2423482358409,
-55.222182383583));
#132536=CARTESIAN_POINT('Ctrl Pts',(-4.55693219186133,45.4776416184102,
-55.3719745613437));
#132537=CARTESIAN_POINT('Ctrl Pts',(-4.75204967627729,45.2264957449184,
-54.9756360521501));
#132538=CARTESIAN_POINT('Ctrl Pts',(-4.67148999584465,45.2327453727894,
-55.2479506024288));
#132539=CARTESIAN_POINT('Ctrl Pts',(-4.64632152753943,45.4720450292502,
-55.3906024673539));
#132540=CARTESIAN_POINT('Ctrl Pts',(-5.02768780679811,45.2032674062285,
-55.1236362709704));
#132541=CARTESIAN_POINT('Ctrl Pts',(-4.85155529671713,45.2181899234016,
-55.3600111127249));
#132542=CARTESIAN_POINT('Ctrl Pts',(-4.78526231654569,45.4785391935409,
-55.4758941943565));
#132543=CARTESIAN_POINT('Ctrl Pts',(-5.13603339661033,45.1937280671781,
-55.2216356337625));
#132544=CARTESIAN_POINT('Ctrl Pts',(-4.91960725641842,45.2125663061104,
-55.4362681462788));
#132545=CARTESIAN_POINT('Ctrl Pts',(-4.83987531604392,45.4877168692796,
-55.5336384447089));
#132546=CARTESIAN_POINT('Ctrl Pts',(-5.30411094495532,45.178640871319,-55.4541550621106));
#132547=CARTESIAN_POINT('Ctrl Pts',(-5.01304731809969,45.2048811773774,
-55.6156547787452));
#132548=CARTESIAN_POINT('Ctrl Pts',(-4.92459268013903,45.5188916935313,
-55.6761597789111));
#132549=CARTESIAN_POINT('Ctrl Pts',(-5.3635004865346,45.1731436419376,-55.5870891782066));
#132550=CARTESIAN_POINT('Ctrl Pts',(-5.03798355387793,45.2028686588533,
-55.7195028114066));
#132551=CARTESIAN_POINT('Ctrl Pts',(-4.95452456181636,45.5407314582523,
-55.7600334675643));
#132552=CARTESIAN_POINT('Ctrl Pts',(-5.44607043400789,45.165473055749,-55.892595119653));
#132553=CARTESIAN_POINT('Ctrl Pts',(-5.04892271004842,45.2022954662183,
-55.9561269088792));
#132554=CARTESIAN_POINT('Ctrl Pts',(-4.99613220506375,45.6005437839053,
-55.9629949137758));
#132555=CARTESIAN_POINT('Ctrl Pts',(-5.45934494047939,45.1642043041266,
-56.0648075138966));
#132556=CARTESIAN_POINT('Ctrl Pts',(-5.0236821379186,45.2047138612132,-56.09030865871));
#132557=CARTESIAN_POINT('Ctrl Pts',(-5.00281283901273,45.6402645497959,
-56.0837699876347));
#132558=CARTESIAN_POINT('Ctrl Pts',(-5.45177805579373,45.1649222445519,
-56.2401344498719));
#132559=CARTESIAN_POINT('Ctrl Pts',(-4.97691572104394,45.208981116778,-56.2185887282704));
#132560=CARTESIAN_POINT('Ctrl Pts',(-4.99898645253332,45.6858523253614,
-56.2175969723113));
#132561=CARTESIAN_POINT('',(-4.51630724703443,45.4845441383223,-55.3818234144838));
#132562=CARTESIAN_POINT('',(-4.49412912371054,45.2467848220337,-54.955514051414));
#132563=CARTESIAN_POINT('Origin',(-4.53261449406992,45.7453014980519,-54.955514051414));
#132564=CARTESIAN_POINT('Ctrl Pts',(-4.51630724703492,45.4845441383302,
-55.3818234144886));
#132565=CARTESIAN_POINT('Ctrl Pts',(-4.58764035252675,45.4759709740095,
-55.3793081773896));
#132566=CARTESIAN_POINT('Ctrl Pts',(-4.6595628053899,45.4726639334208,-55.3987309043929));
#132567=CARTESIAN_POINT('Ctrl Pts',(-4.78526231654569,45.4785391935409,
-55.4758941943565));
#132568=CARTESIAN_POINT('Ctrl Pts',(-4.83987531604392,45.4877168692796,
-55.5336384447089));
#132569=CARTESIAN_POINT('Ctrl Pts',(-4.92459268013903,45.5188916935313,
-55.6761597789111));
#132570=CARTESIAN_POINT('Ctrl Pts',(-4.95452456181636,45.5407314582523,
-55.7600334675643));
#132571=CARTESIAN_POINT('Ctrl Pts',(-4.99216667017373,45.5948431999328,
-55.9436510953457));
#132572=CARTESIAN_POINT('Ctrl Pts',(-4.99999978324149,45.6266502446907,
-56.0420243862498));
#132573=CARTESIAN_POINT('Ctrl Pts',(-4.9999999999955,45.6625902180274,-56.1488949301565));
#132574=CARTESIAN_POINT('Ctrl Pts',(-5.4533007853959,45.1647773033082,-56.1488993661993));
#132575=CARTESIAN_POINT('Ctrl Pts',(-5.4533007853959,45.1647773033082,-56.0055674620926));
#132576=CARTESIAN_POINT('Ctrl Pts',(-5.43788134491899,45.1662336319389,
-55.8645506073504));
#132577=CARTESIAN_POINT('Ctrl Pts',(-5.3637535993023,45.1731199385278,-55.5890146236025));
#132578=CARTESIAN_POINT('Ctrl Pts',(-5.30482297007121,45.1785752810591,
-55.4563513172782));
#132579=CARTESIAN_POINT('Ctrl Pts',(-5.13740816361988,45.1936060305266,
-55.2236271337424));
#132580=CARTESIAN_POINT('Ctrl Pts',(-5.02927744515326,45.2031302456007,
-55.1252272506259));
#132581=CARTESIAN_POINT('Ctrl Pts',(-4.8419870330226,45.2189180089433,-55.0241597383142));
#132582=CARTESIAN_POINT('Ctrl Pts',(-4.77441476074195,45.2245089469405,
-54.9977644123794));
#132583=CARTESIAN_POINT('Ctrl Pts',(-4.63647895825164,45.2356614644569,
-54.9633053694043));
#132584=CARTESIAN_POINT('Ctrl Pts',(-4.56605684297844,45.2412320189915,
-54.9548634767888));
#132585=CARTESIAN_POINT('Ctrl Pts',(-4.49412912371054,45.2467848220337,
-54.955514051414));
#132586=CARTESIAN_POINT('Ctrl Pts',(-4.51630724703493,45.4845441383302,
-55.3818234144886));
#132587=CARTESIAN_POINT('Ctrl Pts',(-4.49662538953713,45.2465921108978,
-55.2355242600995));
#132588=CARTESIAN_POINT('Ctrl Pts',(-4.49412912371062,45.2467848220336,
-54.955514051414));
#132589=CARTESIAN_POINT('Ctrl Pts',(-4.34919298261046,45.4956321595243,
-55.3822130600194));
#132590=CARTESIAN_POINT('Ctrl Pts',(-4.33057507588361,45.2594183143523,
-55.2356268020846));
#132591=CARTESIAN_POINT('Ctrl Pts',(-4.32798628668273,45.2596110100493,
-54.9570167865889));
#132592=CARTESIAN_POINT('Ctrl Pts',(-4.18205130859575,45.5061051687682,
-55.3825645302384));
#132593=CARTESIAN_POINT('Ctrl Pts',(-4.16425328466829,45.2715506006274,
-55.2357229472724));
#132594=CARTESIAN_POINT('Ctrl Pts',(-4.16179087919831,45.271725776299,-54.9584347299645));
#132595=CARTESIAN_POINT('Ctrl Pts',(-4.01487932239355,45.5159631499936,
-55.3828830175977));
#132596=CARTESIAN_POINT('Ctrl Pts',(-3.99772850678838,45.2829791869159,
-55.2358129028006));
#132597=CARTESIAN_POINT('Ctrl Pts',(-3.9955429059226,45.2831291022416,-54.9597685279837));
#132598=CARTESIAN_POINT('',(-4.01487932206326,45.5159631499916,-55.3828830175848));
#132599=CARTESIAN_POINT('',(-3.99554290592262,45.2831291022416,-54.9597685279837));
#132600=CARTESIAN_POINT('Origin',(-4.02975864478749,45.7819570116602,-54.9597685279843));
#132601=CARTESIAN_POINT('Origin',(0.00205740951117972,-22.4761263385902,
-51.448280968311));
#132602=CARTESIAN_POINT('Origin',(-0.000537877419798383,-12.1619648117072,
-48.1393127415158));
#132603=CARTESIAN_POINT('Ctrl Pts',(-2.97452770112504,45.3441826962898,
-56.3263223051814));
#132604=CARTESIAN_POINT('Ctrl Pts',(-3.49999999999616,45.3173779148746,
-56.3263223051846));
#132605=CARTESIAN_POINT('Ctrl Pts',(-3.5,45.8435334367382,-56.3263223051844));
#132606=CARTESIAN_POINT('Ctrl Pts',(-2.97452768320356,45.344182697204,-56.1669325210571));
#132607=CARTESIAN_POINT('Ctrl Pts',(-3.46044927957153,45.3193954300817,
-56.2062114458595));
#132608=CARTESIAN_POINT('Ctrl Pts',(-3.50000000000048,45.8043701107064,
-56.199422183327));
#132609=CARTESIAN_POINT('Ctrl Pts',(-2.98977292660286,45.3434149603554,
-56.0100642332945));
#132610=CARTESIAN_POINT('Ctrl Pts',(-3.43677818882601,45.3204789931111,
-56.08184534982));
#132611=CARTESIAN_POINT('Ctrl Pts',(-3.50768789429957,45.7667515939358,
-56.0829442465191));
#132612=CARTESIAN_POINT('Ctrl Pts',(-3.06428488995232,45.339546776353,-55.7037165501142));
#132613=CARTESIAN_POINT('Ctrl Pts',(-3.43477708310906,45.3200587327755,
-55.8400245162723));
#132614=CARTESIAN_POINT('Ctrl Pts',(-3.54526290572092,45.6961797895947,
-55.8659417020081));
#132615=CARTESIAN_POINT('Ctrl Pts',(-3.12473312373466,45.3363910645469,
-55.5532476192867));
#132616=CARTESIAN_POINT('Ctrl Pts',(-3.45484122335623,45.3186462559097,
-55.719311149436));
#132617=CARTESIAN_POINT('Ctrl Pts',(-3.57574585639141,45.6630233017381,
-55.7649226433931));
#132618=CARTESIAN_POINT('Ctrl Pts',(-3.2545824170552,45.329238556454,-55.3542910788838));
#132619=CARTESIAN_POINT('Ctrl Pts',(-3.52210194558877,45.3142897117584,
-55.5588309593355));
#132620=CARTESIAN_POINT('Ctrl Pts',(-3.64122647661092,45.619502323306,-55.6349498078453));
#132621=CARTESIAN_POINT('Ctrl Pts',(-3.30516068386241,45.3264035474275,
-55.2914116693877));
#132622=CARTESIAN_POINT('Ctrl Pts',(-3.55052601940425,45.3124719950673,
-55.508240833463));
#132623=CARTESIAN_POINT('Ctrl Pts',(-3.66673217579536,45.6057722112868,
-55.5945395207919));
#132624=CARTESIAN_POINT('Ctrl Pts',(-3.4167612791713,45.3199688102369,-55.1805611737224));
#132625=CARTESIAN_POINT('Ctrl Pts',(-3.61713920495138,45.3082025597939,
-55.418990846134));
#132626=CARTESIAN_POINT('Ctrl Pts',(-3.72301031701685,45.5810344345382,
-55.523890140111));
#132627=CARTESIAN_POINT('Ctrl Pts',(-3.47812992567118,45.3163517222977,
-55.1317622002044));
#132628=CARTESIAN_POINT('Ctrl Pts',(-3.65544514044212,45.3057432608012,
-55.3793555355223));
#132629=CARTESIAN_POINT('Ctrl Pts',(-3.75395740734289,45.5698505794225,
-55.4931090773944));
#132630=CARTESIAN_POINT('Ctrl Pts',(-3.68134449873891,45.3039876967517,
-55.0081141730616));
#132631=CARTESIAN_POINT('Ctrl Pts',(-3.78526119814061,45.2973112081201,
-55.2791383019779));
#132632=CARTESIAN_POINT('Ctrl Pts',(-3.85643479923312,45.5394893320724,
-55.41516737719));
#132633=CARTESIAN_POINT('Ctrl Pts',(-3.83550338599139,45.2941065762735,
-54.9610525310383));
#132634=CARTESIAN_POINT('Ctrl Pts',(-3.88948584507314,45.2904098439472,
-55.2390222324507));
#132635=CARTESIAN_POINT('Ctrl Pts',(-3.93416970441329,45.5245403614258,
-55.3854368917654));
#132636=CARTESIAN_POINT('Ctrl Pts',(-3.99554290592259,45.2831291022416,
-54.9597685279837));
#132637=CARTESIAN_POINT('Ctrl Pts',(-3.99772850678843,45.282979186916,-55.2358129028005));
#132638=CARTESIAN_POINT('Ctrl Pts',(-4.01487932239363,45.5159631499936,
-55.3828830175977));
#132639=CARTESIAN_POINT('',(-3.50000000126666,45.8435334367292,-56.3263223051815));
#132640=CARTESIAN_POINT('',(-2.97452770112504,45.3441826962898,-56.3263223051814));
#132641=CARTESIAN_POINT('Origin',(-3.,45.8435334367418,-56.3263223051791));
#132642=CARTESIAN_POINT('Ctrl Pts',(-3.5,45.8435334367294,-56.3263223051813));
#132643=CARTESIAN_POINT('Ctrl Pts',(-3.50000000000048,45.8043701107064,
-56.199422183327));
#132644=CARTESIAN_POINT('Ctrl Pts',(-3.50768789429957,45.7667515939358,
-56.0829442465191));
#132645=CARTESIAN_POINT('Ctrl Pts',(-3.54526290572092,45.6961797895947,
-55.8659417020081));
#132646=CARTESIAN_POINT('Ctrl Pts',(-3.57574585639141,45.6630233017381,
-55.7649226433931));
#132647=CARTESIAN_POINT('Ctrl Pts',(-3.64122647661092,45.619502323306,-55.6349498078453));
#132648=CARTESIAN_POINT('Ctrl Pts',(-3.66673217579536,45.6057722112868,
-55.5945395207919));
#132649=CARTESIAN_POINT('Ctrl Pts',(-3.72301031701685,45.5810344345382,
-55.523890140111));
#132650=CARTESIAN_POINT('Ctrl Pts',(-3.75395740734289,45.5698505794225,
-55.4931090773944));
#132651=CARTESIAN_POINT('Ctrl Pts',(-3.85643479923312,45.5394893320724,
-55.41516737719));
#132652=CARTESIAN_POINT('Ctrl Pts',(-3.93416970441329,45.5245403614258,
-55.3854368917654));
#132653=CARTESIAN_POINT('Ctrl Pts',(-4.01487932239371,45.5159631499936,
-55.3828830175977));
#132654=CARTESIAN_POINT('Ctrl Pts',(-3.99554290592259,45.2831291022416,
-54.9597685279837));
#132655=CARTESIAN_POINT('Ctrl Pts',(-3.94364694050566,45.2866887643361,
-54.9601848912554));
#132656=CARTESIAN_POINT('Ctrl Pts',(-3.89225569969733,45.290140860166,-54.9654203274235));
#132657=CARTESIAN_POINT('Ctrl Pts',(-3.84188163699223,45.2934612214908,
-54.9751546343629));
#132658=CARTESIAN_POINT('Ctrl Pts',(-3.78940342464011,45.2969202759591,
-54.9852955481435));
#132659=CARTESIAN_POINT('Ctrl Pts',(-3.73803006364864,45.3002363143352,
-55.0003187158492));
#132660=CARTESIAN_POINT('Ctrl Pts',(-3.68833368154021,45.3033833815736,
-55.0198046066587));
#132661=CARTESIAN_POINT('Ctrl Pts',(-3.63901329263832,45.3065066387106,
-55.0391430709906));
#132662=CARTESIAN_POINT('Ctrl Pts',(-3.59134547691493,45.3094634363257,
-55.0628761864965));
#132663=CARTESIAN_POINT('Ctrl Pts',(-3.54586890420048,45.3122303325377,
-55.0905475013328));
#132664=CARTESIAN_POINT('Ctrl Pts',(-3.54528805073115,45.3122656729596,
-55.0909009356016));
#132665=CARTESIAN_POINT('Ctrl Pts',(-3.5447076792751,45.3123009754724,-55.0912549191843));
#132666=CARTESIAN_POINT('Ctrl Pts',(-3.54412778939157,45.3123362401396,
-55.0916094513196));
#132667=CARTESIAN_POINT('Ctrl Pts',(-3.4770118322515,45.3164177424284,-55.1326426961998));
#132668=CARTESIAN_POINT('Ctrl Pts',(-3.41622114944532,45.3199999518618,
-55.181103831794));
#132669=CARTESIAN_POINT('Ctrl Pts',(-3.3609625888742,45.3231860861595,-55.2359880590722));
#132670=CARTESIAN_POINT('Ctrl Pts',(-3.360382416735,45.3232195381049,-55.2365643010014));
#132671=CARTESIAN_POINT('Ctrl Pts',(-3.35980281684021,45.3232529482704,
-55.2371413403592));
#132672=CARTESIAN_POINT('Ctrl Pts',(-3.35922379149642,45.3232863165813,
-55.2377191725325));
#132673=CARTESIAN_POINT('Ctrl Pts',(-3.30734351853376,45.3262760943052,
-55.2894925382397));
#132674=CARTESIAN_POINT('Ctrl Pts',(-3.26003938774077,45.3289319621743,
-55.347682131924));
#132675=CARTESIAN_POINT('Ctrl Pts',(-3.21898968010271,45.3311986016842,
-55.4089811023588));
#132676=CARTESIAN_POINT('Ctrl Pts',(-3.21640175023372,45.3313414992693,
-55.4128456228549));
#132677=CARTESIAN_POINT('Ctrl Pts',(-3.21383866111004,45.3314828508093,
-55.4167225044125));
#132678=CARTESIAN_POINT('Ctrl Pts',(-3.21130082579067,45.3316226428383,
-55.4206109203385));
#132679=CARTESIAN_POINT('Ctrl Pts',(-3.2108528415918,45.3316473192307,-55.4212973119574));
#132680=CARTESIAN_POINT('Ctrl Pts',(-3.21040556228037,45.3316719521366,
-55.4219841720788));
#132681=CARTESIAN_POINT('Ctrl Pts',(-3.20995898742772,45.3316965416118,
-55.4226714985032));
#132682=CARTESIAN_POINT('Ctrl Pts',(-3.15429853624867,45.3347613386447,
-55.5083388813912));
#132683=CARTESIAN_POINT('Ctrl Pts',(-3.10954127961322,45.337153729465,-55.6013158854464));
#132684=CARTESIAN_POINT('Ctrl Pts',(-3.07484642277075,45.338981720226,-55.6975623037685));
#132685=CARTESIAN_POINT('Ctrl Pts',(-3.05597305038912,45.3399761140203,
-55.7499186083827));
#132686=CARTESIAN_POINT('Ctrl Pts',(-3.04007792774141,45.34080344662,-55.8032432879277));
#132687=CARTESIAN_POINT('Ctrl Pts',(-3.02702981215949,45.3414808214313,
-55.8568906140328));
#132688=CARTESIAN_POINT('Ctrl Pts',(-3.0269130014781,45.3414868854957,-55.8573708811394));
#132689=CARTESIAN_POINT('Ctrl Pts',(-3.0267964073689,45.3414929380841,-55.8578511838465));
#132690=CARTESIAN_POINT('Ctrl Pts',(-3.02668002962044,45.3414989792089,
-55.8583315221214));
#132691=CARTESIAN_POINT('Ctrl Pts',(-2.9936294563398,45.3432146219472,-55.9947446729532));
#132692=CARTESIAN_POINT('Ctrl Pts',(-2.97802127132001,45.3440061056746,
-56.1340253985183));
#132693=CARTESIAN_POINT('Ctrl Pts',(-2.97505677856548,45.3441559820078,
-56.2753845134639));
#132694=CARTESIAN_POINT('Ctrl Pts',(-2.9747013176472,45.3441739531022,-56.2923343409611));
#132695=CARTESIAN_POINT('Ctrl Pts',(-2.97452770112514,45.3441826962898,
-56.3093140568238));
#132696=CARTESIAN_POINT('Ctrl Pts',(-2.97452770112504,45.3441826962898,
-56.3263223051814));
#132697=CARTESIAN_POINT('Origin',(-3.,45.8435334367418,-55.24995));
#132698=CARTESIAN_POINT('',(-3.5,45.8435334367418,-60.42825533736));
#132699=CARTESIAN_POINT('',(-2.97452770112504,45.3441826962898,-60.42825533736));
#132700=CARTESIAN_POINT('Origin',(-3.,45.8435334367418,-60.42825533736));
#132701=CARTESIAN_POINT('',(-3.5,45.8435334367418,-92.34995));
#132702=CARTESIAN_POINT('',(-2.97452770112504,45.3441826962898,-55.24995));
#132703=CARTESIAN_POINT('Ctrl Pts',(-53.4093468596021,-38.0856478194539,
-55.3542488214713));
#132704=CARTESIAN_POINT('Ctrl Pts',(-52.9364447521332,-38.0597348185281,
-55.3342330819689));
#132705=CARTESIAN_POINT('Ctrl Pts',(-52.9112495105562,-38.347717747534,
-54.9585476429427));
#132706=CARTESIAN_POINT('Ctrl Pts',(-53.4247544927353,-37.9975926380036,
-55.2862331725394));
#132707=CARTESIAN_POINT('Ctrl Pts',(-52.9572784319432,-37.9516014512281,
-55.2598937783695));
#132708=CARTESIAN_POINT('Ctrl Pts',(-52.9283556128915,-38.1521941031454,
-54.8226237570584));
#132709=CARTESIAN_POINT('Ctrl Pts',(-53.4555105552472,-37.889347597856,
-55.24995));
#132710=CARTESIAN_POINT('Ctrl Pts',(-52.9868771633111,-37.8051184700684,
-55.2259980552998));
#132711=CARTESIAN_POINT('Ctrl Pts',(-52.9626456126999,-37.9110442829472,
-54.7499500131212));
#132712=CARTESIAN_POINT('Ctrl Pts',(-53.5055391860638,-37.78000002,-55.24995));
#132713=CARTESIAN_POINT('Ctrl Pts',(-53.0181298732915,-37.6685004154141,
-55.2499499999999));
#132714=CARTESIAN_POINT('Ctrl Pts',(-53.0181298732915,-37.6685004154142,
-54.74995));
#132715=CARTESIAN_POINT('',(-53.4093468596018,-38.0856478194539,-55.3542488214713));
#132716=CARTESIAN_POINT('Origin',(-53.4093468596021,-38.3912956189078,-54.9585476429427));
#132717=CARTESIAN_POINT('',(-53.5055391860638,-37.78000002,-55.24995));
#132718=CARTESIAN_POINT('Origin',(-53.5055391860638,-37.78000002,-54.74995));
#132719=CARTESIAN_POINT('Ctrl Pts',(-53.5055391860638,-37.78000002,-55.24995));
#132720=CARTESIAN_POINT('Ctrl Pts',(-53.4555105552472,-37.889347597856,
-55.24995));
#132721=CARTESIAN_POINT('Ctrl Pts',(-53.4247544927353,-37.9975926380036,
-55.2862331725394));
#132722=CARTESIAN_POINT('Ctrl Pts',(-53.4093468596018,-38.0856478194539,
-55.3542488214713));
#132723=CARTESIAN_POINT('Origin',(-57.8922230010149,-38.7834964612722,-54.74995));
#132724=CARTESIAN_POINT('',(-53.65082011387,-37.28000002,-55.24995));
#132725=CARTESIAN_POINT('Origin',(-53.65082011387,-37.28000002,-54.74995));
#132726=CARTESIAN_POINT('Origin',(-57.8922230010149,-38.7834964612722,-55.24995));
#132727=CARTESIAN_POINT('Ctrl Pts',(-53.65082011387,-37.28000002,-55.24995));
#132728=CARTESIAN_POINT('Ctrl Pts',(-53.1795531264094,-37.1129448598586,
-55.24995));
#132729=CARTESIAN_POINT('Ctrl Pts',(-53.1795531264094,-37.1129448598586,
-54.74995));
#132730=CARTESIAN_POINT('Ctrl Pts',(-53.6913582052585,-37.222820517008,
-55.24995));
#132731=CARTESIAN_POINT('Ctrl Pts',(-53.2071047405196,-37.0352210513017,
-55.2694186883497));
#132732=CARTESIAN_POINT('Ctrl Pts',(-53.2245914375472,-36.9858906030954,
-54.74995002559));
#132733=CARTESIAN_POINT('Ctrl Pts',(-53.7354566371443,-37.1679561903806,
-55.2594951814958));
#132734=CARTESIAN_POINT('Ctrl Pts',(-53.233451048998,-36.9645829953838,
-55.3049428618926));
#132735=CARTESIAN_POINT('Ctrl Pts',(-53.2735999108999,-36.8639446739783,
-54.7690447340998));
#132736=CARTESIAN_POINT('Ctrl Pts',(-53.7823432375838,-37.115384730595,
-55.2778252214784));
#132737=CARTESIAN_POINT('Ctrl Pts',(-53.2549772028919,-36.90570598919,-55.3509337052282));
#132738=CARTESIAN_POINT('Ctrl Pts',(-53.3256899305359,-36.7471331056253,
-54.8057004429567));
#132739=CARTESIAN_POINT('',(-53.7823432375799,-37.1153847305994,-55.2778252214768));
#132740=CARTESIAN_POINT('Origin',(-53.7823432375799,-36.9507694411988,-54.8057004429536));
#132741=CARTESIAN_POINT('Ctrl Pts',(-53.7823432375799,-37.1153847305994,
-55.2778252214768));
#132742=CARTESIAN_POINT('Ctrl Pts',(-53.7654128825011,-37.1343678403332,
-55.271206398986));
#132743=CARTESIAN_POINT('Ctrl Pts',(-53.7488460686483,-37.1536518315554,
-55.265762135374));
#132744=CARTESIAN_POINT('Ctrl Pts',(-53.7326791511753,-37.1732333135577,
-55.261482119382));
#132745=CARTESIAN_POINT('Ctrl Pts',(-53.7167419269871,-37.1925365894685,
-55.2572629121949));
#132746=CARTESIAN_POINT('Ctrl Pts',(-53.7011933167552,-37.2121301535344,
-55.2541749669534));
#132747=CARTESIAN_POINT('Ctrl Pts',(-53.6860681479851,-37.2320179858152,
-55.2522576006252));
#132748=CARTESIAN_POINT('Ctrl Pts',(-53.6740454267308,-37.247826461575,
-55.2507335210425));
#132749=CARTESIAN_POINT('Ctrl Pts',(-53.662290251486,-37.2638212423203,
-55.24995));
#132750=CARTESIAN_POINT('Ctrl Pts',(-53.65082011387,-37.28000002,-55.24995));
#132751=CARTESIAN_POINT('Origin',(-57.8922230010151,12.8484964212155,-55.24995));
#132752=CARTESIAN_POINT('',(-53.3256899305368,10.8121330655672,-54.7553968408231));
#132753=CARTESIAN_POINT('',(-53.3256899305368,10.8121330655672,-52.64995));
#132754=CARTESIAN_POINT('',(-53.3256899305368,10.8121330655672,-55.24995));
#132755=CARTESIAN_POINT('',(-52.9112495105564,12.4127177074772,-52.64995));
#132756=CARTESIAN_POINT('Origin',(-57.8922230010151,12.8484964212155,-52.64995));
#132757=CARTESIAN_POINT('',(-52.9112495105564,12.4127177074773,-55.2016711737242));
#132758=CARTESIAN_POINT('',(-52.9112495105564,12.4127177074773,-55.24995));
#132759=CARTESIAN_POINT('',(-53.0821517130856,11.4835003754205,-54.74995));
#132760=CARTESIAN_POINT('Ctrl Pts',(-53.0821517130856,11.4835003754205,
-54.74995));
#132761=CARTESIAN_POINT('Ctrl Pts',(-53.0315209792098,11.6619165987151,
-54.7499500147364));
#132762=CARTESIAN_POINT('Ctrl Pts',(-52.9911015935698,11.8455806632674,
-54.7902878065788));
#132763=CARTESIAN_POINT('Ctrl Pts',(-52.9359691402844,12.1685120566519,
-54.9455502016771));
#132764=CARTESIAN_POINT('Ctrl Pts',(-52.9201323460278,12.3111864334412,
-55.062291149986));
#132765=CARTESIAN_POINT('Ctrl Pts',(-52.9112495105564,12.4127177074773,
-55.2016711737242));
#132766=CARTESIAN_POINT('',(-53.275786978871,10.927944819865,-54.74995));
#132767=CARTESIAN_POINT('Origin',(-57.8922230010151,12.8484964212155,-54.74995));
#132768=CARTESIAN_POINT('Origin',(-53.6419198431625,11.0805921128927,-56.1036535412916));
#132769=CARTESIAN_POINT('Origin',(0.,-12.9675000200281,-55.24995));
#132770=CARTESIAN_POINT('Origin',(0.,-12.9675000200281,-52.64995));
#132771=CARTESIAN_POINT('',(-53.7129480054761,9.92396941324122,-55.74995));
#132772=CARTESIAN_POINT('Ctrl Pts',(-53.7129480054761,9.92396941324122,
-55.74995));
#132773=CARTESIAN_POINT('Ctrl Pts',(-53.7129480039811,9.9239694167493,-55.6201514218302));
#132774=CARTESIAN_POINT('Ctrl Pts',(-53.702610379063,9.94826762670561,-55.4957569720976));
#132775=CARTESIAN_POINT('Ctrl Pts',(-53.6624100137865,10.0422483461928,
-55.2594857136242));
#132776=CARTESIAN_POINT('Ctrl Pts',(-53.633790842791,10.1090015716016,-55.1553271807471));
#132777=CARTESIAN_POINT('Ctrl Pts',(-53.5254458539065,10.3597364405483,
-54.885939939012));
#132778=CARTESIAN_POINT('Ctrl Pts',(-53.4285862862346,10.5813885818665,
-54.7797862992586));
#132779=CARTESIAN_POINT('Ctrl Pts',(-53.3256899305368,10.8121330655672,
-54.7553968408231));
#132780=CARTESIAN_POINT('',(-53.7129480054761,9.92396941324122,-60.42825533736));
#132781=CARTESIAN_POINT('',(-53.7129480054761,9.92396941324122,-55.24995));
#132782=CARTESIAN_POINT('',(-55.7689460407313,4.32194224278905,-60.42825533736));
#132783=CARTESIAN_POINT('Origin',(0.,-12.9675000200281,-60.42825533736));
#132784=CARTESIAN_POINT('',(-55.7689460407313,4.32194224278905,-55.74995));
#132785=CARTESIAN_POINT('',(-55.7689460407313,4.32194224278906,-55.24995));
#132786=CARTESIAN_POINT('',(-56.066723956657,3.33043300908072,-54.74995));
#132787=CARTESIAN_POINT('Ctrl Pts',(-56.0667239566569,3.33043300908083,
-54.74995));
#132788=CARTESIAN_POINT('Ctrl Pts',(-56.054810110711,3.37141798004119,-54.7499500048111));
#132789=CARTESIAN_POINT('Ctrl Pts',(-56.0428719096528,3.41230937921187,
-54.752573624799));
#132790=CARTESIAN_POINT('Ctrl Pts',(-56.0309991957517,3.45281789175014,
-54.7576881483825));
#132791=CARTESIAN_POINT('Ctrl Pts',(-56.0183308037643,3.4960411783501,-54.7631454338967));
#132792=CARTESIAN_POINT('Ctrl Pts',(-56.0057365602009,3.53882993079307,
-54.7714383768922));
#132793=CARTESIAN_POINT('Ctrl Pts',(-55.9933214348628,3.58084263808002,
-54.7824678791719));
#132794=CARTESIAN_POINT('Ctrl Pts',(-55.9809063095247,3.62285534536697,
-54.7934973814515));
#132795=CARTESIAN_POINT('Ctrl Pts',(-55.9686698102716,3.66409363256125,
-54.8072637702972));
#132796=CARTESIAN_POINT('Ctrl Pts',(-55.9567198801064,3.70420224798085,
-54.8237268632943));
#132797=CARTESIAN_POINT('Ctrl Pts',(-55.9565878111619,3.70464552274758,
-54.8239088110787));
#132798=CARTESIAN_POINT('Ctrl Pts',(-55.9564557655643,3.70508869905399,
-54.8240911044694));
#132799=CARTESIAN_POINT('Ctrl Pts',(-55.9563237434519,3.70553177648158,
-54.8242737432782));
#132800=CARTESIAN_POINT('Ctrl Pts',(-55.9343635745754,3.77923196927974,
-54.8546533441936));
#132801=CARTESIAN_POINT('Ctrl Pts',(-55.9131570003997,3.849848007421,-54.8944556864583));
#132802=CARTESIAN_POINT('Ctrl Pts',(-55.8935222184449,3.91485853316296,
-54.9422511775345));
#132803=CARTESIAN_POINT('Ctrl Pts',(-55.8818370634327,3.95354794017876,
-54.9706954823092));
#132804=CARTESIAN_POINT('Ctrl Pts',(-55.8707083955307,3.99025269895558,
-55.0019703122251));
#132805=CARTESIAN_POINT('Ctrl Pts',(-55.8603061323666,4.0244496930758,-55.0357720069019));
#132806=CARTESIAN_POINT('Ctrl Pts',(-55.8601552265094,4.02494578961079,
-55.0362623688193));
#132807=CARTESIAN_POINT('Ctrl Pts',(-55.8600044604701,4.02544140270094,
-55.0367533059883));
#132808=CARTESIAN_POINT('Ctrl Pts',(-55.859853834661,4.02593653113585,-55.0372448169564));
#132809=CARTESIAN_POINT('Ctrl Pts',(-55.8409688317124,4.08801421894894,
-55.0988689578539));
#132810=CARTESIAN_POINT('Ctrl Pts',(-55.8242867117939,4.14247853961694,
-55.1695258968662));
#132811=CARTESIAN_POINT('Ctrl Pts',(-55.8106050241011,4.1869905311095,-55.2464345690387));
#132812=CARTESIAN_POINT('Ctrl Pts',(-55.8040947258895,4.20817112995897,
-55.2830308137519));
#132813=CARTESIAN_POINT('Ctrl Pts',(-55.7982636966349,4.22709855295219,
-55.3210433783437));
#132814=CARTESIAN_POINT('Ctrl Pts',(-55.7931974644892,4.24352182478376,
-55.3601764970326));
#132815=CARTESIAN_POINT('Ctrl Pts',(-55.7931360049005,4.24372105914634,
-55.3606512295973));
#132816=CARTESIAN_POINT('Ctrl Pts',(-55.7930746570768,4.24391992824447,
-55.3611261391855));
#132817=CARTESIAN_POINT('Ctrl Pts',(-55.7930134210752,4.24411843191566,
-55.3616012250647));
#132818=CARTESIAN_POINT('Ctrl Pts',(-55.7885029443904,4.25873967037657,
-55.3965947538372));
#132819=CARTESIAN_POINT('Ctrl Pts',(-55.784613055677,4.27133328431392,-55.4324278680426));
#132820=CARTESIAN_POINT('Ctrl Pts',(-55.7813486835249,4.28189251196924,
-55.4689029452562));
#132821=CARTESIAN_POINT('Ctrl Pts',(-55.7780780325758,4.29247204957792,
-55.5054481797902));
#132822=CARTESIAN_POINT('Ctrl Pts',(-55.775435211876,4.30100963982809,-55.5426389688295));
#132823=CARTESIAN_POINT('Ctrl Pts',(-55.7734395025711,4.30745180750476,
-55.5802948673858));
#132824=CARTESIAN_POINT('Ctrl Pts',(-55.7714984886898,4.31371741785943,
-55.6169187492453));
#132825=CARTESIAN_POINT('Ctrl Pts',(-55.7701695736421,4.318000949421,-55.6539836247098));
#132826=CARTESIAN_POINT('Ctrl Pts',(-55.7694848260442,4.32020701122527,
-55.6913249513657));
#132827=CARTESIAN_POINT('Ctrl Pts',(-55.7691277073319,4.32135754604051,
-55.7107996987558));
#132828=CARTESIAN_POINT('Ctrl Pts',(-55.7689460418115,4.32194223930484,
-55.730349572429));
#132829=CARTESIAN_POINT('Ctrl Pts',(-55.7689460407313,4.32194224278905,
-55.74995));
#132830=CARTESIAN_POINT('',(-56.208463007634,2.83467839222654,-54.74995));
#132831=CARTESIAN_POINT('Origin',(0.,-12.9675000200281,-54.74995));
#132832=CARTESIAN_POINT('',(-56.4778207328943,1.8431691585182,-55.74995));
#132833=CARTESIAN_POINT('Ctrl Pts',(-56.4778207328943,1.8431691585182,-55.74995));
#132834=CARTESIAN_POINT('Ctrl Pts',(-56.4778207259178,1.84316918512194,
-55.479632471504));
#132835=CARTESIAN_POINT('Ctrl Pts',(-56.4486203895175,1.955305574271,-55.2191289705157));
#132836=CARTESIAN_POINT('Ctrl Pts',(-56.3494613434174,2.32547473937703,
-54.8529437484072));
#132837=CARTESIAN_POINT('Ctrl Pts',(-56.2799098403954,2.5805414908759,-54.7499500372609));
#132838=CARTESIAN_POINT('Ctrl Pts',(-56.208463007634,2.83467839222654,-54.74995));
#132839=CARTESIAN_POINT('',(-56.4778207328943,1.84316915851819,-60.42825533736));
#132840=CARTESIAN_POINT('',(-56.4778207328943,1.84316915851819,-55.24995));
#132841=CARTESIAN_POINT('',(-57.6567521511579,-3.75885801193397,-60.42825533736));
#132842=CARTESIAN_POINT('Origin',(0.,-12.9675000200281,-60.42825533736));
#132843=CARTESIAN_POINT('',(-57.6567521511579,-3.75885801193397,-55.9233081330105));
#132844=CARTESIAN_POINT('',(-57.6567521511579,-3.75885801193397,-55.24995));
#132845=CARTESIAN_POINT('',(-57.8012193907064,-4.71406478367238,-54.8923577774473));
#132846=CARTESIAN_POINT('Ctrl Pts',(-57.8012193907064,-4.71406478367238,
-54.8923577774473));
#132847=CARTESIAN_POINT('Ctrl Pts',(-57.7635403562534,-4.45018749203841,
-54.8876932766828));
#132848=CARTESIAN_POINT('Ctrl Pts',(-57.7251747303172,-4.19619393974228,
-55.0015199525886));
#132849=CARTESIAN_POINT('Ctrl Pts',(-57.6844132682985,-3.93331576897112,
-55.2955533951453));
#132850=CARTESIAN_POINT('Ctrl Pts',(-57.6739991030625,-3.86739163922285,
-55.4096956077557));
#132851=CARTESIAN_POINT('Ctrl Pts',(-57.6600305184041,-3.7792996685362,
-55.6597535514676));
#132852=CARTESIAN_POINT('Ctrl Pts',(-57.6567521506183,-3.75885800855547,
-55.7907772949108));
#132853=CARTESIAN_POINT('Ctrl Pts',(-57.6567521511579,-3.75885801193397,
-55.9233081330105));
#132854=CARTESIAN_POINT('',(-57.8697476022662,-5.20911947359366,-54.9007953984755));
#132855=CARTESIAN_POINT('Origin',(-1.16314418724182,-12.9460285170553,-46.7095980005158));
#132856=CARTESIAN_POINT('',(-57.9983536018174,-6.23763109620483,-56.1192785199305));
#132857=CARTESIAN_POINT('Ctrl Pts',(-57.9983536018174,-6.23763109620483,
-56.1192785199305));
#132858=CARTESIAN_POINT('Ctrl Pts',(-57.9983536018174,-6.23763109620483,
-56.0644455264786));
#132859=CARTESIAN_POINT('Ctrl Pts',(-57.9980221190057,-6.23475814249573,
-56.0098560074895));
#132860=CARTESIAN_POINT('Ctrl Pts',(-57.9973433490653,-6.22891039019456,
-55.9557040569574));
#132861=CARTESIAN_POINT('Ctrl Pts',(-57.9966909788379,-6.22329007722612,
-55.9036582632632));
#132862=CARTESIAN_POINT('Ctrl Pts',(-57.9957178277956,-6.21492191913586,
-55.8520157782166));
#132863=CARTESIAN_POINT('Ctrl Pts',(-57.9944044945626,-6.20366890587322,
-55.8009488806203));
#132864=CARTESIAN_POINT('Ctrl Pts',(-57.9933769792934,-6.19486486234419,
-55.7609955651094));
#132865=CARTESIAN_POINT('Ctrl Pts',(-57.9921411410287,-6.18429413978129,
-55.7213944424274));
#132866=CARTESIAN_POINT('Ctrl Pts',(-57.9906851268661,-6.17186945082616,
-55.682233037996));
#132867=CARTESIAN_POINT('Ctrl Pts',(-57.9906667712501,-6.17171281579784,
-55.6817393397059));
#132868=CARTESIAN_POINT('Ctrl Pts',(-57.9906483809946,-6.17155588913671,
-55.681245721757));
#132869=CARTESIAN_POINT('Ctrl Pts',(-57.9906299560812,-6.17139867071413,
-55.6807521844164));
#132870=CARTESIAN_POINT('Ctrl Pts',(-57.9875046150388,-6.14473036685058,
-55.5970355082689));
#132871=CARTESIAN_POINT('Ctrl Pts',(-57.9833865494891,-6.10971202599361,
-55.5161284707291));
#132872=CARTESIAN_POINT('Ctrl Pts',(-57.9782530724075,-6.06658854500577,
-55.4400802261805));
#132873=CARTESIAN_POINT('Ctrl Pts',(-57.9747553923278,-6.03720648329141,
-55.3882649700042));
#132874=CARTESIAN_POINT('Ctrl Pts',(-57.9707862300964,-6.00406098349662,
-55.3387057443247));
#132875=CARTESIAN_POINT('Ctrl Pts',(-57.9663371613776,-5.96722056379155,
-55.2920615727606));
#132876=CARTESIAN_POINT('Ctrl Pts',(-57.9662786111709,-5.96673574004027,
-55.2914477306162));
#132877=CARTESIAN_POINT('Ctrl Pts',(-57.9662199779913,-5.96625027756548,
-55.2908343949051));
#132878=CARTESIAN_POINT('Ctrl Pts',(-57.9661612618222,-5.96576417654625,
-55.290221567164));
#132879=CARTESIAN_POINT('Ctrl Pts',(-57.9589421887777,-5.90599871813408,
-55.2148752308619));
#132880=CARTESIAN_POINT('Ctrl Pts',(-57.9504117107847,-5.8361745051014,
-55.1470534422475));
#132881=CARTESIAN_POINT('Ctrl Pts',(-57.9407769623035,-5.75872949144323,
-55.0901422818152));
#132882=CARTESIAN_POINT('Ctrl Pts',(-57.9357443409803,-5.71827680833683,
-55.0604152660987));
#132883=CARTESIAN_POINT('Ctrl Pts',(-57.9304104809614,-5.67574542893252,
-55.0336657755841));
#132884=CARTESIAN_POINT('Ctrl Pts',(-57.9248052326105,-5.63148645921459,
-55.0103806480697));
#132885=CARTESIAN_POINT('Ctrl Pts',(-57.9247386150578,-5.63096044786508,
-55.0101039077518));
#132886=CARTESIAN_POINT('Ctrl Pts',(-57.9246719532792,-5.63043414597652,
-55.0098276317698));
#132887=CARTESIAN_POINT('Ctrl Pts',(-57.9246052474285,-5.62990755498803,
-55.0095518217287));
#132888=CARTESIAN_POINT('Ctrl Pts',(-57.9212703682263,-5.6035812685008,
-54.9957630286867));
#132889=CARTESIAN_POINT('Ctrl Pts',(-57.9178139721909,-5.57645251025529,
-54.9831217176361));
#132890=CARTESIAN_POINT('Ctrl Pts',(-57.9142675773717,-5.54877950578676,
-54.9717642717495));
#132891=CARTESIAN_POINT('Ctrl Pts',(-57.9135128174631,-5.54289001085238,
-54.9693471283529));
#132892=CARTESIAN_POINT('Ctrl Pts',(-57.9127539957424,-5.53697595914985,
-54.9669879747415));
#132893=CARTESIAN_POINT('Ctrl Pts',(-57.91199143806,-5.5310399789474,-54.9646878564231));
#132894=CARTESIAN_POINT('Ctrl Pts',(-57.9086784919242,-5.50525100176252,
-54.9546949493021));
#132895=CARTESIAN_POINT('Ctrl Pts',(-57.9052948080902,-5.47904671417076,
-54.9458177116981));
#132896=CARTESIAN_POINT('Ctrl Pts',(-57.9018664479803,-5.45263506176634,
-54.9381157197596));
#132897=CARTESIAN_POINT('Ctrl Pts',(-57.9006211279107,-5.44304127355402,
-54.9353180424943));
#132898=CARTESIAN_POINT('Ctrl Pts',(-57.8993701409321,-5.43342183598762,
-54.9326755439206));
#132899=CARTESIAN_POINT('Ctrl Pts',(-57.8981140995164,-5.42378169739181,
-54.9301886689189));
#132900=CARTESIAN_POINT('Ctrl Pts',(-57.8944762323974,-5.39586100721222,
-54.922985944005));
#132901=CARTESIAN_POINT('Ctrl Pts',(-57.8907870927058,-5.36769806592118,
-54.9170666561107));
#132902=CARTESIAN_POINT('Ctrl Pts',(-57.8870439982323,-5.33928354730618,
-54.9124555883765));
#132903=CARTESIAN_POINT('Ctrl Pts',(-57.883409887184,-5.31169634191705,
-54.9079787758579));
#132904=CARTESIAN_POINT('Ctrl Pts',(-57.8797247293364,-5.28387052582422,
-54.9047349097722));
#132905=CARTESIAN_POINT('Ctrl Pts',(-57.8759849933552,-5.25579526938797,
-54.9027947109811));
#132906=CARTESIAN_POINT('Ctrl Pts',(-57.8739226319616,-5.24031253871428,
-54.9017247447849));
#132907=CARTESIAN_POINT('Ctrl Pts',(-57.8718436840546,-5.22475414416997,
-54.9010521259367));
#132908=CARTESIAN_POINT('Ctrl Pts',(-57.8697476022663,-5.20911947359449,
-54.9007953984755));
#132909=CARTESIAN_POINT('',(-57.9983536018174,-6.23763109620483,-60.42825533736));
#132910=CARTESIAN_POINT('',(-57.9983536018174,-6.23763109620483,-55.24995));
#132911=CARTESIAN_POINT('',(-58.376606009879,-11.839658266657,-60.42825533736));
#132912=CARTESIAN_POINT('Origin',(0.,-12.9675000200281,-60.42825533736));
#132913=CARTESIAN_POINT('',(-58.376606009879,-11.839658266657,-56.2580153373943));
#132914=CARTESIAN_POINT('',(-58.376606009879,-11.839658266657,-55.24995));
#132915=CARTESIAN_POINT('',(-58.3873384184922,-12.8301367871357,-54.9623589764041));
#132916=CARTESIAN_POINT('Ctrl Pts',(-58.3873384184922,-12.8301367871357,
-54.9623589764041));
#132917=CARTESIAN_POINT('Ctrl Pts',(-58.3869791994405,-12.6774478623384,
-54.9623171132768));
#132918=CARTESIAN_POINT('Ctrl Pts',(-58.3859897562866,-12.527917508371,
-55.0050319539282));
#132919=CARTESIAN_POINT('Ctrl Pts',(-58.3840891453349,-12.3330632532853,
-55.1184352970832));
#132920=CARTESIAN_POINT('Ctrl Pts',(-58.3833791647681,-12.2716887773838,
-55.165249378439));
#132921=CARTESIAN_POINT('Ctrl Pts',(-58.3819811265814,-12.1628909733764,
-55.2698289416564));
#132922=CARTESIAN_POINT('Ctrl Pts',(-58.3812857230693,-12.1145902249729,
-55.3279498195379));
#132923=CARTESIAN_POINT('Ctrl Pts',(-58.3780124938151,-11.9012175869243,
-55.6452667274097));
#132924=CARTESIAN_POINT('Ctrl Pts',(-58.3766060091376,-11.8396582282804,
-55.955889104467));
#132925=CARTESIAN_POINT('Ctrl Pts',(-58.376606009879,-11.839658266657,-56.2580153373943));
#132926=CARTESIAN_POINT('',(-58.3863769436068,-13.3296376352283,-54.9622468511542));
#132927=CARTESIAN_POINT('Origin',(-0.783398267377109,-12.9675000260486,
-48.2446835017872));
#132928=CARTESIAN_POINT('',(-58.3718694303385,-14.3184313509278,-56.2531111209796));
#132929=CARTESIAN_POINT('Ctrl Pts',(-58.3718694303385,-14.3184313509278,
-56.2531111209796));
#132930=CARTESIAN_POINT('Ctrl Pts',(-58.3718694303385,-14.3184313509278,
-56.1315282681123));
#132931=CARTESIAN_POINT('Ctrl Pts',(-58.3720934589562,-14.3089057630787,
-56.0113829394871));
#132932=CARTESIAN_POINT('Ctrl Pts',(-58.372602521148,-14.2863749805017,
-55.8932001781189));
#132933=CARTESIAN_POINT('Ctrl Pts',(-58.3727280602367,-14.2808186968923,
-55.8640552987669));
#132934=CARTESIAN_POINT('Ctrl Pts',(-58.3728706983335,-14.274471486997,
-55.8350297744669));
#132935=CARTESIAN_POINT('Ctrl Pts',(-58.3730308041295,-14.2672811529287,
-55.8061314796515));
#132936=CARTESIAN_POINT('Ctrl Pts',(-58.3735850259137,-14.2423911122432,
-55.7060972215946));
#132937=CARTESIAN_POINT('Ctrl Pts',(-58.3743558983076,-14.2072301125135,
-55.6079785795892));
#132938=CARTESIAN_POINT('Ctrl Pts',(-58.3753143408088,-14.1603251811705,
-55.5154726363337));
#132939=CARTESIAN_POINT('Ctrl Pts',(-58.3757555226855,-14.138734313063,
-55.4728911089164));
#132940=CARTESIAN_POINT('Ctrl Pts',(-58.3762357928548,-14.114655053344,
-55.431498836353));
#132941=CARTESIAN_POINT('Ctrl Pts',(-58.3767484727564,-14.0879436829683,
-55.3916564088811));
#132942=CARTESIAN_POINT('Ctrl Pts',(-58.3783749205468,-14.0032033816892,
-55.2652585767906));
#132943=CARTESIAN_POINT('Ctrl Pts',(-58.3803191831255,-13.8924014500595,
-55.1564962213834));
#132944=CARTESIAN_POINT('Ctrl Pts',(-58.382091437956,-13.7622047346492,
-55.0806296262956));
#132945=CARTESIAN_POINT('Ctrl Pts',(-58.3829775653712,-13.6971063769441,
-55.0426963287517));
#132946=CARTESIAN_POINT('Ctrl Pts',(-58.3838281227637,-13.6263468744968,
-55.0125723550395));
#132947=CARTESIAN_POINT('Ctrl Pts',(-58.3845593996408,-13.5534863365101,
-54.9925162587396));
#132948=CARTESIAN_POINT('Ctrl Pts',(-58.385290676518,-13.4806257985234,
-54.9724601624396));
#132949=CARTESIAN_POINT('Ctrl Pts',(-58.3859030562338,-13.4060410952294,
-54.9621915864083));
#132950=CARTESIAN_POINT('Ctrl Pts',(-58.3863769436069,-13.3296376352283,
-54.9622468511542));
#132951=CARTESIAN_POINT('',(-58.3718694303385,-14.3184313509278,-60.42825533736));
#132952=CARTESIAN_POINT('',(-58.3718694303385,-14.3184313509278,-55.24995));
#132953=CARTESIAN_POINT('',(-57.9720322598041,-19.92045852138,-60.42825533736));
#132954=CARTESIAN_POINT('Origin',(0.,-12.9675000200281,-60.42825533736));
#132955=CARTESIAN_POINT('',(-57.9720322598041,-19.92045852138,-56.1088024963483));
#132956=CARTESIAN_POINT('',(-57.9720322598041,-19.92045852138,-55.24995));
#132957=CARTESIAN_POINT('',(-57.8394345625603,-20.9487258492221,-54.8970741880307));
#132958=CARTESIAN_POINT('Ctrl Pts',(-57.8394345625603,-20.948725849222,
-54.8970741880307));
#132959=CARTESIAN_POINT('Ctrl Pts',(-57.8483315717605,-20.8842497909763,
-54.8981689263727));
#132960=CARTESIAN_POINT('Ctrl Pts',(-57.8570330166385,-20.8203546606078,
-54.906184509473));
#132961=CARTESIAN_POINT('Ctrl Pts',(-57.8654251279101,-20.7580154570499,
-54.9205228428093));
#132962=CARTESIAN_POINT('Ctrl Pts',(-57.8742541462894,-20.6924307720817,
-54.9356076533483));
#132963=CARTESIAN_POINT('Ctrl Pts',(-57.8827409478708,-20.6285669203242,
-54.9576909614185));
#132964=CARTESIAN_POINT('Ctrl Pts',(-57.8907523071769,-20.5675574167388,
-54.9861327822154));
#132965=CARTESIAN_POINT('Ctrl Pts',(-57.8925393734151,-20.5539482375843,
-54.9924772009036));
#132966=CARTESIAN_POINT('Ctrl Pts',(-57.8943027736347,-20.5404811271335,
-54.9991382130806));
#132967=CARTESIAN_POINT('Ctrl Pts',(-57.8960410108923,-20.5271687639928,
-55.0061090485496));
#132968=CARTESIAN_POINT('Ctrl Pts',(-57.8961104580828,-20.5266368997638,
-55.0063875519222));
#132969=CARTESIAN_POINT('Ctrl Pts',(-57.8961798575478,-20.5261053444105,
-55.0066665020562));
#132970=CARTESIAN_POINT('Ctrl Pts',(-57.8962492093382,-20.5255740977204,
-55.0069458987164));
#132971=CARTESIAN_POINT('Ctrl Pts',(-57.9046540977694,-20.4611912009517,
-55.0408065639478));
#132972=CARTESIAN_POINT('Ctrl Pts',(-57.9123517927205,-20.4013952311835,
-55.0812026657775));
#132973=CARTESIAN_POINT('Ctrl Pts',(-57.9194238609353,-20.3458803213664,
-55.1276091020937));
#132974=CARTESIAN_POINT('Ctrl Pts',(-57.9194970031007,-20.3453061639072,
-55.1280890560674));
#132975=CARTESIAN_POINT('Ctrl Pts',(-57.9195700843622,-20.3447324149112,
-55.1285697353016));
#132976=CARTESIAN_POINT('Ctrl Pts',(-57.9196431043984,-20.3441590772921,
-55.1290511360631));
#132977=CARTESIAN_POINT('Ctrl Pts',(-57.9261585705979,-20.2930010380242,
-55.172005790074));
#132978=CARTESIAN_POINT('Ctrl Pts',(-57.9321919519937,-20.2450759632068,
-55.2207529417631));
#132979=CARTESIAN_POINT('Ctrl Pts',(-57.9375117382134,-20.2024766660004,
-55.2726481082449));
#132980=CARTESIAN_POINT('Ctrl Pts',(-57.9379542983796,-20.1989327732066,
-55.2769653368986));
#132981=CARTESIAN_POINT('Ctrl Pts',(-57.9383919237742,-20.1954257087619,
-55.2813043482872));
#132982=CARTESIAN_POINT('Ctrl Pts',(-57.938824483381,-20.1919566596153,
-55.2856636195628));
#132983=CARTESIAN_POINT('Ctrl Pts',(-57.938884960972,-20.1914716403672,
-55.2862731037146));
#132984=CARTESIAN_POINT('Ctrl Pts',(-57.9389453520762,-20.1909872680675,
-55.2868830674044));
#132985=CARTESIAN_POINT('Ctrl Pts',(-57.9390056567172,-20.1905035428318,
-55.2874935092313));
#132986=CARTESIAN_POINT('Ctrl Pts',(-57.9476291333812,-20.1213315320002,
-55.3747858097991));
#132987=CARTESIAN_POINT('Ctrl Pts',(-57.9544934737035,-20.0653204626856,
-55.4719393844644));
#132988=CARTESIAN_POINT('Ctrl Pts',(-57.9596779034765,-20.0227139410896,
-55.5751875387902));
#132989=CARTESIAN_POINT('Ctrl Pts',(-57.9612949610577,-20.0094246881199,
-55.607391313942));
#132990=CARTESIAN_POINT('Ctrl Pts',(-57.9627485647957,-19.9974396112336,
-55.6401883807122));
#132991=CARTESIAN_POINT('Ctrl Pts',(-57.964041058706,-19.9867663918423,
-55.6734654024398));
#132992=CARTESIAN_POINT('Ctrl Pts',(-57.9640600250566,-19.9866097705855,
-55.6739537170499));
#132993=CARTESIAN_POINT('Ctrl Pts',(-57.9640789558543,-19.9864534391018,
-55.6744420834267));
#132994=CARTESIAN_POINT('Ctrl Pts',(-57.964097851118,-19.9862973972617,
-55.6749305015429));
#132995=CARTESIAN_POINT('Ctrl Pts',(-57.9681300897667,-19.9529981564454,
-55.7791586525503));
#132996=CARTESIAN_POINT('Ctrl Pts',(-57.9705461679584,-19.9328724060777,
-55.8857647076465));
#132997=CARTESIAN_POINT('Ctrl Pts',(-57.9715251367094,-19.9246984926926,
-55.9945278474376));
#132998=CARTESIAN_POINT('Ctrl Pts',(-57.9718656735483,-19.9218551755562,
-56.0323613899052));
#132999=CARTESIAN_POINT('Ctrl Pts',(-57.9720322597889,-19.9204585215068,
-56.0704559927494));
#133000=CARTESIAN_POINT('Ctrl Pts',(-57.9720322598041,-19.92045852138,-56.1088024963483));
#133001=CARTESIAN_POINT('',(-57.7689991024637,-21.4435190710235,-54.8883584020537));
#133002=CARTESIAN_POINT('Origin',(-1.20679688010735,-12.992434491263,-46.5556728733189));
#133003=CARTESIAN_POINT('',(-57.6206785412152,-22.3992316056509,-55.9136064684106));
#133004=CARTESIAN_POINT('Ctrl Pts',(-57.6206785412152,-22.3992316056509,
-55.9136064684106));
#133005=CARTESIAN_POINT('Ctrl Pts',(-57.6206785412152,-22.3992316056506,
-55.8712576139305));
#133006=CARTESIAN_POINT('Ctrl Pts',(-57.6210388568449,-22.3970387396972,
-55.8289927265008));
#133007=CARTESIAN_POINT('Ctrl Pts',(-57.6217580713774,-22.3926459443346,
-55.7870504595468));
#133008=CARTESIAN_POINT('Ctrl Pts',(-57.6224751991257,-22.3882658945648,
-55.7452298870979));
#133009=CARTESIAN_POINT('Ctrl Pts',(-57.6235491311395,-22.3816988155788,
-55.7037286574054));
#133010=CARTESIAN_POINT('Ctrl Pts',(-57.6249866999782,-22.3728877575666,
-55.6627754268274));
#133011=CARTESIAN_POINT('Ctrl Pts',(-57.6263702144474,-22.3644080062531,
-55.6233620884627));
#133012=CARTESIAN_POINT('Ctrl Pts',(-57.6280905589435,-22.3538497499171,
-55.5844551760954));
#133013=CARTESIAN_POINT('Ctrl Pts',(-57.6301613121382,-22.3411160233781,
-55.5462695907392));
#133014=CARTESIAN_POINT('Ctrl Pts',(-57.6305151022056,-22.3389404546127,
-55.5397455487366));
#133015=CARTESIAN_POINT('Ctrl Pts',(-57.6308791385551,-22.3367012727077,
-55.533242612179));
#133016=CARTESIAN_POINT('Ctrl Pts',(-57.6312535111585,-22.3343978551758,
-55.5267619228708));
#133017=CARTESIAN_POINT('Ctrl Pts',(-57.631280295686,-22.3342330569249,
-55.5262982612688));
#133018=CARTESIAN_POINT('Ctrl Pts',(-57.6313071321696,-22.3340679357285,
-55.525834729741));
#133019=CARTESIAN_POINT('Ctrl Pts',(-57.6313340206222,-22.3339024914829,
-55.525371328865));
#133020=CARTESIAN_POINT('Ctrl Pts',(-57.6359864322557,-22.3052762724673,
-55.4451907525285));
#133021=CARTESIAN_POINT('Ctrl Pts',(-57.6422382498636,-22.2666955115369,
-55.3683025755968));
#133022=CARTESIAN_POINT('Ctrl Pts',(-57.6498495152227,-22.2192637924273,
-55.2978189119865));
#133023=CARTESIAN_POINT('Ctrl Pts',(-57.6538973328722,-22.194038689807,
-55.2603343408809));
#133024=CARTESIAN_POINT('Ctrl Pts',(-57.6583296672913,-22.1663100498317,
-55.2246619070075));
#133025=CARTESIAN_POINT('Ctrl Pts',(-57.6631104665852,-22.1362429894798,
-55.1912758544359));
#133026=CARTESIAN_POINT('Ctrl Pts',(-57.6631864482776,-22.1357651308643,
-55.1907452467652));
#133027=CARTESIAN_POINT('Ctrl Pts',(-57.663262518071,-22.1352866810589,
-55.1902152153126));
#133028=CARTESIAN_POINT('Ctrl Pts',(-57.6633386758179,-22.1348076407422,
-55.1896857620266));
#133029=CARTESIAN_POINT('Ctrl Pts',(-57.6719065247418,-22.0809149610439,
-55.1301215555107));
#133030=CARTESIAN_POINT('Ctrl Pts',(-57.68166029603,-22.0190502353757,-55.0773873317788));
#133031=CARTESIAN_POINT('Ctrl Pts',(-57.6921719467787,-21.9515533423688,
-55.0335672587637));
#133032=CARTESIAN_POINT('Ctrl Pts',(-57.6985643073566,-21.9105070321072,
-55.0069193312439));
#133033=CARTESIAN_POINT('Ctrl Pts',(-57.7052367391672,-21.8673790789986,
-54.983568141199));
#133034=CARTESIAN_POINT('Ctrl Pts',(-57.7120915003347,-21.8227047516213,
-54.9639818384176));
#133035=CARTESIAN_POINT('Ctrl Pts',(-57.7121639633474,-21.8222324906232,
-54.9637747878039));
#133036=CARTESIAN_POINT('Ctrl Pts',(-57.7122364434107,-21.8217600784835,
-54.9635681670512));
#133037=CARTESIAN_POINT('Ctrl Pts',(-57.7123089404443,-21.8212875156173,
-54.9633619764799));
#133038=CARTESIAN_POINT('Ctrl Pts',(-57.7175256896611,-21.7872827868695,
-54.9485248935223));
#133039=CARTESIAN_POINT('Ctrl Pts',(-57.7228431420999,-21.7524063113004,
-54.935873883604));
#133040=CARTESIAN_POINT('Ctrl Pts',(-57.7282261110468,-21.716879990905,
-54.9253981395351));
#133041=CARTESIAN_POINT('Ctrl Pts',(-57.7336334907216,-21.6811925654857,
-54.9148748899835));
#133042=CARTESIAN_POINT('Ctrl Pts',(-57.7391071704681,-21.6448481995525,
-54.9065464760172));
#133043=CARTESIAN_POINT('Ctrl Pts',(-57.7446130540745,-21.6080564477773,
-54.9004521188838));
#133044=CARTESIAN_POINT('Ctrl Pts',(-57.7499689591833,-21.5722668914813,
-54.8945237700776));
#133045=CARTESIAN_POINT('Ctrl Pts',(-57.7553555069844,-21.5360528976767,
-54.8907094534876));
#133046=CARTESIAN_POINT('Ctrl Pts',(-57.7607401663573,-21.4996096687902,
-54.8890935200766));
#133047=CARTESIAN_POINT('Ctrl Pts',(-57.7634952382929,-21.4809634165035,
-54.8882667244556));
#133048=CARTESIAN_POINT('Ctrl Pts',(-57.7662497818651,-21.4622572897839,
-54.8880162223889));
#133049=CARTESIAN_POINT('Ctrl Pts',(-57.7689991024637,-21.4435190710235,
-54.8883584020538));
#133050=CARTESIAN_POINT('',(-57.6206785412152,-22.3992316056509,-60.42825533736));
#133051=CARTESIAN_POINT('',(-57.6206785412152,-22.3992316056509,-55.24995));
#133052=CARTESIAN_POINT('',(-56.418846619879,-28.001258776103,-60.42825533736));
#133053=CARTESIAN_POINT('Origin',(0.,-12.9675000200281,-60.42825533736));
#133054=CARTESIAN_POINT('',(-56.418846619879,-28.0012587761031,-55.74995));
#133055=CARTESIAN_POINT('',(-56.418846619879,-28.0012587761031,-55.24995));
#133056=CARTESIAN_POINT('',(-56.1452664265556,-28.9927680098114,-54.74995));
#133057=CARTESIAN_POINT('Ctrl Pts',(-56.1452664265556,-28.9927680098114,
-54.74995));
#133058=CARTESIAN_POINT('Ctrl Pts',(-56.157135481805,-28.9511842266489,
-54.7499500043992));
#133059=CARTESIAN_POINT('Ctrl Pts',(-56.168934149989,-28.9096618081524,
-54.7526528441348));
#133060=CARTESIAN_POINT('Ctrl Pts',(-56.1805785937552,-28.8685154650404,
-54.7579280669059));
#133061=CARTESIAN_POINT('Ctrl Pts',(-56.192713707601,-28.825635309661,-54.7634255754322));
#133062=CARTESIAN_POINT('Ctrl Pts',(-56.204681702463,-28.7831622366754,
-54.7717167436039));
#133063=CARTESIAN_POINT('Ctrl Pts',(-56.2163892898623,-28.7414427179697,
-54.7827110993106));
#133064=CARTESIAN_POINT('Ctrl Pts',(-56.2280968772615,-28.6997231992639,
-54.7937054550174));
#133065=CARTESIAN_POINT('Ctrl Pts',(-56.239544464813,-28.6587557436148,
-54.8074032739245));
#133066=CARTESIAN_POINT('Ctrl Pts',(-56.2506343384323,-28.6188990877768,
-54.8237679977477));
#133067=CARTESIAN_POINT('Ctrl Pts',(-56.2507584702878,-28.618452961805,
-54.823951172381));
#133068=CARTESIAN_POINT('Ctrl Pts',(-56.2508825687622,-28.618006934334,
-54.8241346982876));
#133069=CARTESIAN_POINT('Ctrl Pts',(-56.2510066337442,-28.6175610058129,
-54.824318575259));
#133070=CARTESIAN_POINT('Ctrl Pts',(-56.2715808747846,-28.5436107200033,
-54.8548117012847));
#133071=CARTESIAN_POINT('Ctrl Pts',(-56.2911418613671,-28.472713004467,
-54.8948321838607));
#133072=CARTESIAN_POINT('Ctrl Pts',(-56.3090294712607,-28.4074824207921,
-54.9428936399892));
#133073=CARTESIAN_POINT('Ctrl Pts',(-56.3196152133156,-28.3688794918939,
-54.9713360188419));
#133074=CARTESIAN_POINT('Ctrl Pts',(-56.329615102025,-28.3322606012612,
-55.0025940679593));
#133075=CARTESIAN_POINT('Ctrl Pts',(-56.3388945722868,-28.2981593218029,
-55.0363576523063));
#133076=CARTESIAN_POINT('Ctrl Pts',(-56.339029993733,-28.2976616592801,
-55.036850386621));
#133077=CARTESIAN_POINT('Ctrl Pts',(-56.3391652743153,-28.297164488402,
-55.0373436962489));
#133078=CARTESIAN_POINT('Ctrl Pts',(-56.3393004137533,-28.2966678103585,
-55.037837579714));
#133079=CARTESIAN_POINT('Ctrl Pts',(-56.3561267590193,-28.2348259352618,
-55.0993314990908));
#133080=CARTESIAN_POINT('Ctrl Pts',(-56.3707655818803,-28.1806225233707,
-55.1697303039922));
#133081=CARTESIAN_POINT('Ctrl Pts',(-56.3826877315599,-28.1363072821442,
-55.2462670316835));
#133082=CARTESIAN_POINT('Ctrl Pts',(-56.388440528518,-28.1149238410887,
-55.2831983122062));
#133083=CARTESIAN_POINT('Ctrl Pts',(-56.3935608278346,-28.0958424992867,
-55.3215595430322));
#133084=CARTESIAN_POINT('Ctrl Pts',(-56.397989272594,-28.0793153399122,
-55.3610440111482));
#133085=CARTESIAN_POINT('Ctrl Pts',(-56.3980423761537,-28.0791171549869,
-55.3615174879381));
#133086=CARTESIAN_POINT('Ctrl Pts',(-56.3980953812291,-28.0789193343635,
-55.3619911356045));
#133087=CARTESIAN_POINT('Ctrl Pts',(-56.3981482877874,-28.0787218781893,
-55.3624649534454));
#133088=CARTESIAN_POINT('Ctrl Pts',(-56.4020846045284,-28.0640308820639,
-55.3977176169507));
#133089=CARTESIAN_POINT('Ctrl Pts',(-56.4054635861547,-28.051402110709,
-55.4337954284411));
#133090=CARTESIAN_POINT('Ctrl Pts',(-56.4082873243379,-28.0408381674741,
-55.4705044074017));
#133091=CARTESIAN_POINT('Ctrl Pts',(-56.4111187646799,-28.0302454095389,
-55.5073135154712));
#133092=CARTESIAN_POINT('Ctrl Pts',(-56.4133919882818,-28.0217284962733,
-55.5447583433606));
#133093=CARTESIAN_POINT('Ctrl Pts',(-56.4150963311521,-28.0153374570684,
-55.5826612239245));
#133094=CARTESIAN_POINT('Ctrl Pts',(-56.4167572958903,-28.0091090795837,
-55.6195994182216));
#133095=CARTESIAN_POINT('Ctrl Pts',(-56.4178779761682,-28.0048996781118,
-55.656973670175));
#133096=CARTESIAN_POINT('Ctrl Pts',(-56.4184359903581,-28.0028025535953,
-55.694620789627));
#133097=CARTESIAN_POINT('Ctrl Pts',(-56.4187084931304,-28.0017784358308,
-55.7130055271627));
#133098=CARTESIAN_POINT('Ctrl Pts',(-56.4188466190161,-28.0012587793416,
-55.7314552635407));
#133099=CARTESIAN_POINT('Ctrl Pts',(-56.418846619879,-28.0012587761031,
-55.74995));
#133100=CARTESIAN_POINT('',(-56.0013925566522,-29.4885226266656,-54.74995));
#133101=CARTESIAN_POINT('Origin',(0.,-12.9675000200281,-54.74995));
#133102=CARTESIAN_POINT('',(-55.6992942935022,-30.4800318603739,-55.74995));
#133103=CARTESIAN_POINT('Ctrl Pts',(-55.6992942935022,-30.4800318603739,
-55.74995));
#133104=CARTESIAN_POINT('Ctrl Pts',(-55.699294301712,-30.4800318342627,
-55.4780587856325));
#133105=CARTESIAN_POINT('Ctrl Pts',(-55.7350468385274,-30.3669899517508,
-55.2177384600888));
#133106=CARTESIAN_POINT('Ctrl Pts',(-55.8207323820705,-30.0892808127342,
-54.9437622390698));
#133107=CARTESIAN_POINT('Ctrl Pts',(-55.8541342694537,-29.9801791700519,
-54.8719723798496));
#133108=CARTESIAN_POINT('Ctrl Pts',(-55.9259713199402,-29.7425201026704,
-54.7747042862246));
#133109=CARTESIAN_POINT('Ctrl Pts',(-55.9637778607192,-29.6160253486821,
-54.7499500197391));
#133110=CARTESIAN_POINT('Ctrl Pts',(-56.0013925566522,-29.4885226266656,
-54.74995));
#133111=CARTESIAN_POINT('',(-55.6992942935022,-30.4800318603739,-60.42825533736));
#133112=CARTESIAN_POINT('',(-55.6992942935022,-30.4800318603739,-55.24995));
#133113=CARTESIAN_POINT('',(-53.6173229282256,-36.0820590308261,-60.42825533736));
#133114=CARTESIAN_POINT('Origin',(0.,-12.9675000200281,-60.42825533736));
#133115=CARTESIAN_POINT('',(-53.6173229282256,-36.0820590308261,-55.74995));
#133116=CARTESIAN_POINT('',(-53.6173229282256,-36.0820590308261,-55.24995));
#133117=CARTESIAN_POINT('Ctrl Pts',(-53.3256899305366,-36.7471331056238,
-54.8057004429536));
#133118=CARTESIAN_POINT('Ctrl Pts',(-53.4080974646291,-36.562334686105,
-54.8706857163843));
#133119=CARTESIAN_POINT('Ctrl Pts',(-53.481339980492,-36.3953483985127,
-54.9914263135601));
#133120=CARTESIAN_POINT('Ctrl Pts',(-53.587398316273,-36.1517305970246,
-55.3270423559178));
#133121=CARTESIAN_POINT('Ctrl Pts',(-53.6173229109667,-36.0820590708605,
-55.5352328299022));
#133122=CARTESIAN_POINT('Ctrl Pts',(-53.6173229282256,-36.0820590308261,
-55.74995));
#133123=CARTESIAN_POINT('Ctrl Pts',(-53.7823432375846,11.067884690566,-55.2526734204115));
#133124=CARTESIAN_POINT('Ctrl Pts',(-53.3054454943535,10.8575310968505,
-55.2747187747876));
#133125=CARTESIAN_POINT('Ctrl Pts',(-53.3256899305368,10.8121330655672,
-54.7553968408231));
#133126=CARTESIAN_POINT('Ctrl Pts',(-53.7669694165083,11.0851225427625,
-55.2508668691012));
#133127=CARTESIAN_POINT('Ctrl Pts',(-53.2957533879043,10.880281535778,-55.2650191833929));
#133128=CARTESIAN_POINT('Ctrl Pts',(-53.3086079255675,10.8504393631076,
-54.7517837407593));
#133129=CARTESIAN_POINT('Ctrl Pts',(-53.7519966717624,11.1024937011227,
-55.24995));
#133130=CARTESIAN_POINT('Ctrl Pts',(-53.2858304006402,10.9038034191885,
-55.2567197573796));
#133131=CARTESIAN_POINT('Ctrl Pts',(-53.2919715007789,10.8890420328302,
-54.7499500043796));
#133132=CARTESIAN_POINT('Ctrl Pts',(-53.7374305810854,11.11999998,-55.24995));
#133133=CARTESIAN_POINT('Ctrl Pts',(-53.275786978871,10.927944819865,-55.24995));
#133134=CARTESIAN_POINT('Ctrl Pts',(-53.275786978871,10.927944819865,-54.74995));
#133135=CARTESIAN_POINT('',(-53.7374305810854,11.11999998,-55.24995));
#133136=CARTESIAN_POINT('Origin',(-53.7374305810854,11.11999998,-54.74995));
#133137=CARTESIAN_POINT('',(-53.7823432375846,11.067884690566,-55.2526734204115));
#133138=CARTESIAN_POINT('Ctrl Pts',(-53.7374305810854,11.11999998,-55.24995));
#133139=CARTESIAN_POINT('Ctrl Pts',(-53.7521098206901,11.1023577124241,
-55.24995));
#133140=CARTESIAN_POINT('Ctrl Pts',(-53.7671137595184,11.084960698582,-55.2508838306004));
#133141=CARTESIAN_POINT('Ctrl Pts',(-53.7823432375846,11.067884690566,-55.2526734204115));
#133142=CARTESIAN_POINT('Origin',(-53.7823432375846,11.015769401132,-54.7553968408231));
#133143=CARTESIAN_POINT('Origin',(-57.8922230010151,12.8484964212155,-54.74995));
#133144=CARTESIAN_POINT('',(-53.5631588418786,11.61999998,-55.24995));
#133145=CARTESIAN_POINT('Origin',(-53.5631588418786,11.61999998,-54.74995));
#133146=CARTESIAN_POINT('Origin',(-57.8922230010151,12.8484964212155,-55.24995));
#133147=CARTESIAN_POINT('Ctrl Pts',(-53.5631588418786,11.61999998,-55.24995));
#133148=CARTESIAN_POINT('Ctrl Pts',(-53.0821517130855,11.4835003754205,
-55.24995));
#133149=CARTESIAN_POINT('Ctrl Pts',(-53.0821517130856,11.4835003754205,
-54.74995));
#133150=CARTESIAN_POINT('Ctrl Pts',(-53.5175339525391,11.7003881248737,
-55.24995));
#133151=CARTESIAN_POINT('Ctrl Pts',(-53.0531569518754,11.5856741846736,
-55.2284398184114));
#133152=CARTESIAN_POINT('Ctrl Pts',(-53.0315209792098,11.6619165987151,
-54.7499500147364));
#133153=CARTESIAN_POINT('Ctrl Pts',(-53.481213741953,11.782936109662,-55.2701189042654));
#133154=CARTESIAN_POINT('Ctrl Pts',(-53.0233020583897,11.6990374932301,
-55.2381992664208));
#133155=CARTESIAN_POINT('Ctrl Pts',(-52.9911015935698,11.8455806632674,
-54.7902878065788));
#133156=CARTESIAN_POINT('Ctrl Pts',(-53.4315945187188,11.9282552364233,
-55.3477500998626));
#133157=CARTESIAN_POINT('Ctrl Pts',(-52.976392393765,11.8900295415054,-55.3145394488894));
#133158=CARTESIAN_POINT('Ctrl Pts',(-52.9359691402844,12.1685120566519,
-54.9455502016771));
#133159=CARTESIAN_POINT('Ctrl Pts',(-53.4173436672944,11.9924457375215,
-55.4061007701193));
#133160=CARTESIAN_POINT('Ctrl Pts',(-52.9577221123402,11.9716892536029,
-55.3811617269574));
#133161=CARTESIAN_POINT('Ctrl Pts',(-52.9201323460278,12.3111864334412,
-55.062291149986));
#133162=CARTESIAN_POINT('Ctrl Pts',(-53.4093468596018,12.0381477794281,
-55.475810586866));
#133163=CARTESIAN_POINT('Ctrl Pts',(-52.9450883668935,12.0259378096739,
-55.4571865884944));
#133164=CARTESIAN_POINT('Ctrl Pts',(-52.9112495105559,12.4127177074828,
-55.2016711737319));
#133165=CARTESIAN_POINT('',(-53.4093468596018,12.0381477794281,-55.475810586866));
#133166=CARTESIAN_POINT('Origin',(-53.4093468596018,12.4562955788561,-55.2016711737319));
#133167=CARTESIAN_POINT('Ctrl Pts',(-53.4093468596018,12.0381477794281,
-55.475810586866));
#133168=CARTESIAN_POINT('Ctrl Pts',(-53.4173436672944,11.9924457375215,
-55.4061007701193));
#133169=CARTESIAN_POINT('Ctrl Pts',(-53.4315945187188,11.9282552364233,
-55.3477500998626));
#133170=CARTESIAN_POINT('Ctrl Pts',(-53.481213741953,11.782936109662,-55.2701189042654));
#133171=CARTESIAN_POINT('Ctrl Pts',(-53.5175339525391,11.7003881248737,
-55.24995));
#133172=CARTESIAN_POINT('Ctrl Pts',(-53.5631588418786,11.61999998,-55.24995));
#133173=CARTESIAN_POINT('Origin',(-48.3718238300661,29.8774509229704,-52.64995));
#133174=CARTESIAN_POINT('',(-51.3604079243413,30.1389181512134,-59.64995));
#133175=CARTESIAN_POINT('',(-51.3604079243413,30.1389181512134,-52.64995));
#133176=CARTESIAN_POINT('',(-51.3604079243413,30.1389181512134,-52.64995));
#133177=CARTESIAN_POINT('',(-50.4931441736257,31.9987712665301,-52.64995));
#133178=CARTESIAN_POINT('Origin',(-48.3718238300661,29.8774509229704,-52.64995));
#133179=CARTESIAN_POINT('',(-50.4931441736257,31.9987712665301,-59.64995));
#133180=CARTESIAN_POINT('',(-50.4931441736257,31.9987712665301,-52.64995));
#133181=CARTESIAN_POINT('Origin',(-48.3718238300661,29.8774509229704,-59.64995));
#133182=CARTESIAN_POINT('Origin',(-51.2652416360248,31.226673804131,-52.64995));
#133183=CARTESIAN_POINT('',(-52.1838946235503,20.7264221086262,-59.64995));
#133184=CARTESIAN_POINT('',(-51.6895836746288,26.3764221086262,-59.64995));
#133185=CARTESIAN_POINT('',(-51.2652416360248,31.226673804131,-59.64995));
#133186=CARTESIAN_POINT('',(-52.1838946235503,20.7264221086262,-55.74995));
#133187=CARTESIAN_POINT('',(-52.1838946235503,20.7264221086262,-52.64995));
#133188=CARTESIAN_POINT('',(-52.2713832870762,19.7264221086262,-54.74995));
#133189=CARTESIAN_POINT('Ctrl Pts',(-52.2713832870762,19.7264221086262,
-54.74995));
#133190=CARTESIAN_POINT('Ctrl Pts',(-52.2484144777976,19.9889568000129,
-54.7499500000658));
#133191=CARTESIAN_POINT('Ctrl Pts',(-52.2257153692336,20.2484087981252,
-54.8577231271255));
#133192=CARTESIAN_POINT('Ctrl Pts',(-52.2095194598201,20.4335288898127,
-55.0428432188135));
#133193=CARTESIAN_POINT('Ctrl Pts',(-52.1933235504066,20.6186489815003,
-55.2279633105015));
#133194=CARTESIAN_POINT('Ctrl Pts',(-52.1838946235561,20.7264221085606,
-55.487415308613));
#133195=CARTESIAN_POINT('Ctrl Pts',(-52.1838946235503,20.7264221086262,
-55.74995));
#133196=CARTESIAN_POINT('',(-52.3151276188392,19.2264221086262,-54.74995));
#133197=CARTESIAN_POINT('',(-51.2652416360248,31.226673804131,-54.74995));
#133198=CARTESIAN_POINT('',(-52.4026162823651,18.2264221086262,-55.74995));
#133199=CARTESIAN_POINT('Ctrl Pts',(-52.4026162823651,18.2264221086262,
-55.74995));
#133200=CARTESIAN_POINT('Ctrl Pts',(-52.4026162823594,18.2264221086918,
-55.4874153086129));
#133201=CARTESIAN_POINT('Ctrl Pts',(-52.3931873555089,18.334195235752,-55.2279633105015));
#133202=CARTESIAN_POINT('Ctrl Pts',(-52.3769914460954,18.5193153274396,
-55.0428432188135));
#133203=CARTESIAN_POINT('Ctrl Pts',(-52.3607955366818,18.7044354191273,
-54.8577231271254));
#133204=CARTESIAN_POINT('Ctrl Pts',(-52.3380964281178,18.9638874172394,
-54.7499500000658));
#133205=CARTESIAN_POINT('Ctrl Pts',(-52.3151276188392,19.2264221086262,
-54.74995));
#133206=CARTESIAN_POINT('',(-52.4026162823651,18.2264221086262,-59.64995));
#133207=CARTESIAN_POINT('',(-52.4026162823651,18.2264221086262,-52.64995));
#133208=CARTESIAN_POINT('',(-52.6206164493001,15.7346687985483,-59.64995));
#133209=CARTESIAN_POINT('',(-51.2652416360248,31.226673804131,-59.64995));
#133210=CARTESIAN_POINT('',(-52.8969272299346,12.5764221085064,-60.0627241236308));
#133211=CARTESIAN_POINT('Ctrl Pts',(-52.8969272285826,12.5764221083881,
-60.0627241236306));
#133212=CARTESIAN_POINT('Ctrl Pts',(-52.8810850690576,12.7574987008071,
-60.0124953264523));
#133213=CARTESIAN_POINT('Ctrl Pts',(-52.8651783101947,12.9393136629347,
-59.9676531117587));
#133214=CARTESIAN_POINT('Ctrl Pts',(-52.8492129207345,13.1217989910892,
-59.9276740961125));
#133215=CARTESIAN_POINT('Ctrl Pts',(-52.8424237249512,13.1993998929342,
-59.910673235274));
#133216=CARTESIAN_POINT('Ctrl Pts',(-52.8356239352219,13.2771218944156,
-59.8945524608641));
#133217=CARTESIAN_POINT('Ctrl Pts',(-52.8288140636153,13.354959116562,-59.8792742373811));
#133218=CARTESIAN_POINT('Ctrl Pts',(-52.8084063492458,13.5882204595985,
-59.8334887014819));
#133219=CARTESIAN_POINT('Ctrl Pts',(-52.7879062369248,13.822537779029,-59.7953375078724));
#133220=CARTESIAN_POINT('Ctrl Pts',(-52.7673307740641,14.0577163898014,
-59.7635551171396));
#133221=CARTESIAN_POINT('Ctrl Pts',(-52.7648947458015,14.0855603195582,
-59.7597922466466));
#133222=CARTESIAN_POINT('Ctrl Pts',(-52.7624575809797,14.1134172399927,
-59.7561214184401));
#133223=CARTESIAN_POINT('Ctrl Pts',(-52.7600192757782,14.1412871946384,
-59.7525428773024));
#133224=CARTESIAN_POINT('Ctrl Pts',(-52.7305287650648,14.4783652583491,
-59.7092615826991));
#133225=CARTESIAN_POINT('Ctrl Pts',(-52.7008776982776,14.8172785115587,
-59.6793561042853));
#133226=CARTESIAN_POINT('Ctrl Pts',(-52.6710582492635,15.1581163818776,
-59.6634323280936));
#133227=CARTESIAN_POINT('Ctrl Pts',(-52.6542978767186,15.3496883214284,
-59.6544821821278));
#133228=CARTESIAN_POINT('Ctrl Pts',(-52.6374843263042,15.541868082155,-59.6499500007379));
#133229=CARTESIAN_POINT('Ctrl Pts',(-52.6206164493001,15.7346687985483,
-59.64995));
#133230=CARTESIAN_POINT('',(-52.8969272312866,12.5764221086262,-55.74995));
#133231=CARTESIAN_POINT('',(-52.8969272312866,12.5764221086262,-52.64995));
#133232=CARTESIAN_POINT('Origin',(-52.9691152015747,11.7513098326049,-55.69773241533));
#133233=CARTESIAN_POINT('',(-51.2652416360248,31.226673804131,-52.64995));
#133234=CARTESIAN_POINT('',(-51.4708620158141,28.8764221086262,-59.64995));
#133235=CARTESIAN_POINT('',(-51.2652416360248,31.226673804131,-59.64995));
#133236=CARTESIAN_POINT('',(-51.4708620158141,28.8764221086262,-55.74995));
#133237=CARTESIAN_POINT('',(-51.4708620158141,28.8764221086262,-52.64995));
#133238=CARTESIAN_POINT('',(-51.55835067934,27.8764221086262,-54.74995));
#133239=CARTESIAN_POINT('Ctrl Pts',(-51.55835067934,27.8764221086262,-54.74995));
#133240=CARTESIAN_POINT('Ctrl Pts',(-51.5353818700614,28.1389568000129,
-54.7499500000658));
#133241=CARTESIAN_POINT('Ctrl Pts',(-51.5126827614974,28.3984087981251,
-54.8577231271254));
#133242=CARTESIAN_POINT('Ctrl Pts',(-51.4964868520838,28.5835288898127,
-55.0428432188135));
#133243=CARTESIAN_POINT('Ctrl Pts',(-51.4802909426703,28.7686489815003,
-55.2279633105015));
#133244=CARTESIAN_POINT('Ctrl Pts',(-51.4708620158198,28.8764221085606,
-55.4874153086129));
#133245=CARTESIAN_POINT('Ctrl Pts',(-51.4708620158141,28.8764221086262,
-55.74995));
#133246=CARTESIAN_POINT('',(-51.6020950111029,27.3764221086262,-54.74995));
#133247=CARTESIAN_POINT('',(-51.2652416360248,31.226673804131,-54.74995));
#133248=CARTESIAN_POINT('',(-51.6895836746288,26.3764221086262,-55.74995));
#133249=CARTESIAN_POINT('Ctrl Pts',(-51.6895836746288,26.3764221086262,
-55.74995));
#133250=CARTESIAN_POINT('Ctrl Pts',(-51.6895836746231,26.3764221086917,
-55.4874153086129));
#133251=CARTESIAN_POINT('Ctrl Pts',(-51.6801547477726,26.484195235752,-55.2279633105015));
#133252=CARTESIAN_POINT('Ctrl Pts',(-51.6639588383591,26.6693153274396,
-55.0428432188135));
#133253=CARTESIAN_POINT('Ctrl Pts',(-51.6477629289455,26.8544354191273,
-54.8577231271254));
#133254=CARTESIAN_POINT('Ctrl Pts',(-51.6250638203816,27.1138874172394,
-54.7499500000658));
#133255=CARTESIAN_POINT('Ctrl Pts',(-51.6020950111029,27.3764221086262,
-54.74995));
#133256=CARTESIAN_POINT('',(-51.6895836746288,26.3764221086262,-52.64995));
#133257=CARTESIAN_POINT('Origin',(-48.3718238300661,29.8774509229704,-59.64995));
#133258=CARTESIAN_POINT('',(-50.3642132262496,30.0517624084658,-60.64995));
#133259=CARTESIAN_POINT('Origin',(-50.3642132262496,30.0517624084658,-59.64995));
#133260=CARTESIAN_POINT('',(-49.7860373924392,31.2916644853436,-60.64995));
#133261=CARTESIAN_POINT('Origin',(-49.7860373924392,31.2916644853435,-59.64995));
#133262=CARTESIAN_POINT('Origin',(-48.3718238300661,29.8774509229704,-60.64995));
#133263=CARTESIAN_POINT('Origin',(-42.8449509429988,35.4043238100378,-52.64995));
#133264=CARTESIAN_POINT('',(-44.9662712865584,37.5256441535974,-59.64995));
#133265=CARTESIAN_POINT('',(-44.9662712865584,37.5256441535974,-52.64995));
#133266=CARTESIAN_POINT('',(-44.9662712865584,37.5256441535974,-52.64995));
#133267=CARTESIAN_POINT('',(-43.1064181712417,38.392907904313,-52.64995));
#133268=CARTESIAN_POINT('Origin',(-42.8449509429988,35.4043238100378,-52.64995));
#133269=CARTESIAN_POINT('',(-43.1064181712417,38.392907904313,-59.64995));
#133270=CARTESIAN_POINT('',(-43.1064181712417,38.392907904313,-52.64995));
#133271=CARTESIAN_POINT('Origin',(-42.8449509429988,35.4043238100378,-59.64995));
#133272=CARTESIAN_POINT('Origin',(-44.1941738241593,38.2977416159964,-52.64995));
#133273=CARTESIAN_POINT('',(-44.1941738241593,38.2977416159964,-52.64995));
#133274=CARTESIAN_POINT('',(-44.1941738241593,38.2977416159964,-59.64995));
#133275=CARTESIAN_POINT('Origin',(-42.8449509429988,35.4043238100378,-59.64995));
#133276=CARTESIAN_POINT('',(-44.2591645053719,36.8185373724109,-60.64995));
#133277=CARTESIAN_POINT('Origin',(-44.2591645053719,36.8185373724109,-59.64995));
#133278=CARTESIAN_POINT('',(-43.019262428494,37.3967132062212,-60.64995));
#133279=CARTESIAN_POINT('Origin',(-43.019262428494,37.3967132062212,-59.64995));
#133280=CARTESIAN_POINT('Origin',(-42.8449509429988,35.4043238100378,-60.64995));
#133281=CARTESIAN_POINT('Origin',(-24.5275331667447,40.0183497231583,-52.64995));
#133282=CARTESIAN_POINT('',(-36.9564221286262,38.9309628387712,-59.64995));
#133283=CARTESIAN_POINT('',(-30.9564221286262,39.4558948199267,-59.64995));
#133284=CARTESIAN_POINT('',(-24.5275331667447,40.0183497231583,-59.64995));
#133285=CARTESIAN_POINT('',(-36.9564221286262,38.9309628387712,-55.74995));
#133286=CARTESIAN_POINT('',(-36.9564221286262,38.9309628387712,-52.64995));
#133287=CARTESIAN_POINT('',(-37.9564221286262,38.8434741752452,-54.74995));
#133288=CARTESIAN_POINT('Ctrl Pts',(-37.9564221286262,38.8434741752452,
-54.74995));
#133289=CARTESIAN_POINT('Ctrl Pts',(-37.6938874372391,38.8664429845239,
-54.7499500000658));
#133290=CARTESIAN_POINT('Ctrl Pts',(-37.4344354391277,38.8891420930878,
-54.8577231271255));
#133291=CARTESIAN_POINT('Ctrl Pts',(-37.2493153474397,38.9053380025014,
-55.0428432188135));
#133292=CARTESIAN_POINT('Ctrl Pts',(-37.0641952557516,38.9215339119149,
-55.2279633105015));
#133293=CARTESIAN_POINT('Ctrl Pts',(-36.9564221286917,38.9309628387654,
-55.487415308613));
#133294=CARTESIAN_POINT('Ctrl Pts',(-36.9564221286262,38.9309628387712,
-55.74995));
#133295=CARTESIAN_POINT('',(-38.4564221286262,38.7997298434823,-54.74995));
#133296=CARTESIAN_POINT('',(-38.,38.8396616055195,-54.74995));
#133297=CARTESIAN_POINT('',(-39.4564221286262,38.7122411799564,-55.74995));
#133298=CARTESIAN_POINT('Ctrl Pts',(-39.4564221286262,38.7122411799564,
-55.74995));
#133299=CARTESIAN_POINT('Ctrl Pts',(-39.4564221285606,38.7122411799621,
-55.487415308613));
#133300=CARTESIAN_POINT('Ctrl Pts',(-39.3486490015007,38.7216701068126,
-55.2279633105015));
#133301=CARTESIAN_POINT('Ctrl Pts',(-39.1635289098127,38.7378660162261,
-55.0428432188135));
#133302=CARTESIAN_POINT('Ctrl Pts',(-38.9784088181247,38.7540619256397,
-54.8577231271255));
#133303=CARTESIAN_POINT('Ctrl Pts',(-38.7189568200132,38.7767610342036,
-54.7499500000658));
#133304=CARTESIAN_POINT('Ctrl Pts',(-38.4564221286262,38.7997298434823,
-54.74995));
#133305=CARTESIAN_POINT('',(-39.4564221286262,38.7122411799564,-59.64995));
#133306=CARTESIAN_POINT('',(-39.4564221286262,38.7122411799564,-55.74995));
#133307=CARTESIAN_POINT('',(-24.5275331667447,40.0183497231583,-59.64995));
#133308=CARTESIAN_POINT('',(-24.5275331667447,40.0183497231583,-52.64995));
#133309=CARTESIAN_POINT('',(-28.4564221286262,39.6746164787415,-59.6524466674074));
#133310=CARTESIAN_POINT('Ctrl Pts',(-28.4564221286157,39.6746164786217,
-59.6524466674074));
#133311=CARTESIAN_POINT('Ctrl Pts',(-28.131799882143,39.7030172440175,-59.6590182799318));
#133312=CARTESIAN_POINT('Ctrl Pts',(-27.8089020756434,39.7312671410702,
-59.6781506934662));
#133313=CARTESIAN_POINT('Ctrl Pts',(-27.4876982951987,39.759368830939,-59.7096215394405));
#133314=CARTESIAN_POINT('Ctrl Pts',(-27.3141484358439,39.7745524764041,
-59.7266255762083));
#133315=CARTESIAN_POINT('Ctrl Pts',(-27.1410937670819,39.7896927982217,
-59.7472310046319));
#133316=CARTESIAN_POINT('Ctrl Pts',(-26.9685328542776,39.8047899206072,
-59.7713974032318));
#133317=CARTESIAN_POINT('Ctrl Pts',(-26.9471826335434,39.8066578227303,
-59.7743874079558));
#133318=CARTESIAN_POINT('Ctrl Pts',(-26.9258394639526,39.8085251079323,
-59.7774303163423));
#133319=CARTESIAN_POINT('Ctrl Pts',(-26.904503506364,39.8103917621319,-59.7805271013239));
#133320=CARTESIAN_POINT('Ctrl Pts',(-26.5372951385281,39.8425183277711,
-59.8338251712089));
#133321=CARTESIAN_POINT('Ctrl Pts',(-26.1722508037018,39.8744555741516,
-59.9028698737186));
#133322=CARTESIAN_POINT('Ctrl Pts',(-25.8100560258455,39.9061435120041,
-59.9926952103956));
#133323=CARTESIAN_POINT('Ctrl Pts',(-25.6663124460746,39.9187194460069,
-60.0283440276549));
#133324=CARTESIAN_POINT('Ctrl Pts',(-25.5230181721787,39.9312560704728,
-60.0672655467087));
#133325=CARTESIAN_POINT('Ctrl Pts',(-25.3802177275058,39.9437494905281,
-60.1097730249189));
#133326=CARTESIAN_POINT('',(-28.4564221286262,39.6746164787415,-55.74995));
#133327=CARTESIAN_POINT('',(-28.4564221286262,39.6746164787415,-52.64995));
#133328=CARTESIAN_POINT('',(-29.4564221286262,39.5871278152156,-54.74995));
#133329=CARTESIAN_POINT('Ctrl Pts',(-29.4564221286262,39.5871278152156,
-54.74995));
#133330=CARTESIAN_POINT('Ctrl Pts',(-29.1938874372394,39.6100966244942,
-54.7499500000658));
#133331=CARTESIAN_POINT('Ctrl Pts',(-28.9344354391271,39.6327957330582,
-54.8577231271255));
#133332=CARTESIAN_POINT('Ctrl Pts',(-28.7493153474396,39.6489916424717,
-55.0428432188135));
#133333=CARTESIAN_POINT('Ctrl Pts',(-28.5641952557521,39.6651875518853,
-55.2279633105015));
#133334=CARTESIAN_POINT('Ctrl Pts',(-28.4564221286917,39.6746164787358,
-55.487415308613));
#133335=CARTESIAN_POINT('Ctrl Pts',(-28.4564221286262,39.6746164787415,
-55.74995));
#133336=CARTESIAN_POINT('',(-29.9564221286262,39.5433834834526,-54.74995));
#133337=CARTESIAN_POINT('',(-29.5,39.5833152454898,-54.74995));
#133338=CARTESIAN_POINT('',(-30.9564221286262,39.4558948199267,-55.74995));
#133339=CARTESIAN_POINT('Ctrl Pts',(-30.9564221286262,39.4558948199267,
-55.74995));
#133340=CARTESIAN_POINT('Ctrl Pts',(-30.9564221285606,39.4558948199325,
-55.4874153086129));
#133341=CARTESIAN_POINT('Ctrl Pts',(-30.8486490015003,39.4653237467829,
-55.2279633105015));
#133342=CARTESIAN_POINT('Ctrl Pts',(-30.6635289098127,39.4815196561965,
-55.0428432188135));
#133343=CARTESIAN_POINT('Ctrl Pts',(-30.4784088181251,39.4977155656101,
-54.8577231271254));
#133344=CARTESIAN_POINT('Ctrl Pts',(-30.218956820013,39.520414674174,-54.7499500000658));
#133345=CARTESIAN_POINT('Ctrl Pts',(-29.9564221286262,39.5433834834526,
-54.74995));
#133346=CARTESIAN_POINT('',(-30.9564221286262,39.4558948199267,-52.64995));
#133347=CARTESIAN_POINT('Ctrl Pts',(-53.6173229282256,-36.0820590308261,
-55.74995));
#133348=CARTESIAN_POINT('Ctrl Pts',(-53.3164388612999,-36.78000002,-55.7499499999999));
#133349=CARTESIAN_POINT('Ctrl Pts',(-54.076473627675,-36.78000002,-55.74995));
#133350=CARTESIAN_POINT('Ctrl Pts',(-53.6173229109667,-36.0820590708605,
-55.5352328299022));
#133351=CARTESIAN_POINT('Ctrl Pts',(-53.3164388632929,-36.7800000140484,
-55.7160682965194));
#133352=CARTESIAN_POINT('Ctrl Pts',(-54.07647361027,-36.78000002,-55.6425914202082));
#133353=CARTESIAN_POINT('Ctrl Pts',(-53.587398316273,-36.1517305970246,
-55.3270423559178));
#133354=CARTESIAN_POINT('Ctrl Pts',(-53.3223470981189,-36.7637806572682,
-55.672084159207));
#133355=CARTESIAN_POINT('Ctrl Pts',(-54.0462927577141,-36.8151341090744,
-55.5384961709319));
#133356=CARTESIAN_POINT('Ctrl Pts',(-53.481339980492,-36.3953483985127,
-54.9914263135601));
#133357=CARTESIAN_POINT('Ctrl Pts',(-53.3111802821853,-36.783202746029,
-55.5229519438579));
#133358=CARTESIAN_POINT('Ctrl Pts',(-53.939326192416,-36.9379861363991,
-55.370688163807));
#133359=CARTESIAN_POINT('Ctrl Pts',(-53.4080974646291,-36.562334686105,
-54.8706857163843));
#133360=CARTESIAN_POINT('Ctrl Pts',(-53.293833750711,-36.8201344622738,
-55.429912748872));
#133361=CARTESIAN_POINT('Ctrl Pts',(-53.8654589377065,-37.0221914881654,
-55.3103188190833));
#133362=CARTESIAN_POINT('Ctrl Pts',(-53.3256899305316,-36.747133105635,
-54.8057004429533));
#133363=CARTESIAN_POINT('Ctrl Pts',(-53.2549772028899,-36.9057059891941,
-55.3509337052243));
#133364=CARTESIAN_POINT('Ctrl Pts',(-53.7823432375794,-37.1153847305999,
-55.2778252214766));
#133365=CARTESIAN_POINT('',(-54.076473627675,-36.78000002,-55.74995));
#133366=CARTESIAN_POINT('Origin',(-54.076473627675,-36.28000002,-55.74995));
#133367=CARTESIAN_POINT('Ctrl Pts',(-54.076473627675,-36.78000002,-55.74995));
#133368=CARTESIAN_POINT('Ctrl Pts',(-54.07647361027,-36.78000002,-55.6425914202082));
#133369=CARTESIAN_POINT('Ctrl Pts',(-54.0462927577141,-36.8151341090744,
-55.5384961709319));
#133370=CARTESIAN_POINT('Ctrl Pts',(-53.939326192416,-36.9379861363991,
-55.370688163807));
#133371=CARTESIAN_POINT('Ctrl Pts',(-53.8654589377065,-37.0221914881654,
-55.3103188190833));
#133372=CARTESIAN_POINT('Ctrl Pts',(-53.7823432375799,-37.1153847305994,
-55.2778252214768));
#133373=CARTESIAN_POINT('Origin',(-54.076473627675,-36.28000002,-55.24995));
#133374=CARTESIAN_POINT('',(-54.076473627675,-36.78000002,-60.42825533736));
#133375=CARTESIAN_POINT('Origin',(-54.076473627675,-36.28000002,-60.42825533736));
#133376=CARTESIAN_POINT('',(-54.076473627675,-36.78000002,-55.24995));
#133377=CARTESIAN_POINT('Origin',(0.,-12.9675000200281,-60.42825533736));
#133378=CARTESIAN_POINT('',(-55.5967474138374,-30.4937575588533,-60.8508735991007));
#133379=CARTESIAN_POINT('',(-53.5074514076768,-36.1001753985996,-60.8508735991007));
#133380=CARTESIAN_POINT('Origin',(0.,-12.9675000200281,-60.8508735991007));
#133381=CARTESIAN_POINT('Origin',(-52.5655138039885,-36.2558013973473,-60.449477355207));
#133382=CARTESIAN_POINT('Origin',(-54.5663882978998,-30.6330498593666,-60.4192568707561));
#133383=CARTESIAN_POINT('Origin',(-56.1762739063772,-30.63000002,-55.24995));
#133384=CARTESIAN_POINT('',(-56.1762739063771,-30.13000002,-55.74995));
#133385=CARTESIAN_POINT('Origin',(-56.1762739063772,-30.63000002,-55.74995));
#133386=CARTESIAN_POINT('',(-56.1762739063772,-30.13000002,-60.42825533736));
#133387=CARTESIAN_POINT('',(-56.1762739063772,-30.13000002,-55.24995));
#133388=CARTESIAN_POINT('Origin',(-56.1762739063772,-30.63000002,-60.42825533736));
#133389=CARTESIAN_POINT('Ctrl Pts',(-56.0013925566522,-29.4885226266656,
-54.74995));
#133390=CARTESIAN_POINT('Ctrl Pts',(-56.0013925566522,-29.4885226266655,
-55.2499499999999));
#133391=CARTESIAN_POINT('Ctrl Pts',(-56.4809591809864,-29.63000002,-55.24995));
#133392=CARTESIAN_POINT('Ctrl Pts',(-55.9637778607192,-29.6160253486821,
-54.7499500197391));
#133393=CARTESIAN_POINT('Ctrl Pts',(-55.9815963325889,-29.5556259878439,
-55.2320894585059));
#133394=CARTESIAN_POINT('Ctrl Pts',(-56.4430235619105,-29.6942952977694,
-55.24995));
#133395=CARTESIAN_POINT('Ctrl Pts',(-55.9259713199402,-29.7425201026704,
-54.7747042862246));
#133396=CARTESIAN_POINT('Ctrl Pts',(-55.9595264494602,-29.6302973578872,
-55.2276198610214));
#133397=CARTESIAN_POINT('Ctrl Pts',(-56.4048920758008,-29.7580863098899,
-55.2623271401185));
#133398=CARTESIAN_POINT('Ctrl Pts',(-55.8541342694537,-29.9801791700519,
-54.8719723798496));
#133399=CARTESIAN_POINT('Ctrl Pts',(-55.9152124797534,-29.7792875750423,
-55.2543206061649));
#133400=CARTESIAN_POINT('Ctrl Pts',(-56.3324398513309,-29.877933435243,
-55.3109611929186));
#133401=CARTESIAN_POINT('Ctrl Pts',(-55.8207323820705,-30.0892808127342,
-54.9437622390698));
#133402=CARTESIAN_POINT('Ctrl Pts',(-55.8932648786607,-29.8526235485765,
-55.2844345178149));
#133403=CARTESIAN_POINT('Ctrl Pts',(-56.2987519266105,-29.9329514036474,
-55.3468561181883));
#133404=CARTESIAN_POINT('Ctrl Pts',(-55.7350468385274,-30.3669899517508,
-55.2177384600888));
#133405=CARTESIAN_POINT('Ctrl Pts',(-55.8363250868006,-30.0417896984651,
-55.4221362713026));
#133406=CARTESIAN_POINT('Ctrl Pts',(-56.2123326186624,-30.0729950473548,
-55.4838442327376));
#133407=CARTESIAN_POINT('Ctrl Pts',(-55.699294301712,-30.4800318342627,
-55.4780587856325));
#133408=CARTESIAN_POINT('Ctrl Pts',(-55.8093485438182,-30.1300000005986,
-55.5818806132723));
#133409=CARTESIAN_POINT('Ctrl Pts',(-56.1762739146114,-30.1300000200003,
-55.614004390749));
#133410=CARTESIAN_POINT('Ctrl Pts',(-55.6992942935022,-30.4800318603742,
-55.74995));
#133411=CARTESIAN_POINT('Ctrl Pts',(-55.8093485379488,-30.1300000200003,
-55.7499499999999));
#133412=CARTESIAN_POINT('Ctrl Pts',(-56.1762739063772,-30.1300000200003,
-55.74995));
#133413=CARTESIAN_POINT('',(-56.4809591809864,-29.63000002,-55.24995));
#133414=CARTESIAN_POINT('Origin',(-56.4809591809864,-29.63000002,-54.74995));
#133415=CARTESIAN_POINT('Ctrl Pts',(-56.4809591809864,-29.63000002,-55.24995));
#133416=CARTESIAN_POINT('Ctrl Pts',(-56.4430235619105,-29.6942952977694,
-55.24995));
#133417=CARTESIAN_POINT('Ctrl Pts',(-56.4048920758008,-29.7580863098899,
-55.2623271401185));
#133418=CARTESIAN_POINT('Ctrl Pts',(-56.3324398513309,-29.877933435243,
-55.3109611929186));
#133419=CARTESIAN_POINT('Ctrl Pts',(-56.2987519266105,-29.9329514036474,
-55.3468561181883));
#133420=CARTESIAN_POINT('Ctrl Pts',(-56.2123326186624,-30.0729950473548,
-55.4838442327376));
#133421=CARTESIAN_POINT('Ctrl Pts',(-56.1762739146114,-30.1300000200003,
-55.614004390749));
#133422=CARTESIAN_POINT('Ctrl Pts',(-56.1762739063771,-30.13000002,-55.74995));
#133423=CARTESIAN_POINT('Origin',(0.,-12.9675000200281,-54.74995));
#133424=CARTESIAN_POINT('',(-56.6260651114328,-29.13000002,-55.24995));
#133425=CARTESIAN_POINT('Origin',(-56.6260651114328,-29.13000002,-54.74995));
#133426=CARTESIAN_POINT('Origin',(0.,-12.9675000200281,-55.24995));
#133427=CARTESIAN_POINT('Ctrl Pts',(-56.418846619879,-28.0012587761031,
-55.74995));
#133428=CARTESIAN_POINT('Ctrl Pts',(-56.2513078496445,-28.6300000199999,
-55.74995));
#133429=CARTESIAN_POINT('Ctrl Pts',(-56.9019881023868,-28.63000002,-55.74995));
#133430=CARTESIAN_POINT('Ctrl Pts',(-56.4188466136678,-28.0012587994123,
-55.6168335059946));
#133431=CARTESIAN_POINT('Ctrl Pts',(-56.2513078484208,-28.6300000235388,
-55.7066092661189));
#133432=CARTESIAN_POINT('Ctrl Pts',(-56.9019880961229,-28.63000002,-55.6833917541491));
#133433=CARTESIAN_POINT('Ctrl Pts',(-56.4116877572674,-28.0281919581543,
-55.4831809085995));
#133434=CARTESIAN_POINT('Ctrl Pts',(-56.2500205046201,-28.6336048267405,
-55.662915181482));
#133435=CARTESIAN_POINT('Ctrl Pts',(-56.8947679354133,-28.6435819282218,
-55.6165654527396));
#133436=CARTESIAN_POINT('Ctrl Pts',(-56.3842918802123,-28.1304346451459,
-55.2389052692862));
#133437=CARTESIAN_POINT('Ctrl Pts',(-56.2435792593614,-28.6535512137473,
-55.5706051556274));
#133438=CARTESIAN_POINT('Ctrl Pts',(-56.8671374536179,-28.6951410554417,
-55.4944276362032));
#133439=CARTESIAN_POINT('Ctrl Pts',(-56.3639882171558,-28.2059422564823,
-55.1276612780425));
#133440=CARTESIAN_POINT('Ctrl Pts',(-56.2384193392041,-28.6700167701719,
-55.5221237308774));
#133441=CARTESIAN_POINT('Ctrl Pts',(-56.8466599215264,-28.733218160043,
-55.438805637664));
#133442=CARTESIAN_POINT('Ctrl Pts',(-56.313802009893,-28.3903724090483,
-54.9450496744345));
#133443=CARTESIAN_POINT('Ctrl Pts',(-56.2221065093684,-28.7248002564605,
-55.4263976661905));
#133444=CARTESIAN_POINT('Ctrl Pts',(-56.7960439448031,-28.8262229205127,
-55.3474998385745));
#133445=CARTESIAN_POINT('Ctrl Pts',(-56.2834891741183,-28.5008198383441,
-54.8722499675113));
#133446=CARTESIAN_POINT('Ctrl Pts',(-56.2109691262328,-28.7630648267862,
-55.3789982403422));
#133447=CARTESIAN_POINT('Ctrl Pts',(-56.7654715266632,-28.8819195410099,
-55.3110999839041));
#133448=CARTESIAN_POINT('Ctrl Pts',(-56.2177799652687,-28.7369766748766,
-54.7752816287617));
#133449=CARTESIAN_POINT('Ctrl Pts',(-56.1824656282838,-28.8623399510796,
-55.300226361809));
#133450=CARTESIAN_POINT('Ctrl Pts',(-56.6991996177705,-29.0010091208419,
-55.2626158142325));
#133451=CARTESIAN_POINT('Ctrl Pts',(-56.1815764992065,-28.8655539935311,
-54.749950013458));
#133452=CARTESIAN_POINT('Ctrl Pts',(-56.1650303807126,-28.9235240815735,
-55.2679072059029));
#133453=CARTESIAN_POINT('Ctrl Pts',(-56.6626879858136,-29.0658450537332,
-55.24995));
#133454=CARTESIAN_POINT('Ctrl Pts',(-56.1452664265556,-28.9927680098115,
-54.74995));
#133455=CARTESIAN_POINT('Ctrl Pts',(-56.1452664265556,-28.9927680098115,
-55.24995));
#133456=CARTESIAN_POINT('Ctrl Pts',(-56.6260651114328,-29.1300000200001,
-55.24995));
#133457=CARTESIAN_POINT('',(-56.9019881023868,-28.63000002,-55.74995));
#133458=CARTESIAN_POINT('Origin',(-56.9019881023868,-28.13000002,-55.74995));
#133459=CARTESIAN_POINT('Ctrl Pts',(-56.9019881023868,-28.63000002,-55.74995));
#133460=CARTESIAN_POINT('Ctrl Pts',(-56.9019880961229,-28.63000002,-55.6833917541491));
#133461=CARTESIAN_POINT('Ctrl Pts',(-56.8947679354133,-28.6435819282218,
-55.6165654527396));
#133462=CARTESIAN_POINT('Ctrl Pts',(-56.8671374536179,-28.6951410554417,
-55.4944276362032));
#133463=CARTESIAN_POINT('Ctrl Pts',(-56.8466599215264,-28.733218160043,
-55.438805637664));
#133464=CARTESIAN_POINT('Ctrl Pts',(-56.7960439448031,-28.8262229205127,
-55.3474998385745));
#133465=CARTESIAN_POINT('Ctrl Pts',(-56.7654715266632,-28.8819195410099,
-55.3110999839041));
#133466=CARTESIAN_POINT('Ctrl Pts',(-56.6991996177705,-29.0010091208419,
-55.2626158142325));
#133467=CARTESIAN_POINT('Ctrl Pts',(-56.6626879858136,-29.0658450537332,
-55.24995));
#133468=CARTESIAN_POINT('Ctrl Pts',(-56.6260651114328,-29.13000002,-55.24995));
#133469=CARTESIAN_POINT('Origin',(-56.9019881023868,-28.13000002,-55.24995));
#133470=CARTESIAN_POINT('',(-56.9019881023868,-28.63000002,-60.42825533736));
#133471=CARTESIAN_POINT('Origin',(-56.9019881023868,-28.13000002,-60.42825533736));
#133472=CARTESIAN_POINT('',(-56.9019881023868,-28.63000002,-55.24995));
#133473=CARTESIAN_POINT('Origin',(0.,-12.9675000200281,-60.42825533736));
#133474=CARTESIAN_POINT('',(-57.5245249214072,-22.4066238608121,-60.8508735991007));
#133475=CARTESIAN_POINT('',(-56.3187331343194,-28.0130417005584,-60.8508735991007));
#133476=CARTESIAN_POINT('Origin',(0.,-12.9675000200281,-60.8508735991007));
#133477=CARTESIAN_POINT('Origin',(-55.0588362446609,-28.1616614222003,-60.3670915993992));
#133478=CARTESIAN_POINT('Origin',(-56.5772574599055,-22.4805096121333,-60.4242148671621));
#133479=CARTESIAN_POINT('Origin',(-58.1141118834647,-22.48000002,-55.24995));
#133480=CARTESIAN_POINT('',(-58.1141118834647,-21.98000002,-60.42825533736));
#133481=CARTESIAN_POINT('Origin',(-58.1141118834647,-22.48000002,-60.42825533736));
#133482=CARTESIAN_POINT('',(-58.1141118834537,-21.9800000069849,-55.913606468422));
#133483=CARTESIAN_POINT('Origin',(-58.1141118834647,-22.48000002,-55.9136064684106));
#133484=CARTESIAN_POINT('',(-58.1141118834647,-21.98000002,-55.24995));
#133485=CARTESIAN_POINT('Ctrl Pts',(-57.7689991024638,-21.4435190710229,
-54.8883584020538));
#133486=CARTESIAN_POINT('Ctrl Pts',(-57.7681097820422,-21.4495803068843,
-55.2303260732311));
#133487=CARTESIAN_POINT('Ctrl Pts',(-58.0831736437665,-21.4980516416407,
-55.3542805420643));
#133488=CARTESIAN_POINT('Ctrl Pts',(-57.7500908600563,-21.5723897392102,
-54.8860050875463));
#133489=CARTESIAN_POINT('Ctrl Pts',(-57.7561082976293,-21.5312836766001,
-55.2240269539559));
#133490=CARTESIAN_POINT('Ctrl Pts',(-58.0674311963076,-21.5630475770342,
-55.3506990738629));
#133491=CARTESIAN_POINT('Ctrl Pts',(-57.7304928612488,-21.702757912867,
-54.9116382623115));
#133492=CARTESIAN_POINT('Ctrl Pts',(-57.7435735661121,-21.6157110452939,
-55.2378962877635));
#133493=CARTESIAN_POINT('Ctrl Pts',(-58.0543804972822,-21.6287810566872,
-55.3623310903062));
#133494=CARTESIAN_POINT('Ctrl Pts',(-57.6941246628956,-21.9398194436421,
-55.0150801896028));
#133495=CARTESIAN_POINT('Ctrl Pts',(-57.720944678806,-21.7667785312353,
-55.3041336540307));
#133496=CARTESIAN_POINT('Ctrl Pts',(-58.0368385085867,-21.7483268550824,
-55.4143541528288));
#133497=CARTESIAN_POINT('Ctrl Pts',(-57.6771952780886,-22.0476481665544,
-55.0933432841215));
#133498=CARTESIAN_POINT('Ctrl Pts',(-57.7106605173207,-21.8347350541072,
-55.3571283178239));
#133499=CARTESIAN_POINT('Ctrl Pts',(-58.0322828839583,-21.8027029130102,
-55.4549704742887));
#133500=CARTESIAN_POINT('Ctrl Pts',(-57.6494812249724,-22.2219724523816,
-55.2860232465006));
#133501=CARTESIAN_POINT('Ctrl Pts',(-57.695076042676,-21.9376161761805,
-55.488705776954));
#133502=CARTESIAN_POINT('Ctrl Pts',(-58.0344578164564,-21.8906114651791,
-55.5576238485917));
#133503=CARTESIAN_POINT('Ctrl Pts',(-57.6385084201743,-22.2897585279143,
-55.4017143890713));
#133504=CARTESIAN_POINT('Ctrl Pts',(-57.6896470027836,-21.9734580917706,
-55.5692031110363));
#133505=CARTESIAN_POINT('Ctrl Pts',(-58.0412481050148,-21.9247947465257,
-55.6203478572209));
#133506=CARTESIAN_POINT('Ctrl Pts',(-57.6241589914286,-22.3780503291714,
-55.6490268368888));
#133507=CARTESIAN_POINT('Ctrl Pts',(-57.6849292160896,-22.0058199931385,
-55.7382976471412));
#133508=CARTESIAN_POINT('Ctrl Pts',(-58.0678405993018,-21.9693186886025,
-55.7585030512593));
#133509=CARTESIAN_POINT('Ctrl Pts',(-57.6206785404325,-22.3992316104322,
-55.7821117710573));
#133510=CARTESIAN_POINT('Ctrl Pts',(-57.6857286259381,-22.0018252542719,
-55.8292768225565));
#133511=CARTESIAN_POINT('Ctrl Pts',(-58.0878569699436,-21.9800000199996,
-55.8347456438184));
#133512=CARTESIAN_POINT('Ctrl Pts',(-57.6206785412152,-22.3992316056509,
-55.9136064684106));
#133513=CARTESIAN_POINT('Ctrl Pts',(-57.6893011240825,-21.9800000200013,
-55.9136064684131));
#133514=CARTESIAN_POINT('Ctrl Pts',(-58.1141118834632,-21.98000002,-55.9136064684135));
#133515=CARTESIAN_POINT('',(-58.0831736436651,-21.4980516422417,-55.3542805420483));
#133516=CARTESIAN_POINT('Origin',(-58.2637025843942,-21.516103263282,-54.8883584020538));
#133517=CARTESIAN_POINT('Ctrl Pts',(-58.0831736437664,-21.4980516416407,
-55.3542805420642));
#133518=CARTESIAN_POINT('Ctrl Pts',(-58.0674311963076,-21.5630475770342,
-55.3506990738629));
#133519=CARTESIAN_POINT('Ctrl Pts',(-58.0543804972822,-21.6287810566872,
-55.3623310903062));
#133520=CARTESIAN_POINT('Ctrl Pts',(-58.0368385085867,-21.7483268550824,
-55.4143541528288));
#133521=CARTESIAN_POINT('Ctrl Pts',(-58.0322828839583,-21.8027029130102,
-55.4549704742887));
#133522=CARTESIAN_POINT('Ctrl Pts',(-58.0344578164564,-21.8906114651791,
-55.5576238485917));
#133523=CARTESIAN_POINT('Ctrl Pts',(-58.0412481050148,-21.9247947465257,
-55.6203478572209));
#133524=CARTESIAN_POINT('Ctrl Pts',(-58.0678405993018,-21.9693186886025,
-55.7585030512593));
#133525=CARTESIAN_POINT('Ctrl Pts',(-58.0878569699436,-21.9800000199996,
-55.8347456438184));
#133526=CARTESIAN_POINT('Ctrl Pts',(-58.1141118834578,-21.98000002,-55.9136064684144));
#133527=CARTESIAN_POINT('Ctrl Pts',(-57.8394345625603,-20.9487258492223,
-54.8970741880307));
#133528=CARTESIAN_POINT('Ctrl Pts',(-57.8386732172432,-20.9542432701794,
-55.231054762791));
#133529=CARTESIAN_POINT('Ctrl Pts',(-58.1440639002148,-20.9985364556095,
-55.3589167601806));
#133530=CARTESIAN_POINT('Ctrl Pts',(-57.8166617235658,-21.1137591610236,
-54.8942721021231));
#133531=CARTESIAN_POINT('Ctrl Pts',(-57.8158059697179,-21.1198442176538,
-55.2308230742677));
#133532=CARTESIAN_POINT('Ctrl Pts',(-58.124377168252,-21.1650956023415,
-55.357473843553));
#133533=CARTESIAN_POINT('Ctrl Pts',(-57.7931832180155,-21.2786902591483,
-54.8913683748515));
#133534=CARTESIAN_POINT('Ctrl Pts',(-57.7922771725925,-21.2849855841189,
-55.2305804544121));
#133535=CARTESIAN_POINT('Ctrl Pts',(-58.1040803997663,-21.3315995267041,
-55.3559321998119));
#133536=CARTESIAN_POINT('Ctrl Pts',(-57.7689991024637,-21.4435190710235,
-54.8883584020537));
#133537=CARTESIAN_POINT('Ctrl Pts',(-57.7681097820422,-21.4495803068845,
-55.2303260732311));
#133538=CARTESIAN_POINT('Ctrl Pts',(-58.0831736437665,-21.4980516416408,
-55.3542805420642));
#133539=CARTESIAN_POINT('',(-58.1440636542725,-20.9985364317146,-55.3589173554775));
#133540=CARTESIAN_POINT('Origin',(-58.3347412169172,-21.017072891219,-54.8970741880307));
#133541=CARTESIAN_POINT('Origin',(8.40472652016414,-13.0339084621842,-43.9483258606649));
#133542=CARTESIAN_POINT('Ctrl Pts',(-57.970850887931,-19.9304072883579,
-56.2895381767097));
#133543=CARTESIAN_POINT('Ctrl Pts',(-57.8976234932917,-20.54001496768,-56.2187331880681));
#133544=CARTESIAN_POINT('Ctrl Pts',(-58.5127149485701,-20.4849816559984,
-56.2328156683283));
#133545=CARTESIAN_POINT('Ctrl Pts',(-57.9735750287413,-19.9074135537666,
-56.0766526555005));
#133546=CARTESIAN_POINT('Ctrl Pts',(-57.9072350111286,-20.4617756146749,
-56.1016741619115));
#133547=CARTESIAN_POINT('Ctrl Pts',(-58.4599257443274,-20.4734298477889,
-56.0837094320831));
#133548=CARTESIAN_POINT('Ctrl Pts',(-57.9717019896149,-19.9235035634186,
-55.8706894656042));
#133549=CARTESIAN_POINT('Ctrl Pts',(-57.9119143840911,-20.421400833978,
-55.9614017711877));
#133550=CARTESIAN_POINT('Ctrl Pts',(-58.4131413827532,-20.4815791649057,
-55.9505952646837));
#133551=CARTESIAN_POINT('Ctrl Pts',(-57.9585693859923,-20.0319506515215,
-55.5325899309841));
#133552=CARTESIAN_POINT('Ctrl Pts',(-57.9099424206244,-20.4307035336697,
-55.7218311799895));
#133553=CARTESIAN_POINT('Ctrl Pts',(-58.337292873758,-20.5363048245876,
-55.740436199424));
#133554=CARTESIAN_POINT('Ctrl Pts',(-57.9502161720285,-20.1005973934661,
-55.4004673410398));
#133555=CARTESIAN_POINT('Ctrl Pts',(-57.9064615881784,-20.4555454071529,
-55.6247135460827));
#133556=CARTESIAN_POINT('Ctrl Pts',(-58.3079048908359,-20.5709315394046,
-55.6609486926888));
#133557=CARTESIAN_POINT('Ctrl Pts',(-57.9331286547812,-20.2376361665866,
-55.2282616560402));
#133558=CARTESIAN_POINT('Ctrl Pts',(-57.897198940496,-20.5238155454433,
-55.4956413947157));
#133559=CARTESIAN_POINT('Ctrl Pts',(-58.2667283591981,-20.6400407226598,
-55.5584509242662));
#133560=CARTESIAN_POINT('Ctrl Pts',(-57.9265619920107,-20.2898468150981,
-55.1744487967193));
#133561=CARTESIAN_POINT('Ctrl Pts',(-57.8934360858788,-20.5517279947688,
-55.4549818870893));
#133562=CARTESIAN_POINT('Ctrl Pts',(-58.2532825451019,-20.6663690401879,
-55.5266431857194));
#133563=CARTESIAN_POINT('Ctrl Pts',(-57.9122860844342,-20.4019110441904,
-55.0807659948788));
#133564=CARTESIAN_POINT('Ctrl Pts',(-57.8849186400004,-20.6149205916457,
-55.3834750893986));
#133565=CARTESIAN_POINT('Ctrl Pts',(-58.2280408271646,-20.7228767370785,
-55.4713148466751));
#133566=CARTESIAN_POINT('Ctrl Pts',(-57.9045197753069,-20.4622337862451,
-55.0401096877444));
#133567=CARTESIAN_POINT('Ctrl Pts',(-57.8801386015543,-20.6503866910324,
-55.3518324750308));
#133568=CARTESIAN_POINT('Ctrl Pts',(-58.2160717164706,-20.753292731466,
-55.4473281588797));
#133569=CARTESIAN_POINT('Ctrl Pts',(-57.8723006909993,-20.7089850131959,
-54.9109039511417));
#133570=CARTESIAN_POINT('Ctrl Pts',(-57.8601439921696,-20.7981658738856,
-55.250541365782));
#133571=CARTESIAN_POINT('Ctrl Pts',(-58.1723605376483,-20.8777067919942,
-55.3705177858243));
#133572=CARTESIAN_POINT('Ctrl Pts',(-57.8438584328939,-20.9197294286556,
-54.8734589342148));
#133573=CARTESIAN_POINT('Ctrl Pts',(-57.8415274164302,-20.9345476815752,
-55.214451085197));
#133574=CARTESIAN_POINT('Ctrl Pts',(-58.145173752928,-20.9839602690723,
-55.346687116762));
#133575=CARTESIAN_POINT('Ctrl Pts',(-57.8147273601029,-21.1255768370871,
-54.9117960309513));
#133576=CARTESIAN_POINT('Ctrl Pts',(-57.8228292490717,-21.0682703109648,
-55.236394534989));
#133577=CARTESIAN_POINT('Ctrl Pts',(-58.1259919089073,-21.0877309864276,
-55.3639580518367));
#133578=CARTESIAN_POINT('',(-58.4684744114517,-20.4800000236652,-56.1088024963483));
#133579=CARTESIAN_POINT('Origin',(-58.4684744114614,-19.98000002,-56.108802496345));
#133580=CARTESIAN_POINT('Ctrl Pts',(-58.4684744114466,-20.4800000273303,
-56.1088024963493));
#133581=CARTESIAN_POINT('Ctrl Pts',(-58.4560594229943,-20.4800036500033,
-56.0736749117289));
#133582=CARTESIAN_POINT('Ctrl Pts',(-58.4439350613241,-20.4813472561768,
-56.0394507359076));
#133583=CARTESIAN_POINT('Ctrl Pts',(-58.4320811979818,-20.4840487563327,
-56.0060462075256));
#133584=CARTESIAN_POINT('Ctrl Pts',(-58.421086555275,-20.4865544397651,
-55.9750629876465));
#133585=CARTESIAN_POINT('Ctrl Pts',(-58.4103249292896,-20.4902278471488,
-55.9447835971118));
#133586=CARTESIAN_POINT('Ctrl Pts',(-58.3997538039955,-20.4951176237352,
-55.9151358942012));
#133587=CARTESIAN_POINT('Ctrl Pts',(-58.3897209301719,-20.4997584268807,
-55.8869977675415));
#133588=CARTESIAN_POINT('Ctrl Pts',(-58.3798599201571,-20.5054949994344,
-55.8594274183296));
#133589=CARTESIAN_POINT('Ctrl Pts',(-58.3701054711661,-20.5124031604037,
-55.8323759729964));
#133590=CARTESIAN_POINT('Ctrl Pts',(-58.369582156849,-20.5127737748324,
-55.8309246958763));
#133591=CARTESIAN_POINT('Ctrl Pts',(-58.3690591414204,-20.5131477694283,
-55.8294749181168));
#133592=CARTESIAN_POINT('Ctrl Pts',(-58.3685364120709,-20.5135251586298,
-55.8280266343692));
#133593=CARTESIAN_POINT('Ctrl Pts',(-58.355322598113,-20.5230649916293,
-55.7914161933879));
#133594=CARTESIAN_POINT('Ctrl Pts',(-58.3424819682759,-20.5346544306425,
-55.7562349549661));
#133595=CARTESIAN_POINT('Ctrl Pts',(-58.3300197127882,-20.5482894757852,
-55.7226770371038));
#133596=CARTESIAN_POINT('Ctrl Pts',(-58.3189876225659,-20.5603597666202,
-55.6929702173479));
#133597=CARTESIAN_POINT('Ctrl Pts',(-58.3082519351362,-20.5740337277965,
-55.6645352898577));
#133598=CARTESIAN_POINT('Ctrl Pts',(-58.297793069529,-20.5892884176472,
-55.6375339573335));
#133599=CARTESIAN_POINT('Ctrl Pts',(-58.2918114955221,-20.5980127917543,
-55.622091511198));
#133600=CARTESIAN_POINT('Ctrl Pts',(-58.2859200261619,-20.6072537934279,
-55.6071185210319));
#133601=CARTESIAN_POINT('Ctrl Pts',(-58.2801113530785,-20.6170020227668,
-55.5926500177757));
#133602=CARTESIAN_POINT('Ctrl Pts',(-58.2739672932451,-20.6273131047414,
-55.5773461181711));
#133603=CARTESIAN_POINT('Ctrl Pts',(-58.2678869023947,-20.638271485625,
-55.562504370203));
#133604=CARTESIAN_POINT('Ctrl Pts',(-58.2619058079972,-20.6497784634518,
-55.5483031281744));
#133605=CARTESIAN_POINT('Ctrl Pts',(-58.2559442889337,-20.6612477804562,
-55.5341483649398));
#133606=CARTESIAN_POINT('Ctrl Pts',(-58.2500813442384,-20.6732615002889,
-55.5206307132331));
#133607=CARTESIAN_POINT('Ctrl Pts',(-58.2443734669305,-20.6856843380992,
-55.5078979452598));
#133608=CARTESIAN_POINT('Ctrl Pts',(-58.2430208618868,-20.6886281983423,
-55.5048806403578));
#133609=CARTESIAN_POINT('Ctrl Pts',(-58.2416770603513,-20.6915948918065,
-55.5019072550467));
#133610=CARTESIAN_POINT('Ctrl Pts',(-58.2403429914197,-20.6945823753937,
-55.4989794498912));
#133611=CARTESIAN_POINT('Ctrl Pts',(-58.2336464050011,-20.7095785585306,
-55.4842828328155));
#133612=CARTESIAN_POINT('Ctrl Pts',(-58.2271276542843,-20.7251842455087,
-55.4706315466689));
#133613=CARTESIAN_POINT('Ctrl Pts',(-58.2207713165789,-20.7414257608518,
-55.4580213750816));
#133614=CARTESIAN_POINT('Ctrl Pts',(-58.2151565865895,-20.7557723433489,
-55.4468824595826));
#133615=CARTESIAN_POINT('Ctrl Pts',(-58.2096680821563,-20.7706159767222,
-55.4365563660369));
#133616=CARTESIAN_POINT('Ctrl Pts',(-58.2042768588887,-20.7859705675371,
-55.4270685753685));
#133617=CARTESIAN_POINT('Ctrl Pts',(-58.1969328174058,-20.8068869247906,
-55.4141441007564));
#133618=CARTESIAN_POINT('Ctrl Pts',(-58.1898412601343,-20.828523501731,
-55.40291734747));
#133619=CARTESIAN_POINT('Ctrl Pts',(-58.1830505367822,-20.8507355057842,
-55.3934981904853));
#133620=CARTESIAN_POINT('Ctrl Pts',(-58.1765582690219,-20.871971281464,
-55.3844930100279));
#133621=CARTESIAN_POINT('Ctrl Pts',(-58.1703405182628,-20.8937334832869,
-55.3771411838376));
#133622=CARTESIAN_POINT('Ctrl Pts',(-58.164427550618,-20.9158503556191,
-55.3715356173205));
#133623=CARTESIAN_POINT('Ctrl Pts',(-58.1587702929555,-20.937010769981,
-55.3661724670316));
#133624=CARTESIAN_POINT('Ctrl Pts',(-58.1533916071063,-20.9584955938527,
-55.3624089485159));
#133625=CARTESIAN_POINT('Ctrl Pts',(-58.1483130703003,-20.9801107627175,
-55.3603068684826));
#133626=CARTESIAN_POINT('Ctrl Pts',(-58.1468720340706,-20.9862440728885,
-55.3597104026891));
#133627=CARTESIAN_POINT('Ctrl Pts',(-58.1454551536744,-20.9923876162956,
-55.3592475231078));
#133628=CARTESIAN_POINT('Ctrl Pts',(-58.1440629164629,-20.9985363600311,
-55.358919141335));
#133629=CARTESIAN_POINT('Origin',(-58.4684744114614,-19.98000002,-55.24995));
#133630=CARTESIAN_POINT('',(-58.4684744114614,-20.48000002,-60.42825533736));
#133631=CARTESIAN_POINT('Origin',(-58.4684744114614,-19.98000002,-60.42825533736));
#133632=CARTESIAN_POINT('',(-58.4684744114614,-20.48000002,-55.24995));
#133633=CARTESIAN_POINT('Origin',(0.,-12.9675000200281,-60.42825533736));
#133634=CARTESIAN_POINT('',(-58.2781275348581,-14.3194901627709,-60.8508735991007));
#133635=CARTESIAN_POINT('',(-57.8770125754992,-19.9259080025173,-60.8508735991007));
#133636=CARTESIAN_POINT('Origin',(0.,-12.9675000200281,-60.8508735991007));
#133637=CARTESIAN_POINT('Origin',(-56.5152414274053,-20.0041958453797,-60.331554578498));
#133638=CARTESIAN_POINT('Origin',(-57.3724390589806,-14.3298873277334,-60.4282477713549));
#133639=CARTESIAN_POINT('Origin',(-58.871735578318,-14.33000002,-55.24995));
#133640=CARTESIAN_POINT('',(-58.871735578318,-13.83000002,-60.42825533736));
#133641=CARTESIAN_POINT('Origin',(-58.871735578318,-14.33000002,-60.42825533736));
#133642=CARTESIAN_POINT('',(-58.871735578318,-13.83000002,-56.2531111209796));
#133643=CARTESIAN_POINT('Origin',(-58.871735578318,-14.33000002,-56.2531111209796));
#133644=CARTESIAN_POINT('',(-58.871735578318,-13.83000002,-55.24995));
#133645=CARTESIAN_POINT('Ctrl Pts',(-58.3870336823786,-13.1950672036472,
-54.9735905576542));
#133646=CARTESIAN_POINT('Ctrl Pts',(-58.386666124584,-13.2389284460928,
-55.245469113786));
#133647=CARTESIAN_POINT('Ctrl Pts',(-58.6192838059339,-13.2635419343739,
-55.3905548168058));
#133648=CARTESIAN_POINT('Ctrl Pts',(-58.3863638568524,-13.3879941755922,
-54.9394842857217));
#133649=CARTESIAN_POINT('Ctrl Pts',(-58.3860638311514,-13.3687276186212,
-55.2176214035434));
#133650=CARTESIAN_POINT('Ctrl Pts',(-58.613439068509,-13.3607847257335,
-55.3701021803697));
#133651=CARTESIAN_POINT('Ctrl Pts',(-58.3844076455848,-13.5917447402541,
-54.9813451387709));
#133652=CARTESIAN_POINT('Ctrl Pts',(-58.3849151617365,-13.5088631788445,
-55.251799877981));
#133653=CARTESIAN_POINT('Ctrl Pts',(-58.6183088754593,-13.4634772759073,
-55.3945154239426));
#133654=CARTESIAN_POINT('Ctrl Pts',(-58.3803446492905,-13.8907806579908,
-55.1547248800286));
#133655=CARTESIAN_POINT('Ctrl Pts',(-58.3829868535489,-13.7025366763559,
-55.3887548371216));
#133656=CARTESIAN_POINT('Ctrl Pts',(-58.6446085400692,-13.614195445683,
-55.5000130596728));
#133657=CARTESIAN_POINT('Ctrl Pts',(-58.3784003210709,-14.0018139117568,
-55.2630289365479));
#133658=CARTESIAN_POINT('Ctrl Pts',(-58.3821831638283,-13.7708280924458,
-55.4756863263615));
#133659=CARTESIAN_POINT('Ctrl Pts',(-58.6620402598172,-13.6701578227605,
-55.566624268873));
#133660=CARTESIAN_POINT('Ctrl Pts',(-58.3751346753983,-14.1721093492982,
-55.5158238508396));
#133661=CARTESIAN_POINT('Ctrl Pts',(-58.3811829168127,-13.8615332852492,
-55.675485688548));
#133662=CARTESIAN_POINT('Ctrl Pts',(-58.7077104063222,-13.7559878496911,
-55.7281943165199));
#133663=CARTESIAN_POINT('Ctrl Pts',(-58.3738439529203,-14.2307758203948,
-55.6580834410202));
#133664=CARTESIAN_POINT('Ctrl Pts',(-58.3810074666823,-13.8830868568037,
-55.788873845676));
#133665=CARTESIAN_POINT('Ctrl Pts',(-58.7356377641522,-13.7855551979282,
-55.8218169965321));
#133666=CARTESIAN_POINT('Ctrl Pts',(-58.371968604942,-14.3149917907957,
-55.9950091948521));
#133667=CARTESIAN_POINT('Ctrl Pts',(-58.3813969201454,-13.8862626584142,
-56.0560043903553));
#133668=CARTESIAN_POINT('Ctrl Pts',(-58.8084294771009,-13.8279974118869,
-56.0558032453046));
#133669=CARTESIAN_POINT('Ctrl Pts',(-58.371685997399,-14.3259563616536,
-56.1910588010128));
#133670=CARTESIAN_POINT('Ctrl Pts',(-58.3822444492649,-13.8506911564217,
-56.212199449184));
#133671=CARTESIAN_POINT('Ctrl Pts',(-58.855449162814,-13.8335191345168,
-56.2004791098763));
#133672=CARTESIAN_POINT('Ctrl Pts',(-58.3719493412616,-14.3151650612744,
-56.3903791996399));
#133673=CARTESIAN_POINT('Ctrl Pts',(-58.3834300043284,-13.791901460541,
-56.360880747514));
#133674=CARTESIAN_POINT('Ctrl Pts',(-58.9064235376792,-13.8280751907923,
-56.3623652529328));
#133675=CARTESIAN_POINT('',(-58.6168863951182,-13.3313694067285,-55.3834094543327));
#133676=CARTESIAN_POINT('Origin',(-58.8863673263393,-13.3327387922841,-54.9622468511542));
#133677=CARTESIAN_POINT('Ctrl Pts',(-58.6168867413708,-13.3313694084883,
-55.383408913088));
#133678=CARTESIAN_POINT('Ctrl Pts',(-58.6166911469594,-13.3517892137721,
-55.3833501769659));
#133679=CARTESIAN_POINT('Ctrl Pts',(-58.6169551454442,-13.3722412722744,
-55.3850753059523));
#133680=CARTESIAN_POINT('Ctrl Pts',(-58.6176634841287,-13.3924918963401,
-55.3885601063615));
#133681=CARTESIAN_POINT('Ctrl Pts',(-58.6183725932892,-13.4127645474659,
-55.3920486972666));
#133682=CARTESIAN_POINT('Ctrl Pts',(-58.6195270688617,-13.4328341668126,
-55.3973004085694));
#133683=CARTESIAN_POINT('Ctrl Pts',(-58.6211188739901,-13.4524818769443,
-55.4042414350838));
#133684=CARTESIAN_POINT('Ctrl Pts',(-58.6227236599655,-13.4722898101543,
-55.4112390642571));
#133685=CARTESIAN_POINT('Ctrl Pts',(-58.6247730789981,-13.4916679682566,
-55.4199529583737));
#133686=CARTESIAN_POINT('Ctrl Pts',(-58.627264754533,-13.5104240755455,
-55.4302654575736));
#133687=CARTESIAN_POINT('Ctrl Pts',(-58.6290008545194,-13.5234925819195,
-55.4374507950986));
#133688=CARTESIAN_POINT('Ctrl Pts',(-58.6309517906365,-13.536259812243,
-55.4454112967302));
#133689=CARTESIAN_POINT('Ctrl Pts',(-58.6331177534659,-13.548672905394,
-55.4540985105411));
#133690=CARTESIAN_POINT('Ctrl Pts',(-58.6364466735685,-13.567750885295,
-55.4674500973265));
#133691=CARTESIAN_POINT('Ctrl Pts',(-58.6402780389743,-13.5860620622833,
-55.4825567103882));
#133692=CARTESIAN_POINT('Ctrl Pts',(-58.6446041270825,-13.6034603706004,
-55.499260499199));
#133693=CARTESIAN_POINT('Ctrl Pts',(-58.6489851274684,-13.6210795206375,
-55.5161763139942));
#133694=CARTESIAN_POINT('Ctrl Pts',(-58.6538736776085,-13.6377624792879,
-55.5347290400659));
#133695=CARTESIAN_POINT('Ctrl Pts',(-58.6592563987165,-13.6534107023946,
-55.5547469245073));
#133696=CARTESIAN_POINT('Ctrl Pts',(-58.6647747031922,-13.6694530827954,
-55.5752690320232));
#133697=CARTESIAN_POINT('Ctrl Pts',(-58.670812549364,-13.6844082085566,
-55.5973300534321));
#133698=CARTESIAN_POINT('Ctrl Pts',(-58.6773471776121,-13.6982235274118,
-55.6207527017991));
#133699=CARTESIAN_POINT('Ctrl Pts',(-58.6797711272743,-13.7033481704979,
-55.629441079843));
#133700=CARTESIAN_POINT('Ctrl Pts',(-58.6822633392963,-13.7083164773331,
-55.6383169613905));
#133701=CARTESIAN_POINT('Ctrl Pts',(-58.6848223131132,-13.7131274153225,
-55.6473719395789));
#133702=CARTESIAN_POINT('Ctrl Pts',(-58.6917189083808,-13.7260931955708,
-55.6717756749011));
#133703=CARTESIAN_POINT('Ctrl Pts',(-58.6990713849487,-13.7378634833018,
-55.697382248317));
#133704=CARTESIAN_POINT('Ctrl Pts',(-58.706853591563,-13.7484649343429,
-55.7240191465997));
#133705=CARTESIAN_POINT('Ctrl Pts',(-58.7148369504267,-13.7593404086564,
-55.7513445478056));
#133706=CARTESIAN_POINT('Ctrl Pts',(-58.7232726197845,-13.7689867245339,
-55.7797537951109));
#133707=CARTESIAN_POINT('Ctrl Pts',(-58.7321217354356,-13.7774700892654,
-55.8091004361974));
#133708=CARTESIAN_POINT('Ctrl Pts',(-58.7413560701509,-13.7863227512184,
-55.8397245931469));
#133709=CARTESIAN_POINT('Ctrl Pts',(-58.7510406560465,-13.7939099084487,
-55.8713692899863));
#133710=CARTESIAN_POINT('Ctrl Pts',(-58.7611190114348,-13.8003330673419,
-55.9039164111607));
#133711=CARTESIAN_POINT('Ctrl Pts',(-58.7631356097838,-13.8016182900911,
-55.9104288299332));
#133712=CARTESIAN_POINT('Ctrl Pts',(-58.7651679353576,-13.802856965918,
-55.9169775323731));
#133713=CARTESIAN_POINT('Ctrl Pts',(-58.7672154801736,-13.804049979403,
-55.9235617984596));
#133714=CARTESIAN_POINT('Ctrl Pts',(-58.7772438220828,-13.80989304913,-55.955809821077));
#133715=CARTESIAN_POINT('Ctrl Pts',(-58.787591444619,-13.8146310037254,
-55.9888239184914));
#133716=CARTESIAN_POINT('Ctrl Pts',(-58.7982713308712,-13.8183831216517,
-56.0226328969941));
#133717=CARTESIAN_POINT('Ctrl Pts',(-58.8094011606195,-13.8222933162669,
-56.057866247407));
#133718=CARTESIAN_POINT('Ctrl Pts',(-58.8208917803897,-13.8251334049964,
-56.0939631676213));
#133719=CARTESIAN_POINT('Ctrl Pts',(-58.8327267583728,-13.8270283739072,
-56.1310025459061));
#133720=CARTESIAN_POINT('Ctrl Pts',(-58.8368443754292,-13.8276876701324,
-56.1438892598484));
#133721=CARTESIAN_POINT('Ctrl Pts',(-58.841003414625,-13.828232439654,-56.1568904311276));
#133722=CARTESIAN_POINT('Ctrl Pts',(-58.8452023822018,-13.8286675259685,
-56.1700105135303));
#133723=CARTESIAN_POINT('Ctrl Pts',(-58.8538987623764,-13.8295686227095,
-56.197183198818));
#133724=CARTESIAN_POINT('Ctrl Pts',(-58.8627548931133,-13.829999537714,
-56.2248738007663));
#133725=CARTESIAN_POINT('Ctrl Pts',(-58.871735578318,-13.8300000195957,
-56.2531111209796));
#133726=CARTESIAN_POINT('Ctrl Pts',(-58.3873384184922,-12.8301367871357,
-54.9623589764042));
#133727=CARTESIAN_POINT('Ctrl Pts',(-58.3873382434228,-12.8300623725117,
-55.2359199480943));
#133728=CARTESIAN_POINT('Ctrl Pts',(-58.6177174583935,-12.8294802501408,
-55.3834349955049));
#133729=CARTESIAN_POINT('Ctrl Pts',(-58.3877301336919,-12.9966384589807,
-54.9624046566442));
#133730=CARTESIAN_POINT('Ctrl Pts',(-58.3877303689833,-12.9966482737696,
-55.2359230050537));
#133731=CARTESIAN_POINT('Ctrl Pts',(-58.6180560895148,-12.9967778686954,
-55.3834453150663));
#133732=CARTESIAN_POINT('Ctrl Pts',(-58.3874096419063,-13.1631387418538,
-54.9623672844226));
#133733=CARTESIAN_POINT('Ctrl Pts',(-58.387409446605,-13.1632604597673,
-55.2359205047867));
#133734=CARTESIAN_POINT('Ctrl Pts',(-58.6177790296338,-13.16407332507,-55.3834369074594));
#133735=CARTESIAN_POINT('Ctrl Pts',(-58.3863769436068,-13.3296376352283,
-54.9622468511542));
#133736=CARTESIAN_POINT('Ctrl Pts',(-58.3863757263072,-13.3298338968435,
-55.2359124429054));
#133737=CARTESIAN_POINT('Ctrl Pts',(-58.6168862797201,-13.3313694061415,
-55.3834096347601));
#133738=CARTESIAN_POINT('',(-58.6177175690985,-12.8294802499273,-55.3834348225703));
#133739=CARTESIAN_POINT('Origin',(-58.8873370347925,-12.8289604802815,-54.9623589764042));
#133740=CARTESIAN_POINT('Origin',(9.50671311766895,-12.9674995491444,-53.303688922601));
#133741=CARTESIAN_POINT('Ctrl Pts',(-58.3767309587969,-11.8448446071682,
-56.4122977393942));
#133742=CARTESIAN_POINT('Ctrl Pts',(-58.3869014365542,-12.3742451521447,
-56.3787762146875));
#133743=CARTESIAN_POINT('Ctrl Pts',(-58.9159388499761,-12.33260651506,-56.3821256036996));
#133744=CARTESIAN_POINT('Ctrl Pts',(-58.3761594576374,-11.8217613269723,
-56.0640428959811));
#133745=CARTESIAN_POINT('Ctrl Pts',(-58.3850096805969,-12.2694751488998,
-56.131480723907));
#133746=CARTESIAN_POINT('Ctrl Pts',(-58.8249733980819,-12.3209870158311,
-56.0943527415187));
#133747=CARTESIAN_POINT('Ctrl Pts',(-58.3775636494613,-11.8719586819063,
-55.6887790791007));
#133748=CARTESIAN_POINT('Ctrl Pts',(-58.3840763820856,-12.2332797983991,
-55.8207298766612));
#133749=CARTESIAN_POINT('Ctrl Pts',(-58.7426223732974,-12.3463167916318,
-55.8395053228666));
#133750=CARTESIAN_POINT('Ctrl Pts',(-58.3812857230693,-12.1145902249729,
-55.3279498195379));
#133751=CARTESIAN_POINT('Ctrl Pts',(-58.3849523847638,-12.3664682018911,
-55.5261704685903));
#133752=CARTESIAN_POINT('Ctrl Pts',(-58.6766505662879,-12.4686699842847,
-55.6084539884381));
#133753=CARTESIAN_POINT('Ctrl Pts',(-58.3819811265814,-12.1628909733764,
-55.2698289416564));
#133754=CARTESIAN_POINT('Ctrl Pts',(-58.3851526533159,-12.3943556730011,
-55.4799801456162));
#133755=CARTESIAN_POINT('Ctrl Pts',(-58.6665193417984,-12.4930264323153,
-55.5718937149656));
#133756=CARTESIAN_POINT('Ctrl Pts',(-58.3833791647681,-12.2716887773838,
-55.165249378439));
#133757=CARTESIAN_POINT('Ctrl Pts',(-58.3856109002795,-12.4605296876876,
-55.3971016982864));
#133758=CARTESIAN_POINT('Ctrl Pts',(-58.6488938487369,-12.5478884692595,
-55.5067940385222));
#133759=CARTESIAN_POINT('Ctrl Pts',(-58.3840891453349,-12.3330632532853,
-55.1184352970832));
#133760=CARTESIAN_POINT('Ctrl Pts',(-58.3858723799976,-12.4994236383624,
-55.3598423864862));
#133761=CARTESIAN_POINT('Ctrl Pts',(-58.6413490671682,-12.5788364831875,
-55.4780465670558));
#133762=CARTESIAN_POINT('Ctrl Pts',(-58.3864241277835,-12.5724501016325,
-54.9791144036392));
#133763=CARTESIAN_POINT('Ctrl Pts',(-58.3867921906799,-12.6537459867802,
-55.2500592167191));
#133764=CARTESIAN_POINT('Ctrl Pts',(-58.6194845317821,-12.6995460488039,
-55.3930474481988));
#133765=CARTESIAN_POINT('Ctrl Pts',(-58.3876249629302,-12.7822769116689,
-54.9368955558876));
#133766=CARTESIAN_POINT('Ctrl Pts',(-58.3874149873687,-12.798358027374,
-55.2152912072037));
#133767=CARTESIAN_POINT('Ctrl Pts',(-58.6140349181668,-12.8053471169491,
-55.3683568445872));
#133768=CARTESIAN_POINT('Ctrl Pts',(-58.3874714544294,-12.9876188791411,
-54.9778741910769));
#133769=CARTESIAN_POINT('Ctrl Pts',(-58.3874999658154,-12.9364675110246,
-55.2486081571874));
#133770=CARTESIAN_POINT('Ctrl Pts',(-58.6203209684042,-12.9088882648831,
-55.3927678988426));
#133771=CARTESIAN_POINT('',(-58.8765127194368,-12.33000002,-56.2580153373943));
#133772=CARTESIAN_POINT('Origin',(-58.8765127194474,-11.83000002,-56.2580153373923));
#133773=CARTESIAN_POINT('Ctrl Pts',(-58.8765127194368,-12.330000020523,
-56.2580153373943));
#133774=CARTESIAN_POINT('Ctrl Pts',(-58.8668469571914,-12.3300006089033,
-56.2275462744181));
#133775=CARTESIAN_POINT('Ctrl Pts',(-58.8572724827484,-12.3304973506903,
-56.1976030412555));
#133776=CARTESIAN_POINT('Ctrl Pts',(-58.8478488263232,-12.3315471370039,
-56.1681943340671));
#133777=CARTESIAN_POINT('Ctrl Pts',(-58.8351276172195,-12.3329642675325,
-56.1284948483541));
#133778=CARTESIAN_POINT('Ctrl Pts',(-58.8227077416393,-12.3353891641161,
-56.0897498595506));
#133779=CARTESIAN_POINT('Ctrl Pts',(-58.8106737837062,-12.3389698977987,
-56.0519640291567));
#133780=CARTESIAN_POINT('Ctrl Pts',(-58.798585967488,-12.3425666571462,
-56.0140090873166));
#133781=CARTESIAN_POINT('Ctrl Pts',(-58.7868877399643,-12.3473304320438,
-55.9770211857099));
#133782=CARTESIAN_POINT('Ctrl Pts',(-58.7756496355396,-12.3534118638669,
-55.9410597318365));
#133783=CARTESIAN_POINT('Ctrl Pts',(-58.7654551148452,-12.3589285667047,
-55.9084377013004));
#133784=CARTESIAN_POINT('Ctrl Pts',(-58.7556391095688,-12.3655302748636,
-55.8766607416699));
#133785=CARTESIAN_POINT('Ctrl Pts',(-58.7462416806977,-12.3733192924399,
-55.8458185837666));
#133786=CARTESIAN_POINT('Ctrl Pts',(-58.7370890065606,-12.3809054461317,
-55.8157797055964));
#133787=CARTESIAN_POINT('Ctrl Pts',(-58.7283333473674,-12.3896186806531,
-55.7866276816044));
#133788=CARTESIAN_POINT('Ctrl Pts',(-58.7200001112973,-12.3995324607904,
-55.7584877378961));
#133789=CARTESIAN_POINT('Ctrl Pts',(-58.7119333700456,-12.4091292007029,
-55.7312477025938));
#133790=CARTESIAN_POINT('Ctrl Pts',(-58.7042623453504,-12.4198516550861,
-55.7049564664655));
#133791=CARTESIAN_POINT('Ctrl Pts',(-58.6970002769998,-12.4317352917216,
-55.679763891269));
#133792=CARTESIAN_POINT('Ctrl Pts',(-58.693993662897,-12.4366553100656,
-55.6693337564626));
#133793=CARTESIAN_POINT('Ctrl Pts',(-58.6910570395936,-12.4417739272228,
-55.6590923450502));
#133794=CARTESIAN_POINT('Ctrl Pts',(-58.688190921677,-12.4470915758791,
-55.6490518746812));
#133795=CARTESIAN_POINT('Ctrl Pts',(-58.6819688096681,-12.4586357644038,
-55.6272548191955));
#133796=CARTESIAN_POINT('Ctrl Pts',(-58.676161566562,-12.4709976964519,
-55.6066383301269));
#133797=CARTESIAN_POINT('Ctrl Pts',(-58.6707625823114,-12.4842111874128,
-55.5871773541376));
#133798=CARTESIAN_POINT('Ctrl Pts',(-58.6660950833367,-12.4956344390189,
-55.570353062519));
#133799=CARTESIAN_POINT('Ctrl Pts',(-58.6617321827839,-12.5076948684914,
-55.5543925885353));
#133800=CARTESIAN_POINT('Ctrl Pts',(-58.6576458797968,-12.5204167509595,
-55.5393004504467));
#133801=CARTESIAN_POINT('Ctrl Pts',(-58.6538203633614,-12.5323267269511,
-55.5251714877913));
#133802=CARTESIAN_POINT('Ctrl Pts',(-58.6502422277945,-12.5448868051958,
-55.5117483046152));
#133803=CARTESIAN_POINT('Ctrl Pts',(-58.6469241897868,-12.5579798460549,
-55.4992040857469));
#133804=CARTESIAN_POINT('Ctrl Pts',(-58.6436008912601,-12.5710936450212,
-55.4866399788907));
#133805=CARTESIAN_POINT('Ctrl Pts',(-58.640538399124,-12.5847413788212,
-55.4749584070027));
#133806=CARTESIAN_POINT('Ctrl Pts',(-58.6377735166986,-12.5987697559786,
-55.4643034363389));
#133807=CARTESIAN_POINT('Ctrl Pts',(-58.636939408858,-12.6030018272128,
-55.4610890520705));
#133808=CARTESIAN_POINT('Ctrl Pts',(-58.6361325568626,-12.6072683399031,
-55.4579678510716));
#133809=CARTESIAN_POINT('Ctrl Pts',(-58.6353544099234,-12.6115646261654,
-55.4549431101388));
#133810=CARTESIAN_POINT('Ctrl Pts',(-58.6319384747262,-12.6304246058457,
-55.4416650022455));
#133811=CARTESIAN_POINT('Ctrl Pts',(-58.6289958183114,-12.6500604145187,
-55.4300757823933));
#133812=CARTESIAN_POINT('Ctrl Pts',(-58.6265511922013,-12.6703334806547,
-55.4203199554195));
#133813=CARTESIAN_POINT('Ctrl Pts',(-58.6241562833628,-12.6901942458945,
-55.4107625363323));
#133814=CARTESIAN_POINT('Ctrl Pts',(-58.6222390524072,-12.7106665739421,
-55.4029656961182));
#133815=CARTESIAN_POINT('Ctrl Pts',(-58.6208117373686,-12.7315745389804,
-55.3970503586626));
#133816=CARTESIAN_POINT('Ctrl Pts',(-58.6194133085358,-12.7520593656347,
-55.3912547366517));
#133817=CARTESIAN_POINT('Ctrl Pts',(-58.6184848265338,-12.77296187318,-55.387266165696));
#133818=CARTESIAN_POINT('Ctrl Pts',(-58.6180318547009,-12.7940763452495,
-55.3851695450414));
#133819=CARTESIAN_POINT('Ctrl Pts',(-58.6177797881602,-12.805825976342,
-55.3840028325064));
#133820=CARTESIAN_POINT('Ctrl Pts',(-58.6176748911857,-12.8176405504773,
-55.3834213832906));
#133821=CARTESIAN_POINT('Ctrl Pts',(-58.617717901229,-12.8294802492869,
-55.3834343037763));
#133822=CARTESIAN_POINT('Origin',(-58.8765127194474,-11.83000002,-55.24995));
#133823=CARTESIAN_POINT('',(-58.8765127194474,-12.33000002,-60.42825533736));
#133824=CARTESIAN_POINT('Origin',(-58.8765127194474,-11.83000002,-60.42825533736));
#133825=CARTESIAN_POINT('',(-58.8765127194474,-12.33000002,-55.24995));
#133826=CARTESIAN_POINT('Origin',(0.,-12.9675000200281,-60.42825533736));
#133827=CARTESIAN_POINT('',(-57.9034184448965,-6.23235646472971,-60.8508735991007));
#133828=CARTESIAN_POINT('',(-58.2828791719688,-11.838774304476,-60.8508735991007));
#133829=CARTESIAN_POINT('Origin',(0.,-12.9675000200281,-60.8508735991007));
#133830=CARTESIAN_POINT('Origin',(-57.3770031434005,-11.8300849588959,-60.4282500608777));
#133831=CARTESIAN_POINT('Origin',(-56.5400850853955,-6.15642395592187,-60.3303328953569));
#133832=CARTESIAN_POINT('Origin',(-58.4950211556756,-6.18000001999999,-55.24995));
#133833=CARTESIAN_POINT('',(-58.4950211556756,-5.68000001999999,-60.42825533736));
#133834=CARTESIAN_POINT('Origin',(-58.4950211556756,-6.18000001999999,-60.42825533736));
#133835=CARTESIAN_POINT('',(-58.4950211556755,-5.6800000188644,-56.1192785199307));
#133836=CARTESIAN_POINT('Origin',(-58.4950211556756,-6.18000001999999,-56.1192785199305));
#133837=CARTESIAN_POINT('',(-58.4950211556756,-5.68000001999999,-55.24995));
#133838=CARTESIAN_POINT('Ctrl Pts',(-57.8697476022663,-5.20911947359449,
-54.9007953984755));
#133839=CARTESIAN_POINT('Ctrl Pts',(-57.8690388195133,-5.20383266421795,
-55.2313599550619));
#133840=CARTESIAN_POINT('Ctrl Pts',(-58.1702690071154,-5.16134039100007,
-55.3608055405082));
#133841=CARTESIAN_POINT('Ctrl Pts',(-57.8892576239528,-5.35464469293038,
-54.9031849800101));
#133842=CARTESIAN_POINT('Ctrl Pts',(-57.8816711167897,-5.29795553030126,
-55.2377699288152));
#133843=CARTESIAN_POINT('Ctrl Pts',(-58.1863681399526,-5.2347113163298,
-55.3646554087878));
#133844=CARTESIAN_POINT('Ctrl Pts',(-57.9082088324435,-5.50047055831863,
-54.9417550134773));
#133845=CARTESIAN_POINT('Ctrl Pts',(-57.8939857420187,-5.39104663027327,
-55.2713483619941));
#133846=CARTESIAN_POINT('Ctrl Pts',(-58.206532806921,-5.30826342386473,
-55.3884755439432));
#133847=CARTESIAN_POINT('Ctrl Pts',(-57.9410017896518,-5.75934555612452,
-55.0773466647676));
#133848=CARTESIAN_POINT('Ctrl Pts',(-57.9146461968408,-5.54837256073304,
-55.3788933751119));
#133849=CARTESIAN_POINT('Ctrl Pts',(-58.2517768983759,-5.43880935502387,
-55.4693790307482));
#133850=CARTESIAN_POINT('Ctrl Pts',(-57.9551095363294,-5.87426883806545,
-55.1748695369358));
#133851=CARTESIAN_POINT('Ctrl Pts',(-57.9231956882672,-5.61406051834577,
-55.4547002829484));
#133852=CARTESIAN_POINT('Ctrl Pts',(-58.2772082041435,-5.49676306934017,
-55.5268083141558));
#133853=CARTESIAN_POINT('Ctrl Pts',(-57.9772132186836,-6.05726143051376,
-55.4055720426652));
#133854=CARTESIAN_POINT('Ctrl Pts',(-57.9351757774934,-5.70509939430376,
-55.6270222213536));
#133855=CARTESIAN_POINT('Ctrl Pts',(-58.3321412809957,-5.58904289089475,
-55.6647824032721));
#133856=CARTESIAN_POINT('Ctrl Pts',(-57.9853419314568,-6.12627634754757,
-55.5391049776385));
#133857=CARTESIAN_POINT('Ctrl Pts',(-57.9385982402169,-5.73028333208738,
-55.725786817627));
#133858=CARTESIAN_POINT('Ctrl Pts',(-58.3618432600141,-5.62384585378313,
-55.7455542887996));
#133859=CARTESIAN_POINT('Ctrl Pts',(-57.9959179918116,-6.21652108864807,
-55.822399360329));
#133860=CARTESIAN_POINT('Ctrl Pts',(-57.9401928503808,-5.73799842569994,
-55.9259333604635));
#133861=CARTESIAN_POINT('Ctrl Pts',(-58.4256102669737,-5.66935462867838,
-55.922812372103));
#133862=CARTESIAN_POINT('Ctrl Pts',(-57.9983536021903,-6.2376310994186,
-55.9707502487912));
#133863=CARTESIAN_POINT('Ctrl Pts',(-57.9381116944449,-5.71846326962232,
-56.0282143296093));
#133864=CARTESIAN_POINT('Ctrl Pts',(-58.4594118188676,-5.68000001999999,
-56.0184103401194));
#133865=CARTESIAN_POINT('Ctrl Pts',(-57.9983536018174,-6.23763109620483,
-56.1192785199305));
#133866=CARTESIAN_POINT('Ctrl Pts',(-57.9336485918015,-5.68000002,-56.1192785199305));
#133867=CARTESIAN_POINT('Ctrl Pts',(-58.4950211556756,-5.68000001999999,
-56.1192785199305));
#133868=CARTESIAN_POINT('',(-58.1702690070839,-5.16134039099922,-55.3608055404948));
#133869=CARTESIAN_POINT('Origin',(-58.3653138416346,-5.14268076199931,-54.9007953984755));
#133870=CARTESIAN_POINT('Ctrl Pts',(-58.1702690071152,-5.16134039100008,
-55.3608055405081));
#133871=CARTESIAN_POINT('Ctrl Pts',(-58.1863681399526,-5.2347113163298,
-55.3646554087878));
#133872=CARTESIAN_POINT('Ctrl Pts',(-58.206532806921,-5.30826342386473,
-55.3884755439432));
#133873=CARTESIAN_POINT('Ctrl Pts',(-58.2517768983759,-5.43880935502387,
-55.4693790307482));
#133874=CARTESIAN_POINT('Ctrl Pts',(-58.2772082041435,-5.49676306934017,
-55.5268083141558));
#133875=CARTESIAN_POINT('Ctrl Pts',(-58.3321412809957,-5.58904289089475,
-55.6647824032721));
#133876=CARTESIAN_POINT('Ctrl Pts',(-58.3618432600141,-5.62384585378313,
-55.7455542887996));
#133877=CARTESIAN_POINT('Ctrl Pts',(-58.4256102669737,-5.66935462867838,
-55.922812372103));
#133878=CARTESIAN_POINT('Ctrl Pts',(-58.4594118188676,-5.68000001999999,
-56.0184103401194));
#133879=CARTESIAN_POINT('Ctrl Pts',(-58.4950211556756,-5.68000001999999,
-56.1192785199305));
#133880=CARTESIAN_POINT('Ctrl Pts',(-57.8012193907063,-4.71406478367217,
-54.8923577774473));
#133881=CARTESIAN_POINT('Ctrl Pts',(-57.8003896508712,-4.70825387307828,
-55.2306628708486));
#133882=CARTESIAN_POINT('Ctrl Pts',(-58.1110275345658,-4.66169335137012,
-55.3564444847807));
#133883=CARTESIAN_POINT('Ctrl Pts',(-57.8247681406176,-4.8789835624615,
-54.8952730204543));
#133884=CARTESIAN_POINT('Ctrl Pts',(-57.8239228782473,-4.87294575633325,
-55.2309062620395));
#133885=CARTESIAN_POINT('Ctrl Pts',(-58.13138502781,-4.82819068711566,-55.3579993904125));
#133886=CARTESIAN_POINT('Ctrl Pts',(-57.8476108954267,-5.04400181406656,
-54.8980841413334));
#133887=CARTESIAN_POINT('Ctrl Pts',(-57.8468132839757,-5.03816723372008,
-55.2311383656919));
#133888=CARTESIAN_POINT('Ctrl Pts',(-58.1511322005955,-4.99473857781996,
-55.3594494677196));
#133889=CARTESIAN_POINT('Ctrl Pts',(-57.8697476022662,-5.20911947359366,
-54.9007953984755));
#133890=CARTESIAN_POINT('Ctrl Pts',(-57.8690388195133,-5.20383266421771,
-55.2313599550618));
#133891=CARTESIAN_POINT('Ctrl Pts',(-58.1702690071153,-5.16134039100007,
-55.3608055405081));
#133892=CARTESIAN_POINT('',(-58.1110275344741,-4.66169335080973,-55.3564444847662));
#133893=CARTESIAN_POINT('Origin',(-58.2961987903268,-4.64338668274023,-54.8923577774473));
#133894=CARTESIAN_POINT('Origin',(8.5361523961935,-12.9121665737653,-44.4738563732989));
#133895=CARTESIAN_POINT('Ctrl Pts',(-57.6567521511579,-3.75885801193397,
-55.9233081330105));
#133896=CARTESIAN_POINT('Ctrl Pts',(-57.7240148019691,-4.18000001999999,
-55.9233081330106));
#133897=CARTESIAN_POINT('Ctrl Pts',(-58.1504944089282,-4.18000001999999,
-55.9233081330105));
#133898=CARTESIAN_POINT('Ctrl Pts',(-57.6567521506183,-3.75885800855547,
-55.7907772949108));
#133899=CARTESIAN_POINT('Ctrl Pts',(-57.720407107403,-4.15741168017902,
-55.8378278694331));
#133900=CARTESIAN_POINT('Ctrl Pts',(-58.1234127965435,-4.18000001999999,
-55.8430054684059));
#133901=CARTESIAN_POINT('Ctrl Pts',(-57.6600305184041,-3.7792996685362,
-55.6597535514676));
#133902=CARTESIAN_POINT('Ctrl Pts',(-57.7195075819602,-4.152660660194,-55.7476211206603));
#133903=CARTESIAN_POINT('Ctrl Pts',(-58.1029269769243,-4.19030837229928,
-55.7671861383685));
#133904=CARTESIAN_POINT('Ctrl Pts',(-57.6739991030625,-3.86739163922285,
-55.4096956077557));
#133905=CARTESIAN_POINT('Ctrl Pts',(-57.7239127922735,-4.18385080200108,
-55.5755351032824));
#133906=CARTESIAN_POINT('Ctrl Pts',(-58.0744257289554,-4.23473154807011,
-55.6263252797207));
#133907=CARTESIAN_POINT('Ctrl Pts',(-57.6844132682985,-3.93331576897112,
-55.2955533951453));
#133908=CARTESIAN_POINT('Ctrl Pts',(-57.7289974028628,-4.21833224283565,
-55.4955276754143));
#133909=CARTESIAN_POINT('Ctrl Pts',(-58.0668966730084,-4.26797587839126,
-55.5640071328243));
#133910=CARTESIAN_POINT('Ctrl Pts',(-57.7251747303172,-4.19619393974228,
-55.0015199525886));
#133911=CARTESIAN_POINT('Ctrl Pts',(-57.7516721739213,-4.37202128884096,
-55.2943853542448));
#133912=CARTESIAN_POINT('Ctrl Pts',(-58.0611013349386,-4.40054054713837,
-55.4063183641287));
#133913=CARTESIAN_POINT('Ctrl Pts',(-57.7635403562534,-4.45018749203841,
-54.8876932766828));
#133914=CARTESIAN_POINT('Ctrl Pts',(-57.7764802977889,-4.54099770957247,
-55.2182493155612));
#133915=CARTESIAN_POINT('Ctrl Pts',(-58.0797561993292,-4.52867484626318,
-55.3492143127724));
#133916=CARTESIAN_POINT('Ctrl Pts',(-57.8012193907063,-4.71406478367227,
-54.8923577774466));
#133917=CARTESIAN_POINT('Ctrl Pts',(-57.8003896508711,-4.70825387307822,
-55.2306628708477));
#133918=CARTESIAN_POINT('Ctrl Pts',(-58.1110275345655,-4.66169335137004,
-55.3564444847799));
#133919=CARTESIAN_POINT('',(-58.1504944089236,-4.18000003396406,-55.9233081330193));
#133920=CARTESIAN_POINT('Origin',(-58.1504944089282,-3.68000001999999,-55.9233081330105));
#133921=CARTESIAN_POINT('Ctrl Pts',(-58.1504944089282,-4.18000001999999,
-55.9233081330105));
#133922=CARTESIAN_POINT('Ctrl Pts',(-58.1234127965435,-4.18000001999999,
-55.8430054684059));
#133923=CARTESIAN_POINT('Ctrl Pts',(-58.1029269769243,-4.19030837229928,
-55.7671861383685));
#133924=CARTESIAN_POINT('Ctrl Pts',(-58.0744257289554,-4.23473154807011,
-55.6263252797207));
#133925=CARTESIAN_POINT('Ctrl Pts',(-58.0668966730084,-4.26797587839126,
-55.5640071328243));
#133926=CARTESIAN_POINT('Ctrl Pts',(-58.0611013349386,-4.40054054713837,
-55.4063183641287));
#133927=CARTESIAN_POINT('Ctrl Pts',(-58.0797561993292,-4.52867484626318,
-55.3492143127724));
#133928=CARTESIAN_POINT('Ctrl Pts',(-58.1110275345658,-4.6616933513699,
-55.3564444847807));
#133929=CARTESIAN_POINT('Origin',(-58.1504944089282,-3.68000001999999,-55.24995));
#133930=CARTESIAN_POINT('',(-58.1504944089282,-4.18000001999999,-60.42825533736));
#133931=CARTESIAN_POINT('Origin',(-58.1504944089282,-3.68000001999999,-60.42825533736));
#133932=CARTESIAN_POINT('',(-58.1504944089282,-4.18000001999999,-55.24995));
#133933=CARTESIAN_POINT('Origin',(0.,-12.9675000200281,-60.42825533736));
#133934=CARTESIAN_POINT('',(-56.377904566775,1.85477723331148,-60.8508735991007));
#133935=CARTESIAN_POINT('',(-57.5607154366947,-3.75164060643487,-60.8508735991007));
#133936=CARTESIAN_POINT('Origin',(0.,-12.9675000200281,-60.8508735991007));
#133937=CARTESIAN_POINT('Origin',(-56.6143043465388,-3.67942422979871,-60.4241466659414));
#133938=CARTESIAN_POINT('Origin',(-55.1148638636367,2.00185121638848,-60.365292836485));
#133939=CARTESIAN_POINT('Origin',(-56.9614672388491,1.96999998000001,-55.24995));
#133940=CARTESIAN_POINT('',(-56.9614672388491,2.46999998000001,-55.74995));
#133941=CARTESIAN_POINT('Origin',(-56.9614672388491,1.96999998000001,-55.74995));
#133942=CARTESIAN_POINT('',(-56.9614672388491,2.46999998000001,-60.42825533736));
#133943=CARTESIAN_POINT('',(-56.9614672388491,2.46999998000001,-55.24995));
#133944=CARTESIAN_POINT('Origin',(-56.9614672388491,1.96999998000001,-60.42825533736));
#133945=CARTESIAN_POINT('Ctrl Pts',(-56.208463007634,2.83467839222654,-54.74995));
#133946=CARTESIAN_POINT('Ctrl Pts',(-56.2084630076339,2.83467839222653,
-55.2499499999999));
#133947=CARTESIAN_POINT('Ctrl Pts',(-56.6898028749653,2.96999998000001,
-55.24995));
#133948=CARTESIAN_POINT('Ctrl Pts',(-56.2799098403954,2.5805414908759,-54.7499500372609));
#133949=CARTESIAN_POINT('Ctrl Pts',(-56.2484819268069,2.69233080251842,
-55.2864232478283));
#133950=CARTESIAN_POINT('Ctrl Pts',(-56.761879333771,2.84181173581483,-55.24995));
#133951=CARTESIAN_POINT('Ctrl Pts',(-56.3494613434174,2.32547473937703,
-54.8529437484072));
#133952=CARTESIAN_POINT('Ctrl Pts',(-56.2763245403096,2.59340567144111,
-55.3787800334104));
#133953=CARTESIAN_POINT('Ctrl Pts',(-56.8320086455423,2.71321787394558,
-55.3014468715073));
#133954=CARTESIAN_POINT('Ctrl Pts',(-56.4486203895175,1.955305574271,-55.2191289705157));
#133955=CARTESIAN_POINT('Ctrl Pts',(-56.3089306288004,2.48216937222065,
-55.5705782077274));
#133956=CARTESIAN_POINT('Ctrl Pts',(-56.9320168401896,2.52654832947528,
-55.4845394879542));
#133957=CARTESIAN_POINT('Ctrl Pts',(-56.4778207259178,1.84316918512194,
-55.479632471504));
#133958=CARTESIAN_POINT('Ctrl Pts',(-56.313441444092,2.46999998405909,-55.6636097943426));
#133959=CARTESIAN_POINT('Ctrl Pts',(-56.9614672318199,2.46999998000001,
-55.614791233664));
#133960=CARTESIAN_POINT('Ctrl Pts',(-56.4778207328943,1.8431691585182,-55.74995));
#133961=CARTESIAN_POINT('Ctrl Pts',(-56.3134414454605,2.46999998000001,
-55.74995));
#133962=CARTESIAN_POINT('Ctrl Pts',(-56.9614672388491,2.46999998000001,
-55.74995));
#133963=CARTESIAN_POINT('',(-56.6898028749653,2.96999998000001,-55.24995));
#133964=CARTESIAN_POINT('Origin',(-56.6898028749653,2.96999998000001,-54.74995));
#133965=CARTESIAN_POINT('Ctrl Pts',(-56.6898028749653,2.96999998000001,
-55.24995));
#133966=CARTESIAN_POINT('Ctrl Pts',(-56.761879333771,2.84181173581483,-55.24995));
#133967=CARTESIAN_POINT('Ctrl Pts',(-56.8320086455423,2.71321787394558,
-55.3014468715073));
#133968=CARTESIAN_POINT('Ctrl Pts',(-56.9320168401896,2.52654832947528,
-55.4845394879542));
#133969=CARTESIAN_POINT('Ctrl Pts',(-56.9614672318199,2.46999998000001,
-55.614791233664));
#133970=CARTESIAN_POINT('Ctrl Pts',(-56.9614672388491,2.46999998000001,
-55.74995));
#133971=CARTESIAN_POINT('Origin',(0.,-12.9675000200281,-54.74995));
#133972=CARTESIAN_POINT('',(-56.5468500449175,3.46999998000001,-55.24995));
#133973=CARTESIAN_POINT('Origin',(-56.5468500449175,3.46999998000001,-54.74995));
#133974=CARTESIAN_POINT('Origin',(0.,-12.9675000200281,-55.24995));
#133975=CARTESIAN_POINT('Ctrl Pts',(-55.7689460407313,4.32194224278906,
-55.74995));
#133976=CARTESIAN_POINT('Ctrl Pts',(-55.8780548882949,3.96999998000002,
-55.74995));
#133977=CARTESIAN_POINT('Ctrl Pts',(-56.2465221147258,3.96999998000001,
-55.74995));
#133978=CARTESIAN_POINT('Ctrl Pts',(-55.7689460480881,4.32194221905895,
-55.6164566007256));
#133979=CARTESIAN_POINT('Ctrl Pts',(-55.8780548935443,3.96999996254405,
-55.6679224120286));
#133980=CARTESIAN_POINT('Ctrl Pts',(-56.2465221221473,3.96999998000001,
-55.683203301545));
#133981=CARTESIAN_POINT('Ctrl Pts',(-55.777377389072,4.29480596539276,-55.4823754218786));
#133982=CARTESIAN_POINT('Ctrl Pts',(-55.8841708256374,3.94968459977806,
-55.5852103705331));
#133983=CARTESIAN_POINT('Ctrl Pts',(-56.2550256651168,3.95631565470027,
-55.6161627093404));
#133984=CARTESIAN_POINT('Ctrl Pts',(-55.8090161453349,4.19224220492976,
-55.2379754767005));
#133985=CARTESIAN_POINT('Ctrl Pts',(-55.9063784289296,3.87553573797955,
-55.4407856273786));
#133986=CARTESIAN_POINT('Ctrl Pts',(-56.2869353583447,3.90459461560065,
-55.4939627399492));
#133987=CARTESIAN_POINT('Ctrl Pts',(-55.832275617124,4.11659879830721,-55.1268557913785));
#133988=CARTESIAN_POINT('Ctrl Pts',(-55.9226989367341,3.8208945781902,-55.3782063812366));
#133989=CARTESIAN_POINT('Ctrl Pts',(-56.3103940129914,3.86644903217756,
-55.4384028944151));
#133990=CARTESIAN_POINT('Ctrl Pts',(-55.888335440433,3.9323045563208,-54.9446837986715));
#133991=CARTESIAN_POINT('Ctrl Pts',(-55.9602568779234,3.69427053570811,
-55.285569160897));
#133992=CARTESIAN_POINT('Ctrl Pts',(-56.366933902262,3.77351280880021,-55.3473169006099));
#133993=CARTESIAN_POINT('Ctrl Pts',(-55.9215848671782,3.82212901679781,
-54.8721313715614));
#133994=CARTESIAN_POINT('Ctrl Pts',(-55.9820168525955,3.62048086904919,
-55.2550739756198));
#133995=CARTESIAN_POINT('Ctrl Pts',(-56.4004680605965,3.71795329740048,
-55.3110406862353));
#133996=CARTESIAN_POINT('Ctrl Pts',(-55.9918544429005,3.58627698995622,
-54.7753183134609));
#133997=CARTESIAN_POINT('Ctrl Pts',(-56.0252324832575,3.47302446308311,
-55.2281701114017));
#133998=CARTESIAN_POINT('Ctrl Pts',(-56.4713393874401,3.59901742755992,
-55.262634156276));
#133999=CARTESIAN_POINT('Ctrl Pts',(-56.0297048503836,3.4577829011709,-54.7499500149493));
#134000=CARTESIAN_POINT('Ctrl Pts',(-56.047279588089,3.39732382739444,-55.2323508865986));
#134001=CARTESIAN_POINT('Ctrl Pts',(-56.50951584811,3.5342168990206,-55.24995));
#134002=CARTESIAN_POINT('Ctrl Pts',(-56.0667239566569,3.33043300908083,
-54.74995));
#134003=CARTESIAN_POINT('Ctrl Pts',(-56.066723956657,3.33043300908077,-55.24995));
#134004=CARTESIAN_POINT('Ctrl Pts',(-56.5468500449175,3.46999998000007,
-55.24995));
#134005=CARTESIAN_POINT('',(-56.2465221147258,3.96999998000001,-55.74995));
#134006=CARTESIAN_POINT('Origin',(-56.2465221147258,4.46999998000001,-55.74995));
#134007=CARTESIAN_POINT('Ctrl Pts',(-56.2465221147258,3.96999998000007,
-55.74995));
#134008=CARTESIAN_POINT('Ctrl Pts',(-56.2465221172463,3.96999998000007,
-55.7272812089341));
#134009=CARTESIAN_POINT('Ctrl Pts',(-56.24750295639,3.96845400764675,-55.7045717667832));
#134010=CARTESIAN_POINT('Ctrl Pts',(-56.2494234122338,3.96537155503915,
-55.6820750956295));
#134011=CARTESIAN_POINT('Ctrl Pts',(-56.2513459831365,3.96228570762857,
-55.6595536481773));
#134012=CARTESIAN_POINT('Ctrl Pts',(-56.2542102415385,3.95766009770567,
-55.6372462305913));
#134013=CARTESIAN_POINT('Ctrl Pts',(-56.2579748311759,3.95155602091719,
-55.615399714024));
#134014=CARTESIAN_POINT('Ctrl Pts',(-56.2615221746811,3.9458041968841,-55.5948139115537));
#134015=CARTESIAN_POINT('Ctrl Pts',(-56.2658689354504,3.9387402676577,-55.5746377942181));
#134016=CARTESIAN_POINT('Ctrl Pts',(-56.2709805117308,3.93045513515051,
-55.5550627246448));
#134017=CARTESIAN_POINT('Ctrl Pts',(-56.2765960817443,3.92135310103939,
-55.5335575826534));
#134018=CARTESIAN_POINT('Ctrl Pts',(-56.2831412261279,3.91075174977411,
-55.5127182769628));
#134019=CARTESIAN_POINT('Ctrl Pts',(-56.2904985464591,3.89878795974976,
-55.4927713297682));
#134020=CARTESIAN_POINT('Ctrl Pts',(-56.2978778612356,3.88678840440414,
-55.4727647518903));
#134021=CARTESIAN_POINT('Ctrl Pts',(-56.3060742151598,3.87341874044962,
-55.4536564757209));
#134022=CARTESIAN_POINT('Ctrl Pts',(-56.3149691537834,3.85885777178856,
-55.4356418426681));
#134023=CARTESIAN_POINT('Ctrl Pts',(-56.3224025873938,3.84668927929807,
-55.4205871487034));
#134024=CARTESIAN_POINT('Ctrl Pts',(-56.330323899967,3.8336897103653,-55.4062957646521));
#134025=CARTESIAN_POINT('Ctrl Pts',(-56.3386639576267,3.81998092048891,
-55.3928598975125));
#134026=CARTESIAN_POINT('Ctrl Pts',(-56.3485367757166,3.80375268871842,
-55.3769547470254));
#134027=CARTESIAN_POINT('Ctrl Pts',(-56.3590516393933,3.78643081276152,
-55.3621527091661));
#134028=CARTESIAN_POINT('Ctrl Pts',(-56.3700653174119,3.76821160325647,
-55.3486149432771));
#134029=CARTESIAN_POINT('Ctrl Pts',(-56.3811000400428,3.74995758102126,
-55.3350513098229));
#134030=CARTESIAN_POINT('Ctrl Pts',(-56.3926354850762,3.73080346228537,
-55.3227572166925));
#134031=CARTESIAN_POINT('Ctrl Pts',(-56.404527598651,3.7109748182806,-55.3118505508841));
#134032=CARTESIAN_POINT('Ctrl Pts',(-56.414753129079,3.69392499771326,-55.3024723657204));
#134033=CARTESIAN_POINT('Ctrl Pts',(-56.4252423645287,3.67637719717626,
-55.2941193424573));
#134034=CARTESIAN_POINT('Ctrl Pts',(-56.4359037240183,3.65848536248023,
-55.2868374212556));
#134035=CARTESIAN_POINT('Ctrl Pts',(-56.4480269746482,3.63814019013509,
-55.2785569992435));
#134036=CARTESIAN_POINT('Ctrl Pts',(-56.4604710249688,3.61717859047507,
-55.2715931459213));
#134037=CARTESIAN_POINT('Ctrl Pts',(-56.4730923955105,3.59582457403251,
-55.2660407403897));
#134038=CARTESIAN_POINT('Ctrl Pts',(-56.485718783795,3.57446206810312,-55.2604861274479));
#134039=CARTESIAN_POINT('Ctrl Pts',(-56.4985226333192,3.55270760676572,
-55.2563443375913));
#134040=CARTESIAN_POINT('Ctrl Pts',(-56.511360293421,3.53080101674991,-55.2536605341334));
#134041=CARTESIAN_POINT('Ctrl Pts',(-56.5231990099542,3.51059905569539,
-55.2511855668795));
#134042=CARTESIAN_POINT('Ctrl Pts',(-56.5350664799457,3.49026837472315,
-55.24995));
#134043=CARTESIAN_POINT('Ctrl Pts',(-56.5468500449175,3.46999998000001,
-55.24995));
#134044=CARTESIAN_POINT('Origin',(-56.2465221147258,4.46999998000001,-55.24995));
#134045=CARTESIAN_POINT('',(-56.2465221147258,3.96999998000001,-60.42825533736));
#134046=CARTESIAN_POINT('Origin',(-56.2465221147258,4.46999998000001,-60.42825533736));
#134047=CARTESIAN_POINT('',(-56.2465221147258,3.96999998000001,-55.24995));
#134048=CARTESIAN_POINT('Origin',(0.,-12.9675000200281,-60.42825533736));
#134049=CARTESIAN_POINT('',(-53.6034226162473,9.94191093135268,-60.8508735991007));
#134050=CARTESIAN_POINT('',(-55.6666368275827,4.33549309160632,-60.8508735991007));
#134051=CARTESIAN_POINT('Origin',(0.,-12.9675000200281,-60.8508735991007));
#134052=CARTESIAN_POINT('Origin',(-54.6351094353318,4.47360462069243,-60.4185055563343));
#134053=CARTESIAN_POINT('Origin',(-52.4761756351917,10.1269382012971,-60.4132827620456));
#134054=CARTESIAN_POINT('Origin',(-54.1729175880533,10.11999998,-55.24995));
#134055=CARTESIAN_POINT('',(-54.1729175880533,10.61999998,-55.74995));
#134056=CARTESIAN_POINT('Origin',(-54.1729175880533,10.11999998,-55.74995));
#134057=CARTESIAN_POINT('',(-54.1729175880533,10.61999998,-60.42825533736));
#134058=CARTESIAN_POINT('',(-54.1729175880533,10.61999998,-55.24995));
#134059=CARTESIAN_POINT('Origin',(-54.1729175880533,10.11999998,-60.42825533736));
#134060=CARTESIAN_POINT('Ctrl Pts',(-53.3256899305368,10.8121330655672,
-54.7553968408231));
#134061=CARTESIAN_POINT('Ctrl Pts',(-53.3054454943535,10.8575310968505,
-55.2747187747876));
#134062=CARTESIAN_POINT('Ctrl Pts',(-53.7823432375846,11.067884690566,-55.2526734204115));
#134063=CARTESIAN_POINT('Ctrl Pts',(-53.4285862862346,10.5813885818665,
-54.7797862992586));
#134064=CARTESIAN_POINT('Ctrl Pts',(-53.3650311600591,10.7244739426765,
-55.3417466734359));
#134065=CARTESIAN_POINT('Ctrl Pts',(-53.8861362179292,10.9515071084652,
-55.2648699557477));
#134066=CARTESIAN_POINT('Ctrl Pts',(-53.5254458539065,10.3597364405483,
-54.885939939012));
#134067=CARTESIAN_POINT('Ctrl Pts',(-53.3983781597441,10.6502596450882,
-55.4540676493459));
#134068=CARTESIAN_POINT('Ctrl Pts',(-53.9838097653667,10.83974934456,-55.3179449795228));
#134069=CARTESIAN_POINT('Ctrl Pts',(-53.633790842791,10.1090015716016,-55.1553271807471));
#134070=CARTESIAN_POINT('Ctrl Pts',(-53.4176451441909,10.6111056725941,
-55.596678279911));
#134071=CARTESIAN_POINT('Ctrl Pts',(-54.0930825652429,10.7133083132261,
-55.4526385853652));
#134072=CARTESIAN_POINT('Ctrl Pts',(-53.6624100137865,10.0422483461928,
-55.2594857136242));
#134073=CARTESIAN_POINT('Ctrl Pts',(-53.4186534680994,10.6106295502708,
-55.6378844781733));
#134074=CARTESIAN_POINT('Ctrl Pts',(-54.1219468150851,10.6796458924645,
-55.5047178594674));
#134075=CARTESIAN_POINT('Ctrl Pts',(-53.702610379063,9.94826762670561,-55.4957569720976));
#134076=CARTESIAN_POINT('Ctrl Pts',(-53.4178589543304,10.6154785181549,
-55.7046481866627));
#134077=CARTESIAN_POINT('Ctrl Pts',(-54.1624914359772,10.6322531187842,
-55.6228534833935));
#134078=CARTESIAN_POINT('Ctrl Pts',(-53.7129480039811,9.9239694167493,-55.6201514218302));
#134079=CARTESIAN_POINT('Ctrl Pts',(-53.4163125940233,10.619999979359,-55.7271468411276));
#134080=CARTESIAN_POINT('Ctrl Pts',(-54.172917586547,10.61999998,-55.685050712911));
#134081=CARTESIAN_POINT('Ctrl Pts',(-53.7129480054761,9.92396941324122,
-55.74995));
#134082=CARTESIAN_POINT('Ctrl Pts',(-53.4163125938068,10.61999998,-55.74995));
#134083=CARTESIAN_POINT('Ctrl Pts',(-54.1729175880533,10.61999998,-55.74995));
#134084=CARTESIAN_POINT('Ctrl Pts',(-53.7823432375846,11.067884690566,-55.2526734204115));
#134085=CARTESIAN_POINT('Ctrl Pts',(-53.8861362179292,10.9515071084652,
-55.2648699557477));
#134086=CARTESIAN_POINT('Ctrl Pts',(-53.9838097653667,10.83974934456,-55.3179449795228));
#134087=CARTESIAN_POINT('Ctrl Pts',(-54.0930825652429,10.7133083132261,
-55.4526385853652));
#134088=CARTESIAN_POINT('Ctrl Pts',(-54.1219468150851,10.6796458924645,
-55.5047178594674));
#134089=CARTESIAN_POINT('Ctrl Pts',(-54.1624914359772,10.6322531187842,
-55.6228534833935));
#134090=CARTESIAN_POINT('Ctrl Pts',(-54.172917586547,10.61999998,-55.685050712911));
#134091=CARTESIAN_POINT('Ctrl Pts',(-54.1729175880533,10.61999998,-55.74995));
#134092=CARTESIAN_POINT('Origin',(-4.6996065532056,-66.6842487255793,-59.64995));
#134093=CARTESIAN_POINT('',(-39.5,-63.6396088127436,-60.64995));
#134094=CARTESIAN_POINT('',(-33.85,-64.1339197616649,-60.64995));
#134095=CARTESIAN_POINT('',(-4.6996065532056,-66.6842487255793,-60.64995));
#134096=CARTESIAN_POINT('Ctrl Pts',(-33.8064221286261,-65.1415521689341,
-59.64995));
#134097=CARTESIAN_POINT('Ctrl Pts',(-33.8064221286289,-65.1415521689339,
-59.7808732880372));
#134098=CARTESIAN_POINT('Ctrl Pts',(-33.8075563441358,-65.1153261907357,
-59.9116978933078));
#134099=CARTESIAN_POINT('Ctrl Pts',(-33.8119222489988,-65.0143752473362,
-60.1535689714224));
#134100=CARTESIAN_POINT('Ctrl Pts',(-33.8151522214979,-64.9396899802014,
-60.2644967268053));
#134101=CARTESIAN_POINT('Ctrl Pts',(-33.8232193617858,-64.7531569593752,
-60.4496168355678));
#134102=CARTESIAN_POINT('Ctrl Pts',(-33.8280533572402,-64.6413825582346,
-60.5237363920407));
#134103=CARTESIAN_POINT('Ctrl Pts',(-33.8385935839748,-64.3976654214474,
-60.6239226729819));
#134104=CARTESIAN_POINT('Ctrl Pts',(-33.8442946417933,-64.2658423095942,
-60.64995));
#134105=CARTESIAN_POINT('Ctrl Pts',(-33.85,-64.1339197616649,-60.64995));
#134106=CARTESIAN_POINT('Ctrl Pts',(-39.5,-63.6396088127436,-60.64995));
#134107=CARTESIAN_POINT('Ctrl Pts',(-39.4942946417933,-63.771531360673,
-60.64995));
#134108=CARTESIAN_POINT('Ctrl Pts',(-39.4885935839748,-63.9033544725257,
-60.623922672982));
#134109=CARTESIAN_POINT('Ctrl Pts',(-39.4780533572402,-64.1470716093135,
-60.5237363920406));
#134110=CARTESIAN_POINT('Ctrl Pts',(-39.4732193617865,-64.2588460104538,
-60.4496168355678));
#134111=CARTESIAN_POINT('Ctrl Pts',(-39.4651522214972,-64.4453790312801,
-60.2644967268053));
#134112=CARTESIAN_POINT('Ctrl Pts',(-39.4619222489981,-64.5200642984147,
-60.153568971423));
#134113=CARTESIAN_POINT('Ctrl Pts',(-39.4575563441365,-64.6210152418146,
-59.9116978933072));
#134114=CARTESIAN_POINT('Ctrl Pts',(-39.4564221286269,-64.6472412200127,
-59.7808732880376));
#134115=CARTESIAN_POINT('Ctrl Pts',(-39.4564221286262,-64.6472412200127,
-59.64995));
#134116=CARTESIAN_POINT('Origin',(-39.5,-65.1453385690586,-52.64995));
#134117=CARTESIAN_POINT('',(-40.,-65.1453385690586,-59.64995));
#134118=CARTESIAN_POINT('Origin',(-39.5,-65.1453385690586,-59.64995));
#134119=CARTESIAN_POINT('',(-40.,-65.1453385690586,-55.74995));
#134120=CARTESIAN_POINT('Origin',(-39.5,-65.1453385690586,-55.74995));
#134121=CARTESIAN_POINT('',(-40.,-65.1453385690586,-55.24995));
#134122=CARTESIAN_POINT('Ctrl Pts',(-40.4564221286262,-64.5597525564868,
-54.74995));
#134123=CARTESIAN_POINT('Ctrl Pts',(-40.4564221286261,-64.5597525564868,
-55.24995));
#134124=CARTESIAN_POINT('Ctrl Pts',(-40.5,-65.0578499055327,-55.24995));
#134125=CARTESIAN_POINT('Ctrl Pts',(-40.1938874372398,-64.5827213657654,
-54.7499500000659));
#134126=CARTESIAN_POINT('Ctrl Pts',(-40.322075011829,-64.5715064061754,
-55.2615708605686));
#134127=CARTESIAN_POINT('Ctrl Pts',(-40.3687326543062,-65.0808187148095,
-55.24995));
#134128=CARTESIAN_POINT('Ctrl Pts',(-39.9344354391268,-64.6054204743294,
-54.8577231271254));
#134129=CARTESIAN_POINT('Ctrl Pts',(-40.2033393021413,-64.581894434738,
-55.3274496218431));
#134130=CARTESIAN_POINT('Ctrl Pts',(-40.2390066552503,-65.1035178233753,
-55.3038365635632));
#134131=CARTESIAN_POINT('Ctrl Pts',(-39.5641952557525,-64.6378122931564,
-55.2279633105016));
#134132=CARTESIAN_POINT('Ctrl Pts',(-40.0417246342956,-64.5960338860327,
-55.5133819370971));
#134133=CARTESIAN_POINT('Ctrl Pts',(-40.0538865635631,-65.1359096422023,
-55.4889566552503));
#134134=CARTESIAN_POINT('Ctrl Pts',(-39.4564221286917,-64.647241220007,
-55.4874153086129));
#134135=CARTESIAN_POINT('Ctrl Pts',(-40.0000000000045,-64.5996843185185,
-55.6317784220497));
#134136=CARTESIAN_POINT('Ctrl Pts',(-40.,-65.1453385690531,-55.6186826543065));
#134137=CARTESIAN_POINT('Ctrl Pts',(-39.4564221286262,-64.6472412200127,
-55.74995));
#134138=CARTESIAN_POINT('Ctrl Pts',(-40.,-64.5996843185239,-55.74995));
#134139=CARTESIAN_POINT('Ctrl Pts',(-40.,-65.1453385690586,-55.74995));
#134140=CARTESIAN_POINT('',(-40.5,-65.0578499055327,-55.24995));
#134141=CARTESIAN_POINT('Origin',(-40.5,-65.0578499055327,-54.74995));
#134142=CARTESIAN_POINT('Ctrl Pts',(-40.5,-65.0578499055327,-55.24995));
#134143=CARTESIAN_POINT('Ctrl Pts',(-40.3687326543062,-65.0808187148095,
-55.24995));
#134144=CARTESIAN_POINT('Ctrl Pts',(-40.2390066552503,-65.1035178233753,
-55.3038365635632));
#134145=CARTESIAN_POINT('Ctrl Pts',(-40.0538865635631,-65.1359096422023,
-55.4889566552503));
#134146=CARTESIAN_POINT('Ctrl Pts',(-40.,-65.1453385690531,-55.6186826543065));
#134147=CARTESIAN_POINT('Ctrl Pts',(-40.,-65.1453385690586,-55.74995));
#134148=CARTESIAN_POINT('Origin',(-44.2377516955329,-64.7308390050988,-54.74995));
#134149=CARTESIAN_POINT('',(-41.,-65.0141055737697,-55.24995));
#134150=CARTESIAN_POINT('Origin',(-41.,-65.0141055737697,-54.74995));
#134151=CARTESIAN_POINT('',(-40.7958880023324,-65.0319630596553,-55.24995));
#134152=CARTESIAN_POINT('Ctrl Pts',(-41.9564221286262,-64.428519561198,
-55.74995));
#134153=CARTESIAN_POINT('Ctrl Pts',(-41.5,-64.4684513232351,-55.74995));
#134154=CARTESIAN_POINT('Ctrl Pts',(-41.5,-64.9266169102438,-55.74995));
#134155=CARTESIAN_POINT('Ctrl Pts',(-41.9564221285606,-64.4285195612037,
-55.487415308613));
#134156=CARTESIAN_POINT('Ctrl Pts',(-41.4999999999489,-64.4684513232351,
-55.6078478088783));
#134157=CARTESIAN_POINT('Ctrl Pts',(-41.5,-64.9266169102493,-55.6186826543063));
#134158=CARTESIAN_POINT('Ctrl Pts',(-41.8486490015007,-64.4379484880542,
-55.2279633105015));
#134159=CARTESIAN_POINT('Ctrl Pts',(-41.4358662151155,-64.4740623023634,
-55.4680441063688));
#134160=CARTESIAN_POINT('Ctrl Pts',(-41.4461134364372,-64.9360458371002,
-55.4889566552508));
#134161=CARTESIAN_POINT('Ctrl Pts',(-41.4784088181247,-64.4703403068813,
-54.8577231271255));
#134162=CARTESIAN_POINT('Ctrl Pts',(-41.2286175782531,-64.4921942086162,
-55.2822894538775));
#134163=CARTESIAN_POINT('Ctrl Pts',(-41.2609933447493,-64.9684376559271,
-55.3038365635627));
#134164=CARTESIAN_POINT('Ctrl Pts',(-41.2189568200132,-64.4930394154452,
-54.7499500000659));
#134165=CARTESIAN_POINT('Ctrl Pts',(-41.0869589695398,-64.5045877309693,
-55.2386587236917));
#134166=CARTESIAN_POINT('Ctrl Pts',(-41.1312673456941,-64.991136764493,
-55.24995));
#134167=CARTESIAN_POINT('Ctrl Pts',(-40.9564221286262,-64.5160082247239,
-54.74995));
#134168=CARTESIAN_POINT('Ctrl Pts',(-40.9564221286262,-64.5160082247238,
-55.24995));
#134169=CARTESIAN_POINT('Ctrl Pts',(-41.,-65.0141055737697,-55.24995));
#134170=CARTESIAN_POINT('',(-41.5,-64.9266169102438,-55.74995));
#134171=CARTESIAN_POINT('Origin',(-42.,-64.9266169102438,-55.74995));
#134172=CARTESIAN_POINT('Ctrl Pts',(-41.5,-64.9266169102438,-55.74995));
#134173=CARTESIAN_POINT('Ctrl Pts',(-41.5,-64.9266169102493,-55.6186826543063));
#134174=CARTESIAN_POINT('Ctrl Pts',(-41.4461134364372,-64.9360458371002,
-55.4889566552508));
#134175=CARTESIAN_POINT('Ctrl Pts',(-41.2609933447493,-64.9684376559271,
-55.3038365635627));
#134176=CARTESIAN_POINT('Ctrl Pts',(-41.1312673456941,-64.991136764493,
-55.24995));
#134177=CARTESIAN_POINT('Ctrl Pts',(-41.,-65.0141055737697,-55.24995));
#134178=CARTESIAN_POINT('Origin',(-42.,-64.9266169102438,-52.64995));
#134179=CARTESIAN_POINT('',(-41.5,-64.9266169102438,-59.64995));
#134180=CARTESIAN_POINT('Origin',(-42.,-64.9266169102438,-59.64995));
#134181=CARTESIAN_POINT('',(-41.5,-64.9266169102438,-177.34995));
#134182=CARTESIAN_POINT('Origin',(-4.6996065532056,-66.6842487255793,-59.64995));
#134183=CARTESIAN_POINT('',(-42.,-63.4208871539288,-60.64995));
#134184=CARTESIAN_POINT('',(-4.6996065532056,-66.6842487255793,-60.64995));
#134185=CARTESIAN_POINT('Ctrl Pts',(-41.9564221286262,-64.428519561198,
-59.64995));
#134186=CARTESIAN_POINT('Ctrl Pts',(-41.9564221286289,-64.4285195611977,
-59.7808732880376));
#134187=CARTESIAN_POINT('Ctrl Pts',(-41.9575563441358,-64.4022935829999,
-59.9116978933072));
#134188=CARTESIAN_POINT('Ctrl Pts',(-41.9619222489988,-64.3013426395998,
-60.153568971423));
#134189=CARTESIAN_POINT('Ctrl Pts',(-41.9651522214979,-64.2266573724653,
-60.2644967268053));
#134190=CARTESIAN_POINT('Ctrl Pts',(-41.9732193617859,-64.0401243516391,
-60.4496168355678));
#134191=CARTESIAN_POINT('Ctrl Pts',(-41.9780533572395,-63.9283499504973,
-60.5237363920413));
#134192=CARTESIAN_POINT('Ctrl Pts',(-41.9885935839755,-63.6846328137124,
-60.6239226729814));
#134193=CARTESIAN_POINT('Ctrl Pts',(-41.9942946417934,-63.5528097018572,
-60.64995));
#134194=CARTESIAN_POINT('Ctrl Pts',(-42.,-63.4208871539288,-60.64995));
#134195=CARTESIAN_POINT('Ctrl Pts',(-25.6564221286262,-65.8545847766702,
-55.74995));
#134196=CARTESIAN_POINT('Ctrl Pts',(-25.2,-65.8945165387074,-55.74995));
#134197=CARTESIAN_POINT('Ctrl Pts',(-25.2,-66.3526821257161,-55.74995));
#134198=CARTESIAN_POINT('Ctrl Pts',(-25.6564221285773,-65.8545847766745,
-55.5542114975488));
#134199=CARTESIAN_POINT('Ctrl Pts',(-25.1999999999616,-65.8945165387115,
-55.6441589529833));
#134200=CARTESIAN_POINT('Ctrl Pts',(-25.2,-66.3526821257202,-55.6520807487743));
#134201=CARTESIAN_POINT('Ctrl Pts',(-25.5974642419416,-65.8597429233806,
-55.3592003264656));
#134202=CARTESIAN_POINT('Ctrl Pts',(-25.1652351487286,-65.8975580690824,
-55.5387129880067));
#134203=CARTESIAN_POINT('Ctrl Pts',(-25.1705210566577,-66.3578402724271,
-55.5545751632329));
#134204=CARTESIAN_POINT('Ctrl Pts',(-25.3809306020242,-65.8786871621453,
-55.033477363834));
#134205=CARTESIAN_POINT('Ctrl Pts',(-25.0420941082282,-65.9083315141418,
-55.3693682972756));
#134206=CARTESIAN_POINT('Ctrl Pts',(-25.062254236699,-66.3767845111906,
-55.391713681917));
#134207=CARTESIAN_POINT('Ctrl Pts',(-25.2239370702218,-65.892422316425,
-54.9036397860402));
#134208=CARTESIAN_POINT('Ctrl Pts',(-24.9535760611327,-65.9160758397827,
-55.3059410651653));
#134209=CARTESIAN_POINT('Ctrl Pts',(-24.9837596261582,-66.3905192883359,
-55.3267957976874));
#134210=CARTESIAN_POINT('Ctrl Pts',(-25.043451507077,-65.9082127571302,
-54.8278826162281));
#134211=CARTESIAN_POINT('Ctrl Pts',(-24.8576734148988,-65.9244662341272,
-55.273872259957));
#134212=CARTESIAN_POINT('Ctrl Pts',(-24.8935146892254,-66.4063101061761,
-55.2889163081141));
#134213=CARTESIAN_POINT('',(-25.2,-66.3526821257161,-55.74995));
#134214=CARTESIAN_POINT('Origin',(-25.7,-66.3526821257161,-55.74995));
#134215=CARTESIAN_POINT('Ctrl Pts',(-25.2,-66.3526821257161,-55.74995));
#134216=CARTESIAN_POINT('Ctrl Pts',(-25.2,-66.3526821257202,-55.6520807487743));
#134217=CARTESIAN_POINT('Ctrl Pts',(-25.1705210566577,-66.3578402724271,
-55.5545751632329));
#134218=CARTESIAN_POINT('Ctrl Pts',(-25.062254236699,-66.3767845111906,
-55.391713681917));
#134219=CARTESIAN_POINT('Ctrl Pts',(-24.9837596261582,-66.3905192883359,
-55.3267957976874));
#134220=CARTESIAN_POINT('Ctrl Pts',(-24.8935146892254,-66.4063101061761,
-55.2889163081141));
#134221=CARTESIAN_POINT('Origin',(-25.7,-66.3526821257161,-52.64995));
#134222=CARTESIAN_POINT('',(-25.2,-66.3526821257161,-60.0322609860583));
#134223=CARTESIAN_POINT('Origin',(-25.7,-66.3526821257161,-60.0322609860583));
#134224=CARTESIAN_POINT('',(-25.2,-66.3526821257161,-55.24995));
#134225=CARTESIAN_POINT('Ctrl Pts',(-28.6150130758292,-64.5919217712362,
-60.64995));
#134226=CARTESIAN_POINT('Ctrl Pts',(-28.7021688185769,-65.588116469328,
-60.64995));
#134227=CARTESIAN_POINT('Ctrl Pts',(-28.7021688185769,-65.588116469328,
-59.64995));
#134228=CARTESIAN_POINT('Ctrl Pts',(-28.0991390263463,-64.7442358506513,
-60.64995));
#134229=CARTESIAN_POINT('Ctrl Pts',(-28.2033028175763,-65.6317615890315,
-60.5485267380177));
#134230=CARTESIAN_POINT('Ctrl Pts',(-28.1296330247306,-65.6382068607523,
-59.649950002333));
#134231=CARTESIAN_POINT('Ctrl Pts',(-27.584859681119,-64.89321892758,-60.6698497986403));
#134232=CARTESIAN_POINT('Ctrl Pts',(-27.6612478839793,-65.6791852507322,
-60.4928259381272));
#134233=CARTESIAN_POINT('Ctrl Pts',(-27.5637794550765,-65.6877126333127,
-59.6897495968387));
#134234=CARTESIAN_POINT('Ctrl Pts',(-26.5596543334024,-65.1843117452004,
-60.7464752559987));
#134235=CARTESIAN_POINT('Ctrl Pts',(-26.5839609508645,-65.7734356447442,
-60.477600868097));
#134236=CARTESIAN_POINT('Ctrl Pts',(-26.4448676457179,-65.7856047321169,
-59.8430005124393));
#134237=CARTESIAN_POINT('Ctrl Pts',(-26.0485518825385,-65.3264611076661,
-60.802611641644));
#134238=CARTESIAN_POINT('Ctrl Pts',(-26.0406038710994,-65.8209732294689,
-60.5097186566584));
#134239=CARTESIAN_POINT('Ctrl Pts',(-25.8914156146746,-65.8340255106386,
-59.9553384305595));
#134240=CARTESIAN_POINT('Ctrl Pts',(-25.5416884892005,-65.4644312001072,
-60.8848189055469));
#134241=CARTESIAN_POINT('Ctrl Pts',(-25.4903329393053,-65.86911569787,-60.5974971539929));
#134242=CARTESIAN_POINT('Ctrl Pts',(-25.3471476467368,-65.8816427877534,
-60.1196878110938));
#134243=CARTESIAN_POINT('',(-28.6150130758292,-64.5919217712362,-60.64995));
#134244=CARTESIAN_POINT('Origin',(-28.6150130758292,-64.5919217712362,-59.64995));
#134245=CARTESIAN_POINT('',(-25.559825688613,-65.4594929016036,-60.8818893816079));
#134246=CARTESIAN_POINT('Ctrl Pts',(-28.6150130758292,-64.5919217712362,
-60.64995));
#134247=CARTESIAN_POINT('Ctrl Pts',(-28.0991390263463,-64.7442358506513,
-60.64995));
#134248=CARTESIAN_POINT('Ctrl Pts',(-27.584859681119,-64.89321892758,-60.6698497986403));
#134249=CARTESIAN_POINT('Ctrl Pts',(-26.5657678476125,-65.1825758977617,
-60.7460183223478));
#134250=CARTESIAN_POINT('Ctrl Pts',(-26.0607433397739,-65.32306995879,-60.8012751647717));
#134251=CARTESIAN_POINT('Ctrl Pts',(-25.5598256882386,-65.4594929016689,
-60.8818893816956));
#134252=CARTESIAN_POINT('Ctrl Pts',(-25.6564221286262,-65.8545847766702,
-60.0322609860583));
#134253=CARTESIAN_POINT('Ctrl Pts',(-25.6369719721911,-65.8562864448621,
-60.1960022731895));
#134254=CARTESIAN_POINT('Ctrl Pts',(-25.6175094928883,-65.8217787894205,
-60.3603674876955));
#134255=CARTESIAN_POINT('Ctrl Pts',(-25.5836282597575,-65.6869336598766,
-60.6533188274199));
#134256=CARTESIAN_POINT('Ctrl Pts',(-25.5689423412454,-65.58489046904,-60.7845618642934));
#134257=CARTESIAN_POINT('Ctrl Pts',(-25.5598256882386,-65.4594929016689,
-60.8818893816956));
#134258=CARTESIAN_POINT('Origin',(-4.6996065532056,-66.6842487255793,-59.64995));
#134259=CARTESIAN_POINT('',(-31.35,-64.3526414204797,-60.64995));
#134260=CARTESIAN_POINT('',(-4.6996065532056,-66.6842487255793,-60.64995));
#134261=CARTESIAN_POINT('Ctrl Pts',(-31.35,-64.3526414204797,-60.64995));
#134262=CARTESIAN_POINT('Ctrl Pts',(-31.3442946417934,-64.4845639684081,
-60.64995));
#134263=CARTESIAN_POINT('Ctrl Pts',(-31.3385935839747,-64.6163870802633,
-60.6239226729814));
#134264=CARTESIAN_POINT('Ctrl Pts',(-31.3280533572402,-64.8601042170482,
-60.5237363920412));
#134265=CARTESIAN_POINT('Ctrl Pts',(-31.3232193617865,-64.9718786181899,
-60.4496168355678));
#134266=CARTESIAN_POINT('Ctrl Pts',(-31.3151522214972,-65.1584116390162,
-60.2644967268053));
#134267=CARTESIAN_POINT('Ctrl Pts',(-31.3119222489988,-65.2330969061508,
-60.1535689714229));
#134268=CARTESIAN_POINT('Ctrl Pts',(-31.3075563441358,-65.3340478495507,
-59.9116978933073));
#134269=CARTESIAN_POINT('Ctrl Pts',(-31.3064221286269,-65.3602738277488,
-59.7808732880376));
#134270=CARTESIAN_POINT('Ctrl Pts',(-31.3064221286262,-65.3602738277489,
-59.64995));
#134271=CARTESIAN_POINT('Origin',(-31.35,-65.8583711767947,-52.64995));
#134272=CARTESIAN_POINT('',(-31.85,-65.8583711767947,-59.64995));
#134273=CARTESIAN_POINT('Origin',(-31.35,-65.8583711767947,-59.64995));
#134274=CARTESIAN_POINT('',(-31.85,-65.8583711767947,-55.74995));
#134275=CARTESIAN_POINT('Origin',(-31.35,-65.8583711767947,-55.74995));
#134276=CARTESIAN_POINT('',(-31.85,-65.8583711767947,-55.24995));
#134277=CARTESIAN_POINT('Ctrl Pts',(-32.3064221286262,-65.2727851642229,
-54.74995));
#134278=CARTESIAN_POINT('Ctrl Pts',(-32.3064221286261,-65.2727851642229,
-55.24995));
#134279=CARTESIAN_POINT('Ctrl Pts',(-32.35,-65.7708825132688,-55.24995));
#134280=CARTESIAN_POINT('Ctrl Pts',(-32.0438874372397,-65.2957539735015,
-54.7499500000659));
#134281=CARTESIAN_POINT('Ctrl Pts',(-32.172075011829,-65.2845390139115,
-55.2615708605686));
#134282=CARTESIAN_POINT('Ctrl Pts',(-32.2187326543062,-65.7938513225456,
-55.24995));
#134283=CARTESIAN_POINT('Ctrl Pts',(-31.7844354391267,-65.3184530820656,
-54.8577231271254));
#134284=CARTESIAN_POINT('Ctrl Pts',(-32.0533393021413,-65.2949270424741,
-55.3274496218431));
#134285=CARTESIAN_POINT('Ctrl Pts',(-32.0890066552503,-65.8165504311115,
-55.3038365635632));
#134286=CARTESIAN_POINT('Ctrl Pts',(-31.4141952557525,-65.3508449008926,
-55.2279633105016));
#134287=CARTESIAN_POINT('Ctrl Pts',(-31.8917246342956,-65.3090664937689,
-55.5133819370971));
#134288=CARTESIAN_POINT('Ctrl Pts',(-31.9038865635631,-65.8489422499384,
-55.4889566552503));
#134289=CARTESIAN_POINT('Ctrl Pts',(-31.3064221286917,-65.3602738277431,
-55.4874153086129));
#134290=CARTESIAN_POINT('Ctrl Pts',(-31.8500000000045,-65.3127169262546,
-55.6317784220497));
#134291=CARTESIAN_POINT('Ctrl Pts',(-31.85,-65.8583711767893,-55.6186826543066));
#134292=CARTESIAN_POINT('Ctrl Pts',(-31.3064221286262,-65.3602738277489,
-55.74995));
#134293=CARTESIAN_POINT('Ctrl Pts',(-31.85,-65.3127169262601,-55.74995));
#134294=CARTESIAN_POINT('Ctrl Pts',(-31.85,-65.8583711767947,-55.74995));
#134295=CARTESIAN_POINT('',(-32.35,-65.7708825132688,-55.24995));
#134296=CARTESIAN_POINT('Origin',(-32.35,-65.7708825132688,-54.74995));
#134297=CARTESIAN_POINT('Ctrl Pts',(-32.35,-65.7708825132688,-55.24995));
#134298=CARTESIAN_POINT('Ctrl Pts',(-32.2187326543062,-65.7938513225456,
-55.24995));
#134299=CARTESIAN_POINT('Ctrl Pts',(-32.0890066552503,-65.8165504311115,
-55.3038365635632));
#134300=CARTESIAN_POINT('Ctrl Pts',(-31.9038865635631,-65.8489422499384,
-55.4889566552503));
#134301=CARTESIAN_POINT('Ctrl Pts',(-31.85,-65.8583711767893,-55.6186826543066));
#134302=CARTESIAN_POINT('Ctrl Pts',(-31.85,-65.8583711767947,-55.74995));
#134303=CARTESIAN_POINT('Origin',(-44.2377516955329,-64.7308390050988,-54.74995));
#134304=CARTESIAN_POINT('',(-32.85,-65.7271381815059,-55.24995));
#134305=CARTESIAN_POINT('Origin',(-32.85,-65.7271381815059,-54.74995));
#134306=CARTESIAN_POINT('',(-40.7958880023324,-65.0319630596553,-55.24995));
#134307=CARTESIAN_POINT('Ctrl Pts',(-33.8064221286261,-65.1415521689341,
-55.74995));
#134308=CARTESIAN_POINT('Ctrl Pts',(-33.3499999999999,-65.1814839309712,
-55.74995));
#134309=CARTESIAN_POINT('Ctrl Pts',(-33.35,-65.63964951798,-55.74995));
#134310=CARTESIAN_POINT('Ctrl Pts',(-33.8064221285606,-65.1415521689398,
-55.487415308613));
#134311=CARTESIAN_POINT('Ctrl Pts',(-33.3499999999488,-65.1814839309712,
-55.607847808877));
#134312=CARTESIAN_POINT('Ctrl Pts',(-33.35,-65.6396495179854,-55.6186826543062));
#134313=CARTESIAN_POINT('Ctrl Pts',(-33.6986490015007,-65.1509810957903,
-55.2279633105015));
#134314=CARTESIAN_POINT('Ctrl Pts',(-33.2858662151155,-65.1870949100978,
-55.4680441063706));
#134315=CARTESIAN_POINT('Ctrl Pts',(-33.2961134364373,-65.6490784448363,
-55.4889566552507));
#134316=CARTESIAN_POINT('Ctrl Pts',(-33.3284088181247,-65.1833729146174,
-54.8577231271255));
#134317=CARTESIAN_POINT('Ctrl Pts',(-33.0786175782532,-65.2052268163542,
-55.2822894538758));
#134318=CARTESIAN_POINT('Ctrl Pts',(-33.1109933447493,-65.6814702636632,
-55.3038365635628));
#134319=CARTESIAN_POINT('Ctrl Pts',(-33.0689568200132,-65.2060720231813,
-54.7499500000659));
#134320=CARTESIAN_POINT('Ctrl Pts',(-32.9369589695398,-65.2176203387053,
-55.2386587236917));
#134321=CARTESIAN_POINT('Ctrl Pts',(-32.981267345694,-65.704169372229,-55.24995));
#134322=CARTESIAN_POINT('Ctrl Pts',(-32.8064221286262,-65.22904083246,-54.74995));
#134323=CARTESIAN_POINT('Ctrl Pts',(-32.8064221286261,-65.22904083246,-55.24995));
#134324=CARTESIAN_POINT('Ctrl Pts',(-32.85,-65.7271381815059,-55.24995));
#134325=CARTESIAN_POINT('',(-33.35,-65.63964951798,-55.74995));
#134326=CARTESIAN_POINT('Origin',(-33.85,-65.63964951798,-55.74995));
#134327=CARTESIAN_POINT('Ctrl Pts',(-33.35,-65.63964951798,-55.74995));
#134328=CARTESIAN_POINT('Ctrl Pts',(-33.35,-65.6396495179854,-55.6186826543062));
#134329=CARTESIAN_POINT('Ctrl Pts',(-33.2961134364373,-65.6490784448363,
-55.4889566552507));
#134330=CARTESIAN_POINT('Ctrl Pts',(-33.1109933447493,-65.6814702636632,
-55.3038365635628));
#134331=CARTESIAN_POINT('Ctrl Pts',(-32.981267345694,-65.704169372229,-55.24995));
#134332=CARTESIAN_POINT('Ctrl Pts',(-32.85,-65.7271381815059,-55.24995));
#134333=CARTESIAN_POINT('Origin',(-33.85,-65.63964951798,-52.64995));
#134334=CARTESIAN_POINT('',(-33.35,-65.63964951798,-59.64995));
#134335=CARTESIAN_POINT('Origin',(-33.85,-65.63964951798,-59.64995));
#134336=CARTESIAN_POINT('',(-33.35,-65.63964951798,-55.24995));
#134337=CARTESIAN_POINT('Origin',(-47.0226009489055,-59.9901009689335,-59.64995));
#134338=CARTESIAN_POINT('',(-47.0226009489055,-59.9901009689335,-60.64995));
#134339=CARTESIAN_POINT('Ctrl Pts',(-25.3802177275058,39.943749490528,-60.1097730249189));
#134340=CARTESIAN_POINT('Ctrl Pts',(-25.5227862062494,39.9312763648619,
-60.5923862926587));
#134341=CARTESIAN_POINT('Ctrl Pts',(-25.572468850428,39.5210489290882,-60.8798615124595));
#134342=CARTESIAN_POINT('Ctrl Pts',(-25.1089972874034,39.9674782043536,
-60.2066542280814));
#134343=CARTESIAN_POINT('Ctrl Pts',(-25.2414738675095,39.9482243711148,
-60.6373384822398));
#134344=CARTESIAN_POINT('Ctrl Pts',(-25.2694477113958,39.6036052974814,
-60.9283242463865));
#134345=CARTESIAN_POINT('Ctrl Pts',(-24.8422602775208,40.0127575956439,
-60.3032659617329));
#134346=CARTESIAN_POINT('Ctrl Pts',(-24.9493186357974,39.9900159541718,
-60.6937268873635));
#134347=CARTESIAN_POINT('Ctrl Pts',(-24.9650212889786,39.6997861053784,
-60.9766079791613));
#134348=CARTESIAN_POINT('Ctrl Pts',(-24.3096510677746,40.1491089179394,
-60.4514911807313));
#134349=CARTESIAN_POINT('Ctrl Pts',(-24.3665512677474,40.1299777240875,
-60.7838744940585));
#134350=CARTESIAN_POINT('Ctrl Pts',(-24.3438778196125,39.9224728282123,
-61.0507205920708));
#134351=CARTESIAN_POINT('Ctrl Pts',(-24.0409609718932,40.24165543605,-60.5010370503254));
#134352=CARTESIAN_POINT('Ctrl Pts',(-24.0669512606435,40.2300655352942,
-60.8169267274199));
#134353=CARTESIAN_POINT('Ctrl Pts',(-24.0238031468177,40.0506166841414,
-61.0754935252291));
#134354=CARTESIAN_POINT('Ctrl Pts',(-23.7796330855957,40.3581899105085,
-60.5010370523946));
#134355=CARTESIAN_POINT('Ctrl Pts',(-23.7796330855957,40.3581899105084,
-60.8169267287601));
#134356=CARTESIAN_POINT('Ctrl Pts',(-23.7057274034393,40.1924568448808,
-61.0754935261973));
#134357=CARTESIAN_POINT('',(-25.572468850428,39.5210489290882,-60.8798615124594));
#134358=CARTESIAN_POINT('Origin',(-25.2930619847582,38.9475547924363,-60.1097730249189));
#134359=CARTESIAN_POINT('Ctrl Pts',(-23.7057274034393,40.1924568448808,
-61.0754935261973));
#134360=CARTESIAN_POINT('Ctrl Pts',(-24.0238031468177,40.0506166841414,
-61.0754935252291));
#134361=CARTESIAN_POINT('Ctrl Pts',(-24.3438778196125,39.9224728282123,
-61.0507205920708));
#134362=CARTESIAN_POINT('Ctrl Pts',(-24.9650212889786,39.6997861053784,
-60.9766079791613));
#134363=CARTESIAN_POINT('Ctrl Pts',(-25.2694477113958,39.6036052974814,
-60.9283242463865));
#134364=CARTESIAN_POINT('Ctrl Pts',(-25.572468850428,39.5210489290882,-60.8798615124594));
#134365=CARTESIAN_POINT('Origin',(-4.69960655320655,40.7492486855235,-59.64995));
#134366=CARTESIAN_POINT('',(-31.,38.4482624126576,-60.64995));
#134367=CARTESIAN_POINT('',(-37.,37.923330431502,-60.64995));
#134368=CARTESIAN_POINT('',(-4.69960655320655,40.7492486855235,-60.64995));
#134369=CARTESIAN_POINT('Ctrl Pts',(-36.9564221286262,38.9309628387712,
-59.64995));
#134370=CARTESIAN_POINT('Ctrl Pts',(-36.9564221286271,38.9309628387711,
-59.7808732880376));
#134371=CARTESIAN_POINT('Ctrl Pts',(-36.9575563441365,38.904736860573,-59.9116978933072));
#134372=CARTESIAN_POINT('Ctrl Pts',(-36.9619222489981,38.8037859171731,
-60.153568971423));
#134373=CARTESIAN_POINT('Ctrl Pts',(-36.9651522214979,38.7291006500388,
-60.2644967268049));
#134374=CARTESIAN_POINT('Ctrl Pts',(-36.9732193617859,38.5425676292119,
-60.4496168355682));
#134375=CARTESIAN_POINT('Ctrl Pts',(-36.9780533572402,38.4307932280718,
-60.5237363920407));
#134376=CARTESIAN_POINT('Ctrl Pts',(-36.9885935839748,38.1870760912844,
-60.6239226729819));
#134377=CARTESIAN_POINT('Ctrl Pts',(-36.9942946417934,38.0552529794313,
-60.64995));
#134378=CARTESIAN_POINT('Ctrl Pts',(-37.,37.923330431502,-60.64995));
#134379=CARTESIAN_POINT('Ctrl Pts',(-31.,38.4482624126576,-60.64995));
#134380=CARTESIAN_POINT('Ctrl Pts',(-30.994294641792,38.5801849605867,-60.64995));
#134381=CARTESIAN_POINT('Ctrl Pts',(-30.9885935839752,38.71200807244,-60.6239226729818));
#134382=CARTESIAN_POINT('Ctrl Pts',(-30.9780533572398,38.9557252092273,
-60.5237363920407));
#134383=CARTESIAN_POINT('Ctrl Pts',(-30.9732193617862,39.0674996103677,
-60.4496168355678));
#134384=CARTESIAN_POINT('Ctrl Pts',(-30.9651522214976,39.2540326311941,
-60.2644967268053));
#134385=CARTESIAN_POINT('Ctrl Pts',(-30.9619222489984,39.3287178983286,
-60.153568971423));
#134386=CARTESIAN_POINT('Ctrl Pts',(-30.9575563441362,39.4296688417285,
-59.9116978933072));
#134387=CARTESIAN_POINT('Ctrl Pts',(-30.9564221286278,39.4558948199266,
-59.7808732880376));
#134388=CARTESIAN_POINT('Ctrl Pts',(-30.9564221286262,39.4558948199267,
-59.64995));
#134389=CARTESIAN_POINT('Origin',(-31.,39.9539921689726,-52.64995));
#134390=CARTESIAN_POINT('',(-30.5,39.9539921689726,-55.74995));
#134391=CARTESIAN_POINT('Origin',(-31.,39.9539921689726,-55.74995));
#134392=CARTESIAN_POINT('',(-30.5,39.9539921689726,-59.64995));
#134393=CARTESIAN_POINT('',(-30.5,39.9539921689726,-92.34995));
#134394=CARTESIAN_POINT('Origin',(-31.,39.9539921689726,-59.64995));
#134395=CARTESIAN_POINT('Ctrl Pts',(-29.9564221286262,39.5433834834526,
-54.74995));
#134396=CARTESIAN_POINT('Ctrl Pts',(-29.9564221286262,39.5433834834526,
-55.24995));
#134397=CARTESIAN_POINT('Ctrl Pts',(-30.,40.0414808324985,-55.24995));
#134398=CARTESIAN_POINT('Ctrl Pts',(-30.218956820013,39.520414674174,-54.7499500000658));
#134399=CARTESIAN_POINT('Ctrl Pts',(-30.0869589695403,39.5319629897042,
-55.2386587236916));
#134400=CARTESIAN_POINT('Ctrl Pts',(-30.131267345694,40.0185120232214,-55.24995));
#134401=CARTESIAN_POINT('Ctrl Pts',(-30.4784088181251,39.4977155656101,
-54.8577231271254));
#134402=CARTESIAN_POINT('Ctrl Pts',(-30.2286175782536,39.5195694673468,
-55.2822894538777));
#134403=CARTESIAN_POINT('Ctrl Pts',(-30.2609933447492,39.9958129146559,
-55.3038365635627));
#134404=CARTESIAN_POINT('Ctrl Pts',(-30.8486490015003,39.4653237467829,
-55.2279633105015));
#134405=CARTESIAN_POINT('Ctrl Pts',(-30.4358662151152,39.5014375610904,
-55.4680441063689));
#134406=CARTESIAN_POINT('Ctrl Pts',(-30.4461134364373,39.9634210958289,
-55.4889566552508));
#134407=CARTESIAN_POINT('Ctrl Pts',(-30.9564221285606,39.4558948199325,
-55.4874153086129));
#134408=CARTESIAN_POINT('Ctrl Pts',(-30.4999999999484,39.4958265819666,
-55.6078478088783));
#134409=CARTESIAN_POINT('Ctrl Pts',(-30.5,39.9539921689781,-55.6186826543063));
#134410=CARTESIAN_POINT('Ctrl Pts',(-30.9564221286262,39.4558948199267,
-55.74995));
#134411=CARTESIAN_POINT('Ctrl Pts',(-30.5,39.4958265819639,-55.74995));
#134412=CARTESIAN_POINT('Ctrl Pts',(-30.5,39.9539921689726,-55.74995));
#134413=CARTESIAN_POINT('',(-30.,40.0414808324985,-55.24995));
#134414=CARTESIAN_POINT('Origin',(-30.,40.0414808324985,-54.74995));
#134415=CARTESIAN_POINT('Ctrl Pts',(-30.,40.0414808324985,-55.24995));
#134416=CARTESIAN_POINT('Ctrl Pts',(-30.131267345694,40.0185120232214,-55.24995));
#134417=CARTESIAN_POINT('Ctrl Pts',(-30.2609933447492,39.9958129146559,
-55.3038365635627));
#134418=CARTESIAN_POINT('Ctrl Pts',(-30.4461134364373,39.9634210958289,
-55.4889566552508));
#134419=CARTESIAN_POINT('Ctrl Pts',(-30.5,39.9539921689781,-55.6186826543063));
#134420=CARTESIAN_POINT('Ctrl Pts',(-30.5,39.9539921689726,-55.74995));
#134421=CARTESIAN_POINT('Origin',(-3.70444879364117,42.3420434642203,-54.74995));
#134422=CARTESIAN_POINT('',(-29.5,40.0852251642615,-55.24995));
#134423=CARTESIAN_POINT('Origin',(-29.5,40.0852251642615,-54.74995));
#134424=CARTESIAN_POINT('',(-30.0435778713739,40.0376682627727,-55.24995));
#134425=CARTESIAN_POINT('Ctrl Pts',(-28.4564221286262,39.6746164787415,
-55.74995));
#134426=CARTESIAN_POINT('Ctrl Pts',(-29.,39.6270595772528,-55.74995));
#134427=CARTESIAN_POINT('Ctrl Pts',(-29.,40.1727138277873,-55.74995));
#134428=CARTESIAN_POINT('Ctrl Pts',(-28.4564221286917,39.6746164787358,
-55.487415308613));
#134429=CARTESIAN_POINT('Ctrl Pts',(-29.0000000000046,39.6270595772536,
-55.6317784220498));
#134430=CARTESIAN_POINT('Ctrl Pts',(-29.,40.1727138277819,-55.6186826543062));
#134431=CARTESIAN_POINT('Ctrl Pts',(-28.5641952557521,39.6651875518853,
-55.2279633105015));
#134432=CARTESIAN_POINT('Ctrl Pts',(-29.0417246342951,39.6234091447624,
-55.5133819370971));
#134433=CARTESIAN_POINT('Ctrl Pts',(-29.0538865635627,40.163284900931,-55.4889566552507));
#134434=CARTESIAN_POINT('Ctrl Pts',(-28.9344354391272,39.6327957330582,
-54.8577231271255));
#134435=CARTESIAN_POINT('Ctrl Pts',(-29.2033393021417,39.6092696934658,
-55.3274496218431));
#134436=CARTESIAN_POINT('Ctrl Pts',(-29.2390066552507,40.1308930821041,
-55.3038365635627));
#134437=CARTESIAN_POINT('Ctrl Pts',(-29.1938874372395,39.6100966244942,
-54.7499500000658));
#134438=CARTESIAN_POINT('Ctrl Pts',(-29.3220750118295,39.5988816649146,
-55.2615708605689));
#134439=CARTESIAN_POINT('Ctrl Pts',(-29.368732654306,40.1081939735386,-55.24995));
#134440=CARTESIAN_POINT('Ctrl Pts',(-29.4564221286262,39.5871278152156,
-54.74995));
#134441=CARTESIAN_POINT('Ctrl Pts',(-29.4564221286262,39.5871278152156,
-55.24995));
#134442=CARTESIAN_POINT('Ctrl Pts',(-29.5,40.0852251642615,-55.24995));
#134443=CARTESIAN_POINT('',(-29.,40.1727138277873,-55.74995));
#134444=CARTESIAN_POINT('Origin',(-28.5,40.1727138277873,-55.74995));
#134445=CARTESIAN_POINT('Ctrl Pts',(-29.,40.1727138277873,-55.74995));
#134446=CARTESIAN_POINT('Ctrl Pts',(-29.,40.1727138277819,-55.6186826543062));
#134447=CARTESIAN_POINT('Ctrl Pts',(-29.0538865635627,40.163284900931,-55.4889566552507));
#134448=CARTESIAN_POINT('Ctrl Pts',(-29.2390066552507,40.1308930821041,
-55.3038365635627));
#134449=CARTESIAN_POINT('Ctrl Pts',(-29.368732654306,40.1081939735386,-55.24995));
#134450=CARTESIAN_POINT('Ctrl Pts',(-29.5,40.0852251642615,-55.24995));
#134451=CARTESIAN_POINT('Origin',(-28.5,40.1727138277873,-52.64995));
#134452=CARTESIAN_POINT('',(-29.,40.1727138277873,-59.6524466674074));
#134453=CARTESIAN_POINT('Origin',(-28.5,40.1727138277873,-59.6524466674074));
#134454=CARTESIAN_POINT('',(-29.,40.1727138277874,-92.34995));
#134455=CARTESIAN_POINT('Ctrl Pts',(-25.572468850428,39.5210489290882,-60.8798615124595));
#134456=CARTESIAN_POINT('Ctrl Pts',(-25.5227862062494,39.9312763648619,
-60.5923862926587));
#134457=CARTESIAN_POINT('Ctrl Pts',(-25.3802177275058,39.9437494905281,
-60.1097730249189));
#134458=CARTESIAN_POINT('Ctrl Pts',(-26.059719336348,39.3883003271754,-60.8019346414671));
#134459=CARTESIAN_POINT('Ctrl Pts',(-26.0512576071349,39.8850411082851,
-60.5102318318317));
#134460=CARTESIAN_POINT('Ctrl Pts',(-25.9036128690389,39.8979583490994,
-59.9539737371434));
#134461=CARTESIAN_POINT('Ctrl Pts',(-26.5494003841727,39.2520983829515,
-60.748049450926));
#134462=CARTESIAN_POINT('Ctrl Pts',(-26.5712796028832,39.8395450788764,
-60.4792397999495));
#134463=CARTESIAN_POINT('Ctrl Pts',(-26.4338688782163,39.8515669595299,
-59.8461489023585));
#134464=CARTESIAN_POINT('Ctrl Pts',(-27.529498834359,38.9740545371747,-60.6732320595124));
#134465=CARTESIAN_POINT('Ctrl Pts',(-27.601298997848,39.7494300586015,-60.4901498725136));
#134466=CARTESIAN_POINT('Ctrl Pts',(-27.5031785292772,39.7580144872632,
-59.6965141185183));
#134467=CARTESIAN_POINT('Ctrl Pts',(-28.0200529940657,38.8321810243987,
-60.6528294999755));
#134468=CARTESIAN_POINT('Ctrl Pts',(-28.1179039179461,39.7042329845701,
-60.5392590138154));
#134469=CARTESIAN_POINT('Ctrl Pts',(-28.0425516254864,39.710825455934,-59.6557090289434));
#134470=CARTESIAN_POINT('Ctrl Pts',(-28.5109323535812,38.6876131939284,
-60.6502266229092));
#134471=CARTESIAN_POINT('Ctrl Pts',(-28.5960141520618,39.6624037591722,
-60.6291816703115));
#134472=CARTESIAN_POINT('Ctrl Pts',(-28.5867228014573,39.663216647019,-59.6505032458185));
#134473=CARTESIAN_POINT('',(-28.4933647440941,38.6927858841383,-60.6503275731476));
#134474=CARTESIAN_POINT('Ctrl Pts',(-25.572468850428,39.5210489290882,-60.8798615124594));
#134475=CARTESIAN_POINT('Ctrl Pts',(-26.059719336348,39.3883003271754,-60.8019346414671));
#134476=CARTESIAN_POINT('Ctrl Pts',(-26.5494003841727,39.2520983829515,
-60.748049450926));
#134477=CARTESIAN_POINT('Ctrl Pts',(-27.5236528204355,38.9757129911733,
-60.673678324387));
#134478=CARTESIAN_POINT('Ctrl Pts',(-28.0083489909001,38.8355655623354,
-60.6533187024567));
#134479=CARTESIAN_POINT('Ctrl Pts',(-28.4933647440612,38.6927858841383,
-60.650327573148));
#134480=CARTESIAN_POINT('Ctrl Pts',(-28.4564221286262,39.6746164787415,
-59.6524466674074));
#134481=CARTESIAN_POINT('Ctrl Pts',(-28.4551199545093,39.6747304042147,
-59.7821590925224));
#134482=CARTESIAN_POINT('Ctrl Pts',(-28.4548707416055,39.6494517959669,
-59.9101257001469));
#134483=CARTESIAN_POINT('Ctrl Pts',(-28.4563005932054,39.5761796095201,
-60.0890325252997));
#134484=CARTESIAN_POINT('Ctrl Pts',(-28.4570887248156,39.5455314661108,
-60.1469471546371));
#134485=CARTESIAN_POINT('Ctrl Pts',(-28.4592438293891,39.4746917169037,
-60.2541491598715));
#134486=CARTESIAN_POINT('Ctrl Pts',(-28.4606134496588,39.434276061177,-60.3041245704241));
#134487=CARTESIAN_POINT('Ctrl Pts',(-28.465656656414,39.2976315760154,-60.4428805969007));
#134488=CARTESIAN_POINT('Ctrl Pts',(-28.4702284641343,39.1877232210837,
-60.5175376561534));
#134489=CARTESIAN_POINT('Ctrl Pts',(-28.4808526630789,38.9512642676271,
-60.6191174333591));
#134490=CARTESIAN_POINT('Ctrl Pts',(-28.4870505338491,38.8213938162437,
-60.647315885492));
#134491=CARTESIAN_POINT('Ctrl Pts',(-28.4933647440612,38.6927858841383,
-60.650327573148));
#134492=CARTESIAN_POINT('Origin',(-4.69960655320655,40.7492486855235,-59.64995));
#134493=CARTESIAN_POINT('',(-39.5,37.7046087726872,-60.64995));
#134494=CARTESIAN_POINT('',(-4.69960655320655,40.7492486855235,-60.64995));
#134495=CARTESIAN_POINT('Ctrl Pts',(-39.5,37.7046087726872,-60.64995));
#134496=CARTESIAN_POINT('Ctrl Pts',(-39.4942946417934,37.8365313206165,
-60.64995));
#134497=CARTESIAN_POINT('Ctrl Pts',(-39.4885935839755,37.9683544324696,
-60.6239226729818));
#134498=CARTESIAN_POINT('Ctrl Pts',(-39.4780533572395,38.2120715692569,
-60.5237363920407));
#134499=CARTESIAN_POINT('Ctrl Pts',(-39.4732193617859,38.3238459703974,
-60.4496168355678));
#134500=CARTESIAN_POINT('Ctrl Pts',(-39.4651522214979,38.5103789912237,
-60.2644967268053));
#134501=CARTESIAN_POINT('Ctrl Pts',(-39.4619222489988,38.5850642583582,
-60.153568971423));
#134502=CARTESIAN_POINT('Ctrl Pts',(-39.4575563441359,38.6860152017583,
-59.9116978933072));
#134503=CARTESIAN_POINT('Ctrl Pts',(-39.4564221286291,38.7122411799561,
-59.7808732880376));
#134504=CARTESIAN_POINT('Ctrl Pts',(-39.4564221286262,38.7122411799564,
-59.64995));
#134505=CARTESIAN_POINT('Origin',(-39.5,39.2103385290023,-129.34995));
#134506=CARTESIAN_POINT('',(-39.,39.2103385290022,-59.64995));
#134507=CARTESIAN_POINT('Origin',(-39.5,39.2103385290022,-59.64995));
#134508=CARTESIAN_POINT('',(-39.,39.2103385290022,-55.74995));
#134509=CARTESIAN_POINT('Origin',(-39.5,39.2103385290022,-55.74995));
#134510=CARTESIAN_POINT('',(-39.,39.2103385290022,-59.64995));
#134511=CARTESIAN_POINT('Ctrl Pts',(-38.4564221286262,38.7997298434823,
-54.74995));
#134512=CARTESIAN_POINT('Ctrl Pts',(-38.4564221286261,38.7997298434823,
-55.2499499999999));
#134513=CARTESIAN_POINT('Ctrl Pts',(-38.5,39.2978271925282,-55.24995));
#134514=CARTESIAN_POINT('Ctrl Pts',(-38.7189568200132,38.7767610342036,
-54.7499500000658));
#134515=CARTESIAN_POINT('Ctrl Pts',(-38.5869589695399,38.788309349734,-55.2386587236917));
#134516=CARTESIAN_POINT('Ctrl Pts',(-38.6312673456941,39.2748583832512,
-55.24995));
#134517=CARTESIAN_POINT('Ctrl Pts',(-38.9784088181247,38.7540619256397,
-54.8577231271255));
#134518=CARTESIAN_POINT('Ctrl Pts',(-38.7286175782541,38.7759158273764,
-55.2822894538767));
#134519=CARTESIAN_POINT('Ctrl Pts',(-38.7609933447493,39.2521592746855,
-55.3038365635627));
#134520=CARTESIAN_POINT('Ctrl Pts',(-39.3486490015007,38.7216701068126,
-55.2279633105015));
#134521=CARTESIAN_POINT('Ctrl Pts',(-38.9358662151147,38.7577839211201,
-55.4680441063697));
#134522=CARTESIAN_POINT('Ctrl Pts',(-38.9461134364373,39.2197674558585,
-55.4889566552507));
#134523=CARTESIAN_POINT('Ctrl Pts',(-39.4564221285606,38.7122411799621,
-55.487415308613));
#134524=CARTESIAN_POINT('Ctrl Pts',(-38.9999999999489,38.7521729419962,
-55.6078478088777));
#134525=CARTESIAN_POINT('Ctrl Pts',(-39.,39.2103385290077,-55.6186826543063));
#134526=CARTESIAN_POINT('Ctrl Pts',(-39.4564221286262,38.7122411799564,
-55.74995));
#134527=CARTESIAN_POINT('Ctrl Pts',(-39.,38.7521729419935,-55.74995));
#134528=CARTESIAN_POINT('Ctrl Pts',(-39.,39.2103385290022,-55.74995));
#134529=CARTESIAN_POINT('',(-38.5,39.2978271925282,-55.24995));
#134530=CARTESIAN_POINT('Origin',(-38.5,39.2978271925282,-54.74995));
#134531=CARTESIAN_POINT('Ctrl Pts',(-38.5,39.2978271925282,-55.24995));
#134532=CARTESIAN_POINT('Ctrl Pts',(-38.6312673456941,39.2748583832512,
-55.24995));
#134533=CARTESIAN_POINT('Ctrl Pts',(-38.7609933447493,39.2521592746855,
-55.3038365635627));
#134534=CARTESIAN_POINT('Ctrl Pts',(-38.9461134364373,39.2197674558585,
-55.4889566552507));
#134535=CARTESIAN_POINT('Ctrl Pts',(-39.,39.2103385290077,-55.6186826543063));
#134536=CARTESIAN_POINT('Ctrl Pts',(-39.,39.2103385290022,-55.74995));
#134537=CARTESIAN_POINT('Origin',(-3.70444879364117,42.3420434642203,-54.74995));
#134538=CARTESIAN_POINT('',(-38.,39.3415715242911,-55.24995));
#134539=CARTESIAN_POINT('Origin',(-38.,39.3415715242911,-54.74995));
#134540=CARTESIAN_POINT('',(-38.5435778713738,39.2940146228024,-55.24995));
#134541=CARTESIAN_POINT('Ctrl Pts',(-36.9564221286262,38.9309628387712,
-55.74995));
#134542=CARTESIAN_POINT('Ctrl Pts',(-37.5000000000001,38.8834059372824,
-55.74995));
#134543=CARTESIAN_POINT('Ctrl Pts',(-37.5,39.4290601878171,-55.74995));
#134544=CARTESIAN_POINT('Ctrl Pts',(-36.9564221286917,38.9309628387654,
-55.487415308613));
#134545=CARTESIAN_POINT('Ctrl Pts',(-37.5000000000036,38.8834059372834,
-55.6317784220504));
#134546=CARTESIAN_POINT('Ctrl Pts',(-37.5,39.4290601878116,-55.6186826543065));
#134547=CARTESIAN_POINT('Ctrl Pts',(-37.0641952557516,38.9215339119149,
-55.2279633105015));
#134548=CARTESIAN_POINT('Ctrl Pts',(-37.5417246342956,38.879755504792,-55.5133819370962));
#134549=CARTESIAN_POINT('Ctrl Pts',(-37.5538865635632,39.4196312609607,
-55.4889566552503));
#134550=CARTESIAN_POINT('Ctrl Pts',(-37.4344354391277,38.8891420930878,
-54.8577231271255));
#134551=CARTESIAN_POINT('Ctrl Pts',(-37.7033393021412,38.8656160534955,
-55.3274496218441));
#134552=CARTESIAN_POINT('Ctrl Pts',(-37.7390066552503,39.3872394421337,
-55.3038365635632));
#134553=CARTESIAN_POINT('Ctrl Pts',(-37.6938874372391,38.8664429845239,
-54.7499500000658));
#134554=CARTESIAN_POINT('Ctrl Pts',(-37.8220750118298,38.855228024944,-55.2615708605686));
#134555=CARTESIAN_POINT('Ctrl Pts',(-37.8687326543062,39.3645403335679,
-55.24995));
#134556=CARTESIAN_POINT('Ctrl Pts',(-37.9564221286262,38.8434741752452,
-54.74995));
#134557=CARTESIAN_POINT('Ctrl Pts',(-37.9564221286261,38.8434741752452,
-55.2499499999999));
#134558=CARTESIAN_POINT('Ctrl Pts',(-38.,39.3415715242911,-55.24995));
#134559=CARTESIAN_POINT('',(-37.5,39.4290601878171,-55.74995));
#134560=CARTESIAN_POINT('Origin',(-37.,39.4290601878171,-55.74995));
#134561=CARTESIAN_POINT('Ctrl Pts',(-37.5,39.4290601878171,-55.74995));
#134562=CARTESIAN_POINT('Ctrl Pts',(-37.5,39.4290601878116,-55.6186826543065));
#134563=CARTESIAN_POINT('Ctrl Pts',(-37.5538865635632,39.4196312609607,
-55.4889566552503));
#134564=CARTESIAN_POINT('Ctrl Pts',(-37.7390066552503,39.3872394421337,
-55.3038365635632));
#134565=CARTESIAN_POINT('Ctrl Pts',(-37.8687326543062,39.3645403335679,
-55.24995));
#134566=CARTESIAN_POINT('Ctrl Pts',(-38.,39.3415715242911,-55.24995));
#134567=CARTESIAN_POINT('Origin',(-37.,39.4290601878171,-92.34995));
#134568=CARTESIAN_POINT('',(-37.5,39.429060187817,-59.64995));
#134569=CARTESIAN_POINT('Origin',(-37.,39.4290601878171,-59.64995));
#134570=CARTESIAN_POINT('',(-37.5,39.4290601878171,-92.34995));
#134571=CARTESIAN_POINT('Origin',(-47.0226009489055,34.0551009288773,-59.64995));
#134572=CARTESIAN_POINT('',(-47.0226009489055,34.0551009288773,-60.64995));
#134573=CARTESIAN_POINT('Origin',(-53.7167487055517,-8.26789346682159,-59.64995));
#134574=CARTESIAN_POINT('',(-50.6819512673597,26.41999998,-60.64995));
#134575=CARTESIAN_POINT('',(-51.1762622162812,20.76999998,-60.64995));
#134576=CARTESIAN_POINT('',(-53.7167487055517,-8.26789346682159,-60.64995));
#134577=CARTESIAN_POINT('Ctrl Pts',(-52.1838946235503,20.7264221086262,
-59.64995));
#134578=CARTESIAN_POINT('Ctrl Pts',(-52.1838946235501,20.7264221086281,
-59.7808732880376));
#134579=CARTESIAN_POINT('Ctrl Pts',(-52.1576686453522,20.7275563241362,
-59.9116978933072));
#134580=CARTESIAN_POINT('Ctrl Pts',(-52.0567177019522,20.7319222289985,
-60.153568971423));
#134581=CARTESIAN_POINT('Ctrl Pts',(-51.9820324348179,20.7351522014979,
-60.264496726805));
#134582=CARTESIAN_POINT('Ctrl Pts',(-51.7954994139911,20.7432193417859,
-60.4496168355681));
#134583=CARTESIAN_POINT('Ctrl Pts',(-51.6837250128509,20.7480533372398,
-60.5237363920407));
#134584=CARTESIAN_POINT('Ctrl Pts',(-51.4400078760636,20.7585935639752,
-60.6239226729818));
#134585=CARTESIAN_POINT('Ctrl Pts',(-51.3081847642104,20.764294621792,-60.64995));
#134586=CARTESIAN_POINT('Ctrl Pts',(-51.1762622162812,20.76999998,-60.64995));
#134587=CARTESIAN_POINT('Ctrl Pts',(-50.6819512673597,26.41999998,-60.64995));
#134588=CARTESIAN_POINT('Ctrl Pts',(-50.8138738152888,26.4142946217921,
-60.64995));
#134589=CARTESIAN_POINT('Ctrl Pts',(-50.9456969271423,26.4085935639752,
-60.6239226729817));
#134590=CARTESIAN_POINT('Ctrl Pts',(-51.1894140639292,26.3980533372399,
-60.5237363920408));
#134591=CARTESIAN_POINT('Ctrl Pts',(-51.3011884650699,26.3932193417862,
-60.4496168355678));
#134592=CARTESIAN_POINT('Ctrl Pts',(-51.4877214858962,26.3851522014976,
-60.2644967268053));
#134593=CARTESIAN_POINT('Ctrl Pts',(-51.5624067530308,26.3819222289988,
-60.1535689714229));
#134594=CARTESIAN_POINT('Ctrl Pts',(-51.6633576964307,26.3775563241358,
-59.9116978933072));
#134595=CARTESIAN_POINT('Ctrl Pts',(-51.6895836746287,26.3764221086278,
-59.7808732880375));
#134596=CARTESIAN_POINT('Ctrl Pts',(-51.6895836746288,26.3764221086262,
-59.64995));
#134597=CARTESIAN_POINT('Origin',(-52.1876810236747,26.41999998,-52.64995));
#134598=CARTESIAN_POINT('',(-52.1876810236747,26.91999998,-55.74995));
#134599=CARTESIAN_POINT('Origin',(-52.1876810236747,26.41999998,-55.74995));
#134600=CARTESIAN_POINT('',(-52.1876810236747,26.91999998,-59.64995));
#134601=CARTESIAN_POINT('',(-52.1876810236747,26.91999998,-55.24995));
#134602=CARTESIAN_POINT('Origin',(-52.1876810236747,26.41999998,-59.64995));
#134603=CARTESIAN_POINT('Ctrl Pts',(-51.6020950111029,27.3764221086262,
-54.74995));
#134604=CARTESIAN_POINT('Ctrl Pts',(-51.6020950111029,27.3764221086262,
-55.2499499999999));
#134605=CARTESIAN_POINT('Ctrl Pts',(-52.1001923601488,27.41999998,-55.24995));
#134606=CARTESIAN_POINT('Ctrl Pts',(-51.6250638203816,27.1138874172394,
-54.7499500000658));
#134607=CARTESIAN_POINT('Ctrl Pts',(-51.6138488608016,27.2420749918296,
-55.2615708605686));
#134608=CARTESIAN_POINT('Ctrl Pts',(-52.1231611694256,27.2887326343059,
-55.24995));
#134609=CARTESIAN_POINT('Ctrl Pts',(-51.6477629289455,26.8544354191273,
-54.8577231271254));
#134610=CARTESIAN_POINT('Ctrl Pts',(-51.6242368893532,27.1233392821413,
-55.3274496218423));
#134611=CARTESIAN_POINT('Ctrl Pts',(-52.1458602779915,27.1590066352508,
-55.3038365635627));
#134612=CARTESIAN_POINT('Ctrl Pts',(-51.6801547477726,26.484195235752,-55.2279633105015));
#134613=CARTESIAN_POINT('Ctrl Pts',(-51.6383763406497,26.9617246142954,
-55.5133819370981));
#134614=CARTESIAN_POINT('Ctrl Pts',(-52.1782520968184,26.9738865435627,
-55.4889566552508));
#134615=CARTESIAN_POINT('Ctrl Pts',(-51.6895836746231,26.3764221086917,
-55.4874153086129));
#134616=CARTESIAN_POINT('Ctrl Pts',(-51.6420267731401,26.9199999800045,
-55.6317784220491));
#134617=CARTESIAN_POINT('Ctrl Pts',(-52.1876810236693,26.91999998,-55.6186826543062));
#134618=CARTESIAN_POINT('Ctrl Pts',(-51.6895836746288,26.3764221086262,
-55.74995));
#134619=CARTESIAN_POINT('Ctrl Pts',(-51.6420267731401,26.91999998,-55.74995));
#134620=CARTESIAN_POINT('Ctrl Pts',(-52.1876810236747,26.91999998,-55.74995));
#134621=CARTESIAN_POINT('',(-52.1001923601488,27.41999998,-55.24995));
#134622=CARTESIAN_POINT('Origin',(-52.1001923601488,27.41999998,-54.74995));
#134623=CARTESIAN_POINT('Ctrl Pts',(-52.1001923601488,27.41999998,-55.24995));
#134624=CARTESIAN_POINT('Ctrl Pts',(-52.1231611694256,27.2887326343059,
-55.24995));
#134625=CARTESIAN_POINT('Ctrl Pts',(-52.1458602779915,27.1590066352508,
-55.3038365635627));
#134626=CARTESIAN_POINT('Ctrl Pts',(-52.1782520968184,26.9738865435627,
-55.4889566552508));
#134627=CARTESIAN_POINT('Ctrl Pts',(-52.1876810236693,26.91999998,-55.6186826543062));
#134628=CARTESIAN_POINT('Ctrl Pts',(-52.1876810236747,26.91999998,-55.74995));
#134629=CARTESIAN_POINT('Origin',(-51.7633389850707,31.2702516755049,-54.74995));
#134630=CARTESIAN_POINT('',(-52.0564480283858,27.91999998,-55.24995));
#134631=CARTESIAN_POINT('Origin',(-52.0564480283858,27.91999998,-54.74995));
#134632=CARTESIAN_POINT('',(-52.0733761857257,27.7265102562164,-55.24995));
#134633=CARTESIAN_POINT('Ctrl Pts',(-51.4708620158141,28.8764221086262,
-55.74995));
#134634=CARTESIAN_POINT('Ctrl Pts',(-51.5107937778512,28.41999998,-55.74995));
#134635=CARTESIAN_POINT('Ctrl Pts',(-51.9689593648599,28.41999998,-55.74995));
#134636=CARTESIAN_POINT('Ctrl Pts',(-51.4708620158198,28.8764221085606,
-55.4874153086129));
#134637=CARTESIAN_POINT('Ctrl Pts',(-51.5107937778567,28.4199999799462,
-55.6078478088784));
#134638=CARTESIAN_POINT('Ctrl Pts',(-51.9689593648654,28.41999998,-55.6186826543062));
#134639=CARTESIAN_POINT('Ctrl Pts',(-51.4802909426703,28.7686489815003,
-55.2279633105015));
#134640=CARTESIAN_POINT('Ctrl Pts',(-51.5164047569777,28.3558661951151,
-55.4680441063688));
#134641=CARTESIAN_POINT('Ctrl Pts',(-51.9783882917162,28.3661134164373,
-55.4889566552507));
#134642=CARTESIAN_POINT('Ctrl Pts',(-51.5126827614974,28.3984087981251,
-54.8577231271254));
#134643=CARTESIAN_POINT('Ctrl Pts',(-51.5345366632341,28.1486175582537,
-55.2822894538777));
#134644=CARTESIAN_POINT('Ctrl Pts',(-52.0107801105432,28.1809933247493,
-55.3038365635627));
#134645=CARTESIAN_POINT('Ctrl Pts',(-51.5353818700614,28.1389568000129,
-54.7499500000658));
#134646=CARTESIAN_POINT('Ctrl Pts',(-51.5469301855916,28.0069589495408,
-55.2386587236988));
#134647=CARTESIAN_POINT('Ctrl Pts',(-52.033479219109,28.0512673256941,-55.24995));
#134648=CARTESIAN_POINT('Ctrl Pts',(-51.55835067934,27.8764221086262,-54.74995));
#134649=CARTESIAN_POINT('Ctrl Pts',(-51.5583506793399,27.8764221086261,
-55.24995));
#134650=CARTESIAN_POINT('Ctrl Pts',(-52.0564480283858,27.91999998,-55.24995));
#134651=CARTESIAN_POINT('',(-51.9689593648599,28.41999998,-55.74995));
#134652=CARTESIAN_POINT('Origin',(-51.9689593648599,28.91999998,-55.74995));
#134653=CARTESIAN_POINT('Ctrl Pts',(-51.9689593648599,28.41999998,-55.74995));
#134654=CARTESIAN_POINT('Ctrl Pts',(-51.9689593648654,28.41999998,-55.6186826543062));
#134655=CARTESIAN_POINT('Ctrl Pts',(-51.9783882917162,28.3661134164373,
-55.4889566552507));
#134656=CARTESIAN_POINT('Ctrl Pts',(-52.0107801105432,28.1809933247493,
-55.3038365635627));
#134657=CARTESIAN_POINT('Ctrl Pts',(-52.033479219109,28.0512673256941,-55.24995));
#134658=CARTESIAN_POINT('Ctrl Pts',(-52.0564480283858,27.91999998,-55.24995));
#134659=CARTESIAN_POINT('Origin',(-51.9689593648599,28.91999998,-52.64995));
#134660=CARTESIAN_POINT('',(-51.9689593648599,28.41999998,-59.64995));
#134661=CARTESIAN_POINT('Origin',(-51.9689593648599,28.91999998,-59.64995));
#134662=CARTESIAN_POINT('',(-51.9689593648599,28.41999998,-55.24995));
#134663=CARTESIAN_POINT('Origin',(-53.7167487055517,-8.26789346682159,-59.64995));
#134664=CARTESIAN_POINT('',(-50.4632296085449,28.91999998,-60.64995));
#134665=CARTESIAN_POINT('',(-53.7167487055517,-8.26789346682159,-60.64995));
#134666=CARTESIAN_POINT('Ctrl Pts',(-51.4708620158141,28.8764221086262,
-59.64995));
#134667=CARTESIAN_POINT('Ctrl Pts',(-51.4708620158139,28.8764221086278,
-59.7808732880376));
#134668=CARTESIAN_POINT('Ctrl Pts',(-51.4446360376159,28.8775563241362,
-59.9116978933072));
#134669=CARTESIAN_POINT('Ctrl Pts',(-51.343685094216,28.8819222289984,-60.153568971423));
#134670=CARTESIAN_POINT('Ctrl Pts',(-51.2689998270813,28.8851522014976,
-60.2644967268053));
#134671=CARTESIAN_POINT('Ctrl Pts',(-51.0824668062551,28.8932193417862,
-60.4496168355678));
#134672=CARTESIAN_POINT('Ctrl Pts',(-50.9706924051143,28.8980533372399,
-60.5237363920408));
#134673=CARTESIAN_POINT('Ctrl Pts',(-50.7269752683276,28.9085935639752,
-60.6239226729817));
#134674=CARTESIAN_POINT('Ctrl Pts',(-50.5951521564739,28.9142946217921,
-60.64995));
#134675=CARTESIAN_POINT('Ctrl Pts',(-50.4632296085449,28.91999998,-60.64995));
#134676=CARTESIAN_POINT('Ctrl Pts',(-52.8969272312866,12.5764221086262,
-55.74995));
#134677=CARTESIAN_POINT('Ctrl Pts',(-52.9368589933237,12.11999998,-55.74995));
#134678=CARTESIAN_POINT('Ctrl Pts',(-53.3950245803324,12.11999998,-55.74995));
#134679=CARTESIAN_POINT('Ctrl Pts',(-52.8969272312908,12.5764221085778,
-55.5560711921817));
#134680=CARTESIAN_POINT('Ctrl Pts',(-52.9368589933258,12.1199999799653,
-55.6451138110298));
#134681=CARTESIAN_POINT('Ctrl Pts',(-53.3950245803365,12.11999998,-55.6530085475485));
#134682=CARTESIAN_POINT('Ctrl Pts',(-52.9019494572905,12.5190178027248,
-55.3638118539785));
#134683=CARTESIAN_POINT('Ctrl Pts',(-52.9398152308639,12.0862100303001,
-55.5412722521129));
#134684=CARTESIAN_POINT('Ctrl Pts',(-53.4000464934415,12.0912996152796,
-55.5568836545521));
#134685=CARTESIAN_POINT('Ctrl Pts',(-52.9112495105564,12.4127177074772,
-55.2016711737242));
#134686=CARTESIAN_POINT('Ctrl Pts',(-52.9450883668941,12.0259378096709,
-55.4571865884902));
#134687=CARTESIAN_POINT('Ctrl Pts',(-53.4093468596023,12.0381477794255,
-55.4758105868621));
#134688=CARTESIAN_POINT('',(-53.3950245803324,12.11999998,-55.74995));
#134689=CARTESIAN_POINT('Origin',(-53.3950245803325,12.61999998,-55.74995));
#134690=CARTESIAN_POINT('Origin',(-53.4672819406082,11.7070472760343,-55.7239598691462));
#134691=CARTESIAN_POINT('Origin',(-53.3950245803324,12.61999998,-55.24995));
#134692=CARTESIAN_POINT('',(-53.3950245803324,12.11999998,-60.0627241236309));
#134693=CARTESIAN_POINT('Origin',(-53.3950245803325,12.61999998,-60.0627241236309));
#134694=CARTESIAN_POINT('',(-53.3950245803324,12.11999998,-55.24995));
#134695=CARTESIAN_POINT('Ctrl Pts',(-51.6244217512084,15.6475130558006,
-60.64995));
#134696=CARTESIAN_POINT('Ctrl Pts',(-52.6206164493002,15.7346687985482,
-60.64995));
#134697=CARTESIAN_POINT('Ctrl Pts',(-52.6206164493001,15.7346687985483,
-59.64995));
#134698=CARTESIAN_POINT('Ctrl Pts',(-51.7744992817202,15.1392139958173,
-60.64995));
#134699=CARTESIAN_POINT('Ctrl Pts',(-52.6636514122595,15.2427769209991,
-60.5499446302911));
#134700=CARTESIAN_POINT('Ctrl Pts',(-52.6699713539896,15.1705396565499,
-59.6499500021592));
#134701=CARTESIAN_POINT('Ctrl Pts',(-51.921686259274,14.6313008059217,-60.6692877368673));
#134702=CARTESIAN_POINT('Ctrl Pts',(-52.7104450878319,14.7079227618566,
-60.4941916839025));
#134703=CARTESIAN_POINT('Ctrl Pts',(-52.7188714030742,14.6116095379051,
-59.6886254732604));
#134704=CARTESIAN_POINT('Ctrl Pts',(-52.209973495227,13.6164898397673,-60.7441942307015));
#134705=CARTESIAN_POINT('Ctrl Pts',(-52.8037229951722,13.64175140224,-60.4769182500017));
#134706=CARTESIAN_POINT('Ctrl Pts',(-52.8157906892286,13.5038170280144,
-59.8384384618772));
#134707=CARTESIAN_POINT('Ctrl Pts',(-52.3511088881553,13.109439201609,-60.799180633384));
#134708=CARTESIAN_POINT('Ctrl Pts',(-52.850859560631,13.1029779936029,-60.5072438893719));
#134709=CARTESIAN_POINT('Ctrl Pts',(-52.8638414531199,12.954594283549,-59.9484723594913));
#134710=CARTESIAN_POINT('Ctrl Pts',(-52.4885489491165,12.6049688303995,
-60.8798615124595));
#134711=CARTESIAN_POINT('Ctrl Pts',(-52.8987763848902,12.5552861862208,
-60.5923862926586));
#134712=CARTESIAN_POINT('Ctrl Pts',(-52.9112495105564,12.4127177074772,
-60.1097730249189));
#134713=CARTESIAN_POINT('',(-51.6244217512084,15.6475130558006,-60.64995));
#134714=CARTESIAN_POINT('Origin',(-51.6244217512084,15.6475130558006,-59.64995));
#134715=CARTESIAN_POINT('',(-52.4885489491165,12.6049688303995,-60.8798615124595));
#134716=CARTESIAN_POINT('Ctrl Pts',(-51.6244217512084,15.6475130558006,
-60.64995));
#134717=CARTESIAN_POINT('Ctrl Pts',(-51.7744993530724,15.1392140041279,
-60.6499499919748));
#134718=CARTESIAN_POINT('Ctrl Pts',(-51.9216863254076,14.6313008123461,
-60.6692877221863));
#134719=CARTESIAN_POINT('Ctrl Pts',(-52.2099735489448,13.6164898420528,
-60.7441942065205));
#134720=CARTESIAN_POINT('Ctrl Pts',(-52.3511089348818,13.1094392010049,
-60.799180606088));
#134721=CARTESIAN_POINT('Ctrl Pts',(-52.4885489491165,12.6049688303995,
-60.8798615124595));
#134722=CARTESIAN_POINT('',(-52.81219032515,12.5218539749099,-60.5055220850798));
#134723=CARTESIAN_POINT('Origin',(-51.9150548124647,12.3255619647296,-60.1097730249189));
#134724=CARTESIAN_POINT('Ctrl Pts',(-52.8969272285826,12.5764221083876,
-60.0627241236307));
#134725=CARTESIAN_POINT('Ctrl Pts',(-52.8973718975191,12.5713069363321,
-60.1041418566377));
#134726=CARTESIAN_POINT('Ctrl Pts',(-52.895580098221,12.5662216141313,-60.1452630246831));
#134727=CARTESIAN_POINT('Ctrl Pts',(-52.8916250763018,12.5611890572108,
-60.1859586821439));
#134728=CARTESIAN_POINT('Ctrl Pts',(-52.8875910253699,12.5560559400376,
-60.2274675178095));
#134729=CARTESIAN_POINT('Ctrl Pts',(-52.8813073672434,12.550978356838,-60.2685357471677));
#134730=CARTESIAN_POINT('Ctrl Pts',(-52.872806509014,12.5459803352207,-60.3090583620907));
#134731=CARTESIAN_POINT('Ctrl Pts',(-52.8644535955316,12.5410692967085,
-60.3488757413946));
#134732=CARTESIAN_POINT('Ctrl Pts',(-52.8539596832267,12.5362356727488,
-60.3881685164046));
#134733=CARTESIAN_POINT('Ctrl Pts',(-52.8413080863257,12.5314926818733,
-60.4268350961324));
#134734=CARTESIAN_POINT('Ctrl Pts',(-52.8326250159684,12.5282374624889,
-60.4533728237313));
#134735=CARTESIAN_POINT('Ctrl Pts',(-52.8229245067539,12.5250247275077,
-60.4796155210117));
#134736=CARTESIAN_POINT('Ctrl Pts',(-52.81219032515,12.5218539749099,-60.5055220850798));
#134737=CARTESIAN_POINT('Origin',(-53.7167487055517,-8.26789346682159,-59.64995));
#134738=CARTESIAN_POINT('',(-51.394983875096,18.26999998,-60.64995));
#134739=CARTESIAN_POINT('',(-53.7167487055517,-8.26789346682159,-60.64995));
#134740=CARTESIAN_POINT('Ctrl Pts',(-51.394983875096,18.26999998,-60.64995));
#134741=CARTESIAN_POINT('Ctrl Pts',(-51.5269064230252,18.264294621793,-60.64995));
#134742=CARTESIAN_POINT('Ctrl Pts',(-51.6587295348784,18.2585935639752,
-60.6239226729819));
#134743=CARTESIAN_POINT('Ctrl Pts',(-51.9024466716657,18.2480533372399,
-60.5237363920407));
#134744=CARTESIAN_POINT('Ctrl Pts',(-52.0142210728062,18.2432193417862,
-60.4496168355678));
#134745=CARTESIAN_POINT('Ctrl Pts',(-52.2007540936325,18.2351522014976,
-60.2644967268053));
#134746=CARTESIAN_POINT('Ctrl Pts',(-52.2754393607673,18.2319222289985,
-60.1535689714224));
#134747=CARTESIAN_POINT('Ctrl Pts',(-52.3763903041667,18.2275563241362,
-59.9116978933078));
#134748=CARTESIAN_POINT('Ctrl Pts',(-52.402616282365,18.2264221086281,-59.7808732880371));
#134749=CARTESIAN_POINT('Ctrl Pts',(-52.4026162823651,18.2264221086262,
-59.64995));
#134750=CARTESIAN_POINT('Origin',(-52.900713631411,18.26999998,-52.64995));
#134751=CARTESIAN_POINT('',(-52.900713631411,18.76999998,-59.64995));
#134752=CARTESIAN_POINT('Origin',(-52.900713631411,18.26999998,-59.64995));
#134753=CARTESIAN_POINT('',(-52.900713631411,18.76999998,-55.74995));
#134754=CARTESIAN_POINT('Origin',(-52.900713631411,18.26999998,-55.74995));
#134755=CARTESIAN_POINT('',(-52.900713631411,18.76999998,-55.24995));
#134756=CARTESIAN_POINT('Ctrl Pts',(-52.3151276188392,19.2264221086262,
-54.74995));
#134757=CARTESIAN_POINT('Ctrl Pts',(-52.3151276188392,19.2264221086262,
-55.2499499999999));
#134758=CARTESIAN_POINT('Ctrl Pts',(-52.8132249678851,19.26999998,-55.24995));
#134759=CARTESIAN_POINT('Ctrl Pts',(-52.3380964281178,18.9638874172394,
-54.7499500000658));
#134760=CARTESIAN_POINT('Ctrl Pts',(-52.3268814685379,19.09207499183,-55.2615708605685));
#134761=CARTESIAN_POINT('Ctrl Pts',(-52.8361937771619,19.1387326343059,
-55.24995));
#134762=CARTESIAN_POINT('Ctrl Pts',(-52.3607955366818,18.7044354191273,
-54.8577231271254));
#134763=CARTESIAN_POINT('Ctrl Pts',(-52.3372694970894,18.9733392821407,
-55.3274496218431));
#134764=CARTESIAN_POINT('Ctrl Pts',(-52.8588928857277,19.0090066352508,
-55.3038365635627));
#134765=CARTESIAN_POINT('Ctrl Pts',(-52.3931873555089,18.334195235752,-55.2279633105015));
#134766=CARTESIAN_POINT('Ctrl Pts',(-52.351408948386,18.8117246142959,-55.5133819370972));
#134767=CARTESIAN_POINT('Ctrl Pts',(-52.8912847045547,18.8238865435627,
-55.4889566552508));
#134768=CARTESIAN_POINT('Ctrl Pts',(-52.4026162823594,18.2264221086918,
-55.4874153086129));
#134769=CARTESIAN_POINT('Ctrl Pts',(-52.3550593808763,18.7699999800045,
-55.6317784220498));
#134770=CARTESIAN_POINT('Ctrl Pts',(-52.9007136314055,18.76999998,-55.6186826543062));
#134771=CARTESIAN_POINT('Ctrl Pts',(-52.4026162823651,18.2264221086262,
-55.74995));
#134772=CARTESIAN_POINT('Ctrl Pts',(-52.3550593808763,18.76999998,-55.74995));
#134773=CARTESIAN_POINT('Ctrl Pts',(-52.900713631411,18.76999998,-55.74995));
#134774=CARTESIAN_POINT('',(-52.8132249678851,19.26999998,-55.24995));
#134775=CARTESIAN_POINT('Origin',(-52.8132249678851,19.26999998,-54.74995));
#134776=CARTESIAN_POINT('Ctrl Pts',(-52.8132249678851,19.26999998,-55.24995));
#134777=CARTESIAN_POINT('Ctrl Pts',(-52.8361937771619,19.1387326343059,
-55.24995));
#134778=CARTESIAN_POINT('Ctrl Pts',(-52.8588928857277,19.0090066352508,
-55.3038365635627));
#134779=CARTESIAN_POINT('Ctrl Pts',(-52.8912847045547,18.8238865435627,
-55.4889566552508));
#134780=CARTESIAN_POINT('Ctrl Pts',(-52.9007136314055,18.76999998,-55.6186826543062));
#134781=CARTESIAN_POINT('Ctrl Pts',(-52.900713631411,18.76999998,-55.74995));
#134782=CARTESIAN_POINT('Origin',(-51.7633389850707,31.2702516755049,-54.74995));
#134783=CARTESIAN_POINT('',(-52.7694806361221,19.76999998,-55.24995));
#134784=CARTESIAN_POINT('Origin',(-52.7694806361221,19.76999998,-54.74995));
#134785=CARTESIAN_POINT('',(-52.0733761857257,27.7265102562164,-55.24995));
#134786=CARTESIAN_POINT('Ctrl Pts',(-52.1838946235503,20.7264221086262,
-55.74995));
#134787=CARTESIAN_POINT('Ctrl Pts',(-52.2238263855875,20.26999998,-55.74995));
#134788=CARTESIAN_POINT('Ctrl Pts',(-52.6819919725962,20.26999998,-55.74995));
#134789=CARTESIAN_POINT('Ctrl Pts',(-52.1838946235561,20.7264221085606,
-55.487415308613));
#134790=CARTESIAN_POINT('Ctrl Pts',(-52.2238263855902,20.2699999799516,
-55.6078478088784));
#134791=CARTESIAN_POINT('Ctrl Pts',(-52.6819919726017,20.26999998,-55.6186826543063));
#134792=CARTESIAN_POINT('Ctrl Pts',(-52.1933235504066,20.6186489815003,
-55.2279633105015));
#134793=CARTESIAN_POINT('Ctrl Pts',(-52.229437364714,20.2058661951152,-55.4680441063689));
#134794=CARTESIAN_POINT('Ctrl Pts',(-52.6914208994525,20.2161134164373,
-55.4889566552507));
#134795=CARTESIAN_POINT('Ctrl Pts',(-52.2257153692336,20.2484087981252,
-54.8577231271255));
#134796=CARTESIAN_POINT('Ctrl Pts',(-52.2475692709704,19.9986175582537,
-55.2822894538776));
#134797=CARTESIAN_POINT('Ctrl Pts',(-52.7238127182794,20.0309933247493,
-55.3038365635627));
#134798=CARTESIAN_POINT('Ctrl Pts',(-52.2484144777976,19.9889568000129,
-54.7499500000658));
#134799=CARTESIAN_POINT('Ctrl Pts',(-52.2599627933277,19.8569589495402,
-55.2386587236914));
#134800=CARTESIAN_POINT('Ctrl Pts',(-52.746511826845,19.901267325694,-55.24995));
#134801=CARTESIAN_POINT('Ctrl Pts',(-52.2713832870762,19.7264221086262,
-54.74995));
#134802=CARTESIAN_POINT('Ctrl Pts',(-52.2713832870762,19.7264221086262,
-55.2499499999999));
#134803=CARTESIAN_POINT('Ctrl Pts',(-52.7694806361221,19.76999998,-55.24995));
#134804=CARTESIAN_POINT('',(-52.6819919725962,20.26999998,-55.74995));
#134805=CARTESIAN_POINT('Origin',(-52.6819919725962,20.76999998,-55.74995));
#134806=CARTESIAN_POINT('Ctrl Pts',(-52.6819919725962,20.26999998,-55.74995));
#134807=CARTESIAN_POINT('Ctrl Pts',(-52.6819919726017,20.26999998,-55.6186826543063));
#134808=CARTESIAN_POINT('Ctrl Pts',(-52.6914208994525,20.2161134164373,
-55.4889566552507));
#134809=CARTESIAN_POINT('Ctrl Pts',(-52.7238127182794,20.0309933247493,
-55.3038365635627));
#134810=CARTESIAN_POINT('Ctrl Pts',(-52.746511826845,19.901267325694,-55.24995));
#134811=CARTESIAN_POINT('Ctrl Pts',(-52.7694806361221,19.76999998,-55.24995));
#134812=CARTESIAN_POINT('Origin',(-52.6819919725962,20.76999998,-52.64995));
#134813=CARTESIAN_POINT('',(-52.6819919725962,20.26999998,-59.64995));
#134814=CARTESIAN_POINT('Origin',(-52.6819919725962,20.76999998,-59.64995));
#134815=CARTESIAN_POINT('',(-52.6819919725962,20.26999998,-55.24995));
#134816=CARTESIAN_POINT('Ctrl Pts',(-52.4648996019023,-38.6266655296175,
-60.866265313415));
#134817=CARTESIAN_POINT('Ctrl Pts',(-52.8907789702838,-38.5816970935142,
-60.5786901973488));
#134818=CARTESIAN_POINT('Ctrl Pts',(-52.903095448475,-38.4409191036023,
-60.08258062683));
#134819=CARTESIAN_POINT('Ctrl Pts',(-52.3309754745585,-39.1170130132287,
-60.7908684306025));
#134820=CARTESIAN_POINT('Ctrl Pts',(-52.8442212423788,-39.1138543585791,
-60.5019204415683));
#134821=CARTESIAN_POINT('Ctrl Pts',(-52.8569709369232,-38.9681246830787,
-59.9318336272105));
#134822=CARTESIAN_POINT('Ctrl Pts',(-52.1936254351686,-39.6095793654924,
-60.7389129305601));
#134823=CARTESIAN_POINT('Ctrl Pts',(-52.7984570004479,-39.6369420374376,
-60.4756484953684));
#134824=CARTESIAN_POINT('Ctrl Pts',(-52.8102637225239,-39.5019905865797,
-59.8278758615346));
#134825=CARTESIAN_POINT('Ctrl Pts',(-51.9132529272684,-40.5953951229239,
-60.6682257074536));
#134826=CARTESIAN_POINT('Ctrl Pts',(-52.7078841622538,-40.6721943151964,
-60.4973085875933));
#134827=CARTESIAN_POINT('Ctrl Pts',(-52.7160699755127,-40.5786300415107,
-59.6865014144928));
#134828=CARTESIAN_POINT('Ctrl Pts',(-51.7702028983306,-41.0887654988916,
-60.64995));
#134829=CARTESIAN_POINT('Ctrl Pts',(-52.662477767809,-41.1911917785403,
-60.5526719649898));
#134830=CARTESIAN_POINT('Ctrl Pts',(-52.6685584273161,-41.1216895223836,
-59.6499500020974));
#134831=CARTESIAN_POINT('Ctrl Pts',(-51.6244217512083,-41.5825130958571,
-60.64995));
#134832=CARTESIAN_POINT('Ctrl Pts',(-52.6206164493,-41.6696688386047,-60.64995));
#134833=CARTESIAN_POINT('Ctrl Pts',(-52.6206164493,-41.6696688386047,-59.64995));
#134834=CARTESIAN_POINT('',(-52.4601060488076,-38.6442121690347,-60.8635779995146));
#134835=CARTESIAN_POINT('',(-51.6244217512083,-41.5825130958571,-60.64995));
#134836=CARTESIAN_POINT('Ctrl Pts',(-52.4601060488526,-38.6442121687577,
-60.8635779995784));
#134837=CARTESIAN_POINT('Ctrl Pts',(-52.327698644121,-39.1287630233132,
-60.7896314173872));
#134838=CARTESIAN_POINT('Ctrl Pts',(-52.1919533933421,-39.6154584197261,
-60.7384913771257));
#134839=CARTESIAN_POINT('Ctrl Pts',(-51.9132529272684,-40.5953951229239,
-60.6682257074536));
#134840=CARTESIAN_POINT('Ctrl Pts',(-51.7702028983306,-41.0887654988916,
-60.64995));
#134841=CARTESIAN_POINT('Ctrl Pts',(-51.6244217512083,-41.5825130958571,
-60.64995));
#134842=CARTESIAN_POINT('Origin',(-51.6244217512083,-41.5825130958571,-59.64995));
#134843=CARTESIAN_POINT('Ctrl Pts',(-52.4601060488526,-38.6442121687577,
-60.8635779995784));
#134844=CARTESIAN_POINT('Ctrl Pts',(-52.5917711956707,-38.6521075044106,
-60.7679496692827));
#134845=CARTESIAN_POINT('Ctrl Pts',(-52.6988044737759,-38.6656865171052,
-60.6372698562504));
#134846=CARTESIAN_POINT('Ctrl Pts',(-52.8422535332614,-38.6982739394415,
-60.3389622441799));
#134847=CARTESIAN_POINT('Ctrl Pts',(-52.8788986395818,-38.7174898948119,
-60.1690974501184));
#134848=CARTESIAN_POINT('Ctrl Pts',(-52.877242281998,-38.7364221486262,
-60.0032396521562));
#134849=CARTESIAN_POINT('Origin',(-53.3753396310439,-38.78000002,-55.2499500000007));
#134850=CARTESIAN_POINT('',(-53.3753396310439,-38.28000002,-55.74995));
#134851=CARTESIAN_POINT('Origin',(-53.3753396310439,-38.78000002,-55.74995));
#134852=CARTESIAN_POINT('',(-53.3753396310439,-38.28000002,-60.0032396521563));
#134853=CARTESIAN_POINT('',(-53.3753396310439,-38.28000002,-55.2499500000007));
#134854=CARTESIAN_POINT('Origin',(-53.3753396310439,-38.78000002,-60.0032396521563));
#134855=CARTESIAN_POINT('Ctrl Pts',(-52.9112502355242,-38.3477094636814,
-54.9585223635782));
#134856=CARTESIAN_POINT('Ctrl Pts',(-52.9364314216307,-38.0597244105783,
-55.3342259538136));
#134857=CARTESIAN_POINT('Ctrl Pts',(-53.4093483797613,-38.0856391317044,
-55.3542421110299));
#134858=CARTESIAN_POINT('Ctrl Pts',(-52.889976625843,-38.5908679349475,
-55.1463344612842));
#134859=CARTESIAN_POINT('Ctrl Pts',(-52.9247563553464,-38.1931762538392,
-55.4246794702588));
#134860=CARTESIAN_POINT('Ctrl Pts',(-53.3880736387225,-38.2072248331335,
-55.448153047952));
#134861=CARTESIAN_POINT('Ctrl Pts',(-52.87724039479,-38.7364437219894,-55.4427310705271));
#134862=CARTESIAN_POINT('Ctrl Pts',(-52.9171601694684,-38.2800041317283,
-55.5832548498195));
#134863=CARTESIAN_POINT('Ctrl Pts',(-53.375339024416,-38.2800034869308,
-55.5963379967406));
#134864=CARTESIAN_POINT('Ctrl Pts',(-52.8772410016055,-38.736436786057,
-55.7499719536926));
#134865=CARTESIAN_POINT('Ctrl Pts',(-52.9171605282557,-38.2800000198531,
-55.7499619127669));
#134866=CARTESIAN_POINT('Ctrl Pts',(-53.3753396310656,-38.2800000198761,
-55.7499609770277));
#134867=CARTESIAN_POINT('Origin',(-53.4522675625606,-37.8403548794211,-55.7203077484906));
#134868=CARTESIAN_POINT('Origin',(-53.7167487055513,-17.6671065732338,-59.64995));
#134869=CARTESIAN_POINT('',(-50.4435446592566,-55.08000002,-60.64995));
#134870=CARTESIAN_POINT('',(-53.7167487055513,-17.6671065732338,-60.64995));
#134871=CARTESIAN_POINT('Ctrl Pts',(-50.4435446592566,-55.08000002,-60.64995));
#134872=CARTESIAN_POINT('Ctrl Pts',(-50.5754672071858,-55.0742946617933,
-60.64995));
#134873=CARTESIAN_POINT('Ctrl Pts',(-50.707290319039,-55.0685936039748,
-60.6239226729819));
#134874=CARTESIAN_POINT('Ctrl Pts',(-50.9510074558263,-55.0580533772402,
-60.5237363920407));
#134875=CARTESIAN_POINT('Ctrl Pts',(-51.0627818569665,-55.0532193817859,
-60.4496168355682));
#134876=CARTESIAN_POINT('Ctrl Pts',(-51.2493148777934,-55.0451522414979,
-60.2644967268049));
#134877=CARTESIAN_POINT('Ctrl Pts',(-51.3240001449277,-55.0419222689988,
-60.153568971423));
#134878=CARTESIAN_POINT('Ctrl Pts',(-51.4249510883276,-55.0375563641359,
-59.9116978933072));
#134879=CARTESIAN_POINT('Ctrl Pts',(-51.4511770665255,-55.0364221486294,
-59.7808732880376));
#134880=CARTESIAN_POINT('Ctrl Pts',(-51.4511770665258,-55.0364221486262,
-59.64995));
#134881=CARTESIAN_POINT('Origin',(-51.9492744155716,-55.08000002,-52.64995));
#134882=CARTESIAN_POINT('',(-51.9492744155716,-54.58000002,-59.64995));
#134883=CARTESIAN_POINT('Origin',(-51.9492744155716,-55.08000002,-59.64995));
#134884=CARTESIAN_POINT('',(-51.9492744155716,-54.58000002,-55.74995));
#134885=CARTESIAN_POINT('Origin',(-51.9492744155716,-55.08000002,-55.74995));
#134886=CARTESIAN_POINT('',(-51.9492744155716,-54.58000002,-55.24995));
#134887=CARTESIAN_POINT('Ctrl Pts',(-51.5386657300517,-54.0364221486262,
-54.74995));
#134888=CARTESIAN_POINT('Ctrl Pts',(-51.5386657300516,-54.0364221486262,
-55.24995));
#134889=CARTESIAN_POINT('Ctrl Pts',(-52.0367630790975,-54.08000002,-55.24995));
#134890=CARTESIAN_POINT('Ctrl Pts',(-51.5156969207731,-54.2989568400126,
-54.7499500000658));
#134891=CARTESIAN_POINT('Ctrl Pts',(-51.5272452363036,-54.1669589895393,
-55.2386587236848));
#134892=CARTESIAN_POINT('Ctrl Pts',(-52.0137942698207,-54.2112673656937,
-55.24995));
#134893=CARTESIAN_POINT('Ctrl Pts',(-51.4929978122091,-54.5584088381255,
-54.8577231271254));
#134894=CARTESIAN_POINT('Ctrl Pts',(-51.5148517139458,-54.308617598254,
-55.2822894538766));
#134895=CARTESIAN_POINT('Ctrl Pts',(-51.9910951612549,-54.3409933647497,
-55.3038365635632));
#134896=CARTESIAN_POINT('Ctrl Pts',(-51.460605993382,-54.9286490214999,
-55.2279633105015));
#134897=CARTESIAN_POINT('Ctrl Pts',(-51.4967198076894,-54.5158662351146,
-55.4680441063697));
#134898=CARTESIAN_POINT('Ctrl Pts',(-51.958703342428,-54.5261134564368,
-55.4889566552503));
#134899=CARTESIAN_POINT('Ctrl Pts',(-51.4511770665315,-55.0364221485606,
-55.4874153086129));
#134900=CARTESIAN_POINT('Ctrl Pts',(-51.491108828562,-54.5800000199489,
-55.6078478088776));
#134901=CARTESIAN_POINT('Ctrl Pts',(-51.9492744155771,-54.58000002,-55.6186826543065));
#134902=CARTESIAN_POINT('Ctrl Pts',(-51.4511770665258,-55.0364221486262,
-55.74995));
#134903=CARTESIAN_POINT('Ctrl Pts',(-51.491108828563,-54.58000002,-55.74995));
#134904=CARTESIAN_POINT('Ctrl Pts',(-51.9492744155716,-54.58000002,-55.74995));
#134905=CARTESIAN_POINT('',(-52.0367630790975,-54.08000002,-55.24995));
#134906=CARTESIAN_POINT('Origin',(-52.0367630790975,-54.08000002,-54.74995));
#134907=CARTESIAN_POINT('Ctrl Pts',(-52.0367630790975,-54.08000002,-55.24995));
#134908=CARTESIAN_POINT('Ctrl Pts',(-52.0137942698207,-54.2112673656937,
-55.24995));
#134909=CARTESIAN_POINT('Ctrl Pts',(-51.9910951612549,-54.3409933647497,
-55.3038365635632));
#134910=CARTESIAN_POINT('Ctrl Pts',(-51.958703342428,-54.5261134564368,
-55.4889566552503));
#134911=CARTESIAN_POINT('Ctrl Pts',(-51.9492744155771,-54.58000002,-55.6186826543065));
#134912=CARTESIAN_POINT('Ctrl Pts',(-51.9492744155716,-54.58000002,-55.74995));
#134913=CARTESIAN_POINT('Origin',(-53.4839470922323,-37.5386110581466,-54.74995));
#134914=CARTESIAN_POINT('',(-52.0805074108605,-53.58000002,-55.24995));
#134915=CARTESIAN_POINT('Origin',(-52.0805074108605,-53.58000002,-54.74995));
#134916=CARTESIAN_POINT('',(-59.2602401389193,28.4847205815761,-55.24995));
#134917=CARTESIAN_POINT('Ctrl Pts',(-51.6698987253405,-52.5364221486262,
-55.74995));
#134918=CARTESIAN_POINT('Ctrl Pts',(-51.6223418238518,-53.08000002,-55.74995));
#134919=CARTESIAN_POINT('Ctrl Pts',(-52.1679960743864,-53.08000002,-55.74995));
#134920=CARTESIAN_POINT('Ctrl Pts',(-51.6698987253348,-52.5364221486917,
-55.4874153086129));
#134921=CARTESIAN_POINT('Ctrl Pts',(-51.6223418238527,-53.0800000200045,
-55.6317784220505));
#134922=CARTESIAN_POINT('Ctrl Pts',(-52.1679960743809,-53.08000002,-55.6186826543066));
#134923=CARTESIAN_POINT('Ctrl Pts',(-51.6604697984843,-52.6441952757516,
-55.2279633105015));
#134924=CARTESIAN_POINT('Ctrl Pts',(-51.6186913913614,-53.1217246542964,
-55.5133819370962));
#134925=CARTESIAN_POINT('Ctrl Pts',(-52.1585671475301,-53.1338865835632,
-55.4889566552503));
#134926=CARTESIAN_POINT('Ctrl Pts',(-51.6280779796571,-53.0144354591276,
-54.8577231271254));
#134927=CARTESIAN_POINT('Ctrl Pts',(-51.6045519400649,-53.2833393221403,
-55.327449621844));
#134928=CARTESIAN_POINT('Ctrl Pts',(-52.1261753287031,-53.3190066752503,
-55.3038365635632));
#134929=CARTESIAN_POINT('Ctrl Pts',(-51.6053788710933,-53.2738874572391,
-54.7499500000658));
#134930=CARTESIAN_POINT('Ctrl Pts',(-51.5941639115132,-53.4020750318305,
-55.2615708605685));
#134931=CARTESIAN_POINT('Ctrl Pts',(-52.1034762201372,-53.4487326743062,
-55.24995));
#134932=CARTESIAN_POINT('Ctrl Pts',(-51.5824100618146,-53.5364221486262,
-54.74995));
#134933=CARTESIAN_POINT('Ctrl Pts',(-51.5824100618146,-53.5364221486261,
-55.2499499999999));
#134934=CARTESIAN_POINT('Ctrl Pts',(-52.0805074108605,-53.58000002,-55.24995));
#134935=CARTESIAN_POINT('',(-52.1679960743864,-53.08000002,-55.74995));
#134936=CARTESIAN_POINT('Origin',(-52.1679960743864,-52.58000002,-55.74995));
#134937=CARTESIAN_POINT('Ctrl Pts',(-52.1679960743864,-53.08000002,-55.74995));
#134938=CARTESIAN_POINT('Ctrl Pts',(-52.1679960743809,-53.08000002,-55.6186826543066));
#134939=CARTESIAN_POINT('Ctrl Pts',(-52.1585671475301,-53.1338865835632,
-55.4889566552503));
#134940=CARTESIAN_POINT('Ctrl Pts',(-52.1261753287031,-53.3190066752503,
-55.3038365635632));
#134941=CARTESIAN_POINT('Ctrl Pts',(-52.1034762201372,-53.4487326743062,
-55.24995));
#134942=CARTESIAN_POINT('Ctrl Pts',(-52.0805074108605,-53.58000002,-55.24995));
#134943=CARTESIAN_POINT('Origin',(-52.1679960743864,-52.58000002,-55.2499500000008));
#134944=CARTESIAN_POINT('',(-52.1679960743864,-53.08000002,-59.64995));
#134945=CARTESIAN_POINT('Origin',(-52.1679960743864,-52.58000002,-59.64995));
#134946=CARTESIAN_POINT('',(-52.1679960743864,-53.08000002,-55.2499500000008));
#134947=CARTESIAN_POINT('Origin',(-53.7167487055513,-17.6671065732338,-59.64995));
#134948=CARTESIAN_POINT('',(-51.1565772669927,-46.93000002,-60.64995));
#134949=CARTESIAN_POINT('',(-50.6622663180714,-52.58000002,-60.64995));
#134950=CARTESIAN_POINT('',(-53.7167487055513,-17.6671065732338,-60.64995));
#134951=CARTESIAN_POINT('Ctrl Pts',(-51.6698987253405,-52.5364221486262,
-59.64995));
#134952=CARTESIAN_POINT('Ctrl Pts',(-51.6698987253403,-52.5364221486294,
-59.7808732880376));
#134953=CARTESIAN_POINT('Ctrl Pts',(-51.6436727471424,-52.5375563641358,
-59.9116978933072));
#134954=CARTESIAN_POINT('Ctrl Pts',(-51.5427218037424,-52.5419222689988,
-60.153568971423));
#134955=CARTESIAN_POINT('Ctrl Pts',(-51.4680365366082,-52.5451522414979,
-60.2644967268049));
#134956=CARTESIAN_POINT('Ctrl Pts',(-51.2815035157812,-52.5532193817859,
-60.4496168355682));
#134957=CARTESIAN_POINT('Ctrl Pts',(-51.1697291146411,-52.5580533772395,
-60.5237363920407));
#134958=CARTESIAN_POINT('Ctrl Pts',(-50.9260119778537,-52.5685936039755,
-60.6239226729819));
#134959=CARTESIAN_POINT('Ctrl Pts',(-50.7941888660007,-52.5742946617934,
-60.64995));
#134960=CARTESIAN_POINT('Ctrl Pts',(-50.6622663180714,-52.58000002,-60.64995));
#134961=CARTESIAN_POINT('Ctrl Pts',(-51.1565772669927,-46.93000002,-60.64995));
#134962=CARTESIAN_POINT('Ctrl Pts',(-51.288499814922,-46.9242946617933,
-60.64995));
#134963=CARTESIAN_POINT('Ctrl Pts',(-51.4203229267752,-46.9185936039748,
-60.6239226729819));
#134964=CARTESIAN_POINT('Ctrl Pts',(-51.6640400635624,-46.9080533772402,
-60.5237363920407));
#134965=CARTESIAN_POINT('Ctrl Pts',(-51.7758144647026,-46.9032193817865,
-60.4496168355682));
#134966=CARTESIAN_POINT('Ctrl Pts',(-51.9623474855296,-46.8951522414972,
-60.264496726805));
#134967=CARTESIAN_POINT('Ctrl Pts',(-52.0370327526638,-46.8919222689988,
-60.153568971423));
#134968=CARTESIAN_POINT('Ctrl Pts',(-52.1379836960638,-46.8875563641358,
-59.9116978933072));
#134969=CARTESIAN_POINT('Ctrl Pts',(-52.1642096742618,-46.8864221486274,
-59.7808732880376));
#134970=CARTESIAN_POINT('Ctrl Pts',(-52.1642096742619,-46.8864221486262,
-59.64995));
#134971=CARTESIAN_POINT('Origin',(-52.6623070233078,-46.93000002,-52.64995));
#134972=CARTESIAN_POINT('',(-52.6623070233077,-46.43000002,-59.64995));
#134973=CARTESIAN_POINT('Origin',(-52.6623070233077,-46.93000002,-59.64995));
#134974=CARTESIAN_POINT('',(-52.6623070233078,-46.43000002,-55.74995));
#134975=CARTESIAN_POINT('Origin',(-52.6623070233078,-46.93000002,-55.74995));
#134976=CARTESIAN_POINT('',(-52.6623070233078,-46.43000002,-55.2499500000008));
#134977=CARTESIAN_POINT('Ctrl Pts',(-52.2516983377878,-45.8864221486262,
-54.74995));
#134978=CARTESIAN_POINT('Ctrl Pts',(-52.2516983377878,-45.8864221486262,
-55.24995));
#134979=CARTESIAN_POINT('Ctrl Pts',(-52.7497956868337,-45.93000002,-55.24995));
#134980=CARTESIAN_POINT('Ctrl Pts',(-52.2287295285091,-46.1489568400132,
-54.7499500000658));
#134981=CARTESIAN_POINT('Ctrl Pts',(-52.2402778440398,-46.0169589895406,
-55.2386587236919));
#134982=CARTESIAN_POINT('Ctrl Pts',(-52.7268268775569,-46.0612673656941,
-55.24995));
#134983=CARTESIAN_POINT('Ctrl Pts',(-52.2060304199453,-46.4084088381247,
-54.8577231271255));
#134984=CARTESIAN_POINT('Ctrl Pts',(-52.227884321682,-46.1586175982532,
-55.2822894538777));
#134985=CARTESIAN_POINT('Ctrl Pts',(-52.704127768991,-46.1909933647493,
-55.3038365635627));
#134986=CARTESIAN_POINT('Ctrl Pts',(-52.1736386011181,-46.7786490215007,
-55.2279633105015));
#134987=CARTESIAN_POINT('Ctrl Pts',(-52.2097524154255,-46.3658662351156,
-55.4680441063688));
#134988=CARTESIAN_POINT('Ctrl Pts',(-52.6717359501641,-46.3761134564373,
-55.4889566552507));
#134989=CARTESIAN_POINT('Ctrl Pts',(-52.1642096742676,-46.8864221485606,
-55.487415308613));
#134990=CARTESIAN_POINT('Ctrl Pts',(-52.2041414362981,-46.4300000199443,
-55.6078478088784));
#134991=CARTESIAN_POINT('Ctrl Pts',(-52.6623070233132,-46.43000002,-55.6186826543062));
#134992=CARTESIAN_POINT('Ctrl Pts',(-52.1642096742619,-46.8864221486262,
-55.74995));
#134993=CARTESIAN_POINT('Ctrl Pts',(-52.2041414362991,-46.43000002,-55.74995));
#134994=CARTESIAN_POINT('Ctrl Pts',(-52.6623070233078,-46.43000002,-55.74995));
#134995=CARTESIAN_POINT('',(-52.7497956868337,-45.93000002,-55.24995));
#134996=CARTESIAN_POINT('Origin',(-52.7497956868337,-45.93000002,-54.74995));
#134997=CARTESIAN_POINT('Ctrl Pts',(-52.7497956868337,-45.93000002,-55.24995));
#134998=CARTESIAN_POINT('Ctrl Pts',(-52.7268268775569,-46.0612673656941,
-55.24995));
#134999=CARTESIAN_POINT('Ctrl Pts',(-52.704127768991,-46.1909933647493,
-55.3038365635627));
#135000=CARTESIAN_POINT('Ctrl Pts',(-52.6717359501641,-46.3761134564373,
-55.4889566552507));
#135001=CARTESIAN_POINT('Ctrl Pts',(-52.6623070233132,-46.43000002,-55.6186826543062));
#135002=CARTESIAN_POINT('Ctrl Pts',(-52.6623070233078,-46.43000002,-55.74995));
#135003=CARTESIAN_POINT('Origin',(-53.4839470922323,-37.5386110581466,-54.74995));
#135004=CARTESIAN_POINT('',(-52.7935400185966,-45.43000002,-55.24995));
#135005=CARTESIAN_POINT('Origin',(-52.7935400185966,-45.43000002,-54.74995));
#135006=CARTESIAN_POINT('',(-59.2602401389193,28.4847205815761,-55.24995));
#135007=CARTESIAN_POINT('Ctrl Pts',(-52.3829313330767,-44.3864221486262,
-55.74995));
#135008=CARTESIAN_POINT('Ctrl Pts',(-52.3353744315879,-44.93000002,-55.74995));
#135009=CARTESIAN_POINT('Ctrl Pts',(-52.8810286821225,-44.93000002,-55.74995));
#135010=CARTESIAN_POINT('Ctrl Pts',(-52.3829313330709,-44.3864221486917,
-55.4874153086129));
#135011=CARTESIAN_POINT('Ctrl Pts',(-52.3353744315888,-44.9300000200045,
-55.6317784220498));
#135012=CARTESIAN_POINT('Ctrl Pts',(-52.8810286821171,-44.93000002,-55.6186826543063));
#135013=CARTESIAN_POINT('Ctrl Pts',(-52.3735024062205,-44.4941952757516,
-55.2279633105015));
#135014=CARTESIAN_POINT('Ctrl Pts',(-52.3317239990966,-44.9717246542945,
-55.5133819370972));
#135015=CARTESIAN_POINT('Ctrl Pts',(-52.8715997552662,-44.9838865835627,
-55.4889566552507));
#135016=CARTESIAN_POINT('Ctrl Pts',(-52.3411105873933,-44.8644354591276,
-54.8577231271254));
#135017=CARTESIAN_POINT('Ctrl Pts',(-52.317584547802,-45.1333393221421,
-55.3274496218433));
#135018=CARTESIAN_POINT('Ctrl Pts',(-52.8392079364393,-45.1690066752507,
-55.3038365635627));
#135019=CARTESIAN_POINT('Ctrl Pts',(-52.3184114788294,-45.1238874572391,
-54.7499500000658));
#135020=CARTESIAN_POINT('Ctrl Pts',(-52.3071965192496,-45.252075031829,
-55.2615708605687));
#135021=CARTESIAN_POINT('Ctrl Pts',(-52.8165088278734,-45.2987326743059,
-55.24995));
#135022=CARTESIAN_POINT('Ctrl Pts',(-52.2954426695508,-45.3864221486262,
-54.74995));
#135023=CARTESIAN_POINT('Ctrl Pts',(-52.2954426695507,-45.3864221486261,
-55.2499499999999));
#135024=CARTESIAN_POINT('Ctrl Pts',(-52.7935400185966,-45.43000002,-55.24995));
#135025=CARTESIAN_POINT('',(-52.3810286821225,-44.43000002,-55.74995));
#135026=CARTESIAN_POINT('Origin',(-52.8810286821225,-44.43000002,-55.74995));
#135027=CARTESIAN_POINT('',(-52.8810286821225,-44.93000002,-55.74995));
#135028=CARTESIAN_POINT('Origin',(-52.8810286821225,-44.43000002,-55.74995));
#135029=CARTESIAN_POINT('Ctrl Pts',(-52.8810286821225,-44.93000002,-55.74995));
#135030=CARTESIAN_POINT('Ctrl Pts',(-52.8810286821171,-44.93000002,-55.6186826543063));
#135031=CARTESIAN_POINT('Ctrl Pts',(-52.8715997552662,-44.9838865835627,
-55.4889566552507));
#135032=CARTESIAN_POINT('Ctrl Pts',(-52.8392079364393,-45.1690066752507,
-55.3038365635627));
#135033=CARTESIAN_POINT('Ctrl Pts',(-52.8165088278734,-45.2987326743059,
-55.24995));
#135034=CARTESIAN_POINT('Ctrl Pts',(-52.7935400185966,-45.43000002,-55.24995));
#135035=CARTESIAN_POINT('Origin',(-52.8810286821225,-44.43000002,-52.64995));
#135036=CARTESIAN_POINT('',(-52.3810286821225,-44.43000002,-59.64995));
#135037=CARTESIAN_POINT('Origin',(-52.8810286821225,-44.43000002,-59.64995));
#135038=CARTESIAN_POINT('',(-52.8810286821225,-44.93000002,-59.64995));
#135039=CARTESIAN_POINT('Origin',(-52.8810286821225,-44.43000002,-59.64995));
#135040=CARTESIAN_POINT('',(-52.8810286821225,-44.93000002,-55.2499500000007));
#135041=CARTESIAN_POINT('Origin',(-53.7167487055513,-17.6671065732338,-59.64995));
#135042=CARTESIAN_POINT('',(-51.3752989258075,-44.43000002,-60.64995));
#135043=CARTESIAN_POINT('',(-53.7167487055513,-17.6671065732338,-60.64995));
#135044=CARTESIAN_POINT('Ctrl Pts',(-52.3829313330767,-44.3864221486262,
-59.64995));
#135045=CARTESIAN_POINT('Ctrl Pts',(-52.3829313330764,-44.3864221486294,
-59.7808732880376));
#135046=CARTESIAN_POINT('Ctrl Pts',(-52.3567053548786,-44.3875563641358,
-59.9116978933072));
#135047=CARTESIAN_POINT('Ctrl Pts',(-52.2557544114786,-44.3919222689988,
-60.153568971423));
#135048=CARTESIAN_POINT('Ctrl Pts',(-52.1810691443443,-44.3951522414979,
-60.2644967268049));
#135049=CARTESIAN_POINT('Ctrl Pts',(-51.9945361235173,-44.4032193817859,
-60.4496168355682));
#135050=CARTESIAN_POINT('Ctrl Pts',(-51.8827617223772,-44.4080533772395,
-60.5237363920407));
#135051=CARTESIAN_POINT('Ctrl Pts',(-51.6390445855899,-44.4185936039755,
-60.6239226729819));
#135052=CARTESIAN_POINT('Ctrl Pts',(-51.5072214737368,-44.4242946617934,
-60.64995));
#135053=CARTESIAN_POINT('Ctrl Pts',(-51.3752989258075,-44.43000002,-60.64995));
#135054=CARTESIAN_POINT('Origin',(0.,-12.9675000200281,-60.64995));
#135055=CARTESIAN_POINT('',(-39.5,31.080768958446,-60.64995));
#135056=CARTESIAN_POINT('',(-39.5,37.7483531044501,-60.64995));
#135057=CARTESIAN_POINT('',(-39.6638655462185,30.7106154376184,-60.64995));
#135058=CARTESIAN_POINT('Origin',(-40.,31.080768958446,-60.64995));
#135059=CARTESIAN_POINT('',(-41.4049466656476,29.0638025010082,-60.64995));
#135060=CARTESIAN_POINT('Origin',(0.,-12.9675000200281,-60.64995));
#135061=CARTESIAN_POINT('',(-41.7558360441701,28.91999998,-60.64995));
#135062=CARTESIAN_POINT('Origin',(-41.7558360441701,29.41999998,-60.64995));
#135063=CARTESIAN_POINT('',(-43.6738487993976,28.91999998,-60.64995));
#135064=CARTESIAN_POINT('',(-1.8346904061005E-14,28.9199999800001,-60.64995));
#135065=CARTESIAN_POINT('',(-45.342056117244,28.91999998,-60.64995));
#135066=CARTESIAN_POINT('Origin',(-44.5079524583208,31.5404524382925,-60.64995));
#135067=CARTESIAN_POINT('',(-1.8346904061005E-14,28.9199999800001,-60.64995));
#135068=CARTESIAN_POINT('Origin',(0.,-12.9675000200281,-60.64995));
#135069=CARTESIAN_POINT('',(-45.8586217441897,-55.08000002,-60.64995));
#135070=CARTESIAN_POINT('',(1.8445455022812E-14,-55.08000002,-60.64995));
#135071=CARTESIAN_POINT('',(-44.5079524583206,-60.2254524783489,-60.64995));
#135072=CARTESIAN_POINT('Origin',(-44.5079524583206,-57.4754524783489,-60.64995));
#135073=CARTESIAN_POINT('',(-42.,-58.6035812240174,-60.64995));
#135074=CARTESIAN_POINT('Origin',(-44.5079524583206,-57.4754524783489,-60.64995));
#135075=CARTESIAN_POINT('',(-42.,-12.9675000200281,-60.64995));
#135076=CARTESIAN_POINT('Origin',(-41.5,-73.08000002,-55.24995));
#135077=CARTESIAN_POINT('',(-24.7,-70.08000002,-55.24995));
#135078=CARTESIAN_POINT('',(-24.7,-73.08000002,-55.24995));
#135079=CARTESIAN_POINT('',(-24.2,-70.08000002,-55.24995));
#135080=CARTESIAN_POINT('',(-41.5,-70.08000002,-55.24995));
#135081=CARTESIAN_POINT('',(-24.2,-73.08000002,-55.24995));
#135082=CARTESIAN_POINT('Origin',(-24.7,67.7009572055632,-55.74995));
#135083=CARTESIAN_POINT('',(-25.2,-70.08000002,-55.74995));
#135084=CARTESIAN_POINT('',(-25.2,67.7009572055632,-55.74995));
#135085=CARTESIAN_POINT('Origin',(-24.7,-70.08000002,-55.74995));
#135086=CARTESIAN_POINT('Ctrl Pts',(-2.97685902995381,45.2502493063675,
-60.8508735991007));
#135087=CARTESIAN_POINT('Ctrl Pts',(-3.50000000000001,45.2282873890497,
-60.8406192095206));
#135088=CARTESIAN_POINT('Ctrl Pts',(-3.5,45.7028119503364,-61.0621827299711));
#135089=CARTESIAN_POINT('Ctrl Pts',(-2.97532164922327,45.3120457868827,
-60.7186918897092));
#135090=CARTESIAN_POINT('Ctrl Pts',(-3.49999999999858,45.2871516612883,
-60.7107288313429));
#135091=CARTESIAN_POINT('Ctrl Pts',(-3.5,45.7953890262578,-60.8639095446885));
#135092=CARTESIAN_POINT('Ctrl Pts',(-2.97452770132487,45.3441826962796,
-60.5756208725641));
#135093=CARTESIAN_POINT('Ctrl Pts',(-3.50000000000077,45.317377912702,-60.5716465029099));
#135094=CARTESIAN_POINT('Ctrl Pts',(-3.5,45.8435334327792,-60.6493041067215));
#135095=CARTESIAN_POINT('Ctrl Pts',(-2.97452770112504,45.3441826962898,
-60.42825533736));
#135096=CARTESIAN_POINT('Ctrl Pts',(-3.5,45.3173779148743,-60.42825533736));
#135097=CARTESIAN_POINT('Ctrl Pts',(-3.5,45.8435334367418,-60.42825533736));
#135098=CARTESIAN_POINT('',(-2.97685902995381,45.2502493063675,-60.8508735991007));
#135099=CARTESIAN_POINT('',(-3.5,45.7028119503364,-61.0621827299711));
#135100=CARTESIAN_POINT('Origin',(-3.,45.7028119503364,-61.0621827299711));
#135101=CARTESIAN_POINT('Origin',(-3.5,43.6249324139852,-60.2700376788023));
#135102=CARTESIAN_POINT('Origin',(-3.01135515498232,43.8637384804388,-60.3228490285208));
#135103=CARTESIAN_POINT('Ctrl Pts',(-2.96960200166493,31.2017108282785,
-90.9273317382593));
#135104=CARTESIAN_POINT('Ctrl Pts',(-3.5,31.1724436113174,-90.9136534008893));
#135105=CARTESIAN_POINT('Ctrl Pts',(-3.5,31.6538440087773,-91.1386408691297));
#135106=CARTESIAN_POINT('Ctrl Pts',(-2.97277930784816,35.8865598281193,
-80.9028133775132));
#135107=CARTESIAN_POINT('Ctrl Pts',(-3.50000000000001,35.8447898541155,
-80.9243218897256));
#135108=CARTESIAN_POINT('Ctrl Pts',(-3.5,36.338906312512,-81.114123180147));
#135109=CARTESIAN_POINT('Ctrl Pts',(-2.97501738453455,40.5689313038002,
-70.8770956617078));
#135110=CARTESIAN_POINT('Ctrl Pts',(-3.49999999995192,40.5360321489106,
-70.8854859061211));
#135111=CARTESIAN_POINT('Ctrl Pts',(-3.5,41.0213995348936,-71.0884053145847));
#135112=CARTESIAN_POINT('Ctrl Pts',(-2.97685902995381,45.2502493063675,
-60.8508735991007));
#135113=CARTESIAN_POINT('Ctrl Pts',(-3.5,45.2282873890496,-60.8406192095206));
#135114=CARTESIAN_POINT('Ctrl Pts',(-3.5,45.7028119503364,-61.0621827299711));
#135115=CARTESIAN_POINT('',(-2.96960200166493,31.2017108282785,-90.9273317382593));
#135116=CARTESIAN_POINT('Ctrl Pts',(-2.97685902995381,45.2502493063675,
-60.8508735991007));
#135117=CARTESIAN_POINT('Ctrl Pts',(-2.97501738453455,40.5689313038002,
-70.8770956617078));
#135118=CARTESIAN_POINT('Ctrl Pts',(-2.97277930784816,35.8865598281193,
-80.9028133775132));
#135119=CARTESIAN_POINT('Ctrl Pts',(-2.96960200166493,31.2017108282785,
-90.9273317382593));
#135120=CARTESIAN_POINT('',(-3.5,31.6538440087773,-91.1386408691296));
#135121=CARTESIAN_POINT('Origin',(-3.,31.6538440087773,-91.1386408691297));
#135122=CARTESIAN_POINT('Ctrl Pts',(-3.5,31.6538440087773,-91.1386408691296));
#135123=CARTESIAN_POINT('Ctrl Pts',(-3.5,36.3389063125119,-81.1141231801469));
#135124=CARTESIAN_POINT('Ctrl Pts',(-3.5,41.0213995348935,-71.0884053145847));
#135125=CARTESIAN_POINT('Ctrl Pts',(-3.5,45.7028119503364,-61.0621827299711));
#135126=CARTESIAN_POINT('Ctrl Pts',(-3.49999922403526,31.7061080469582,
-91.0538938313493));
#135127=CARTESIAN_POINT('Ctrl Pts',(-3.50093050801352,31.2817393765698,
-90.7398753859638));
#135128=CARTESIAN_POINT('Ctrl Pts',(-2.97306337601761,31.3045907584141,
-90.7567937156446));
#135129=CARTESIAN_POINT('Ctrl Pts',(-3.49999921701682,31.6355825669373,
-91.145911917233));
#135130=CARTESIAN_POINT('Ctrl Pts',(-3.50094379952756,31.1316678238861,
-90.9272671499976));
#135131=CARTESIAN_POINT('Ctrl Pts',(-2.96829288576189,31.1636053620749,
-90.9411478319373));
#135132=CARTESIAN_POINT('Ctrl Pts',(-3.49999921357759,31.6011902598928,
-91.2666067024717));
#135133=CARTESIAN_POINT('Ctrl Pts',(-3.5009502924524,31.0578568420018,-91.1768604568285));
#135134=CARTESIAN_POINT('Ctrl Pts',(-2.96595524421095,31.0948516197048,
-91.1829668200116));
#135135=CARTESIAN_POINT('Ctrl Pts',(-3.49999921461707,31.6116002328841,
-91.4242502749333));
#135136=CARTESIAN_POINT('Ctrl Pts',(-3.500948315334,31.0802325137817,-91.5041422369424));
#135137=CARTESIAN_POINT('Ctrl Pts',(-2.96666178933019,31.1156621951816,
-91.4988147743607));
#135138=CARTESIAN_POINT('Ctrl Pts',(-3.49999921542421,31.6196822275484,
-91.4659533973627));
#135139=CARTESIAN_POINT('Ctrl Pts',(-3.50094678207594,31.0975814779846,
-91.5905416925536));
#135140=CARTESIAN_POINT('Ctrl Pts',(-2.96721040786793,31.131818851425,-91.5823690954228));
#135141=CARTESIAN_POINT('Ctrl Pts',(-3.49999921802616,31.6457674414273,
-91.5452519327685));
#135142=CARTESIAN_POINT('Ctrl Pts',(-3.50094185515329,31.1534209463481,
-91.7542131679878));
#135143=CARTESIAN_POINT('Ctrl Pts',(-2.96897896666049,31.1839656512662,
-91.7412467109364));
#135144=CARTESIAN_POINT('Ctrl Pts',(-3.49999921980098,31.6635702854767,
-91.582854393305));
#135145=CARTESIAN_POINT('Ctrl Pts',(-3.50093850621097,31.1914043311977,
-91.8314070942134));
#135146=CARTESIAN_POINT('Ctrl Pts',(-2.97018531781006,31.2195550726727,
-91.8165839823916));
#135147=CARTESIAN_POINT('Ctrl Pts',(-3.49999922431731,31.7089557758124,
-91.6538544608224));
#135148=CARTESIAN_POINT('Ctrl Pts',(-3.50093003210323,31.2877585223428,
-91.9760692084669));
#135149=CARTESIAN_POINT('Ctrl Pts',(-2.97325503421203,31.3102843159908,
-91.9588322867574));
#135150=CARTESIAN_POINT('Ctrl Pts',(-3.4999992269732,31.7356790255681,-91.6858710465136));
#135151=CARTESIAN_POINT('Ctrl Pts',(-3.50092507815379,31.344184586453,-92.0406734083645));
#135152=CARTESIAN_POINT('Ctrl Pts',(-2.9750602060129,31.3637060404082,-92.0229763012619));
#135153=CARTESIAN_POINT('Ctrl Pts',(-3.49999923301664,31.7966270247391,
-91.7428001834818));
#135154=CARTESIAN_POINT('Ctrl Pts',(-3.50091389005982,31.4720263066748,
-92.1541680580386));
#135155=CARTESIAN_POINT('Ctrl Pts',(-2.97916779726235,31.4855450265412,
-92.1370294700019));
#135156=CARTESIAN_POINT('Ctrl Pts',(-3.49999923642963,31.8311111796843,
-91.7677027010548));
#135157=CARTESIAN_POINT('Ctrl Pts',(-3.50090762073163,31.5438509901872,
-92.2030328175872));
#135158=CARTESIAN_POINT('Ctrl Pts',(-2.98148749783816,31.5544807156723,
-92.1869184533145));
#135159=CARTESIAN_POINT('Ctrl Pts',(-3.49999925011377,31.9697383525658,
-91.8435168239899));
#135160=CARTESIAN_POINT('Ctrl Pts',(-3.50088282112773,31.8290423663707,
-92.3480552642004));
#135161=CARTESIAN_POINT('Ctrl Pts',(-2.99078795925646,31.831600651801,-92.3387960611338));
#135162=CARTESIAN_POINT('Ctrl Pts',(-3.49999926225773,32.0935311034211,
-91.8633729799761));
#135163=CARTESIAN_POINT('Ctrl Pts',(-3.50086127365168,32.0791885144776,
-92.3794664923917));
#135164=CARTESIAN_POINT('Ctrl Pts',(-2.99904131966573,32.0790639293044,
-92.3785629066546));
#135165=CARTESIAN_POINT('Ctrl Pts',(-3.49999927329452,32.2071461725455,
-91.8385626593204));
#135166=CARTESIAN_POINT('Ctrl Pts',(-3.50084210619723,32.3047109063527,
-92.3225314465932));
#135167=CARTESIAN_POINT('Ctrl Pts',(-3.00654191745144,32.3061822047335,
-92.3288444828576));
#135168=CARTESIAN_POINT('',(-2.96642434956618,31.1080206316559,-91.3499499999828));
#135169=CARTESIAN_POINT('Ctrl Pts',(-2.96960200166493,31.2017108282784,
-90.9273317382593));
#135170=CARTESIAN_POINT('Ctrl Pts',(-2.96907626063775,31.1861935567743,
-90.9606093101452));
#135171=CARTESIAN_POINT('Ctrl Pts',(-2.96861263948861,31.1725578229795,
-90.9946439154509));
#135172=CARTESIAN_POINT('Ctrl Pts',(-2.968215225744,31.1608577587541,-91.0291939475198));
#135173=CARTESIAN_POINT('Ctrl Pts',(-2.96801651887169,31.1550077266415,
-91.0464689635542));
#135174=CARTESIAN_POINT('Ctrl Pts',(-2.96783433959547,31.1496412337337,
-91.0638723528608));
#135175=CARTESIAN_POINT('Ctrl Pts',(-2.9676690065049,31.144762087643,-91.0813717845137));
#135176=CARTESIAN_POINT('Ctrl Pts',(-2.9675863399596,31.1423225145976,-91.0901215003401));
#135177=CARTESIAN_POINT('Ctrl Pts',(-2.96750788278562,31.1400047458653,
-91.0988951964481));
#135178=CARTESIAN_POINT('Ctrl Pts',(-2.9674336594212,31.1378090219179,-91.1076887806881));
#135179=CARTESIAN_POINT('Ctrl Pts',(-2.96739654773899,31.1367111599442,
-91.1120855728081));
#135180=CARTESIAN_POINT('Ctrl Pts',(-2.96736049435837,31.1356438069241,
-91.1164873356036));
#135181=CARTESIAN_POINT('Ctrl Pts',(-2.96732550136397,31.1346069783171,
-91.1208935530637));
#135182=CARTESIAN_POINT('Ctrl Pts',(-2.96730800486679,31.1340885640136,
-91.1230966617938));
#135183=CARTESIAN_POINT('Ctrl Pts',(-2.96729077345614,31.1335777806645,
-91.1253008841207));
#135184=CARTESIAN_POINT('Ctrl Pts',(-2.96727380732783,31.1330746292164,
-91.1275061555234));
#135185=CARTESIAN_POINT('Ctrl Pts',(-2.96726030613665,31.1326742347498,
-91.1292610515298));
#135186=CARTESIAN_POINT('Ctrl Pts',(-2.96723992575453,31.1320713979023,
-91.131945205737));
#135187=CARTESIAN_POINT('Ctrl Pts',(-2.96722952789365,31.1317615130644,
-91.1333418601676));
#135188=CARTESIAN_POINT('Ctrl Pts',(-2.96722685939323,31.1316819844165,
-91.1337002966734));
#135189=CARTESIAN_POINT('Ctrl Pts',(-2.96722483060121,31.1316214861816,
-91.1339738745067));
#135190=CARTESIAN_POINT('Ctrl Pts',(-2.96722370494375,31.1315880708905,
-91.1341250523127));
#135191=CARTESIAN_POINT('Ctrl Pts',(-2.96719059076607,31.1306050721212,
-91.1385723455124));
#135192=CARTESIAN_POINT('Ctrl Pts',(-2.96714968507035,31.1292784394994,
-91.1446972176635));
#135193=CARTESIAN_POINT('Ctrl Pts',(-2.96710052166565,31.127704189862,-91.1525124220698));
#135194=CARTESIAN_POINT('Ctrl Pts',(-2.9670513411666,31.1261293928509,-91.160330343858));
#135195=CARTESIAN_POINT('Ctrl Pts',(-2.96699389511064,31.1243067798829,
-91.1698401921196));
#135196=CARTESIAN_POINT('Ctrl Pts',(-2.96693120584415,31.1223842739554,
-91.1810590360774));
#135197=CARTESIAN_POINT('Ctrl Pts',(-2.96686889195463,31.1204732797982,
-91.1922107027374));
#135198=CARTESIAN_POINT('Ctrl Pts',(-2.96680140002913,31.1184636257961,
-91.2050515373047));
#135199=CARTESIAN_POINT('Ctrl Pts',(-2.96673513845011,31.1165516198435,
-91.2195950992161));
#135200=CARTESIAN_POINT('Ctrl Pts',(-2.96666947809326,31.1146569624116,
-91.2340067006156));
#135201=CARTESIAN_POINT('Ctrl Pts',(-2.96660503372642,31.112858304374,-91.2500909687296));
#135202=CARTESIAN_POINT('Ctrl Pts',(-2.96655135114763,31.1113957530503,
-91.2678484443061));
#135203=CARTESIAN_POINT('Ctrl Pts',(-2.96649881526904,31.109964442921,-91.2852266068699));
#135204=CARTESIAN_POINT('Ctrl Pts',(-2.96645660610933,31.1088553216018,
-91.3042079708774));
#135205=CARTESIAN_POINT('Ctrl Pts',(-2.96643664336358,31.1083375749915,
-91.3247705156409));
#135206=CARTESIAN_POINT('Ctrl Pts',(-2.96642873475368,31.1081324601229,
-91.3329167469847));
#135207=CARTESIAN_POINT('Ctrl Pts',(-2.96642434935722,31.1080206316701,
-91.3413108330902));
#135208=CARTESIAN_POINT('Ctrl Pts',(-2.96642434956618,31.1080206316559,
-91.3499499999828));
#135209=CARTESIAN_POINT('',(-3.,32.1080106234021,-92.34995));
#135210=CARTESIAN_POINT('Ctrl Pts',(-2.96642434956619,31.1080206316559,
-91.3499499999828));
#135211=CARTESIAN_POINT('Ctrl Pts',(-2.9664271070228,31.108045768609,-91.37190912875));
#135212=CARTESIAN_POINT('Ctrl Pts',(-2.96645079020869,31.1087442225408,
-91.3938431330336));
#135213=CARTESIAN_POINT('Ctrl Pts',(-2.96668560519294,31.1156606164675,
-91.4988150117475));
#135214=CARTESIAN_POINT('Ctrl Pts',(-2.96723421322274,31.1318173249492,
-91.5823694597986));
#135215=CARTESIAN_POINT('Ctrl Pts',(-2.96900273785673,31.1839642868761,
-91.7412472901304));
#135216=CARTESIAN_POINT('Ctrl Pts',(-2.97020906550757,31.2195538136165,
-91.8165846453629));
#135217=CARTESIAN_POINT('Ctrl Pts',(-2.97327872125958,31.3102833052691,
-91.95883306017));
#135218=CARTESIAN_POINT('Ctrl Pts',(-2.97508385688375,31.3637051628446,
-92.0229770968143));
#135219=CARTESIAN_POINT('Ctrl Pts',(-2.97919136429243,31.485544416253,-92.1370302437053));
#135220=CARTESIAN_POINT('Ctrl Pts',(-2.98151101664575,31.5544802346756,
-92.1869191824921));
#135221=CARTESIAN_POINT('Ctrl Pts',(-2.98885332885225,31.7732594207181,
-92.3068223160387));
#135222=CARTESIAN_POINT('Ctrl Pts',(-2.99446266807111,31.9411884844373,
-92.349950020068));
#135223=CARTESIAN_POINT('Ctrl Pts',(-3.,32.1080106234021,-92.34995));
#135224=CARTESIAN_POINT('',(-3.5,32.1080106234021,-91.84995));
#135225=CARTESIAN_POINT('Origin',(-3.,32.1080106234021,-91.84995));
#135226=CARTESIAN_POINT('Ctrl Pts',(-3.5,32.1080106234021,-91.84995));
#135227=CARTESIAN_POINT('Ctrl Pts',(-3.5,31.9390236361236,-91.84995));
#135228=CARTESIAN_POINT('Ctrl Pts',(-3.5,31.7764555346939,-91.7610777969008));
#135229=CARTESIAN_POINT('Ctrl Pts',(-3.5,31.5945841314222,-91.476580999558));
#135230=CARTESIAN_POINT('Ctrl Pts',(-3.5,31.5822909477801,-91.2917412718895));
#135231=CARTESIAN_POINT('Ctrl Pts',(-3.5,31.6538440087773,-91.1386408691296));
#135232=CARTESIAN_POINT('Origin',(-38.,46.41999998,-91.84995));
#135233=CARTESIAN_POINT('',(-37.,46.41999998,-92.34995));
#135234=CARTESIAN_POINT('',(-37.5,46.41999998,-91.84995));
#135235=CARTESIAN_POINT('Origin',(-37.,46.41999998,-91.84995));
#135236=CARTESIAN_POINT('',(-38.,47.41999998,-92.34995));
#135237=CARTESIAN_POINT('Origin',(-38.,46.41999998,-92.34995));
#135238=CARTESIAN_POINT('',(-38.,46.91999998,-91.84995));
#135239=CARTESIAN_POINT('Origin',(-38.,47.41999998,-91.84995));
#135240=CARTESIAN_POINT('Origin',(-38.,46.41999998,-91.84995));
#135241=CARTESIAN_POINT('Origin',(41.5,47.41999998,-91.84995));
#135242=CARTESIAN_POINT('',(-38.5,47.41999998,-92.34995));
#135243=CARTESIAN_POINT('',(41.5,47.41999998,-92.34995));
#135244=CARTESIAN_POINT('',(-38.5,46.91999998,-91.84995));
#135245=CARTESIAN_POINT('Origin',(-38.5,47.41999998,-91.84995));
#135246=CARTESIAN_POINT('',(39.,46.91999998,-91.84995));
#135247=CARTESIAN_POINT('Origin',(-38.5,58.91999998,-95.34995));
#135248=CARTESIAN_POINT('',(-40.9899542848408,29.0638025010082,-93.6765918018241));
#135249=CARTESIAN_POINT('',(-41.2907166092886,28.91999998,-94.2490863360338));
#135250=CARTESIAN_POINT('Ctrl Pts',(-40.9899542848408,29.0638025010082,
-93.6765918018241));
#135251=CARTESIAN_POINT('Ctrl Pts',(-41.0445777715999,29.0010249744694,
-93.7578714615268));
#135252=CARTESIAN_POINT('Ctrl Pts',(-41.1012013116007,28.9670983124193,
-93.8513385014916));
#135253=CARTESIAN_POINT('Ctrl Pts',(-41.203906529354,28.9262911739198,-94.0457359962981));
#135254=CARTESIAN_POINT('Ctrl Pts',(-41.2500626594833,28.9199999557335,
-94.1460275680244));
#135255=CARTESIAN_POINT('Ctrl Pts',(-41.2907166092886,28.91999998,-94.2490863360338));
#135256=CARTESIAN_POINT('',(-39.4975990396159,30.7106154376184,-92.5206751536556));
#135257=CARTESIAN_POINT('Ctrl Pts',(-39.4975990396159,30.7106154376184,
-92.5206751536556));
#135258=CARTESIAN_POINT('Ctrl Pts',(-39.7830757934441,30.4081688522969,
-92.6213339269874));
#135259=CARTESIAN_POINT('Ctrl Pts',(-40.0606440851126,30.1068692044787,
-92.7683994467215));
#135260=CARTESIAN_POINT('Ctrl Pts',(-40.5646325235533,29.548843193136,-93.1505624120075));
#135261=CARTESIAN_POINT('Ctrl Pts',(-40.7930602005308,29.2900891143653,
-93.3836137237161));
#135262=CARTESIAN_POINT('Ctrl Pts',(-40.9899542848408,29.0638025010082,
-93.6765918018241));
#135263=CARTESIAN_POINT('',(-39.3571428571429,31.080768958446,-92.4750054575003));
#135264=CARTESIAN_POINT('Ctrl Pts',(-39.3571428571429,31.080768958446,-92.4750054575003));
#135265=CARTESIAN_POINT('Ctrl Pts',(-39.3571429430277,30.9391538899445,
-92.4750054831062));
#135266=CARTESIAN_POINT('Ctrl Pts',(-39.410274588038,30.8031308123719,-92.4898846529936));
#135267=CARTESIAN_POINT('Ctrl Pts',(-39.4975990396159,30.7106154376184,
-92.5206751536556));
#135268=CARTESIAN_POINT('',(-39.3571428571429,46.41999998,-92.4750054575003));
#135269=CARTESIAN_POINT('',(-39.3571428571429,58.91999998,-92.4750054575003));
#135270=CARTESIAN_POINT('Ctrl Pts',(-38.5,47.41999998,-92.34995));
#135271=CARTESIAN_POINT('Ctrl Pts',(-38.6117163199788,47.4199999701223,
-92.34995));
#135272=CARTESIAN_POINT('Ctrl Pts',(-38.7257728904125,47.3934379073013,
-92.3566603033275));
#135273=CARTESIAN_POINT('Ctrl Pts',(-38.9319509445986,47.2935007246494,
-92.3793987064332));
#135274=CARTESIAN_POINT('Ctrl Pts',(-39.0271570378558,47.2191189043121,
-92.3955365750638));
#135275=CARTESIAN_POINT('Ctrl Pts',(-39.1845108402481,47.0356954006484,
-92.4279818041452));
#135276=CARTESIAN_POINT('Ctrl Pts',(-39.2481885236226,46.925205464765,-92.444400991043));
#135277=CARTESIAN_POINT('Ctrl Pts',(-39.3344873999803,46.6833015096169,
-92.4680006788624));
#135278=CARTESIAN_POINT('Ctrl Pts',(-39.3571428368889,46.5515558031783,
-92.4750054514617));
#135279=CARTESIAN_POINT('Ctrl Pts',(-39.3571428571429,46.41999998,-92.4750054575003));
#135280=CARTESIAN_POINT('',(-38.5,58.91999998,-92.34995));
#135281=CARTESIAN_POINT('',(-38.5,58.91999998,-92.34995));
#135282=CARTESIAN_POINT('',(-41.5,58.91999998,-95.34995));
#135283=CARTESIAN_POINT('Origin',(-38.5,58.91999998,-95.34995));
#135284=CARTESIAN_POINT('',(-41.5,28.91999998,-95.34995));
#135285=CARTESIAN_POINT('',(-41.5,58.91999998,-95.34995));
#135286=CARTESIAN_POINT('Origin',(-38.5,28.91999998,-95.34995));
#135287=CARTESIAN_POINT('Origin',(-3.,58.91999998,-91.84995));
#135288=CARTESIAN_POINT('',(-3.,46.41999998,-92.34995));
#135289=CARTESIAN_POINT('',(-3.,46.41999998,-92.34995));
#135290=CARTESIAN_POINT('',(-3.5,46.41999998,-91.84995));
#135291=CARTESIAN_POINT('Origin',(-3.,46.41999998,-91.84995));
#135292=CARTESIAN_POINT('',(-3.5,32.0719455778696,-91.84995));
#135293=CARTESIAN_POINT('Origin',(-4.,46.41999998,-91.84995));
#135294=CARTESIAN_POINT('',(-4.,47.41999998,-92.34995));
#135295=CARTESIAN_POINT('Origin',(-4.,46.41999998,-92.34995));
#135296=CARTESIAN_POINT('',(-4.,46.91999998,-91.84995));
#135297=CARTESIAN_POINT('Origin',(-4.,47.41999998,-91.84995));
#135298=CARTESIAN_POINT('Origin',(-4.,46.41999998,-91.84995));
#135299=CARTESIAN_POINT('Origin',(41.5,47.41999998,-91.84995));
#135300=CARTESIAN_POINT('',(-4.5,47.41999998,-92.34995));
#135301=CARTESIAN_POINT('',(41.5,47.41999998,-92.34995));
#135302=CARTESIAN_POINT('',(-4.5,46.91999998,-91.84995));
#135303=CARTESIAN_POINT('Origin',(-4.5,47.41999998,-91.84995));
#135304=CARTESIAN_POINT('',(39.,46.91999998,-91.84995));
#135305=CARTESIAN_POINT('Origin',(-4.5,46.41999998,-91.84995));
#135306=CARTESIAN_POINT('',(-5.5,46.41999998,-92.34995));
#135307=CARTESIAN_POINT('Origin',(-4.5,46.41999998,-92.34995));
#135308=CARTESIAN_POINT('',(-5.,46.41999998,-91.84995));
#135309=CARTESIAN_POINT('Origin',(-5.5,46.41999998,-91.84995));
#135310=CARTESIAN_POINT('Origin',(-4.5,46.41999998,-91.84995));
#135311=CARTESIAN_POINT('Origin',(-5.5,-9.33460238845303,-91.84995));
#135312=CARTESIAN_POINT('',(-5.5,31.8716754827171,-92.34995));
#135313=CARTESIAN_POINT('',(-5.5,31.9301798728793,-92.34995));
#135314=CARTESIAN_POINT('',(-5.,31.8716754827171,-91.84995));
#135315=CARTESIAN_POINT('Origin',(-5.5,31.8716754827171,-91.84995));
#135316=CARTESIAN_POINT('',(-5.,46.41999998,-91.84995));
#135317=CARTESIAN_POINT('Origin',(-1.1373643128445E-15,-12.9675000200281,
-91.34995));
#135318=CARTESIAN_POINT('',(-11.3834743397155,29.812801930373,-90.9273317382593));
#135319=CARTESIAN_POINT('',(-11.3712933400039,29.7190889970661,-91.3499500007659));
#135320=CARTESIAN_POINT('Origin',(-11.4527257127636,30.3470007156979,-91.2823260948233));
#135321=CARTESIAN_POINT('',(-5.44427033638568,30.9653765476951,-90.9273317382593));
#135322=CARTESIAN_POINT('Origin',(-1.1373643128445E-15,-12.9675000200281,
-90.9273317382593));
#135323=CARTESIAN_POINT('',(-5.43844464087133,30.8716892291688,-91.34995));
#135324=CARTESIAN_POINT('Origin',(-5.47960007965946,31.5342994497431,-91.2881238021625));
#135325=CARTESIAN_POINT('Ctrl Pts',(-5.5,31.8716754827171,-92.34995));
#135326=CARTESIAN_POINT('Ctrl Pts',(-5.48989377680063,31.7056523166615,
-92.34995));
#135327=CARTESIAN_POINT('Ctrl Pts',(-5.47963373781052,31.538103809625,-92.3071746231476));
#135328=CARTESIAN_POINT('Ctrl Pts',(-5.46619042199875,31.3196047327668,
-92.1878686007335));
#135329=CARTESIAN_POINT('Ctrl Pts',(-5.46194839019336,31.2508398250121,
-92.1383294170381));
#135330=CARTESIAN_POINT('Ctrl Pts',(-5.45439667136824,31.1286541135227,
-92.0244078521253));
#135331=CARTESIAN_POINT('Ctrl Pts',(-5.45108997919633,31.0752759499814,
-91.9605552262364));
#135332=CARTESIAN_POINT('Ctrl Pts',(-5.44262999595016,30.938884482232,-91.7477840212027));
#135333=CARTESIAN_POINT('Ctrl Pts',(-5.43928039898085,30.8851161679224,
-91.5835323055617));
#135334=CARTESIAN_POINT('Ctrl Pts',(-5.43849137201243,30.8724399372431,
-91.3946568152791));
#135335=CARTESIAN_POINT('Ctrl Pts',(-5.43844622689811,30.8717137358109,
-91.3723154432813));
#135336=CARTESIAN_POINT('Ctrl Pts',(-5.43844464087133,30.8716892291688,
-91.34995));
#135337=CARTESIAN_POINT('',(-11.5,30.7194735506599,-92.34995));
#135338=CARTESIAN_POINT('Origin',(-1.1373643128445E-15,-12.9675000200281,
-92.34995));
#135339=CARTESIAN_POINT('Ctrl Pts',(-11.3712933400038,29.719088997066,-91.3499500007659));
#135340=CARTESIAN_POINT('Ctrl Pts',(-11.3713013356712,29.7190868671284,
-91.3885031985189));
#135341=CARTESIAN_POINT('Ctrl Pts',(-11.3715900563149,29.7213217313681,
-91.4271147023396));
#135342=CARTESIAN_POINT('Ctrl Pts',(-11.3721684286715,29.7257851411112,
-91.4654778746805));
#135343=CARTESIAN_POINT('Ctrl Pts',(-11.3727466124145,29.7302470952876,
-91.5038285363716));
#135344=CARTESIAN_POINT('Ctrl Pts',(-11.373614238183,29.736936078301,-91.5419303731955));
#135345=CARTESIAN_POINT('Ctrl Pts',(-11.3747663901512,29.7457936995826,
-91.579482237));
#135346=CARTESIAN_POINT('Ctrl Pts',(-11.3759196281462,29.7546596701221,
-91.6170694974632));
#135347=CARTESIAN_POINT('Ctrl Pts',(-11.3773578751843,29.7656981886916,
-91.654105115319));
#135348=CARTESIAN_POINT('Ctrl Pts',(-11.3790628963733,29.7788024661424,
-91.6903019838639));
#135349=CARTESIAN_POINT('Ctrl Pts',(-11.3798254998803,29.7846636061715,
-91.7064917292316));
#135350=CARTESIAN_POINT('Ctrl Pts',(-11.3806412991493,29.7909373746637,
-91.7225139392306));
#135351=CARTESIAN_POINT('Ctrl Pts',(-11.3815078564561,29.7976112818844,
-91.7383443849165));
#135352=CARTESIAN_POINT('Ctrl Pts',(-11.3834559407968,29.8126147144873,
-91.7739323871261));
#135353=CARTESIAN_POINT('Ctrl Pts',(-11.3856671264025,29.8296923799048,
-91.8086655197473));
#135354=CARTESIAN_POINT('Ctrl Pts',(-11.388129442384,29.8487050388042,-91.8422692512968));
#135355=CARTESIAN_POINT('Ctrl Pts',(-11.3905921149091,29.8677204507392,
-91.875877848671));
#135356=CARTESIAN_POINT('Ctrl Pts',(-11.3933058886042,29.8886710747684,
-91.9083561622676));
#135357=CARTESIAN_POINT('Ctrl Pts',(-11.3962472964129,29.911374995788,-91.9394573269113));
#135358=CARTESIAN_POINT('Ctrl Pts',(-11.3991934464272,29.9341155205936,
-91.9706086335712));
#135359=CARTESIAN_POINT('Ctrl Pts',(-11.4023678382941,29.9586145652146,
-92.0003778665942));
#135360=CARTESIAN_POINT('Ctrl Pts',(-11.4057370832413,29.9846524195957,
-92.0285526540719));
#135361=CARTESIAN_POINT('Ctrl Pts',(-11.4071664410782,29.9956986367154,
-92.0405054369404));
#135362=CARTESIAN_POINT('Ctrl Pts',(-11.408630758751,30.0070213892768,-92.0521717366627));
#135363=CARTESIAN_POINT('Ctrl Pts',(-11.410127046267,30.0186022152685,-92.0635375721449));
#135364=CARTESIAN_POINT('Ctrl Pts',(-11.4142954954677,30.0508647880247,
-92.0952012112017));
#135365=CARTESIAN_POINT('Ctrl Pts',(-11.4187247812978,30.0852050202082,
-92.1246026482632));
#135366=CARTESIAN_POINT('Ctrl Pts',(-11.4233738906191,30.1212889057877,
-92.1515089998868));
#135367=CARTESIAN_POINT('Ctrl Pts',(-11.4280432727768,30.157530138217,-92.1785326789434));
#135368=CARTESIAN_POINT('Ctrl Pts',(-11.432934281018,30.1955298850529,-92.2030393156081));
#135369=CARTESIAN_POINT('Ctrl Pts',(-11.438000215523,30.2349279316181,-92.2248405680941));
#135370=CARTESIAN_POINT('Ctrl Pts',(-11.4430983663307,30.2745765261115,
-92.2467804634601));
#135371=CARTESIAN_POINT('Ctrl Pts',(-11.4483735571548,30.3156408743999,
-92.265980333651));
#135372=CARTESIAN_POINT('Ctrl Pts',(-11.4537747777112,30.3577375734027,
-92.2822984029973));
#135373=CARTESIAN_POINT('Ctrl Pts',(-11.4591922473244,30.3999609163087,
-92.2986655636985));
#135374=CARTESIAN_POINT('Ctrl Pts',(-11.4647363885862,30.4432224293095,
-92.3121335087565));
#135375=CARTESIAN_POINT('Ctrl Pts',(-11.4703540873708,30.4871248827319,
-92.3226107580528));
#135376=CARTESIAN_POINT('Ctrl Pts',(-11.4759973775821,30.5312273337798,
-92.3331357364579));
#135377=CARTESIAN_POINT('Ctrl Pts',(-11.4817147834776,30.5759761761234,
-92.3406426903389));
#135378=CARTESIAN_POINT('Ctrl Pts',(-11.4874525496363,30.6209643473028,
-92.3450913875843));
#135379=CARTESIAN_POINT('Ctrl Pts',(-11.4916309796454,30.6537262130378,
-92.3483310752184));
#135380=CARTESIAN_POINT('Ctrl Pts',(-11.495820204077,30.6866148885679,-92.34995));
#135381=CARTESIAN_POINT('Ctrl Pts',(-11.5,30.7194735506599,-92.34995));
#135382=CARTESIAN_POINT('Origin',(-11.5,58.91999998,-91.84995));
#135383=CARTESIAN_POINT('',(-12.,30.7194735506599,-91.84995));
#135384=CARTESIAN_POINT('Origin',(-11.5,30.7194735506599,-91.84995));
#135385=CARTESIAN_POINT('',(-11.5,46.41999998,-92.34995));
#135386=CARTESIAN_POINT('',(-11.5,46.41999998,-92.34995));
#135387=CARTESIAN_POINT('',(-12.,46.41999998,-91.84995));
#135388=CARTESIAN_POINT('Origin',(-11.5,46.41999998,-91.84995));
#135389=CARTESIAN_POINT('',(-12.,30.5847864844252,-91.84995));
#135390=CARTESIAN_POINT('Origin',(-12.5,46.41999998,-91.84995));
#135391=CARTESIAN_POINT('',(-12.5,47.41999998,-92.34995));
#135392=CARTESIAN_POINT('Origin',(-12.5,46.41999998,-92.34995));
#135393=CARTESIAN_POINT('',(-12.5,46.91999998,-91.84995));
#135394=CARTESIAN_POINT('Origin',(-12.5,47.41999998,-91.84995));
#135395=CARTESIAN_POINT('Origin',(-12.5,46.41999998,-91.84995));
#135396=CARTESIAN_POINT('Origin',(41.5,47.41999998,-91.84995));
#135397=CARTESIAN_POINT('',(-13.,47.41999998,-92.34995));
#135398=CARTESIAN_POINT('',(41.5,47.41999998,-92.34995));
#135399=CARTESIAN_POINT('',(-13.,46.91999998,-91.84995));
#135400=CARTESIAN_POINT('Origin',(-13.,47.41999998,-91.84995));
#135401=CARTESIAN_POINT('',(39.,46.91999998,-91.84995));
#135402=CARTESIAN_POINT('Origin',(-13.,46.41999998,-91.84995));
#135403=CARTESIAN_POINT('',(-14.,46.41999998,-92.34995));
#135404=CARTESIAN_POINT('Origin',(-13.,46.41999998,-92.34995));
#135405=CARTESIAN_POINT('',(-13.5,46.41999998,-91.84995));
#135406=CARTESIAN_POINT('Origin',(-14.,46.41999998,-91.84995));
#135407=CARTESIAN_POINT('Origin',(-13.,46.41999998,-91.84995));
#135408=CARTESIAN_POINT('Origin',(-14.,-9.33460238845303,-91.84995));
#135409=CARTESIAN_POINT('',(-14.,29.9836543272765,-92.34995));
#135410=CARTESIAN_POINT('',(-14.,30.1434227231235,-92.34995));
#135411=CARTESIAN_POINT('',(-13.5,29.9836543272765,-91.84995));
#135412=CARTESIAN_POINT('Origin',(-14.,29.9836543272765,-91.84995));
#135413=CARTESIAN_POINT('',(-13.5,46.41999998,-91.84995));
#135414=CARTESIAN_POINT('Origin',(-1.1373643128445E-15,-12.9675000200281,
-91.34995));
#135415=CARTESIAN_POINT('',(-14.0295223410747,29.9740202447141,-92.34995));
#135416=CARTESIAN_POINT('Origin',(-1.1373643128445E-15,-12.9675000200281,
-92.34995));
#135417=CARTESIAN_POINT('',(-13.9704776589253,29.7932964571609,-92.3317099697081));
#135418=CARTESIAN_POINT('Origin',(-14.0295223410747,29.9740202447144,-91.34995));
#135419=CARTESIAN_POINT('Origin',(-13.9965098969202,29.9839599889458,-91.3260842600189));
#135420=CARTESIAN_POINT('Ctrl Pts',(-17.5283605562717,29.4199999800001,
-92.34995));
#135421=CARTESIAN_POINT('Ctrl Pts',(-17.5283605562716,28.41999998,-92.34995));
#135422=CARTESIAN_POINT('Ctrl Pts',(-17.5283605562717,28.4199999800001,
-91.34995));
#135423=CARTESIAN_POINT('Ctrl Pts',(-16.9294484484718,29.4199999819522,
-92.34995));
#135424=CARTESIAN_POINT('Ctrl Pts',(-16.8501904102942,28.3452044605545,
-92.3499500000001));
#135425=CARTESIAN_POINT('Ctrl Pts',(-16.8748117549663,28.4199999800001,
-91.2778699709694));
#135426=CARTESIAN_POINT('Ctrl Pts',(-16.3387077693293,29.4682775272991,
-92.34995));
#135427=CARTESIAN_POINT('Ctrl Pts',(-16.1934854928648,28.3221299458475,
-92.34995));
#135428=CARTESIAN_POINT('Ctrl Pts',(-16.233134779349,28.4803469141606,-91.2065756291954));
#135429=CARTESIAN_POINT('Ctrl Pts',(-15.1723882243972,29.6527167118161,
-92.34995));
#135430=CARTESIAN_POINT('Ctrl Pts',(-14.8701093399109,28.3452025116243,
-92.34995));
#135431=CARTESIAN_POINT('Ctrl Pts',(-14.9727946058278,28.7108958947333,
-91.0656179778369));
#135432=CARTESIAN_POINT('Ctrl Pts',(-14.5966754937866,29.7887243470281,
-92.34995));
#135433=CARTESIAN_POINT('Ctrl Pts',(-14.194875318369,28.3987342821361,-92.3499499999805));
#135434=CARTESIAN_POINT('Ctrl Pts',(-14.3539522178783,28.8809201843631,
-90.9959326732687));
#135435=CARTESIAN_POINT('Ctrl Pts',(-14.0295223410746,29.9740202447142,
-92.34995));
#135436=CARTESIAN_POINT('Ctrl Pts',(-13.5420441920761,28.4819485757734,
-92.3499500000002));
#135437=CARTESIAN_POINT('Ctrl Pts',(-13.7480613600421,29.1125253108927,
-90.92733173826));
#135438=CARTESIAN_POINT('',(-17.5283605562717,29.41999998,-92.34995));
#135439=CARTESIAN_POINT('Ctrl Pts',(-14.0295223410747,29.9740202447141,
-92.34995));
#135440=CARTESIAN_POINT('Ctrl Pts',(-14.5967291533814,29.7887068092282,
-92.34995));
#135441=CARTESIAN_POINT('Ctrl Pts',(-15.1723882243932,29.6527167117912,
-92.34995));
#135442=CARTESIAN_POINT('Ctrl Pts',(-16.3387077693334,29.4682775273239,
-92.34995));
#135443=CARTESIAN_POINT('Ctrl Pts',(-16.9293976390415,29.4199999800001,
-92.34995));
#135444=CARTESIAN_POINT('Ctrl Pts',(-17.5283605562717,29.41999998,-92.34995));
#135445=CARTESIAN_POINT('',(-17.5283474636365,28.4199999800081,-91.3499485560105));
#135446=CARTESIAN_POINT('Origin',(-17.5283605562717,29.41999998,-91.34995));
#135447=CARTESIAN_POINT('',(-13.862967014578,29.069410410554,-90.9403371832688));
#135448=CARTESIAN_POINT('Ctrl Pts',(-17.5283474636365,28.4199999800081,
-91.3499485560106));
#135449=CARTESIAN_POINT('Ctrl Pts',(-16.8748031850957,28.4200007859617,
-91.2778690188029));
#135450=CARTESIAN_POINT('Ctrl Pts',(-16.2331305712531,28.4803476839308,
-91.2065751585579));
#135451=CARTESIAN_POINT('Ctrl Pts',(-15.0125763307461,28.7036187831106,
-91.0700672040294));
#135452=CARTESIAN_POINT('Ctrl Pts',(-14.4321306085786,28.8596715997071,
-91.0047341003281));
#135453=CARTESIAN_POINT('Ctrl Pts',(-13.8629670146618,29.0694104105324,
-90.9403371832586));
#135454=CARTESIAN_POINT('Ctrl Pts',(-13.9704776589253,29.7932964571609,
-92.3317099697081));
#135455=CARTESIAN_POINT('Ctrl Pts',(-13.9485824763266,29.6507732526529,
-92.3041572803908));
#135456=CARTESIAN_POINT('Ctrl Pts',(-13.9277414892694,29.5120300570818,
-92.2444171371624));
#135457=CARTESIAN_POINT('Ctrl Pts',(-13.8924131672203,29.2732201982241,
-92.0703719609639));
#135458=CARTESIAN_POINT('Ctrl Pts',(-13.8776710606793,29.1715523493698,
-91.9547463954628));
#135459=CARTESIAN_POINT('Ctrl Pts',(-13.8571693529918,29.0291974882966,
-91.6899374203782));
#135460=CARTESIAN_POINT('Ctrl Pts',(-13.851254772454,28.9875557647693,-91.5391474846049));
#135461=CARTESIAN_POINT('Ctrl Pts',(-13.8496827900737,28.9765232161018,
-91.2324126084916));
#135462=CARTESIAN_POINT('Ctrl Pts',(-13.8539744318671,29.0067940350096,
-91.0793665022882));
#135463=CARTESIAN_POINT('Ctrl Pts',(-13.8629670146618,29.0694104105324,
-90.9403371832586));
#135464=CARTESIAN_POINT('Origin',(-60.,29.41999998,-91.34995));
#135465=CARTESIAN_POINT('',(-20.,28.4199999800001,-91.34995));
#135466=CARTESIAN_POINT('',(-16.1621051845127,28.4199999800001,-91.34995));
#135467=CARTESIAN_POINT('',(-20.,29.41999998,-92.34995));
#135468=CARTESIAN_POINT('',(-20.5,29.41999998,-92.34995));
#135469=CARTESIAN_POINT('Origin',(-20.,29.41999998,-91.34995));
#135470=CARTESIAN_POINT('Origin',(-20.,58.91999998,-91.84995));
#135471=CARTESIAN_POINT('',(-20.5,29.41999998,-91.84995));
#135472=CARTESIAN_POINT('Origin',(-20.,29.41999998,-91.84995));
#135473=CARTESIAN_POINT('',(-20.,46.41999998,-92.34995));
#135474=CARTESIAN_POINT('',(-20.,46.41999998,-92.34995));
#135475=CARTESIAN_POINT('',(-20.5,46.41999998,-91.84995));
#135476=CARTESIAN_POINT('Origin',(-20.,46.41999998,-91.84995));
#135477=CARTESIAN_POINT('',(-20.5,29.41999998,-91.84995));
#135478=CARTESIAN_POINT('Origin',(-21.,46.41999998,-91.84995));
#135479=CARTESIAN_POINT('',(-21.,47.41999998,-92.34995));
#135480=CARTESIAN_POINT('Origin',(-21.,46.41999998,-92.34995));
#135481=CARTESIAN_POINT('',(-21.,46.91999998,-91.84995));
#135482=CARTESIAN_POINT('Origin',(-21.,47.41999998,-91.84995));
#135483=CARTESIAN_POINT('Origin',(-21.,46.41999998,-91.84995));
#135484=CARTESIAN_POINT('Origin',(41.5,47.41999998,-91.84995));
#135485=CARTESIAN_POINT('',(-21.5,47.41999998,-92.34995));
#135486=CARTESIAN_POINT('',(41.5,47.41999998,-92.34995));
#135487=CARTESIAN_POINT('',(-21.5,46.91999998,-91.84995));
#135488=CARTESIAN_POINT('Origin',(-21.5,47.41999998,-91.84995));
#135489=CARTESIAN_POINT('',(39.,46.91999998,-91.84995));
#135490=CARTESIAN_POINT('Origin',(-21.5,46.41999998,-91.84995));
#135491=CARTESIAN_POINT('',(-22.5,46.41999998,-92.34995));
#135492=CARTESIAN_POINT('Origin',(-21.5,46.41999998,-92.34995));
#135493=CARTESIAN_POINT('',(-22.,46.41999998,-91.84995));
#135494=CARTESIAN_POINT('Origin',(-22.5,46.41999998,-91.84995));
#135495=CARTESIAN_POINT('Origin',(-21.5,46.41999998,-91.84995));
#135496=CARTESIAN_POINT('Origin',(-22.5,-9.33460238845303,-91.84995));
#135497=CARTESIAN_POINT('',(-22.5,29.41999998,-92.34995));
#135498=CARTESIAN_POINT('',(-22.5,29.41999998,-92.34995));
#135499=CARTESIAN_POINT('',(-22.,29.41999998,-91.84995));
#135500=CARTESIAN_POINT('Origin',(-22.5,29.41999998,-91.84995));
#135501=CARTESIAN_POINT('',(-22.,46.41999998,-91.84995));
#135502=CARTESIAN_POINT('Origin',(-60.,29.41999998,-91.34995));
#135503=CARTESIAN_POINT('',(-28.5,29.41999998,-92.34995));
#135504=CARTESIAN_POINT('',(-29.,29.41999998,-92.34995));
#135505=CARTESIAN_POINT('',(-28.5,28.41999998,-91.34995));
#135506=CARTESIAN_POINT('Origin',(-28.5,29.41999998,-91.34995));
#135507=CARTESIAN_POINT('',(-22.5,28.4199999800001,-91.34995));
#135508=CARTESIAN_POINT('',(-22.,28.4199999800001,-91.34995));
#135509=CARTESIAN_POINT('Origin',(-22.5,29.41999998,-91.34995));
#135510=CARTESIAN_POINT('Origin',(-28.5,58.91999998,-91.84995));
#135511=CARTESIAN_POINT('',(-29.,29.41999998,-91.84995));
#135512=CARTESIAN_POINT('Origin',(-28.5,29.41999998,-91.84995));
#135513=CARTESIAN_POINT('',(-28.5,46.41999998,-92.34995));
#135514=CARTESIAN_POINT('',(-28.5,46.41999998,-92.34995));
#135515=CARTESIAN_POINT('',(-29.,46.41999998,-91.84995));
#135516=CARTESIAN_POINT('Origin',(-28.5,46.41999998,-91.84995));
#135517=CARTESIAN_POINT('',(-29.,29.41999998,-91.84995));
#135518=CARTESIAN_POINT('Origin',(-29.5,46.41999998,-91.84995));
#135519=CARTESIAN_POINT('',(-29.5,47.41999998,-92.34995));
#135520=CARTESIAN_POINT('Origin',(-29.5,46.41999998,-92.34995));
#135521=CARTESIAN_POINT('',(-29.5,46.91999998,-91.84995));
#135522=CARTESIAN_POINT('Origin',(-29.5,47.41999998,-91.84995));
#135523=CARTESIAN_POINT('Origin',(-29.5,46.41999998,-91.84995));
#135524=CARTESIAN_POINT('Origin',(41.5,47.41999998,-91.84995));
#135525=CARTESIAN_POINT('',(-30.,47.41999998,-92.34995));
#135526=CARTESIAN_POINT('',(41.5,47.41999998,-92.34995));
#135527=CARTESIAN_POINT('',(-30.,46.91999998,-91.84995));
#135528=CARTESIAN_POINT('Origin',(-30.,47.41999998,-91.84995));
#135529=CARTESIAN_POINT('',(39.,46.91999998,-91.84995));
#135530=CARTESIAN_POINT('Origin',(-30.,46.41999998,-91.84995));
#135531=CARTESIAN_POINT('',(-31.,46.41999998,-92.34995));
#135532=CARTESIAN_POINT('Origin',(-30.,46.41999998,-92.34995));
#135533=CARTESIAN_POINT('',(-30.5,46.41999998,-91.84995));
#135534=CARTESIAN_POINT('Origin',(-31.,46.41999998,-91.84995));
#135535=CARTESIAN_POINT('Origin',(-30.,46.41999998,-91.84995));
#135536=CARTESIAN_POINT('Origin',(-31.,-9.33460238845303,-91.84995));
#135537=CARTESIAN_POINT('',(-31.,29.41999998,-92.34995));
#135538=CARTESIAN_POINT('',(-31.,29.41999998,-92.34995));
#135539=CARTESIAN_POINT('',(-30.5,29.41999998,-91.84995));
#135540=CARTESIAN_POINT('Origin',(-31.,29.41999998,-91.84995));
#135541=CARTESIAN_POINT('',(-30.5,46.41999998,-91.84995));
#135542=CARTESIAN_POINT('Origin',(-60.,29.41999998,-91.34995));
#135543=CARTESIAN_POINT('',(-37.,29.41999998,-92.34995));
#135544=CARTESIAN_POINT('',(-37.5,29.41999998,-92.34995));
#135545=CARTESIAN_POINT('',(-37.,28.41999998,-91.34995));
#135546=CARTESIAN_POINT('Origin',(-37.,29.41999998,-91.34995));
#135547=CARTESIAN_POINT('',(-31.,28.41999998,-91.34995));
#135548=CARTESIAN_POINT('',(-30.5,28.41999998,-91.34995));
#135549=CARTESIAN_POINT('Origin',(-31.,29.41999998,-91.34995));
#135550=CARTESIAN_POINT('Origin',(-37.,58.91999998,-91.84995));
#135551=CARTESIAN_POINT('',(-37.5,29.41999998,-91.84995));
#135552=CARTESIAN_POINT('Origin',(-37.,29.41999998,-91.84995));
#135553=CARTESIAN_POINT('',(-37.,46.41999998,-92.34995));
#135554=CARTESIAN_POINT('',(-37.5,29.41999998,-91.84995));
#135555=CARTESIAN_POINT('Origin',(-41.5,58.91999998,-92.34995));
#135556=CARTESIAN_POINT('',(-41.5,28.91999998,-171.14995));
#135557=CARTESIAN_POINT('',(-41.5,28.91999998,-171.64995));
#135558=CARTESIAN_POINT('',(-41.5,58.91999998,-174.34995));
#135559=CARTESIAN_POINT('',(-41.5,58.91999998,-92.34995));
#135560=CARTESIAN_POINT('',(-41.5,37.8417754273786,-174.34995));
#135561=CARTESIAN_POINT('',(-41.5,58.91999998,-174.34995));
#135562=CARTESIAN_POINT('',(-41.5,37.8417754273786,-172.64995));
#135563=CARTESIAN_POINT('',(-41.5,37.8417754273786,-92.34995));
#135564=CARTESIAN_POINT('',(-41.5,36.3270340686007,-171.14995));
#135565=CARTESIAN_POINT('Ctrl Pts',(-41.5,36.3270340686007,-171.14995));
#135566=CARTESIAN_POINT('Ctrl Pts',(-41.5,36.5253489879757,-171.149950000016));
#135567=CARTESIAN_POINT('Ctrl Pts',(-41.5,36.7235144279567,-171.18899099047));
#135568=CARTESIAN_POINT('Ctrl Pts',(-41.5,37.0898865538897,-171.339270411997));
#135569=CARTESIAN_POINT('Ctrl Pts',(-41.5,37.2579134125323,-171.450449746589));
#135570=CARTESIAN_POINT('Ctrl Pts',(-41.5,37.5383224977403,-171.728129909852));
#135571=CARTESIAN_POINT('Ctrl Pts',(-41.5,37.6505944553831,-171.894521542842));
#135572=CARTESIAN_POINT('Ctrl Pts',(-41.5,37.8023507586648,-172.257328160063));
#135573=CARTESIAN_POINT('Ctrl Pts',(-41.5,37.8417754273637,-172.453565067926));
#135574=CARTESIAN_POINT('Ctrl Pts',(-41.5,37.8417754273786,-172.64995));
#135575=CARTESIAN_POINT('',(-41.5,32.6685811839606,-171.14995));
#135576=CARTESIAN_POINT('',(-41.5,36.3973044859519,-171.14995));
#135577=CARTESIAN_POINT('',(-41.5,30.4123236926243,-171.14995));
#135578=CARTESIAN_POINT('Ctrl Pts',(-41.5,30.4123236926243,-171.14995));
#135579=CARTESIAN_POINT('Ctrl Pts',(-41.5,30.6002475127106,-171.149950044596));
#135580=CARTESIAN_POINT('Ctrl Pts',(-41.4999999999992,30.7880947817855,
-171.167358426712));
#135581=CARTESIAN_POINT('Ctrl Pts',(-41.5000000000009,30.9759786884911,
-171.183208448531));
#135582=CARTESIAN_POINT('Ctrl Pts',(-41.5000000000009,30.976120931185,-171.183220448228));
#135583=CARTESIAN_POINT('Ctrl Pts',(-41.5000000000009,30.9762631739402,
-171.183232446501));
#135584=CARTESIAN_POINT('Ctrl Pts',(-41.5000000000009,30.9764054167567,
-171.183244443348));
#135585=CARTESIAN_POINT('Ctrl Pts',(-41.5000000000023,31.1369344019092,
-171.196783556864));
#135586=CARTESIAN_POINT('Ctrl Pts',(-41.4999999999993,31.2974626498935,
-171.208492413821));
#135587=CARTESIAN_POINT('Ctrl Pts',(-41.500000000002,31.4579880082369,-171.211623701833));
#135588=CARTESIAN_POINT('Ctrl Pts',(-41.5000000000025,31.4852425169035,
-171.212155341925));
#135589=CARTESIAN_POINT('Ctrl Pts',(-41.5000000000032,31.5124969442739,
-171.212439843791));
#135590=CARTESIAN_POINT('Ctrl Pts',(-41.5000000000045,31.5397512823877,
-171.212444366369));
#135591=CARTESIAN_POINT('Ctrl Pts',(-41.5000000000045,31.5399934772056,
-171.212444406558));
#135592=CARTESIAN_POINT('Ctrl Pts',(-41.5000000000045,31.5402356720169,
-171.212444424596));
#135593=CARTESIAN_POINT('Ctrl Pts',(-41.5000000000045,31.5404778668211,
-171.212444420506));
#135594=CARTESIAN_POINT('Ctrl Pts',(-41.5000000000123,31.7017281895667,
-171.21244169735));
#135595=CARTESIAN_POINT('Ctrl Pts',(-41.5000000000007,31.8629751163933,
-171.202628065385));
#135596=CARTESIAN_POINT('Ctrl Pts',(-41.5000000000001,32.0242208996094,
-171.189830777503));
#135597=CARTESIAN_POINT('Ctrl Pts',(-41.5,32.0508620129899,-171.187716402848));
#135598=CARTESIAN_POINT('Ctrl Pts',(-41.5,32.0775031023629,-171.185520466759));
#135599=CARTESIAN_POINT('Ctrl Pts',(-41.5,32.1041441836616,-171.183273657173));
#135600=CARTESIAN_POINT('Ctrl Pts',(-41.5,32.1042728698424,-171.18326280426));
#135601=CARTESIAN_POINT('Ctrl Pts',(-41.5,32.1044015560177,-171.183251950612));
#135602=CARTESIAN_POINT('Ctrl Pts',(-41.5,32.1045302421874,-171.183241096235));
#135603=CARTESIAN_POINT('Ctrl Pts',(-41.5000000000001,32.2434923963757,
-171.171519963656));
#135604=CARTESIAN_POINT('Ctrl Pts',(-41.5,32.3824542184576,-171.158942972389));
#135605=CARTESIAN_POINT('Ctrl Pts',(-41.5,32.5214184450654,-171.153174108104));
#135606=CARTESIAN_POINT('Ctrl Pts',(-41.5,32.5704723625825,-171.151137717878));
#135607=CARTESIAN_POINT('Ctrl Pts',(-41.5,32.6195265765183,-171.149950012104));
#135608=CARTESIAN_POINT('Ctrl Pts',(-41.5,32.6685811839606,-171.14995));
#135609=CARTESIAN_POINT('',(-41.5,36.3973044859519,-171.14995));
#135610=CARTESIAN_POINT('Origin',(-38.5,58.91999998,-174.34995));
#135611=CARTESIAN_POINT('',(-38.5,58.91999998,-177.34995));
#135612=CARTESIAN_POINT('Origin',(-38.5,58.91999998,-174.34995));
#135613=CARTESIAN_POINT('',(-38.5,38.333668348837,-177.34995));
#135614=CARTESIAN_POINT('',(-38.5,58.91999998,-177.34995));
#135615=CARTESIAN_POINT('Ctrl Pts',(-41.5,37.8417754273786,-174.34995));
#135616=CARTESIAN_POINT('Ctrl Pts',(-41.5,37.8417754273818,-174.742719880575));
#135617=CARTESIAN_POINT('Ctrl Pts',(-41.4219180279654,37.8545780838243,
-175.135193658002));
#135618=CARTESIAN_POINT('Ctrl Pts',(-41.1213591671024,37.9038590092046,
-175.860806936189));
#135619=CARTESIAN_POINT('Ctrl Pts',(-40.8990005234543,37.9403178901501,
-176.193590163665));
#135620=CARTESIAN_POINT('Ctrl Pts',(-40.343640163665,38.0313771667621,-176.748950523454));
#135621=CARTESIAN_POINT('Ctrl Pts',(-40.0108569362568,38.0859417380754,
-176.971309167074));
#135622=CARTESIAN_POINT('Ctrl Pts',(-39.2852436579338,38.204916416519,-177.271868027993));
#135623=CARTESIAN_POINT('Ctrl Pts',(-38.8927698806272,38.2692681074913,
-177.34995));
#135624=CARTESIAN_POINT('Ctrl Pts',(-38.5,38.333668348837,-177.34995));
#135625=CARTESIAN_POINT('Origin',(-27.0372992073901,44.4888699625078,-177.84995));
#135626=CARTESIAN_POINT('',(-26.4110202530699,40.0326636531708,-177.34995));
#135627=CARTESIAN_POINT('',(-26.3414337025898,39.5375296188,-177.84995));
#135628=CARTESIAN_POINT('Origin',(-26.4110202530699,40.0326636531708,-177.84995));
#135629=CARTESIAN_POINT('',(-25.121270129701,40.4171587039029,-177.34995));
#135630=CARTESIAN_POINT('Origin',(-27.0372992073901,44.4888699625078,-177.34995));
#135631=CARTESIAN_POINT('',(-24.9083780099579,39.9647463418357,-177.84995));
#135632=CARTESIAN_POINT('Origin',(-25.121270129701,40.4171587039029,-177.84995));
#135633=CARTESIAN_POINT('Origin',(-27.0372992073901,44.4888699625078,-177.84995));
#135634=CARTESIAN_POINT('Origin',(-45.6308101826775,37.3314983336592,-177.84995));
#135635=CARTESIAN_POINT('',(-38.43041344952,37.8385343144662,-177.84995));
#135636=CARTESIAN_POINT('Origin',(-38.5,38.333668348837,-177.84995));
#135637=CARTESIAN_POINT('',(42.7876488459256,49.7579023686377,-177.34995));
#135638=CARTESIAN_POINT('',(-45.5612236321975,36.8363642992885,-177.84995));
#135639=CARTESIAN_POINT('Origin',(-27.0372992073901,44.4888699625078,-179.64995));
#135640=CARTESIAN_POINT('',(-24.9083780099579,39.9647463418357,-179.39995));
#135641=CARTESIAN_POINT('',(-24.9083780099579,39.9647463418357,-179.64995));
#135642=CARTESIAN_POINT('',(-26.3414337025898,39.5375296188,-179.39995));
#135643=CARTESIAN_POINT('Origin',(-27.0372992073901,44.4888699625078,-179.39995));
#135644=CARTESIAN_POINT('',(-26.3414337025898,39.5375296188,-171.64995));
#135645=CARTESIAN_POINT('Origin',(-27.0372992073901,44.4888699625078,-179.39995));
#135646=CARTESIAN_POINT('',(-26.3066404273498,39.2899626016146,-179.64995));
#135647=CARTESIAN_POINT('Origin',(-26.3066404273498,39.2899626016146,-179.39995));
#135648=CARTESIAN_POINT('',(-24.8019319500862,39.7385401608021,-179.64995));
#135649=CARTESIAN_POINT('Origin',(-24.8019319500862,39.7385401608021,-179.39995));
#135650=CARTESIAN_POINT('Origin',(-27.0372992073901,44.4888699625078,-179.64995));
#135651=CARTESIAN_POINT('Origin',(-62.8299850317005,34.1569412647963,-179.39995));
#135652=CARTESIAN_POINT('',(-44.628608857647,36.9674347581595,-179.39995));
#135653=CARTESIAN_POINT('',(-44.593815582407,36.7198677409741,-179.64995));
#135654=CARTESIAN_POINT('Origin',(-44.593815582407,36.7198677409741,-179.39995));
#135655=CARTESIAN_POINT('',(-26.3414337025898,39.5375296188,-179.39995));
#135656=CARTESIAN_POINT('',(-44.593815582407,36.7198677409741,-179.64995));
#135657=CARTESIAN_POINT('Origin',(-44.2110895547669,33.9966305519348,-179.39995));
#135658=CARTESIAN_POINT('',(-46.2674193015002,36.1810087180727,-179.39995));
#135659=CARTESIAN_POINT('',(-46.0960584892724,35.9989772042278,-179.64995));
#135660=CARTESIAN_POINT('Origin',(-46.0960584892724,35.9989772042278,-179.39995));
#135661=CARTESIAN_POINT('Origin',(-44.2110895547669,33.9966305519348,-179.39995));
#135662=CARTESIAN_POINT('Origin',(-44.2110895547669,33.9966305519348,-179.64995));
#135663=CARTESIAN_POINT('Origin',(0.,-12.9675000200281,-179.39995));
#135664=CARTESIAN_POINT('',(-49.1485087381009,33.2999192814719,-179.39995));
#135665=CARTESIAN_POINT('',(-48.9664772242561,33.1285584692441,-179.64995));
#135666=CARTESIAN_POINT('Origin',(-48.9664772242561,33.1285584692441,-179.39995));
#135667=CARTESIAN_POINT('Origin',(0.,-12.9675000200281,-179.39995));
#135668=CARTESIAN_POINT('Origin',(0.,-12.9675000200281,-179.64995));
#135669=CARTESIAN_POINT('Origin',(-46.9641305719631,31.2435895347386,-179.39995));
#135670=CARTESIAN_POINT('',(-49.9349347781878,31.6611088376188,-179.39995));
#135671=CARTESIAN_POINT('',(-49.6873677610025,31.6263155623787,-179.64995));
#135672=CARTESIAN_POINT('Origin',(-49.6873677610024,31.6263155623787,-179.39995));
#135673=CARTESIAN_POINT('Origin',(-46.9641305719631,31.2435895347386,-179.39995));
#135674=CARTESIAN_POINT('Origin',(-46.9641305719631,31.2435895347386,-179.64995));
#135675=CARTESIAN_POINT('Origin',(-61.3785689046687,-51.5609030735669,-179.39995));
#135676=CARTESIAN_POINT('',(-52.5050296388285,13.3739336825608,-179.39995));
#135677=CARTESIAN_POINT('',(-52.2574626216432,13.3391404073208,-179.64995));
#135678=CARTESIAN_POINT('Origin',(-52.2574626216431,13.3391404073208,-179.39995));
#135679=CARTESIAN_POINT('',(-49.9349347781878,31.6611088376188,-179.39995));
#135680=CARTESIAN_POINT('',(-52.2574626216432,13.3391404073208,-179.64995));
#135681=CARTESIAN_POINT('Origin',(-57.4563699825364,14.0697991873612,-179.39995));
#135682=CARTESIAN_POINT('',(-52.9322463618642,11.9408779899289,-179.39995));
#135683=CARTESIAN_POINT('',(-52.7060401808306,11.8344319300573,-179.64995));
#135684=CARTESIAN_POINT('Origin',(-52.7060401808306,11.8344319300573,-179.39995));
#135685=CARTESIAN_POINT('Origin',(-57.4563699825364,14.0697991873612,-179.39995));
#135686=CARTESIAN_POINT('Origin',(-57.4563699825364,14.0697991873612,-179.64995));
#135687=CARTESIAN_POINT('Origin',(0.,-12.9675000200281,-179.39995));
#135688=CARTESIAN_POINT('',(-52.9322463618642,-37.8758780299853,-179.39995));
#135689=CARTESIAN_POINT('',(-52.7060401808306,-37.7694319701137,-179.64995));
#135690=CARTESIAN_POINT('Origin',(-52.7060401808306,-37.7694319701137,-179.39995));
#135691=CARTESIAN_POINT('Origin',(0.,-12.9675000200281,-179.39995));
#135692=CARTESIAN_POINT('Origin',(0.,-12.9675000200281,-179.64995));
#135693=CARTESIAN_POINT('Origin',(-57.4563699825363,-40.0047992274175,-179.39995));
#135694=CARTESIAN_POINT('',(-52.5050296388285,-39.3089337226171,-179.39995));
#135695=CARTESIAN_POINT('',(-52.2574626216431,-39.2741404473771,-179.64995));
#135696=CARTESIAN_POINT('Origin',(-52.2574626216431,-39.2741404473771,-179.39995));
#135697=CARTESIAN_POINT('Origin',(-57.4563699825363,-40.0047992274175,-179.39995));
#135698=CARTESIAN_POINT('Origin',(-57.4563699825363,-40.0047992274175,-179.64995));
#135699=CARTESIAN_POINT('Origin',(-50.3220654694669,-53.04520674476,-179.39995));
#135700=CARTESIAN_POINT('',(-49.9349347781878,-57.596108877675,-179.39995));
#135701=CARTESIAN_POINT('',(-49.6873677610024,-57.561315602435,-179.64995));
#135702=CARTESIAN_POINT('Origin',(-49.6873677610024,-57.561315602435,-179.39995));
#135703=CARTESIAN_POINT('',(-52.5050296388285,-39.3089337226171,-179.39995));
#135704=CARTESIAN_POINT('',(-49.6873677610024,-57.561315602435,-179.64995));
#135705=CARTESIAN_POINT('Origin',(-46.9641305719631,-57.1785895747948,-179.39995));
#135706=CARTESIAN_POINT('',(-49.148508738101,-59.2349193215281,-179.39995));
#135707=CARTESIAN_POINT('',(-48.9664772242561,-59.0635585093003,-179.64995));
#135708=CARTESIAN_POINT('Origin',(-48.9664772242561,-59.0635585093003,-179.39995));
#135709=CARTESIAN_POINT('Origin',(-46.9641305719631,-57.1785895747948,-179.39995));
#135710=CARTESIAN_POINT('Origin',(-46.9641305719631,-57.1785895747948,-179.64995));
#135711=CARTESIAN_POINT('Origin',(0.,-12.9675000200281,-179.39995));
#135712=CARTESIAN_POINT('',(-46.2674193015002,-62.1160087581289,-179.39995));
#135713=CARTESIAN_POINT('',(-46.0960584892725,-61.9339772442841,-179.64995));
#135714=CARTESIAN_POINT('Origin',(-46.0960584892725,-61.9339772442841,-179.39995));
#135715=CARTESIAN_POINT('Origin',(0.,-12.9675000200281,-179.39995));
#135716=CARTESIAN_POINT('Origin',(0.,-12.9675000200281,-179.64995));
#135717=CARTESIAN_POINT('Origin',(-44.2110895547669,-59.9316305919911,-179.39995));
#135718=CARTESIAN_POINT('',(-44.628608857647,-62.9024347982158,-179.39995));
#135719=CARTESIAN_POINT('',(-44.5938155824071,-62.6548677810304,-179.64995));
#135720=CARTESIAN_POINT('Origin',(-44.5938155824071,-62.6548677810303,-179.39995));
#135721=CARTESIAN_POINT('Origin',(-44.2110895547669,-59.9316305919911,-179.39995));
#135722=CARTESIAN_POINT('Origin',(-44.2110895547669,-59.9316305919911,-179.64995));
#135723=CARTESIAN_POINT('Origin',(-51.7734815964994,-61.6458315265255,-179.39995));
#135724=CARTESIAN_POINT('',(-26.0394480946395,-65.5149709682656,-179.39995));
#135725=CARTESIAN_POINT('',(-26.0046548193995,-65.2674039510802,-179.64995));
#135726=CARTESIAN_POINT('Origin',(-26.0046548193995,-65.2674039510803,-179.39995));
#135727=CARTESIAN_POINT('',(-44.628608857647,-62.9024347982158,-179.39995));
#135728=CARTESIAN_POINT('',(-26.0046548193995,-65.2674039510802,-179.64995));
#135729=CARTESIAN_POINT('Origin',(-26.4569673975197,-68.4857751744904,-179.39995));
#135730=CARTESIAN_POINT('',(-25.166383622031,-65.7775666303703,-179.39995));
#135731=CARTESIAN_POINT('',(-25.0588349740736,-65.5518825850269,-179.64995));
#135732=CARTESIAN_POINT('Origin',(-25.0588349740736,-65.5518825850269,-179.39995));
#135733=CARTESIAN_POINT('Origin',(-26.4569673975197,-68.4857751744904,-179.39995));
#135734=CARTESIAN_POINT('Origin',(-26.4569673975197,-68.4857751744904,-179.64995));
#135735=CARTESIAN_POINT('Origin',(-44.5079524583208,-57.4754524783487,-171.64995));
#135736=CARTESIAN_POINT('',(-43.1572831724514,-55.08000002,-171.64995));
#135737=CARTESIAN_POINT('',(-45.8586217441902,-55.08000002,-171.64995));
#135738=CARTESIAN_POINT('Ctrl Pts',(-45.8586217441902,-55.08000002,-171.64995));
#135739=CARTESIAN_POINT('Ctrl Pts',(-45.7689536596569,-55.0294409169463,
-171.64995));
#135740=CARTESIAN_POINT('Ctrl Pts',(-45.6765174633176,-54.9839564622376,
-171.649937574984));
#135741=CARTESIAN_POINT('Ctrl Pts',(-45.4778485953858,-54.8996925932595,
-171.64992638429));
#135742=CARTESIAN_POINT('Ctrl Pts',(-45.371333860312,-54.8620619965585,
-171.649947040217));
#135743=CARTESIAN_POINT('Ctrl Pts',(-45.1857602021761,-54.8090884744686,
-171.649951805482));
#135744=CARTESIAN_POINT('Ctrl Pts',(-45.1077985401449,-54.7904750984752,
-171.649838856786));
#135745=CARTESIAN_POINT('Ctrl Pts',(-44.9203791059924,-54.7542997329157,
-171.649614268465));
#135746=CARTESIAN_POINT('Ctrl Pts',(-44.8104650288131,-54.73989862651,-171.649606832116));
#135747=CARTESIAN_POINT('Ctrl Pts',(-44.6361116415896,-54.7276946232682,
-171.649829887348));
#135748=CARTESIAN_POINT('Ctrl Pts',(-44.572121425011,-54.7254562445457,
-171.649942496644));
#135749=CARTESIAN_POINT('Ctrl Pts',(-44.4919713617221,-54.7254515344574,
-171.649951467562));
#135750=CARTESIAN_POINT('Ctrl Pts',(-44.4758287519422,-54.7255927281285,
-171.649946189807));
#135751=CARTESIAN_POINT('Ctrl Pts',(-44.3973353016952,-54.7269705335247,
-171.649899299462));
#135752=CARTESIAN_POINT('Ctrl Pts',(-44.3350361171979,-54.7301856687744,
-171.649800793763));
#135753=CARTESIAN_POINT('Ctrl Pts',(-44.24589448532,-54.7378330706293,-171.64971310718));
#135754=CARTESIAN_POINT('Ctrl Pts',(-44.2189296557681,-54.7405484163111,
-171.649692645932));
#135755=CARTESIAN_POINT('Ctrl Pts',(-44.1669378685671,-54.7465614902616,
-171.649670825756));
#135756=CARTESIAN_POINT('Ctrl Pts',(-44.141907947472,-54.7498060612266,
-171.649668207626));
#135757=CARTESIAN_POINT('Ctrl Pts',(-44.0251905251421,-54.7665726407083,
-171.649692857457));
#135758=CARTESIAN_POINT('Ctrl Pts',(-43.9341908339778,-54.7843774385806,
-171.64983557602));
#135759=CARTESIAN_POINT('Ctrl Pts',(-43.7178584587823,-54.8381778103583,
-171.650016020842));
#135760=CARTESIAN_POINT('Ctrl Pts',(-43.5938526567541,-54.8785531161362,
-171.649916571135));
#135761=CARTESIAN_POINT('Ctrl Pts',(-43.3647423777249,-54.9716018333704,
-171.649923778305));
#135762=CARTESIAN_POINT('Ctrl Pts',(-43.2592299860174,-55.0225175893235,
-171.64995));
#135763=CARTESIAN_POINT('Ctrl Pts',(-43.1572831724514,-55.08000002,-171.64995));
#135764=CARTESIAN_POINT('',(-44.5079524583208,-60.2254524783487,-171.64995));
#135765=CARTESIAN_POINT('Origin',(-44.5079524583208,-57.4754524783487,-171.64995));
#135766=CARTESIAN_POINT('',(-44.5079524583208,-60.2254524783487,-179.64995));
#135767=CARTESIAN_POINT('',(-44.5079524583208,-60.2254524783487,-171.64995));
#135768=CARTESIAN_POINT('Origin',(-44.5079524583208,-57.4754524783487,-179.64995));
#135769=CARTESIAN_POINT('',(-42.,-58.6035812240168,-171.64995));
#135770=CARTESIAN_POINT('Origin',(-44.5079524583208,-57.4754524783487,-171.64995));
#135771=CARTESIAN_POINT('',(-42.,-56.3473237326807,-171.64995));
#135772=CARTESIAN_POINT('Ctrl Pts',(-42.,-58.6035812240168,-171.64995));
#135773=CARTESIAN_POINT('Ctrl Pts',(-41.9586127577212,-58.5115728992446,
-171.64995));
#135774=CARTESIAN_POINT('Ctrl Pts',(-41.9223200866005,-58.4173567491321,
-171.649936040447));
#135775=CARTESIAN_POINT('Ctrl Pts',(-41.8579031946499,-58.2180944893019,
-171.649932806722));
#135776=CARTESIAN_POINT('Ctrl Pts',(-41.8306620008006,-58.1129431414185,
-171.649968769067));
#135777=CARTESIAN_POINT('Ctrl Pts',(-41.7951274186659,-57.9323775711287,
-171.649917110529));
#135778=CARTESIAN_POINT('Ctrl Pts',(-41.7836058362705,-57.8577298063974,
-171.649879920008));
#135779=CARTESIAN_POINT('Ctrl Pts',(-41.7636999883713,-57.6806798505216,
-171.649872834512));
#135780=CARTESIAN_POINT('Ctrl Pts',(-41.7579524619681,-57.5781054625683,
-171.649950538122));
#135781=CARTESIAN_POINT('Ctrl Pts',(-41.7579524619681,-57.3728595819388,
-171.649949462193));
#135782=CARTESIAN_POINT('Ctrl Pts',(-41.7636932451378,-57.2703453579385,
-171.649869923244));
#135783=CARTESIAN_POINT('Ctrl Pts',(-41.7835828980498,-57.09333489844,-171.649877908044));
#135784=CARTESIAN_POINT('Ctrl Pts',(-41.7951032511141,-57.0186677636544,
-171.649916441382));
#135785=CARTESIAN_POINT('Ctrl Pts',(-41.8306429216695,-56.8380335332052,
-171.649969369358));
#135786=CARTESIAN_POINT('Ctrl Pts',(-41.857894634129,-56.7328337987611,
-171.64993233013));
#135787=CARTESIAN_POINT('Ctrl Pts',(-41.9223259722371,-56.5335329279264,
-171.649935735269));
#135788=CARTESIAN_POINT('Ctrl Pts',(-41.9586161144824,-56.4393245950087,
-171.64995));
#135789=CARTESIAN_POINT('Ctrl Pts',(-42.,-56.3473237326807,-171.64995));
#135790=CARTESIAN_POINT('Origin',(-44.5079524583208,-57.4754524783487,-171.64995));
#135791=CARTESIAN_POINT('Origin',(-44.5079524583208,31.5404524382925,-171.64995));
#135792=CARTESIAN_POINT('',(-42.,32.6685811839606,-171.64995));
#135793=CARTESIAN_POINT('',(-45.342056117244,28.91999998,-171.64995));
#135794=CARTESIAN_POINT('Origin',(-44.5079524583208,31.5404524382925,-171.64995));
#135795=CARTESIAN_POINT('',(-44.507948362235,28.7904524382955,-171.649949999922));
#135796=CARTESIAN_POINT('Ctrl Pts',(-45.342056117244,28.91999998,-171.64995));
#135797=CARTESIAN_POINT('Ctrl Pts',(-45.2444197705179,28.8889218225657,
-171.64995));
#135798=CARTESIAN_POINT('Ctrl Pts',(-45.145122736077,28.8633247324813,-171.649944548176));
#135799=CARTESIAN_POINT('Ctrl Pts',(-44.9394245210704,28.8223946394273,
-171.649950242553));
#135800=CARTESIAN_POINT('Ctrl Pts',(-44.8330844822692,28.8076342035681,
-171.649941034682));
#135801=CARTESIAN_POINT('Ctrl Pts',(-44.6535626787428,28.7933447394312,
-171.649939912182));
#135802=CARTESIAN_POINT('Ctrl Pts',(-44.5807739260493,28.7904524382925,
-171.649950037878));
#135803=CARTESIAN_POINT('Ctrl Pts',(-44.5079524583208,28.7904524382925,
-171.649949999924));
#135804=CARTESIAN_POINT('',(-44.5079524583208,28.7904524382925,-179.64995));
#135805=CARTESIAN_POINT('',(-44.5079524583208,28.7904524382925,-171.64995));
#135806=CARTESIAN_POINT('Origin',(-44.5079524583208,31.5404524382925,-179.64995));
#135807=CARTESIAN_POINT('',(-43.6738487993976,28.91999998,-171.64995));
#135808=CARTESIAN_POINT('Ctrl Pts',(-44.507948362235,28.7904524382955,-171.649949999922));
#135809=CARTESIAN_POINT('Ctrl Pts',(-44.4351555237766,28.7904525467194,
-171.64994996145));
#135810=CARTESIAN_POINT('Ctrl Pts',(-44.3623912990527,28.7933428984961,
-171.649939477139));
#135811=CARTESIAN_POINT('Ctrl Pts',(-44.1829187602443,28.8076233386202,
-171.649940713495));
#135812=CARTESIAN_POINT('Ctrl Pts',(-44.0765991739455,28.8223766210747,
-171.649950205311));
#135813=CARTESIAN_POINT('Ctrl Pts',(-43.8708734141959,28.8633012176256,
-171.649945186597));
#135814=CARTESIAN_POINT('Ctrl Pts',(-43.7715300191675,28.8889075392422,
-171.64995));
#135815=CARTESIAN_POINT('Ctrl Pts',(-43.6738487993977,28.91999998,-171.64995));
#135816=CARTESIAN_POINT('',(-42.,30.4123236926243,-171.64995));
#135817=CARTESIAN_POINT('Origin',(-44.5079524583208,31.5404524382925,-171.64995));
#135818=CARTESIAN_POINT('Ctrl Pts',(-42.,30.4123236926244,-171.64995));
#135819=CARTESIAN_POINT('Ctrl Pts',(-41.9586127577212,30.5043320173966,
-171.64995));
#135820=CARTESIAN_POINT('Ctrl Pts',(-41.9223200866006,30.5985481675089,
-171.649936040447));
#135821=CARTESIAN_POINT('Ctrl Pts',(-41.85790319465,30.7978104273388,-171.649932806722));
#135822=CARTESIAN_POINT('Ctrl Pts',(-41.8306620008007,30.902961775222,-171.649968769066));
#135823=CARTESIAN_POINT('Ctrl Pts',(-41.7951274186661,31.0835273455116,
-171.649917110529));
#135824=CARTESIAN_POINT('Ctrl Pts',(-41.7836058362707,31.1581751102429,
-171.649879920008));
#135825=CARTESIAN_POINT('Ctrl Pts',(-41.7636999883716,31.3352250661166,
-171.649872834512));
#135826=CARTESIAN_POINT('Ctrl Pts',(-41.7579524619681,31.4377994540703,
-171.649950538122));
#135827=CARTESIAN_POINT('Ctrl Pts',(-41.7579524619681,31.6430453346998,
-171.649949462193));
#135828=CARTESIAN_POINT('Ctrl Pts',(-41.7636932451375,31.7455595586996,
-171.649869923244));
#135829=CARTESIAN_POINT('Ctrl Pts',(-41.7835828980496,31.9225700182004,
-171.649877908044));
#135830=CARTESIAN_POINT('Ctrl Pts',(-41.795103251114,31.9972371529859,-171.649916441382));
#135831=CARTESIAN_POINT('Ctrl Pts',(-41.8306429216694,32.1778713834354,
-171.649969369358));
#135832=CARTESIAN_POINT('Ctrl Pts',(-41.8578946341289,32.2830711178797,
-171.64993233013));
#135833=CARTESIAN_POINT('Ctrl Pts',(-41.922325972237,32.4823719887145,-171.649935735269));
#135834=CARTESIAN_POINT('Ctrl Pts',(-41.9586161144823,32.5765803216321,
-171.64995));
#135835=CARTESIAN_POINT('Ctrl Pts',(-42.,32.6685811839606,-171.64995));
#135836=CARTESIAN_POINT('Ctrl Pts',(-24.2000000000011,-66.7760495265879,
-177.34995));
#135837=CARTESIAN_POINT('Ctrl Pts',(-23.9949152542386,-66.320044869753,
-177.34995));
#135838=CARTESIAN_POINT('Ctrl Pts',(-23.9949152542395,-66.3200448697526,
-177.84995));
#135839=CARTESIAN_POINT('Ctrl Pts',(-24.1371859654851,-66.8325498277328,
-177.34995));
#135840=CARTESIAN_POINT('Ctrl Pts',(-23.9206657457682,-66.3534380400361,
-177.323497139763));
#135841=CARTESIAN_POINT('Ctrl Pts',(-23.8703538324233,-66.3760654545035,
-177.849949984965));
#135842=CARTESIAN_POINT('Ctrl Pts',(-24.0753687900163,-66.8876168115863,
-177.338353763422));
#135843=CARTESIAN_POINT('Ctrl Pts',(-23.85857311611,-66.3812761568117,-177.28202856183));
#135844=CARTESIAN_POINT('Ctrl Pts',(-23.7477652296632,-66.4306666697135,
-177.82675752222));
#135845=CARTESIAN_POINT('Ctrl Pts',(-23.9567084144264,-66.9924080535444,
-177.291402578445));
#135846=CARTESIAN_POINT('Ctrl Pts',(-23.7605684693856,-66.4255018631538,
-177.182659406882));
#135847=CARTESIAN_POINT('Ctrl Pts',(-23.5124556672824,-66.534569849442,
-177.732855161513));
#135848=CARTESIAN_POINT('Ctrl Pts',(-23.9022748831747,-67.0400066306863,
-177.256984676403));
#135849=CARTESIAN_POINT('Ctrl Pts',(-23.728650188117,-66.4401283754592,
-177.126465197113));
#135850=CARTESIAN_POINT('Ctrl Pts',(-23.4045112120254,-66.5817650498296,
-177.66401934989));
#135851=CARTESIAN_POINT('Ctrl Pts',(-23.8072189577995,-67.1225998569154,
-177.166241836555));
#135852=CARTESIAN_POINT('Ctrl Pts',(-23.6923095199098,-66.4575908379652,
-177.01948600884));
#135853=CARTESIAN_POINT('Ctrl Pts',(-23.2160104726183,-66.6636583322845,
-177.482533676026));
#135854=CARTESIAN_POINT('Ctrl Pts',(-23.7683864506384,-67.1560455904002,
-177.111255395708));
#135855=CARTESIAN_POINT('Ctrl Pts',(-23.6901782519314,-66.4593985440301,
-176.972463316884));
#135856=CARTESIAN_POINT('Ctrl Pts',(-23.1390036429345,-66.6968206283899,
-177.372560789955));
#135857=CARTESIAN_POINT('Ctrl Pts',(-23.7144895325829,-67.2023409665867,
-176.987246583524));
#135858=CARTESIAN_POINT('Ctrl Pts',(-23.6945043498585,-66.4589699067553,
-176.898771091495));
#135859=CARTESIAN_POINT('Ctrl Pts',(-23.0321233068433,-66.742723669979,
-177.12454316851));
#135860=CARTESIAN_POINT('Ctrl Pts',(-23.7,-67.2147119253083,-176.919839157335));
#135861=CARTESIAN_POINT('Ctrl Pts',(-23.6999999982817,-66.4570693060762,
-176.874118380146));
#135862=CARTESIAN_POINT('Ctrl Pts',(-23.0033898412675,-66.7549897905191,
-176.989728313577));
#135863=CARTESIAN_POINT('Ctrl Pts',(-23.7,-67.2147119299503,-176.84995));
#135864=CARTESIAN_POINT('Ctrl Pts',(-23.6999999999999,-66.45706930551,-176.84995));
#135865=CARTESIAN_POINT('Ctrl Pts',(-23.0033898305084,-66.7549897951205,
-176.84995));
#135866=CARTESIAN_POINT('',(-23.0033898305085,-66.7549897951205,-176.84995));
#135867=CARTESIAN_POINT('',(-23.7,-67.2147119299503,-176.84995));
#135868=CARTESIAN_POINT('Origin',(-23.2,-67.2147119299503,-176.84995));
#135869=CARTESIAN_POINT('',(-24.2,-66.7760495265873,-177.34995));
#135870=CARTESIAN_POINT('Ctrl Pts',(-23.7,-67.2147119299503,-176.84995));
#135871=CARTESIAN_POINT('Ctrl Pts',(-23.7,-67.2147119253083,-176.919839157335));
#135872=CARTESIAN_POINT('Ctrl Pts',(-23.7144895325829,-67.2023409665867,
-176.987246583524));
#135873=CARTESIAN_POINT('Ctrl Pts',(-23.7683864506384,-67.1560455904002,
-177.111255395708));
#135874=CARTESIAN_POINT('Ctrl Pts',(-23.8072189577995,-67.1225998569154,
-177.166241836555));
#135875=CARTESIAN_POINT('Ctrl Pts',(-23.9022748831747,-67.0400066306863,
-177.256984676403));
#135876=CARTESIAN_POINT('Ctrl Pts',(-23.9567084144264,-66.9924080535444,
-177.291402578445));
#135877=CARTESIAN_POINT('Ctrl Pts',(-24.0753687900163,-66.8876168115863,
-177.338353763422));
#135878=CARTESIAN_POINT('Ctrl Pts',(-24.1371859654851,-66.8325498277328,
-177.34995));
#135879=CARTESIAN_POINT('Ctrl Pts',(-24.2,-66.7760495265873,-177.34995));
#135880=CARTESIAN_POINT('',(-23.9949152542395,-66.3200448697526,-177.84995));
#135881=CARTESIAN_POINT('Origin',(-24.200000000006,-66.7760495265862,-177.84995));
#135882=CARTESIAN_POINT('Ctrl Pts',(-23.9949152542395,-66.3200448697526,
-177.84995));
#135883=CARTESIAN_POINT('Ctrl Pts',(-23.9428551887952,-66.3434585018855,
-177.849949993716));
#135884=CARTESIAN_POINT('Ctrl Pts',(-23.8912891629459,-66.3665571088585,
-177.845903065055));
#135885=CARTESIAN_POINT('Ctrl Pts',(-23.8403424606444,-66.3892926538626,
-177.83781160242));
#135886=CARTESIAN_POINT('Ctrl Pts',(-23.7898936124076,-66.4118060258313,
-177.829799210017));
#135887=CARTESIAN_POINT('Ctrl Pts',(-23.7400516011853,-66.4339635775754,
-177.817820923568));
#135888=CARTESIAN_POINT('Ctrl Pts',(-23.6909420374961,-66.4557157061562,
-177.80182839125));
#135889=CARTESIAN_POINT('Ctrl Pts',(-23.6705352998627,-66.4647544747293,
-177.795182935934));
#135890=CARTESIAN_POINT('Ctrl Pts',(-23.6502551185152,-66.4737231883063,
-177.787843738039));
#135891=CARTESIAN_POINT('Ctrl Pts',(-23.6301109846052,-66.4826180228466,
-177.779804722709));
#135892=CARTESIAN_POINT('Ctrl Pts',(-23.6296825902114,-66.4828071844789,
-177.779633761321));
#135893=CARTESIAN_POINT('Ctrl Pts',(-23.6292543206867,-66.4829962847601,
-177.77946250822));
#135894=CARTESIAN_POINT('Ctrl Pts',(-23.6288261761769,-66.4831853236383,
-177.779290963367));
#135895=CARTESIAN_POINT('Ctrl Pts',(-23.5490836050341,-66.5183941044508,
-177.747340471671));
#135896=CARTESIAN_POINT('Ctrl Pts',(-23.4738664381495,-66.551389542848,
-177.705344056616));
#135897=CARTESIAN_POINT('Ctrl Pts',(-23.4044230513275,-66.5817044398146,
-177.653364341176));
#135898=CARTESIAN_POINT('Ctrl Pts',(-23.3717123604324,-66.5959840029173,
-177.628879757656));
#135899=CARTESIAN_POINT('Ctrl Pts',(-23.3402823397949,-66.6096689890227,
-177.60218062654));
#135900=CARTESIAN_POINT('Ctrl Pts',(-23.3102608826734,-66.6227116735265,
-177.57327646271));
#135901=CARTESIAN_POINT('Ctrl Pts',(-23.3097552045839,-66.6229313630558,
-177.572789604185));
#135902=CARTESIAN_POINT('Ctrl Pts',(-23.3092500282568,-66.6231508261632,
-177.572302197161));
#135903=CARTESIAN_POINT('Ctrl Pts',(-23.3087453546535,-66.6233700624813,
-177.571814242488));
#135904=CARTESIAN_POINT('Ctrl Pts',(-23.2428791470164,-66.6519831398301,
-177.508130064148));
#135905=CARTESIAN_POINT('Ctrl Pts',(-23.1855484931334,-66.6767452815916,
-177.435089847605));
#135906=CARTESIAN_POINT('Ctrl Pts',(-23.1388722340375,-66.6968462861646,
-177.354542469169));
#135907=CARTESIAN_POINT('Ctrl Pts',(-23.1191486795941,-66.7053401814712,
-177.320506309575));
#135908=CARTESIAN_POINT('Ctrl Pts',(-23.1013269939373,-66.7130020216597,
-177.285129627946));
#135909=CARTESIAN_POINT('Ctrl Pts',(-23.0855644128598,-66.7197717463454,
-177.248551496375));
#135910=CARTESIAN_POINT('Ctrl Pts',(-23.0853517691174,-66.7198630727333,
-177.248058042242));
#135911=CARTESIAN_POINT('Ctrl Pts',(-23.0851395181392,-66.7199542292592,
-177.24756442059));
#135912=CARTESIAN_POINT('Ctrl Pts',(-23.0849276601638,-66.7200452158304,
-177.247070631801));
#135913=CARTESIAN_POINT('Ctrl Pts',(-23.0685067964826,-66.7270974784524,
-177.208797640755));
#135914=CARTESIAN_POINT('Ctrl Pts',(-23.0544044796131,-66.7331469401741,
-177.169412579499));
#135915=CARTESIAN_POINT('Ctrl Pts',(-23.04278734195,-66.738126397354,-177.129172865924));
#135916=CARTESIAN_POINT('Ctrl Pts',(-23.0313107069198,-66.7430456308484,
-177.089419828659));
#135917=CARTESIAN_POINT('Ctrl Pts',(-23.0222597634207,-66.7469204858851,
-177.048833228894));
#135918=CARTESIAN_POINT('Ctrl Pts',(-23.0157509005018,-66.7497052241092,
-177.007676413083));
#135919=CARTESIAN_POINT('Ctrl Pts',(-23.0093646056921,-66.7524375230512,
-176.967294619447));
#135920=CARTESIAN_POINT('Ctrl Pts',(-23.0054256948344,-66.7541203250939,
-176.926364378223));
#135921=CARTESIAN_POINT('Ctrl Pts',(-23.0039983429947,-66.7547299427615,
-176.885141466357));
#135922=CARTESIAN_POINT('Ctrl Pts',(-23.0035929213886,-66.7549030971072,
-176.873432608966));
#135923=CARTESIAN_POINT('Ctrl Pts',(-23.0033898314129,-66.7549897947337,
-176.861700158873));
#135924=CARTESIAN_POINT('Ctrl Pts',(-23.0033898305084,-66.7549897951205,
-176.84995));
#135925=CARTESIAN_POINT('Origin',(-23.2,-67.2147119299503,-179.64995));
#135926=CARTESIAN_POINT('',(-23.0033898305084,-66.7549897951204,-171.871644662643));
#135927=CARTESIAN_POINT('',(-23.0033898305085,-66.7549897951205,-179.64995));
#135928=CARTESIAN_POINT('',(-23.7,-67.2147119299503,-171.871644662643));
#135929=CARTESIAN_POINT('Origin',(-23.2,-67.2147119299503,-171.871644662643));
#135930=CARTESIAN_POINT('',(-23.7,-67.2147119299503,-176.84995));
#135931=CARTESIAN_POINT('Origin',(0.,-12.9675000200281,-171.871644662643));
#135932=CARTESIAN_POINT('',(-17.4012711864406,-68.8194987407181,-171.871644662643));
#135933=CARTESIAN_POINT('Origin',(0.,-12.9675000200281,-171.871644662643));
#135934=CARTESIAN_POINT('',(-17.4148840712406,-68.7171063154928,-171.449026400902));
#135935=CARTESIAN_POINT('Origin',(-17.5530339837215,-67.6883802890115,-171.880603003797));
#135936=CARTESIAN_POINT('',(-23.0213852109847,-66.6453596297547,-171.449026400902));
#135937=CARTESIAN_POINT('Origin',(0.,-12.9675000200281,-171.449026400902));
#135938=CARTESIAN_POINT('Origin',(-23.2064336390783,-65.5202502275577,-171.885329893835));
#135939=CARTESIAN_POINT('Origin',(-17.55,-69.2968662511513,-179.64995));
#135940=CARTESIAN_POINT('',(-17.05,-69.2968662511513,-176.84995));
#135941=CARTESIAN_POINT('',(-17.4012711864406,-68.8194987407181,-176.84995));
#135942=CARTESIAN_POINT('Origin',(-17.55,-69.2968662511513,-176.84995));
#135943=CARTESIAN_POINT('',(-17.05,-69.2968662511513,-171.871644662643));
#135944=CARTESIAN_POINT('',(-17.05,-69.2968662511513,-171.871644662643));
#135945=CARTESIAN_POINT('Origin',(-17.55,-69.2968662511513,-171.871644662643));
#135946=CARTESIAN_POINT('',(-17.4012711864406,-68.8194987407181,-179.64995));
#135947=CARTESIAN_POINT('Ctrl Pts',(-17.0492479950133,-69.297368111594,
-176.822948722429));
#135948=CARTESIAN_POINT('Ctrl Pts',(-17.0488576004114,-68.9292870000689,
-176.816737185091));
#135949=CARTESIAN_POINT('Ctrl Pts',(-17.3997798690686,-68.8199646773016,
-176.79594636526));
#135950=CARTESIAN_POINT('Ctrl Pts',(-17.053474034057,-69.2947264864225,
-176.89849934037));
#135951=CARTESIAN_POINT('Ctrl Pts',(-17.0551529338767,-68.9273807085645,
-176.909574260456));
#135952=CARTESIAN_POINT('Ctrl Pts',(-17.4081606356245,-68.8173454677221,
-176.947050609194));
#135953=CARTESIAN_POINT('Ctrl Pts',(-17.0398006752804,-69.3032834461013,
-176.975516985737));
#135954=CARTESIAN_POINT('Ctrl Pts',(-17.0345718967367,-68.933617729428,
-177.005206223573));
#135955=CARTESIAN_POINT('Ctrl Pts',(-17.3810445025101,-68.8258298172436,
-177.101089109421));
#135956=CARTESIAN_POINT('Ctrl Pts',(-16.984573721817,-69.3375281363239,
-177.105974674662));
#135957=CARTESIAN_POINT('Ctrl Pts',(-16.9553753472294,-68.9574616796934,
-177.159342510638));
#135958=CARTESIAN_POINT('Ctrl Pts',(-17.271522613636,-68.8597838444499,
-177.362008470827));
#135959=CARTESIAN_POINT('Ctrl Pts',(-16.9464194670572,-69.3611108992158,
-177.16153439432));
#135960=CARTESIAN_POINT('Ctrl Pts',(-16.9006584936516,-68.9738907873115,
-177.221947407359));
#135961=CARTESIAN_POINT('Ctrl Pts',(-17.1958580434816,-68.8831664553272,
-177.473129011102));
#135962=CARTESIAN_POINT('Ctrl Pts',(-16.8534774852002,-69.4179436363549,
-177.252609444331));
#135963=CARTESIAN_POINT('Ctrl Pts',(-16.7738840954457,-69.0116922167351,
-177.31458111062));
#135964=CARTESIAN_POINT('Ctrl Pts',(-17.0115440055365,-68.9395167543114,
-177.65527913718));
#135965=CARTESIAN_POINT('Ctrl Pts',(-16.7979218519985,-69.4516483772983,
-177.28887581796));
#135966=CARTESIAN_POINT('Ctrl Pts',(-16.7000151738869,-69.0335912458224,
-177.345046470341));
#135967=CARTESIAN_POINT('Ctrl Pts',(-16.901371584146,-68.9729353808306,
-177.727810792065));
#135968=CARTESIAN_POINT('Ctrl Pts',(-16.6709738473584,-69.5276893376271,
-177.340535368617));
#135969=CARTESIAN_POINT('Ctrl Pts',(-16.5421185639685,-69.0801133097091,
-177.373722750586));
#135970=CARTESIAN_POINT('Ctrl Pts',(-16.6496229232295,-69.0483307385377,
-177.831125967842));
#135971=CARTESIAN_POINT('Ctrl Pts',(-16.5966263844035,-69.5716604942096,
-177.353161582598));
#135972=CARTESIAN_POINT('Ctrl Pts',(-16.4557762619242,-69.1053726143953,
-177.36608299368));
#135973=CARTESIAN_POINT('Ctrl Pts',(-16.5021951424801,-69.091926058946,
-177.856375144043));
#135974=CARTESIAN_POINT('Ctrl Pts',(-16.5240599846146,-69.6139181916527,
-177.349254788131));
#135975=CARTESIAN_POINT('Ctrl Pts',(-16.3826215477911,-69.1267402936733,
-177.341852229526));
#135976=CARTESIAN_POINT('Ctrl Pts',(-16.3582807548912,-69.1338282608016,
-177.848558467037));
#135977=CARTESIAN_POINT('',(-16.55,-69.5987413979107,-177.34995));
#135978=CARTESIAN_POINT('',(-16.4097457627119,-69.1188156235219,-177.84995));
#135979=CARTESIAN_POINT('Origin',(-16.55,-69.5987413979107,-177.84995));
#135980=CARTESIAN_POINT('Ctrl Pts',(-16.55,-69.5987413979107,-177.34995));
#135981=CARTESIAN_POINT('Ctrl Pts',(-16.571974857016,-69.5858974666297,
-177.34995));
#135982=CARTESIAN_POINT('Ctrl Pts',(-16.5940231568532,-69.5729545882568,
-177.348496976456));
#135983=CARTESIAN_POINT('Ctrl Pts',(-16.6159015410091,-69.5600570385675,
-177.345587959495));
#135984=CARTESIAN_POINT('Ctrl Pts',(-16.637789232771,-69.5471540019415,
-177.342677704967));
#135985=CARTESIAN_POINT('Ctrl Pts',(-16.6595060527741,-69.5342963325752,
-177.338310277277));
#135986=CARTESIAN_POINT('Ctrl Pts',(-16.6808128321261,-69.521628490458,
-177.332534710648));
#135987=CARTESIAN_POINT('Ctrl Pts',(-16.7004320836829,-69.5099639597905,
-177.327216577264));
#135988=CARTESIAN_POINT('Ctrl Pts',(-16.7197032679559,-69.4984603779473,
-177.320705253509));
#135989=CARTESIAN_POINT('Ctrl Pts',(-16.7384517689056,-69.4872305273618,
-177.313076257943));
#135990=CARTESIAN_POINT('Ctrl Pts',(-16.7592707344465,-69.4747605238669,
-177.304604764877));
#135991=CARTESIAN_POINT('Ctrl Pts',(-16.7796238303514,-69.4625248975477,
-177.294681953488));
#135992=CARTESIAN_POINT('Ctrl Pts',(-16.7992696834622,-69.4506685598544,
-177.283383529975));
#135993=CARTESIAN_POINT('Ctrl Pts',(-16.8188916910297,-69.4388266130258,
-177.272098820148));
#135994=CARTESIAN_POINT('Ctrl Pts',(-16.8378074309329,-69.4273630346438,
-177.259442107775));
#135995=CARTESIAN_POINT('Ctrl Pts',(-16.8557951920564,-69.4164222091315,
-177.245537285583));
#135996=CARTESIAN_POINT('Ctrl Pts',(-16.8712360041473,-69.4070305327747,
-177.233601295042));
#135997=CARTESIAN_POINT('Ctrl Pts',(-16.8859930975071,-69.3980240530471,
-177.22074657705));
#135998=CARTESIAN_POINT('Ctrl Pts',(-16.8999432516754,-69.389494096997,
-177.207077037071));
#135999=CARTESIAN_POINT('Ctrl Pts',(-16.91634277459,-69.3794664508494,-177.191007398598));
#136000=CARTESIAN_POINT('Ctrl Pts',(-16.9317275329241,-69.3700407193404,
-177.17371192959));
#136001=CARTESIAN_POINT('Ctrl Pts',(-16.9458910222967,-69.3613359641857,
-177.155351863886));
#136002=CARTESIAN_POINT('Ctrl Pts',(-16.9600211165384,-69.3526517333829,
-177.137035088135));
#136003=CARTESIAN_POINT('Ctrl Pts',(-16.9729351002459,-69.3446850830602,
-177.117659209345));
#136004=CARTESIAN_POINT('Ctrl Pts',(-16.9844613282345,-69.3375542347348,
-177.097423946646));
#136005=CARTESIAN_POINT('Ctrl Pts',(-16.9941214124636,-69.3315779001078,
-177.080464856278));
#136006=CARTESIAN_POINT('Ctrl Pts',(-17.0028071808333,-69.3261886367402,
-177.062903012023));
#136007=CARTESIAN_POINT('Ctrl Pts',(-17.0104398994491,-69.32145603957,-177.044873315679));
#136008=CARTESIAN_POINT('Ctrl Pts',(-17.0192225481519,-69.3160104387965,
-177.024127301425));
#136009=CARTESIAN_POINT('Ctrl Pts',(-17.0266333838746,-69.3114281239145,
-177.002705007449));
#136010=CARTESIAN_POINT('Ctrl Pts',(-17.0325650959538,-69.3077506027218,
-176.980835171685));
#136011=CARTESIAN_POINT('Ctrl Pts',(-17.0384951751614,-69.3040740938709,
-176.958971356213));
#136012=CARTESIAN_POINT('Ctrl Pts',(-17.0429466552163,-69.3013018806378,
-176.936660984636));
#136013=CARTESIAN_POINT('Ctrl Pts',(-17.0458611190542,-69.2994754365511,
-176.914150861446));
#136014=CARTESIAN_POINT('Ctrl Pts',(-17.0486180997703,-69.2977476844135,
-176.892857073289));
#136015=CARTESIAN_POINT('Ctrl Pts',(-17.05,-69.2968662535477,-176.871385242631));
#136016=CARTESIAN_POINT('Ctrl Pts',(-17.05,-69.2968662511513,-176.84995));
#136017=CARTESIAN_POINT('Ctrl Pts',(-17.4012711864406,-68.8194987407181,
-176.84995));
#136018=CARTESIAN_POINT('Ctrl Pts',(-17.4012711797275,-68.8194987428096,
-176.887694684675));
#136019=CARTESIAN_POINT('Ctrl Pts',(-17.3991058038741,-68.8201748588276,
-176.925251096234));
#136020=CARTESIAN_POINT('Ctrl Pts',(-17.3948976591097,-68.8214863041692,
-176.962447012708));
#136021=CARTESIAN_POINT('Ctrl Pts',(-17.3906053585138,-68.8228239762163,
-177.000386785074));
#136022=CARTESIAN_POINT('Ctrl Pts',(-17.3841876175728,-68.8248226995135,
-177.037952567699));
#136023=CARTESIAN_POINT('Ctrl Pts',(-17.3757224555706,-68.8274555088436,
-177.074968429999));
#136024=CARTESIAN_POINT('Ctrl Pts',(-17.3672590966796,-68.8300877573754,
-177.11197640778));
#136025=CARTESIAN_POINT('Ctrl Pts',(-17.356748909814,-68.8333539190401,
-177.148435801525));
#136026=CARTESIAN_POINT('Ctrl Pts',(-17.3442218215212,-68.837241948804,
-177.184161144092));
#136027=CARTESIAN_POINT('Ctrl Pts',(-17.3378147381211,-68.839230513934,
-177.202433167405));
#136028=CARTESIAN_POINT('Ctrl Pts',(-17.3308793073379,-68.8413819840089,
-177.22051291325));
#136029=CARTESIAN_POINT('Ctrl Pts',(-17.3234150119905,-68.84369613616,-177.238373157981));
#136030=CARTESIAN_POINT('Ctrl Pts',(-17.323216781765,-68.8437575933882,
-177.238847474735));
#136031=CARTESIAN_POINT('Ctrl Pts',(-17.3230181873272,-68.8438191626283,
-177.239321615502));
#136032=CARTESIAN_POINT('Ctrl Pts',(-17.3228192288394,-68.8438808438229,
-177.23979557955));
#136033=CARTESIAN_POINT('Ctrl Pts',(-17.2882744024226,-68.8545904455368,
-177.322089157366));
#136034=CARTESIAN_POINT('Ctrl Pts',(-17.24265513348,-68.868699441709,-177.399426405929));
#136035=CARTESIAN_POINT('Ctrl Pts',(-17.1883023464399,-68.8854065190392,
-177.469044916629));
#136036=CARTESIAN_POINT('Ctrl Pts',(-17.1624825557968,-68.8933430621755,
-177.502116548628));
#136037=CARTESIAN_POINT('Ctrl Pts',(-17.1346920798658,-68.9018658361705,
-177.533445664935));
#136038=CARTESIAN_POINT('Ctrl Pts',(-17.1051831298931,-68.9108884594799,
-177.562732114831));
#136039=CARTESIAN_POINT('Ctrl Pts',(-17.104688915706,-68.9110395698531,
-177.5632226026));
#136040=CARTESIAN_POINT('Ctrl Pts',(-17.1041942190907,-68.9111908205538,
-177.563712518466));
#136041=CARTESIAN_POINT('Ctrl Pts',(-17.1036990412529,-68.9113422111695,
-177.564201860987));
#136042=CARTESIAN_POINT('Ctrl Pts',(-17.0462278720989,-68.9289128595717,
-177.620995773434));
#136043=CARTESIAN_POINT('Ctrl Pts',(-16.9816775189031,-68.9485450280228,
-177.67064989156));
#136044=CARTESIAN_POINT('Ctrl Pts',(-16.9125398584879,-68.9694257059549,
-177.711729306558));
#136045=CARTESIAN_POINT('Ctrl Pts',(-16.8713991530587,-68.9818508562248,
-177.736173814827));
#136046=CARTESIAN_POINT('Ctrl Pts',(-16.8286352683543,-68.9947177370478,
-177.7575822379));
#136047=CARTESIAN_POINT('Ctrl Pts',(-16.7847809634131,-69.007852694924,
-177.775654990622));
#136048=CARTESIAN_POINT('Ctrl Pts',(-16.78433889104,-69.007985101583,-177.775837172615));
#136049=CARTESIAN_POINT('Ctrl Pts',(-16.7838967203631,-69.008117531739,
-177.776019010763));
#136050=CARTESIAN_POINT('Ctrl Pts',(-16.7834544517973,-69.0082499852542,
-177.776200504879));
#136051=CARTESIAN_POINT('Ctrl Pts',(-16.7449698092192,-69.0197756205532,
-177.791993479437));
#136052=CARTESIAN_POINT('Ctrl Pts',(-16.7054466746896,-69.031566259125,
-177.805303057386));
#136053=CARTESIAN_POINT('Ctrl Pts',(-16.6651986963189,-69.0435261398609,
-177.816095296664));
#136054=CARTESIAN_POINT('Ctrl Pts',(-16.6237252999666,-69.0558501594555,
-177.827216123976));
#136055=CARTESIAN_POINT('Ctrl Pts',(-16.5814808439819,-69.0683543171784,
-177.835664557351));
#136056=CARTESIAN_POINT('Ctrl Pts',(-16.5387947985049,-69.0809368867564,
-177.841347934728));
#136057=CARTESIAN_POINT('Ctrl Pts',(-16.4988275773255,-69.0927180282444,
-177.84666931782));
#136058=CARTESIAN_POINT('Ctrl Pts',(-16.4584720658829,-69.1045682551434,
-177.849566394706));
#136059=CARTESIAN_POINT('Ctrl Pts',(-16.4180055598672,-69.1164010707452,
-177.849914459328));
#136060=CARTESIAN_POINT('Ctrl Pts',(-16.415252771043,-69.1172060140367,
-177.849938136895));
#136061=CARTESIAN_POINT('Ctrl Pts',(-16.41249947515,-69.1180108744163,-177.849949999677));
#136062=CARTESIAN_POINT('Ctrl Pts',(-16.4097457627119,-69.1188156235219,
-177.84995));
#136063=CARTESIAN_POINT('Origin',(0.,-12.9675000200281,-177.84995));
#136064=CARTESIAN_POINT('',(-16.05,-69.7424724991055,-177.34995));
#136065=CARTESIAN_POINT('',(-15.9139830508475,-69.2613286645371,-177.84995));
#136066=CARTESIAN_POINT('Origin',(-16.0500000000002,-69.7424724991055,-177.84995));
#136067=CARTESIAN_POINT('Origin',(0.,-12.9675000200281,-177.34995));
#136068=CARTESIAN_POINT('Origin',(0.,-12.9675000200281,-177.84995));
#136069=CARTESIAN_POINT('Ctrl Pts',(-16.05,-69.7424724991056,-177.34995));
#136070=CARTESIAN_POINT('Ctrl Pts',(-15.9139830508475,-69.2613286645371,
-177.34995));
#136071=CARTESIAN_POINT('Ctrl Pts',(-15.9139830508475,-69.2613286645371,
-177.84995));
#136072=CARTESIAN_POINT('Ctrl Pts',(-15.9218377669144,-69.8149341395249,
-177.34995));
#136073=CARTESIAN_POINT('Ctrl Pts',(-15.7715232212968,-69.3016013426613,
-177.313287744377));
#136074=CARTESIAN_POINT('Ctrl Pts',(-15.6598936117711,-69.3331584747352,
-177.849949962799));
#136075=CARTESIAN_POINT('Ctrl Pts',(-15.7932661099729,-69.8854545791845,
-177.298481825532));
#136076=CARTESIAN_POINT('Ctrl Pts',(-15.6726841471448,-69.3295726985644,
-177.220678605763));
#136077=CARTESIAN_POINT('Ctrl Pts',(-15.4048666982144,-69.4030990332408,
-177.747013645666));
#136078=CARTESIAN_POINT('Ctrl Pts',(-15.6065726131672,-69.9860620159006,
-177.115402898665));
#136079=CARTESIAN_POINT('Ctrl Pts',(-15.5618471106836,-69.3622450871995,
-177.028739897256));
#136080=CARTESIAN_POINT('Ctrl Pts',(-15.0346439900464,-69.5028538622254,
-177.380855802727));
#136081=CARTESIAN_POINT('Ctrl Pts',(-15.55,-70.0157033150841,-176.985144891356));
#136082=CARTESIAN_POINT('Ctrl Pts',(-15.5500000039846,-69.3666907690031,
-176.935931672441));
#136083=CARTESIAN_POINT('Ctrl Pts',(-14.922457653694,-69.5322439651191,
-177.120339778533));
#136084=CARTESIAN_POINT('Ctrl Pts',(-15.55,-70.015703322148,-176.84995));
#136085=CARTESIAN_POINT('Ctrl Pts',(-15.5499999999999,-69.3666907703604,
-176.84995));
#136086=CARTESIAN_POINT('Ctrl Pts',(-14.9224576271186,-69.53224397213,-176.84995));
#136087=CARTESIAN_POINT('',(-14.9224576271186,-69.53224397213,-176.84995));
#136088=CARTESIAN_POINT('Ctrl Pts',(-15.9139830508475,-69.2613286645371,
-177.84995));
#136089=CARTESIAN_POINT('Ctrl Pts',(-15.6598936117711,-69.3331584747352,
-177.849949962799));
#136090=CARTESIAN_POINT('Ctrl Pts',(-15.4048666982144,-69.4030990332408,
-177.747013645666));
#136091=CARTESIAN_POINT('Ctrl Pts',(-15.0346439900464,-69.5028538622254,
-177.380855802727));
#136092=CARTESIAN_POINT('Ctrl Pts',(-14.922457653694,-69.5322439651191,
-177.120339778533));
#136093=CARTESIAN_POINT('Ctrl Pts',(-14.9224576271186,-69.53224397213,-176.84995));
#136094=CARTESIAN_POINT('',(-15.55,-70.015703322148,-176.84995));
#136095=CARTESIAN_POINT('Origin',(-15.05,-70.015703322148,-176.84995));
#136096=CARTESIAN_POINT('Ctrl Pts',(-15.55,-70.015703322148,-176.84995));
#136097=CARTESIAN_POINT('Ctrl Pts',(-15.55,-70.0157033150841,-176.985144891356));
#136098=CARTESIAN_POINT('Ctrl Pts',(-15.6065726131672,-69.9860620159006,
-177.115402898665));
#136099=CARTESIAN_POINT('Ctrl Pts',(-15.7932661099729,-69.8854545791845,
-177.298481825532));
#136100=CARTESIAN_POINT('Ctrl Pts',(-15.9218377669144,-69.8149341395249,
-177.34995));
#136101=CARTESIAN_POINT('Ctrl Pts',(-16.05,-69.7424724991055,-177.34995));
#136102=CARTESIAN_POINT('Origin',(-15.05,-70.015703322148,-179.64995));
#136103=CARTESIAN_POINT('',(-14.9224576271186,-69.5322439721301,-171.871644662643));
#136104=CARTESIAN_POINT('',(-14.9224576271186,-69.5322439721301,-179.64995));
#136105=CARTESIAN_POINT('',(-15.55,-70.015703322148,-171.871644662643));
#136106=CARTESIAN_POINT('Origin',(-15.05,-70.015703322148,-171.871644662643));
#136107=CARTESIAN_POINT('',(-15.55,-70.015703322148,-176.84995));
#136108=CARTESIAN_POINT('Origin',(0.,-12.9675000200281,-171.871644662643));
#136109=CARTESIAN_POINT('',(-9.32033898305081,-70.7202599648223,-171.871644662643));
#136110=CARTESIAN_POINT('Origin',(0.,-12.9675000200281,-171.871644662643));
#136111=CARTESIAN_POINT('',(-9.3276302147955,-70.6241744288951,-171.449026400902));
#136112=CARTESIAN_POINT('Origin',(-9.40047870352405,-69.677975233741,-171.875589094873));
#136113=CARTESIAN_POINT('',(-14.9341313545396,-69.4322546019744,-171.449026400902));
#136114=CARTESIAN_POINT('Origin',(0.,-12.9675000200281,-171.449026400902));
#136115=CARTESIAN_POINT('Origin',(-15.0818193009629,-68.1701112854949,-171.933582810381));
#136116=CARTESIAN_POINT('Origin',(-9.4,-71.2138732976838,-179.64995));
#136117=CARTESIAN_POINT('',(-8.89999998637947,-71.2138732976795,-176.681036188732));
#136118=CARTESIAN_POINT('',(-9.32033898305081,-70.7202599648223,-176.681036188741));
#136119=CARTESIAN_POINT('Origin',(-9.4,-71.2138732976838,-176.681036188741));
#136120=CARTESIAN_POINT('',(-8.9,-71.2138732976838,-171.871644662643));
#136121=CARTESIAN_POINT('',(-8.9,-71.2138732976838,-171.871644662643));
#136122=CARTESIAN_POINT('Origin',(-9.4,-71.2138732976838,-171.871644662643));
#136123=CARTESIAN_POINT('',(-9.32033898305081,-70.7202599648223,-179.64995));
#136124=CARTESIAN_POINT('Ctrl Pts',(-8.9,-71.2138732976838,-176.681036188741));
#136125=CARTESIAN_POINT('Ctrl Pts',(-8.89999999999995,-70.7880957152449,
-176.681036188741));
#136126=CARTESIAN_POINT('Ctrl Pts',(-9.32033898305081,-70.7202599648223,
-176.681036188741));
#136127=CARTESIAN_POINT('Ctrl Pts',(-8.9,-71.1871171480823,-176.760825627325));
#136128=CARTESIAN_POINT('Ctrl Pts',(-8.92228717603221,-70.7844989338608,
-176.766146975383));
#136129=CARTESIAN_POINT('Ctrl Pts',(-9.32033898600605,-70.7202599643454,
-176.813381110627));
#136130=CARTESIAN_POINT('Ctrl Pts',(-8.88962568872291,-71.1669786363603,
-176.836281093745));
#136131=CARTESIAN_POINT('Ctrl Pts',(-8.92671149441355,-70.7836436470507,
-176.856038553599));
#136132=CARTESIAN_POINT('Ctrl Pts',(-9.29976619260072,-70.7235936461789,
-176.944341025131));
#136133=CARTESIAN_POINT('Ctrl Pts',(-8.84506581279844,-71.1392355158483,
-176.976329963003));
#136134=CARTESIAN_POINT('Ctrl Pts',(-8.89496802003281,-70.7881886691942,
-177.027264022804));
#136135=CARTESIAN_POINT('Ctrl Pts',(-9.21140170024677,-70.7377525805495,
-177.193900303459));
#136136=CARTESIAN_POINT('Ctrl Pts',(-8.81169873029936,-71.1320753660863,
-177.038360991276));
#136137=CARTESIAN_POINT('Ctrl Pts',(-8.86020506502259,-70.7933743404483,
-177.1069029419));
#136138=CARTESIAN_POINT('Ctrl Pts',(-9.14523307029305,-70.748315066844,
-177.307880650604));
#136139=CARTESIAN_POINT('Ctrl Pts',(-8.67906488297454,-71.1273471571499,
-177.195002198461));
#136140=CARTESIAN_POINT('Ctrl Pts',(-8.70620726441098,-70.816353148992,
-177.306646407394));
#136141=CARTESIAN_POINT('Ctrl Pts',(-8.88221342209322,-70.789535493208,
-177.600825160592));
#136142=CARTESIAN_POINT('Ctrl Pts',(-8.55095696965989,-71.1465765189117,
-177.251701888337));
#136143=CARTESIAN_POINT('Ctrl Pts',(-8.53744099317464,-70.8414090832674,
-177.381970537377));
#136144=CARTESIAN_POINT('Ctrl Pts',(-8.62826388004552,-70.8283148356172,
-177.714106286858));
#136145=CARTESIAN_POINT('Ctrl Pts',(-8.41817827172749,-71.1781985203564,
-177.244444626905));
#136146=CARTESIAN_POINT('Ctrl Pts',(-8.37078242155037,-70.8655141261624,
-177.369392503913));
#136147=CARTESIAN_POINT('Ctrl Pts',(-8.36486199647655,-70.8663694716841,
-177.709383806606));
#136148=CARTESIAN_POINT('',(-8.41817827230434,-71.1781985202609,-177.244444626919));
#136149=CARTESIAN_POINT('',(-8.36486199647649,-70.8663694716841,-177.709383806605));
#136150=CARTESIAN_POINT('Origin',(-8.43635654345535,-71.3612316037495,-177.709383806605));
#136151=CARTESIAN_POINT('Ctrl Pts',(-8.4181782717274,-71.1781985203566,
-177.244444626904));
#136152=CARTESIAN_POINT('Ctrl Pts',(-8.55095696965989,-71.1465765189117,
-177.251701888337));
#136153=CARTESIAN_POINT('Ctrl Pts',(-8.67906488297454,-71.1273471571499,
-177.195002198461));
#136154=CARTESIAN_POINT('Ctrl Pts',(-8.81169873029936,-71.1320753660863,
-177.038360991276));
#136155=CARTESIAN_POINT('Ctrl Pts',(-8.84506581279844,-71.1392355158483,
-176.976329963003));
#136156=CARTESIAN_POINT('Ctrl Pts',(-8.88962568872291,-71.1669786363603,
-176.836281093745));
#136157=CARTESIAN_POINT('Ctrl Pts',(-8.9,-71.1871171480823,-176.760825627325));
#136158=CARTESIAN_POINT('Ctrl Pts',(-8.9,-71.2138732976838,-176.681036188741));
#136159=CARTESIAN_POINT('Ctrl Pts',(-9.32033898305081,-70.7202599648223,
-176.681036188741));
#136160=CARTESIAN_POINT('Ctrl Pts',(-9.32033898600605,-70.7202599643454,
-176.813381110627));
#136161=CARTESIAN_POINT('Ctrl Pts',(-9.29976619260072,-70.7235936461789,
-176.944341025131));
#136162=CARTESIAN_POINT('Ctrl Pts',(-9.21140170024677,-70.7377525805495,
-177.193900303459));
#136163=CARTESIAN_POINT('Ctrl Pts',(-9.14523307029305,-70.748315066844,
-177.307880650604));
#136164=CARTESIAN_POINT('Ctrl Pts',(-8.88221342209322,-70.789535493208,
-177.600825160592));
#136165=CARTESIAN_POINT('Ctrl Pts',(-8.62826388004552,-70.8283148356172,
-177.714106286858));
#136166=CARTESIAN_POINT('Ctrl Pts',(-8.36486199647649,-70.8663694716841,
-177.709383806605));
#136167=CARTESIAN_POINT('Ctrl Pts',(-7.86991817520098,-70.935718794764,
-177.700825662763));
#136168=CARTESIAN_POINT('Ctrl Pts',(-7.87530650495358,-70.9349872609141,
-177.368681451894));
#136169=CARTESIAN_POINT('Ctrl Pts',(-7.91859121655416,-71.2381488509313,
-177.239961484006));
#136170=CARTESIAN_POINT('Ctrl Pts',(-8.03499989482399,-70.9133068653807,
-177.703576433696));
#136171=CARTESIAN_POINT('Ctrl Pts',(-8.04094447940713,-70.9124841487064,
-177.368907517599));
#136172=CARTESIAN_POINT('Ctrl Pts',(-8.08517348178868,-71.21877443556,-177.241356202481));
#136173=CARTESIAN_POINT('Ctrl Pts',(-8.19998119128136,-70.8901904062617,
-177.706427680957));
#136174=CARTESIAN_POINT('Ctrl Pts',(-8.20613182703653,-70.889318969813,
-177.369144269326));
#136175=CARTESIAN_POINT('Ctrl Pts',(-8.25170137526425,-71.1987909763519,
-177.242846915875));
#136176=CARTESIAN_POINT('Ctrl Pts',(-8.36486199647703,-70.866369471684,
-177.709383806605));
#136177=CARTESIAN_POINT('Ctrl Pts',(-8.3707824215504,-70.8655141261623,
-177.369392503912));
#136178=CARTESIAN_POINT('Ctrl Pts',(-8.41817827172741,-71.1781985203567,
-177.244444626904));
#136179=CARTESIAN_POINT('',(-7.91859121655529,-71.238148850898,-177.239961484019));
#136180=CARTESIAN_POINT('',(-7.86991817520075,-70.935718794764,-177.700825662763));
#136181=CARTESIAN_POINT('Origin',(-7.93718243310846,-71.4311736560866,-177.700825662763));
#136182=CARTESIAN_POINT('Origin',(-0.0604498207115989,-4.47548892910441,
-188.389030577756));
#136183=CARTESIAN_POINT('Origin',(-0.0230368112449109,-14.1525797482743,
-185.975887614352));
#136184=CARTESIAN_POINT('Ctrl Pts',(-7.91859121655422,-71.2381488509314,
-177.239961484007));
#136185=CARTESIAN_POINT('Ctrl Pts',(-7.87530650495354,-70.9349872609141,
-177.368681451895));
#136186=CARTESIAN_POINT('Ctrl Pts',(-7.86991817520074,-70.935718794764,
-177.700825662764));
#136187=CARTESIAN_POINT('Ctrl Pts',(-7.84535391894273,-71.2544423085659,
-177.236091643156));
#136188=CARTESIAN_POINT('Ctrl Pts',(-7.78148695261579,-70.9477382671599,
-177.362180852783));
#136189=CARTESIAN_POINT('Ctrl Pts',(-7.72465595207765,-70.9554399770617,
-177.698405110518));
#136190=CARTESIAN_POINT('Ctrl Pts',(-7.77193648886645,-71.274739088698,
-177.212399058377));
#136191=CARTESIAN_POINT('Ctrl Pts',(-7.68873678647519,-70.9601668953933,
-177.328725158091));
#136192=CARTESIAN_POINT('Ctrl Pts',(-7.57909439591914,-70.9746058127342,
-177.660005031717));
#136193=CARTESIAN_POINT('Ctrl Pts',(-7.64153051403658,-71.3201342851139,
-177.131947985374));
#136194=CARTESIAN_POINT('Ctrl Pts',(-7.53187921075035,-70.98103712284,-177.221702886533));
#136195=CARTESIAN_POINT('Ctrl Pts',(-7.32049271153216,-71.0078082615326,
-177.524965998388));
#136196=CARTESIAN_POINT('Ctrl Pts',(-7.58359051438092,-71.3455846992379,
-177.074841178091));
#136197=CARTESIAN_POINT('Ctrl Pts',(-7.46634030528468,-70.9896817811965,
-177.14630380948));
#136198=CARTESIAN_POINT('Ctrl Pts',(-7.20559474882705,-71.0221114770482,
-177.427818678983));
#136199=CARTESIAN_POINT('Ctrl Pts',(-7.49125858243999,-71.4004398176271,
-176.937641167035));
#136200=CARTESIAN_POINT('Ctrl Pts',(-7.3754100247025,-71.0018071186815,
-176.974926941462));
#136201=CARTESIAN_POINT('Ctrl Pts',(-7.0224958330043,-71.0445441888331,
-177.19789774704));
#136202=CARTESIAN_POINT('Ctrl Pts',(-7.45636610731683,-71.4300660132009,
-176.85726439743));
#136203=CARTESIAN_POINT('Ctrl Pts',(-7.35016748493995,-71.0052818262832,
-176.876651794266));
#136204=CARTESIAN_POINT('Ctrl Pts',(-6.95330228061017,-71.0528136932555,
-177.064676392973));
#136205=CARTESIAN_POINT('Ctrl Pts',(-7.41072271257901,-71.4935573295699,
-176.680998879949));
#136206=CARTESIAN_POINT('Ctrl Pts',(-7.34226626007839,-71.0069144630253,
-176.677678014477));
#136207=CARTESIAN_POINT('Ctrl Pts',(-6.86278910799687,-71.0635773642165,
-176.782076502575));
#136208=CARTESIAN_POINT('Ctrl Pts',(-7.4,-71.5272255526701,-176.585813210379));
#136209=CARTESIAN_POINT('Ctrl Pts',(-7.36167840976143,-71.0048156182876,
-176.575906600101));
#136210=CARTESIAN_POINT('Ctrl Pts',(-6.8415254209523,-71.06606738545,-176.633819401763));
#136211=CARTESIAN_POINT('Ctrl Pts',(-7.4,-71.5626363369615,-176.485569595297));
#136212=CARTESIAN_POINT('Ctrl Pts',(-7.40000000000002,-71.0003029749946,
-176.485569595297));
#136213=CARTESIAN_POINT('Ctrl Pts',(-6.84152542372878,-71.066067385123,
-176.485569595297));
#136214=CARTESIAN_POINT('',(-6.84152542372878,-71.066067385123,-176.485569595297));
#136215=CARTESIAN_POINT('Ctrl Pts',(-7.86991817520075,-70.935718794764,
-177.700825662763));
#136216=CARTESIAN_POINT('Ctrl Pts',(-7.84145915028904,-70.9395824669992,
-177.700351440663));
#136217=CARTESIAN_POINT('Ctrl Pts',(-7.81325306985418,-70.9433890026599,
-177.698505055736));
#136218=CARTESIAN_POINT('Ctrl Pts',(-7.78529419147434,-70.9471417642783,
-177.695385832037));
#136219=CARTESIAN_POINT('Ctrl Pts',(-7.77696163598821,-70.9482601959259,
-177.694456213038));
#136220=CARTESIAN_POINT('Ctrl Pts',(-7.76865098308068,-70.9493738524319,
-177.693413186647));
#136221=CARTESIAN_POINT('Ctrl Pts',(-7.76036198762536,-70.9504828203398,
-177.692258509338));
#136222=CARTESIAN_POINT('Ctrl Pts',(-7.73171720388245,-70.9543151479204,
-177.688268221013));
#136223=CARTESIAN_POINT('Ctrl Pts',(-7.7033289936209,-70.9580918229642,
-177.682948350417));
#136224=CARTESIAN_POINT('Ctrl Pts',(-7.67518610521715,-70.9618160028387,
-177.676335993945));
#136225=CARTESIAN_POINT('Ctrl Pts',(-7.66343218081719,-70.9633714127906,
-177.673574332209));
#136226=CARTESIAN_POINT('Ctrl Pts',(-7.65172493396012,-70.9649171451445,
-177.670587723936));
#136227=CARTESIAN_POINT('Ctrl Pts',(-7.64004659109474,-70.9664556187744,
-177.667371199654));
#136228=CARTESIAN_POINT('Ctrl Pts',(-7.60920468563951,-70.9705186488451,
-177.658876523743));
#136229=CARTESIAN_POINT('Ctrl Pts',(-7.57859346492051,-70.9745271017095,
-177.64877837365));
#136230=CARTESIAN_POINT('Ctrl Pts',(-7.54854310099584,-70.9784389453262,
-177.637166030246));
#136231=CARTESIAN_POINT('Ctrl Pts',(-7.52067144326531,-70.9820671731458,
-177.626395602919));
#136232=CARTESIAN_POINT('Ctrl Pts',(-7.49328227206125,-70.9856123005525,
-177.614321694518));
#136233=CARTESIAN_POINT('Ctrl Pts',(-7.4666388775123,-70.9890415496571,
-177.601070367657));
#136234=CARTESIAN_POINT('Ctrl Pts',(-7.46098971645269,-70.9897686484684,
-177.598260707666));
#136235=CARTESIAN_POINT('Ctrl Pts',(-7.45537399181997,-70.9904905521545,
-177.595398277761));
#136236=CARTESIAN_POINT('Ctrl Pts',(-7.44979405295274,-70.9912069730377,
-177.59248453496));
#136237=CARTESIAN_POINT('Ctrl Pts',(-7.44926963945517,-70.9912743036645,
-177.59221069575));
#136238=CARTESIAN_POINT('Ctrl Pts',(-7.44874551143164,-70.9913415902563,
-177.591936395013));
#136239=CARTESIAN_POINT('Ctrl Pts',(-7.44822167031191,-70.9914088326578,
-177.591661634332));
#136240=CARTESIAN_POINT('Ctrl Pts',(-7.36341668567551,-71.0022947494168,
-177.547180446307));
#136241=CARTESIAN_POINT('Ctrl Pts',(-7.2849205420624,-71.0121779828215,
-177.489997024843));
#136242=CARTESIAN_POINT('Ctrl Pts',(-7.21521422000437,-71.0208423096892,
-177.423514614708));
#136243=CARTESIAN_POINT('Ctrl Pts',(-7.17900585545438,-71.0253429216357,
-177.388980884176));
#136244=CARTESIAN_POINT('Ctrl Pts',(-7.14516858275053,-71.029514703104,
-177.351937503402));
#136245=CARTESIAN_POINT('Ctrl Pts',(-7.1140463350679,-71.0333277050162,
-177.3128573618));
#136246=CARTESIAN_POINT('Ctrl Pts',(-7.11356074608129,-71.0333871978829,
-177.312247608721));
#136247=CARTESIAN_POINT('Ctrl Pts',(-7.11307579006789,-71.0334466073515,
-177.311637347152));
#136248=CARTESIAN_POINT('Ctrl Pts',(-7.11259146723154,-71.0335059334348,
-177.311026578643));
#136249=CARTESIAN_POINT('Ctrl Pts',(-7.05806005588037,-71.0401856412925,
-177.242258256475));
#136250=CARTESIAN_POINT('Ctrl Pts',(-7.01156780676673,-71.0458068303072,
-177.1670831198));
#136251=CARTESIAN_POINT('Ctrl Pts',(-6.97337953736936,-71.0503909874129,
-177.087652956333));
#136252=CARTESIAN_POINT('Ctrl Pts',(-6.94786514373973,-71.0534537601099,
-177.034583977593));
#136253=CARTESIAN_POINT('Ctrl Pts',(-6.9260581499733,-71.0560535184276,
-176.97961441076));
#136254=CARTESIAN_POINT('Ctrl Pts',(-6.90804579110999,-71.058195517224,
-176.923376416061));
#136255=CARTESIAN_POINT('Ctrl Pts',(-6.90788807893848,-71.0582142720847,
-176.922884008801));
#136256=CARTESIAN_POINT('Ctrl Pts',(-6.90773065840123,-71.0582329917957,
-176.922391517884));
#136257=CARTESIAN_POINT('Ctrl Pts',(-6.90757352937676,-71.0582516763749,
-176.921898943596));
#136258=CARTESIAN_POINT('Ctrl Pts',(-6.89200677785444,-71.0601027551398,
-176.873099674503));
#136259=CARTESIAN_POINT('Ctrl Pts',(-6.87933106860593,-71.0616054747708,
-176.82359063585));
#136260=CARTESIAN_POINT('Ctrl Pts',(-6.86938539001926,-71.0627821611453,
-176.773553029938));
#136261=CARTESIAN_POINT('Ctrl Pts',(-6.85903549341789,-71.0640066710871,
-176.72148176674));
#136262=CARTESIAN_POINT('Ctrl Pts',(-6.85164206564099,-71.0648780949575,
-176.668837206011));
#136263=CARTESIAN_POINT('Ctrl Pts',(-6.84707944646844,-71.065414925157,
-176.615812182358));
#136264=CARTESIAN_POINT('Ctrl Pts',(-6.84336254226504,-71.0658522499369,
-176.572615736228));
#136265=CARTESIAN_POINT('Ctrl Pts',(-6.84152542372878,-71.066067385123,
-176.529166339213));
#136266=CARTESIAN_POINT('Ctrl Pts',(-6.84152542372878,-71.066067385123,
-176.485569595297));
#136267=CARTESIAN_POINT('',(-7.40000000143918,-71.5626363369615,-176.485569595296));
#136268=CARTESIAN_POINT('Origin',(-6.9,-71.5626363369615,-176.485569595297));
#136269=CARTESIAN_POINT('Ctrl Pts',(-7.4,-71.5626363369618,-176.485569595297));
#136270=CARTESIAN_POINT('Ctrl Pts',(-7.4,-71.5272255526701,-176.585813210379));
#136271=CARTESIAN_POINT('Ctrl Pts',(-7.41072271257901,-71.4935573295699,
-176.680998879949));
#136272=CARTESIAN_POINT('Ctrl Pts',(-7.45636610731683,-71.4300660132009,
-176.85726439743));
#136273=CARTESIAN_POINT('Ctrl Pts',(-7.49125858243999,-71.4004398176271,
-176.937641167035));
#136274=CARTESIAN_POINT('Ctrl Pts',(-7.58359051438092,-71.3455846992379,
-177.074841178091));
#136275=CARTESIAN_POINT('Ctrl Pts',(-7.64153051403658,-71.3201342851139,
-177.131947985374));
#136276=CARTESIAN_POINT('Ctrl Pts',(-7.77193648886645,-71.274739088698,
-177.212399058377));
#136277=CARTESIAN_POINT('Ctrl Pts',(-7.84535391894273,-71.2544423085659,
-177.236091643156));
#136278=CARTESIAN_POINT('Ctrl Pts',(-7.91859121655449,-71.2381488509313,
-177.239961484006));
#136279=CARTESIAN_POINT('Origin',(-6.9,-71.5626363369615,-179.64995));
#136280=CARTESIAN_POINT('',(-6.84152542372877,-71.066067385123,-171.871644662643));
#136281=CARTESIAN_POINT('',(-6.84152542372878,-71.066067385123,-179.64995));
#136282=CARTESIAN_POINT('',(-7.4,-71.5626363369615,-171.871644662643));
#136283=CARTESIAN_POINT('Origin',(-6.9,-71.5626363369615,-171.871644662643));
#136284=CARTESIAN_POINT('',(-7.4,-71.5626363369615,-176.798439391084));
#136285=CARTESIAN_POINT('Origin',(0.,-12.9675000200281,-171.871644662643));
#136286=CARTESIAN_POINT('',(-1.23940677966098,-71.4543692372681,-171.871644662643));
#136287=CARTESIAN_POINT('Origin',(0.,-12.9675000200281,-171.871644662643));
#136288=CARTESIAN_POINT('',(-1.24037635835043,-71.360635368318,-171.449026400902));
#136289=CARTESIAN_POINT('Origin',(-1.24989913208291,-70.4548469135707,-171.87165100631));
#136290=CARTESIAN_POINT('',(-6.84687749809456,-70.9710952348089,-171.449026400902));
#136291=CARTESIAN_POINT('Origin',(0.,-12.9675000200281,-171.449026400902));
#136292=CARTESIAN_POINT('Origin',(-6.92386407101644,-69.6082647247615,-171.968716884213));
#136293=CARTESIAN_POINT('Origin',(-1.24999999999996,-71.9542570083556,-179.64995));
#136294=CARTESIAN_POINT('',(-0.749999999999965,-71.9542570083556,-176.344247731786));
#136295=CARTESIAN_POINT('',(-1.23940677966098,-71.4543692372681,-176.344247731786));
#136296=CARTESIAN_POINT('Origin',(-1.24999999999996,-71.9542570083556,-176.344247731786));
#136297=CARTESIAN_POINT('',(-0.749999999999965,-71.9542570083556,-171.871644662643));
#136298=CARTESIAN_POINT('',(-0.749999999999965,-71.9542570083556,-171.871644662643));
#136299=CARTESIAN_POINT('Origin',(-1.24999999999996,-71.9542570083556,-171.871644662643));
#136300=CARTESIAN_POINT('',(-1.23940677966098,-71.4543692372681,-179.64995));
#136301=CARTESIAN_POINT('Ctrl Pts',(-0.747421739247287,-71.9934178165856,
-176.221164796295));
#136302=CARTESIAN_POINT('Ctrl Pts',(-0.70616503121794,-71.4656369062186,
-176.224399921719));
#136303=CARTESIAN_POINT('Ctrl Pts',(-1.23427661107857,-71.4545023028019,
-176.191083684094));
#136304=CARTESIAN_POINT('Ctrl Pts',(-0.758975746064385,-71.9025894407889,
-176.507953684521));
#136305=CARTESIAN_POINT('Ctrl Pts',(-0.81048947165755,-71.4635573472225,
-176.471174785183));
#136306=CARTESIAN_POINT('Ctrl Pts',(-1.25722997205992,-71.45389181123,-176.53857099329));
#136307=CARTESIAN_POINT('Ctrl Pts',(-0.733576267199836,-71.8205532116895,
-176.762007115851));
#136308=CARTESIAN_POINT('Ctrl Pts',(-0.846229070149368,-71.4625657314852,
-176.781098235956));
#136309=CARTESIAN_POINT('Ctrl Pts',(-1.20689317142187,-71.4553901565039,
-176.912968106426));
#136310=CARTESIAN_POINT('Ctrl Pts',(-0.61137645617211,-71.7551248751779,
-176.992297889673));
#136311=CARTESIAN_POINT('Ctrl Pts',(-0.713096236824655,-71.463696805273,
-177.074741700705));
#136312=CARTESIAN_POINT('Ctrl Pts',(-0.964561766455219,-71.4595630740809,
-177.27289534809));
#136313=CARTESIAN_POINT('Ctrl Pts',(-0.587032103695945,-71.7450861570452,
-177.028762667147));
#136314=CARTESIAN_POINT('Ctrl Pts',(-0.685202146366885,-71.4639504420806,
-177.120826376552));
#136315=CARTESIAN_POINT('Ctrl Pts',(-0.916284213905676,-71.4603489737626,
-177.330911863332));
#136316=CARTESIAN_POINT('Ctrl Pts',(-0.532211729471667,-71.7276623467411,
-177.093668859127));
#136317=CARTESIAN_POINT('Ctrl Pts',(-0.619044665129952,-71.4645348847711,
-177.203483227351));
#136318=CARTESIAN_POINT('Ctrl Pts',(-0.807567270427997,-71.4619509584614,
-177.435272175182));
#136319=CARTESIAN_POINT('Ctrl Pts',(-0.501290424235228,-71.7202266627171,
-177.122322890028));
#136320=CARTESIAN_POINT('Ctrl Pts',(-0.580169914453843,-71.4648703870088,
-177.240630878936));
#136321=CARTESIAN_POINT('Ctrl Pts',(-0.746244778353079,-71.4627761544078,
-177.481978941987));
#136322=CARTESIAN_POINT('Ctrl Pts',(-0.380827972894088,-71.6987946446081,
-177.206922015165));
#136323=CARTESIAN_POINT('Ctrl Pts',(-0.426114111673254,-71.4660826321625,
-177.349931905848));
#136324=CARTESIAN_POINT('Ctrl Pts',(-0.507344188737427,-71.4655588391503,
-177.620801033149));
#136325=CARTESIAN_POINT('Ctrl Pts',(-0.275357886911095,-71.6936685153208,
-177.231454787208));
#136326=CARTESIAN_POINT('Ctrl Pts',(-0.28195822162906,-71.4669790634829,
-177.384469640037));
#136327=CARTESIAN_POINT('Ctrl Pts',(-0.298170239974036,-71.4671552685673,
-177.662854386168));
#136328=CARTESIAN_POINT('Ctrl Pts',(-0.17210844915256,-71.7001976451323,
-177.207208612955));
#136329=CARTESIAN_POINT('Ctrl Pts',(-0.144256214768473,-71.4673303402777,
-177.351394652173));
#136330=CARTESIAN_POINT('Ctrl Pts',(-0.093404169259408,-71.4674008940711,
-177.622262820987));
#136331=CARTESIAN_POINT('',(-0.250942966392183,-71.6973964039529,-177.216474976116));
#136332=CARTESIAN_POINT('',(-0.249751305446096,-71.4669668918333,-177.637584354353));
#136333=CARTESIAN_POINT('Origin',(-0.25188593198836,-71.966962335182,-177.637584354353));
#136334=CARTESIAN_POINT('Ctrl Pts',(-0.250942967586682,-71.6973967453598,
-177.21647550955));
#136335=CARTESIAN_POINT('Ctrl Pts',(-0.272289386377385,-71.6972560147929,
-177.21651778088));
#136336=CARTESIAN_POINT('Ctrl Pts',(-0.29355234382452,-71.6975963514289,
-177.214625541668));
#136337=CARTESIAN_POINT('Ctrl Pts',(-0.314505400471286,-71.6984140417121,
-177.210861644173));
#136338=CARTESIAN_POINT('Ctrl Pts',(-0.335712123041887,-71.6992416312746,
-177.207052179459));
#136339=CARTESIAN_POINT('Ctrl Pts',(-0.356600655403705,-71.7005585587564,
-177.201326394673));
#136340=CARTESIAN_POINT('Ctrl Pts',(-0.376973851059467,-71.7023574770162,
-177.193788200059));
#136341=CARTESIAN_POINT('Ctrl Pts',(-0.397939430005541,-71.7042087017054,
-177.186030820365));
#136342=CARTESIAN_POINT('Ctrl Pts',(-0.418358881240999,-71.7065707314756,
-177.176355157432));
#136343=CARTESIAN_POINT('Ctrl Pts',(-0.438065962998032,-71.7094261265985,
-177.164899868662));
#136344=CARTESIAN_POINT('Ctrl Pts',(-0.448444784692127,-71.7109299330581,
-177.15886689021));
#136345=CARTESIAN_POINT('Ctrl Pts',(-0.458626866764958,-71.7125703880655,
-177.152340621388));
#136346=CARTESIAN_POINT('Ctrl Pts',(-0.468593349490525,-71.7143434487124,
-177.145342538011));
#136347=CARTESIAN_POINT('Ctrl Pts',(-0.482831780147209,-71.7168764989135,
-177.135344856017));
#136348=CARTESIAN_POINT('Ctrl Pts',(-0.49674155482062,-71.7197238945552,
-177.124284610517));
#136349=CARTESIAN_POINT('Ctrl Pts',(-0.510160832381796,-71.7228419069474,
-177.112294550298));
#136350=CARTESIAN_POINT('Ctrl Pts',(-0.523556614986982,-71.7259544602108,
-177.100325482711));
#136351=CARTESIAN_POINT('Ctrl Pts',(-0.536462801325541,-71.7293367437336,
-177.087430553005));
#136352=CARTESIAN_POINT('Ctrl Pts',(-0.548750322054646,-71.7329694869921,
-177.073774966279));
#136353=CARTESIAN_POINT('Ctrl Pts',(-0.552444173025322,-71.7340615553196,
-177.069669849926));
#136354=CARTESIAN_POINT('Ctrl Pts',(-0.556082376451407,-71.7351764190293,
-177.065496177473));
#136355=CARTESIAN_POINT('Ctrl Pts',(-0.559662137354108,-71.7363139575646,
-177.061258859581));
#136356=CARTESIAN_POINT('Ctrl Pts',(-0.574421398896868,-71.7410039995011,
-177.043788507593));
#136357=CARTESIAN_POINT('Ctrl Pts',(-0.588291608237107,-71.746070304877,
-177.025148207316));
#136358=CARTESIAN_POINT('Ctrl Pts',(-0.601309402288751,-71.7515531186499,
-177.005343891899));
#136359=CARTESIAN_POINT('Ctrl Pts',(-0.612473327545254,-71.7562551229153,
-176.988359916258));
#136360=CARTESIAN_POINT('Ctrl Pts',(-0.623010909387807,-71.7612627209243,
-176.97051897202));
#136361=CARTESIAN_POINT('Ctrl Pts',(-0.632942561425503,-71.7665782772395,
-176.951804930916));
#136362=CARTESIAN_POINT('Ctrl Pts',(-0.645798430805969,-71.7734589147622,
-176.927580837371));
#136363=CARTESIAN_POINT('Ctrl Pts',(-0.657488093972069,-71.7807562798892,
-176.902183776764));
#136364=CARTESIAN_POINT('Ctrl Pts',(-0.66803034729961,-71.7884603514116,
-176.875777760919));
#136365=CARTESIAN_POINT('Ctrl Pts',(-0.67883683320761,-71.7963575189103,
-176.848709900827));
#136366=CARTESIAN_POINT('Ctrl Pts',(-0.688438466109612,-71.8046821807652,
-176.820582401159));
#136367=CARTESIAN_POINT('Ctrl Pts',(-0.696894970215001,-71.8134135310904,
-176.791534794693));
#136368=CARTESIAN_POINT('Ctrl Pts',(-0.705747603657008,-71.8225538854166,
-176.761126506682));
#136369=CARTESIAN_POINT('Ctrl Pts',(-0.713346151475314,-71.8321400413436,
-176.729710293235));
#136370=CARTESIAN_POINT('Ctrl Pts',(-0.719789108725433,-71.8421351271434,
-176.69739845248));
#136371=CARTESIAN_POINT('Ctrl Pts',(-0.726420722863542,-71.8524228800694,
-176.664140485421));
#136372=CARTESIAN_POINT('Ctrl Pts',(-0.731829007749542,-71.8631438606517,
-176.629933637363));
#136373=CARTESIAN_POINT('Ctrl Pts',(-0.736138331198896,-71.8742435001081,
-176.594848190457));
#136374=CARTESIAN_POINT('Ctrl Pts',(-0.740663192872281,-71.8858983071225,
-176.55800788458));
#136375=CARTESIAN_POINT('Ctrl Pts',(-0.743977251576075,-71.8979705598559,
-176.520198759072));
#136376=CARTESIAN_POINT('Ctrl Pts',(-0.746228912135858,-71.9103817043686,
-176.481446564245));
#136377=CARTESIAN_POINT('Ctrl Pts',(-0.747198200169345,-71.9157244163533,
-176.464764636522));
#136378=CARTESIAN_POINT('Ctrl Pts',(-0.747970592530854,-71.9211297455964,
-176.447907285908));
#136379=CARTESIAN_POINT('Ctrl Pts',(-0.748557632300597,-71.9265906597324,
-176.430873773194));
#136380=CARTESIAN_POINT('Ctrl Pts',(-0.749535729765846,-71.9356893725448,
-176.402493352533));
#136381=CARTESIAN_POINT('Ctrl Pts',(-0.749999463873935,-71.9449293580282,
-176.373615401923));
#136382=CARTESIAN_POINT('Ctrl Pts',(-0.749999999535633,-71.9542570083556,
-176.344247731786));
#136383=CARTESIAN_POINT('Ctrl Pts',(-1.23940677966098,-71.4543692372681,
-176.344247731786));
#136384=CARTESIAN_POINT('Ctrl Pts',(-1.23940681800414,-71.4543692364556,
-176.64594121493));
#136385=CARTESIAN_POINT('Ctrl Pts',(-1.17782106642746,-71.4558907746468,
-176.956147992919));
#136386=CARTESIAN_POINT('Ctrl Pts',(-0.964561766455219,-71.4595630740809,
-177.27289534809));
#136387=CARTESIAN_POINT('Ctrl Pts',(-0.916284213905676,-71.4603489737626,
-177.330911863332));
#136388=CARTESIAN_POINT('Ctrl Pts',(-0.807567270427997,-71.4619509584614,
-177.435272175182));
#136389=CARTESIAN_POINT('Ctrl Pts',(-0.746244778353079,-71.4627761544078,
-177.481978941987));
#136390=CARTESIAN_POINT('Ctrl Pts',(-0.55157424298232,-71.4650436529077,
-177.595099511724));
#136391=CARTESIAN_POINT('Ctrl Pts',(-0.402234283661645,-71.4663158974755,
-177.637660247068));
#136392=CARTESIAN_POINT('Ctrl Pts',(-0.249751305446096,-71.4669668918333,
-177.637584354353));
#136393=CARTESIAN_POINT('Origin',(-26.4569673975197,-68.4857751744904,-179.64995));
#136394=CARTESIAN_POINT('',(-25.548606520418,-65.6266003779886,-171.854014632027));
#136395=CARTESIAN_POINT('',(-25.548606520496,-65.6266003779638,-176.84995));
#136396=CARTESIAN_POINT('',(-25.548606520496,-65.6266003779638,-179.64995));
#136397=CARTESIAN_POINT('',(-26.0394480946395,-65.5149709682656,-172.038055421481));
#136398=CARTESIAN_POINT('Ctrl Pts',(-26.0394480946395,-65.5149709682656,
-172.038055421481));
#136399=CARTESIAN_POINT('Ctrl Pts',(-25.8744525829839,-65.5381595751959,
-171.964276677778));
#136400=CARTESIAN_POINT('Ctrl Pts',(-25.7113823551758,-65.5748168753238,
-171.898042693471));
#136401=CARTESIAN_POINT('Ctrl Pts',(-25.5486065204936,-65.6266003779646,
-171.854014632593));
#136402=CARTESIAN_POINT('',(-26.0394480946395,-65.5149709682656,-171.64995));
#136403=CARTESIAN_POINT('',(-25.166383622031,-65.7775666303703,-177.581785882201));
#136404=CARTESIAN_POINT('',(-25.166383622031,-65.7775666303703,-179.64995));
#136405=CARTESIAN_POINT('Ctrl Pts',(-25.548606520496,-65.6266003779638,
-176.84995));
#136406=CARTESIAN_POINT('Ctrl Pts',(-25.5486064910184,-65.6266003873288,
-176.988420898571));
#136407=CARTESIAN_POINT('Ctrl Pts',(-25.5128982512925,-65.6373177084965,
-177.128208340634));
#136408=CARTESIAN_POINT('Ctrl Pts',(-25.3800542465628,-65.6848405887261,
-177.37909156612));
#136409=CARTESIAN_POINT('Ctrl Pts',(-25.2828559308331,-65.7220623109706,
-177.491403988801));
#136410=CARTESIAN_POINT('Ctrl Pts',(-25.166383622031,-65.7775666303703,
-177.581785882201));
#136411=CARTESIAN_POINT('Ctrl Pts',(-25.0407404589729,-66.228934721057,
-177.2158679411));
#136412=CARTESIAN_POINT('Ctrl Pts',(-24.9516549782085,-65.8798945343463,
-177.298823774072));
#136413=CARTESIAN_POINT('Ctrl Pts',(-25.166383622031,-65.7775666303703,
-177.581785882201));
#136414=CARTESIAN_POINT('Ctrl Pts',(-24.9465334973015,-66.3187224932389,
-177.303592864513));
#136415=CARTESIAN_POINT('Ctrl Pts',(-24.8039770572177,-65.9493003143299,
-177.391803085524));
#136416=CARTESIAN_POINT('Ctrl Pts',(-24.9795558812766,-65.8665984929838,
-177.757245548006));
#136417=CARTESIAN_POINT('Ctrl Pts',(-24.8237985595108,-66.4342348178924,
-177.34995));
#136418=CARTESIAN_POINT('Ctrl Pts',(-24.6278738771108,-66.0310529650264,
-177.399536111675));
#136419=CARTESIAN_POINT('Ctrl Pts',(-24.7362442762044,-65.9810957924573,
-177.84994999494));
#136420=CARTESIAN_POINT('Ctrl Pts',(-24.7,-66.548373473155,-177.34995));
#136421=CARTESIAN_POINT('Ctrl Pts',(-24.4906779661017,-66.0942982743998,
-177.34995));
#136422=CARTESIAN_POINT('Ctrl Pts',(-24.4906779661017,-66.0942982743997,
-177.84995));
#136423=CARTESIAN_POINT('',(-24.7,-66.5483734731532,-177.34995));
#136424=CARTESIAN_POINT('',(-24.4906779661044,-66.0942982743985,-177.84995));
#136425=CARTESIAN_POINT('Origin',(-24.7000000000027,-66.5483734731538,-177.84995));
#136426=CARTESIAN_POINT('',(-25.0407404589729,-66.228934721057,-177.2158679411));
#136427=CARTESIAN_POINT('Ctrl Pts',(-24.7,-66.5483734731532,-177.34995));
#136428=CARTESIAN_POINT('Ctrl Pts',(-24.8237985595108,-66.4342348178924,
-177.34995));
#136429=CARTESIAN_POINT('Ctrl Pts',(-24.9465334973015,-66.3187224932389,
-177.303592864513));
#136430=CARTESIAN_POINT('Ctrl Pts',(-25.0407404589729,-66.228934721057,
-177.2158679411));
#136431=CARTESIAN_POINT('Origin',(-25.3814809179458,-66.228934721057,-177.581785882201));
#136432=CARTESIAN_POINT('Ctrl Pts',(-25.166383622031,-65.7775666303703,
-177.581785882201));
#136433=CARTESIAN_POINT('Ctrl Pts',(-24.9795558812766,-65.8665984929838,
-177.757245548006));
#136434=CARTESIAN_POINT('Ctrl Pts',(-24.7362442762044,-65.9810957924573,
-177.84994999494));
#136435=CARTESIAN_POINT('Ctrl Pts',(-24.4906779661044,-66.0942982743985,
-177.84995));
#136436=CARTESIAN_POINT('Origin',(0.,-12.9675000200281,-177.84995));
#136437=CARTESIAN_POINT('Origin',(0.,-12.9675000200281,-177.34995));
#136438=CARTESIAN_POINT('Origin',(0.,-12.9675000200281,-177.84995));
#136439=CARTESIAN_POINT('Ctrl Pts',(-0.749999999999964,-72.58000002,-174.689806803097));
#136440=CARTESIAN_POINT('Ctrl Pts',(-0.749999999999964,-73.08000002,-174.689806803097));
#136441=CARTESIAN_POINT('Ctrl Pts',(-0.249999999999964,-73.08000002,-174.689806803097));
#136442=CARTESIAN_POINT('Ctrl Pts',(-0.749999999999964,-72.5800000142362,
-174.901707787501));
#136443=CARTESIAN_POINT('Ctrl Pts',(-0.749999999999999,-73.0799033011073,
-174.944063234271));
#136444=CARTESIAN_POINT('Ctrl Pts',(-0.250096721285987,-73.08000002,-174.944087763949));
#136445=CARTESIAN_POINT('Ctrl Pts',(-0.749999999999964,-72.5534802154039,
-175.109145968138));
#136446=CARTESIAN_POINT('Ctrl Pts',(-0.749999999999976,-73.047991321912,
-175.192966486363));
#136447=CARTESIAN_POINT('Ctrl Pts',(-0.25019084538922,-73.0481762528639,
-175.193013365813));
#136448=CARTESIAN_POINT('Ctrl Pts',(-0.749999999999964,-72.4491003622499,
-175.515225349862));
#136449=CARTESIAN_POINT('Ctrl Pts',(-0.749999999999953,-72.9225699879354,
-175.680169902411));
#136450=CARTESIAN_POINT('Ctrl Pts',(-0.250374112266224,-72.9229204323206,
-175.680308208816));
#136451=CARTESIAN_POINT('Ctrl Pts',(-0.749999999999965,-72.3702407172373,
-175.713745513771));
#136452=CARTESIAN_POINT('Ctrl Pts',(-0.750000000001358,-72.8278715101479,
-175.918330718485));
#136453=CARTESIAN_POINT('Ctrl Pts',(-0.250463183534996,-72.8282888567225,
-175.918532203572));
#136454=CARTESIAN_POINT('Ctrl Pts',(-0.749999999999965,-72.1685246628573,
-176.079670924798));
#136455=CARTESIAN_POINT('Ctrl Pts',(-0.749999999998571,-72.5857133666792,
-176.357282462775));
#136456=CARTESIAN_POINT('Ctrl Pts',(-0.25062659166413,-72.5862295913911,
-176.357642327882));
#136457=CARTESIAN_POINT('Ctrl Pts',(-0.749999999999965,-72.0428483696925,
-176.252247715791));
#136458=CARTESIAN_POINT('Ctrl Pts',(-0.749999999997964,-72.4348744309047,
-176.56428717754));
#136459=CARTESIAN_POINT('Ctrl Pts',(-0.250703242845797,-72.4354180409157,
-176.564734305741));
#136460=CARTESIAN_POINT('Ctrl Pts',(-0.749999999999965,-71.7551070954922,
-176.557430126179));
#136461=CARTESIAN_POINT('Ctrl Pts',(-0.750000000001966,-72.0895755229708,
-176.930319469104));
#136462=CARTESIAN_POINT('Ctrl Pts',(-0.250838284668646,-72.090128509306,
-176.930952892336));
#136463=CARTESIAN_POINT('Ctrl Pts',(-0.749999999999965,-71.5938796749303,
-176.690562238895));
#136464=CARTESIAN_POINT('Ctrl Pts',(-0.749999999997485,-71.8961205198801,
-177.08999030776));
#136465=CARTESIAN_POINT('Ctrl Pts',(-0.250896921774036,-71.8966556096658,
-177.090711302921));
#136466=CARTESIAN_POINT('Ctrl Pts',(-0.749999999999965,-71.414849447251,
-176.803618488051));
#136467=CARTESIAN_POINT('Ctrl Pts',(-0.749999999999965,-71.6813148644928,
-177.225579834422));
#136468=CARTESIAN_POINT('Ctrl Pts',(-0.250946592270043,-71.6818193327012,
-177.226378685119));
#136469=CARTESIAN_POINT('',(-0.249999999999962,-73.08000002,-174.689806803098));
#136470=CARTESIAN_POINT('Ctrl Pts',(-0.250942965994136,-71.6973962901632,
-177.216474798313));
#136471=CARTESIAN_POINT('Ctrl Pts',(-0.250894093572665,-71.906018225657,
-177.082956409594));
#136472=CARTESIAN_POINT('Ctrl Pts',(-0.250836667095525,-72.0943113105341,
-176.926516558683));
#136473=CARTESIAN_POINT('Ctrl Pts',(-0.250703261157637,-72.4354180408958,
-176.564734305724));
#136474=CARTESIAN_POINT('Ctrl Pts',(-0.250626609977381,-72.5862295913722,
-176.357642327869));
#136475=CARTESIAN_POINT('Ctrl Pts',(-0.250463201851249,-72.8282888567072,
-175.918532203564));
#136476=CARTESIAN_POINT('Ctrl Pts',(-0.250374130584112,-72.9229204323078,
-175.680308208811));
#136477=CARTESIAN_POINT('Ctrl Pts',(-0.250190863710472,-73.0481762528571,
-175.193013365811));
#136478=CARTESIAN_POINT('Ctrl Pts',(-0.250096739608965,-73.0800000199965,
-174.944087763948));
#136479=CARTESIAN_POINT('Ctrl Pts',(-0.249999999999962,-73.08000002,-174.689806803098));
#136480=CARTESIAN_POINT('',(-0.749999999999964,-72.58000002,-174.689806803098));
#136481=CARTESIAN_POINT('Origin',(-0.249999999999964,-72.58000002,-174.689806803098));
#136482=CARTESIAN_POINT('Ctrl Pts',(-0.749999999999964,-72.58000002,-174.689806803098));
#136483=CARTESIAN_POINT('Ctrl Pts',(-0.749999999999964,-72.58000002,-174.831376286945));
#136484=CARTESIAN_POINT('Ctrl Pts',(-0.750000000181377,-72.5681788618565,
-174.970941599173));
#136485=CARTESIAN_POINT('Ctrl Pts',(-0.749999999141365,-72.5447649315039,
-175.108599805088));
#136486=CARTESIAN_POINT('Ctrl Pts',(-0.749999998625103,-72.5331422713358,
-175.176933251143));
#136487=CARTESIAN_POINT('Ctrl Pts',(-0.749999997778457,-72.5186622030691,
-175.244796569616));
#136488=CARTESIAN_POINT('Ctrl Pts',(-0.749999996441189,-72.501348066122,
-175.312200510247));
#136489=CARTESIAN_POINT('Ctrl Pts',(-0.749999994685787,-72.4786201957877,
-175.400680116672));
#136490=CARTESIAN_POINT('Ctrl Pts',(-0.749999992058193,-72.4508191867992,
-175.488345833607));
#136491=CARTESIAN_POINT('Ctrl Pts',(-0.749999988588697,-72.4183069147095,
-175.574298130555));
#136492=CARTESIAN_POINT('Ctrl Pts',(-0.749999986546665,-72.3991712571468,
-175.624886834925));
#136493=CARTESIAN_POINT('Ctrl Pts',(-0.749999987460588,-72.3784930875005,
-175.674621364586));
#136494=CARTESIAN_POINT('Ctrl Pts',(-0.749999990785369,-72.3562980983182,
-175.723514264023));
#136495=CARTESIAN_POINT('Ctrl Pts',(-0.749999992115961,-72.347415567763,
-175.7430814136));
#136496=CARTESIAN_POINT('Ctrl Pts',(-0.749999993758535,-72.3382895360997,
-175.762513592358));
#136497=CARTESIAN_POINT('Ctrl Pts',(-0.749999995341683,-72.3289194940821,
-175.781810711456));
#136498=CARTESIAN_POINT('Ctrl Pts',(-0.749999998527987,-72.3100609827057,
-175.820648844665));
#136499=CARTESIAN_POINT('Ctrl Pts',(-0.749999999364237,-72.2901904086323,
-175.8590152493));
#136500=CARTESIAN_POINT('Ctrl Pts',(-0.749999999592108,-72.2694003762988,
-175.896717968815));
#136501=CARTESIAN_POINT('Ctrl Pts',(-0.749999999760363,-72.2540495109209,
-175.924556760134));
#136502=CARTESIAN_POINT('Ctrl Pts',(-0.749999999832536,-72.2381324361931,
-175.952153763115));
#136503=CARTESIAN_POINT('Ctrl Pts',(-0.749999998887563,-72.22169996255,
-175.979441154676));
#136504=CARTESIAN_POINT('Ctrl Pts',(-0.749999996495687,-72.1801067750961,
-176.048509854675));
#136505=CARTESIAN_POINT('Ctrl Pts',(-0.749999993208358,-72.1348499287488,
-176.116013152087));
#136506=CARTESIAN_POINT('Ctrl Pts',(-0.749999994093549,-72.0863465370676,
-176.181265394643));
#136507=CARTESIAN_POINT('Ctrl Pts',(-0.749999994855056,-72.0446203524745,
-176.237400172514));
#136508=CARTESIAN_POINT('Ctrl Pts',(-0.749999998190332,-72.0004927389796,
-176.291868658539));
#136509=CARTESIAN_POINT('Ctrl Pts',(-0.749999999535633,-71.9542570083556,
-176.344247731786));
#136510=CARTESIAN_POINT('Origin',(-0.249999999999964,-72.58000002,-55.24995));
#136511=CARTESIAN_POINT('',(-0.249999999999964,-73.08000002,-57.9657868813819));
#136512=CARTESIAN_POINT('',(-0.249999999999964,-73.08000002,-57.9678366169137));
#136513=CARTESIAN_POINT('',(-0.749999999999964,-72.58000002,-57.9657868813819));
#136514=CARTESIAN_POINT('Origin',(-0.249999999999964,-72.58000002,-57.9657868813819));
#136515=CARTESIAN_POINT('',(-0.749999999999964,-72.58000002,-174.687529226493));
#136516=CARTESIAN_POINT('Ctrl Pts',(-0.249999999999964,-73.08000002,-57.9657868813819));
#136517=CARTESIAN_POINT('Ctrl Pts',(-0.749999999999964,-73.08000002,-57.9657868813819));
#136518=CARTESIAN_POINT('Ctrl Pts',(-0.749999999999964,-72.58000002,-57.9657868813819));
#136519=CARTESIAN_POINT('Ctrl Pts',(-0.250090304006367,-73.08000002,-57.7020110302663));
#136520=CARTESIAN_POINT('Ctrl Pts',(-0.749999999999964,-73.0799097169388,
-57.7020347823602));
#136521=CARTESIAN_POINT('Ctrl Pts',(-0.749999999999964,-72.5800000140225,
-57.7459735178474));
#136522=CARTESIAN_POINT('Ctrl Pts',(-0.250178150913126,-73.0457949912512,
-57.4439860415223));
#136523=CARTESIAN_POINT('Ctrl Pts',(-0.749999999999964,-73.0456227684187,
-57.4440313928443));
#136524=CARTESIAN_POINT('Ctrl Pts',(-0.749999999999964,-72.5514958309333,
-57.5309525432158));
#136525=CARTESIAN_POINT('Ctrl Pts',(-0.250306370454135,-72.9447005728246,
-57.0654831530319));
#136526=CARTESIAN_POINT('Ctrl Pts',(-0.749999999999965,-72.9444091558477,
-57.0655786327141));
#136527=CARTESIAN_POINT('Ctrl Pts',(-0.749999999999964,-72.4672504799085,
-57.2155332517716));
#136528=CARTESIAN_POINT('Ctrl Pts',(-0.25034879630597,-72.9021819864826,
-56.9399108365871));
#136529=CARTESIAN_POINT('Ctrl Pts',(-0.749999999999971,-72.9018554492066,
-56.9400333127282));
#136530=CARTESIAN_POINT('Ctrl Pts',(-0.749999999999964,-72.4318183244811,
-57.1108895827629));
#136531=CARTESIAN_POINT('Ctrl Pts',(-0.250430320614374,-72.8021179994285,
-56.6980298209841));
#136532=CARTESIAN_POINT('Ctrl Pts',(-0.749999999999958,-72.8017292323873,
-56.6982147960383));
#136533=CARTESIAN_POINT('Ctrl Pts',(-0.749999999999964,-72.3484316704448,
-56.9093219305338));
#136534=CARTESIAN_POINT('Ctrl Pts',(-0.250469580226035,-72.744578160532,
-56.5812500750007));
#136535=CARTESIAN_POINT('Ctrl Pts',(-0.74999999999997,-72.7441631076294,
-56.581469426742));
#136536=CARTESIAN_POINT('Ctrl Pts',(-0.749999999999965,-72.300481803901,
-56.8120054092621));
#136537=CARTESIAN_POINT('Ctrl Pts',(-0.250582991914968,-72.5498603521484,
-56.2431574556907));
#136538=CARTESIAN_POINT('Ctrl Pts',(-0.749999999999952,-72.5493874743356,
-56.2435031793822));
#136539=CARTESIAN_POINT('Ctrl Pts',(-0.749999999999965,-72.1382169632082,
-56.5302613678863));
#136540=CARTESIAN_POINT('Ctrl Pts',(-0.250653625589273,-72.3879279481205,
-56.0315291953545));
#136541=CARTESIAN_POINT('Ctrl Pts',(-0.749999999999435,-72.3874332788213,
-56.0319576106046));
#136542=CARTESIAN_POINT('Ctrl Pts',(-0.749999999999965,-72.0032732927043,
-56.3539043654751));
#136543=CARTESIAN_POINT('Ctrl Pts',(-0.250776334581247,-72.0199436379809,
-55.6626353009023));
#136544=CARTESIAN_POINT('Ctrl Pts',(-0.750000000000494,-72.0194499168863,
-55.6632379181992));
#136545=CARTESIAN_POINT('Ctrl Pts',(-0.749999999999965,-71.6966197023802,
-56.0464925782632));
#136546=CARTESIAN_POINT('Ctrl Pts',(-0.250829232083772,-71.8132859417639,
-55.5029329728744));
#136547=CARTESIAN_POINT('Ctrl Pts',(-0.749999999997384,-71.8128142650138,
-55.5036164406727));
#136548=CARTESIAN_POINT('Ctrl Pts',(-0.749999999999965,-71.5244049571092,
-55.9134072123415));
#136549=CARTESIAN_POINT('Ctrl Pts',(-0.250873059487692,-71.5845312649516,
-55.3703284570208));
#136550=CARTESIAN_POINT('Ctrl Pts',(-0.749999999999965,-71.5840941797283,
-55.3710824677091));
#136551=CARTESIAN_POINT('Ctrl Pts',(-0.749999999999965,-71.3337760574596,
-55.8029033796444));
#136552=CARTESIAN_POINT('Ctrl Pts',(-0.749999999999965,-71.8417319269067,
-56.1920012792715));
#136553=CARTESIAN_POINT('Ctrl Pts',(-0.749999999999965,-71.8444758759865,
-56.1947266143563));
#136554=CARTESIAN_POINT('Ctrl Pts',(-0.749999999999854,-71.8472142189877,
-56.1974588803415));
#136555=CARTESIAN_POINT('Ctrl Pts',(-0.749999999999599,-71.849946925556,
-56.200198044911));
#136556=CARTESIAN_POINT('Ctrl Pts',(-0.749999999995322,-71.895797123968,
-56.246156597672));
#136557=CARTESIAN_POINT('Ctrl Pts',(-0.750000000361229,-71.9401028597185,
-56.2942420626362));
#136558=CARTESIAN_POINT('Ctrl Pts',(-0.74999999895657,-71.982527737009,
-56.344035893725));
#136559=CARTESIAN_POINT('Ctrl Pts',(-0.749999998672542,-71.9911062235921,
-56.3541044134048));
#136560=CARTESIAN_POINT('Ctrl Pts',(-0.749999998292393,-71.999607928201,
-56.3642426607214));
#136561=CARTESIAN_POINT('Ctrl Pts',(-0.749999997746176,-72.0080302616703,
-56.3744470046658));
#136562=CARTESIAN_POINT('Ctrl Pts',(-0.74999999604191,-72.0343090036282,
-56.4062858439066));
#136563=CARTESIAN_POINT('Ctrl Pts',(-0.749999992814762,-72.0598149071135,
-56.4387765753063));
#136564=CARTESIAN_POINT('Ctrl Pts',(-0.749999990764931,-72.0844669777911,
-56.471823595159));
#136565=CARTESIAN_POINT('Ctrl Pts',(-0.7499999887151,-72.1091190484687,
-56.5048706150117));
#136566=CARTESIAN_POINT('Ctrl Pts',(-0.74999998878556,-72.1329172515315,
-56.5384738714876));
#136567=CARTESIAN_POINT('Ctrl Pts',(-0.749999992523647,-72.1557838559918,
-56.5725357961293));
#136568=CARTESIAN_POINT('Ctrl Pts',(-0.749999997741391,-72.1877018007307,
-56.6200805302109));
#136569=CARTESIAN_POINT('Ctrl Pts',(-0.749999998819484,-72.2179714721241,
-56.6686674551481));
#136570=CARTESIAN_POINT('Ctrl Pts',(-0.749999999429074,-72.2464142286222,
-56.7180788042009));
#136571=CARTESIAN_POINT('Ctrl Pts',(-0.750000000419556,-72.2926289656521,
-56.7983640080249));
#136572=CARTESIAN_POINT('Ctrl Pts',(-0.749999999999578,-72.3344223494509,
-56.8812169184746));
#136573=CARTESIAN_POINT('Ctrl Pts',(-0.749999999999555,-72.3716419026398,
-56.9665912683841));
#136574=CARTESIAN_POINT('Ctrl Pts',(-0.749999999999551,-72.3771587620856,
-56.9792458611551));
#136575=CARTESIAN_POINT('Ctrl Pts',(-0.749999999999476,-72.382575206817,
-56.991955795638));
#136576=CARTESIAN_POINT('Ctrl Pts',(-0.749999999999378,-72.3878908196251,
-57.0047208623372));
#136577=CARTESIAN_POINT('Ctrl Pts',(-0.749999999999364,-72.3886377760633,
-57.0065146251825));
#136578=CARTESIAN_POINT('Ctrl Pts',(-0.749999999999346,-72.389382748593,
-57.0083094879105));
#136579=CARTESIAN_POINT('Ctrl Pts',(-0.749999999999324,-72.3901257364801,
-57.0101054509239));
#136580=CARTESIAN_POINT('Ctrl Pts',(-0.749999999998099,-72.4318199510488,
-57.1108894186501));
#136581=CARTESIAN_POINT('Ctrl Pts',(-0.749999999915445,-72.4672597866091,
-57.2155313871763));
#136582=CARTESIAN_POINT('Ctrl Pts',(-0.749999999861768,-72.4953436211357,
-57.3206699820974));
#136583=CARTESIAN_POINT('Ctrl Pts',(-0.749999999835408,-72.5091351036103,
-57.3723017166415));
#136584=CARTESIAN_POINT('Ctrl Pts',(-0.749999999849788,-72.5212576085903,
-57.4242193465116));
#136585=CARTESIAN_POINT('Ctrl Pts',(-0.749999999908996,-72.53169711994,
-57.4764233217448));
#136586=CARTESIAN_POINT('Ctrl Pts',(-0.75000000009092,-72.5637736078163,
-57.6368254825897));
#136587=CARTESIAN_POINT('Ctrl Pts',(-0.749999999999964,-72.58000002,-57.7999242188348));
#136588=CARTESIAN_POINT('Ctrl Pts',(-0.749999999999964,-72.58000002,-57.9657868813819));
#136589=CARTESIAN_POINT('Ctrl Pts',(-0.249999999999964,-73.08000002,-57.9657868813819));
#136590=CARTESIAN_POINT('Ctrl Pts',(-0.250090304006367,-73.08000002,-57.7020110302663));
#136591=CARTESIAN_POINT('Ctrl Pts',(-0.250178150913126,-73.0457949912512,
-57.4439860415223));
#136592=CARTESIAN_POINT('Ctrl Pts',(-0.250306370454135,-72.9447005728246,
-57.0654831530319));
#136593=CARTESIAN_POINT('Ctrl Pts',(-0.25034879630597,-72.9021819864826,
-56.9399108365871));
#136594=CARTESIAN_POINT('Ctrl Pts',(-0.250430320614374,-72.8021179994285,
-56.6980298209841));
#136595=CARTESIAN_POINT('Ctrl Pts',(-0.250469580226035,-72.744578160532,
-56.5812500750007));
#136596=CARTESIAN_POINT('Ctrl Pts',(-0.250582991914968,-72.5498603521484,
-56.2431574556907));
#136597=CARTESIAN_POINT('Ctrl Pts',(-0.250653625589273,-72.3879279481205,
-56.0315291953545));
#136598=CARTESIAN_POINT('Ctrl Pts',(-0.250774861685046,-72.0243606141434,
-55.6670631949548));
#136599=CARTESIAN_POINT('Ctrl Pts',(-0.250826687460303,-71.8231950647151,
-55.5106149664713));
#136600=CARTESIAN_POINT('Ctrl Pts',(-0.250869887203096,-71.6009673739964,
-55.3799259279342));
#136601=CARTESIAN_POINT('Ctrl Pts',(-1.24035792914739,-71.2481103336038,
-60.8508735991007));
#136602=CARTESIAN_POINT('Ctrl Pts',(-0.749999999999965,-71.2566817467534,
-60.8548714197835));
#136603=CARTESIAN_POINT('Ctrl Pts',(-0.749999999999965,-71.701161634982,
-61.0621827299711));
#136604=CARTESIAN_POINT('Ctrl Pts',(-1.23971725581624,-71.3097847042778,
-60.7186716617645));
#136605=CARTESIAN_POINT('Ctrl Pts',(-0.74999999999993,-71.3194598672011,
-60.7217601410269));
#136606=CARTESIAN_POINT('Ctrl Pts',(-0.749999999999965,-71.7936527766986,
-60.8638797025928));
#136607=CARTESIAN_POINT('Ctrl Pts',(-1.23938654221847,-71.3418443611191,
-60.5756111021815));
#136608=CARTESIAN_POINT('Ctrl Pts',(-0.749999999999964,-71.3522348667501,
-60.5771488614746));
#136609=CARTESIAN_POINT('Ctrl Pts',(-0.749999999999965,-71.8417316989903,
-60.6492890757558));
#136610=CARTESIAN_POINT('Ctrl Pts',(-1.2393865421354,-71.3418443611208,
-60.42825533736));
#136611=CARTESIAN_POINT('Ctrl Pts',(-0.749999999999964,-71.3522348691612,
-60.4282553373599));
#136612=CARTESIAN_POINT('Ctrl Pts',(-0.749999999999965,-71.8417317029411,
-60.42825533736));
#136613=CARTESIAN_POINT('',(-0.749999999999965,-71.701161634982,-61.0621827299711));
#136614=CARTESIAN_POINT('Origin',(-1.24999999999996,-71.701161634982,-61.0621827299711));
#136615=CARTESIAN_POINT('Origin',(-0.749999999999965,-69.6146150315905,
-60.2676349698354));
#136616=CARTESIAN_POINT('Origin',(-0.750000000000035,67.7009572055632,-55.24995));
#136617=CARTESIAN_POINT('',(-0.749999999999973,-55.5033748716332,-95.7875912885257));
#136618=CARTESIAN_POINT('Ctrl Pts',(-0.749999999999971,-55.5033748716332,
-95.7875912885257));
#136619=CARTESIAN_POINT('Ctrl Pts',(-0.749999999999969,-60.9031648374056,
-84.2127012585751));
#136620=CARTESIAN_POINT('Ctrl Pts',(-0.749999999999967,-66.3022815738571,
-72.6374971882577));
#136621=CARTESIAN_POINT('Ctrl Pts',(-0.749999999999965,-71.701161634982,
-61.062182729971));
#136622=CARTESIAN_POINT('',(-0.749999999999973,-55.08000002,-97.6965903014517));
#136623=CARTESIAN_POINT('Origin',(-0.749999999999973,-61.7707294446428,
-98.17800342417));
#136624=CARTESIAN_POINT('',(-0.749999999999973,-55.08000002,-134.362052670054));
#136625=CARTESIAN_POINT('',(-0.749999999999973,-55.08000002,-97.7195882395211));
#136626=CARTESIAN_POINT('',(-0.749999999999973,-55.5033748716332,-136.27105168298));
#136627=CARTESIAN_POINT('Origin',(-0.749999999999977,-61.7710312680802,
-133.877753475464));
#136628=CARTESIAN_POINT('',(-0.749999999999965,-71.813687061541,-171.237717270032));
#136629=CARTESIAN_POINT('Ctrl Pts',(-0.749999999999965,-71.813687061541,
-171.237717270032));
#136630=CARTESIAN_POINT('Ctrl Pts',(-0.749999999999967,-66.3773023734559,
-159.58198200727));
#136631=CARTESIAN_POINT('Ctrl Pts',(-0.74999999999997,-60.9406796476674,
-147.926357767621));
#136632=CARTESIAN_POINT('Ctrl Pts',(-0.749999999999973,-55.5033748716332,
-136.27105168298));
#136633=CARTESIAN_POINT('Origin',(-0.749999999999965,-69.7273331732481,
-172.033160909053));
#136634=CARTESIAN_POINT('Origin',(0.,-12.9675000200281,-60.64995));
#136635=CARTESIAN_POINT('',(-1.23668888567854,-55.0504149642627,-95.576281431058));
#136636=CARTESIAN_POINT('',(-6.82752391182554,-55.1067946037879,-94.3158809919512));
#136637=CARTESIAN_POINT('Ctrl Pts',(-1.23668874794468,-55.0504102916018,
-95.5762792512635));
#136638=CARTESIAN_POINT('Ctrl Pts',(-2.16407513351987,-55.0533526605647,
-95.5113527668491));
#136639=CARTESIAN_POINT('Ctrl Pts',(-3.10799502527407,-55.0597210848585,
-95.3707630380922));
#136640=CARTESIAN_POINT('Ctrl Pts',(-4.02669441069485,-55.0690422663978,
-95.16328981846));
#136641=CARTESIAN_POINT('Ctrl Pts',(-4.98118226589344,-55.0787265599944,
-94.9477343586866));
#136642=CARTESIAN_POINT('Ctrl Pts',(-5.91348766496874,-55.0915160415816,
-94.6617302601372));
#136643=CARTESIAN_POINT('Ctrl Pts',(-6.82752392642188,-55.1067946087991,
-94.3158810345077));
#136644=CARTESIAN_POINT('Ctrl Pts',(-1.24035792914739,-71.2481103336038,
-60.8508735991007));
#136645=CARTESIAN_POINT('Ctrl Pts',(-1.24033480878609,-71.1072117831156,
-61.1529641634137));
#136646=CARTESIAN_POINT('Ctrl Pts',(-1.24031152212174,-70.9663130484708,
-61.4550546418214));
#136647=CARTESIAN_POINT('Ctrl Pts',(-1.24019423907957,-70.2618184344542,
-62.9655065950025));
#136648=CARTESIAN_POINT('Ctrl Pts',(-1.2400976958218,-69.6982197351968,
-64.1738667543558));
#136649=CARTESIAN_POINT('Ctrl Pts',(-1.23999818500278,-69.1346177525067,
-65.3822253820002));
#136650=CARTESIAN_POINT('Ctrl Pts',(-1.23960014172664,-66.8802098214716,
-70.2156598931668));
#136651=CARTESIAN_POINT('Ctrl Pts',(-1.23915545083688,-64.6257502610154,
-75.0490703206921));
#136652=CARTESIAN_POINT('Ctrl Pts',(-1.23864216610312,-62.3712150282457,
-79.8824454429464));
#136653=CARTESIAN_POINT('Ctrl Pts',(-1.23808662039688,-59.9310540692955,
-85.1137734354556));
#136654=CARTESIAN_POINT('Ctrl Pts',(-1.23745196892516,-57.4908058054248,
-90.3450606997508));
#136655=CARTESIAN_POINT('Ctrl Pts',(-1.23668893165476,-55.0504165218147,
-95.5762821576554));
#136656=CARTESIAN_POINT('Ctrl Pts',(-6.82752390105444,-55.106794611208,
-94.3158809605474));
#136657=CARTESIAN_POINT('Ctrl Pts',(-6.83625690025051,-60.3715570323219,
-83.1679040708394));
#136658=CARTESIAN_POINT('Ctrl Pts',(-6.84206094040904,-65.61805576689,-72.0110063808198));
#136659=CARTESIAN_POINT('Ctrl Pts',(-6.84677576889373,-70.8578246683297,
-60.8508735991007));
#136660=CARTESIAN_POINT('Ctrl Pts',(-6.84141371258755,-70.9528017323285,
-60.42825533736));
#136661=CARTESIAN_POINT('Ctrl Pts',(-7.39999999999997,-70.886896756869,
-60.42825533736));
#136662=CARTESIAN_POINT('Ctrl Pts',(-7.4,-71.449357516634,-60.42825533736));
#136663=CARTESIAN_POINT('Ctrl Pts',(-6.84141371452047,-70.9528017321005,
-60.574175588166));
#136664=CARTESIAN_POINT('Ctrl Pts',(-7.39999999999996,-70.8868967471692,
-60.5644399462782));
#136665=CARTESIAN_POINT('Ctrl Pts',(-7.4,-71.4493574998816,-60.6471383113761));
#136666=CARTESIAN_POINT('Ctrl Pts',(-6.84320633698782,-70.9209010052172,
-60.7174412822399));
#136667=CARTESIAN_POINT('Ctrl Pts',(-7.39999999999997,-70.85979500338,-60.6978441698658));
#136668=CARTESIAN_POINT('Ctrl Pts',(-7.4,-71.4018249198588,-60.8620307958147));
#136669=CARTESIAN_POINT('Ctrl Pts',(-6.84677576889373,-70.8578246683297,
-60.8508735991007));
#136670=CARTESIAN_POINT('Ctrl Pts',(-7.39999999999996,-70.8042142666047,
-60.8257004209668));
#136671=CARTESIAN_POINT('Ctrl Pts',(-7.4,-71.3078420373655,-61.0621827299711));
#136672=CARTESIAN_POINT('',(-7.4,-71.3078420373655,-61.0621827299711));
#136673=CARTESIAN_POINT('Origin',(-6.9,-71.3078420373655,-61.0621827299711));
#136674=CARTESIAN_POINT('Origin',(-7.4,-69.2744516168521,-60.2813964156253));
#136675=CARTESIAN_POINT('Origin',(-7.4,67.7009572055632,-55.24995));
#136676=CARTESIAN_POINT('',(-7.4,-72.58000002,-58.1594740865074));
#136677=CARTESIAN_POINT('Ctrl Pts',(-7.4,-72.58000002,-58.1594740865074));
#136678=CARTESIAN_POINT('Ctrl Pts',(-7.4,-72.58000002,-58.0551776270551));
#136679=CARTESIAN_POINT('Ctrl Pts',(-7.4,-72.5736287847411,-57.9519715312753));
#136680=CARTESIAN_POINT('Ctrl Pts',(-7.4,-72.5609286762394,-57.8498358231105));
#136681=CARTESIAN_POINT('Ctrl Pts',(-7.4,-72.5482285677376,-57.7477001149457));
#136682=CARTESIAN_POINT('Ctrl Pts',(-7.39999999935597,-72.529198463361,
-57.6466357793308));
#136683=CARTESIAN_POINT('Ctrl Pts',(-7.40000000064314,-72.5039045953935,
-57.5466462680235));
#136684=CARTESIAN_POINT('Ctrl Pts',(-7.40000000122792,-72.4924131270627,
-57.5012191983453));
#136685=CARTESIAN_POINT('Ctrl Pts',(-7.40000000179748,-72.4796171505751,
-57.4560136230692));
#136686=CARTESIAN_POINT('Ctrl Pts',(-7.40000000193861,-72.4655224562879,
-57.4110306599075));
#136687=CARTESIAN_POINT('Ctrl Pts',(-7.40000000231984,-72.4274510918893,
-57.2895265855827));
#136688=CARTESIAN_POINT('Ctrl Pts',(-7.4000000004226,-72.3798384459848,
-57.1705512406855));
#136689=CARTESIAN_POINT('Ctrl Pts',(-7.40000000013593,-72.3241837880397,
-57.0571398660674));
#136690=CARTESIAN_POINT('Ctrl Pts',(-7.40000000006153,-72.3097383663643,
-57.0277034237349));
#136691=CARTESIAN_POINT('Ctrl Pts',(-7.40000000003645,-72.2947325387355,
-56.9985778271777));
#136692=CARTESIAN_POINT('Ctrl Pts',(-7.40000000002765,-72.279165204543,
-56.9697637092871));
#136693=CARTESIAN_POINT('Ctrl Pts',(-7.40000000000257,-72.2347715487634,
-56.8875939546328));
#136694=CARTESIAN_POINT('Ctrl Pts',(-7.40000000007907,-72.1857795264399,
-56.8079051030792));
#136695=CARTESIAN_POINT('Ctrl Pts',(-7.40000000044821,-72.1321711779398,
-56.7307944085666));
#136696=CARTESIAN_POINT('Ctrl Pts',(-7.40000000085049,-72.0737492661558,
-56.6467598445767));
#136697=CARTESIAN_POINT('Ctrl Pts',(-7.40000000144702,-72.0094938737877,
-56.565563603203));
#136698=CARTESIAN_POINT('Ctrl Pts',(-7.40000000089367,-71.9411026567194,
-56.4892360541678));
#136699=CARTESIAN_POINT('Ctrl Pts',(-7.40000000083676,-71.9340690507491,
-56.481386246435));
#136700=CARTESIAN_POINT('Ctrl Pts',(-7.40000000077119,-71.926991725805,
-56.4735878952515));
#136701=CARTESIAN_POINT('Ctrl Pts',(-7.4000000007,-71.9198725431757,-56.465843179204));
#136702=CARTESIAN_POINT('Ctrl Pts',(-7.40000000060499,-71.9103706657815,
-56.4555064107617));
#136703=CARTESIAN_POINT('Ctrl Pts',(-7.40000000052617,-71.9007927917902,
-56.4452629042245));
#136704=CARTESIAN_POINT('Ctrl Pts',(-7.40000000046129,-71.8911429761284,
-56.4351175107121));
#136705=CARTESIAN_POINT('Ctrl Pts',(-7.39999999996768,-71.8177272070187,
-56.3579313867758));
#136706=CARTESIAN_POINT('Ctrl Pts',(-7.39999999939412,-71.7397944141598,
-56.2857954012954));
#136707=CARTESIAN_POINT('Ctrl Pts',(-7.40000000114364,-71.6572752456072,
-56.2186315211966));
#136708=CARTESIAN_POINT('Ctrl Pts',(-7.40000000147217,-71.641779599927,
-56.2060193280932));
#136709=CARTESIAN_POINT('Ctrl Pts',(-7.40000000193345,-71.6261221119207,
-56.1935825531791));
#136710=CARTESIAN_POINT('Ctrl Pts',(-7.40000000264863,-71.6103021593138,
-56.1813208069962));
#136711=CARTESIAN_POINT('Ctrl Pts',(-7.40000000499281,-71.558447829008,
-56.1411294959033));
#136712=CARTESIAN_POINT('Ctrl Pts',(-7.40000000927177,-71.5046891439978,
-56.1028356287387));
#136713=CARTESIAN_POINT('Ctrl Pts',(-7.40000002552836,-71.4493575166296,
-56.0666111687568));
#136714=CARTESIAN_POINT('',(-7.4,-72.58000002,-174.471034982976));
#136715=CARTESIAN_POINT('',(-7.4,-72.58000002,-58.1419820049528));
#136716=CARTESIAN_POINT('Ctrl Pts',(-7.40000000575672,-71.5626363369612,
-176.485569595296));
#136717=CARTESIAN_POINT('Ctrl Pts',(-7.39999999964314,-71.5963334703268,
-176.460729295267));
#136718=CARTESIAN_POINT('Ctrl Pts',(-7.40000000050213,-71.6293602055438,
-176.435105116127));
#136719=CARTESIAN_POINT('Ctrl Pts',(-7.40000000080687,-71.6616524595397,
-176.408710325206));
#136720=CARTESIAN_POINT('Ctrl Pts',(-7.40000000085713,-71.6669782225453,
-176.404357194544));
#136721=CARTESIAN_POINT('Ctrl Pts',(-7.40000000093686,-71.6722864874059,
-176.399982537289));
#136722=CARTESIAN_POINT('Ctrl Pts',(-7.40000000105475,-71.6775773354997,
-176.395586157876));
#136723=CARTESIAN_POINT('Ctrl Pts',(-7.40000000288459,-71.7597041196625,
-176.327343695267));
#136724=CARTESIAN_POINT('Ctrl Pts',(-7.40000000086288,-71.8372393620123,
-176.253983607122));
#136725=CARTESIAN_POINT('Ctrl Pts',(-7.40000000055521,-71.9102228395748,
-176.175469994329));
#136726=CARTESIAN_POINT('Ctrl Pts',(-7.40000000052935,-71.916356742894,
-176.168871310268));
#136727=CARTESIAN_POINT('Ctrl Pts',(-7.40000000051231,-71.9224585008182,
-176.162236193811));
#136728=CARTESIAN_POINT('Ctrl Pts',(-7.40000000050508,-71.9285281400417,
-176.15556460665));
#136729=CARTESIAN_POINT('Ctrl Pts',(-7.40000000048088,-71.9488281698803,
-176.133251349886));
#136730=CARTESIAN_POINT('Ctrl Pts',(-7.4000000005302,-71.9687792955913,
-176.110498872159));
#136731=CARTESIAN_POINT('Ctrl Pts',(-7.40000000090086,-71.9883433756989,
-176.087359845977));
#136732=CARTESIAN_POINT('Ctrl Pts',(-7.40000000204431,-72.0486965657351,
-176.01597831223));
#136733=CARTESIAN_POINT('Ctrl Pts',(-7.40000000174205,-72.1052822109679,
-175.940916275219));
#136734=CARTESIAN_POINT('Ctrl Pts',(-7.40000000104438,-72.1569369843104,
-175.863739490819));
#136735=CARTESIAN_POINT('Ctrl Pts',(-7.40000000027758,-72.2137093550038,
-175.778916564894));
#136736=CARTESIAN_POINT('Ctrl Pts',(-7.39999999999849,-72.2650200455803,
-175.691076839899));
#136737=CARTESIAN_POINT('Ctrl Pts',(-7.40000000003311,-72.3109220293856,
-175.600232860702));
#136738=CARTESIAN_POINT('Ctrl Pts',(-7.4000000000402,-72.3203292671906,
-175.5816151269));
#136739=CARTESIAN_POINT('Ctrl Pts',(-7.40000000005342,-72.3295088745487,
-175.562871130851));
#136740=CARTESIAN_POINT('Ctrl Pts',(-7.40000000007737,-72.3384609015072,
-175.544000911756));
#136741=CARTESIAN_POINT('Ctrl Pts',(-7.40000000021819,-72.3910932309574,
-175.433055804823));
#136742=CARTESIAN_POINT('Ctrl Pts',(-7.4000000012263,-72.436127459958,-175.316747505601));
#136743=CARTESIAN_POINT('Ctrl Pts',(-7.40000000110901,-72.4720179137164,
-175.198544593051));
#136744=CARTESIAN_POINT('Ctrl Pts',(-7.40000000106035,-72.4869106518372,
-175.14949631315));
#136745=CARTESIAN_POINT('Ctrl Pts',(-7.40000000071105,-72.5002693294562,
-175.100185099317));
#136746=CARTESIAN_POINT('Ctrl Pts',(-7.4000000003472,-72.5120857612517,
-175.050611983827));
#136747=CARTESIAN_POINT('Ctrl Pts',(-7.39999999965227,-72.534654114155,
-174.955931662031));
#136748=CARTESIAN_POINT('Ctrl Pts',(-7.4,-72.5516373021817,-174.860293425931));
#136749=CARTESIAN_POINT('Ctrl Pts',(-7.4,-72.5629735391251,-174.763699740561));
#136750=CARTESIAN_POINT('Ctrl Pts',(-7.4,-72.5743097760684,-174.667106055192));
#136751=CARTESIAN_POINT('Ctrl Pts',(-7.4,-72.58000002,-174.569557605373));
#136752=CARTESIAN_POINT('Ctrl Pts',(-7.4,-72.58000002,-174.471034982976));
#136753=CARTESIAN_POINT('',(-7.4,-71.4211246238516,-171.237717270032));
#136754=CARTESIAN_POINT('Origin',(-7.4,-69.3873379576789,-172.017654079519));
#136755=CARTESIAN_POINT('',(-7.4,-55.5541151520872,-137.531452880088));
#136756=CARTESIAN_POINT('Ctrl Pts',(-7.4,-55.5541151520872,-137.531452880088));
#136757=CARTESIAN_POINT('Ctrl Pts',(-7.4,-60.858236996045,-148.759754479668));
#136758=CARTESIAN_POINT('Ctrl Pts',(-7.4,-66.1431501582269,-159.997106821727));
#136759=CARTESIAN_POINT('Ctrl Pts',(-7.4,-71.4211246238516,-171.237717270032));
#136760=CARTESIAN_POINT('',(-7.4,-55.08000002,-135.415380765739));
#136761=CARTESIAN_POINT('Ctrl Pts',(-7.4,-55.08000002,-135.415380765739));
#136762=CARTESIAN_POINT('Ctrl Pts',(-7.4,-55.08000002,-135.642528198476));
#136763=CARTESIAN_POINT('Ctrl Pts',(-7.4,-55.0958102967125,-135.869567477787));
#136764=CARTESIAN_POINT('Ctrl Pts',(-7.4,-55.1266901212419,-136.093433076237));
#136765=CARTESIAN_POINT('Ctrl Pts',(-7.4,-55.1457148268974,-136.231354103373));
#136766=CARTESIAN_POINT('Ctrl Pts',(-7.4,-55.170458313014,-136.368070310456));
#136767=CARTESIAN_POINT('Ctrl Pts',(-7.4,-55.2007376448274,-136.502866089854));
#136768=CARTESIAN_POINT('Ctrl Pts',(-7.4,-55.2691608068266,-136.807468367981));
#136769=CARTESIAN_POINT('Ctrl Pts',(-7.4,-55.3655723350956,-137.104245532218));
#136770=CARTESIAN_POINT('Ctrl Pts',(-7.4,-55.4912205286389,-137.392848584318));
#136771=CARTESIAN_POINT('Ctrl Pts',(-7.4,-55.511427368581,-137.439261951006));
#136772=CARTESIAN_POINT('Ctrl Pts',(-7.4,-55.5323904712551,-137.485463878382));
#136773=CARTESIAN_POINT('Ctrl Pts',(-7.4,-55.5541151520872,-137.531452880088));
#136774=CARTESIAN_POINT('',(-7.4,-55.08000002,-96.6432622057672));
#136775=CARTESIAN_POINT('',(-7.4,-55.08000002,-135.57795249279));
#136776=CARTESIAN_POINT('',(-7.4,-55.5541151520872,-94.5271900914178));
#136777=CARTESIAN_POINT('Ctrl Pts',(-7.4,-55.5541151520872,-94.5271900914178));
#136778=CARTESIAN_POINT('Ctrl Pts',(-7.4,-55.4646684466484,-94.7165399244892));
#136779=CARTESIAN_POINT('Ctrl Pts',(-7.4,-55.3874966670382,-94.9115657139063));
#136780=CARTESIAN_POINT('Ctrl Pts',(-7.4,-55.3230550301945,-95.1098279145052));
#136781=CARTESIAN_POINT('Ctrl Pts',(-7.4,-55.2745243397284,-95.2591382355908));
#136782=CARTESIAN_POINT('Ctrl Pts',(-7.4,-55.2332126733285,-95.410283167727));
#136783=CARTESIAN_POINT('Ctrl Pts',(-7.4,-55.199296044664,-95.5622145003849));
#136784=CARTESIAN_POINT('Ctrl Pts',(-7.4,-55.1306219000049,-95.8698439649878));
#136785=CARTESIAN_POINT('Ctrl Pts',(-7.4,-55.0911602505268,-96.1824496093173));
#136786=CARTESIAN_POINT('Ctrl Pts',(-7.4,-55.0820478268083,-96.500225074923));
#136787=CARTESIAN_POINT('Ctrl Pts',(-7.4,-55.0806839263472,-96.5477880633723));
#136788=CARTESIAN_POINT('Ctrl Pts',(-7.4,-55.08000002,-96.595466884908));
#136789=CARTESIAN_POINT('Ctrl Pts',(-7.4,-55.08000002,-96.6432622057672));
#136790=CARTESIAN_POINT('Ctrl Pts',(-7.4,-71.3078420373655,-61.0621827299711));
#136791=CARTESIAN_POINT('Ctrl Pts',(-7.4,-66.0675133276181,-72.2223201517098));
#136792=CARTESIAN_POINT('Ctrl Pts',(-7.4,-60.8202894597531,-83.3792196747323));
#136793=CARTESIAN_POINT('Ctrl Pts',(-7.4,-55.5541151520872,-94.5271900914177));
#136794=CARTESIAN_POINT('Ctrl Pts',(-7.4,-72.58000002,-58.1594740865074));
#136795=CARTESIAN_POINT('Ctrl Pts',(-7.39999999999995,-73.0800000199999,
-58.1594740865073));
#136796=CARTESIAN_POINT('Ctrl Pts',(-7.9,-73.08000002,-58.1594740865074));
#136797=CARTESIAN_POINT('Ctrl Pts',(-7.4,-72.5800000130548,-57.9035537157173));
#136798=CARTESIAN_POINT('Ctrl Pts',(-7.39999999999997,-73.0817635435305,
-57.8518911502671));
#136799=CARTESIAN_POINT('Ctrl Pts',(-7.9017604405896,-73.08000002,-57.8524302618023));
#136800=CARTESIAN_POINT('Ctrl Pts',(-7.4,-72.5416326919704,-57.6540534055839));
#136801=CARTESIAN_POINT('Ctrl Pts',(-7.39999999999995,-73.0373043377172,
-57.5520537815894));
#136802=CARTESIAN_POINT('Ctrl Pts',(-7.90348019558611,-73.0339592231946,
-57.5530891712348));
#136803=CARTESIAN_POINT('Ctrl Pts',(-7.4,-72.42740431593,-57.2895390365225));
#136804=CARTESIAN_POINT('Ctrl Pts',(-7.39999999999995,-72.9025581822962,
-57.1135670536862));
#136805=CARTESIAN_POINT('Ctrl Pts',(-7.90599716341333,-72.896885176701,
-57.1157587646024));
#136806=CARTESIAN_POINT('Ctrl Pts',(-7.4,-72.3798159344887,-57.1705597381646));
#136807=CARTESIAN_POINT('Ctrl Pts',(-7.39999999999996,-72.846103402619,
-56.9702086770063));
#136808=CARTESIAN_POINT('Ctrl Pts',(-7.90681948691283,-72.8397791179241,
-56.9730119912525));
#136809=CARTESIAN_POINT('Ctrl Pts',(-7.4,-72.2685307073729,-56.9437302645456));
#136810=CARTESIAN_POINT('Ctrl Pts',(-7.39999999999997,-72.7136696095191,
-56.6966550709085));
#136811=CARTESIAN_POINT('Ctrl Pts',(-7.9083884819823,-72.7062368443098,
-56.70087080336));
#136812=CARTESIAN_POINT('Ctrl Pts',(-7.4,-72.2045576741781,-56.8349322106875));
#136813=CARTESIAN_POINT('Ctrl Pts',(-7.40000000000002,-72.6373398680779,
-56.5653507289509));
#136814=CARTESIAN_POINT('Ctrl Pts',(-7.90914169806791,-72.6294692039913,
-56.5703391604345));
#136815=CARTESIAN_POINT('Ctrl Pts',(-7.4,-72.0597499182548,-56.6266807792285));
#136816=CARTESIAN_POINT('Ctrl Pts',(-7.39999999999991,-72.4642201336178,
-56.3138046122562));
#136817=CARTESIAN_POINT('Ctrl Pts',(-7.91058447423394,-72.4556998989282,
-56.3204873030743));
#136818=CARTESIAN_POINT('Ctrl Pts',(-7.4,-71.9783757021874,-56.5268811589555));
#136819=CARTESIAN_POINT('Ctrl Pts',(-7.39999999999996,-72.366765643856,
-56.1931795440353));
#136820=CARTESIAN_POINT('Ctrl Pts',(-7.91127644455456,-72.3580508393546,
-56.2007516828216));
#136821=CARTESIAN_POINT('Ctrl Pts',(-7.4,-71.8038791222482,-56.3433834633767));
#136822=CARTESIAN_POINT('Ctrl Pts',(-7.39999999999996,-72.1574857101496,
-55.9712111947932));
#136823=CARTESIAN_POINT('Ctrl Pts',(-7.91254952666346,-72.1486549419682,
-55.9805984788111));
#136824=CARTESIAN_POINT('Ctrl Pts',(-7.4,-71.710253472938,-56.2588007503857));
#136825=CARTESIAN_POINT('Ctrl Pts',(-7.39999999999963,-72.0450577059424,
-55.8688410357779));
#136826=CARTESIAN_POINT('Ctrl Pts',(-7.91313676360239,-72.0363041630141,
-55.879119540041));
#136827=CARTESIAN_POINT('Ctrl Pts',(-7.4,-71.4103049905956,-56.0264829839341));
#136828=CARTESIAN_POINT('Ctrl Pts',(-7.40000000000062,-71.6842770741658,
-55.5873067274671));
#136829=CARTESIAN_POINT('Ctrl Pts',(-7.9147504864484,-71.6763659857377,
-55.6003940631938));
#136830=CARTESIAN_POINT('Ctrl Pts',(-7.4,-71.1825473819866,-55.9004387386915));
#136831=CARTESIAN_POINT('Ctrl Pts',(-7.39999999999996,-71.4100611802463,
-55.4345719679896));
#136832=CARTESIAN_POINT('Ctrl Pts',(-7.91562717321909,-71.4030569333749,
-55.449171357324));
#136833=CARTESIAN_POINT('Ctrl Pts',(-7.4,-70.9475727253686,-55.8134402200258));
#136834=CARTESIAN_POINT('Ctrl Pts',(-7.39999999999996,-71.1269094387434,
-55.3290689454198));
#136835=CARTESIAN_POINT('Ctrl Pts',(-7.91623251645313,-71.1210872664424,
-55.3447940747887));
#136836=CARTESIAN_POINT('',(-7.9,-73.08000002,-58.1594740865074));
#136837=CARTESIAN_POINT('Ctrl Pts',(-7.91618843693208,-71.1413940909408,
-55.3523946663949));
#136838=CARTESIAN_POINT('Ctrl Pts',(-7.91558486059001,-71.4161690172318,
-55.4564569226562));
#136839=CARTESIAN_POINT('Ctrl Pts',(-7.91472456568273,-71.6821304827593,
-55.6048579163084));
#136840=CARTESIAN_POINT('Ctrl Pts',(-7.91313668710487,-72.036304164319,
-55.8791195385087));
#136841=CARTESIAN_POINT('Ctrl Pts',(-7.91254945020742,-72.1486549432855,
-55.9805984774108));
#136842=CARTESIAN_POINT('Ctrl Pts',(-7.91127636818889,-72.3580508406563,
-56.2007516816906));
#136843=CARTESIAN_POINT('Ctrl Pts',(-7.91058439791765,-72.4556999002017,
-56.3204873020754));
#136844=CARTESIAN_POINT('Ctrl Pts',(-7.90914162185518,-72.6294692051695,
-56.5703391596878));
#136845=CARTESIAN_POINT('Ctrl Pts',(-7.90838840582395,-72.7062368454232,
-56.7008708027285));
#136846=CARTESIAN_POINT('Ctrl Pts',(-7.90681941086846,-72.839779118873,
-56.9730119908319));
#136847=CARTESIAN_POINT('Ctrl Pts',(-7.90599708742908,-72.8968851775529,
-57.1157587642733));
#136848=CARTESIAN_POINT('Ctrl Pts',(-7.90348011978738,-73.0339592236982,
-57.5530891710789));
#136849=CARTESIAN_POINT('Ctrl Pts',(-7.90176036491906,-73.0800000202659,
-57.852430261721));
#136850=CARTESIAN_POINT('Ctrl Pts',(-7.9,-73.08000002,-58.1594740865074));
#136851=CARTESIAN_POINT('Origin',(-7.9,-72.58000002,-58.1594740865074));
#136852=CARTESIAN_POINT('Ctrl Pts',(-7.91297989639778,-71.1218111846181,
-55.3449495350315));
#136853=CARTESIAN_POINT('Ctrl Pts',(-7.88787222497776,-73.08000002,-56.0696654600803));
#136854=CARTESIAN_POINT('Ctrl Pts',(-7.81557216061084,-73.08000002,-58.1565578346149));
#136855=CARTESIAN_POINT('Ctrl Pts',(-8.10803398103311,-71.097847913879,
-55.3428278238724));
#136856=CARTESIAN_POINT('Ctrl Pts',(-8.08415144386284,-73.08000002,-56.0574351382547));
#136857=CARTESIAN_POINT('Ctrl Pts',(-8.01154341310344,-73.08000002,-58.1633472285775));
#136858=CARTESIAN_POINT('Ctrl Pts',(-8.30261637240508,-71.0730051020417,
-55.3405756034006));
#136859=CARTESIAN_POINT('Ctrl Pts',(-8.27957773898596,-73.0800000199964,
-56.044305254623));
#136860=CARTESIAN_POINT('Ctrl Pts',(-8.20751459242944,-73.08000002,-58.1699994619964));
#136861=CARTESIAN_POINT('Ctrl Pts',(-8.49667612019033,-71.047290072049,
-55.338183503385));
#136862=CARTESIAN_POINT('Ctrl Pts',(-8.47395476319521,-73.08000002,-56.030195271658));
#136863=CARTESIAN_POINT('Ctrl Pts',(-8.40348565122521,-73.08000002,-58.176433931325));
#136864=CARTESIAN_POINT('',(-8.4,-73.08000002,-58.1763194612681));
#136865=CARTESIAN_POINT('Ctrl Pts',(-8.4,-73.08000002,-58.1763194612681));
#136866=CARTESIAN_POINT('Ctrl Pts',(-8.40172135040051,-73.08000002,-57.8616056776356));
#136867=CARTESIAN_POINT('Ctrl Pts',(-8.40340362484077,-73.0316819589995,
-57.5549684855522));
#136868=CARTESIAN_POINT('Ctrl Pts',(-8.40668695336401,-72.8395715451724,
-56.9580994114807));
#136869=CARTESIAN_POINT('Ctrl Pts',(-8.40822820346396,-72.6984881279278,
-56.6787458682451));
#136870=CARTESIAN_POINT('Ctrl Pts',(-8.41033280652841,-72.4250329770282,
-56.2980850295082));
#136871=CARTESIAN_POINT('Ctrl Pts',(-8.41100144942456,-72.322979355276,
-56.1772949390326));
#136872=CARTESIAN_POINT('Ctrl Pts',(-8.41222718544652,-72.1044079319076,
-55.9560708595913));
#136873=CARTESIAN_POINT('Ctrl Pts',(-8.41279083164671,-71.9871179192065,
-55.8544512596825));
#136874=CARTESIAN_POINT('Ctrl Pts',(-8.41427813867351,-71.6242920428588,
-55.5865039897334));
#136875=CARTESIAN_POINT('Ctrl Pts',(-8.41506374698045,-71.3572532546422,
-55.4452391148706));
#136876=CARTESIAN_POINT('Ctrl Pts',(-8.41560835021378,-71.0814043774777,
-55.3473655916165));
#136877=CARTESIAN_POINT('Ctrl Pts',(-8.4,-73.08000002,-58.1763194612681));
#136878=CARTESIAN_POINT('Ctrl Pts',(-8.23332974561635,-73.08000002,-58.1708448514923));
#136879=CARTESIAN_POINT('Ctrl Pts',(-8.06666350196851,-73.08000002,-58.1652131587787));
#136880=CARTESIAN_POINT('Ctrl Pts',(-7.9,-73.08000002,-58.1594740865074));
#136881=CARTESIAN_POINT('Ctrl Pts',(-8.4,-73.08000002,-58.1763194612681));
#136882=CARTESIAN_POINT('Ctrl Pts',(-8.89999999999996,-73.0800000199999,
-58.1763194612681));
#136883=CARTESIAN_POINT('Ctrl Pts',(-8.9,-72.58000002,-58.1763194612681));
#136884=CARTESIAN_POINT('Ctrl Pts',(-8.40172135040051,-73.08000002,-57.8616056776356));
#136885=CARTESIAN_POINT('Ctrl Pts',(-8.89999999999996,-73.0782816065607,
-57.8621442504892));
#136886=CARTESIAN_POINT('Ctrl Pts',(-8.9,-72.5800000128814,-57.9140108579591));
#136887=CARTESIAN_POINT('Ctrl Pts',(-8.40340362484077,-73.0316819589995,
-57.5549684855522));
#136888=CARTESIAN_POINT('Ctrl Pts',(-8.89999999999997,-73.0284577192567,
-57.5559934180811));
#136889=CARTESIAN_POINT('Ctrl Pts',(-8.9,-72.5397349720259,-57.6584337450815));
#136890=CARTESIAN_POINT('Ctrl Pts',(-8.40668695336401,-72.8395715451724,
-56.9580994114807));
#136891=CARTESIAN_POINT('Ctrl Pts',(-8.89999999999997,-72.8336034512039,
-56.9611013895289));
#136892=CARTESIAN_POINT('Ctrl Pts',(-8.9,-72.3796429547841,-57.1609527205255));
#136893=CARTESIAN_POINT('Ctrl Pts',(-8.40822820346396,-72.6984881279278,
-56.6787458682451));
#136894=CARTESIAN_POINT('Ctrl Pts',(-8.89999999999995,-72.6915892789857,
-56.6830185073362));
#136895=CARTESIAN_POINT('Ctrl Pts',(-8.9,-72.262073445265,-56.9281157265161));
#136896=CARTESIAN_POINT('Ctrl Pts',(-8.41033280652841,-72.4250329770282,
-56.2980850295082));
#136897=CARTESIAN_POINT('Ctrl Pts',(-8.89999999999996,-72.4171612181699,
-56.3044762227344));
#136898=CARTESIAN_POINT('Ctrl Pts',(-8.9,-72.0341941498609,-56.6108404408522));
#136899=CARTESIAN_POINT('Ctrl Pts',(-8.41100144942456,-72.322979355276,
-56.1772949390326));
#136900=CARTESIAN_POINT('Ctrl Pts',(-8.9000000000003,-72.3149747479787,
-56.1845060329552));
#136901=CARTESIAN_POINT('Ctrl Pts',(-8.9,-71.9491494655935,-56.5101636182542));
#136902=CARTESIAN_POINT('Ctrl Pts',(-8.41222718544652,-72.1044079319076,
-55.9560708595913));
#136903=CARTESIAN_POINT('Ctrl Pts',(-8.89999999999963,-72.0963975739119,
-55.9649406347444));
#136904=CARTESIAN_POINT('Ctrl Pts',(-8.9,-71.7670066137261,-56.3257764465383));
#136905=CARTESIAN_POINT('Ctrl Pts',(-8.41279083164671,-71.9871179192065,
-55.8544512596825));
#136906=CARTESIAN_POINT('Ctrl Pts',(-8.89999999999951,-71.9792314944188,
-55.8641264120645));
#136907=CARTESIAN_POINT('Ctrl Pts',(-8.9,-71.6692649365715,-56.2410779083558));
#136908=CARTESIAN_POINT('Ctrl Pts',(-8.41433230457371,-71.6110783688472,
-55.5767456783554));
#136909=CARTESIAN_POINT('Ctrl Pts',(-8.90000000000086,-71.6041352856071,
-55.588933048404));
#136910=CARTESIAN_POINT('Ctrl Pts',(-8.9,-71.3558986429072,-56.0096140831459));
#136911=CARTESIAN_POINT('Ctrl Pts',(-8.41515058995443,-71.3274449382984,
-55.429624391176));
#136912=CARTESIAN_POINT('Ctrl Pts',(-8.89999999999818,-71.3214288330036,
-55.443108937543));
#136913=CARTESIAN_POINT('Ctrl Pts',(-8.9,-71.1195373961099,-55.8869904035305));
#136914=CARTESIAN_POINT('Ctrl Pts',(-8.41569693570581,-71.0352755960629,
-55.3314460318215));
#136915=CARTESIAN_POINT('Ctrl Pts',(-8.89999999999995,-71.0304294360218,
-55.3458650785795));
#136916=CARTESIAN_POINT('Ctrl Pts',(-8.9,-70.8760630000525,-55.8051600336001));
#136917=CARTESIAN_POINT('',(-8.9,-72.58000002,-58.1763194612681));
#136918=CARTESIAN_POINT('Ctrl Pts',(-8.89999996628377,-71.0999148696861,
-55.8925850873112));
#136919=CARTESIAN_POINT('Ctrl Pts',(-8.89999995709263,-71.1271912455156,
-55.9047800168435));
#136920=CARTESIAN_POINT('Ctrl Pts',(-8.89999995405378,-71.1542893399126,
-55.9174976277302));
#136921=CARTESIAN_POINT('Ctrl Pts',(-8.89999995711454,-71.1811814737311,
-55.9307199810309));
#136922=CARTESIAN_POINT('Ctrl Pts',(-8.89999996594249,-71.2587447432665,
-55.9688563728797));
#136923=CARTESIAN_POINT('Ctrl Pts',(-8.89999997989509,-71.3347385769612,
-56.0111644614659));
#136924=CARTESIAN_POINT('Ctrl Pts',(-8.89999998822403,-71.4082909897931,
-56.0572656901905));
#136925=CARTESIAN_POINT('Ctrl Pts',(-8.89999999429182,-71.4618752880513,
-56.0908512911917));
#136926=CARTESIAN_POINT('Ctrl Pts',(-8.89999999762151,-71.5141639062437,
-56.1264488763503));
#136927=CARTESIAN_POINT('Ctrl Pts',(-8.89999999894661,-71.5648287885728,
-56.1638971934456));
#136928=CARTESIAN_POINT('Ctrl Pts',(-8.90000000021706,-71.6134037334432,
-56.1998007592839));
#136929=CARTESIAN_POINT('Ctrl Pts',(-8.9,-71.6605183672425,-56.2373236964706));
#136930=CARTESIAN_POINT('Ctrl Pts',(-8.9,-71.7061534805117,-56.276424902386));
#136931=CARTESIAN_POINT('Ctrl Pts',(-8.9,-71.7586958576709,-56.3214444095464));
#136932=CARTESIAN_POINT('Ctrl Pts',(-8.90000000000525,-71.8093442969672,
-56.3686312342462));
#136933=CARTESIAN_POINT('Ctrl Pts',(-8.89999999994877,-71.8580831316161,
-56.4179650024181));
#136934=CARTESIAN_POINT('Ctrl Pts',(-8.89999999986101,-71.9338178277776,
-56.4946241587137));
#136935=CARTESIAN_POINT('Ctrl Pts',(-8.89999999955086,-72.0053843762033,
-56.5771518376495));
#136936=CARTESIAN_POINT('Ctrl Pts',(-8.89999999953632,-72.0709679837644,
-56.6635131964772));
#136937=CARTESIAN_POINT('Ctrl Pts',(-8.89999999953336,-72.084287167389,
-56.6810520730208));
#136938=CARTESIAN_POINT('Ctrl Pts',(-8.89999999954423,-72.0973597365665,
-56.6987489820051));
#136939=CARTESIAN_POINT('Ctrl Pts',(-8.89999999957055,-72.1101707466964,
-56.7165867802331));
#136940=CARTESIAN_POINT('Ctrl Pts',(-8.89999999961887,-72.1337005884472,
-56.7493492685329));
#136941=CARTESIAN_POINT('Ctrl Pts',(-8.89999999972697,-72.1563957720432,
-56.7826109127347));
#136942=CARTESIAN_POINT('Ctrl Pts',(-8.89999999983668,-72.1782434639423,
-56.8163461536645));
#136943=CARTESIAN_POINT('Ctrl Pts',(-8.90000000003969,-72.2186712712158,
-56.8787711377289));
#136944=CARTESIAN_POINT('Ctrl Pts',(-8.89999999999795,-72.2562052259131,
-56.9428012878323));
#136945=CARTESIAN_POINT('Ctrl Pts',(-8.89999999999952,-72.2908444043662,
-57.0084360093237));
#136946=CARTESIAN_POINT('Ctrl Pts',(-8.90000000000048,-72.311901730162,
-57.0483356771474));
#136947=CARTESIAN_POINT('Ctrl Pts',(-8.9,-72.3318884210689,-57.0888288165436));
#136948=CARTESIAN_POINT('Ctrl Pts',(-8.9,-72.3507957900478,-57.1299193914404));
#136949=CARTESIAN_POINT('Ctrl Pts',(-8.9,-72.3746230901592,-57.1817022418682));
#136950=CARTESIAN_POINT('Ctrl Pts',(-8.89999999998365,-72.3967864402965,
-57.2345342704724));
#136951=CARTESIAN_POINT('Ctrl Pts',(-8.89999999972024,-72.4171503424455,
-57.2881976322959));
#136952=CARTESIAN_POINT('Ctrl Pts',(-8.89999999952357,-72.4323543754486,
-57.3282636038495));
#136953=CARTESIAN_POINT('Ctrl Pts',(-8.89999999921991,-72.4465562092313,
-57.3687924002643));
#136954=CARTESIAN_POINT('Ctrl Pts',(-8.89999999918092,-72.4597162071225,
-57.4096844656319));
#136955=CARTESIAN_POINT('Ctrl Pts',(-8.89999999916252,-72.4659246935418,
-57.428976097332));
#136956=CARTESIAN_POINT('Ctrl Pts',(-8.89999999920802,-72.4718879323416,
-57.4482939264422));
#136957=CARTESIAN_POINT('Ctrl Pts',(-8.89999999932168,-72.4776042453442,
-57.4676297862024));
#136958=CARTESIAN_POINT('Ctrl Pts',(-8.90000000038933,-72.5312977767194,
-57.6492522047483));
#136959=CARTESIAN_POINT('Ctrl Pts',(-8.89999999999947,-72.5639591690306,
-57.834465787063));
#136960=CARTESIAN_POINT('Ctrl Pts',(-8.89999999999994,-72.5753897578134,
-58.0232925565627));
#136961=CARTESIAN_POINT('Ctrl Pts',(-8.90000000000006,-72.5784617700053,
-58.0740404357044));
#136962=CARTESIAN_POINT('Ctrl Pts',(-8.9,-72.58000002,-58.1250492743192));
#136963=CARTESIAN_POINT('Ctrl Pts',(-8.9,-72.58000002,-58.1763194612681));
#136964=CARTESIAN_POINT('Origin',(-8.4,-72.58000002,-58.1763194612681));
#136965=CARTESIAN_POINT('Ctrl Pts',(-9.32900358361251,-70.4903946571405,
-60.8901185898343));
#136966=CARTESIAN_POINT('Ctrl Pts',(-8.89988778396231,-70.5448235085214,
-60.918842206156));
#136967=CARTESIAN_POINT('Ctrl Pts',(-8.90000001675659,-70.9282729174771,
-61.1211126854556));
#136968=CARTESIAN_POINT('Ctrl Pts',(-9.32267960676823,-70.5733355012344,
-60.7345408641471));
#136969=CARTESIAN_POINT('Ctrl Pts',(-8.89989004681883,-70.6365947859941,
-60.7567344379852));
#136970=CARTESIAN_POINT('Ctrl Pts',(-8.90000001650961,-71.0511602413471,
-60.887714756578));
#136971=CARTESIAN_POINT('Ctrl Pts',(-9.31966069353146,-70.6132825269153,
-60.5618033393074));
#136972=CARTESIAN_POINT('Ctrl Pts',(-8.89989111303311,-70.682184857852,
-60.5709595618158));
#136973=CARTESIAN_POINT('Ctrl Pts',(-8.9000000163917,-71.1103503405761,
-60.6286014156989));
#136974=CARTESIAN_POINT('Ctrl Pts',(-9.32026185019719,-70.6053339699646,
-60.3838922942772));
#136975=CARTESIAN_POINT('Ctrl Pts',(-8.89989090319396,-70.6731622220975,
-60.380823819096));
#136976=CARTESIAN_POINT('Ctrl Pts',(-8.90000001641518,-71.0985729052349,
-60.3617033877878));
#136977=CARTESIAN_POINT('',(-8.9,-70.9575466375288,-61.0621827299711));
#136978=CARTESIAN_POINT('Origin',(-9.4,-70.9575466375288,-61.0621827299711));
#136979=CARTESIAN_POINT('Origin',(-8.89999938777026,-69.7158521499215,-60.4580628686544));
#136980=CARTESIAN_POINT('Origin',(-8.9,67.7009572055632,-55.24995));
#136981=CARTESIAN_POINT('',(-8.9,-72.58000002,-174.451268889151));
#136982=CARTESIAN_POINT('Ctrl Pts',(-8.9,-72.58000002,-174.451268889151));
#136983=CARTESIAN_POINT('Ctrl Pts',(-8.9,-72.58000002,-174.643662890522));
#136984=CARTESIAN_POINT('Ctrl Pts',(-8.90000000018189,-72.5583230934377,
-174.832372832512));
#136985=CARTESIAN_POINT('Ctrl Pts',(-8.89999999981754,-72.5152520259488,
-175.017431778767));
#136986=CARTESIAN_POINT('Ctrl Pts',(-8.89999999974365,-72.5065182587111,
-175.054957242055));
#136987=CARTESIAN_POINT('Ctrl Pts',(-8.89999999963418,-72.4969046367721,
-175.09233259596));
#136988=CARTESIAN_POINT('Ctrl Pts',(-8.89999999944856,-72.4864132528962,
-175.129558133433));
#136989=CARTESIAN_POINT('Ctrl Pts',(-8.89999999933697,-72.4801056624026,
-175.151938731556));
#136990=CARTESIAN_POINT('Ctrl Pts',(-8.89999999923514,-72.4734752856604,
-175.174281489137));
#136991=CARTESIAN_POINT('Ctrl Pts',(-8.8999999991621,-72.4665241218154,
-175.196577428232));
#136992=CARTESIAN_POINT('Ctrl Pts',(-8.89999999896656,-72.4479148757584,
-175.256266801974));
#136993=CARTESIAN_POINT('Ctrl Pts',(-8.89999999902277,-72.4269795805932,
-175.315421893863));
#136994=CARTESIAN_POINT('Ctrl Pts',(-8.89999999928889,-72.4039589917986,
-175.373505006315));
#136995=CARTESIAN_POINT('Ctrl Pts',(-8.89999999941373,-72.3931602367398,
-175.400751281813));
#136996=CARTESIAN_POINT('Ctrl Pts',(-8.8999999995758,-72.3819033245036,
-175.427761928544));
#136997=CARTESIAN_POINT('Ctrl Pts',(-8.899999999719,-72.3702165277834,-175.454483443826));
#136998=CARTESIAN_POINT('Ctrl Pts',(-8.89999999989012,-72.356250141463,
-175.486417173351));
#136999=CARTESIAN_POINT('Ctrl Pts',(-8.89999999994017,-72.3416346359546,
-175.518026103028));
#137000=CARTESIAN_POINT('Ctrl Pts',(-8.89999999996783,-72.3264029998066,
-175.549231269472));
#137001=CARTESIAN_POINT('Ctrl Pts',(-8.90000000003108,-72.2915692635033,
-175.620595404528));
#137002=CARTESIAN_POINT('Ctrl Pts',(-8.90000000000045,-72.2533993434512,
-175.690229109067));
#137003=CARTESIAN_POINT('Ctrl Pts',(-8.89999999999886,-72.2119321367876,
-175.757979856507));
#137004=CARTESIAN_POINT('Ctrl Pts',(-8.89999999999793,-72.1877543610133,
-175.797482454149));
#137005=CARTESIAN_POINT('Ctrl Pts',(-8.89999999999706,-72.1624481423419,
-175.836359594911));
#137006=CARTESIAN_POINT('Ctrl Pts',(-8.89999999999683,-72.1360090283531,
-175.874608824138));
#137007=CARTESIAN_POINT('Ctrl Pts',(-8.8999999999962,-72.0642253375692,
-175.978457646179));
#137008=CARTESIAN_POINT('Ctrl Pts',(-8.89999999999926,-71.9835064480419,
-176.078093573446));
#137009=CARTESIAN_POINT('Ctrl Pts',(-8.89999999999979,-71.8969230956058,
-176.169773703533));
#137010=CARTESIAN_POINT('Ctrl Pts',(-8.90000000000003,-71.8581752387953,
-176.210802474689));
#137011=CARTESIAN_POINT('Ctrl Pts',(-8.9,-71.8181601276395,-176.250407223135));
#137012=CARTESIAN_POINT('Ctrl Pts',(-8.9,-71.7768804944358,-176.288591148433));
#137013=CARTESIAN_POINT('Ctrl Pts',(-8.9,-71.7350069729775,-176.327324424174));
#137014=CARTESIAN_POINT('Ctrl Pts',(-8.9,-71.6916833325441,-176.364727207912));
#137015=CARTESIAN_POINT('Ctrl Pts',(-8.9,-71.6470438920773,-176.40066126947));
#137016=CARTESIAN_POINT('Ctrl Pts',(-8.9,-71.6374948625339,-176.408348091075));
#137017=CARTESIAN_POINT('Ctrl Pts',(-8.9,-71.6278871345229,-176.415966736531));
#137018=CARTESIAN_POINT('Ctrl Pts',(-8.9,-71.6182220181434,-176.423516347907));
#137019=CARTESIAN_POINT('Ctrl Pts',(-8.9,-71.5940005454252,-176.442436213824));
#137020=CARTESIAN_POINT('Ctrl Pts',(-8.9,-71.5693801206575,-176.460921216669));
#137021=CARTESIAN_POINT('Ctrl Pts',(-8.9,-71.5444197215458,-176.478940580039));
#137022=CARTESIAN_POINT('Ctrl Pts',(-8.9,-71.4920391665984,-176.516755049627));
#137023=CARTESIAN_POINT('Ctrl Pts',(-8.89999999451621,-71.4381757456861,
-176.552638667358));
#137024=CARTESIAN_POINT('Ctrl Pts',(-8.89999997064355,-71.3830164241513,
-176.586384312661));
#137025=CARTESIAN_POINT('Ctrl Pts',(-8.89999995870723,-71.3554367633839,
-176.603257135313));
#137026=CARTESIAN_POINT('Ctrl Pts',(-8.89999994562374,-71.3275333910231,
-176.61959527903));
#137027=CARTESIAN_POINT('Ctrl Pts',(-8.89999993949196,-71.299333729225,
-176.635377629733));
#137028=CARTESIAN_POINT('Ctrl Pts',(-8.89999993336017,-71.2711340674268,
-176.651159980436));
#137029=CARTESIAN_POINT('Ctrl Pts',(-8.89999993496576,-71.242638116192,
-176.666386538126));
#137030=CARTESIAN_POINT('Ctrl Pts',(-8.89999994551797,-71.2138732976723,
-176.681036188718));
#137031=CARTESIAN_POINT('',(-8.9,-72.58000002,-174.432329119515));
#137032=CARTESIAN_POINT('',(-8.9,-55.5972887473416,-93.4294586200098));
#137033=CARTESIAN_POINT('Ctrl Pts',(-8.9,-55.5972887473416,-93.4294586200098));
#137034=CARTESIAN_POINT('Ctrl Pts',(-8.9,-60.7433024895534,-82.6526792495127));
#137035=CARTESIAN_POINT('Ctrl Pts',(-8.9,-65.8565639782118,-71.8603324984455));
#137036=CARTESIAN_POINT('Ctrl Pts',(-8.9,-70.9575466375288,-61.0621827299711));
#137037=CARTESIAN_POINT('',(-8.9,-55.08000002,-95.7201877838351));
#137038=CARTESIAN_POINT('Ctrl Pts',(-8.9,-55.08000002,-95.7201877838351));
#137039=CARTESIAN_POINT('Ctrl Pts',(-8.9,-55.08000002,-95.3987883664371));
#137040=CARTESIAN_POINT('Ctrl Pts',(-8.9,-55.109467211452,-95.0775170946566));
#137041=CARTESIAN_POINT('Ctrl Pts',(-8.9,-55.1665218943413,-94.7639046607142));
#137042=CARTESIAN_POINT('Ctrl Pts',(-8.9,-55.1800381380422,-94.6896099337934));
#137043=CARTESIAN_POINT('Ctrl Pts',(-8.9,-55.1951028648176,-94.6157450444869));
#137044=CARTESIAN_POINT('Ctrl Pts',(-8.9,-55.2116915002618,-94.5424101933588));
#137045=CARTESIAN_POINT('Ctrl Pts',(-8.9,-55.2822535698941,-94.2304701975012));
#137046=CARTESIAN_POINT('Ctrl Pts',(-8.9,-55.3800515517497,-93.9262693259458));
#137047=CARTESIAN_POINT('Ctrl Pts',(-8.9,-55.5065195348463,-93.6302150671016));
#137048=CARTESIAN_POINT('Ctrl Pts',(-8.9,-55.5352865893775,-93.5628730505705));
#137049=CARTESIAN_POINT('Ctrl Pts',(-8.9,-55.5655372445571,-93.4959526010439));
#137050=CARTESIAN_POINT('Ctrl Pts',(-8.9,-55.5972887473416,-93.4294586200098));
#137051=CARTESIAN_POINT('',(-8.9,-55.08000002,-136.338455187671));
#137052=CARTESIAN_POINT('',(-8.9,-55.08000002,-95.926725859984));
#137053=CARTESIAN_POINT('',(-8.9,-55.5972887473373,-138.629184351487));
#137054=CARTESIAN_POINT('Ctrl Pts',(-8.9,-55.5972887473373,-138.629184351487));
#137055=CARTESIAN_POINT('Ctrl Pts',(-8.9,-55.4856871847905,-138.39546841578));
#137056=CARTESIAN_POINT('Ctrl Pts',(-8.9,-55.3917128230604,-138.153503053561));
#137057=CARTESIAN_POINT('Ctrl Pts',(-8.9,-55.3159696737979,-137.907364658656));
#137058=CARTESIAN_POINT('Ctrl Pts',(-8.9,-55.275425284041,-137.775609759179));
#137059=CARTESIAN_POINT('Ctrl Pts',(-8.9,-55.240103934472,-137.642659649441));
#137060=CARTESIAN_POINT('Ctrl Pts',(-8.9,-55.2100924708571,-137.509141392841));
#137061=CARTESIAN_POINT('Ctrl Pts',(-8.9,-55.1385732376637,-137.190958865929));
#137062=CARTESIAN_POINT('Ctrl Pts',(-8.9,-55.0960936141251,-136.867828326659));
#137063=CARTESIAN_POINT('Ctrl Pts',(-8.9,-55.0837682332387,-136.53955984602));
#137064=CARTESIAN_POINT('Ctrl Pts',(-8.9,-55.0812593131255,-136.472738430829));
#137065=CARTESIAN_POINT('Ctrl Pts',(-8.9,-55.08000002,-136.405704093546));
#137066=CARTESIAN_POINT('Ctrl Pts',(-8.9,-55.08000002,-136.338455187671));
#137067=CARTESIAN_POINT('',(-8.9,-71.0715121820529,-171.237717270032));
#137068=CARTESIAN_POINT('Ctrl Pts',(-8.9,-71.0715121820529,-171.237717270032));
#137069=CARTESIAN_POINT('Ctrl Pts',(-8.9,-65.932751045448,-160.359049360718));
#137070=CARTESIAN_POINT('Ctrl Pts',(-8.9,-60.7816272203214,-149.486223352848));
#137071=CARTESIAN_POINT('Ctrl Pts',(-8.9,-55.5972887473373,-138.629184351487));
#137072=CARTESIAN_POINT('Origin',(-8.9,-69.0831852719725,-172.006057477089));
#137073=CARTESIAN_POINT('Origin',(0.,-12.9675000200281,-60.64995));
#137074=CARTESIAN_POINT('',(-9.30242220813418,-55.1547652725561,-93.2181494891177));
#137075=CARTESIAN_POINT('',(-14.8995694557399,-55.305434517314,-89.6101049856477));
#137076=CARTESIAN_POINT('Ctrl Pts',(-9.30242220787995,-55.1547652726018,
-93.2181494891395));
#137077=CARTESIAN_POINT('Ctrl Pts',(-10.1477584234389,-55.1733150950176,
-92.7890451196444));
#137078=CARTESIAN_POINT('Ctrl Pts',(-10.9772737219349,-55.1936535277891,
-92.3131807748197));
#137079=CARTESIAN_POINT('Ctrl Pts',(-12.8655985312176,-55.243800840887,
-91.1207823248442));
#137080=CARTESIAN_POINT('Ctrl Pts',(-13.8974380553098,-55.2740994408045,
-90.3869238925609));
#137081=CARTESIAN_POINT('Ctrl Pts',(-14.8995694550283,-55.3054345175152,
-89.6101049857472));
#137082=CARTESIAN_POINT('Ctrl Pts',(-9.32749162718857,-70.5102313269446,
-60.8508735991008));
#137083=CARTESIAN_POINT('Ctrl Pts',(-9.32127686111114,-65.4102595348795,
-71.6490160142261));
#137084=CARTESIAN_POINT('Ctrl Pts',(-9.31365506232303,-60.2983072126764,
-82.4413594866477));
#137085=CARTESIAN_POINT('Ctrl Pts',(-9.30242220787995,-55.1547652726018,
-93.2181494891395));
#137086=CARTESIAN_POINT('Ctrl Pts',(-14.8995694550283,-55.3054345175152,
-89.6101049857472));
#137087=CARTESIAN_POINT('Ctrl Pts',(-14.9143624117001,-60.0265024281888,
-80.0493410623047));
#137088=CARTESIAN_POINT('Ctrl Pts',(-14.9250579803326,-64.6843968356381,
-70.4566455899725));
#137089=CARTESIAN_POINT('Ctrl Pts',(-14.9339094669349,-69.3159372152925,
-60.8508735991008));
#137090=CARTESIAN_POINT('Ctrl Pts',(-14.9223321947707,-69.4149357692034,
-60.3843514923986));
#137091=CARTESIAN_POINT('Ctrl Pts',(-15.5501315664229,-69.2493490991427,
-60.3919718313355));
#137092=CARTESIAN_POINT('Ctrl Pts',(-15.5499999897346,-69.8979710840161,
-60.3623910423524));
#137093=CARTESIAN_POINT('Ctrl Pts',(-14.9213859066283,-69.4230681799894,
-60.5602124639497));
#137094=CARTESIAN_POINT('Ctrl Pts',(-15.5501319338923,-69.254225424885,
-60.5374367820963));
#137095=CARTESIAN_POINT('Ctrl Pts',(-15.5499999897191,-69.909794297014,
-60.6262209796107));
#137096=CARTESIAN_POINT('Ctrl Pts',(-14.9261257169452,-69.3823033916894,
-60.7335097961699));
#137097=CARTESIAN_POINT('Ctrl Pts',(-15.5501300981793,-69.2303831032415,
-60.678769908775));
#137098=CARTESIAN_POINT('Ctrl Pts',(-15.5499999897966,-69.8505276805174,
-60.8861498986541));
#137099=CARTESIAN_POINT('Ctrl Pts',(-14.9363515075123,-69.2951068303029,
-60.89043888838));
#137100=CARTESIAN_POINT('Ctrl Pts',(-15.5501262723864,-69.1690548338264,
-60.822436019398));
#137101=CARTESIAN_POINT('Ctrl Pts',(-15.5499999899638,-69.7237798948102,
-61.1215831761309));
#137102=CARTESIAN_POINT('',(-15.55,-69.7539685376239,-61.0621827299711));
#137103=CARTESIAN_POINT('Origin',(-15.05,-69.753968537624,-61.0621827299711));
#137104=CARTESIAN_POINT('Origin',(-15.5500003881169,-68.4591876507942,-60.4515855208217));
#137105=CARTESIAN_POINT('Origin',(-15.55,67.7009572055632,-55.24995));
#137106=CARTESIAN_POINT('',(-15.55,-70.08000002,-55.74995));
#137107=CARTESIAN_POINT('',(-15.55,67.7009572055632,-55.74995));
#137108=CARTESIAN_POINT('',(-15.55,-72.58000002,-58.24995));
#137109=CARTESIAN_POINT('Origin',(-15.55,-70.08000002,-58.24995));
#137110=CARTESIAN_POINT('',(-15.55,-72.58000002,-174.34995));
#137111=CARTESIAN_POINT('',(-15.55,-72.58000002,-58.24995));
#137112=CARTESIAN_POINT('',(-15.55,-70.08000002,-176.84995));
#137113=CARTESIAN_POINT('Origin',(-15.55,-70.08000002,-174.34995));
#137114=CARTESIAN_POINT('',(-15.55,67.7009572055632,-176.84995));
#137115=CARTESIAN_POINT('',(-15.55,-69.870344670579,-171.237717270032));
#137116=CARTESIAN_POINT('Origin',(-15.5500003878738,-68.5755848712236,-171.847853238442));
#137117=CARTESIAN_POINT('',(-15.55,-55.7328910677637,-142.237228854888));
#137118=CARTESIAN_POINT('Ctrl Pts',(-15.55,-55.7328910677637,-142.237228854888));
#137119=CARTESIAN_POINT('Ctrl Pts',(-15.55,-60.4987378575172,-151.878044750548));
#137120=CARTESIAN_POINT('Ctrl Pts',(-15.55,-65.1981545194713,-161.551244681819));
#137121=CARTESIAN_POINT('Ctrl Pts',(-15.55,-69.870344670579,-171.237717270032));
#137122=CARTESIAN_POINT('',(-15.55,-55.08000002,-139.407335470919));
#137123=CARTESIAN_POINT('Ctrl Pts',(-15.55,-55.08000002,-139.407335470919));
#137124=CARTESIAN_POINT('Ctrl Pts',(-15.55,-55.08000002,-139.59083822256));
#137125=CARTESIAN_POINT('Ctrl Pts',(-15.55,-55.0879005396309,-139.774357162878));
#137126=CARTESIAN_POINT('Ctrl Pts',(-15.55,-55.1034481519512,-139.956947178511));
#137127=CARTESIAN_POINT('Ctrl Pts',(-15.55,-55.1192595423617,-140.142634984636));
#137128=CARTESIAN_POINT('Ctrl Pts',(-15.55,-55.1429798052606,-140.327363292663));
#137129=CARTESIAN_POINT('Ctrl Pts',(-15.55,-55.1743956555241,-140.510141133111));
#137130=CARTESIAN_POINT('Ctrl Pts',(-15.55,-55.1948438531121,-140.629109022404));
#137131=CARTESIAN_POINT('Ctrl Pts',(-15.55,-55.2185534084275,-140.747250607227));
#137132=CARTESIAN_POINT('Ctrl Pts',(-15.55,-55.2454769784191,-140.864289524316));
#137133=CARTESIAN_POINT('Ctrl Pts',(-15.55,-55.3211274089245,-141.193148010259));
#137134=CARTESIAN_POINT('Ctrl Pts',(-15.55,-55.4215956233193,-141.514575802571));
#137135=CARTESIAN_POINT('Ctrl Pts',(-15.55,-55.5489107707142,-141.827965375896));
#137136=CARTESIAN_POINT('Ctrl Pts',(-15.55,-55.6049725527698,-141.965962922282));
#137137=CARTESIAN_POINT('Ctrl Pts',(-15.55,-55.666240524002,-142.102401687737));
#137138=CARTESIAN_POINT('Ctrl Pts',(-15.55,-55.7328910677637,-142.237228854888));
#137139=CARTESIAN_POINT('',(-15.55,-55.08000002,-92.6513075005872));
#137140=CARTESIAN_POINT('',(-15.55,-55.08000002,-139.74173251362));
#137141=CARTESIAN_POINT('',(-15.55,-55.7328910677637,-89.8214141166176));
#137142=CARTESIAN_POINT('Ctrl Pts',(-15.55,-55.7328910677637,-89.8214141166176));
#137143=CARTESIAN_POINT('Ctrl Pts',(-15.55,-55.6023063246601,-90.085573566672));
#137144=CARTESIAN_POINT('Ctrl Pts',(-15.55,-55.4913767816585,-90.3592181628692));
#137145=CARTESIAN_POINT('Ctrl Pts',(-15.55,-55.4001499318839,-90.6379301892029));
#137146=CARTESIAN_POINT('Ctrl Pts',(-15.55,-55.3390449811731,-90.824615191192));
#137147=CARTESIAN_POINT('Ctrl Pts',(-15.55,-55.2867806294645,-91.0135745317695));
#137148=CARTESIAN_POINT('Ctrl Pts',(-15.55,-55.2433833364682,-91.2034849476131));
#137149=CARTESIAN_POINT('Ctrl Pts',(-15.55,-55.1636960311292,-91.5522036867216));
#137150=CARTESIAN_POINT('Ctrl Pts',(-15.55,-55.1127619110561,-91.9058298380985));
#137151=CARTESIAN_POINT('Ctrl Pts',(-15.55,-55.0914526404125,-92.2645121879592));
#137152=CARTESIAN_POINT('Ctrl Pts',(-15.55,-55.0838313896103,-92.3927947647004));
#137153=CARTESIAN_POINT('Ctrl Pts',(-15.55,-55.08000002,-92.5217241762754));
#137154=CARTESIAN_POINT('Ctrl Pts',(-15.55,-55.08000002,-92.6513075005872));
#137155=CARTESIAN_POINT('Ctrl Pts',(-15.55,-69.7539685376239,-61.0621827299711));
#137156=CARTESIAN_POINT('Ctrl Pts',(-15.55,-65.1200645664474,-70.6679914124205));
#137157=CARTESIAN_POINT('Ctrl Pts',(-15.55,-60.459169452046,-80.2606410189155));
#137158=CARTESIAN_POINT('Ctrl Pts',(-15.55,-55.7328910677637,-89.8214141166175));
#137159=CARTESIAN_POINT('Origin',(-16.05,-73.08000002,-55.74995));
#137160=CARTESIAN_POINT('',(-16.05,-70.08000002,-55.24995));
#137161=CARTESIAN_POINT('',(-16.05,-73.08000002,-55.24995));
#137162=CARTESIAN_POINT('Origin',(-16.05,-70.08000002,-55.74995));
#137163=CARTESIAN_POINT('Origin',(-41.5,-73.08000002,-55.24995));
#137164=CARTESIAN_POINT('',(-16.55,-70.08000002,-55.24995));
#137165=CARTESIAN_POINT('',(-16.55,-73.08000002,-55.24995));
#137166=CARTESIAN_POINT('',(-41.5,-70.08000002,-55.24995));
#137167=CARTESIAN_POINT('Origin',(-16.55,67.7009572055632,-55.74995));
#137168=CARTESIAN_POINT('',(-17.05,-70.08000002,-55.74995));
#137169=CARTESIAN_POINT('',(-17.05,67.7009572055632,-55.74995));
#137170=CARTESIAN_POINT('Origin',(-16.55,-70.08000002,-55.74995));
#137171=CARTESIAN_POINT('Ctrl Pts',(-17.4174322081753,-68.5782862263167,
-60.8898940315426));
#137172=CARTESIAN_POINT('Ctrl Pts',(-17.0499351254479,-68.6669792326861,
-60.938279139678));
#137173=CARTESIAN_POINT('Ctrl Pts',(-17.0500000072447,-69.0016232241721,
-61.1207587448991));
#137174=CARTESIAN_POINT('Ctrl Pts',(-17.4057007122192,-68.6661491518679,
-60.7353408116852));
#137175=CARTESIAN_POINT('Ctrl Pts',(-17.0499377736316,-68.768366090799,
-60.7724682610327));
#137176=CARTESIAN_POINT('Ctrl Pts',(-17.0500000070135,-69.1279231312629,
-60.8888915170785));
#137177=CARTESIAN_POINT('Ctrl Pts',(-17.3999941136478,-68.7092345420341,
-60.5620638496915));
#137178=CARTESIAN_POINT('Ctrl Pts',(-17.0499390370914,-68.8203021885316,
-60.5773600099809));
#137179=CARTESIAN_POINT('Ctrl Pts',(-17.0500000069009,-69.1898773189587,
-60.6289947788348));
#137180=CARTESIAN_POINT('Ctrl Pts',(-17.4011286297274,-68.7006746954154,
-60.3838015812945));
#137181=CARTESIAN_POINT('Ctrl Pts',(-17.0499387884128,-68.8100686727309,
-60.3786737910309));
#137182=CARTESIAN_POINT('Ctrl Pts',(-17.0500000069233,-69.1775691162164,
-60.3615671969807));
#137183=CARTESIAN_POINT('',(-17.05,-69.0317756926871,-61.0621827299711));
#137184=CARTESIAN_POINT('Origin',(-17.55,-69.0317756926871,-61.0621827299711));
#137185=CARTESIAN_POINT('Origin',(-17.0499997344964,-67.7007635583902,-60.4478804500804));
#137186=CARTESIAN_POINT('Origin',(-17.05,67.7009572055632,-55.24995));
#137187=CARTESIAN_POINT('',(-17.05,-70.08000002,-176.84995));
#137188=CARTESIAN_POINT('',(-17.05,67.7009572055632,-176.84995));
#137189=CARTESIAN_POINT('',(-17.05,-72.58000002,-174.34995));
#137190=CARTESIAN_POINT('Origin',(-17.05,-70.08000002,-174.34995));
#137191=CARTESIAN_POINT('',(-17.05,-72.58000002,-58.24995));
#137192=CARTESIAN_POINT('',(-17.05,-72.58000002,-174.34995));
#137193=CARTESIAN_POINT('Origin',(-17.05,-70.08000002,-58.24995));
#137194=CARTESIAN_POINT('',(-17.05,-55.8060398696737,-87.7674469593951));
#137195=CARTESIAN_POINT('Ctrl Pts',(-17.05,-55.8060398696737,-87.7674469593951));
#137196=CARTESIAN_POINT('Ctrl Pts',(-17.05,-60.2764102501238,-78.896294484622));
#137197=CARTESIAN_POINT('Ctrl Pts',(-17.05,-64.6707000732441,-69.9874632456984));
#137198=CARTESIAN_POINT('Ctrl Pts',(-17.05,-69.0317756926871,-61.0621827299711));
#137199=CARTESIAN_POINT('',(-17.05,-55.08000002,-90.8821060618472));
#137200=CARTESIAN_POINT('Ctrl Pts',(-17.05,-55.08000002,-90.8821060618472));
#137201=CARTESIAN_POINT('Ctrl Pts',(-17.05,-55.0800000198976,-90.704401128278));
#137202=CARTESIAN_POINT('Ctrl Pts',(-17.05,-55.0867609195444,-90.5266735432516));
#137203=CARTESIAN_POINT('Ctrl Pts',(-17.05,-55.1000918811982,-90.3496297314767));
#137204=CARTESIAN_POINT('Ctrl Pts',(-17.05,-55.1137303582781,-90.1685019155126));
#137205=CARTESIAN_POINT('Ctrl Pts',(-17.05,-55.1342455055613,-89.9880886440527));
#137206=CARTESIAN_POINT('Ctrl Pts',(-17.05,-55.1614876321832,-89.8091398363497));
#137207=CARTESIAN_POINT('Ctrl Pts',(-17.05,-55.1887297588051,-89.6301910286466));
#137208=CARTESIAN_POINT('Ctrl Pts',(-17.05,-55.2226990580678,-89.4527054855484));
#137209=CARTESIAN_POINT('Ctrl Pts',(-17.05,-55.2632981110657,-89.2774444065539));
#137210=CARTESIAN_POINT('Ctrl Pts',(-17.05,-55.3408916382115,-88.9424827686241));
#137211=CARTESIAN_POINT('Ctrl Pts',(-17.05,-55.4420234811604,-88.614774521522));
#137212=CARTESIAN_POINT('Ctrl Pts',(-17.05,-55.5689958159337,-88.2950290565654));
#137213=CARTESIAN_POINT('Ctrl Pts',(-17.05,-55.6398317020692,-88.1166480463363));
#137214=CARTESIAN_POINT('Ctrl Pts',(-17.05,-55.7187108542616,-87.9407455779088));
#137215=CARTESIAN_POINT('Ctrl Pts',(-17.05,-55.8060398696737,-87.7674469593951));
#137216=CARTESIAN_POINT('',(-17.05,-55.08000002,-141.176536909659));
#137217=CARTESIAN_POINT('',(-17.05,-55.08000002,-91.2551956845905));
#137218=CARTESIAN_POINT('',(-17.05,-55.8060398696787,-144.291196012121));
#137219=CARTESIAN_POINT('Ctrl Pts',(-17.05,-55.8060398696787,-144.291196012121));
#137220=CARTESIAN_POINT('Ctrl Pts',(-17.05,-55.6831540655477,-144.047337313036));
#137221=CARTESIAN_POINT('Ctrl Pts',(-17.05,-55.5762002500337,-143.795681932952));
#137222=CARTESIAN_POINT('Ctrl Pts',(-17.05,-55.4849662480647,-143.539333784836));
#137223=CARTESIAN_POINT('Ctrl Pts',(-17.05,-55.3950897214903,-143.286799853964));
#137224=CARTESIAN_POINT('Ctrl Pts',(-17.05,-55.3204688827058,-143.029710172843));
#137225=CARTESIAN_POINT('Ctrl Pts',(-17.05,-55.2609467896032,-142.77101380861));
#137226=CARTESIAN_POINT('Ctrl Pts',(-17.05,-55.1772261529236,-142.407145147557));
#137227=CARTESIAN_POINT('Ctrl Pts',(-17.05,-55.1222258452589,-142.038367265734));
#137228=CARTESIAN_POINT('Ctrl Pts',(-17.05,-55.0966366319634,-141.664562069113));
#137229=CARTESIAN_POINT('Ctrl Pts',(-17.05,-55.0855652067498,-141.502831568412));
#137230=CARTESIAN_POINT('Ctrl Pts',(-17.05,-55.0800000200001,-141.340159872037));
#137231=CARTESIAN_POINT('Ctrl Pts',(-17.05,-55.08000002,-141.176536909659));
#137232=CARTESIAN_POINT('',(-17.05,-69.1496478013716,-171.237717270032));
#137233=CARTESIAN_POINT('Ctrl Pts',(-17.05,-69.1496478013716,-171.237717270032));
#137234=CARTESIAN_POINT('Ctrl Pts',(-17.05,-64.7499424271364,-162.231693289135));
#137235=CARTESIAN_POINT('Ctrl Pts',(-17.05,-60.3166901832211,-153.242281332924));
#137236=CARTESIAN_POINT('Ctrl Pts',(-17.05,-55.8060398696787,-144.291196012121));
#137237=CARTESIAN_POINT('Origin',(-17.0499997303009,-67.8195562478302,-171.852380930964));
#137238=CARTESIAN_POINT('Origin',(0.,-12.9675000200281,-60.64995));
#137239=CARTESIAN_POINT('',(-17.3782102443508,-55.3867109640818,-87.5561378285247));
#137240=CARTESIAN_POINT('',(-22.9849163801915,-55.5914230811224,-82.0118419126005));
#137241=CARTESIAN_POINT('Ctrl Pts',(-17.3782874559398,-55.3867051038986,
-87.5562252660302));
#137242=CARTESIAN_POINT('Ctrl Pts',(-18.121577867119,-55.4121156870237,
-86.9015665730796));
#137243=CARTESIAN_POINT('Ctrl Pts',(-18.8518378359084,-55.4379479436565,
-86.2242613702274));
#137244=CARTESIAN_POINT('Ctrl Pts',(-19.5713894980264,-55.4639865475406,
-85.5280522873859));
#137245=CARTESIAN_POINT('Ctrl Pts',(-20.7455454946912,-55.5064760371838,
-84.3919864389039));
#137246=CARTESIAN_POINT('Ctrl Pts',(-21.8822352961522,-55.5492052310813,
-83.2139191382355));
#137247=CARTESIAN_POINT('Ctrl Pts',(-22.9849164160517,-55.5914231002813,
-82.0118419843783));
#137248=CARTESIAN_POINT('Ctrl Pts',(-17.4146253252297,-68.5993151180197,
-60.8508735991007));
#137249=CARTESIAN_POINT('Ctrl Pts',(-17.4050346480916,-64.2412639468132,
-69.7761085955077));
#137250=CARTESIAN_POINT('Ctrl Pts',(-17.3935606665343,-59.8507835974011,
-78.6850032438638));
#137251=CARTESIAN_POINT('Ctrl Pts',(-17.3782102443508,-55.3867109640818,
-87.5561378285247));
#137252=CARTESIAN_POINT('Ctrl Pts',(-22.9849163103247,-55.591423110293,
-82.011841880507));
#137253=CARTESIAN_POINT('Ctrl Pts',(-22.9993168926453,-59.3018045077389,
-74.9936336228867));
#137254=CARTESIAN_POINT('Ctrl Pts',(-23.0109831737233,-62.9327835325611,
-67.9329755599233));
#137255=CARTESIAN_POINT('Ctrl Pts',(-23.0210431649761,-66.5230748737403,
-60.8508735991007));
#137256=CARTESIAN_POINT('Ctrl Pts',(-23.0030676793156,-66.6324461755808,
-60.4045898193565));
#137257=CARTESIAN_POINT('Ctrl Pts',(-23.7000444961004,-66.3339120499585,
-60.4123961703627));
#137258=CARTESIAN_POINT('Ctrl Pts',(-23.6999999991391,-67.091907941907,
-60.3927543614167));
#137259=CARTESIAN_POINT('Ctrl Pts',(-23.0023333098327,-66.6369323384221,
-60.5671687383203));
#137260=CARTESIAN_POINT('Ctrl Pts',(-23.7000445996745,-66.3350862497419,
-60.5213661743307));
#137261=CARTESIAN_POINT('Ctrl Pts',(-23.6999999991382,-67.0981649919418,
-60.6366434264749));
#137262=CARTESIAN_POINT('Ctrl Pts',(-23.0091746715062,-66.5951265090932,
-60.7272889592981));
#137263=CARTESIAN_POINT('Ctrl Pts',(-23.7000436587853,-66.3247262225065,
-60.6279370962779));
#137264=CARTESIAN_POINT('Ctrl Pts',(-23.6999999991466,-67.0398545336995,
-60.8767984170799));
#137265=CARTESIAN_POINT('Ctrl Pts',(-23.0230090051547,-66.5111384208438,
-60.8720725996219));
#137266=CARTESIAN_POINT('Ctrl Pts',(-23.7000418676227,-66.2856006591993,
-60.7504731407162));
#137267=CARTESIAN_POINT('Ctrl Pts',(-23.6999999991637,-66.9227827756709,
-61.0939974638476));
#137268=CARTESIAN_POINT('',(-23.7,-66.9393955463102,-61.0621827299711));
#137269=CARTESIAN_POINT('Origin',(-23.2,-66.9393955463102,-61.0621827299711));
#137270=CARTESIAN_POINT('Origin',(-23.7000000338414,-65.5006105045681,-60.4353544160189));
#137271=CARTESIAN_POINT('Origin',(-23.7,67.7009572055632,-55.24995));
#137272=CARTESIAN_POINT('',(-23.7,-70.08000002,-55.74995));
#137273=CARTESIAN_POINT('',(-23.7,67.7009572055632,-55.74995));
#137274=CARTESIAN_POINT('',(-23.7,-72.58000002,-58.24995));
#137275=CARTESIAN_POINT('Origin',(-23.7,-70.08000002,-58.24995));
#137276=CARTESIAN_POINT('',(-23.7,-72.58000002,-174.34995));
#137277=CARTESIAN_POINT('',(-23.7,-72.58000002,-58.24995));
#137278=CARTESIAN_POINT('',(-23.7,-70.08000002,-176.84995));
#137279=CARTESIAN_POINT('Origin',(-23.7,-70.08000002,-174.34995));
#137280=CARTESIAN_POINT('',(-23.7,67.7009572055632,-176.84995));
#137281=CARTESIAN_POINT('',(-23.7,-67.0618271655313,-171.237717270032));
#137282=CARTESIAN_POINT('Origin',(-23.7000000319865,-65.6225360751686,-171.864194562605));
#137283=CARTESIAN_POINT('',(-23.7,-55.9902808012637,-149.835491960129));
#137284=CARTESIAN_POINT('Ctrl Pts',(-23.7,-55.9902808012637,-149.835491960129));
#137285=CARTESIAN_POINT('Ctrl Pts',(-23.7,-59.7506641394806,-156.933423835337));
#137286=CARTESIAN_POINT('Ctrl Pts',(-23.7,-63.4273897219659,-164.074632552453));
#137287=CARTESIAN_POINT('Ctrl Pts',(-23.7,-67.0618271655313,-171.237717270032));
#137288=CARTESIAN_POINT('',(-23.7,-55.08000002,-146.023178055809));
#137289=CARTESIAN_POINT('Ctrl Pts',(-23.7,-55.08000002,-146.023178055809));
#137290=CARTESIAN_POINT('Ctrl Pts',(-23.7,-55.08000002,-146.158053606653));
#137291=CARTESIAN_POINT('Ctrl Pts',(-23.7000000000707,-55.0831707493112,
-146.292669951121));
#137292=CARTESIAN_POINT('Ctrl Pts',(-23.6999999992499,-55.0894565008802,
-146.427026468199));
#137293=CARTESIAN_POINT('Ctrl Pts',(-23.6999999984213,-55.0958009827676,
-146.562638332538));
#137294=CARTESIAN_POINT('Ctrl Pts',(-23.6999999964552,-55.1053189899911,
-146.697986218052));
#137295=CARTESIAN_POINT('Ctrl Pts',(-23.6999999951529,-55.1180059197239,
-146.833072917223));
#137296=CARTESIAN_POINT('Ctrl Pts',(-23.6999999945721,-55.1236634789143,
-146.893312944754));
#137297=CARTESIAN_POINT('Ctrl Pts',(-23.6999999941814,-55.1299519000527,
-146.953501011813));
#137298=CARTESIAN_POINT('Ctrl Pts',(-23.6999999942164,-55.1368740952971,
-147.013636993293));
#137299=CARTESIAN_POINT('Ctrl Pts',(-23.6999999943017,-55.1537261451255,
-147.160037740543));
#137300=CARTESIAN_POINT('Ctrl Pts',(-23.6999999965898,-55.1743560689035,
-147.306288458156));
#137301=CARTESIAN_POINT('Ctrl Pts',(-23.6999999980531,-55.1987232126615,
-147.451788749127));
#137302=CARTESIAN_POINT('Ctrl Pts',(-23.6999999995039,-55.2228814172672,
-147.596041429472));
#137303=CARTESIAN_POINT('Ctrl Pts',(-23.699999999956,-55.2507128773882,
-147.73955572536));
#137304=CARTESIAN_POINT('Ctrl Pts',(-23.6999999999927,-55.2821282400235,
-147.881757850267));
#137305=CARTESIAN_POINT('Ctrl Pts',(-23.700000000002,-55.2901469859131,
-147.918054827572));
#137306=CARTESIAN_POINT('Ctrl Pts',(-23.7,-55.2983989829638,-147.954266404712));
#137307=CARTESIAN_POINT('Ctrl Pts',(-23.7,-55.3068822390434,-147.990383251025));
#137308=CARTESIAN_POINT('Ctrl Pts',(-23.7,-55.3875157587021,-148.333674601646));
#137309=CARTESIAN_POINT('Ctrl Pts',(-23.7,-55.4886143890992,-148.670181748614));
#137310=CARTESIAN_POINT('Ctrl Pts',(-23.7,-55.6129610034727,-148.998982220287));
#137311=CARTESIAN_POINT('Ctrl Pts',(-23.7,-55.7206760510249,-149.283805081125));
#137312=CARTESIAN_POINT('Ctrl Pts',(-23.7,-55.8458362712923,-149.562844907631));
#137313=CARTESIAN_POINT('Ctrl Pts',(-23.7,-55.9902808012637,-149.835491960129));
#137314=CARTESIAN_POINT('',(-23.7,-55.08000002,-86.035464915697));
#137315=CARTESIAN_POINT('',(-23.7,-55.08000002,-146.505061715151));
#137316=CARTESIAN_POINT('',(-23.7,-55.9902808012638,-82.2231510113773));
#137317=CARTESIAN_POINT('Ctrl Pts',(-23.7,-55.9902808012637,-82.2231510113773));
#137318=CARTESIAN_POINT('Ctrl Pts',(-23.7,-55.895308966207,-82.4024156114538));
#137319=CARTESIAN_POINT('Ctrl Pts',(-23.7,-55.8083129339554,-82.5857246305521));
#137320=CARTESIAN_POINT('Ctrl Pts',(-23.7,-55.7290034297554,-82.7720704820173));
#137321=CARTESIAN_POINT('Ctrl Pts',(-23.7,-55.6467059711238,-82.9654368402719));
#137322=CARTESIAN_POINT('Ctrl Pts',(-23.7,-55.5726850268912,-83.1620740930088));
#137323=CARTESIAN_POINT('Ctrl Pts',(-23.7,-55.5066653875374,-83.3608873091131));
#137324=CARTESIAN_POINT('Ctrl Pts',(-23.7,-55.4379479535128,-83.5678247325012));
#137325=CARTESIAN_POINT('Ctrl Pts',(-23.7,-55.3778989830438,-83.7771208288598));
#137326=CARTESIAN_POINT('Ctrl Pts',(-23.7,-55.326260979212,-83.9875567996247));
#137327=CARTESIAN_POINT('Ctrl Pts',(-23.7,-55.3186643927326,-84.0185145232327));
#137328=CARTESIAN_POINT('Ctrl Pts',(-23.7,-55.3112499282573,-84.0494969228628));
#137329=CARTESIAN_POINT('Ctrl Pts',(-23.7,-55.304016859788,-84.0805001191198));
#137330=CARTESIAN_POINT('Ctrl Pts',(-23.7,-55.2100486983101,-84.4832770822498));
#137331=CARTESIAN_POINT('Ctrl Pts',(-23.7,-55.1455757138289,-84.8909305418239));
#137332=CARTESIAN_POINT('Ctrl Pts',(-23.7,-55.1107223807414,-85.3034811063171));
#137333=CARTESIAN_POINT('Ctrl Pts',(-23.7,-55.090251973458,-85.5457844194304));
#137334=CARTESIAN_POINT('Ctrl Pts',(-23.7,-55.0800000200001,-85.7897771817878));
#137335=CARTESIAN_POINT('Ctrl Pts',(-23.7,-55.08000002,-86.035464915697));
#137336=CARTESIAN_POINT('Ctrl Pts',(-23.7,-66.9393955463102,-61.0621827299711));
#137337=CARTESIAN_POINT('Ctrl Pts',(-23.7,-63.3447563953728,-68.1443309684329));
#137338=CARTESIAN_POINT('Ctrl Pts',(-23.7,-59.7084420726901,-75.2049156266561));
#137339=CARTESIAN_POINT('Ctrl Pts',(-23.7,-55.9902808012637,-82.2231510113772));
#137340=CARTESIAN_POINT('Origin',(-24.2,-73.08000002,-55.74995));
#137341=CARTESIAN_POINT('Origin',(-24.2,-70.08000002,-55.74995));
#137342=CARTESIAN_POINT('Origin',(0.,-12.9675000200281,-61.64995));
#137343=CARTESIAN_POINT('',(-22.3259225534138,40.6914751389564,-61.2273317382593));
#137344=CARTESIAN_POINT('',(-28.2795019009908,37.8065307949999,-61.2273317382593));
#137345=CARTESIAN_POINT('Origin',(0.,-12.9675000200281,-61.2273317382593));
#137346=CARTESIAN_POINT('Ctrl Pts',(-28.4933647440612,38.6927858841383,
-60.650327573148));
#137347=CARTESIAN_POINT('Ctrl Pts',(-28.4508217728044,38.5151017970219,
-60.6551690977179));
#137348=CARTESIAN_POINT('Ctrl Pts',(-28.4075947879363,38.335472514688,-60.707925961796));
#137349=CARTESIAN_POINT('Ctrl Pts',(-28.3514280416523,38.1029959208976,
-60.8540715547449));
#137350=CARTESIAN_POINT('Ctrl Pts',(-28.3338483525148,38.0303960306507,
-60.9145171861254));
#137351=CARTESIAN_POINT('Ctrl Pts',(-28.302912455342,37.9028346914031,-61.0569005178125));
#137352=CARTESIAN_POINT('Ctrl Pts',(-28.28982523324,37.8489775515987,-61.1370349799883));
#137353=CARTESIAN_POINT('Ctrl Pts',(-28.2795019009908,37.8065307949999,
-61.2273317382593));
#137354=CARTESIAN_POINT('Origin',(-22.4949668999609,41.5737931892869,-61.6552254095787));
#137355=CARTESIAN_POINT('Ctrl Pts',(-22.3089577584378,40.9899884313956,
-60.5010370523947));
#137356=CARTESIAN_POINT('Ctrl Pts',(-22.,41.1177283573993,-60.5010370523946));
#137357=CARTESIAN_POINT('Ctrl Pts',(-22.,41.4520521304013,-60.5010370523947));
#137358=CARTESIAN_POINT('Ctrl Pts',(-22.3089577682091,40.9899884273556,
-60.7079658702078));
#137359=CARTESIAN_POINT('Ctrl Pts',(-22.,41.1177283336776,-60.7368788147381));
#137360=CARTESIAN_POINT('Ctrl Pts',(-22.,41.4520521024983,-60.811367390836));
#137361=CARTESIAN_POINT('Ctrl Pts',(-22.3211558478618,40.913825471773,-60.9106181484486));
#137362=CARTESIAN_POINT('Ctrl Pts',(-21.9999999999979,41.0241336396768,
-60.969503986646));
#137363=CARTESIAN_POINT('Ctrl Pts',(-22.,41.345292929857,-61.115492429943));
#137364=CARTESIAN_POINT('Ctrl Pts',(-22.3428990418276,40.7794755973204,
-61.0754935261973));
#137365=CARTESIAN_POINT('Ctrl Pts',(-22.,40.8698280768405,-61.1441646043173));
#137366=CARTESIAN_POINT('Ctrl Pts',(-22.,41.1573899115079,-61.3627217630986));
#137367=CARTESIAN_POINT('',(-22.,41.1573899115079,-61.3627217630986));
#137368=CARTESIAN_POINT('Origin',(-22.,40.1816528161032,-60.6046736522198));
#137369=CARTESIAN_POINT('Origin',(-22.5,41.1573899115079,-61.3627217630986));
#137370=CARTESIAN_POINT('Origin',(-22.,-9.33460238845303,-92.34995));
#137371=CARTESIAN_POINT('',(-22.,43.91999998,-55.74995));
#137372=CARTESIAN_POINT('',(-22.,41.1166950488946,-55.74995));
#137373=CARTESIAN_POINT('',(-22.,46.41999998,-58.24995));
#137374=CARTESIAN_POINT('Origin',(-22.,43.91999998,-58.24995));
#137375=CARTESIAN_POINT('',(-22.,46.41999998,-58.24995));
#137376=CARTESIAN_POINT('',(-22.,28.9199999800001,-91.34995));
#137377=CARTESIAN_POINT('Origin',(-22.,29.41999998,-91.34995));
#137378=CARTESIAN_POINT('',(-22.,28.9199999800001,-87.1305533863517));
#137379=CARTESIAN_POINT('',(-22.,28.9199999800001,-91.34995));
#137380=CARTESIAN_POINT('',(-22.,29.8104512658091,-83.3922397161652));
#137381=CARTESIAN_POINT('Ctrl Pts',(-22.,29.8104512658092,-83.3922397161652));
#137382=CARTESIAN_POINT('Ctrl Pts',(-22.,29.7130107699212,-83.5771800425296));
#137383=CARTESIAN_POINT('Ctrl Pts',(-22.,29.6241027734271,-83.7664339874128));
#137384=CARTESIAN_POINT('Ctrl Pts',(-22.,29.5434345930966,-83.9588738468729));
#137385=CARTESIAN_POINT('Ctrl Pts',(-22.,29.4578017187799,-84.1631573478911));
#137386=CARTESIAN_POINT('Ctrl Pts',(-22.,29.3814538044553,-84.3710319263885));
#137387=CARTESIAN_POINT('Ctrl Pts',(-22.,29.3140928258487,-84.5811807101613));
#137388=CARTESIAN_POINT('Ctrl Pts',(-22.,29.2470690502147,-84.7902775081102));
#137389=CARTESIAN_POINT('Ctrl Pts',(-22.,29.1889427079809,-85.0016271465761));
#137390=CARTESIAN_POINT('Ctrl Pts',(-22.,29.1394698146751,-85.2139452109128));
#137391=CARTESIAN_POINT('Ctrl Pts',(-22.,29.0466872110909,-85.6121313989602));
#137392=CARTESIAN_POINT('Ctrl Pts',(-22.,28.9832164657706,-86.0152044949726));
#137393=CARTESIAN_POINT('Ctrl Pts',(-22.,28.9492578229232,-86.4231979120772));
#137394=CARTESIAN_POINT('Ctrl Pts',(-22.,28.9297677681886,-86.6573596265608));
#137395=CARTESIAN_POINT('Ctrl Pts',(-22.,28.9199999800002,-86.893142259867));
#137396=CARTESIAN_POINT('Ctrl Pts',(-22.,28.91999998,-87.1305533863517));
#137397=CARTESIAN_POINT('',(-22.,41.1098595241823,-61.4386408691296));
#137398=CARTESIAN_POINT('Ctrl Pts',(-22.,41.1098595241823,-61.4386408691296));
#137399=CARTESIAN_POINT('Ctrl Pts',(-22.,37.3993520818416,-68.7853105030709));
#137400=CARTESIAN_POINT('Ctrl Pts',(-22.,33.6470396305176,-76.1104633065809));
#137401=CARTESIAN_POINT('Ctrl Pts',(-22.,29.8104512658091,-83.3922397161652));
#137402=CARTESIAN_POINT('Origin',(-22.,41.5483105744971,-61.66030212062));
#137403=CARTESIAN_POINT('Origin',(-21.5,0.,-55.74995));
#137404=CARTESIAN_POINT('',(-21.5,43.91999998,-55.24995));
#137405=CARTESIAN_POINT('',(-21.5,43.91999998,-55.24995));
#137406=CARTESIAN_POINT('Origin',(-21.5,43.91999998,-55.74995));
#137407=CARTESIAN_POINT('Origin',(0.,0.,-55.24995));
#137408=CARTESIAN_POINT('',(-21.,43.91999998,-55.24995));
#137409=CARTESIAN_POINT('',(-21.,41.7028772994424,-55.24995));
#137410=CARTESIAN_POINT('',(0.,43.91999998,-55.24995));
#137411=CARTESIAN_POINT('Origin',(-21.,-9.33460238845303,-55.74995));
#137412=CARTESIAN_POINT('',(-20.5,43.91999998,-55.74995));
#137413=CARTESIAN_POINT('',(-20.5,43.91999998,-55.74995));
#137414=CARTESIAN_POINT('Origin',(-21.,43.91999998,-55.74995));
#137415=CARTESIAN_POINT('Origin',(-20.5,-9.33460238845303,-92.34995));
#137416=CARTESIAN_POINT('',(-20.5,42.270218132516,-61.0621827299711));
#137417=CARTESIAN_POINT('Origin',(-20.5000001497348,40.8982420778451,-60.4432551283365));
#137418=CARTESIAN_POINT('',(-20.5,29.726759920701,-85.9392854774869));
#137419=CARTESIAN_POINT('Ctrl Pts',(-20.5,29.726759920701,-85.9392854774869));
#137420=CARTESIAN_POINT('Ctrl Pts',(-20.5,33.9784770268254,-77.682497649623));
#137421=CARTESIAN_POINT('Ctrl Pts',(-20.5,38.1440239783714,-69.3822613645965));
#137422=CARTESIAN_POINT('Ctrl Pts',(-20.5,42.270218132516,-61.0621827299711));
#137423=CARTESIAN_POINT('',(-20.5,28.9199999800001,-89.3628471840452));
#137424=CARTESIAN_POINT('Ctrl Pts',(-20.5,28.9199999800001,-89.3628471840452));
#137425=CARTESIAN_POINT('Ctrl Pts',(-20.5,28.9199999800001,-89.0651820878934));
#137426=CARTESIAN_POINT('Ctrl Pts',(-20.5,28.93706429112,-88.7687961767652));
#137427=CARTESIAN_POINT('Ctrl Pts',(-20.5,29.004819730958,-88.1785451079783));
#137428=CARTESIAN_POINT('Ctrl Pts',(-20.5,29.0556764864843,-87.8849108068938));
#137429=CARTESIAN_POINT('Ctrl Pts',(-20.5,29.2565698843866,-87.0234827289138));
#137430=CARTESIAN_POINT('Ctrl Pts',(-20.5,29.453814841029,-86.4693418183145));
#137431=CARTESIAN_POINT('Ctrl Pts',(-20.5,29.726759920701,-85.9392854774869));
#137432=CARTESIAN_POINT('',(-20.5,28.9199999800001,-91.34995));
#137433=CARTESIAN_POINT('',(-20.5,28.9199999800001,-88.9338641536579));
#137434=CARTESIAN_POINT('Origin',(-20.5,29.41999998,-91.34995));
#137435=CARTESIAN_POINT('',(-20.5,46.41999998,-58.24995));
#137436=CARTESIAN_POINT('',(-20.5,46.41999998,-92.34995));
#137437=CARTESIAN_POINT('Origin',(-20.5,43.91999998,-58.24995));
#137438=CARTESIAN_POINT('Ctrl Pts',(-19.8489174898872,41.8225779837155,
-60.8897941554007));
#137439=CARTESIAN_POINT('Ctrl Pts',(-20.5000844423968,41.6420275017582,
-60.7898798297297));
#137440=CARTESIAN_POINT('Ctrl Pts',(-20.4999999961793,42.2396703210244,
-61.1205979678028));
#137441=CARTESIAN_POINT('Ctrl Pts',(-19.8355865710622,41.9126116301234,
-60.7356962259096));
#137442=CARTESIAN_POINT('Ctrl Pts',(-20.5000878549352,41.6934063086951,
-60.6536629857367));
#137443=CARTESIAN_POINT('Ctrl Pts',(-20.4999999961011,42.3674932175841,
-60.8894198661636));
#137444=CARTESIAN_POINT('Ctrl Pts',(-19.8290476963325,41.9571155016239,
-60.5621838877489));
#137445=CARTESIAN_POINT('Ctrl Pts',(-20.5000896090863,41.710625264557,-60.5273413240715));
#137446=CARTESIAN_POINT('Ctrl Pts',(-20.4999999960627,42.4307087138456,
-60.6291716490909));
#137447=CARTESIAN_POINT('Ctrl Pts',(-19.8303467534611,41.9482798096484,
-60.383760106758));
#137448=CARTESIAN_POINT('Ctrl Pts',(-20.5000892602552,41.7070302221805,
-60.3953720501034));
#137449=CARTESIAN_POINT('Ctrl Pts',(-20.4999999960704,42.4181586164624,
-60.3615059809689));
#137450=CARTESIAN_POINT('Origin',(-20.,42.270218132516,-61.0621827299711));
#137451=CARTESIAN_POINT('Origin',(0.,-12.9675000200281,-60.64995));
#137452=CARTESIAN_POINT('',(-19.8077681423597,29.3163998849126,-85.7279763868962));
#137453=CARTESIAN_POINT('',(-13.8582614853459,29.115831713372,-90.8469388041467));
#137454=CARTESIAN_POINT('Ctrl Pts',(-19.8077680666401,29.3163999141123,
-85.7279763466165));
#137455=CARTESIAN_POINT('Ctrl Pts',(-18.8664797933811,29.281909340585,-86.6512762314539));
#137456=CARTESIAN_POINT('Ctrl Pts',(-17.899945936779,29.2474791030901,-87.5495367943307));
#137457=CARTESIAN_POINT('Ctrl Pts',(-15.9119634012864,29.1799677018946,
-89.269473055814));
#137458=CARTESIAN_POINT('Ctrl Pts',(-14.8954908494031,29.1470358100342,
-90.0876330868643));
#137459=CARTESIAN_POINT('Ctrl Pts',(-13.8582614853459,29.115831713372,-90.8469388041467));
#137460=CARTESIAN_POINT('Ctrl Pts',(-19.8457268663587,41.8441333387867,
-60.8508735991007));
#137461=CARTESIAN_POINT('Ctrl Pts',(-19.8355385600285,37.7216554195719,
-69.1708971047811));
#137462=CARTESIAN_POINT('Ctrl Pts',(-19.8234665452012,33.5607487699413,
-77.4712163753771));
#137463=CARTESIAN_POINT('Ctrl Pts',(-19.8077680666401,29.3163999141123,
-85.7279763466165));
#137464=CARTESIAN_POINT('Ctrl Pts',(-13.8582614853459,29.115831713372,-90.8469388041467));
#137465=CARTESIAN_POINT('Ctrl Pts',(-13.8729899561679,34.0078013158341,
-80.8725774674286));
#137466=CARTESIAN_POINT('Ctrl Pts',(-13.8834224238665,38.8394159067996,
-70.867726207482));
#137467=CARTESIAN_POINT('Ctrl Pts',(-13.8920088064511,43.6468101642065,
-60.8508735991007));
#137468=CARTESIAN_POINT('Ctrl Pts',(-13.8812391026075,43.7449355503387,
-60.3843616038035));
#137469=CARTESIAN_POINT('Ctrl Pts',(-13.4999161431562,43.8380646295733,
-60.380129448632));
#137470=CARTESIAN_POINT('Ctrl Pts',(-13.5000000114112,44.2302441743789,
-60.3624063574045));
#137471=CARTESIAN_POINT('Ctrl Pts',(-13.8803600752771,43.7529853273083,
-60.5601847150614));
#137472=CARTESIAN_POINT('Ctrl Pts',(-13.4999163945295,43.8475317166231,
-60.5727811392321));
#137473=CARTESIAN_POINT('Ctrl Pts',(-13.5000000113849,44.2419957581614,
-60.6261785981702));
#137474=CARTESIAN_POINT('Ctrl Pts',(-13.884762026428,43.7126430688856,-60.7334063315744));
#137475=CARTESIAN_POINT('Ctrl Pts',(-13.4999151269544,43.7997377261502,
-60.7643333157514));
#137476=CARTESIAN_POINT('Ctrl Pts',(-13.5000000115167,44.1831007301226,
-60.8859969728056));
#137477=CARTESIAN_POINT('Ctrl Pts',(-13.8942821039575,43.6261495705425,
-60.8904677863889));
#137478=CARTESIAN_POINT('Ctrl Pts',(-13.4999123453879,43.7012956163656,
-60.9308210213385));
#137479=CARTESIAN_POINT('Ctrl Pts',(-13.5000000118016,44.0568479860271,
-61.1216298968641));
#137480=CARTESIAN_POINT('',(-13.5,44.086908282047,-61.0621827299711));
#137481=CARTESIAN_POINT('Origin',(-13.4999995641033,42.8035277780889,-60.452854070096));
#137482=CARTESIAN_POINT('Origin',(-14.,44.086908282047,-61.0621827299711));
#137483=CARTESIAN_POINT('Origin',(-13.5,-9.33460238845303,-92.34995));
#137484=CARTESIAN_POINT('',(-13.5,46.41999998,-58.2497627936531));
#137485=CARTESIAN_POINT('Ctrl Pts',(-13.5,46.41999998,-58.2497627936531));
#137486=CARTESIAN_POINT('Ctrl Pts',(-13.5,46.41999998,-58.1672776827351));
#137487=CARTESIAN_POINT('Ctrl Pts',(-13.5,46.4159357655689,-58.0853150765278));
#137488=CARTESIAN_POINT('Ctrl Pts',(-13.5,46.4079129436513,-58.0040039069954));
#137489=CARTESIAN_POINT('Ctrl Pts',(-13.5,46.3998480609524,-57.9222664521287));
#137490=CARTESIAN_POINT('Ctrl Pts',(-13.5,46.3877828714201,-57.8411867135011));
#137491=CARTESIAN_POINT('Ctrl Pts',(-13.4999999999999,46.371771733687,-57.7608954152445));
#137492=CARTESIAN_POINT('Ctrl Pts',(-13.4999999999999,46.3557907741679,
-57.6807554521414));
#137493=CARTESIAN_POINT('Ctrl Pts',(-13.4999999999998,46.3358786103981,
-57.6014003971059));
#137494=CARTESIAN_POINT('Ctrl Pts',(-13.4999999999993,46.3120383093697,
-57.5229684754948));
#137495=CARTESIAN_POINT('Ctrl Pts',(-13.499999999999,46.2959527721241,-57.4700488586319));
#137496=CARTESIAN_POINT('Ctrl Pts',(-13.4999999999985,46.2780779115088,
-57.4175496722019));
#137497=CARTESIAN_POINT('Ctrl Pts',(-13.4999999999976,46.2584018781846,
-57.3655174652213));
#137498=CARTESIAN_POINT('Ctrl Pts',(-13.4999999999975,46.2569427240896,
-57.361658811059));
#137499=CARTESIAN_POINT('Ctrl Pts',(-13.4999999999974,46.2554739003334,
-57.3578033707196));
#137500=CARTESIAN_POINT('Ctrl Pts',(-13.4999999999974,46.2539954124749,
-57.3539511680007));
#137501=CARTESIAN_POINT('Ctrl Pts',(-13.4999999999961,46.2196721389242,
-57.264521818319));
#137502=CARTESIAN_POINT('Ctrl Pts',(-13.4999999999986,46.1805716042443,
-57.1778714284216));
#137503=CARTESIAN_POINT('Ctrl Pts',(-13.4999999999971,46.1367457679121,
-57.0938423224747));
#137504=CARTESIAN_POINT('Ctrl Pts',(-13.4999999999963,46.1131655316067,
-57.048630950814));
#137505=CARTESIAN_POINT('Ctrl Pts',(-13.4999999999953,46.0882165583818,
-57.0041788421782));
#137506=CARTESIAN_POINT('Ctrl Pts',(-13.4999999999852,46.0619014378574,
-56.9604643403199));
#137507=CARTESIAN_POINT('Ctrl Pts',(-13.499999999984,46.0587398032398,-56.9552122540816));
#137508=CARTESIAN_POINT('Ctrl Pts',(-13.4999999999826,46.0555586143243,
-56.9499710767904));
#137509=CARTESIAN_POINT('Ctrl Pts',(-13.4999999999808,46.0523578866491,
-56.9447407904478));
#137510=CARTESIAN_POINT('Ctrl Pts',(-13.4999999999437,45.9841670777506,
-56.8333106743423));
#137511=CARTESIAN_POINT('Ctrl Pts',(-13.4999999995698,45.9062654719925,
-56.7259689765242));
#137512=CARTESIAN_POINT('Ctrl Pts',(-13.4999999997703,45.8207975744209,
-56.6258771140548));
#137513=CARTESIAN_POINT('Ctrl Pts',(-13.4999999997905,45.8121551558504,
-56.6157559364485));
#137514=CARTESIAN_POINT('Ctrl Pts',(-13.4999999998158,45.803435351972,-56.6057089285391));
#137515=CARTESIAN_POINT('Ctrl Pts',(-13.4999999998434,45.7946403691178,
-56.5957393884661));
#137516=CARTESIAN_POINT('Ctrl Pts',(-13.4999999998604,45.7891977407958,
-56.5895699050165));
#137517=CARTESIAN_POINT('Ctrl Pts',(-13.4999999998752,45.7837267069276,
-56.5834303340926));
#137518=CARTESIAN_POINT('Ctrl Pts',(-13.4999999998881,45.7782278023011,
-56.5773214434301));
#137519=CARTESIAN_POINT('Ctrl Pts',(-13.5000000001116,45.6828400874147,
-56.4713524986363));
#137520=CARTESIAN_POINT('Ctrl Pts',(-13.5000000000272,45.5794120988332,
-56.3745067808491));
#137521=CARTESIAN_POINT('Ctrl Pts',(-13.4999999999695,45.4679575974401,
-56.2866310284186));
#137522=CARTESIAN_POINT('Ctrl Pts',(-13.4999999999653,45.4599257124734,
-56.2802983282937));
#137523=CARTESIAN_POINT('Ctrl Pts',(-13.4999999999594,45.4518518043016,
-56.2740118496438));
#137524=CARTESIAN_POINT('Ctrl Pts',(-13.4999999999509,45.443735968515,-56.2677716701563));
#137525=CARTESIAN_POINT('Ctrl Pts',(-13.4999999998703,45.3663292591539,
-56.2082544777619));
#137526=CARTESIAN_POINT('Ctrl Pts',(-13.4999999992365,45.2845712727005,
-56.1527648487186));
#137527=CARTESIAN_POINT('Ctrl Pts',(-13.4999999991445,45.2001155591245,
-56.1023854625873));
#137528=CARTESIAN_POINT('Ctrl Pts',(-13.4999999991047,45.1634675983669,
-56.0805242801078));
#137529=CARTESIAN_POINT('Ctrl Pts',(-13.4999999992486,45.1263121785351,
-56.0596248906736));
#137530=CARTESIAN_POINT('Ctrl Pts',(-13.4999999995196,45.0887860427418,
-56.0397731680737));
#137531=CARTESIAN_POINT('Ctrl Pts',(-13.4999999995982,45.0778983802498,
-56.0340134794998));
#137532=CARTESIAN_POINT('Ctrl Pts',(-13.4999999996575,45.0669811451102,
-56.0283421588346));
#137533=CARTESIAN_POINT('Ctrl Pts',(-13.4999999997046,45.0560369222135,
-56.022760797256));
#137534=CARTESIAN_POINT('Ctrl Pts',(-13.4999999999911,44.9893496905534,
-55.9887514796382));
#137535=CARTESIAN_POINT('Ctrl Pts',(-13.4999999999377,44.9212851553075,
-55.9578058140964));
#137536=CARTESIAN_POINT('Ctrl Pts',(-13.4999999999181,44.8519312666028,
-55.929946672226));
#137537=CARTESIAN_POINT('Ctrl Pts',(-13.4999999999016,44.7935541183746,
-55.9064968371143));
#137538=CARTESIAN_POINT('Ctrl Pts',(-13.4999999998496,44.7342628547594,
-55.8852345670545));
#137539=CARTESIAN_POINT('Ctrl Pts',(-13.4999999998385,44.6741009867898,
-55.8662006918549));
#137540=CARTESIAN_POINT('Ctrl Pts',(-13.4999999998288,44.62199348368,-55.8497150383234));
#137541=CARTESIAN_POINT('Ctrl Pts',(-13.4999999998617,44.5690884019707,
-55.834861773659));
#137542=CARTESIAN_POINT('Ctrl Pts',(-13.4999999998979,44.5156559887649,
-55.8217533863187));
#137543=CARTESIAN_POINT('Ctrl Pts',(-13.4999999999339,44.4624243034299,
-55.808694242846));
#137544=CARTESIAN_POINT('Ctrl Pts',(-13.4999999999687,44.4086696615078,
-55.7973670287965));
#137545=CARTESIAN_POINT('Ctrl Pts',(-13.4999999999845,44.3546736478475,
-55.7878333559404));
#137546=CARTESIAN_POINT('Ctrl Pts',(-13.4999999999965,44.3137472492199,
-55.7806072873986));
#137547=CARTESIAN_POINT('Ctrl Pts',(-13.4999999999993,44.27268252233,-55.7744105877407));
#137548=CARTESIAN_POINT('Ctrl Pts',(-13.4999999999998,44.2316053598049,
-55.7692503840784));
#137549=CARTESIAN_POINT('',(-13.5,46.41999998,-58.24995));
#137550=CARTESIAN_POINT('',(-13.5,29.8836583509375,-91.8408299848543));
#137551=CARTESIAN_POINT('Origin',(-13.5,29.9835150560362,-91.2987164399481));
#137552=CARTESIAN_POINT('',(-13.5,29.5044693674792,-91.1451435916293));
#137553=CARTESIAN_POINT('Ctrl Pts',(-13.5,29.5044693674792,-91.1451435916293));
#137554=CARTESIAN_POINT('Ctrl Pts',(-13.5,29.4871798972865,-91.1818706195726));
#137555=CARTESIAN_POINT('Ctrl Pts',(-13.5,29.4746493543107,-91.2204653406996));
#137556=CARTESIAN_POINT('Ctrl Pts',(-13.5,29.4670724885977,-91.259957519387));
#137557=CARTESIAN_POINT('Ctrl Pts',(-13.5,29.4602667842095,-91.2954302470261));
#137558=CARTESIAN_POINT('Ctrl Pts',(-13.5,29.4574580326191,-91.3316285116295));
#137559=CARTESIAN_POINT('Ctrl Pts',(-13.5000000000001,29.4588194335385,
-91.3678650371612));
#137560=CARTESIAN_POINT('Ctrl Pts',(-13.5000000000001,29.4588222728777,
-91.367940612098));
#137561=CARTESIAN_POINT('Ctrl Pts',(-13.5000000000001,29.4588251305407,
-91.3680161857943));
#137562=CARTESIAN_POINT('Ctrl Pts',(-13.5000000000001,29.4588280065244,
-91.3680917582431));
#137563=CARTESIAN_POINT('Ctrl Pts',(-13.5000000000004,29.4617431600592,
-91.4446934778138));
#137564=CARTESIAN_POINT('Ctrl Pts',(-13.4999999999999,29.483485076552,-91.5200098118263));
#137565=CARTESIAN_POINT('Ctrl Pts',(-13.5000000000001,29.5206532241076,
-91.5861460983069));
#137566=CARTESIAN_POINT('Ctrl Pts',(-13.5000000000001,29.5206776694618,
-91.5861895958997));
#137567=CARTESIAN_POINT('Ctrl Pts',(-13.5000000000001,29.5207021217052,
-91.5862330898687));
#137568=CARTESIAN_POINT('Ctrl Pts',(-13.5000000000001,29.5207265808359,
-91.5862765802124));
#137569=CARTESIAN_POINT('Ctrl Pts',(-13.5000000000003,29.5579279046594,
-91.6524235901087));
#137570=CARTESIAN_POINT('Ctrl Pts',(-13.5,29.6110672833213,-91.710189265371));
#137571=CARTESIAN_POINT('Ctrl Pts',(-13.5,29.6735560708361,-91.7536723853085));
#137572=CARTESIAN_POINT('Ctrl Pts',(-13.5,29.6735766131945,-91.7536866798063));
#137573=CARTESIAN_POINT('Ctrl Pts',(-13.5,29.6735971566538,-91.7537009728318));
#137574=CARTESIAN_POINT('Ctrl Pts',(-13.5,29.6736177012137,-91.753715264385));
#137575=CARTESIAN_POINT('Ctrl Pts',(-13.5,29.6935761704139,-91.7675991112376));
#137576=CARTESIAN_POINT('Ctrl Pts',(-13.5,29.7144903240442,-91.7800410703758));
#137577=CARTESIAN_POINT('Ctrl Pts',(-13.5,29.7361680987988,-91.7910278638481));
#137578=CARTESIAN_POINT('Ctrl Pts',(-13.5,29.7580697930564,-91.8021281448607));
#137579=CARTESIAN_POINT('Ctrl Pts',(-13.5,29.7807523109198,-91.8117435399084));
#137580=CARTESIAN_POINT('Ctrl Pts',(-13.5,29.8040427282676,-91.8198138783841));
#137581=CARTESIAN_POINT('Ctrl Pts',(-13.5,29.826683860785,-91.8276592338433));
#137582=CARTESIAN_POINT('Ctrl Pts',(-13.5,29.8499007708162,-91.8340446948145));
#137583=CARTESIAN_POINT('Ctrl Pts',(-13.5,29.8735386060562,-91.8388665069537));
#137584=CARTESIAN_POINT('Ctrl Pts',(-13.5,29.8769034909808,-91.8395528998831));
#137585=CARTESIAN_POINT('Ctrl Pts',(-13.5,29.88027689369,-91.8402075213397));
#137586=CARTESIAN_POINT('Ctrl Pts',(-13.5,29.8836583509375,-91.8408299848543));
#137587=CARTESIAN_POINT('',(-13.5,29.5462485400348,-91.058247935017));
#137588=CARTESIAN_POINT('Ctrl Pts',(-13.5,29.5462485400348,-91.058247935017));
#137589=CARTESIAN_POINT('Ctrl Pts',(-13.5,29.5320849211775,-91.0870978945881));
#137590=CARTESIAN_POINT('Ctrl Pts',(-13.5,29.5181581265359,-91.1160653155134));
#137591=CARTESIAN_POINT('Ctrl Pts',(-13.5,29.5044693674783,-91.1451435916289));
#137592=CARTESIAN_POINT('Ctrl Pts',(-13.5,44.086908282047,-61.0621827299711));
#137593=CARTESIAN_POINT('Ctrl Pts',(-13.5,39.2774232822218,-71.079001631676));
#137594=CARTESIAN_POINT('Ctrl Pts',(-13.5,34.4431166252676,-81.0837881795346));
#137595=CARTESIAN_POINT('Ctrl Pts',(-13.5,29.5462485400348,-91.058247935017));
#137596=CARTESIAN_POINT('Ctrl Pts',(-13.5,46.41999998,-58.2497627936531));
#137597=CARTESIAN_POINT('Ctrl Pts',(-13.5,46.9199999800001,-58.2497627936531));
#137598=CARTESIAN_POINT('Ctrl Pts',(-13.,46.91999998,-58.2497627936531));
#137599=CARTESIAN_POINT('Ctrl Pts',(-13.5,46.4199999716718,-57.9435058971265));
#137600=CARTESIAN_POINT('Ctrl Pts',(-13.5,46.9198475451862,-57.8823102041449));
#137601=CARTESIAN_POINT('Ctrl Pts',(-13.0001524477397,46.91999998,-57.8822548982638));
#137602=CARTESIAN_POINT('Ctrl Pts',(-13.5,46.363911922201,-57.6403398562409));
#137603=CARTESIAN_POINT('Ctrl Pts',(-13.5000000000013,46.8524085179432,
-57.5185641386525));
#137604=CARTESIAN_POINT('Ctrl Pts',(-13.0003057176052,46.8526943145044,
-57.5184560311191));
#137605=CARTESIAN_POINT('Ctrl Pts',(-13.5,46.1990348882699,-57.2107576948721));
#137606=CARTESIAN_POINT('Ctrl Pts',(-13.4999999999993,46.6543661205181,
-57.0031847607698));
#137607=CARTESIAN_POINT('Ctrl Pts',(-13.0005259614006,46.6548418679923,
-57.0029579960184));
#137608=CARTESIAN_POINT('Ctrl Pts',(-13.5,46.1317137634759,-57.0744145874655));
#137609=CARTESIAN_POINT('Ctrl Pts',(-13.5000000000001,46.5735338055633,
-56.8396334804064));
#137610=CARTESIAN_POINT('Ctrl Pts',(-13.0005963858014,46.5740565196337,
-56.8393464452647));
#137611=CARTESIAN_POINT('Ctrl Pts',(-13.5,45.9729945411748,-56.8150715642796));
#137612=CARTESIAN_POINT('Ctrl Pts',(-13.4999999999999,46.3829981626758,
-56.5285611340859));
#137613=CARTESIAN_POINT('Ctrl Pts',(-13.0007311732941,46.3835934539471,
-56.5281351595755));
#137614=CARTESIAN_POINT('Ctrl Pts',(-13.5,45.8804524549659,-56.6909184744131));
#137615=CARTESIAN_POINT('Ctrl Pts',(-13.4999999999992,46.2719244986749,
-56.3796526797414));
#137616=CARTESIAN_POINT('Ctrl Pts',(-13.0007961467471,46.2725429511699,
-56.3791516167841));
#137617=CARTESIAN_POINT('Ctrl Pts',(-13.5,45.6759874229978,-56.4637385666375));
#137618=CARTESIAN_POINT('Ctrl Pts',(-13.5000000000008,46.0265477969208,
-56.1071944318285));
#137619=CARTESIAN_POINT('Ctrl Pts',(-13.0009156805798,46.0271849103864,
-56.1065360355095));
#137620=CARTESIAN_POINT('Ctrl Pts',(-13.5,45.5644586309065,-56.3605915480362));
#137621=CARTESIAN_POINT('Ctrl Pts',(-13.5,45.892718112414,-55.9834952073023));
#137622=CARTESIAN_POINT('Ctrl Pts',(-13.0009702923331,45.8933503604458,
-55.9827597531144));
#137623=CARTESIAN_POINT('Ctrl Pts',(-13.5,45.3230047666778,-56.1749628998404));
#137624=CARTESIAN_POINT('Ctrl Pts',(-13.5,45.6030118434335,-55.7608945639374));
#137625=CARTESIAN_POINT('Ctrl Pts',(-13.0010689871371,45.6036057246554,
-55.7600056274797));
#137626=CARTESIAN_POINT('Ctrl Pts',(-13.5,45.1917816064929,-56.0920265457655));
#137627=CARTESIAN_POINT('Ctrl Pts',(-13.5,45.4455768559353,-55.6614429290966));
#137628=CARTESIAN_POINT('Ctrl Pts',(-13.0011133171869,45.4461379323356,
-55.6604821166903));
#137629=CARTESIAN_POINT('Ctrl Pts',(-13.5,44.7845241217188,-55.8842752341532));
#137630=CARTESIAN_POINT('Ctrl Pts',(-13.5,44.9570225707288,-55.4123450088757));
#137631=CARTESIAN_POINT('Ctrl Pts',(-13.0012246935303,44.9574289489744,
-55.4111808336381));
#137632=CARTESIAN_POINT('Ctrl Pts',(-13.5,44.4886526268701,-55.795999572546));
#137633=CARTESIAN_POINT('Ctrl Pts',(-13.4999999999989,44.6020983302816,
-55.3064963379004));
#137634=CARTESIAN_POINT('Ctrl Pts',(-13.0012724779463,44.6023831565444,
-55.3052501647884));
#137635=CARTESIAN_POINT('Ctrl Pts',(-13.5,44.1833084789809,-55.7636597096568));
#137636=CARTESIAN_POINT('Ctrl Pts',(-13.5,44.2358346644988,-55.2677218601875));
#137637=CARTESIAN_POINT('Ctrl Pts',(-13.0012899687735,44.235970178777,-55.2664423715086));
#137638=CARTESIAN_POINT('',(-13.,46.91999998,-58.2497627936531));
#137639=CARTESIAN_POINT('Ctrl Pts',(-13.0012809038513,44.3884784473357,
-55.2865609247418));
#137640=CARTESIAN_POINT('Ctrl Pts',(-13.0012586427657,44.7007920382812,
-55.3359516716537));
#137641=CARTESIAN_POINT('Ctrl Pts',(-13.0012143439801,45.00284180769,-55.4343469392968));
#137642=CARTESIAN_POINT('Ctrl Pts',(-13.0011133171869,45.4461379323356,
-55.6604821166903));
#137643=CARTESIAN_POINT('Ctrl Pts',(-13.0010689871371,45.6036057246554,
-55.7600056274797));
#137644=CARTESIAN_POINT('Ctrl Pts',(-13.0009702923331,45.8933503604458,
-55.9827597531144));
#137645=CARTESIAN_POINT('Ctrl Pts',(-13.0009156805798,46.0271849103864,
-56.1065360355095));
#137646=CARTESIAN_POINT('Ctrl Pts',(-13.0007961467471,46.2725429511699,
-56.3791516167841));
#137647=CARTESIAN_POINT('Ctrl Pts',(-13.0007311732941,46.3835934539471,
-56.5281351595755));
#137648=CARTESIAN_POINT('Ctrl Pts',(-13.0005963858014,46.5740565196337,
-56.8393464452647));
#137649=CARTESIAN_POINT('Ctrl Pts',(-13.0005259614006,46.6548418679923,
-57.0029579960184));
#137650=CARTESIAN_POINT('Ctrl Pts',(-13.0003057176052,46.8526943145044,
-57.5184560311191));
#137651=CARTESIAN_POINT('Ctrl Pts',(-13.0001524477397,46.91999998,-57.8822548982638));
#137652=CARTESIAN_POINT('Ctrl Pts',(-13.,46.91999998,-58.2497627936531));
#137653=CARTESIAN_POINT('Origin',(-13.,46.41999998,-58.2497627936531));
#137654=CARTESIAN_POINT('Ctrl Pts',(-12.4707855792057,46.91999998,-58.2462412559184));
#137655=CARTESIAN_POINT('Ctrl Pts',(-12.4974463012635,46.91999998,-55.7446487532608));
#137656=CARTESIAN_POINT('Ctrl Pts',(-12.5022360800201,44.4589702388884,
-55.2952207669972));
#137657=CARTESIAN_POINT('Ctrl Pts',(-12.6482571751841,46.91999998,-58.2481326596478));
#137658=CARTESIAN_POINT('Ctrl Pts',(-12.669673221037,46.9199999799984,-55.7170654011474));
#137659=CARTESIAN_POINT('Ctrl Pts',(-12.6722965314191,44.424983519038,-55.2908259090656));
#137660=CARTESIAN_POINT('Ctrl Pts',(-12.8257146119078,46.91999998,-58.2493381002745));
#137661=CARTESIAN_POINT('Ctrl Pts',(-12.840428652506,46.9199999800016,-55.6879841619109));
#137662=CARTESIAN_POINT('Ctrl Pts',(-12.841697295306,44.3903034748056,-55.2862462023721));
#137663=CARTESIAN_POINT('Ctrl Pts',(-13.0031560751435,46.91999998,-58.2497705672942));
#137664=CARTESIAN_POINT('Ctrl Pts',(-13.0094744794619,46.91999998,-55.6573244385171));
#137665=CARTESIAN_POINT('Ctrl Pts',(-13.0103905133279,44.3549359954418,
-55.2814750420178));
#137666=CARTESIAN_POINT('',(-12.5,46.91999998,-58.2465463958495));
#137667=CARTESIAN_POINT('Ctrl Pts',(-12.5,46.91999998,-58.2465463958495));
#137668=CARTESIAN_POINT('Ctrl Pts',(-12.5005968089278,46.91999998,-57.8965394261518));
#137669=CARTESIAN_POINT('Ctrl Pts',(-12.5011890520215,46.8598614514991,
-57.5537408849781));
#137670=CARTESIAN_POINT('Ctrl Pts',(-12.5023407943396,46.6211347792778,
-56.8949802448316));
#137671=CARTESIAN_POINT('Ctrl Pts',(-12.5028756040753,46.4475853737583,
-56.5931100772464));
#137672=CARTESIAN_POINT('Ctrl Pts',(-12.503595797933,46.111455620038,-56.190236748787));
#137673=CARTESIAN_POINT('Ctrl Pts',(-12.5038165641686,45.9892097344963,
-56.0674068194903));
#137674=CARTESIAN_POINT('Ctrl Pts',(-12.5042197091625,45.7249560267766,
-55.8439466125607));
#137675=CARTESIAN_POINT('Ctrl Pts',(-12.5044033037043,45.5817611915078,
-55.7426504905235));
#137676=CARTESIAN_POINT('Ctrl Pts',(-12.5048753578165,45.1362912829311,
-55.482949899381));
#137677=CARTESIAN_POINT('Ctrl Pts',(-12.5050937333589,44.8192497088676,
-55.3638128672415));
#137678=CARTESIAN_POINT('Ctrl Pts',(-12.5052115625557,44.4820814550628,
-55.2995670619079));
#137679=CARTESIAN_POINT('Origin',(-13.1654225534,46.91999998,6.33069708304167));
#137680=CARTESIAN_POINT('Ctrl Pts',(-12.5,46.91999998,-58.2465463958495));
#137681=CARTESIAN_POINT('Ctrl Pts',(-12.,46.91999998,-58.2465463958495));
#137682=CARTESIAN_POINT('Ctrl Pts',(-12.,46.41999998,-58.2465463958495));
#137683=CARTESIAN_POINT('Ctrl Pts',(-12.5005968089278,46.91999998,-57.8965394261518));
#137684=CARTESIAN_POINT('Ctrl Pts',(-12.0000000000051,46.9205971329195,
-57.8963321594437));
#137685=CARTESIAN_POINT('Ctrl Pts',(-12.,46.4199999720693,-57.9548688319462));
#137686=CARTESIAN_POINT('Ctrl Pts',(-12.5011890520215,46.8598614514991,
-57.5537408849781));
#137687=CARTESIAN_POINT('Ctrl Pts',(-12.,46.8609831927853,-57.553339017633));
#137688=CARTESIAN_POINT('Ctrl Pts',(-12.,46.3698845360764,-57.6691983000707));
#137689=CARTESIAN_POINT('Ctrl Pts',(-12.5023407943396,46.6211347792778,
-56.8949802448316));
#137690=CARTESIAN_POINT('Ctrl Pts',(-12.,46.6232060214067,-56.8937940810153));
#137691=CARTESIAN_POINT('Ctrl Pts',(-12.,46.170945649571,-57.1202211534365));
#137692=CARTESIAN_POINT('Ctrl Pts',(-12.5028756040753,46.4475853737583,
-56.5931100772464));
#137693=CARTESIAN_POINT('Ctrl Pts',(-11.9999999999992,46.4499499105921,
-56.5914299423666));
#137694=CARTESIAN_POINT('Ctrl Pts',(-12.,46.0263211387953,-56.8686580359845));
#137695=CARTESIAN_POINT('Ctrl Pts',(-12.503595797933,46.111455620038,-56.190236748787));
#137696=CARTESIAN_POINT('Ctrl Pts',(-12.0000000000004,46.1140832559457,
-56.187732860667));
#137697=CARTESIAN_POINT('Ctrl Pts',(-12.,45.7462130147,-56.5329239712738));
#137698=CARTESIAN_POINT('Ctrl Pts',(-12.5038165641686,45.9892097344963,
-56.0674068194903));
#137699=CARTESIAN_POINT('Ctrl Pts',(-12.0000000000004,45.9918445187629,
-56.0645984007596));
#137700=CARTESIAN_POINT('Ctrl Pts',(-12.,45.64434144227,-56.430563765138));
#137701=CARTESIAN_POINT('Ctrl Pts',(-12.5042197091625,45.7249560267766,
-55.8439466125607));
#137702=CARTESIAN_POINT('Ctrl Pts',(-11.9999999999996,45.7274985396918,
-55.840523660562));
#137703=CARTESIAN_POINT('Ctrl Pts',(-12.,45.4241300187908,-56.2443433906185));
#137704=CARTESIAN_POINT('Ctrl Pts',(-12.5044033037043,45.5817611915078,
-55.7426504905235));
#137705=CARTESIAN_POINT('Ctrl Pts',(-12.,45.584205738319,-55.7389336239012));
#137706=CARTESIAN_POINT('Ctrl Pts',(-12.,45.3048009887765,-56.159928342783));
#137707=CARTESIAN_POINT('Ctrl Pts',(-12.5048829251119,45.1291501474361,
-55.4787867514921));
#137708=CARTESIAN_POINT('Ctrl Pts',(-12.,45.1310727951979,-55.4742001436884));
#137709=CARTESIAN_POINT('Ctrl Pts',(-12.,44.9276251211566,-55.9400376669437));
#137710=CARTESIAN_POINT('Ctrl Pts',(-12.5051042651495,44.8038662560613,
-55.3580679820572));
#137711=CARTESIAN_POINT('Ctrl Pts',(-12.0000000000043,44.8053592277238,
-55.3530984350278));
#137712=CARTESIAN_POINT('Ctrl Pts',(-12.,44.6565552133068,-55.8394367317102));
#137713=CARTESIAN_POINT('Ctrl Pts',(-12.5052199580625,44.4575274683141,
-55.2949893590463));
#137714=CARTESIAN_POINT('Ctrl Pts',(-12.,44.4584726259965,-55.289799987766));
#137715=CARTESIAN_POINT('Ctrl Pts',(-12.,44.367939553595,-55.7868701958087));
#137716=CARTESIAN_POINT('',(-12.,46.41999998,-58.2465463958495));
#137717=CARTESIAN_POINT('Ctrl Pts',(-12.,44.7862606093016,-55.9010529569358));
#137718=CARTESIAN_POINT('Ctrl Pts',(-12.,44.8788753121625,-55.9352619713505));
#137719=CARTESIAN_POINT('Ctrl Pts',(-11.9999999998966,44.9692347958817,
-55.97494450417));
#137720=CARTESIAN_POINT('Ctrl Pts',(-12.0000000001034,45.0573639465272,
-56.0200426809306));
#137721=CARTESIAN_POINT('Ctrl Pts',(-12.0000000001611,45.0819593060305,
-56.0326288214102));
#137722=CARTESIAN_POINT('Ctrl Pts',(-12.0000000002553,45.106380862283,-56.0456370713463));
#137723=CARTESIAN_POINT('Ctrl Pts',(-12.0000000004528,45.1306289434624,
-56.0590668658914));
#137724=CARTESIAN_POINT('Ctrl Pts',(-12.0000000005851,45.1468544406639,
-56.0680533540261));
#137725=CARTESIAN_POINT('Ctrl Pts',(-12.0000000007159,45.1630095639554,
-56.0772339702066));
#137726=CARTESIAN_POINT('Ctrl Pts',(-12.0000000008214,45.179090134652,-56.0866066905108));
#137727=CARTESIAN_POINT('Ctrl Pts',(-12.0000000011901,45.2352779195468,
-56.1193562988592));
#137728=CARTESIAN_POINT('Ctrl Pts',(-12.0000000011541,45.2902554021734,
-56.1543787808436));
#137729=CARTESIAN_POINT('Ctrl Pts',(-12.0000000008796,45.3436294771403,
-56.1913642361009));
#137730=CARTESIAN_POINT('Ctrl Pts',(-12.0000000006945,45.3796048513584,
-56.2162932975288));
#137731=CARTESIAN_POINT('Ctrl Pts',(-12.0000000004393,45.4148522843585,
-56.242113151159));
#137732=CARTESIAN_POINT('Ctrl Pts',(-12.0000000002603,45.4492603972454,
-56.268719019813));
#137733=CARTESIAN_POINT('Ctrl Pts',(-12.0000000001101,45.478118138608,-56.2910330966957));
#137734=CARTESIAN_POINT('Ctrl Pts',(-12.0000000000612,45.5064639161954,
-56.3139578240496));
#137735=CARTESIAN_POINT('Ctrl Pts',(-12.0000000000338,45.5342394837982,
-56.3374491395215));
#137736=CARTESIAN_POINT('Ctrl Pts',(-11.9999999999739,45.5949303219838,
-56.3887786981631));
#137737=CARTESIAN_POINT('Ctrl Pts',(-12.,45.653197014408,-56.4429844895127));
#137738=CARTESIAN_POINT('Ctrl Pts',(-12.,45.7088856859487,-56.5000343749642));
#137739=CARTESIAN_POINT('Ctrl Pts',(-12.,45.7160867166438,-56.5074114224843));
#137740=CARTESIAN_POINT('Ctrl Pts',(-12.,45.7232446868776,-56.5148359705652));
#137741=CARTESIAN_POINT('Ctrl Pts',(-12.,45.7303593052335,-56.522307900516));
#137742=CARTESIAN_POINT('Ctrl Pts',(-12.,45.7679171901077,-56.5617520239876));
#137743=CARTESIAN_POINT('Ctrl Pts',(-12.,45.8043465692001,-56.6026021164951));
#137744=CARTESIAN_POINT('Ctrl Pts',(-12.,45.8395823893984,-56.6448353261774));
#137745=CARTESIAN_POINT('Ctrl Pts',(-12.,45.8717319797964,-56.6833694197455));
#137746=CARTESIAN_POINT('Ctrl Pts',(-12.,45.9026476453863,-56.7227444562638));
#137747=CARTESIAN_POINT('Ctrl Pts',(-12.,45.9322838293524,-56.7628973708158));
#137748=CARTESIAN_POINT('Ctrl Pts',(-12.,45.9443118404255,-56.7791936558369));
#137749=CARTESIAN_POINT('Ctrl Pts',(-12.,45.9561292093552,-56.7956179994232));
#137750=CARTESIAN_POINT('Ctrl Pts',(-12.,45.9677333561082,-56.8121658958829));
#137751=CARTESIAN_POINT('Ctrl Pts',(-12.,45.9798251441557,-56.8294091849313));
#137752=CARTESIAN_POINT('Ctrl Pts',(-12.,45.9916897000447,-56.846792620521));
#137753=CARTESIAN_POINT('Ctrl Pts',(-12.,46.003328510704,-56.8643184852464));
#137754=CARTESIAN_POINT('Ctrl Pts',(-12.,46.0482762655415,-56.9320013691808));
#137755=CARTESIAN_POINT('Ctrl Pts',(-12.,46.0898342762661,-57.0017828739964));
#137756=CARTESIAN_POINT('Ctrl Pts',(-12.,46.1278764894281,-57.0734367367413));
#137757=CARTESIAN_POINT('Ctrl Pts',(-12.,46.1404078986294,-57.0970400920742));
#137758=CARTESIAN_POINT('Ctrl Pts',(-12.,46.1525581757035,-57.1208464092072));
#137759=CARTESIAN_POINT('Ctrl Pts',(-12.,46.164323905515,-57.144847012895));
#137760=CARTESIAN_POINT('Ctrl Pts',(-12.,46.1884069401606,-57.193973363694));
#137761=CARTESIAN_POINT('Ctrl Pts',(-12.0000000000007,46.2108248057518,
-57.2437789527952));
#137762=CARTESIAN_POINT('Ctrl Pts',(-12.0000000001545,46.2316525803282,
-57.2944049984523));
#137763=CARTESIAN_POINT('Ctrl Pts',(-12.000000000255,46.2452564476152,-57.3274719016808));
#137764=CARTESIAN_POINT('Ctrl Pts',(-12.0000000004148,46.258181019402,-57.3608893383372));
#137765=CARTESIAN_POINT('Ctrl Pts',(-12.0000000005167,46.2704364630794,
-57.3947019825787));
#137766=CARTESIAN_POINT('Ctrl Pts',(-12.0000000006197,46.2828321131732,
-57.4289014548942));
#137767=CARTESIAN_POINT('Ctrl Pts',(-12.0000000006374,46.2944781423923,
-57.4633231278189));
#137768=CARTESIAN_POINT('Ctrl Pts',(-12.0000000004958,46.3053795309571,
-57.4980138584003));
#137769=CARTESIAN_POINT('Ctrl Pts',(-12.0000000001659,46.330773911604,-57.5788246296214));
#137770=CARTESIAN_POINT('Ctrl Pts',(-12.0000000000875,46.3519200542249,
-57.660361761354));
#137771=CARTESIAN_POINT('Ctrl Pts',(-12.0000000000438,46.3688636122319,
-57.7426155626072));
#137772=CARTESIAN_POINT('Ctrl Pts',(-12.,46.3858667849632,-57.8251587681094));
#137773=CARTESIAN_POINT('Ctrl Pts',(-12.0000000000021,46.3986378015382,
-57.9084239530159));
#137774=CARTESIAN_POINT('Ctrl Pts',(-12.0000000000007,46.4071710877912,
-57.9924112496631));
#137775=CARTESIAN_POINT('Ctrl Pts',(-11.9999999999993,46.4157043740442,
-58.0763985463103));
#137776=CARTESIAN_POINT('Ctrl Pts',(-12.,46.41999998,-58.1611082160511));
#137777=CARTESIAN_POINT('Ctrl Pts',(-12.,46.41999998,-58.2465463958495));
#137778=CARTESIAN_POINT('Origin',(-12.5,46.41999998,-58.2465463958495));
#137779=CARTESIAN_POINT('Ctrl Pts',(-11.4131406659365,44.1784219329664,
-60.890075338912));
#137780=CARTESIAN_POINT('Ctrl Pts',(-12.0001420550745,44.0869928457662,
-60.8415158913113));
#137781=CARTESIAN_POINT('Ctrl Pts',(-11.9999999857978,44.6134318801692,
-61.1210441133877));
#137782=CARTESIAN_POINT('Ctrl Pts',(-11.4054134166098,44.2623189763507,
-60.7346949078221));
#137783=CARTESIAN_POINT('Ctrl Pts',(-12.000145286376,44.1531002254807,-60.6958383983959));
#137784=CARTESIAN_POINT('Ctrl Pts',(-11.9999999856108,44.7369792722067,
-60.8879413106956));
#137785=CARTESIAN_POINT('Ctrl Pts',(-11.4017112009619,44.3028668820624,
-60.5618538448931));
#137786=CARTESIAN_POINT('Ctrl Pts',(-12.0001468655555,44.1818517612737,
-60.5455762622013));
#137787=CARTESIAN_POINT('Ctrl Pts',(-11.9999999855212,44.7966973993881,
-60.6286788556915));
#137788=CARTESIAN_POINT('Ctrl Pts',(-11.4024481915019,44.294801171802,-60.3838747332568));
#137789=CARTESIAN_POINT('Ctrl Pts',(-12.0001465537004,44.1760490867645,
-60.3893137401235));
#137790=CARTESIAN_POINT('Ctrl Pts',(-11.9999999855391,44.7848185198866,
-60.3616767025499));
#137791=CARTESIAN_POINT('',(-12.,44.6428767076058,-61.062182729971));
#137792=CARTESIAN_POINT('Origin',(-11.5,44.6428767076058,-61.062182729971));
#137793=CARTESIAN_POINT('Origin',(-12.0000005388085,43.3853963400589,-60.4562959717164));
#137794=CARTESIAN_POINT('Origin',(-12.,-9.33460238845303,-92.34995));
#137795=CARTESIAN_POINT('',(-12.,30.2507177004773,-91.1386408691297));
#137796=CARTESIAN_POINT('Ctrl Pts',(-12.,30.2507177004773,-91.1386408691297));
#137797=CARTESIAN_POINT('Ctrl Pts',(-12.,35.0808027196733,-81.1288017666048));
#137798=CARTESIAN_POINT('Ctrl Pts',(-12.,39.8700874953717,-71.0994389691951));
#137799=CARTESIAN_POINT('Ctrl Pts',(-12.,44.6428767076058,-61.062182729971));
#137800=CARTESIAN_POINT('Ctrl Pts',(-12.,30.7194735506599,-91.84995));
#137801=CARTESIAN_POINT('Ctrl Pts',(-12.,30.6947425199752,-91.84995));
#137802=CARTESIAN_POINT('Ctrl Pts',(-12.,30.6701386971986,-91.8481899526742));
#137803=CARTESIAN_POINT('Ctrl Pts',(-12.,30.6458464406133,-91.8447815200538));
#137804=CARTESIAN_POINT('Ctrl Pts',(-12.,30.6209700785576,-91.841291131929));
#137805=CARTESIAN_POINT('Ctrl Pts',(-12.,30.5964191072391,-91.8360720015142));
#137806=CARTESIAN_POINT('Ctrl Pts',(-12.,30.5723817191875,-91.8291895987897));
#137807=CARTESIAN_POINT('Ctrl Pts',(-12.,30.5485535835649,-91.8223671093754));
#137808=CARTESIAN_POINT('Ctrl Pts',(-12.,30.5252287940053,-91.8139098291041));
#137809=CARTESIAN_POINT('Ctrl Pts',(-12.,30.5026013041074,-91.8038327530221));
#137810=CARTESIAN_POINT('Ctrl Pts',(-12.,30.4932234054493,-91.7996563375783));
#137811=CARTESIAN_POINT('Ctrl Pts',(-12.,30.4839655197029,-91.7952011432061));
#137812=CARTESIAN_POINT('Ctrl Pts',(-12.,30.4748428234451,-91.7904659511164));
#137813=CARTESIAN_POINT('Ctrl Pts',(-12.,30.3998197342529,-91.7515247512294));
#137814=CARTESIAN_POINT('Ctrl Pts',(-12.,30.3342288071963,-91.6940226895201));
#137815=CARTESIAN_POINT('Ctrl Pts',(-12.,30.2865222597932,-91.6234713302197));
#137816=CARTESIAN_POINT('Ctrl Pts',(-12.,30.2626689858469,-91.5881956502075));
#137817=CARTESIAN_POINT('Ctrl Pts',(-12.,30.2434629741256,-91.5500105562497));
#137818=CARTESIAN_POINT('Ctrl Pts',(-12.,30.2294961429083,-91.5100899134078));
#137819=CARTESIAN_POINT('Ctrl Pts',(-12.,30.2155293119778,-91.4701692713854));
#137820=CARTESIAN_POINT('Ctrl Pts',(-12.,30.2066913177853,-91.427825927269));
#137821=CARTESIAN_POINT('Ctrl Pts',(-12.,30.20356593057,-91.3857257541517));
#137822=CARTESIAN_POINT('Ctrl Pts',(-12.,30.2016706004034,-91.360194924649));
#137823=CARTESIAN_POINT('Ctrl Pts',(-12.,30.2018789661756,-91.3345298932575));
#137824=CARTESIAN_POINT('Ctrl Pts',(-12.,30.20409423165,-91.309005170562));
#137825=CARTESIAN_POINT('Ctrl Pts',(-12.,30.2063233672374,-91.2833206337071));
#137826=CARTESIAN_POINT('Ctrl Pts',(-12.,30.2105848815978,-91.2577766407636));
#137827=CARTESIAN_POINT('Ctrl Pts',(-12.,30.2168325161083,-91.232654980275));
#137828=CARTESIAN_POINT('Ctrl Pts',(-12.,30.2228393598885,-91.2085015363114));
#137829=CARTESIAN_POINT('Ctrl Pts',(-12.,30.2306827015458,-91.1847372739699));
#137830=CARTESIAN_POINT('Ctrl Pts',(-12.,30.2403633283693,-91.1616344702758));
#137831=CARTESIAN_POINT('Ctrl Pts',(-12.,30.24360775786,-91.1538916433916));
#137832=CARTESIAN_POINT('Ctrl Pts',(-12.,30.2470588833976,-91.1462233796087));
#137833=CARTESIAN_POINT('Ctrl Pts',(-12.,30.2507177004773,-91.1386408691297));
#137834=CARTESIAN_POINT('',(-12.,46.41999998,-92.34995));
#137835=CARTESIAN_POINT('Origin',(0.,-12.9675000200281,-60.64995));
#137836=CARTESIAN_POINT('Ctrl Pts',(-11.4112929481563,44.1984900402045,
-60.8508735991007));
#137837=CARTESIAN_POINT('Ctrl Pts',(-11.4042255504145,39.4271199662976,
-70.8881122426161));
#137838=CARTESIAN_POINT('Ctrl Pts',(-11.3956361798112,34.6396513996494,
-80.9174913671817));
#137839=CARTESIAN_POINT('Ctrl Pts',(-11.3834743397155,29.812801930373,-90.9273317382593));
#137840=CARTESIAN_POINT('Ctrl Pts',(-5.44427033638568,30.9653765476951,
-90.9273317382593));
#137841=CARTESIAN_POINT('Ctrl Pts',(-5.4500940393161,35.6738220550387,-80.9051511012611));
#137842=CARTESIAN_POINT('Ctrl Pts',(-5.45419794131935,40.3738290579191,
-70.8788685457756));
#137843=CARTESIAN_POINT('Ctrl Pts',(-5.45757488824865,45.0702713246265,
-60.8508735991007));
#137844=CARTESIAN_POINT('Ctrl Pts',(-5.4533007853959,45.1647773033082,-60.42825533736));
#137845=CARTESIAN_POINT('Ctrl Pts',(-5.,45.2073007626125,-60.42825533736));
#137846=CARTESIAN_POINT('Ctrl Pts',(-5.,45.6625917098448,-60.42825533736));
#137847=CARTESIAN_POINT('Ctrl Pts',(-5.45330078693253,45.1647773031641,
-60.574158272758));
#137848=CARTESIAN_POINT('Ctrl Pts',(-5.00000000000228,45.2073007505585,
-60.5804098497461));
#137849=CARTESIAN_POINT('Ctrl Pts',(-5.,45.6625916931772,-60.6471114271654));
#137850=CARTESIAN_POINT('Ctrl Pts',(-5.45472878287372,45.1330538591303,
-60.717398791161));
#137851=CARTESIAN_POINT('Ctrl Pts',(-4.99999999999914,45.1727790578482,
-60.730071400192));
#137852=CARTESIAN_POINT('Ctrl Pts',(-5.,45.6152082879987,-60.8619682722934));
#137853=CARTESIAN_POINT('Ctrl Pts',(-5.45757488824865,45.0702713246265,
-60.8508735991007));
#137854=CARTESIAN_POINT('Ctrl Pts',(-4.99999999999999,45.1055585268382,
-60.8674008824012));
#137855=CARTESIAN_POINT('Ctrl Pts',(-5.,45.5214348882082,-61.0621827299711));
#137856=CARTESIAN_POINT('',(-5.,45.5214348882082,-61.062182729971));
#137857=CARTESIAN_POINT('Origin',(-5.00000000000003,43.4682849809988,-60.27593181757));
#137858=CARTESIAN_POINT('Origin',(-5.5,45.5214348882082,-61.062182729971));
#137859=CARTESIAN_POINT('Origin',(-5.,-9.33460238845303,-92.34995));
#137860=CARTESIAN_POINT('',(-5.,46.41999998,-57.9428177527387));
#137861=CARTESIAN_POINT('Ctrl Pts',(-5.,46.41999998,-57.9428177527387));
#137862=CARTESIAN_POINT('Ctrl Pts',(-5.,46.41999998,-57.7745740624592));
#137863=CARTESIAN_POINT('Ctrl Pts',(-5.00000000017611,46.4033211412152,
-57.6091706164621));
#137864=CARTESIAN_POINT('Ctrl Pts',(-4.99999999982344,46.3703757696924,
-57.4465347800693));
#137865=CARTESIAN_POINT('Ctrl Pts',(-4.99999999972182,46.3608819639002,
-57.3996683167638));
#137866=CARTESIAN_POINT('Ctrl Pts',(-4.9999999996722,46.3500332431698,-57.3530322594102));
#137867=CARTESIAN_POINT('Ctrl Pts',(-4.99999999969245,46.3378403217705,
-57.3066263304899));
#137868=CARTESIAN_POINT('Ctrl Pts',(-4.99999999973771,46.3105877995303,
-57.202903968263));
#137869=CARTESIAN_POINT('Ctrl Pts',(-4.99999999996081,46.2762003337234,
-57.0996231221188));
#137870=CARTESIAN_POINT('Ctrl Pts',(-4.9999999999857,46.2356732197596,-56.9999496853278));
#137871=CARTESIAN_POINT('Ctrl Pts',(-4.99999999998832,46.2314106238701,
-56.9894661462744));
#137872=CARTESIAN_POINT('Ctrl Pts',(-4.99999999999009,46.2270807552915,
-56.9790199139327));
#137873=CARTESIAN_POINT('Ctrl Pts',(-4.99999999999128,46.2226837784916,
-56.9686108996226));
#137874=CARTESIAN_POINT('Ctrl Pts',(-5.00000000000135,46.1852595852369,
-56.8800161717309));
#137875=CARTESIAN_POINT('Ctrl Pts',(-5.00000000035917,46.1429808775709,
-56.7941365878385));
#137876=CARTESIAN_POINT('Ctrl Pts',(-4.99999999927331,46.0959886291946,
-56.7109637993559));
#137877=CARTESIAN_POINT('Ctrl Pts',(-4.99999999847595,46.061481441272,-56.6498886403374));
#137878=CARTESIAN_POINT('Ctrl Pts',(-4.9999999969677,46.0241995329013,-56.5900309298165));
#137879=CARTESIAN_POINT('Ctrl Pts',(-4.9999999904409,45.9844424230139,-56.5317775549116));
#137880=CARTESIAN_POINT('Ctrl Pts',(-4.99999998658713,45.9609677338277,
-56.4973816978229));
#137881=CARTESIAN_POINT('Ctrl Pts',(-4.99999998917526,45.9365437147868,
-56.4634809785609));
#137882=CARTESIAN_POINT('Ctrl Pts',(-4.99999999269503,45.9112549501108,
-56.4301707952614));
#137883=CARTESIAN_POINT('Ctrl Pts',(-4.99999999800588,45.8730976568612,
-56.379910276464));
#137884=CARTESIAN_POINT('Ctrl Pts',(-4.99999999856442,45.8329742633927,
-56.3309419284987));
#137885=CARTESIAN_POINT('Ctrl Pts',(-4.99999999917036,45.7911678591844,
-56.2836825816832));
#137886=CARTESIAN_POINT('Ctrl Pts',(-4.99999999955207,45.7648322159121,
-56.2539118964834));
#137887=CARTESIAN_POINT('Ctrl Pts',(-4.99999999973279,45.7378296447701,
-56.2248189288369));
#137888=CARTESIAN_POINT('Ctrl Pts',(-4.99999999986749,45.7102390019053,
-56.1965009486372));
#137889=CARTESIAN_POINT('Ctrl Pts',(-4.99999999994411,45.6945455669802,
-56.1803938074714));
#137890=CARTESIAN_POINT('Ctrl Pts',(-5.,45.6786637148754,-56.1645219339327));
#137891=CARTESIAN_POINT('Ctrl Pts',(-5.,45.6625994185597,-56.1488914421297));
#137892=CARTESIAN_POINT('',(-5.,46.41999998,-57.9628508566217));
#137893=CARTESIAN_POINT('',(-5.,31.415090518797,-91.1386408691297));
#137894=CARTESIAN_POINT('Ctrl Pts',(-5.,31.415090518797,-91.1386408691297));
#137895=CARTESIAN_POINT('Ctrl Pts',(-5.,31.3430615709327,-91.2919348798756));
#137896=CARTESIAN_POINT('Ctrl Pts',(-5.,31.355929990322,-91.4779432828738));
#137897=CARTESIAN_POINT('Ctrl Pts',(-5.,31.5391820921123,-91.7616382083514));
#137898=CARTESIAN_POINT('Ctrl Pts',(-5.,31.7023337675853,-91.84995));
#137899=CARTESIAN_POINT('Ctrl Pts',(-5.,31.8716754827171,-91.84995));
#137900=CARTESIAN_POINT('Ctrl Pts',(-5.,45.5214348882082,-61.0621827299711));
#137901=CARTESIAN_POINT('Ctrl Pts',(-5.,40.8246742459034,-71.0901794372786));
#137902=CARTESIAN_POINT('Ctrl Pts',(-5.,36.1242566254946,-81.1164625478583));
#137903=CARTESIAN_POINT('Ctrl Pts',(-5.,31.4150905187971,-91.1386408691297));
#137904=CARTESIAN_POINT('Ctrl Pts',(-5.,46.41999998,-57.9428177527387));
#137905=CARTESIAN_POINT('Ctrl Pts',(-4.99999999999999,46.91999998,-57.9428177527387));
#137906=CARTESIAN_POINT('Ctrl Pts',(-4.5,46.91999998,-57.9428177527387));
#137907=CARTESIAN_POINT('Ctrl Pts',(-5.,46.4199999741246,-57.7261203908743));
#137908=CARTESIAN_POINT('Ctrl Pts',(-4.99999999999699,46.9183271035242,
-57.6832796231231));
#137909=CARTESIAN_POINT('Ctrl Pts',(-4.50167566539267,46.91999998,-57.6828458026853));
#137910=CARTESIAN_POINT('Ctrl Pts',(-5.,46.3923260879484,-57.5140768479069));
#137911=CARTESIAN_POINT('Ctrl Pts',(-4.99999999999981,46.8836068729329,
-57.4292829235226));
#137912=CARTESIAN_POINT('Ctrl Pts',(-4.50330917749558,46.8867913077729,
-57.4284566847483));
#137913=CARTESIAN_POINT('Ctrl Pts',(-5.,46.310571996574,-57.2029077562381));
#137914=CARTESIAN_POINT('Ctrl Pts',(-5.00000000000009,46.7833158134961,
-57.0568766116336));
#137915=CARTESIAN_POINT('Ctrl Pts',(-4.50569802055499,46.7886864007714,
-57.055145939945));
#137916=CARTESIAN_POINT('Ctrl Pts',(-5.,46.2761936631225,-57.0996254934279));
#137917=CARTESIAN_POINT('Ctrl Pts',(-4.99999999999935,46.7414185265942,
-56.9334556299756));
#137918=CARTESIAN_POINT('Ctrl Pts',(-4.50648947498932,46.7474324008918,
-56.931237732302));
#137919=CARTESIAN_POINT('Ctrl Pts',(-5.,46.1951457708619,-56.9002767254212));
#137920=CARTESIAN_POINT('Ctrl Pts',(-5.00000000000066,46.6430202500091,
-56.6954228782697));
#137921=CARTESIAN_POINT('Ctrl Pts',(-4.50801451396916,46.6501749278894,
-56.6920779475246));
#137922=CARTESIAN_POINT('Ctrl Pts',(-5.,46.1485348528389,-56.8039757263989));
#137923=CARTESIAN_POINT('Ctrl Pts',(-4.99999999999985,46.5866051720245,
-56.5805088850576));
#137924=CARTESIAN_POINT('Ctrl Pts',(-4.50874992208284,46.5942418273256,
-56.5765450470161));
#137925=CARTESIAN_POINT('Ctrl Pts',(-5.,45.9908257800341,-56.5249797415912));
#137926=CARTESIAN_POINT('Ctrl Pts',(-5.00000000000027,46.3962887395937,
-56.2480691534848));
#137927=CARTESIAN_POINT('Ctrl Pts',(-4.51087720078722,46.404990940203,-56.2418316606537));
#137928=CARTESIAN_POINT('Ctrl Pts',(-5.,45.859682945468,-56.349946411749));
#137929=CARTESIAN_POINT('Ctrl Pts',(-4.99999999999943,46.2385095854938,
-56.0395648256266));
#137930=CARTESIAN_POINT('Ctrl Pts',(-4.51220710564129,46.2476195396021,
-56.0318427103247));
#137931=CARTESIAN_POINT('Ctrl Pts',(-5.,45.5607785663138,-56.0430715492057));
#137932=CARTESIAN_POINT('Ctrl Pts',(-5.00000000000056,45.8798007876186,
-55.6745387763548));
#137933=CARTESIAN_POINT('Ctrl Pts',(-4.51453310829638,45.888934282536,-55.6636820506581));
#137934=CARTESIAN_POINT('Ctrl Pts',(-5.,45.3931752587345,-55.909838595577));
#137935=CARTESIAN_POINT('Ctrl Pts',(-5.,45.6790509243108,-55.5161529972778));
#137936=CARTESIAN_POINT('Ctrl Pts',(-4.51553991135993,45.6878102784858,
-55.5038410313454));
#137937=CARTESIAN_POINT('Ctrl Pts',(-5.,45.207055184053,-55.7979884638099));
#137938=CARTESIAN_POINT('Ctrl Pts',(-5.00000000000001,45.4562991060438,
-55.383243356978));
#137939=CARTESIAN_POINT('Ctrl Pts',(-4.51638378732469,45.4644662248635,
-55.3696531657294));
#137940=CARTESIAN_POINT('',(-4.5,46.91999998,-57.9428177527387));
#137941=CARTESIAN_POINT('Ctrl Pts',(-4.51630724703492,45.4845441383302,
-55.3818234144886));
#137942=CARTESIAN_POINT('Ctrl Pts',(-4.51547928405129,45.699880758685,-55.5134714456491));
#137943=CARTESIAN_POINT('Ctrl Pts',(-4.51449818831776,45.8943246894343,
-55.6692148576343));
#137944=CARTESIAN_POINT('Ctrl Pts',(-4.51220714147383,46.2476195389329,
-56.031842710892));
#137945=CARTESIAN_POINT('Ctrl Pts',(-4.51087723667079,46.4049909395646,
-56.2418316611113));
#137946=CARTESIAN_POINT('Ctrl Pts',(-4.50874995804734,46.5942418267665,
-56.5765450473063));
#137947=CARTESIAN_POINT('Ctrl Pts',(-4.50801454996146,46.650174927366,-56.6920779477693));
#137948=CARTESIAN_POINT('Ctrl Pts',(-4.50648951103895,46.7474324004525,
-56.931237732464));
#137949=CARTESIAN_POINT('Ctrl Pts',(-4.50569805663421,46.7886864003794,
-57.0551459400713));
#137950=CARTESIAN_POINT('Ctrl Pts',(-4.50330921366347,46.886791307541,-57.4284566848085));
#137951=CARTESIAN_POINT('Ctrl Pts',(-4.50167570162058,46.9199999798784,
-57.6828458027168));
#137952=CARTESIAN_POINT('Ctrl Pts',(-4.5,46.91999998,-57.9428177527387));
#137953=CARTESIAN_POINT('Origin',(-4.5,46.41999998,-57.9428177527387));
#137954=CARTESIAN_POINT('Ctrl Pts',(-3.92215684205867,46.91999998,-57.921448793088));
#137955=CARTESIAN_POINT('Ctrl Pts',(-3.98080144737804,46.91999998,-56.25271405939));
#137956=CARTESIAN_POINT('Ctrl Pts',(-4.0117049092053,45.5008851266717,-55.3733547413106));
#137957=CARTESIAN_POINT('Ctrl Pts',(-4.11592937444032,46.91999998,-57.928258571556));
#137958=CARTESIAN_POINT('Ctrl Pts',(-4.17733814927362,46.9199999800019,
-56.2502970131512));
#137959=CARTESIAN_POINT('Ctrl Pts',(-4.20907605864164,45.4888071699388,
-55.3727975967628));
#137960=CARTESIAN_POINT('Ctrl Pts',(-4.30969200192382,46.91999998,-57.9354449440051));
#137961=CARTESIAN_POINT('Ctrl Pts',(-4.37353389556205,46.9199999800001,
-56.2475777730216));
#137962=CARTESIAN_POINT('Ctrl Pts',(-4.40621163658902,45.4758414047932,
-55.3721833857804));
#137963=CARTESIAN_POINT('Ctrl Pts',(-4.50344622215482,46.91999998,-57.9429512300502));
#137964=CARTESIAN_POINT('Ctrl Pts',(-4.56924626651609,46.91999998,-56.2445032348437));
#137965=CARTESIAN_POINT('Ctrl Pts',(-4.60306732532639,45.461992503193,-55.3715051982969));
#137966=CARTESIAN_POINT('',(-4.,46.91999998,-57.9242045702762));
#137967=CARTESIAN_POINT('Ctrl Pts',(-4.,46.91999998,-57.9242045702762));
#137968=CARTESIAN_POINT('Ctrl Pts',(-4.00152248707584,46.91999998,-57.6677551135179));
#137969=CARTESIAN_POINT('Ctrl Pts',(-4.00300631304518,46.8876664373662,
-57.4167435210981));
#137970=CARTESIAN_POINT('Ctrl Pts',(-4.00589913432669,46.76036485013,-56.9254492364038));
#137971=CARTESIAN_POINT('Ctrl Pts',(-4.00730581971222,46.6642417866207,
-56.6855258491379));
#137972=CARTESIAN_POINT('Ctrl Pts',(-4.00988782131373,46.4183727996822,
-56.2436081635303));
#137973=CARTESIAN_POINT('Ctrl Pts',(-4.01109981373647,46.2651121552776,
-56.0353451211632));
#137974=CARTESIAN_POINT('Ctrl Pts',(-4.01320487516091,45.9189819724219,
-55.6726195336341));
#137975=CARTESIAN_POINT('Ctrl Pts',(-4.01411057746497,45.7278522136539,
-55.5160338046631));
#137976=CARTESIAN_POINT('Ctrl Pts',(-4.01487932239371,45.5159631499936,
-55.3828830175977));
#137977=CARTESIAN_POINT('Ctrl Pts',(-4.,46.91999998,-57.9242045702762));
#137978=CARTESIAN_POINT('Ctrl Pts',(-4.16667353124555,46.91999998,-57.9301478976981));
#137979=CARTESIAN_POINT('Ctrl Pts',(-4.33333987978916,46.91999998,-57.9363643903873));
#137980=CARTESIAN_POINT('Ctrl Pts',(-4.5,46.91999998,-57.9428177527387));
#137981=CARTESIAN_POINT('Ctrl Pts',(-4.,46.91999998,-57.9242045702762));
#137982=CARTESIAN_POINT('Ctrl Pts',(-3.5,46.91999998,-57.9242045702762));
#137983=CARTESIAN_POINT('Ctrl Pts',(-3.5,46.41999998,-57.9242045702762));
#137984=CARTESIAN_POINT('Ctrl Pts',(-4.00152248707584,46.91999998,-57.6677551135179));
#137985=CARTESIAN_POINT('Ctrl Pts',(-3.49999999999684,46.9215247752432,
-57.6673651906402));
#137986=CARTESIAN_POINT('Ctrl Pts',(-3.5,46.4199999742014,-57.7104514486517));
#137987=CARTESIAN_POINT('Ctrl Pts',(-4.00300631304518,46.8876664373662,
-57.4167435210981));
#137988=CARTESIAN_POINT('Ctrl Pts',(-3.50000000000037,46.8905945241102,
-57.4159945765447));
#137989=CARTESIAN_POINT('Ctrl Pts',(-3.5,46.3930553625334,-57.5012311233074));
#137990=CARTESIAN_POINT('Ctrl Pts',(-4.00589913432669,46.76036485013,-56.9254492364038));
#137991=CARTESIAN_POINT('Ctrl Pts',(-3.49999999999963,46.7659528393486,
-56.9232257271801));
#137992=CARTESIAN_POINT('Ctrl Pts',(-3.5,46.2869707037134,-57.0917336115785));
#137993=CARTESIAN_POINT('Ctrl Pts',(-4.00730581971222,46.6642417866207,
-56.6855258491379));
#137994=CARTESIAN_POINT('Ctrl Pts',(-3.50000000000004,46.6709152176612,
-56.6822760272594));
#137995=CARTESIAN_POINT('Ctrl Pts',(-3.5,46.2068681522152,-56.8917559154199));
#137996=CARTESIAN_POINT('Ctrl Pts',(-4.00988782131373,46.4183727996822,
-56.2436081635303));
#137997=CARTESIAN_POINT('Ctrl Pts',(-3.49999999999995,46.4266646204127,
-56.237771148346));
#137998=CARTESIAN_POINT('Ctrl Pts',(-3.5,46.0019773297039,-56.5234150618225));
#137999=CARTESIAN_POINT('Ctrl Pts',(-4.01109981373647,46.2651121552776,
-56.0353451211632));
#138000=CARTESIAN_POINT('Ctrl Pts',(-3.50000000000055,46.2738584100651,
-56.0280733151404));
#138001=CARTESIAN_POINT('Ctrl Pts',(-3.5,45.8742601250717,-56.3498268696058));
#138002=CARTESIAN_POINT('Ctrl Pts',(-4.01323028458345,45.9148039622378,
-55.6682412064214));
#138003=CARTESIAN_POINT('Ctrl Pts',(-3.49999999999944,45.923712698628,-55.6579003398743));
#138004=CARTESIAN_POINT('Ctrl Pts',(-3.5,45.5823366328578,-56.0438443443254));
#138005=CARTESIAN_POINT('Ctrl Pts',(-4.01415476126711,45.7184991995766,
-55.5083945642206));
#138006=CARTESIAN_POINT('Ctrl Pts',(-3.50000000000342,45.7271164793515,
-55.4966052387911));
#138007=CARTESIAN_POINT('Ctrl Pts',(-3.5,45.4187493558633,-55.9106117044594));
#138008=CARTESIAN_POINT('Ctrl Pts',(-4.01493543718735,45.5003931325255,
-55.3731631297134));
#138009=CARTESIAN_POINT('Ctrl Pts',(-3.49999999999999,45.5085033459109,
-55.3600853439128));
#138010=CARTESIAN_POINT('Ctrl Pts',(-3.5,45.2369942737712,-55.7978959562326));
#138011=CARTESIAN_POINT('',(-3.5,46.41999998,-57.9242045702762));
#138012=CARTESIAN_POINT('Ctrl Pts',(-3.50000000506663,45.8435334367288,
-56.3263223051818));
#138013=CARTESIAN_POINT('Ctrl Pts',(-3.50000001032463,45.8894626566105,
-56.3816811876747));
#138014=CARTESIAN_POINT('Ctrl Pts',(-3.50000001775255,45.9328922004512,
-56.4388763829609));
#138015=CARTESIAN_POINT('Ctrl Pts',(-3.50000002291889,45.9736813029623,
-56.4976009415834));
#138016=CARTESIAN_POINT('Ctrl Pts',(-3.50000002818049,46.0152224330362,
-56.5574082032807));
#138017=CARTESIAN_POINT('Ctrl Pts',(-3.50000003120722,46.0540257195003,
-56.6188027368888));
#138018=CARTESIAN_POINT('Ctrl Pts',(-3.50000003122783,46.0899059446863,
-56.6814984159273));
#138019=CARTESIAN_POINT('Ctrl Pts',(-3.50000003123068,46.0948520295369,
-56.6901410079592));
#138020=CARTESIAN_POINT('Ctrl Pts',(-3.50000003118087,46.0997425008543,
-56.6988083694207));
#138021=CARTESIAN_POINT('Ctrl Pts',(-3.5000000310803,46.1045768057904,-56.7074997895477));
#138022=CARTESIAN_POINT('Ctrl Pts',(-3.50000003035461,46.1394632249472,
-56.7702208072801));
#138023=CARTESIAN_POINT('Ctrl Pts',(-3.50000002687238,46.1717681199833,
-56.8347988963915));
#138024=CARTESIAN_POINT('Ctrl Pts',(-3.50000002225516,46.2013495572015,
-56.9009409523226));
#138025=CARTESIAN_POINT('Ctrl Pts',(-3.5000000182853,46.2267835376252,-56.957809580555));
#138026=CARTESIAN_POINT('Ctrl Pts',(-3.50000001353393,46.2502037235481,
-57.0158352648144));
#138027=CARTESIAN_POINT('Ctrl Pts',(-3.50000000945277,46.2714898142467,
-57.0748386052854));
#138028=CARTESIAN_POINT('Ctrl Pts',(-3.50000000440193,46.2978334233143,
-57.1478609820601));
#138029=CARTESIAN_POINT('Ctrl Pts',(-3.5000000025334,46.3207458812431,-57.221900953307));
#138030=CARTESIAN_POINT('Ctrl Pts',(-3.50000000146594,46.3400500971326,
-57.2964727656199));
#138031=CARTESIAN_POINT('Ctrl Pts',(-3.50000000013692,46.3640841940101,
-57.3893160166336));
#138032=CARTESIAN_POINT('Ctrl Pts',(-3.5000000001043,46.3827251371296,-57.4829234266614));
#138033=CARTESIAN_POINT('Ctrl Pts',(-3.50000000003929,46.3959468792823,
-57.5774099701229));
#138034=CARTESIAN_POINT('Ctrl Pts',(-3.49999999997472,46.4090811642661,
-57.6712715183691));
#138035=CARTESIAN_POINT('Ctrl Pts',(-3.50000000000001,46.4168677320184,
-57.7660006115246));
#138036=CARTESIAN_POINT('Ctrl Pts',(-3.5,46.4192300563852,-57.8617170363508));
#138037=CARTESIAN_POINT('Ctrl Pts',(-3.5,46.4197429699982,-57.882499219346));
#138038=CARTESIAN_POINT('Ctrl Pts',(-3.5,46.41999998,-57.9033279738498));
#138039=CARTESIAN_POINT('Ctrl Pts',(-3.5,46.41999998,-57.9242045702762));
#138040=CARTESIAN_POINT('Origin',(-4.,46.41999998,-57.9242045702762));
#138041=CARTESIAN_POINT('Origin',(-3.5,-9.33460238845303,-92.34995));
#138042=CARTESIAN_POINT('',(-3.5,46.41999998,-92.34995));
#138043=CARTESIAN_POINT('Origin',(-60.,11.11999998,-55.74995));
#138044=CARTESIAN_POINT('',(-57.,11.11999998,-55.24995));
#138045=CARTESIAN_POINT('',(-60.,11.11999998,-55.24995));
#138046=CARTESIAN_POINT('',(-57.,10.61999998,-55.74995));
#138047=CARTESIAN_POINT('Origin',(-57.,11.11999998,-55.74995));
#138048=CARTESIAN_POINT('',(83.2809572255632,10.6199999800001,-55.74995));
#138049=CARTESIAN_POINT('Origin',(-60.,28.41999998,-55.24995));
#138050=CARTESIAN_POINT('',(-57.,11.61999998,-55.24995));
#138051=CARTESIAN_POINT('',(-60.,11.61999998,-55.24995));
#138052=CARTESIAN_POINT('',(-57.,28.41999998,-55.24995));
#138053=CARTESIAN_POINT('Origin',(83.2809572255632,11.6199999800001,-55.74995));
#138054=CARTESIAN_POINT('',(-57.,12.11999998,-55.74995));
#138055=CARTESIAN_POINT('',(83.2809572255632,12.1199999800001,-55.74995));
#138056=CARTESIAN_POINT('Origin',(-57.,11.61999998,-55.74995));
#138057=CARTESIAN_POINT('Origin',(-60.,-37.78000002,-55.74995));
#138058=CARTESIAN_POINT('',(-57.,-37.78000002,-55.24995));
#138059=CARTESIAN_POINT('',(-60.,-37.78000002,-55.24995));
#138060=CARTESIAN_POINT('',(-57.,-38.28000002,-55.74995));
#138061=CARTESIAN_POINT('Origin',(-57.,-37.78000002,-55.74995));
#138062=CARTESIAN_POINT('',(83.2809572255632,-38.28000002,-55.74995));
#138063=CARTESIAN_POINT('Origin',(-60.,28.41999998,-55.24995));
#138064=CARTESIAN_POINT('',(-57.,-37.28000002,-55.24995));
#138065=CARTESIAN_POINT('',(-60.,-37.28000002,-55.24995));
#138066=CARTESIAN_POINT('',(-57.,28.41999998,-55.24995));
#138067=CARTESIAN_POINT('Origin',(83.2809572255632,-37.28000002,-55.74995));
#138068=CARTESIAN_POINT('',(-57.,-36.78000002,-55.74995));
#138069=CARTESIAN_POINT('',(83.2809572255632,-36.78000002,-55.74995));
#138070=CARTESIAN_POINT('Origin',(-57.,-37.28000002,-55.74995));
#138071=CARTESIAN_POINT('Origin',(83.2809572255632,-36.78000002,-55.24995));
#138072=CARTESIAN_POINT('',(-57.,-36.78000002,-176.84995));
#138073=CARTESIAN_POINT('',(-54.1989607257493,-36.78000002,-176.84995));
#138074=CARTESIAN_POINT('',(83.2809572255632,-36.78000002,-176.84995));
#138075=CARTESIAN_POINT('',(-59.5,-36.78000002,-174.34995));
#138076=CARTESIAN_POINT('Origin',(-57.,-36.78000002,-174.34995));
#138077=CARTESIAN_POINT('',(-59.5,-36.78000002,-58.24995));
#138078=CARTESIAN_POINT('',(-59.5,-36.78000002,-174.34995));
#138079=CARTESIAN_POINT('Origin',(-57.,-36.78000002,-58.24995));
#138080=CARTESIAN_POINT('',(-53.9233979868778,-36.78000002,-61.0621827299711));
#138081=CARTESIAN_POINT('Origin',(-52.6143300187798,-36.78000002,-60.4624709867148));
#138082=CARTESIAN_POINT('',(-40.4661024946855,-36.78000002,-86.8949524600738));
#138083=CARTESIAN_POINT('Ctrl Pts',(-40.4661024946855,-36.78000002,-86.8949524600738));
#138084=CARTESIAN_POINT('Ctrl Pts',(-42.7668758174593,-36.78000002,-82.6196483790844));
#138085=CARTESIAN_POINT('Ctrl Pts',(-45.0302107640621,-36.78000002,-78.3248411901957));
#138086=CARTESIAN_POINT('Ctrl Pts',(-47.2696870908413,-36.78000002,-74.0176051177503));
#138087=CARTESIAN_POINT('Ctrl Pts',(-49.5091634176204,-36.78000002,-69.7103690453049));
#138088=CARTESIAN_POINT('Ctrl Pts',(-51.7244980141576,-36.78000002,-65.3905566052077));
#138089=CARTESIAN_POINT('Ctrl Pts',(-53.9233979868778,-36.78000002,-61.0621827299711));
#138090=CARTESIAN_POINT('',(-39.5,-36.78000002,-90.9091273827666));
#138091=CARTESIAN_POINT('Ctrl Pts',(-39.5,-36.78000002,-90.9091273827666));
#138092=CARTESIAN_POINT('Ctrl Pts',(-39.5,-36.78000002,-90.7679100061195));
#138093=CARTESIAN_POINT('Ctrl Pts',(-39.5033096444594,-36.7800000200224,
-90.6269761431622));
#138094=CARTESIAN_POINT('Ctrl Pts',(-39.5098707684965,-36.7800000197587,
-90.4863271086497));
#138095=CARTESIAN_POINT('Ctrl Pts',(-39.5164908621435,-36.7800000194927,
-90.3444139586223));
#138096=CARTESIAN_POINT('Ctrl Pts',(-39.5264211472601,-36.7800000188623,
-90.2027900769894));
#138097=CARTESIAN_POINT('Ctrl Pts',(-39.5396544427957,-36.7800000184551,
-90.0614520511805));
#138098=CARTESIAN_POINT('Ctrl Pts',(-39.5457621647725,-36.7800000182671,
-89.9962186129895));
#138099=CARTESIAN_POINT('Ctrl Pts',(-39.5525742276006,-36.780000018147,
-89.931046067388));
#138100=CARTESIAN_POINT('Ctrl Pts',(-39.5600936571067,-36.7800000181768,
-89.8659343821325));
#138101=CARTESIAN_POINT('Ctrl Pts',(-39.5772069508046,-36.7800000182445,
-89.7177482209288));
#138102=CARTESIAN_POINT('Ctrl Pts',(-39.5980137125873,-36.7800000189104,
-89.569651212334));
#138103=CARTESIAN_POINT('Ctrl Pts',(-39.6224903903717,-36.7800000193564,
-89.4222267568288));
#138104=CARTESIAN_POINT('Ctrl Pts',(-39.6467595279693,-36.7800000197985,
-89.2760523279532));
#138105=CARTESIAN_POINT('Ctrl Pts',(-39.6746364995126,-36.780000019972,
-89.1305398192676));
#138106=CARTESIAN_POINT('Ctrl Pts',(-39.7060481712982,-36.780000019994,
-88.9862487847464));
#138107=CARTESIAN_POINT('Ctrl Pts',(-39.716927298473,-36.7800000200016,
-88.9362749875714));
#138108=CARTESIAN_POINT('Ctrl Pts',(-39.7282299820617,-36.78000002,-88.8864475773876));
#138109=CARTESIAN_POINT('Ctrl Pts',(-39.7399518035734,-36.78000002,-88.8367893012138));
#138110=CARTESIAN_POINT('Ctrl Pts',(-39.8212039955528,-36.78000002,-88.492572851151));
#138111=CARTESIAN_POINT('Ctrl Pts',(-39.9220601466534,-36.78000002,-88.1550003033698));
#138112=CARTESIAN_POINT('Ctrl Pts',(-40.0453748819469,-36.78000002,-87.8250390461022));
#138113=CARTESIAN_POINT('Ctrl Pts',(-40.1639808073533,-36.78000002,-87.5076774576977));
#138114=CARTESIAN_POINT('Ctrl Pts',(-40.3033623182004,-36.78000002,-87.1973567576838));
#138115=CARTESIAN_POINT('Ctrl Pts',(-40.4661024946855,-36.78000002,-86.8949524600738));
#138116=CARTESIAN_POINT('',(-39.5,-36.78000002,-141.149515588739));
#138117=CARTESIAN_POINT('',(-39.5,-36.78000002,-55.24995));
#138118=CARTESIAN_POINT('',(-40.4661024946856,-36.78000002,-145.163690511432));
#138119=CARTESIAN_POINT('Ctrl Pts',(-40.4661024946855,-36.78000002,-145.163690511432));
#138120=CARTESIAN_POINT('Ctrl Pts',(-40.4051245273349,-36.78000002,-145.05038106453));
#138121=CARTESIAN_POINT('Ctrl Pts',(-40.3473970436743,-36.78000002,-144.935666150371));
#138122=CARTESIAN_POINT('Ctrl Pts',(-40.2927291183484,-36.78000002,-144.819632460353));
#138123=CARTESIAN_POINT('Ctrl Pts',(-40.2359907375983,-36.78000002,-144.699204190122));
#138124=CARTESIAN_POINT('Ctrl Pts',(-40.1825479091664,-36.78000002,-144.57735479297));
#138125=CARTESIAN_POINT('Ctrl Pts',(-40.1322366185216,-36.78000002,-144.454153170973));
#138126=CARTESIAN_POINT('Ctrl Pts',(-40.0991220934984,-36.78000002,-144.373062760805));
#138127=CARTESIAN_POINT('Ctrl Pts',(-40.0673652289499,-36.78000002,-144.291385980202));
#138128=CARTESIAN_POINT('Ctrl Pts',(-40.0369306905871,-36.78000002,-144.209138150939));
#138129=CARTESIAN_POINT('Ctrl Pts',(-39.9567208320419,-36.78000002,-143.992374989553));
#138130=CARTESIAN_POINT('Ctrl Pts',(-39.8859370925007,-36.78000002,-143.772269498048));
#138131=CARTESIAN_POINT('Ctrl Pts',(-39.8243406671268,-36.78000002,-143.550546349417));
#138132=CARTESIAN_POINT('Ctrl Pts',(-39.7928424603828,-36.78000002,-143.43716506904));
#138133=CARTESIAN_POINT('Ctrl Pts',(-39.7637458267523,-36.78000002,-143.323361070994));
#138134=CARTESIAN_POINT('Ctrl Pts',(-39.737013701299,-36.78000002,-143.209365754044));
#138135=CARTESIAN_POINT('Ctrl Pts',(-39.639900448195,-36.78000002,-142.795240207349));
#138136=CARTESIAN_POINT('Ctrl Pts',(-39.5726401857973,-36.78000002,-142.376286688263));
#138137=CARTESIAN_POINT('Ctrl Pts',(-39.5352116792783,-36.78000002,-141.952508599961));
#138138=CARTESIAN_POINT('Ctrl Pts',(-39.5117389237074,-36.78000002,-141.686742198676));
#138139=CARTESIAN_POINT('Ctrl Pts',(-39.5000000000007,-36.78000002,-141.419078129349));
#138140=CARTESIAN_POINT('Ctrl Pts',(-39.5,-36.78000002,-141.149515588739));
#138141=CARTESIAN_POINT('',(-54.0459394689003,-36.78000002,-171.237717270032));
#138142=CARTESIAN_POINT('Ctrl Pts',(-54.0459394689003,-36.78000002,-171.237717270032));
#138143=CARTESIAN_POINT('Ctrl Pts',(-51.8272412193298,-36.78000002,-166.868813514854));
#138144=CARTESIAN_POINT('Ctrl Pts',(-49.5919157423625,-36.78000002,-162.508569528244));
#138145=CARTESIAN_POINT('Ctrl Pts',(-47.3320947234338,-36.78000002,-158.161083274436));
#138146=CARTESIAN_POINT('Ctrl Pts',(-45.0722737045051,-36.78000002,-153.813597020627));
#138147=CARTESIAN_POINT('Ctrl Pts',(-42.7882516015473,-36.78000002,-149.478715140467));
#138148=CARTESIAN_POINT('Ctrl Pts',(-40.4661024946855,-36.78000002,-145.163690511432));
#138149=CARTESIAN_POINT('',(-54.1989607257493,-36.78000002,-171.871644662643));
#138150=CARTESIAN_POINT('Origin',(-52.6055188872069,-36.7800000520242,-171.864725026464));
#138151=CARTESIAN_POINT('',(-54.1989607257493,-36.78000002,-171.871644662643));
#138152=CARTESIAN_POINT('Ctrl Pts',(-53.5074514076768,-36.1001753985996,
-60.8508735991007));
#138153=CARTESIAN_POINT('Ctrl Pts',(-53.2738374538032,-36.78000002,-60.732193066502));
#138154=CARTESIAN_POINT('Ctrl Pts',(-53.9233979868778,-36.78000002,-61.0621827299711));
#138155=CARTESIAN_POINT('Ctrl Pts',(-53.5793517884845,-36.0882972935914,
-60.7194512531293));
#138156=CARTESIAN_POINT('Ctrl Pts',(-53.3063595996785,-36.7800000199961,
-60.6234805422192));
#138157=CARTESIAN_POINT('Ctrl Pts',(-54.0235433277796,-36.78000002,-60.8650539582955));
#138158=CARTESIAN_POINT('Ctrl Pts',(-53.6173229302591,-36.0820590261091,
-60.5748771537519));
#138159=CARTESIAN_POINT('Ctrl Pts',(-53.3164388644065,-36.7800000200045,
-60.5261947762596));
#138160=CARTESIAN_POINT('Ctrl Pts',(-54.0764736407615,-36.78000002,-60.6481844964965));
#138161=CARTESIAN_POINT('Ctrl Pts',(-53.6173229282256,-36.0820590308261,
-60.42825533736));
#138162=CARTESIAN_POINT('Ctrl Pts',(-53.3164388612998,-36.78000002,-60.42825533736));
#138163=CARTESIAN_POINT('Ctrl Pts',(-54.076473627675,-36.78000002,-60.42825533736));
#138164=CARTESIAN_POINT('Origin',(-53.9233979868778,-36.28000002,-61.0621827299711));
#138165=CARTESIAN_POINT('Origin',(0.,-12.9675000200281,-60.64995));
#138166=CARTESIAN_POINT('',(-40.0734472026555,-36.0537916247009,-86.6836434020945));
#138167=CARTESIAN_POINT('',(-39.850159149164,-30.447965242174,-92.5429803300057));
#138168=CARTESIAN_POINT('Ctrl Pts',(-40.0734472049734,-36.0537916894494,
-86.683643483585));
#138169=CARTESIAN_POINT('Ctrl Pts',(-40.0273699242565,-34.9400863872175,
-87.9615139033166));
#138170=CARTESIAN_POINT('Ctrl Pts',(-39.9805444369969,-33.7936306360731,
-89.2147954597336));
#138171=CARTESIAN_POINT('Ctrl Pts',(-39.9335716691851,-32.6056714694524,
-90.4294303486513));
#138172=CARTESIAN_POINT('Ctrl Pts',(-39.9055799708467,-31.8977507702987,
-91.1532474662255));
#138173=CARTESIAN_POINT('Ctrl Pts',(-39.8776986413925,-31.1793505068417,
-91.8590535072933));
#138174=CARTESIAN_POINT('Ctrl Pts',(-39.8501516349657,-30.4480624602042,
-92.5430839619263));
#138175=CARTESIAN_POINT('Ctrl Pts',(-53.5074514076768,-36.1001753985996,
-60.8508735991007));
#138176=CARTESIAN_POINT('Ctrl Pts',(-51.3114449995927,-36.0939978420838,
-65.1788088203991));
#138177=CARTESIAN_POINT('Ctrl Pts',(-49.0993449598848,-36.0872029674615,
-69.4983516680729));
#138178=CARTESIAN_POINT('Ctrl Pts',(-44.6279666678641,-36.07192692476,-78.1127593263175));
#138179=CARTESIAN_POINT('Ctrl Pts',(-42.3689613386823,-36.0634493757596,
-82.407773086312));
#138180=CARTESIAN_POINT('Ctrl Pts',(-40.0734472163172,-36.0537915241817,
-86.6836433292035));
#138181=CARTESIAN_POINT('Ctrl Pts',(-39.850159149164,-30.447965242174,-92.5429803300057));
#138182=CARTESIAN_POINT('Ctrl Pts',(-42.5227129344255,-30.4581147715466,
-87.2856833539494));
#138183=CARTESIAN_POINT('Ctrl Pts',(-45.1629315870884,-30.4666308723541,
-82.01174695052));
#138184=CARTESIAN_POINT('Ctrl Pts',(-50.405384759569,-30.4815921581836,
-71.4443972343972));
#138185=CARTESIAN_POINT('Ctrl Pts',(-53.0072677069205,-30.4880260434848,
-66.1508000801069));
#138186=CARTESIAN_POINT('Ctrl Pts',(-55.5967474138374,-30.4937575588533,
-60.8508735991007));
#138187=CARTESIAN_POINT('Ctrl Pts',(-55.6982488612463,-30.4801711525811,
-60.3843213671005));
#138188=CARTESIAN_POINT('Ctrl Pts',(-55.8081167820838,-30.1299397177969,
-60.3792327034747));
#138189=CARTESIAN_POINT('Ctrl Pts',(-56.1748536617521,-30.1300000267474,
-60.3623460050376));
#138190=CARTESIAN_POINT('Ctrl Pts',(-55.7066195808876,-30.47905606799,-60.5602959714918));
#138191=CARTESIAN_POINT('Ctrl Pts',(-55.8181378939596,-30.1299399603517,
-60.5754394884542));
#138192=CARTESIAN_POINT('Ctrl Pts',(-56.1868831687146,-30.1300000267259,
-60.6263466339184));
#138193=CARTESIAN_POINT('Ctrl Pts',(-55.6646352974887,-30.4846448609915,
-60.733808800051));
#138194=CARTESIAN_POINT('Ctrl Pts',(-55.7674480546492,-30.1299387371113,
-60.7710090719053));
#138195=CARTESIAN_POINT('Ctrl Pts',(-56.1265462537084,-30.1300000268336,
-60.8865882025091));
#138196=CARTESIAN_POINT('Ctrl Pts',(-55.5754321736229,-30.4966175475299,
-60.8903552940655));
#138197=CARTESIAN_POINT('Ctrl Pts',(-55.6644710959107,-30.1299360711904,
-60.9390296786082));
#138198=CARTESIAN_POINT('Ctrl Pts',(-55.9983862620519,-30.1300000270643,
-61.1214514057001));
#138199=CARTESIAN_POINT('',(-56.0289353856639,-30.13000002,-61.0621827299711));
#138200=CARTESIAN_POINT('Origin',(-54.6965997031483,-30.1299997573522,-60.447263207802));
#138201=CARTESIAN_POINT('Origin',(-56.0289353856639,-30.63000002,-61.0621827299711));
#138202=CARTESIAN_POINT('Origin',(83.2809572255632,-30.13000002,-55.24995));
#138203=CARTESIAN_POINT('',(-57.,-30.13000002,-55.74995));
#138204=CARTESIAN_POINT('',(83.2809572255632,-30.13000002,-55.74995));
#138205=CARTESIAN_POINT('',(-59.5,-30.13000002,-58.24995));
#138206=CARTESIAN_POINT('Origin',(-57.,-30.13000002,-58.24995));
#138207=CARTESIAN_POINT('',(-59.5,-30.13000002,-174.34995));
#138208=CARTESIAN_POINT('',(-59.5,-30.13000002,-58.24995));
#138209=CARTESIAN_POINT('',(-57.,-30.13000002,-176.84995));
#138210=CARTESIAN_POINT('Origin',(-57.,-30.13000002,-174.34995));
#138211=CARTESIAN_POINT('',(-56.294192362543,-30.13000002,-176.84995));
#138212=CARTESIAN_POINT('',(83.2809572255632,-30.13000002,-176.84995));
#138213=CARTESIAN_POINT('',(-56.294192362543,-30.13000002,-171.871644662643));
#138214=CARTESIAN_POINT('',(-56.294192362543,-30.13000002,-176.84995));
#138215=CARTESIAN_POINT('',(-56.1468816861249,-30.13000002,-171.237717270032));
#138216=CARTESIAN_POINT('Origin',(-54.8146431262804,-30.1299997583388,-171.852158294274));
#138217=CARTESIAN_POINT('',(-40.2651432342477,-30.13000002,-139.30435351063));
#138218=CARTESIAN_POINT('Ctrl Pts',(-40.2651432342477,-30.13000002,-139.30435351063));
#138219=CARTESIAN_POINT('Ctrl Pts',(-42.96245845912,-30.13000002,-144.601535351275));
#138220=CARTESIAN_POINT('Ctrl Pts',(-45.6258101137032,-30.13000002,-149.915608633243));
#138221=CARTESIAN_POINT('Ctrl Pts',(-48.2693741701893,-30.13000002,-155.239523078828));
#138222=CARTESIAN_POINT('Ctrl Pts',(-50.9129382266755,-30.13000002,-160.563437524412));
#138223=CARTESIAN_POINT('Ctrl Pts',(-53.5363337714711,-30.13000002,-165.897382577172));
#138224=CARTESIAN_POINT('Ctrl Pts',(-56.1468816861249,-30.13000002,-171.237717270032));
#138225=CARTESIAN_POINT('',(-39.5,-30.13000002,-136.04214564125));
#138226=CARTESIAN_POINT('Ctrl Pts',(-39.5,-30.13000002,-136.04214564125));
#138227=CARTESIAN_POINT('Ctrl Pts',(-39.5,-30.13000002,-136.325718326755));
#138228=CARTESIAN_POINT('Ctrl Pts',(-39.5162728499327,-30.13000002,-136.608122039194));
#138229=CARTESIAN_POINT('Ctrl Pts',(-39.5808560770791,-30.13000002,-137.170628022919));
#138230=CARTESIAN_POINT('Ctrl Pts',(-39.6292470494507,-30.13000002,-137.450036957971));
#138231=CARTESIAN_POINT('Ctrl Pts',(-39.8201451199495,-30.13000002,-138.270288236609));
#138232=CARTESIAN_POINT('Ctrl Pts',(-40.0074751366267,-30.13000002,-138.798326348879));
#138233=CARTESIAN_POINT('Ctrl Pts',(-40.2651432342477,-30.13000002,-139.30435351063));
#138234=CARTESIAN_POINT('',(-39.5,-30.13000002,-96.0164973302555));
#138235=CARTESIAN_POINT('',(-39.5,-30.13000002,-55.24995));
#138236=CARTESIAN_POINT('',(-40.2651432342477,-30.13000002,-92.754289460876));
#138237=CARTESIAN_POINT('Ctrl Pts',(-40.2651432342476,-30.13000002,-92.7542894608761));
#138238=CARTESIAN_POINT('Ctrl Pts',(-40.1497681189566,-30.13000002,-92.980871419087));
#138239=CARTESIAN_POINT('Ctrl Pts',(-40.0478331438212,-30.13000002,-93.2140840893041));
#138240=CARTESIAN_POINT('Ctrl Pts',(-39.9590875376232,-30.13000002,-93.4515644892626));
#138241=CARTESIAN_POINT('Ctrl Pts',(-39.8658509560187,-30.13000002,-93.7010625955778));
#138242=CARTESIAN_POINT('Ctrl Pts',(-39.7871721235835,-30.13000002,-93.9552726783301));
#138243=CARTESIAN_POINT('Ctrl Pts',(-39.7228113496722,-30.13000002,-94.2114776823651));
#138244=CARTESIAN_POINT('Ctrl Pts',(-39.7115691395802,-30.13000002,-94.2562302592367));
#138245=CARTESIAN_POINT('Ctrl Pts',(-39.700763918709,-30.13000002,-94.3010437266483));
#138246=CARTESIAN_POINT('Ctrl Pts',(-39.6903945692724,-30.13000002,-94.3459036197334));
#138247=CARTESIAN_POINT('Ctrl Pts',(-39.604671908225,-30.13000002,-94.7167571079927));
#138248=CARTESIAN_POINT('Ctrl Pts',(-39.5475807634113,-30.13000002,-95.0925075650422));
#138249=CARTESIAN_POINT('Ctrl Pts',(-39.5197593574043,-30.13000002,-95.4732641712576));
#138250=CARTESIAN_POINT('Ctrl Pts',(-39.506610251674,-30.13000002,-95.6532194499864));
#138251=CARTESIAN_POINT('Ctrl Pts',(-39.5000000000002,-30.13000002,-95.8342931017841));
#138252=CARTESIAN_POINT('Ctrl Pts',(-39.5,-30.13000002,-96.0164973302556));
#138253=CARTESIAN_POINT('Ctrl Pts',(-56.0289353856639,-30.13000002,-61.0621827299711));
#138254=CARTESIAN_POINT('Ctrl Pts',(-53.4376473376604,-30.13000002,-66.3621123698348));
#138255=CARTESIAN_POINT('Ctrl Pts',(-50.8336218773754,-30.13000002,-71.6557063652599));
#138256=CARTESIAN_POINT('Ctrl Pts',(-48.2096546190285,-30.13000002,-76.9393812233288));
#138257=CARTESIAN_POINT('Ctrl Pts',(-45.5856873606815,-30.13000002,-82.2230560813977));
#138258=CARTESIAN_POINT('Ctrl Pts',(-42.9421476228591,-30.13000002,-87.4969955027855));
#138259=CARTESIAN_POINT('Ctrl Pts',(-40.2651432342477,-30.13000002,-92.754289460876));
#138260=CARTESIAN_POINT('Origin',(-60.,-29.63000002,-55.74995));
#138261=CARTESIAN_POINT('',(-57.,-29.63000002,-55.24995));
#138262=CARTESIAN_POINT('',(-60.,-29.63000002,-55.24995));
#138263=CARTESIAN_POINT('Origin',(-57.,-29.63000002,-55.74995));
#138264=CARTESIAN_POINT('Origin',(-60.,28.41999998,-55.24995));
#138265=CARTESIAN_POINT('',(-57.,-29.13000002,-55.24995));
#138266=CARTESIAN_POINT('',(-60.,-29.13000002,-55.24995));
#138267=CARTESIAN_POINT('',(-57.,28.41999998,-55.24995));
#138268=CARTESIAN_POINT('Origin',(83.2809572255632,-29.13000002,-55.74995));
#138269=CARTESIAN_POINT('',(-57.,-28.63000002,-55.74995));
#138270=CARTESIAN_POINT('',(83.2809572255632,-28.6300000199999,-55.74995));
#138271=CARTESIAN_POINT('Origin',(-57.,-29.13000002,-55.74995));
#138272=CARTESIAN_POINT('Ctrl Pts',(-56.2981381510249,-28.0154717851087,
-60.8899762078857));
#138273=CARTESIAN_POINT('Ctrl Pts',(-56.1708458184293,-28.6301256542592,
-60.8213741500007));
#138274=CARTESIAN_POINT('Ctrl Pts',(-56.7267007677588,-28.6300000101017,
-61.1208879979441));
#138275=CARTESIAN_POINT('Ctrl Pts',(-56.3842107337159,-28.0053123694987,
-60.7350480688662));
#138276=CARTESIAN_POINT('Ctrl Pts',(-56.231166166104,-28.630129440528,-60.6796100628425));
#138277=CARTESIAN_POINT('Ctrl Pts',(-56.8517546922174,-28.6300000099381,
-60.8884604222472));
#138278=CARTESIAN_POINT('Ctrl Pts',(-56.4261416440025,-28.000404297649,
-60.56196856935));
#138279=CARTESIAN_POINT('Ctrl Pts',(-56.2556311178187,-28.6301313253205,
-60.5386217481864));
#138280=CARTESIAN_POINT('Ctrl Pts',(-56.9126898510831,-28.630000009859,
-60.6288526395369));
#138281=CARTESIAN_POINT('Ctrl Pts',(-56.4178064988838,-28.0013806349218,
-60.3838347631883));
#138282=CARTESIAN_POINT('Ctrl Pts',(-56.25064863923,-28.6301309522558,-60.3916281028846));
#138283=CARTESIAN_POINT('Ctrl Pts',(-56.900577244494,-28.6300000098747,
-60.3616165536491));
#138284=CARTESIAN_POINT('',(-56.7565335485771,-28.63000002,-61.0621827299711));
#138285=CARTESIAN_POINT('Origin',(-56.7565335485771,-28.13000002,-61.0621827299711));
#138286=CARTESIAN_POINT('Origin',(-55.4600042524658,-28.6300004012304,-60.4518437845537));
#138287=CARTESIAN_POINT('Origin',(83.2809572255632,-28.6300000199999,-55.24995));
#138288=CARTESIAN_POINT('',(-40.1842134716234,-28.63000002,-94.9396273673639));
#138289=CARTESIAN_POINT('Ctrl Pts',(-40.1842134716234,-28.63000002,-94.9396273673639));
#138290=CARTESIAN_POINT('Ctrl Pts',(-42.9880935290232,-28.63000002,-89.3138475723767));
#138291=CARTESIAN_POINT('Ctrl Pts',(-45.7634210292107,-28.63000002,-83.6741003095903));
#138292=CARTESIAN_POINT('Ctrl Pts',(-48.5225556597151,-28.63000002,-78.026431746297));
#138293=CARTESIAN_POINT('Ctrl Pts',(-51.2816902902195,-28.63000002,-72.3787631830038));
#138294=CARTESIAN_POINT('Ctrl Pts',(-54.0242783838037,-28.63000002,-66.7230003106817));
#138295=CARTESIAN_POINT('Ctrl Pts',(-56.7565335485771,-28.63000002,-61.0621827299711));
#138296=CARTESIAN_POINT('',(-39.5,-28.63000002,-97.8896208912436));
#138297=CARTESIAN_POINT('Ctrl Pts',(-39.5,-28.63000002,-97.8896208912436));
#138298=CARTESIAN_POINT('Ctrl Pts',(-39.5,-28.63000002,-97.7089321417027));
#138299=CARTESIAN_POINT('Ctrl Pts',(-39.50738071193,-28.63000002,-97.5282244682258));
#138300=CARTESIAN_POINT('Ctrl Pts',(-39.5219120167721,-28.63000002,-97.3483295034428));
#138301=CARTESIAN_POINT('Ctrl Pts',(-39.5366966813148,-28.63000002,-97.1652979907105));
#138302=CARTESIAN_POINT('Ctrl Pts',(-39.5588835421167,-28.63000002,-96.9831066045018));
#138303=CARTESIAN_POINT('Ctrl Pts',(-39.5882836977188,-28.63000002,-96.802626732815));
#138304=CARTESIAN_POINT('Ctrl Pts',(-39.6119618388165,-28.63000002,-96.6572728127559));
#138305=CARTESIAN_POINT('Ctrl Pts',(-39.6403197974461,-28.63000002,-96.5130286888782));
#138306=CARTESIAN_POINT('Ctrl Pts',(-39.6732827765156,-28.63000002,-96.3703554408507));
#138307=CARTESIAN_POINT('Ctrl Pts',(-39.7499154654027,-28.63000002,-96.0386671366605));
#138308=CARTESIAN_POINT('Ctrl Pts',(-39.8508333618867,-28.63000002,-95.7143394136885));
#138309=CARTESIAN_POINT('Ctrl Pts',(-39.9781561959401,-28.63000002,-95.3980147135165));
#138310=CARTESIAN_POINT('Ctrl Pts',(-40.0404386993086,-28.63000002,-95.243278178232));
#138311=CARTESIAN_POINT('Ctrl Pts',(-40.1090402739363,-28.63000002,-95.0904568779003));
#138312=CARTESIAN_POINT('Ctrl Pts',(-40.1842134716234,-28.63000002,-94.9396273673639));
#138313=CARTESIAN_POINT('',(-39.5,-28.63000002,-134.169022080262));
#138314=CARTESIAN_POINT('',(-39.5,-28.63000002,-55.24995));
#138315=CARTESIAN_POINT('',(-40.1842134716234,-28.63000002,-137.119015604142));
#138316=CARTESIAN_POINT('Ctrl Pts',(-40.1842134716234,-28.63000002,-137.119015604142));
#138317=CARTESIAN_POINT('Ctrl Pts',(-40.063259300405,-28.63000002,-136.876329926221));
#138318=CARTESIAN_POINT('Ctrl Pts',(-39.9584937855378,-28.63000002,-136.625775901222));
#138319=CARTESIAN_POINT('Ctrl Pts',(-39.8698562579308,-28.63000002,-136.370603923321));
#138320=CARTESIAN_POINT('Ctrl Pts',(-39.7907547390424,-28.63000002,-136.142884450829));
#138321=CARTESIAN_POINT('Ctrl Pts',(-39.7244982953546,-28.63000002,-135.911485835381));
#138322=CARTESIAN_POINT('Ctrl Pts',(-39.6710763875084,-28.63000002,-135.678705638911));
#138323=CARTESIAN_POINT('Ctrl Pts',(-39.5896852679394,-28.63000002,-135.324052621675));
#138324=CARTESIAN_POINT('Ctrl Pts',(-39.5369428910349,-28.63000002,-134.964508495217));
#138325=CARTESIAN_POINT('Ctrl Pts',(-39.5136924175149,-28.63000002,-134.599929291455));
#138326=CARTESIAN_POINT('Ctrl Pts',(-39.5045817727589,-28.63000002,-134.457069766118));
#138327=CARTESIAN_POINT('Ctrl Pts',(-39.5,-28.63000002,-134.313437038192));
#138328=CARTESIAN_POINT('Ctrl Pts',(-39.5,-28.63000002,-134.169022080262));
#138329=CARTESIAN_POINT('',(-56.8729709358987,-28.63000002,-171.237717270032));
#138330=CARTESIAN_POINT('Ctrl Pts',(-56.8729709358987,-28.63000002,-171.237717270032));
#138331=CARTESIAN_POINT('Ctrl Pts',(-54.1216123272523,-28.63000002,-165.536543461238));
#138332=CARTESIAN_POINT('Ctrl Pts',(-51.3598402340142,-28.63000002,-159.840463284682));
#138333=CARTESIAN_POINT('Ctrl Pts',(-48.5813487526192,-28.63000002,-154.152561198155));
#138334=CARTESIAN_POINT('Ctrl Pts',(-45.8028572712242,-28.63000002,-148.464659111628));
#138335=CARTESIAN_POINT('Ctrl Pts',(-43.0080103715946,-28.63000002,-142.784757083568));
#138336=CARTESIAN_POINT('Ctrl Pts',(-40.1842134716234,-28.63000002,-137.119015604142));
#138337=CARTESIAN_POINT('',(-57.0184057454332,-28.63000002,-171.871644662643));
#138338=CARTESIAN_POINT('Origin',(-55.5771425539593,-28.6300004042112,-171.848433760986));
#138339=CARTESIAN_POINT('',(-57.0184057454332,-28.63000002,-176.849882244789));
#138340=CARTESIAN_POINT('',(-57.0184057454332,-28.63000002,-171.871644662643));
#138341=CARTESIAN_POINT('',(-59.5,-28.63000002,-174.34995));
#138342=CARTESIAN_POINT('Origin',(-57.,-28.63000002,-174.34995));
#138343=CARTESIAN_POINT('',(-59.5,-28.63000002,-58.24995));
#138344=CARTESIAN_POINT('',(-59.5,-28.63000002,-174.34995));
#138345=CARTESIAN_POINT('Origin',(-57.,-28.63000002,-58.24995));
#138346=CARTESIAN_POINT('Origin',(0.,-12.9675000200281,-60.64995));
#138347=CARTESIAN_POINT('',(-39.7602371875712,-27.9700232835192,-94.7283182633411));
#138348=CARTESIAN_POINT('',(-39.5912209089345,-22.3752378108151,-98.5946087902607));
#138349=CARTESIAN_POINT('Ctrl Pts',(-39.760237187334,-27.9700232996177,
-94.7283182916262));
#138350=CARTESIAN_POINT('Ctrl Pts',(-39.7429528415391,-27.4727630876175,
-95.1394632520645));
#138351=CARTESIAN_POINT('Ctrl Pts',(-39.725890220247,-26.9675166669193,
-95.540293140202));
#138352=CARTESIAN_POINT('Ctrl Pts',(-39.7091463075091,-26.4529290005184,
-95.9291550328498));
#138353=CARTESIAN_POINT('Ctrl Pts',(-39.6919956601185,-25.9258412309992,
-96.3274629617598));
#138354=CARTESIAN_POINT('Ctrl Pts',(-39.6751334260609,-25.3873798477127,
-96.7142461865699));
#138355=CARTESIAN_POINT('Ctrl Pts',(-39.6588811036972,-24.8421814727703,
-97.0830011825413));
#138356=CARTESIAN_POINT('Ctrl Pts',(-39.6348426135811,-24.0357892874514,
-97.6284194389328));
#138357=CARTESIAN_POINT('Ctrl Pts',(-39.6121111132943,-23.2146690372305,
-98.1350071075587));
#138358=CARTESIAN_POINT('Ctrl Pts',(-39.5912173600306,-22.3752713037076,
-98.5946697908795));
#138359=CARTESIAN_POINT('Ctrl Pts',(-56.3187331343194,-28.0130417005584,
-60.8508735991007));
#138360=CARTESIAN_POINT('Ctrl Pts',(-53.5878832423519,-28.007786404225,
-66.5116884426402));
#138361=CARTESIAN_POINT('Ctrl Pts',(-50.8469740031282,-28.0018438144749,
-72.167454052164));
#138362=CARTESIAN_POINT('Ctrl Pts',(-45.3330806261693,-27.9878402480257,
-83.4627911786916));
#138363=CARTESIAN_POINT('Ctrl Pts',(-42.560432140096,-27.9797945689747,
-89.1025347299149));
#138364=CARTESIAN_POINT('Ctrl Pts',(-39.7602371906927,-27.9700232578782,
-94.7283182364936));
#138365=CARTESIAN_POINT('Ctrl Pts',(-39.5912209089345,-22.3752378108151,
-98.5946087902606));
#138366=CARTESIAN_POINT('Ctrl Pts',(-45.6084483277559,-22.3901517769159,
-86.0327992158248));
#138367=CARTESIAN_POINT('Ctrl Pts',(-51.5741970786256,-22.399288356509,
-73.4455439777502));
#138368=CARTESIAN_POINT('Ctrl Pts',(-57.5245249214072,-22.4066238608121,
-60.8508735991007));
#138369=CARTESIAN_POINT('Ctrl Pts',(-57.6206785412152,-22.3992316056509,
-60.42825533736));
#138370=CARTESIAN_POINT('Ctrl Pts',(-57.6893011240826,-21.98000002,-60.42825533736));
#138371=CARTESIAN_POINT('Ctrl Pts',(-58.1141118834647,-21.98000002,-60.42825533736));
#138372=CARTESIAN_POINT('Ctrl Pts',(-57.6206785407758,-22.3992316083349,
-60.574219492927));
#138373=CARTESIAN_POINT('Ctrl Pts',(-57.6893011111963,-21.9800000199989,
-60.5843987403017));
#138374=CARTESIAN_POINT('Ctrl Pts',(-58.1141118664761,-21.98000002,-60.6472062522327));
#138375=CARTESIAN_POINT('Ctrl Pts',(-57.5883338458808,-22.4017068994087,
-60.7175481239357));
#138376=CARTESIAN_POINT('Ctrl Pts',(-57.6525421683829,-21.98000002,-60.7382102053579));
#138377=CARTESIAN_POINT('Ctrl Pts',(-58.0662048046675,-21.98000002,-60.8621882839625));
#138378=CARTESIAN_POINT('Ctrl Pts',(-57.5245249214072,-22.4066238608121,
-60.8508735991007));
#138379=CARTESIAN_POINT('Ctrl Pts',(-57.5817506954797,-21.98000002,-60.8779152752782));
#138380=CARTESIAN_POINT('Ctrl Pts',(-57.9716987024741,-21.98000002,-61.0621827299711));
#138381=CARTESIAN_POINT('',(-57.9716987024741,-21.98000002,-61.0621827299711));
#138382=CARTESIAN_POINT('Origin',(-57.9716987024741,-22.48000002,-61.0621827299711));
#138383=CARTESIAN_POINT('Origin',(-55.9860799622262,-21.98000002,-60.2945890942193));
#138384=CARTESIAN_POINT('Origin',(83.2809572255632,-21.9800000199999,-55.24995));
#138385=CARTESIAN_POINT('',(-59.5,-21.98000002,-58.1532962439713));
#138386=CARTESIAN_POINT('Ctrl Pts',(-59.5,-21.98000002,-58.1532962439713));
#138387=CARTESIAN_POINT('Ctrl Pts',(-59.5,-21.98000002,-57.9611810443356));
#138388=CARTESIAN_POINT('Ctrl Pts',(-59.4783898617064,-21.9800000201789,
-57.7727385086896));
#138389=CARTESIAN_POINT('Ctrl Pts',(-59.435440674215,-21.9800000198205,
-57.587937528972));
#138390=CARTESIAN_POINT('Ctrl Pts',(-59.4262406555698,-21.9800000197437,
-57.5483518567313));
#138391=CARTESIAN_POINT('Ctrl Pts',(-59.4160613127736,-21.9800000196281,
-57.5089332628346));
#138392=CARTESIAN_POINT('Ctrl Pts',(-59.4049049949538,-21.9800000194259,
-57.469681421663));
#138393=CARTESIAN_POINT('Ctrl Pts',(-59.3987196130206,-21.9800000193138,
-57.4479190773891));
#138394=CARTESIAN_POINT('Ctrl Pts',(-59.3922287663824,-21.9800000192153,
-57.4261931844644));
#138395=CARTESIAN_POINT('Ctrl Pts',(-59.3854342581924,-21.9800000191476,
-57.4045116647966));
#138396=CARTESIAN_POINT('Ctrl Pts',(-59.366537060127,-21.9800000189591,
-57.3442100270524));
#138397=CARTESIAN_POINT('Ctrl Pts',(-59.3452714576318,-21.9800000190536,
-57.2844762659556));
#138398=CARTESIAN_POINT('Ctrl Pts',(-59.3218795388589,-21.9800000193212,
-57.2258422130826));
#138399=CARTESIAN_POINT('Ctrl Pts',(-59.3106878533869,-21.9800000194493,
-57.1977891968217));
#138400=CARTESIAN_POINT('Ctrl Pts',(-59.2990101624398,-21.9800000196077,
-57.1699876439618));
#138401=CARTESIAN_POINT('Ctrl Pts',(-59.2868766202345,-21.9800000197421,
-57.1424936459686));
#138402=CARTESIAN_POINT('Ctrl Pts',(-59.2731919149499,-21.9800000198936,
-57.1114847902475));
#138403=CARTESIAN_POINT('Ctrl Pts',(-59.2588942022727,-21.9800000199412,
-57.0807856309711));
#138404=CARTESIAN_POINT('Ctrl Pts',(-59.2440132425671,-21.9800000199676,
-57.0504664636976));
#138405=CARTESIAN_POINT('Ctrl Pts',(-59.2100364625762,-21.9800000200278,
-56.981240573947));
#138406=CARTESIAN_POINT('Ctrl Pts',(-59.1729132668602,-21.9800000200007,
-56.9136446874655));
#138407=CARTESIAN_POINT('Ctrl Pts',(-59.1326772603361,-21.9800000199982,
-56.8478208127099));
#138408=CARTESIAN_POINT('Ctrl Pts',(-59.1305108981493,-21.9800000199981,
-56.8442767643418));
#138409=CARTESIAN_POINT('Ctrl Pts',(-59.1283355234414,-21.9800000199979,
-56.8407378470944));
#138410=CARTESIAN_POINT('Ctrl Pts',(-59.1261511452891,-21.9800000199978,
-56.8372040811614));
#138411=CARTESIAN_POINT('Ctrl Pts',(-59.1024586951323,-21.980000019996,
-56.7988757481558));
#138412=CARTESIAN_POINT('Ctrl Pts',(-59.0776978833329,-21.9800000199944,
-56.7611395583364));
#138413=CARTESIAN_POINT('Ctrl Pts',(-59.051864196737,-21.9800000199939,
-56.7239980129523));
#138414=CARTESIAN_POINT('Ctrl Pts',(-58.9794118018617,-21.9800000199925,
-56.6198319311016));
#138415=CARTESIAN_POINT('Ctrl Pts',(-58.897983005211,-21.9800000199984,
-56.5200000236488));
#138416=CARTESIAN_POINT('Ctrl Pts',(-58.8106774361301,-21.9800000199995,
-56.4282264859168));
#138417=CARTESIAN_POINT('Ctrl Pts',(-58.7700668687888,-21.9800000200001,
-56.3855376234141));
#138418=CARTESIAN_POINT('Ctrl Pts',(-58.7280754192644,-21.98000002,-56.3444004714051));
#138419=CARTESIAN_POINT('Ctrl Pts',(-58.6847050658881,-21.98000002,-56.3048126520436));
#138420=CARTESIAN_POINT('Ctrl Pts',(-58.6494885520011,-21.98000002,-56.2726675371952));
#138421=CARTESIAN_POINT('Ctrl Pts',(-58.6132573779918,-21.98000002,-56.2414509676698));
#138422=CARTESIAN_POINT('Ctrl Pts',(-58.5760924792892,-21.98000002,-56.2112492084164));
#138423=CARTESIAN_POINT('Ctrl Pts',(-58.5607621926284,-21.98000002,-56.1987911729265));
#138424=CARTESIAN_POINT('Ctrl Pts',(-58.5452724940588,-21.98000002,-56.1865050278631));
#138425=CARTESIAN_POINT('Ctrl Pts',(-58.5296351858009,-21.98000002,-56.174399760192));
#138426=CARTESIAN_POINT('Ctrl Pts',(-58.50318856599,-21.98000002,-56.1539267090422));
#138427=CARTESIAN_POINT('Ctrl Pts',(-58.4762743935287,-21.98000002,-56.1339724230775));
#138428=CARTESIAN_POINT('Ctrl Pts',(-58.4489601509993,-21.98000002,-56.1145700874369));
#138429=CARTESIAN_POINT('Ctrl Pts',(-58.3958489442448,-21.98000002,-56.0768431961047));
#138430=CARTESIAN_POINT('Ctrl Pts',(-58.3412467373532,-21.9800000154289,
-56.0410944834472));
#138431=CARTESIAN_POINT('Ctrl Pts',(-58.2853645640813,-21.9799999916842,
-56.0075334770553));
#138432=CARTESIAN_POINT('Ctrl Pts',(-58.2574234774454,-21.9799999798118,
-55.9907529738594));
#138433=CARTESIAN_POINT('Ctrl Pts',(-58.2291619777336,-21.9799999666902,
-55.9745206253323));
#138434=CARTESIAN_POINT('Ctrl Pts',(-58.2006099144576,-21.9799999607144,
-55.9588587007899));
#138435=CARTESIAN_POINT('Ctrl Pts',(-58.1720578511817,-21.9799999547386,
-55.9431967762476));
#138436=CARTESIAN_POINT('Ctrl Pts',(-58.1432152243425,-21.9799999567774,
-55.9281052756887));
#138437=CARTESIAN_POINT('Ctrl Pts',(-58.1141118834472,-21.9799999679397,
-55.9136064684357));
#138438=CARTESIAN_POINT('',(-59.5,-21.98000002,-174.47822483969));
#138439=CARTESIAN_POINT('',(-59.5,-21.98000002,-58.1720074546108));
#138440=CARTESIAN_POINT('',(-58.2281061322626,-21.9800000072249,-176.657965001847));
#138441=CARTESIAN_POINT('Ctrl Pts',(-58.2281061322555,-21.9799999688995,
-176.657965001835));
#138442=CARTESIAN_POINT('Ctrl Pts',(-58.276338147052,-21.9799999587489,
-176.630735497029));
#138443=CARTESIAN_POINT('Ctrl Pts',(-58.3235842378115,-21.9799999676447,
-176.601941540627));
#138444=CARTESIAN_POINT('Ctrl Pts',(-58.3697659029187,-21.9799999836463,
-176.571657891927));
#138445=CARTESIAN_POINT('Ctrl Pts',(-58.4333419149396,-21.9800000056749,
-176.529967892024));
#138446=CARTESIAN_POINT('Ctrl Pts',(-58.4951281469291,-21.9800000132519,
-176.485368653424));
#138447=CARTESIAN_POINT('Ctrl Pts',(-58.554457957275,-21.9800000168151,
-176.438221543424));
#138448=CARTESIAN_POINT('Ctrl Pts',(-58.5638633718778,-21.98000001738,-176.430747423512));
#138449=CARTESIAN_POINT('Ctrl Pts',(-58.5732071081931,-21.9800000178323,
-176.423209364713));
#138450=CARTESIAN_POINT('Ctrl Pts',(-58.582486579001,-21.9800000181999,
-176.415608906189));
#138451=CARTESIAN_POINT('Ctrl Pts',(-58.6422321318881,-21.9800000205672,
-176.366673616007));
#138452=CARTESIAN_POINT('Ctrl Pts',(-58.6996264562076,-21.9800000199999,
-176.315076489292));
#138453=CARTESIAN_POINT('Ctrl Pts',(-58.754548274659,-21.9800000199988,
-176.260908374673));
#138454=CARTESIAN_POINT('Ctrl Pts',(-58.7869024533102,-21.9800000199981,
-176.228998199318));
#138455=CARTESIAN_POINT('Ctrl Pts',(-58.8184303801206,-21.9800000199976,
-176.196159475715));
#138456=CARTESIAN_POINT('Ctrl Pts',(-58.8491278703888,-21.9800000199976,
-176.162387482235));
#138457=CARTESIAN_POINT('Ctrl Pts',(-58.9319941632242,-21.9800000199974,
-176.071221726439));
#138458=CARTESIAN_POINT('Ctrl Pts',(-59.0089727564858,-21.9800000199996,
-175.972743969313));
#138459=CARTESIAN_POINT('Ctrl Pts',(-59.0773246245197,-21.9800000199999,
-175.870559516175));
#138460=CARTESIAN_POINT('Ctrl Pts',(-59.1060118933486,-21.98000002,-175.82767271642));
#138461=CARTESIAN_POINT('Ctrl Pts',(-59.1333062996812,-21.98000002,-175.784013939838));
#138462=CARTESIAN_POINT('Ctrl Pts',(-59.1592107352546,-21.98000002,-175.739584721266));
#138463=CARTESIAN_POINT('Ctrl Pts',(-59.1950270177852,-21.98000002,-175.678155494582));
#138464=CARTESIAN_POINT('Ctrl Pts',(-59.2281939400895,-21.9800000200315,
-175.615256612429));
#138465=CARTESIAN_POINT('Ctrl Pts',(-59.2587125449347,-21.9800000196412,
-175.550888840134));
#138466=CARTESIAN_POINT('Ctrl Pts',(-59.311304650302,-21.9800000189686,
-175.439965137037));
#138467=CARTESIAN_POINT('Ctrl Pts',(-59.356300154325,-21.98000001654,-175.323678961831));
#138468=CARTESIAN_POINT('Ctrl Pts',(-59.3921466355886,-21.9800000173947,
-175.205510135853));
#138469=CARTESIAN_POINT('Ctrl Pts',(-59.3996691193178,-21.9800000175741,
-175.180712079269));
#138470=CARTESIAN_POINT('Ctrl Pts',(-59.4067991608449,-21.9800000178929,
-175.15584684927));
#138471=CARTESIAN_POINT('Ctrl Pts',(-59.4135356395821,-21.9800000182925,
-175.130914599889));
#138472=CARTESIAN_POINT('Ctrl Pts',(-59.4621021364636,-21.9800000211732,
-174.95116609046));
#138473=CARTESIAN_POINT('Ctrl Pts',(-59.4903344201326,-21.9800000199997,
-174.767951128816));
#138474=CARTESIAN_POINT('Ctrl Pts',(-59.4979153635687,-21.98000002,-174.581221680408));
#138475=CARTESIAN_POINT('Ctrl Pts',(-59.4993044120658,-21.98000002,-174.547007434931));
#138476=CARTESIAN_POINT('Ctrl Pts',(-59.5,-21.98000002,-174.51267523574));
#138477=CARTESIAN_POINT('Ctrl Pts',(-59.5,-21.98000002,-174.47822483969));
#138478=CARTESIAN_POINT('',(-58.2281061322669,-21.98000002,-171.871644662643));
#138479=CARTESIAN_POINT('',(-58.2281061322669,-21.98000002,-176.848603273909));
#138480=CARTESIAN_POINT('',(-58.085700246061,-21.98000002,-171.237717270032));
#138481=CARTESIAN_POINT('Origin',(-56.8433387827296,-21.9799994107774,-171.841912580654));
#138482=CARTESIAN_POINT('',(-40.032098818041,-21.98000002,-133.252725050377));
#138483=CARTESIAN_POINT('Ctrl Pts',(-40.0320988180411,-21.98000002,-133.252725050377));
#138484=CARTESIAN_POINT('Ctrl Pts',(-46.0913111616059,-21.98000002,-145.894738473846));
#138485=CARTESIAN_POINT('Ctrl Pts',(-52.0964027110273,-21.98000002,-158.56247456275));
#138486=CARTESIAN_POINT('Ctrl Pts',(-58.085700246061,-21.98000002,-171.237717270032));
#138487=CARTESIAN_POINT('',(-39.5,-21.98000002,-130.903539806302));
#138488=CARTESIAN_POINT('Ctrl Pts',(-39.5,-21.98000002,-130.903539806302));
#138489=CARTESIAN_POINT('Ctrl Pts',(-39.5,-21.98000002,-131.168997483201));
#138490=CARTESIAN_POINT('Ctrl Pts',(-39.5196729008534,-21.98000002,-131.434381070373));
#138491=CARTESIAN_POINT('Ctrl Pts',(-39.5579798343684,-21.98000002,-131.695636340074));
#138492=CARTESIAN_POINT('Ctrl Pts',(-39.5785131750233,-21.98000002,-131.83567478634));
#138493=CARTESIAN_POINT('Ctrl Pts',(-39.6044013642058,-21.98000002,-131.974527214008));
#138494=CARTESIAN_POINT('Ctrl Pts',(-39.6354904757816,-21.98000002,-132.111568426422));
#138495=CARTESIAN_POINT('Ctrl Pts',(-39.7067779603525,-21.98000002,-132.425804595305));
#138496=CARTESIAN_POINT('Ctrl Pts',(-39.8050570910391,-21.98000002,-132.732328205563));
#138497=CARTESIAN_POINT('Ctrl Pts',(-39.9318010945657,-21.98000002,-133.030718310503));
#138498=CARTESIAN_POINT('Ctrl Pts',(-39.9634506501685,-21.98000002,-133.105230034567));
#138499=CARTESIAN_POINT('Ctrl Pts',(-39.9968754124349,-21.98000002,-133.179234513781));
#138500=CARTESIAN_POINT('Ctrl Pts',(-40.032098818041,-21.98000002,-133.252725050377));
#138501=CARTESIAN_POINT('',(-39.5,-21.98000002,-101.155103165204));
#138502=CARTESIAN_POINT('',(-39.5,-21.98000002,-55.24995));
#138503=CARTESIAN_POINT('',(-40.032098818038,-21.98000002,-98.8059179211358));
#138504=CARTESIAN_POINT('Ctrl Pts',(-40.032098818038,-21.98000002,-98.8059179211359));
#138505=CARTESIAN_POINT('Ctrl Pts',(-39.9030508971582,-21.98000002,-99.0751650535143));
#138506=CARTESIAN_POINT('Ctrl Pts',(-39.796952812407,-21.98000002,-99.355201219722));
#138507=CARTESIAN_POINT('Ctrl Pts',(-39.7146317074507,-21.98000002,-99.6400255235421));
#138508=CARTESIAN_POINT('Ctrl Pts',(-39.6845025786603,-21.98000002,-99.7442698499147));
#138509=CARTESIAN_POINT('Ctrl Pts',(-39.6575579700037,-21.98000002,-99.8491553321735));
#138510=CARTESIAN_POINT('Ctrl Pts',(-39.6338367806139,-21.98000002,-99.9543872911712));
#138511=CARTESIAN_POINT('Ctrl Pts',(-39.5613885485579,-21.98000002,-100.275782195106));
#138512=CARTESIAN_POINT('Ctrl Pts',(-39.5178914194315,-21.98000002,-100.602110104163));
#138513=CARTESIAN_POINT('Ctrl Pts',(-39.5044747449633,-21.98000002,-100.933563458968));
#138514=CARTESIAN_POINT('Ctrl Pts',(-39.5014958184563,-21.98000002,-101.007156597626));
#138515=CARTESIAN_POINT('Ctrl Pts',(-39.5,-21.98000002,-101.081002444678));
#138516=CARTESIAN_POINT('Ctrl Pts',(-39.5,-21.98000002,-101.155103165204));
#138517=CARTESIAN_POINT('Ctrl Pts',(-57.9716987024741,-21.98000002,-61.0621827299711));
#138518=CARTESIAN_POINT('Ctrl Pts',(-52.0201508381868,-21.98000002,-73.6568877040663));
#138519=CARTESIAN_POINT('Ctrl Pts',(-46.0528675815424,-21.98000002,-86.2441136451113));
#138520=CARTESIAN_POINT('Ctrl Pts',(-40.032098818038,-21.98000002,-98.8059179211357));
#138521=CARTESIAN_POINT('Ctrl Pts',(-59.5,-21.98000002,-58.1532962439713));
#138522=CARTESIAN_POINT('Ctrl Pts',(-60.,-21.98000002,-58.1532962439712));
#138523=CARTESIAN_POINT('Ctrl Pts',(-60.,-21.48000002,-58.1532962439713));
#138524=CARTESIAN_POINT('Ctrl Pts',(-59.4999999930587,-21.98000002,-57.8972567292831));
#138525=CARTESIAN_POINT('Ctrl Pts',(-59.9980388947882,-21.98000002,-57.846724408982));
#138526=CARTESIAN_POINT('Ctrl Pts',(-60.,-21.4819649551771,-57.8461243349599));
#138527=CARTESIAN_POINT('Ctrl Pts',(-59.4616086582853,-21.98000002,-57.6476410381502));
#138528=CARTESIAN_POINT('Ctrl Pts',(-59.9502437945621,-21.9800000199991,
-57.5478013960511));
#138529=CARTESIAN_POINT('Ctrl Pts',(-59.9539303867693,-21.4838860106857,
-57.5466594347187));
#138530=CARTESIAN_POINT('Ctrl Pts',(-59.34730526825,-21.98000002,-57.282960076491));
#138531=CARTESIAN_POINT('Ctrl Pts',(-59.8105866338858,-21.9800000200004,
-57.1115394631459));
#138532=CARTESIAN_POINT('Ctrl Pts',(-59.8167663234865,-21.4866995950233,
-57.1091506902012));
#138533=CARTESIAN_POINT('Ctrl Pts',(-59.29968672466,-21.98000002,-57.1639308209523));
#138534=CARTESIAN_POINT('Ctrl Pts',(-59.7527585815745,-21.9800000200004,
-56.9693956543515));
#138535=CARTESIAN_POINT('Ctrl Pts',(-59.7596240701279,-21.4876191423699,
-56.9663510387935));
#138536=CARTESIAN_POINT('Ctrl Pts',(-59.1883295347111,-21.98000002,-56.9370071244832));
#138537=CARTESIAN_POINT('Ctrl Pts',(-59.6179788443353,-21.9800000199995,
-56.6986593938776));
#138538=CARTESIAN_POINT('Ctrl Pts',(-59.6259954411174,-21.4893742131836,
-56.694110313108));
#138539=CARTESIAN_POINT('Ctrl Pts',(-59.1243146931145,-21.98000002,-56.8281652030541));
#138540=CARTESIAN_POINT('Ctrl Pts',(-59.5407153644089,-21.9800000200004,
-56.5688983662156));
#138541=CARTESIAN_POINT('Ctrl Pts',(-59.5491776307125,-21.4902170457339,
-56.5635325439996));
#138542=CARTESIAN_POINT('Ctrl Pts',(-58.9794096363452,-21.98000002,-56.6198336495764));
#138543=CARTESIAN_POINT('Ctrl Pts',(-59.3661855631985,-21.9800000199995,
-56.3207427939796));
#138544=CARTESIAN_POINT('Ctrl Pts',(-59.3752915646391,-21.4918319317587,
-56.3135970508604));
#138545=CARTESIAN_POINT('Ctrl Pts',(-58.897981763705,-21.98000002,-56.5200008958119));
#138546=CARTESIAN_POINT('Ctrl Pts',(-59.268291108539,-21.98000002,-56.2019010018047));
#138547=CARTESIAN_POINT('Ctrl Pts',(-59.2775781171727,-21.4926066631124,
-56.1938276864606));
#138548=CARTESIAN_POINT('Ctrl Pts',(-58.7233721306083,-21.98000002,-56.3364530063454));
#138549=CARTESIAN_POINT('Ctrl Pts',(-59.058685939558,-21.98000002,-55.9835815924875));
#138550=CARTESIAN_POINT('Ctrl Pts',(-59.0680465560033,-21.4940322909708,
-55.9736253396869));
#138551=CARTESIAN_POINT('Ctrl Pts',(-58.6296851267041,-21.98000002,-56.251851153689));
#138552=CARTESIAN_POINT('Ctrl Pts',(-58.9463663728276,-21.98000002,-55.8830032045419));
#138553=CARTESIAN_POINT('Ctrl Pts',(-58.9556221515304,-21.4946900550471,
-55.8721285607086));
#138554=CARTESIAN_POINT('Ctrl Pts',(-58.3295353039945,-21.98000002,-56.0194969731979));
#138555=CARTESIAN_POINT('Ctrl Pts',(-58.587136508474,-21.98000002,-55.607131606824));
#138556=CARTESIAN_POINT('Ctrl Pts',(-58.5954423658223,-21.4964978360334,
-55.5933734977247));
#138557=CARTESIAN_POINT('Ctrl Pts',(-58.1016300300823,-21.98000002,-55.8934667289665));
#138558=CARTESIAN_POINT('Ctrl Pts',(-58.3146314565664,-21.9800000200043,
-55.4574637281066));
#138559=CARTESIAN_POINT('Ctrl Pts',(-58.3219561351612,-21.4974802329133,
-55.4421752934307));
#138560=CARTESIAN_POINT('Ctrl Pts',(-57.866513770968,-21.98000002,-55.8065234638013));
#138561=CARTESIAN_POINT('Ctrl Pts',(-58.0337433152366,-21.98000002,-55.3542930871701));
#138562=CARTESIAN_POINT('Ctrl Pts',(-58.0398165251616,-21.4981583243581,
-55.3378696135325));
#138563=CARTESIAN_POINT('',(-60.,-21.48000002,-58.1532962439713));
#138564=CARTESIAN_POINT('Ctrl Pts',(-58.0831736437664,-21.4980516416407,
-55.3542805420642));
#138565=CARTESIAN_POINT('Ctrl Pts',(-58.3499299718387,-21.4973788455131,
-55.4577804898745));
#138566=CARTESIAN_POINT('Ctrl Pts',(-58.6077613800678,-21.4964360055793,
-55.6029075907754));
#138567=CARTESIAN_POINT('Ctrl Pts',(-58.9556221515304,-21.4946900550471,
-55.8721285607086));
#138568=CARTESIAN_POINT('Ctrl Pts',(-59.0680465560033,-21.4940322909708,
-55.9736253396869));
#138569=CARTESIAN_POINT('Ctrl Pts',(-59.2775781171727,-21.4926066631124,
-56.1938276864606));
#138570=CARTESIAN_POINT('Ctrl Pts',(-59.3752915646391,-21.4918319317587,
-56.3135970508604));
#138571=CARTESIAN_POINT('Ctrl Pts',(-59.5491776307125,-21.4902170457339,
-56.5635325439996));
#138572=CARTESIAN_POINT('Ctrl Pts',(-59.6259954411174,-21.4893742131836,
-56.694110313108));
#138573=CARTESIAN_POINT('Ctrl Pts',(-59.7596240701279,-21.4876191423699,
-56.9663510387935));
#138574=CARTESIAN_POINT('Ctrl Pts',(-59.8167663234865,-21.4866995950233,
-57.1091506902012));
#138575=CARTESIAN_POINT('Ctrl Pts',(-59.9539303867693,-21.4838860106857,
-57.5466594347187));
#138576=CARTESIAN_POINT('Ctrl Pts',(-60.,-21.4819649551771,-57.8461243349599));
#138577=CARTESIAN_POINT('Ctrl Pts',(-60.,-21.48000002,-58.1532962439713));
#138578=CARTESIAN_POINT('Origin',(-59.5,-21.48000002,-58.1532962439713));
#138579=CARTESIAN_POINT('Ctrl Pts',(-58.04813900635,-21.5914605167321,-55.3445609916381));
#138580=CARTESIAN_POINT('Ctrl Pts',(-59.9999999999999,-21.563522065113,
-56.0718305306275));
#138581=CARTESIAN_POINT('Ctrl Pts',(-60.,-21.4835561881163,-58.1534328789326));
#138582=CARTESIAN_POINT('Ctrl Pts',(-58.0747408021895,-21.3932704964989,
-55.3468739572293));
#138583=CARTESIAN_POINT('Ctrl Pts',(-60.,-21.3649831049967,-56.0851953591942));
#138584=CARTESIAN_POINT('Ctrl Pts',(-60.,-21.2836204844253,-58.1457522408661));
#138585=CARTESIAN_POINT('Ctrl Pts',(-58.1004355836544,-21.1945366814225,
-55.3490436413214));
#138586=CARTESIAN_POINT('Ctrl Pts',(-59.9999999999994,-21.1653697703472,
-56.0975649789358));
#138587=CARTESIAN_POINT('Ctrl Pts',(-60.,-21.0836896865644,-58.1378552621726));
#138588=CARTESIAN_POINT('Ctrl Pts',(-58.1252156299349,-20.9953105578148,
-55.3510803367174));
#138589=CARTESIAN_POINT('Ctrl Pts',(-60.,-20.9648839320844,-56.1090266406884));
#138590=CARTESIAN_POINT('Ctrl Pts',(-60.,-20.883761812232,-58.1298294552074));
#138591=CARTESIAN_POINT('',(-60.,-20.98000002,-58.1336824582564));
#138592=CARTESIAN_POINT('Ctrl Pts',(-60.,-20.98000002,-58.1336824582564));
#138593=CARTESIAN_POINT('Ctrl Pts',(-60.,-20.9819903749844,-57.8341710601268));
#138594=CARTESIAN_POINT('Ctrl Pts',(-59.9561544625383,-20.9839354847036,
-57.5420008057396));
#138595=CARTESIAN_POINT('Ctrl Pts',(-59.8258072839812,-20.986783840298,
-57.1148311652303));
#138596=CARTESIAN_POINT('Ctrl Pts',(-59.7713392035954,-20.9877182523804,
-56.9748142265907));
#138597=CARTESIAN_POINT('Ctrl Pts',(-59.6439928678614,-20.9895019296767,
-56.7077325083257));
#138598=CARTESIAN_POINT('Ctrl Pts',(-59.5707888728218,-20.9903591646404,
-56.5794722449985));
#138599=CARTESIAN_POINT('Ctrl Pts',(-59.4052064654638,-20.9920036864946,
-56.333575365965));
#138600=CARTESIAN_POINT('Ctrl Pts',(-59.3119800474081,-20.9927961294943,
-56.2151695770875));
#138601=CARTESIAN_POINT('Ctrl Pts',(-59.1114408594098,-20.9942622260151,
-55.9962288706011));
#138602=CARTESIAN_POINT('Ctrl Pts',(-59.0038498495005,-20.9949406197357,
-55.8949841496734));
#138603=CARTESIAN_POINT('Ctrl Pts',(-58.6648804276695,-20.9967833899732,
-55.6200886254342));
#138604=CARTESIAN_POINT('Ctrl Pts',(-58.4095966121519,-20.9978001101244,
-55.4685923770156));
#138605=CARTESIAN_POINT('Ctrl Pts',(-58.1440639002148,-20.9985364556097,
-55.3589167601806));
#138606=CARTESIAN_POINT('Ctrl Pts',(-60.,-20.98000002,-58.1336824582564));
#138607=CARTESIAN_POINT('Ctrl Pts',(-60.,-21.1466635001965,-58.1403364979909));
#138608=CARTESIAN_POINT('Ctrl Pts',(-60.,-21.3133297017902,-58.1468913732678));
#138609=CARTESIAN_POINT('Ctrl Pts',(-60.,-21.48000002,-58.1532962439713));
#138610=CARTESIAN_POINT('Ctrl Pts',(-60.,-20.98000002,-58.1336824582564));
#138611=CARTESIAN_POINT('Ctrl Pts',(-60.,-20.48000002,-58.1336824582564));
#138612=CARTESIAN_POINT('Ctrl Pts',(-59.5,-20.48000002,-58.1336824582564));
#138613=CARTESIAN_POINT('Ctrl Pts',(-60.,-20.9819903749844,-57.8341710601268));
#138614=CARTESIAN_POINT('Ctrl Pts',(-60.0019943000202,-20.4800000199965,
-57.8335762296713));
#138615=CARTESIAN_POINT('Ctrl Pts',(-59.4999999932334,-20.48000002,-57.8840234061944));
#138616=CARTESIAN_POINT('Ctrl Pts',(-59.9561544625383,-20.9839354847036,
-57.5420008057396));
#138617=CARTESIAN_POINT('Ctrl Pts',(-59.9599487537765,-20.48000002,-57.5408569976555));
#138618=CARTESIAN_POINT('Ctrl Pts',(-59.4634620545497,-20.48000002,-57.6404834185301));
#138619=CARTESIAN_POINT('Ctrl Pts',(-59.8258072839812,-20.986783840298,
-57.1148311652303));
#138620=CARTESIAN_POINT('Ctrl Pts',(-59.8322564407851,-20.48000002,-57.1124079291466));
#138621=CARTESIAN_POINT('Ctrl Pts',(-59.3548394021004,-20.48000002,-57.2844137892711));
#138622=CARTESIAN_POINT('Ctrl Pts',(-59.7713392035954,-20.9877182523804,
-56.9748142265907));
#138623=CARTESIAN_POINT('Ctrl Pts',(-59.7785418471728,-20.4800000199998,
-56.971709946724));
#138624=CARTESIAN_POINT('Ctrl Pts',(-59.3094493357903,-20.48000002,-57.1677018516063));
#138625=CARTESIAN_POINT('Ctrl Pts',(-59.6439928678614,-20.9895019296767,
-56.7077325083257));
#138626=CARTESIAN_POINT('Ctrl Pts',(-59.6524902953505,-20.4800000200002,
-56.7030545690594));
#138627=CARTESIAN_POINT('Ctrl Pts',(-59.2033273904236,-20.48000002,-56.945074258738));
#138628=CARTESIAN_POINT('Ctrl Pts',(-59.5707888728218,-20.9903591646404,
-56.5794722449985));
#138629=CARTESIAN_POINT('Ctrl Pts',(-59.5798070038494,-20.4800000200006,
-56.5739310816022));
#138630=CARTESIAN_POINT('Ctrl Pts',(-59.1423240613999,-20.48000002,-56.8381621017045));
#138631=CARTESIAN_POINT('Ctrl Pts',(-59.4052064654638,-20.9920036864946,
-56.333575365965));
#138632=CARTESIAN_POINT('Ctrl Pts',(-59.4150201769345,-20.4800000199993,
-56.3261371955428));
#138633=CARTESIAN_POINT('Ctrl Pts',(-59.0043387205048,-20.48000002,-56.6331931445326));
#138634=CARTESIAN_POINT('Ctrl Pts',(-59.3119800474081,-20.9927961294943,
-56.2151695770875));
#138635=CARTESIAN_POINT('Ctrl Pts',(-59.322050076116,-20.4800000199998,
-56.2067284595684));
#138636=CARTESIAN_POINT('Ctrl Pts',(-58.9266500387652,-20.48000002,-56.5344951934464));
#138637=CARTESIAN_POINT('Ctrl Pts',(-59.1114408594098,-20.9942622260151,
-55.9962288706011));
#138638=CARTESIAN_POINT('Ctrl Pts',(-59.1217230649246,-20.4800000200002,
-55.9857285998647));
#138639=CARTESIAN_POINT('Ctrl Pts',(-58.7595340502496,-20.48000002,-56.3519956346149));
#138640=CARTESIAN_POINT('Ctrl Pts',(-59.0038498495005,-20.9949406197357,
-55.8949841496734));
#138641=CARTESIAN_POINT('Ctrl Pts',(-59.0140876322601,-20.4800000199996,
-55.8834675579712));
#138642=CARTESIAN_POINT('Ctrl Pts',(-58.6698748748721,-20.48000002,-56.2676023678844));
#138643=CARTESIAN_POINT('Ctrl Pts',(-58.6593792112359,-20.9968132967355,
-55.6156272797255));
#138644=CARTESIAN_POINT('Ctrl Pts',(-58.6688057859238,-20.4800000200008,
-55.6008859078189));
#138645=CARTESIAN_POINT('Ctrl Pts',(-58.3828160087866,-20.48000002,-56.0347423933717));
#138646=CARTESIAN_POINT('Ctrl Pts',(-58.3970469849622,-20.9978498953169,
-55.4611742661273));
#138647=CARTESIAN_POINT('Ctrl Pts',(-58.4055356761976,-20.48000002,-55.4446537909846));
#138648=CARTESIAN_POINT('Ctrl Pts',(-58.1642057412792,-20.48000002,-55.9059968521648));
#138649=CARTESIAN_POINT('Ctrl Pts',(-58.124493706486,-20.9985901469525,
-55.3509197556537));
#138650=CARTESIAN_POINT('Ctrl Pts',(-58.1317309492636,-20.48000002,-55.333033840343));
#138651=CARTESIAN_POINT('Ctrl Pts',(-57.9370780887383,-20.48000002,-55.8140933660895));
#138652=CARTESIAN_POINT('',(-59.5,-20.48000002,-58.1336824582564));
#138653=CARTESIAN_POINT('Ctrl Pts',(-58.4684744114494,-20.4800000273303,
-56.1088024963514));
#138654=CARTESIAN_POINT('Ctrl Pts',(-58.5045026577924,-20.4800000196856,
-56.1349726812033));
#138655=CARTESIAN_POINT('Ctrl Pts',(-58.5397642385231,-20.48000002049,-56.1620276028478));
#138656=CARTESIAN_POINT('Ctrl Pts',(-58.5742078503022,-20.4800000209351,
-56.1899586284693));
#138657=CARTESIAN_POINT('Ctrl Pts',(-58.5777936723552,-20.4800000209814,
-56.1928664445334));
#138658=CARTESIAN_POINT('Ctrl Pts',(-58.5813717160946,-20.4800000210458,
-56.1957839761557));
#138659=CARTESIAN_POINT('Ctrl Pts',(-58.5849420358152,-20.480000021133,
-56.198711293078));
#138660=CARTESIAN_POINT('Ctrl Pts',(-58.6712575877011,-20.4800000232427,
-56.2694816989427));
#138661=CARTESIAN_POINT('Ctrl Pts',(-58.7525761505105,-20.4800000208245,
-56.3458655479582));
#138662=CARTESIAN_POINT('Ctrl Pts',(-58.8289004828144,-20.4800000205608,
-56.4278416205229));
#138663=CARTESIAN_POINT('Ctrl Pts',(-58.8336560351637,-20.4800000205444,
-56.4329493167544));
#138664=CARTESIAN_POINT('Ctrl Pts',(-58.8383922119778,-20.4800000205339,
-56.438078733635));
#138665=CARTESIAN_POINT('Ctrl Pts',(-58.8431090189103,-20.4800000205297,
-56.4432298704634));
#138666=CARTESIAN_POINT('Ctrl Pts',(-58.8623175352579,-20.480000020513,
-56.4642071327073));
#138667=CARTESIAN_POINT('Ctrl Pts',(-58.8812170617046,-20.4800000205714,
-56.4855758533909));
#138668=CARTESIAN_POINT('Ctrl Pts',(-58.8997746305286,-20.4800000209296,
-56.5072905946435));
#138669=CARTESIAN_POINT('Ctrl Pts',(-58.9619336923861,-20.4800000221292,
-56.580024688077));
#138670=CARTESIAN_POINT('Ctrl Pts',(-59.0202267572587,-20.4800000217717,
-56.6567158251598));
#138671=CARTESIAN_POINT('Ctrl Pts',(-59.0733581645971,-20.4800000210417,
-56.73565959907));
#138672=CARTESIAN_POINT('Ctrl Pts',(-59.1299234282924,-20.4800000202645,
-56.8197054697148));
#138673=CARTESIAN_POINT('Ctrl Pts',(-59.1811132500064,-20.480000019999,
-56.9067351897848));
#138674=CARTESIAN_POINT('Ctrl Pts',(-59.2269658512281,-20.4800000200342,
-56.9966989899188));
#138675=CARTESIAN_POINT('Ctrl Pts',(-59.2370332340863,-20.4800000200419,
-57.016451413886));
#138676=CARTESIAN_POINT('Ctrl Pts',(-59.2468434784441,-20.4800000200569,
-57.0363464697384));
#138677=CARTESIAN_POINT('Ctrl Pts',(-59.2563966865596,-20.480000020085,
-57.0563840875553));
#138678=CARTESIAN_POINT('Ctrl Pts',(-59.3094659573343,-20.4800000202415,
-57.167695570854));
#138679=CARTESIAN_POINT('Ctrl Pts',(-59.354874917347,-20.4800000213417,
-57.2844044844238));
#138680=CARTESIAN_POINT('Ctrl Pts',(-59.3910801060422,-20.4800000212014,
-57.4030935519939));
#138681=CARTESIAN_POINT('Ctrl Pts',(-59.4059237316432,-20.4800000211439,
-57.4517544247977));
#138682=CARTESIAN_POINT('Ctrl Pts',(-59.4192561241221,-20.4800000207682,
-57.5006743231195));
#138683=CARTESIAN_POINT('Ctrl Pts',(-59.4310694056707,-20.480000020378,
-57.5498521826326));
#138684=CARTESIAN_POINT('Ctrl Pts',(-59.453976422087,-20.4800000196214,
-57.6452124794769));
#138685=CARTESIAN_POINT('Ctrl Pts',(-59.4712138943901,-20.48000002,-57.7415452546604));
#138686=CARTESIAN_POINT('Ctrl Pts',(-59.4827195432934,-20.48000002,-57.8388478504797));
#138687=CARTESIAN_POINT('Ctrl Pts',(-59.4942251921967,-20.48000002,-57.936150446299));
#138688=CARTESIAN_POINT('Ctrl Pts',(-59.5,-20.48000002,-58.0344221425213));
#138689=CARTESIAN_POINT('Ctrl Pts',(-59.5,-20.48000002,-58.1336824582564));
#138690=CARTESIAN_POINT('Origin',(-59.5,-20.98000002,-58.1336824582564));
#138691=CARTESIAN_POINT('Ctrl Pts',(-57.8770125754992,-19.9259080025173,
-60.8508735991007));
#138692=CARTESIAN_POINT('Ctrl Pts',(-57.8224346115608,-20.48000002,-60.8252402001721));
#138693=CARTESIAN_POINT('Ctrl Pts',(-58.3269264615434,-20.48000002,-61.0621827299711));
#138694=CARTESIAN_POINT('Ctrl Pts',(-57.9394736727847,-19.9223173742648,
-60.7188022088811));
#138695=CARTESIAN_POINT('Ctrl Pts',(-57.8773360553627,-20.480000020003,
-60.6987815996246));
#138696=CARTESIAN_POINT('Ctrl Pts',(-58.4199720320461,-20.48000002,-60.8640724920291));
#138697=CARTESIAN_POINT('Ctrl Pts',(-57.9720322597472,-19.9204585218543,
-60.5756740647443));
#138698=CARTESIAN_POINT('Ctrl Pts',(-57.9049228489562,-20.4800000199977,
-60.5656525957412));
#138699=CARTESIAN_POINT('Ctrl Pts',(-58.4684744074159,-20.48000002,-60.6493857962184));
#138700=CARTESIAN_POINT('Ctrl Pts',(-57.9720322598041,-19.92045852138,-60.42825533736));
#138701=CARTESIAN_POINT('Ctrl Pts',(-57.9049228508695,-20.48000002,-60.42825533736));
#138702=CARTESIAN_POINT('Ctrl Pts',(-58.4684744114614,-20.48000002,-60.42825533736));
#138703=CARTESIAN_POINT('',(-58.3269264615434,-20.48000002,-61.0621827299711));
#138704=CARTESIAN_POINT('Origin',(-58.3269264615434,-19.98000002,-61.0621827299711));
#138705=CARTESIAN_POINT('Origin',(-56.2951177527026,-20.48000002,-60.2827926082911));
#138706=CARTESIAN_POINT('Origin',(83.2809572255632,-20.4800000199999,-55.24995));
#138707=CARTESIAN_POINT('',(-59.5,-20.48000002,-174.500886972636));
#138708=CARTESIAN_POINT('',(-58.5817791104913,-20.48000002,-176.438901946458));
#138709=CARTESIAN_POINT('Ctrl Pts',(-59.5,-20.48000002,-174.500886972636));
#138710=CARTESIAN_POINT('Ctrl Pts',(-59.5,-20.48000002,-174.594133457896));
#138711=CARTESIAN_POINT('Ctrl Pts',(-59.4948998873889,-20.48000002,-174.686506499847));
#138712=CARTESIAN_POINT('Ctrl Pts',(-59.484743418878,-20.48000002,-174.778024581704));
#138713=CARTESIAN_POINT('Ctrl Pts',(-59.4745869503671,-20.48000002,-174.869542663562));
#138714=CARTESIAN_POINT('Ctrl Pts',(-59.4593733052792,-20.4800000198432,
-174.96020535248));
#138715=CARTESIAN_POINT('Ctrl Pts',(-59.4391579117629,-20.4800000201565,
-175.050010672616));
#138716=CARTESIAN_POINT('Ctrl Pts',(-59.4270641008619,-20.4800000203439,
-175.103736490952));
#138717=CARTESIAN_POINT('Ctrl Pts',(-59.4131703468088,-20.4800000205099,
-175.157156500734));
#138718=CARTESIAN_POINT('Ctrl Pts',(-59.3974877716946,-20.4800000205022,
-175.210269911122));
#138719=CARTESIAN_POINT('Ctrl Pts',(-59.3634319732391,-20.4800000204854,
-175.325609361837));
#138720=CARTESIAN_POINT('Ctrl Pts',(-59.3206017517199,-20.4800000200584,
-175.43951508737));
#138721=CARTESIAN_POINT('Ctrl Pts',(-59.2705225473981,-20.480000020021,
-175.548294250575));
#138722=CARTESIAN_POINT('Ctrl Pts',(-59.2665668880551,-20.4800000200181,
-175.556886505965));
#138723=CARTESIAN_POINT('Ctrl Pts',(-59.2625645131408,-20.4800000200159,
-175.56545285612));
#138724=CARTESIAN_POINT('Ctrl Pts',(-59.2585154363462,-20.4800000200145,
-175.573993307709));
#138725=CARTESIAN_POINT('Ctrl Pts',(-59.223512146378,-20.4800000200017,
-175.647823446921));
#138726=CARTESIAN_POINT('Ctrl Pts',(-59.1850753506041,-20.4800000200467,
-175.719619366777));
#138727=CARTESIAN_POINT('Ctrl Pts',(-59.143147619382,-20.4800000203096,
-175.789501989862));
#138728=CARTESIAN_POINT('Ctrl Pts',(-59.1284714749915,-20.4800000204017,
-175.813963305486));
#138729=CARTESIAN_POINT('Ctrl Pts',(-59.1133672159704,-20.4800000205138,
-175.838189938605));
#138730=CARTESIAN_POINT('Ctrl Pts',(-59.0978311232235,-20.4800000206151,
-175.862186246726));
#138731=CARTESIAN_POINT('Ctrl Pts',(-59.057684395778,-20.4800000208766,
-175.924194967805));
#138732=CARTESIAN_POINT('Ctrl Pts',(-59.0143956166168,-20.4800000209379,
-175.984944386851));
#138733=CARTESIAN_POINT('Ctrl Pts',(-58.9683824813746,-20.4800000205207,
-176.043771514579));
#138734=CARTESIAN_POINT('Ctrl Pts',(-58.939956521226,-20.4800000202629,
-176.080113693386));
#138735=CARTESIAN_POINT('Ctrl Pts',(-58.9105390187326,-20.480000020158,
-176.115667750748));
#138736=CARTESIAN_POINT('Ctrl Pts',(-58.8802525752657,-20.4800000200989,
-176.150262230717));
#138737=CARTESIAN_POINT('Ctrl Pts',(-58.8008883718402,-20.4800000199439,
-176.240915441575));
#138738=CARTESIAN_POINT('Ctrl Pts',(-58.7158063838685,-20.4800000199516,
-176.324965650418));
#138739=CARTESIAN_POINT('Ctrl Pts',(-58.6252060810682,-20.4800000201162,
-176.402568149682));
#138740=CARTESIAN_POINT('Ctrl Pts',(-58.6108845926547,-20.4800000201422,
-176.414835032459));
#138741=CARTESIAN_POINT('Ctrl Pts',(-58.596406444494,-20.4800000201761,
-176.426947791328));
#138742=CARTESIAN_POINT('Ctrl Pts',(-58.5817791104913,-20.4800000202216,
-176.438901946458));
#138743=CARTESIAN_POINT('',(-59.5,-20.48000002,-174.524030413304));
#138744=CARTESIAN_POINT('',(-39.9829309662066,-20.48000002,-99.9929964369266));
#138745=CARTESIAN_POINT('Ctrl Pts',(-39.9829309662066,-20.48000002,-99.9929964369266));
#138746=CARTESIAN_POINT('Ctrl Pts',(-46.1212593572987,-20.48000002,-87.0272166609364));
#138747=CARTESIAN_POINT('Ctrl Pts',(-52.2285110086243,-20.48000002,-74.0467697366574));
#138748=CARTESIAN_POINT('Ctrl Pts',(-58.3269264615434,-20.48000002,-61.0621827299711));
#138749=CARTESIAN_POINT('',(-39.5,-20.48000002,-102.144196959718));
#138750=CARTESIAN_POINT('Ctrl Pts',(-39.5,-20.48000002,-102.144196959718));
#138751=CARTESIAN_POINT('Ctrl Pts',(-39.5,-20.48000002,-101.901224059727));
#138752=CARTESIAN_POINT('Ctrl Pts',(-39.5178405979396,-20.48000002,-101.658367298417));
#138753=CARTESIAN_POINT('Ctrl Pts',(-39.5526223904373,-20.48000002,-101.419269624472));
#138754=CARTESIAN_POINT('Ctrl Pts',(-39.5712680114436,-20.48000002,-101.291095534188));
#138755=CARTESIAN_POINT('Ctrl Pts',(-39.5947811831661,-20.48000002,-101.164001820978));
#138756=CARTESIAN_POINT('Ctrl Pts',(-39.6230172792885,-20.48000002,-101.038548856259));
#138757=CARTESIAN_POINT('Ctrl Pts',(-39.6919421332755,-20.48000002,-100.732315755265));
#138758=CARTESIAN_POINT('Ctrl Pts',(-39.7887207445114,-20.48000002,-100.433895586513));
#138759=CARTESIAN_POINT('Ctrl Pts',(-39.9146180003308,-20.48000002,-100.143643141333));
#138760=CARTESIAN_POINT('Ctrl Pts',(-39.9365064258825,-20.48000002,-100.093180015698));
#138761=CARTESIAN_POINT('Ctrl Pts',(-39.9592751462328,-20.48000002,-100.04296381121));
#138762=CARTESIAN_POINT('Ctrl Pts',(-39.9829309662065,-20.48000002,-99.9929964369266));
#138763=CARTESIAN_POINT('',(-39.5,-20.48000002,-129.914446011788));
#138764=CARTESIAN_POINT('',(-39.5,-20.48000002,-55.24995));
#138765=CARTESIAN_POINT('',(-39.9829309662066,-20.48000002,-132.065646534579));
#138766=CARTESIAN_POINT('Ctrl Pts',(-39.9829309662066,-20.48000002,-132.065646534579));
#138767=CARTESIAN_POINT('Ctrl Pts',(-39.8887941972359,-20.48000002,-131.866804677725));
#138768=CARTESIAN_POINT('Ctrl Pts',(-39.808012721684,-20.48000002,-131.661768384106));
#138769=CARTESIAN_POINT('Ctrl Pts',(-39.7410867352538,-20.48000002,-131.45329068418));
#138770=CARTESIAN_POINT('Ctrl Pts',(-39.6944643395886,-20.48000002,-131.308059656117));
#138771=CARTESIAN_POINT('Ctrl Pts',(-39.6545649019171,-20.48000002,-131.161159371035));
#138772=CARTESIAN_POINT('Ctrl Pts',(-39.6215434069806,-20.48000002,-131.013525238712));
#138773=CARTESIAN_POINT('Ctrl Pts',(-39.5522800663325,-20.48000002,-130.703859270587));
#138774=CARTESIAN_POINT('Ctrl Pts',(-39.5121705688285,-20.48000002,-130.389227115401));
#138775=CARTESIAN_POINT('Ctrl Pts',(-39.5023709529557,-20.48000002,-130.069431842175));
#138776=CARTESIAN_POINT('Ctrl Pts',(-39.5007919718943,-20.48000002,-130.017904242881));
#138777=CARTESIAN_POINT('Ctrl Pts',(-39.5,-20.48000002,-129.96624258113));
#138778=CARTESIAN_POINT('Ctrl Pts',(-39.5,-20.48000002,-129.914446011788));
#138779=CARTESIAN_POINT('',(-58.4402350532158,-20.48000002,-171.237717270032));
#138780=CARTESIAN_POINT('Ctrl Pts',(-58.4402350532158,-20.48000002,-171.237717270032));
#138781=CARTESIAN_POINT('Ctrl Pts',(-52.3041884424236,-20.48000002,-158.172646387016));
#138782=CARTESIAN_POINT('Ctrl Pts',(-46.1592765266851,-20.48000002,-145.111728668187));
#138783=CARTESIAN_POINT('Ctrl Pts',(-39.9829309662066,-20.48000002,-132.065646534579));
#138784=CARTESIAN_POINT('',(-58.5817791104913,-20.48000002,-171.871644662643));
#138785=CARTESIAN_POINT('Origin',(-56.4084014798071,-20.48000002,-172.018072886377));
#138786=CARTESIAN_POINT('',(-58.5817791104913,-20.48000002,-171.871644662643));
#138787=CARTESIAN_POINT('Origin',(0.,-12.9675000200281,-60.64995));
#138788=CARTESIAN_POINT('',(-39.5365899453791,-19.9017174926824,-99.7816873656535));
#138789=CARTESIAN_POINT('',(-39.4710976496823,-14.3145440753906,-101.167027481326));
#138790=CARTESIAN_POINT('Ctrl Pts',(-39.5365899624517,-19.9017174575869,
-99.7816873060563));
#138791=CARTESIAN_POINT('Ctrl Pts',(-39.5191359427996,-18.9900458934628,
-100.156305085366));
#138792=CARTESIAN_POINT('Ctrl Pts',(-39.5043113435924,-18.0551324974974,
-100.470115458113));
#138793=CARTESIAN_POINT('Ctrl Pts',(-39.4820945526735,-16.1678764290028,
-100.937768877564));
#138794=CARTESIAN_POINT('Ctrl Pts',(-39.474721832796,-15.2403172398251,
-101.091495325969));
#138795=CARTESIAN_POINT('Ctrl Pts',(-39.4710976496822,-14.3145440753934,
-101.167027481325));
#138796=CARTESIAN_POINT('Ctrl Pts',(-57.8770125754992,-19.9259080025173,
-60.8508735991007));
#138797=CARTESIAN_POINT('Ctrl Pts',(-51.7792721519529,-19.9203329617956,
-73.8354504791465));
#138798=CARTESIAN_POINT('Ctrl Pts',(-45.6728806072717,-19.9133770457548,
-86.8158923265289));
#138799=CARTESIAN_POINT('Ctrl Pts',(-39.5365899624517,-19.9017174575869,
-99.7816873060563));
#138800=CARTESIAN_POINT('Ctrl Pts',(-39.4710976496822,-14.3145440753934,
-101.167027481325));
#138801=CARTESIAN_POINT('Ctrl Pts',(-45.7410317152176,-14.3169685900793,
-87.7287563851229));
#138802=CARTESIAN_POINT('Ctrl Pts',(-52.0097486856907,-14.3183690440453,
-74.2898953083048));
#138803=CARTESIAN_POINT('Ctrl Pts',(-58.2781275348581,-14.3194901627709,
-60.8508735991007));
#138804=CARTESIAN_POINT('Ctrl Pts',(-58.3718694303385,-14.3184313509278,
-60.42825533736));
#138805=CARTESIAN_POINT('Ctrl Pts',(-58.383173457336,-13.83000002,-60.42825533736));
#138806=CARTESIAN_POINT('Ctrl Pts',(-58.871735578318,-13.83000002,-60.42825533736));
#138807=CARTESIAN_POINT('Ctrl Pts',(-58.3718694303297,-14.3184313513064,
-60.574130507918));
#138808=CARTESIAN_POINT('Ctrl Pts',(-58.3831734460811,-13.83000002,-60.57578605024));
#138809=CARTESIAN_POINT('Ctrl Pts',(-58.871735561804,-13.83000002,-60.6470682084222));
#138810=CARTESIAN_POINT('Ctrl Pts',(-58.3404329537672,-14.3187847426543,
-60.7173302229433));
#138811=CARTESIAN_POINT('Ctrl Pts',(-58.3509717578384,-13.8300000200006,
-60.7206801175402));
#138812=CARTESIAN_POINT('Ctrl Pts',(-58.8245931841484,-13.83000002,-60.8618675123431));
#138813=CARTESIAN_POINT('Ctrl Pts',(-58.2781275348581,-14.3194901627709,
-60.8508735991007));
#138814=CARTESIAN_POINT('Ctrl Pts',(-58.2874540965012,-13.83000002,-60.8552238163692));
#138815=CARTESIAN_POINT('Ctrl Pts',(-58.7311595360587,-13.83000002,-61.0621827299711));
#138816=CARTESIAN_POINT('',(-58.7311595360587,-13.83000002,-61.0621827299711));
#138817=CARTESIAN_POINT('Origin',(-58.7311595360587,-14.33000002,-61.0621827299711));
#138818=CARTESIAN_POINT('Origin',(-56.6451562406488,-13.83000002,-60.2668362080947));
#138819=CARTESIAN_POINT('Origin',(83.2809572255632,-13.8300000199999,-55.24995));
#138820=CARTESIAN_POINT('',(-59.5,-13.83000002,-57.9104088126279));
#138821=CARTESIAN_POINT('Ctrl Pts',(-59.5,-13.83000002,-57.9104088126279));
#138822=CARTESIAN_POINT('Ctrl Pts',(-59.5,-13.83000002,-57.7635265772534));
#138823=CARTESIAN_POINT('Ctrl Pts',(-59.4872752713112,-13.8300000201995,
-57.6187932998334));
#138824=CARTESIAN_POINT('Ctrl Pts',(-59.4620787130117,-13.8300000189704,
-57.4761129700909));
#138825=CARTESIAN_POINT('Ctrl Pts',(-59.4509269987809,-13.8300000184264,
-57.4129642557014));
#138826=CARTESIAN_POINT('Ctrl Pts',(-59.437331564423,-13.8300000175808,
-57.3502178600945));
#138827=CARTESIAN_POINT('Ctrl Pts',(-59.4213112185568,-13.8300000163283,
-57.287866292));
#138828=CARTESIAN_POINT('Ctrl Pts',(-59.3984317821363,-13.8300000145396,
-57.198818979923));
#138829=CARTESIAN_POINT('Ctrl Pts',(-59.370414675224,-13.8300000118888,
-57.1106006512125));
#138830=CARTESIAN_POINT('Ctrl Pts',(-59.3376309673359,-13.8300000085315,
-57.0241300655718));
#138831=CARTESIAN_POINT('Ctrl Pts',(-59.3184526052596,-13.8300000065676,
-56.9735450552971));
#138832=CARTESIAN_POINT('Ctrl Pts',(-59.2977312649336,-13.8300000075911,
-56.9238144825175));
#138833=CARTESIAN_POINT('Ctrl Pts',(-59.2754924251822,-13.8300000109221,
-56.8749259088891));
#138834=CARTESIAN_POINT('Ctrl Pts',(-59.2665370422079,-13.8300000122635,
-56.8552389151069));
#138835=CARTESIAN_POINT('Ctrl Pts',(-59.2573350139603,-13.8300000139055,
-56.8356886347887));
#138836=CARTESIAN_POINT('Ctrl Pts',(-59.2478858052507,-13.8300000154741,
-56.8162751713274));
#138837=CARTESIAN_POINT('Ctrl Pts',(-59.2292919233252,-13.8300000185606,
-56.778073914645));
#138838=CARTESIAN_POINT('Ctrl Pts',(-59.209718687562,-13.8300000193634,
-56.7403307398674));
#138839=CARTESIAN_POINT('Ctrl Pts',(-59.1892544368187,-13.8300000195901,
-56.7032294252422));
#138840=CARTESIAN_POINT('Ctrl Pts',(-59.1734934512784,-13.8300000197646,
-56.6746550449402));
#138841=CARTESIAN_POINT('Ctrl Pts',(-59.1571354382929,-13.8300000198488,
-56.6463349492494));
#138842=CARTESIAN_POINT('Ctrl Pts',(-59.140235511425,-13.8300000188361,
-56.6183428976771));
#138843=CARTESIAN_POINT('Ctrl Pts',(-59.0995076542868,-13.8300000163955,
-56.55088365443));
#138844=CARTESIAN_POINT('Ctrl Pts',(-59.0552769615241,-13.8300000132201,
-56.484916810245));
#138845=CARTESIAN_POINT('Ctrl Pts',(-59.0079404245038,-13.8300000140848,
-56.4210933496162));
#138846=CARTESIAN_POINT('Ctrl Pts',(-58.9649853093651,-13.8300000148695,
-56.3631773238055));
#138847=CARTESIAN_POINT('Ctrl Pts',(-58.9194738360321,-13.8300000183267,
-56.3070268147763));
#138848=CARTESIAN_POINT('Ctrl Pts',(-58.871735578318,-13.8300000195957,
-56.2531111209796));
#138849=CARTESIAN_POINT('',(-59.5,-13.83000002,-174.751208632418));
#138850=CARTESIAN_POINT('',(-59.5,-13.83000002,-57.9132014677655));
#138851=CARTESIAN_POINT('',(-58.9842656455866,-13.8300000191192,-176.271971760299));
#138852=CARTESIAN_POINT('Ctrl Pts',(-58.9842656455851,-13.8300000182384,
-176.271971760298));
#138853=CARTESIAN_POINT('Ctrl Pts',(-59.0284765648189,-13.8300000166394,
-176.214285352614));
#138854=CARTESIAN_POINT('Ctrl Pts',(-59.0700022374986,-13.8300000137057,
-176.154919321393));
#138855=CARTESIAN_POINT('Ctrl Pts',(-59.1087690495582,-13.8300000102313,
-176.094105263608));
#138856=CARTESIAN_POINT('Ctrl Pts',(-59.1458171677555,-13.830000006911,
-176.035987345698));
#138857=CARTESIAN_POINT('Ctrl Pts',(-59.1803457899704,-13.8300000031738,
-175.976545944297));
#138858=CARTESIAN_POINT('Ctrl Pts',(-59.2122555343191,-13.8300000007997,
-175.915955958697));
#138859=CARTESIAN_POINT('Ctrl Pts',(-59.2455714173138,-13.829999998321,
-175.852696007478));
#138860=CARTESIAN_POINT('Ctrl Pts',(-59.2762989800145,-13.8299999975166,
-175.787603392926));
#138861=CARTESIAN_POINT('Ctrl Pts',(-59.3042804787194,-13.8299999996639,
-175.721026919923));
#138862=CARTESIAN_POINT('Ctrl Pts',(-59.3272704921692,-13.8300000014281,
-175.666326704401));
#138863=CARTESIAN_POINT('Ctrl Pts',(-59.3484061154264,-13.8300000052622,
-175.610623961591));
#138864=CARTESIAN_POINT('Ctrl Pts',(-59.3675737697888,-13.8300000097259,
-175.554108016098));
#138865=CARTESIAN_POINT('Ctrl Pts',(-59.3904098382371,-13.830000015044,
-175.486775729355));
#138866=CARTESIAN_POINT('Ctrl Pts',(-59.4103356014117,-13.830000017107,
-175.418690311177));
#138867=CARTESIAN_POINT('Ctrl Pts',(-59.4272061992403,-13.8300000182966,
-175.350275598526));
#138868=CARTESIAN_POINT('Ctrl Pts',(-59.4492409439888,-13.8300000198503,
-175.260918911488));
#138869=CARTESIAN_POINT('Ctrl Pts',(-59.4663032629515,-13.8300000198819,
-175.170862100583));
#138870=CARTESIAN_POINT('Ctrl Pts',(-59.4783606526566,-13.8300000199558,
-175.079983307974));
#138871=CARTESIAN_POINT('Ctrl Pts',(-59.4903258960551,-13.8300000200293,
-174.989799039245));
#138872=CARTESIAN_POINT('Ctrl Pts',(-59.4973624498085,-13.83000002,-174.898805302285));
#138873=CARTESIAN_POINT('Ctrl Pts',(-59.4993876311078,-13.83000002,-174.80687604146));
#138874=CARTESIAN_POINT('Ctrl Pts',(-59.4997955668077,-13.83000002,-174.78835857472));
#138875=CARTESIAN_POINT('Ctrl Pts',(-59.5,-13.83000002,-174.769803126626));
#138876=CARTESIAN_POINT('Ctrl Pts',(-59.5,-13.83000002,-174.751208632418));
#138877=CARTESIAN_POINT('',(-58.9842656455947,-13.83000002,-171.871644662643));
#138878=CARTESIAN_POINT('',(-58.9842656455947,-13.83000002,-176.75597498356));
#138879=CARTESIAN_POINT('',(-58.8436897472855,-13.83000002,-171.237717270032));
#138880=CARTESIAN_POINT('Origin',(-56.7574781748151,-13.83000002,-172.032172120179));
#138881=CARTESIAN_POINT('',(-39.923987884714,-13.83000002,-130.68030635931));
#138882=CARTESIAN_POINT('Ctrl Pts',(-39.923987884714,-13.83000002,-130.68030635931));
#138883=CARTESIAN_POINT('Ctrl Pts',(-46.2315241188232,-13.83000002,-144.198991310165));
#138884=CARTESIAN_POINT('Ctrl Pts',(-52.5377799111353,-13.83000002,-157.718273616974));
#138885=CARTESIAN_POINT('Ctrl Pts',(-58.8436897472855,-13.83000002,-171.237717270032));
#138886=CARTESIAN_POINT('',(-39.5,-13.83000002,-128.768820397718));
#138887=CARTESIAN_POINT('Origin',(-46.1927888980657,-13.83000002,-128.28832565251));
#138888=CARTESIAN_POINT('',(-39.5,-13.83000002,-103.289822573788));
#138889=CARTESIAN_POINT('',(-39.5,-13.83000002,-55.24995));
#138890=CARTESIAN_POINT('',(-39.923987884714,-13.83000002,-101.378336612196));
#138891=CARTESIAN_POINT('Origin',(-46.1924380476731,-13.83000002,-103.773062785017));
#138892=CARTESIAN_POINT('Ctrl Pts',(-58.7311595360587,-13.83000002,-61.0621827299711));
#138893=CARTESIAN_POINT('Ctrl Pts',(-52.4627544636864,-13.83000002,-74.5012048985427));
#138894=CARTESIAN_POINT('Ctrl Pts',(-46.194004389791,-13.83000002,-87.9400661652057));
#138895=CARTESIAN_POINT('Ctrl Pts',(-39.923987884714,-13.83000002,-101.378336612196));
#138896=CARTESIAN_POINT('Ctrl Pts',(-59.5,-13.83000002,-57.9104088126279));
#138897=CARTESIAN_POINT('Ctrl Pts',(-60.,-13.83000002,-57.9104088126279));
#138898=CARTESIAN_POINT('Ctrl Pts',(-60.,-13.33000002,-57.9104088126279));
#138899=CARTESIAN_POINT('Ctrl Pts',(-59.4999999942362,-13.83000002,-57.6984561889535));
#138900=CARTESIAN_POINT('Ctrl Pts',(-59.9998595361682,-13.830000019997,
-57.6561017631169));
#138901=CARTESIAN_POINT('Ctrl Pts',(-60.,-13.3301404965737,-57.6560661294349));
#138902=CARTESIAN_POINT('Ctrl Pts',(-59.4734676164696,-13.83000002,-57.4909684574329));
#138903=CARTESIAN_POINT('Ctrl Pts',(-59.9678925924923,-13.8300000200007,
-57.4071493963694));
#138904=CARTESIAN_POINT('Ctrl Pts',(-59.9681611381428,-13.3302771999651,
-57.4070813040103));
#138905=CARTESIAN_POINT('Ctrl Pts',(-59.3690374493417,-13.83000002,-57.084794303535));
#138906=CARTESIAN_POINT('Ctrl Pts',(-59.8423361500656,-13.8300000199993,
-56.9198740502323));
#138907=CARTESIAN_POINT('Ctrl Pts',(-59.8428449408308,-13.3305433698035,
-56.9196731955795));
#138908=CARTESIAN_POINT('Ctrl Pts',(-59.2901412046916,-13.83000002,-56.8862343787282));
#138909=CARTESIAN_POINT('Ctrl Pts',(-59.7475635896442,-13.8300000199991,
-56.6816942845782));
#138910=CARTESIAN_POINT('Ctrl Pts',(-59.7481694456677,-13.3306727288355,
-56.6814017112205));
#138911=CARTESIAN_POINT('Ctrl Pts',(-59.0883322092721,-13.83000002,-56.5202440244056));
#138912=CARTESIAN_POINT('Ctrl Pts',(-59.5052494150047,-13.8300000200009,
-56.2427365274425));
#138913=CARTESIAN_POINT('Ctrl Pts',(-59.5059986510887,-13.3309100420639,
-56.2422140639419));
#138914=CARTESIAN_POINT('Ctrl Pts',(-58.9625961123716,-13.83000002,-56.3476402489859));
#138915=CARTESIAN_POINT('Ctrl Pts',(-59.3543264440767,-13.8300000199994,
-56.0357389914811));
#138916=CARTESIAN_POINT('Ctrl Pts',(-59.3551153361278,-13.3310213578394,
-56.0350898960933));
#138917=CARTESIAN_POINT('Ctrl Pts',(-58.6747340315543,-13.83000002,-56.0424403288692));
#138918=CARTESIAN_POINT('Ctrl Pts',(-59.0088785326184,-13.8300000200005,
-55.6697700183809));
#138919=CARTESIAN_POINT('Ctrl Pts',(-59.0096808365833,-13.3312174510841,
-55.6688506341933));
#138920=CARTESIAN_POINT('Ctrl Pts',(-58.5134387215907,-13.83000002,-55.9093078011895));
#138921=CARTESIAN_POINT('Ctrl Pts',(-58.8153502371001,-13.8300000200007,
-55.510138275251));
#138922=CARTESIAN_POINT('Ctrl Pts',(-58.8161264695431,-13.3313025928017,
-55.509091871258));
#138923=CARTESIAN_POINT('Ctrl Pts',(-58.3343300343787,-13.83000002,-55.796263236946));
#138924=CARTESIAN_POINT('Ctrl Pts',(-58.6004643384094,-13.83000002,-55.3745979500414));
#138925=CARTESIAN_POINT('Ctrl Pts',(-58.6011960412544,-13.3313747072047,
-55.3734386342923));
#138926=CARTESIAN_POINT('',(-60.,-13.33000002,-57.9104088126279));
#138927=CARTESIAN_POINT('Ctrl Pts',(-58.616886279706,-13.331369406142,-55.3834096347511));
#138928=CARTESIAN_POINT('Ctrl Pts',(-58.8255570887224,-13.3312984580582,
-55.5168999903146));
#138929=CARTESIAN_POINT('Ctrl Pts',(-59.0138940511391,-13.3312150861459,
-55.6733176015169));
#138930=CARTESIAN_POINT('Ctrl Pts',(-59.3551153360854,-13.3310213846274,
-56.0350898961282));
#138931=CARTESIAN_POINT('Ctrl Pts',(-59.5059986510485,-13.3309100688549,
-56.2422140639699));
#138932=CARTESIAN_POINT('Ctrl Pts',(-59.7481694456352,-13.3306727556329,
-56.6814017112362));
#138933=CARTESIAN_POINT('Ctrl Pts',(-59.8428449408035,-13.3305433966043,
-56.9196731955903));
#138934=CARTESIAN_POINT('Ctrl Pts',(-59.9681611381284,-13.3302772267731,
-57.4070813040139));
#138935=CARTESIAN_POINT('Ctrl Pts',(-59.9999999999925,-13.3301405233853,
-57.6560661294368));
#138936=CARTESIAN_POINT('Ctrl Pts',(-60.,-13.33000002,-57.9104088126279));
#138937=CARTESIAN_POINT('Origin',(-59.5,-13.33000002,-57.9104088126279));
#138938=CARTESIAN_POINT('Ctrl Pts',(-58.6015900410175,-13.341475878746,
-55.3737206461527));
#138939=CARTESIAN_POINT('Ctrl Pts',(-59.9999999999999,-13.3385258667613,
-56.2566220904403));
#138940=CARTESIAN_POINT('Ctrl Pts',(-60.,-13.3330000856764,-57.9104187956072));
#138941=CARTESIAN_POINT('Ctrl Pts',(-58.60257249872,-13.168900596776,-55.3737643179337));
#138942=CARTESIAN_POINT('Ctrl Pts',(-59.9999999999979,-13.1673253991122,
-56.2568074836807));
#138943=CARTESIAN_POINT('Ctrl Pts',(-60.,-13.1643269532066,-57.9098552131434));
#138944=CARTESIAN_POINT('Ctrl Pts',(-58.6028748593257,-12.996307708263,
-55.373777702491));
#138945=CARTESIAN_POINT('Ctrl Pts',(-60.0000000000015,-12.9960742306928,
-56.2568641234304));
#138946=CARTESIAN_POINT('Ctrl Pts',(-60.,-12.9956563413871,-57.9096813403539));
#138947=CARTESIAN_POINT('Ctrl Pts',(-58.6024972248876,-12.82373973381,-55.3737609414448));
#138948=CARTESIAN_POINT('Ctrl Pts',(-60.,-12.8248749582876,-56.2567930570856));
#138949=CARTESIAN_POINT('Ctrl Pts',(-60.,-12.827000187199,-57.9098981644024));
#138950=CARTESIAN_POINT('',(-60.,-12.83000002,-57.909894348981));
#138951=CARTESIAN_POINT('Ctrl Pts',(-60.,-12.83000002,-57.909894348981));
#138952=CARTESIAN_POINT('Ctrl Pts',(-59.9999999999994,-12.8299467047078,
-57.6556666887755));
#138953=CARTESIAN_POINT('Ctrl Pts',(-59.9681892936708,-12.8298948271699,
-57.4067922228919));
#138954=CARTESIAN_POINT('Ctrl Pts',(-59.8429857054854,-12.8297938186589,
-56.9195951650652));
#138955=CARTESIAN_POINT('Ctrl Pts',(-59.7483921213374,-12.8297447259539,
-56.6814121423212));
#138956=CARTESIAN_POINT('Ctrl Pts',(-59.5064293021062,-12.8296546610246,
-56.2423688578594));
#138957=CARTESIAN_POINT('Ctrl Pts',(-59.355679816355,-12.829612413403,-56.035304631569));
#138958=CARTESIAN_POINT('Ctrl Pts',(-59.0146398555283,-12.8295388666295,
-55.6734793535298));
#138959=CARTESIAN_POINT('Ctrl Pts',(-58.8263448628416,-12.8295072025013,
-55.5169944929564));
#138960=CARTESIAN_POINT('Ctrl Pts',(-58.6177174583935,-12.8294802501407,
-55.3834349955049));
#138961=CARTESIAN_POINT('Origin',(-60.,-12.9674754043409,-167.271246742335));
#138962=CARTESIAN_POINT('Ctrl Pts',(-60.,-12.83000002,-57.909894348981));
#138963=CARTESIAN_POINT('Ctrl Pts',(-60.,-12.33000002,-57.909894348981));
#138964=CARTESIAN_POINT('Ctrl Pts',(-59.5,-12.33000002,-57.909894348981));
#138965=CARTESIAN_POINT('Ctrl Pts',(-60.,-12.8299467103192,-57.6556666887753));
#138966=CARTESIAN_POINT('Ctrl Pts',(-59.9999466862306,-12.33000002,-57.6556802065741));
#138967=CARTESIAN_POINT('Ctrl Pts',(-59.4999999942389,-12.33000002,-57.6980379098391));
#138968=CARTESIAN_POINT('Ctrl Pts',(-59.9681892936719,-12.8298948327809,
-57.4067922228916));
#138969=CARTESIAN_POINT('Ctrl Pts',(-59.9680873501793,-12.33000002,-57.4068180594886));
#138970=CARTESIAN_POINT('Ctrl Pts',(-59.4734910794084,-12.33000002,-57.4906424667705));
#138971=CARTESIAN_POINT('Ctrl Pts',(-59.8429857054876,-12.8297938242694,
-56.9195951650643));
#138972=CARTESIAN_POINT('Ctrl Pts',(-59.8427924853442,-12.33000002,-56.9196714028451));
#138973=CARTESIAN_POINT('Ctrl Pts',(-59.3691547532245,-12.33000002,-57.0846448139696));
#138974=CARTESIAN_POINT('Ctrl Pts',(-59.74839212134,-12.8297447315641,-56.6814121423199));
#138975=CARTESIAN_POINT('Ctrl Pts',(-59.748161991806,-12.3300000200005,
-56.6815232165248));
#138976=CARTESIAN_POINT('Ctrl Pts',(-59.290326767749,-12.33000002,-56.8861589103251));
#138977=CARTESIAN_POINT('Ctrl Pts',(-59.5064293021094,-12.8296546666343,
-56.2423688578572));
#138978=CARTESIAN_POINT('Ctrl Pts',(-59.5061445952809,-12.3300000199994,
-56.2425672751971));
#138979=CARTESIAN_POINT('Ctrl Pts',(-59.0886910851255,-12.33000002,-56.5202894131685));
#138980=CARTESIAN_POINT('Ctrl Pts',(-59.3556798163584,-12.8296124190124,
-56.0353046315662));
#138981=CARTESIAN_POINT('Ctrl Pts',(-59.3553799746847,-12.3300000199993,
-56.035551183714));
#138982=CARTESIAN_POINT('Ctrl Pts',(-58.9630665125599,-12.33000002,-56.3477358485963));
#138983=CARTESIAN_POINT('Ctrl Pts',(-59.0105155640199,-12.8295379828168,
-55.6691036993668));
#138984=CARTESIAN_POINT('Ctrl Pts',(-59.010210485167,-12.3300000200007,
-55.6694530297022));
#138985=CARTESIAN_POINT('Ctrl Pts',(-58.6754296377554,-12.33000002,-56.0425683262376));
#138986=CARTESIAN_POINT('Ctrl Pts',(-58.8171130576816,-12.8295056604635,
-55.509345500426));
#138987=CARTESIAN_POINT('Ctrl Pts',(-58.8168178148591,-12.3300000200035,
-55.5097431582292));
#138988=CARTESIAN_POINT('Ctrl Pts',(-58.5142608782156,-12.33000002,-55.909436466106));
#138989=CARTESIAN_POINT('Ctrl Pts',(-58.6023581204233,-12.8294782784431,
-55.3736658212353));
#138990=CARTESIAN_POINT('Ctrl Pts',(-58.6020797386365,-12.33000002,-55.3741064461589));
#138991=CARTESIAN_POINT('Ctrl Pts',(-58.3352984336861,-12.33000002,-55.7963700340195));
#138992=CARTESIAN_POINT('',(-59.5,-12.33000002,-57.909894348981));
#138993=CARTESIAN_POINT('Ctrl Pts',(-58.8765127194368,-12.330000020523,
-56.2580153373943));
#138994=CARTESIAN_POINT('Ctrl Pts',(-58.9314422323999,-12.3300000222489,
-56.3204146345372));
#138995=CARTESIAN_POINT('Ctrl Pts',(-58.9833702988531,-12.3300000263278,
-56.3857545682232));
#138996=CARTESIAN_POINT('Ctrl Pts',(-59.03181875348,-12.3300000260899,-56.4533283814535));
#138997=CARTESIAN_POINT('Ctrl Pts',(-59.0712668703441,-12.3300000258961,
-56.5083489120731));
#138998=CARTESIAN_POINT('Ctrl Pts',(-59.1084086074742,-12.3300000229817,
-56.5648494607718));
#138999=CARTESIAN_POINT('Ctrl Pts',(-59.1430095719442,-12.3300000210667,
-56.6224388634737));
#139000=CARTESIAN_POINT('Ctrl Pts',(-59.159023041084,-12.3300000201805,
-56.6490914766905));
#139001=CARTESIAN_POINT('Ctrl Pts',(-59.1745444070377,-12.3300000202428,
-56.6760375771056));
#139002=CARTESIAN_POINT('Ctrl Pts',(-59.1895265613474,-12.3300000204054,
-56.7032144429067));
#139003=CARTESIAN_POINT('Ctrl Pts',(-59.2106099692481,-12.3300000206343,
-56.7414586723615));
#139004=CARTESIAN_POINT('Ctrl Pts',(-59.2307479204425,-12.3300000215029,
-56.7803865151708));
#139005=CARTESIAN_POINT('Ctrl Pts',(-59.2498439227782,-12.3300000247794,
-56.8197986433709));
#139006=CARTESIAN_POINT('Ctrl Pts',(-59.2732105276413,-12.3300000287887,
-56.868024843299));
#139007=CARTESIAN_POINT('Ctrl Pts',(-59.2950576358119,-12.3300000325183,
-56.9170923843778));
#139008=CARTESIAN_POINT('Ctrl Pts',(-59.3153788043346,-12.330000032611,
-56.9670066834514));
#139009=CARTESIAN_POINT('Ctrl Pts',(-59.3234660778806,-12.3300000326479,
-56.9868712197854));
#139010=CARTESIAN_POINT('Ctrl Pts',(-59.3313111418656,-12.3300000321978,
-57.0068701006058));
#139011=CARTESIAN_POINT('Ctrl Pts',(-59.3389114029545,-12.3300000313575,
-57.0270043936979));
#139012=CARTESIAN_POINT('Ctrl Pts',(-59.3711805702217,-12.3300000277898,
-57.1124905189758));
#139013=CARTESIAN_POINT('Ctrl Pts',(-59.398787967634,-12.3300000251841,
-57.1996595335916));
#139014=CARTESIAN_POINT('Ctrl Pts',(-59.4213798740153,-12.3300000234584,
-57.2876290029532));
#139015=CARTESIAN_POINT('Ctrl Pts',(-59.4552355589985,-12.3300000208724,
-57.4194579240094));
#139016=CARTESIAN_POINT('Ctrl Pts',(-59.4782525129323,-12.3300000202447,
-57.5530362590468));
#139017=CARTESIAN_POINT('Ctrl Pts',(-59.4902475546029,-12.3300000200727,
-57.6884558476609));
#139018=CARTESIAN_POINT('Ctrl Pts',(-59.4967374324384,-12.3300000199797,
-57.7617241705875));
#139019=CARTESIAN_POINT('Ctrl Pts',(-59.5,-12.33000002,-57.8355316833216));
#139020=CARTESIAN_POINT('Ctrl Pts',(-59.5,-12.33000002,-57.909894348981));
#139021=CARTESIAN_POINT('Origin',(-59.5,-12.83000002,-57.909894348981));
#139022=CARTESIAN_POINT('Ctrl Pts',(-58.2828791719688,-11.838774304476,
-60.8508735991007));
#139023=CARTESIAN_POINT('Ctrl Pts',(-58.2906927660831,-12.33000002,-60.8545178210735));
#139024=CARTESIAN_POINT('Ctrl Pts',(-58.7359481105893,-12.33000002,-61.0621827299711));
#139025=CARTESIAN_POINT('Ctrl Pts',(-58.3445491382077,-11.8393573204241,
-60.7186709323925));
#139026=CARTESIAN_POINT('Ctrl Pts',(-58.3533698277338,-12.3300000200013,
-60.7214865958624));
#139027=CARTESIAN_POINT('Ctrl Pts',(-58.8284361535292,-12.33000002,-60.863878626764));
#139028=CARTESIAN_POINT('Ctrl Pts',(-58.3766060098775,-11.8396582665817,
-60.575610749785));
#139029=CARTESIAN_POINT('Ctrl Pts',(-58.3860794582448,-12.330000020003,
-60.5770127531963));
#139030=CARTESIAN_POINT('Ctrl Pts',(-58.8765127155019,-12.33000002,-60.64928853347));
#139031=CARTESIAN_POINT('Ctrl Pts',(-58.376606009879,-11.839658266657,-60.42825533736));
#139032=CARTESIAN_POINT('Ctrl Pts',(-58.3860794606436,-12.33000002,-60.42825533736));
#139033=CARTESIAN_POINT('Ctrl Pts',(-58.8765127194474,-12.33000002,-60.42825533736));
#139034=CARTESIAN_POINT('',(-58.7359481105893,-12.33000002,-61.0621827299711));
#139035=CARTESIAN_POINT('Origin',(-58.7359481105893,-11.83000002,-61.0621827299711));
#139036=CARTESIAN_POINT('Origin',(-56.649087690066,-12.33000002,-60.2675479548571));
#139037=CARTESIAN_POINT('Origin',(83.2809572255632,-12.3300000199999,-55.24995));
#139038=CARTESIAN_POINT('',(-39.9232693735648,-12.33000002,-101.394976652855));
#139039=CARTESIAN_POINT('Ctrl Pts',(-39.9232693735648,-12.33000002,-101.394976652855));
#139040=CARTESIAN_POINT('Ctrl Pts',(-46.1948314689912,-12.33000002,-87.9510241496856));
#139041=CARTESIAN_POINT('Ctrl Pts',(-52.4655100689676,-12.33000002,-74.5066595330064));
#139042=CARTESIAN_POINT('Ctrl Pts',(-58.7359481105893,-12.33000002,-61.0621827299711));
#139043=CARTESIAN_POINT('',(-39.5,-12.33000002,-103.303524786513));
#139044=CARTESIAN_POINT('Origin',(-46.1908778693233,-12.33000002,-103.784865184756));
#139045=CARTESIAN_POINT('',(-39.5,-12.33000002,-128.755118184993));
#139046=CARTESIAN_POINT('',(-39.5,-12.33000002,-55.24995));
#139047=CARTESIAN_POINT('',(-39.9232693735648,-12.33000002,-130.663666318651));
#139048=CARTESIAN_POINT('Origin',(-46.1904260133999,-12.33000002,-128.271059668218));
#139049=CARTESIAN_POINT('',(-58.8484691650909,-12.33000002,-171.237717270032));
#139050=CARTESIAN_POINT('Ctrl Pts',(-58.8484691650909,-12.33000002,-171.237717270032));
#139051=CARTESIAN_POINT('Ctrl Pts',(-52.5405278046811,-12.33000002,-157.712819732223));
#139052=CARTESIAN_POINT('Ctrl Pts',(-46.2323452217992,-12.33000002,-144.188034690057));
#139053=CARTESIAN_POINT('Ctrl Pts',(-39.9232693735648,-12.33000002,-130.663666318651));
#139054=CARTESIAN_POINT('',(-58.9890336736409,-12.33000002,-171.871644662643));
#139055=CARTESIAN_POINT('Origin',(-56.7618024059963,-12.33000002,-172.033247591146));
#139056=CARTESIAN_POINT('',(-58.9890336736409,-12.3300000204739,-176.26629097911));
#139057=CARTESIAN_POINT('',(-58.9890336736409,-12.33000002,-171.871644662643));
#139058=CARTESIAN_POINT('',(-59.5,-12.33000002,-174.751778045594));
#139059=CARTESIAN_POINT('Ctrl Pts',(-59.5,-12.33000002,-174.751778045594));
#139060=CARTESIAN_POINT('Ctrl Pts',(-59.5,-12.33000002,-174.844927230273));
#139061=CARTESIAN_POINT('Ctrl Pts',(-59.4948737621761,-12.3300000199839,
-174.937101433735));
#139062=CARTESIAN_POINT('Ctrl Pts',(-59.4847164002782,-12.3300000200162,
-175.028427073489));
#139063=CARTESIAN_POINT('Ctrl Pts',(-59.474481566957,-12.3300000200487,
-175.120449264903));
#139064=CARTESIAN_POINT('Ctrl Pts',(-59.4591385334095,-12.3300000199961,
-175.211609900805));
#139065=CARTESIAN_POINT('Ctrl Pts',(-59.4387322722171,-12.3300000210573,
-175.302031274496));
#139066=CARTESIAN_POINT('Ctrl Pts',(-59.4350695133288,-12.3300000212478,
-175.318261179968));
#139067=CARTESIAN_POINT('Ctrl Pts',(-59.4312434964565,-12.3300000214808,
-175.334467250166));
#139068=CARTESIAN_POINT('Ctrl Pts',(-59.4272543062711,-12.330000021774,
-175.350650168439));
#139069=CARTESIAN_POINT('Ctrl Pts',(-59.4106840236565,-12.3300000229918,
-175.417870711165));
#139070=CARTESIAN_POINT('Ctrl Pts',(-59.3911649601375,-12.3300000250948,
-175.484771053152));
#139071=CARTESIAN_POINT('Ctrl Pts',(-59.3688362082559,-12.3300000304207,
-175.550947464116));
#139072=CARTESIAN_POINT('Ctrl Pts',(-59.3452983767326,-12.330000036035,
-175.620707261724));
#139073=CARTESIAN_POINT('Ctrl Pts',(-59.318757276387,-12.3300000404266,
-175.689252183756));
#139074=CARTESIAN_POINT('Ctrl Pts',(-59.2894219594715,-12.3300000414655,
-175.756217087946));
#139075=CARTESIAN_POINT('Ctrl Pts',(-59.265578831198,-12.3300000423099,
-175.810644752902));
#139076=CARTESIAN_POINT('Ctrl Pts',(-59.2398885853161,-12.3300000411891,
-175.864029149378));
#139077=CARTESIAN_POINT('Ctrl Pts',(-59.2124386122788,-12.330000039031,
-175.916169632722));
#139078=CARTESIAN_POINT('Ctrl Pts',(-59.1785809256147,-12.3300000363691,
-175.980481395257));
#139079=CARTESIAN_POINT('Ctrl Pts',(-59.1417731864694,-12.3300000322739,
-176.043500821863));
#139080=CARTESIAN_POINT('Ctrl Pts',(-59.1021371288072,-12.3300000288604,
-176.105011973128));
#139081=CARTESIAN_POINT('Ctrl Pts',(-59.0666804433847,-12.3300000258069,
-176.16003716153));
#139082=CARTESIAN_POINT('Ctrl Pts',(-59.0289595515132,-12.3300000233307,
-176.21385559589));
#139083=CARTESIAN_POINT('Ctrl Pts',(-58.9890336736408,-12.3300000218957,
-176.26629097911));
#139084=CARTESIAN_POINT('',(-59.5,-12.33000002,-174.749818876635));
#139085=CARTESIAN_POINT('Origin',(0.,-12.9675000200281,-60.64995));
#139086=CARTESIAN_POINT('',(-39.4702993039609,-11.842906113671,-101.183667521985));
#139087=CARTESIAN_POINT('',(-39.532390596215,-6.25584930029837,-99.8717339663452));
#139088=CARTESIAN_POINT('Ctrl Pts',(-39.4702993039609,-11.842906113671,
-101.183667521985));
#139089=CARTESIAN_POINT('Ctrl Pts',(-39.4717448060415,-11.4004606629204,
-101.15354495628));
#139090=CARTESIAN_POINT('Ctrl Pts',(-39.4740433475117,-10.9574131907765,
-101.105623514581));
#139091=CARTESIAN_POINT('Ctrl Pts',(-39.4806656803776,-10.023475093596,
-100.967196709792));
#139092=CARTESIAN_POINT('Ctrl Pts',(-39.4851934915317,-9.53196093055967,
-100.872391456905));
#139093=CARTESIAN_POINT('Ctrl Pts',(-39.5012939059505,-8.09530479773136,
-100.533838938409));
#139094=CARTESIAN_POINT('Ctrl Pts',(-39.5154754399064,-7.1657280964986,
-100.234102969279));
#139095=CARTESIAN_POINT('Ctrl Pts',(-39.532390596256,-6.25584930059377,
-99.8717339663646));
#139096=CARTESIAN_POINT('Ctrl Pts',(-58.2828791719688,-11.838774304476,
-60.8508735991007));
#139097=CARTESIAN_POINT('Ctrl Pts',(-52.0124594137882,-11.8397106642502,
-74.2953500811619));
#139098=CARTESIAN_POINT('Ctrl Pts',(-45.741803891981,-11.8408803347909,
-87.7397145657271));
#139099=CARTESIAN_POINT('Ctrl Pts',(-39.4702993039609,-11.842906113671,
-101.183667521985));
#139100=CARTESIAN_POINT('Ctrl Pts',(-39.532390596256,-6.25584930059377,
-99.8717339663646));
#139101=CARTESIAN_POINT('Ctrl Pts',(-45.6775416784359,-6.24451367567336,
-86.8752616232929));
#139102=CARTESIAN_POINT('Ctrl Pts',(-51.7945419641194,-6.23776491028108,
-73.8650082774501));
#139103=CARTESIAN_POINT('Ctrl Pts',(-57.9034184448965,-6.23235646472971,
-60.8508735991007));
#139104=CARTESIAN_POINT('Ctrl Pts',(-57.9983536018174,-6.23763109620483,
-60.42825533736));
#139105=CARTESIAN_POINT('Ctrl Pts',(-57.9336485918015,-5.68000002,-60.4282553373601));
#139106=CARTESIAN_POINT('Ctrl Pts',(-58.4950211556756,-5.68000001999999,
-60.42825533736));
#139107=CARTESIAN_POINT('Ctrl Pts',(-57.9983536015968,-6.23763109430342,
-60.5741740417057));
#139108=CARTESIAN_POINT('Ctrl Pts',(-57.9336485820782,-5.68000001999705,
-60.5646181976572));
#139109=CARTESIAN_POINT('Ctrl Pts',(-58.4950211389271,-5.68000001999999,
-60.6471359124214));
#139110=CARTESIAN_POINT('Ctrl Pts',(-57.9664686566087,-6.23586779901857,
-60.7174374956191));
#139111=CARTESIAN_POINT('Ctrl Pts',(-57.9064697980399,-5.68000002000461,
-60.6982006050192));
#139112=CARTESIAN_POINT('Ctrl Pts',(-58.4475018470026,-5.68000001999999,
-60.8620252214211));
#139113=CARTESIAN_POINT('Ctrl Pts',(-57.9034184448965,-6.23235646472971,
-60.8508735991007));
#139114=CARTESIAN_POINT('Ctrl Pts',(-57.8507724536939,-5.68000001999999,
-60.826158857425));
#139115=CARTESIAN_POINT('Ctrl Pts',(-58.3535376001277,-5.68000001999999,
-61.0621827299711));
#139116=CARTESIAN_POINT('',(-58.3535376001277,-5.68000001999999,-61.0621827299711));
#139117=CARTESIAN_POINT('Origin',(-58.3535376001277,-6.18000001999999,-61.0621827299711));
#139118=CARTESIAN_POINT('Origin',(-56.3184043809282,-5.68000001999999,-60.2809146158445));
#139119=CARTESIAN_POINT('Origin',(83.2809572255632,-5.68000001999993,-55.24995));
#139120=CARTESIAN_POINT('',(-59.5,-5.68000001999999,-58.1246434856214));
#139121=CARTESIAN_POINT('Ctrl Pts',(-59.5,-5.68000001999999,-58.1246434856214));
#139122=CARTESIAN_POINT('Ctrl Pts',(-59.5,-5.68000001999999,-58.0267693974302));
#139123=CARTESIAN_POINT('Ctrl Pts',(-59.4943836373774,-5.68000001999999,
-57.9298568609375));
#139124=CARTESIAN_POINT('Ctrl Pts',(-59.4831953566826,-5.68000001999999,
-57.8338865707097));
#139125=CARTESIAN_POINT('Ctrl Pts',(-59.4720070759879,-5.68000001999999,
-57.7379162804819));
#139126=CARTESIAN_POINT('Ctrl Pts',(-59.455245939737,-5.68000002032169,
-57.6428888905768));
#139127=CARTESIAN_POINT('Ctrl Pts',(-59.4329732446822,-5.68000001967878,
-57.548806713199));
#139128=CARTESIAN_POINT('Ctrl Pts',(-59.4211509304573,-5.68000001933753,
-57.4988680299284));
#139129=CARTESIAN_POINT('Ctrl Pts',(-59.4077647649328,-5.68000001901105,
-57.4491949286452));
#139130=CARTESIAN_POINT('Ctrl Pts',(-59.392823215944,-5.68000001896984,
-57.3997884127162));
#139131=CARTESIAN_POINT('Ctrl Pts',(-59.3572029910943,-5.68000001887159,
-57.2820046937892));
#139132=CARTESIAN_POINT('Ctrl Pts',(-59.3124912608683,-5.68000001980192,
-57.1660436798562));
#139133=CARTESIAN_POINT('Ctrl Pts',(-59.2602343180242,-5.68000001992935,
-57.0554150259142));
#139134=CARTESIAN_POINT('Ctrl Pts',(-59.2518183841936,-5.68000001994988,
-57.0375983803036));
#139135=CARTESIAN_POINT('Ctrl Pts',(-59.2431998624486,-5.68000001996158,
-57.0198940947568));
#139136=CARTESIAN_POINT('Ctrl Pts',(-59.2343787360437,-5.68000001996808,
-57.002302188435));
#139137=CARTESIAN_POINT('Ctrl Pts',(-59.1884199680699,-5.68000002000192,
-56.9106469616823));
#139138=CARTESIAN_POINT('Ctrl Pts',(-59.136987353068,-5.68000001969244,
-56.8220653476532));
#139139=CARTESIAN_POINT('Ctrl Pts',(-59.0800102832677,-5.68000001903091,
-56.7365294000527));
#139140=CARTESIAN_POINT('Ctrl Pts',(-59.0296633903434,-5.68000001844636,
-56.6609469032671));
#139141=CARTESIAN_POINT('Ctrl Pts',(-58.974589118716,-5.68000001849974,
-56.587361786818));
#139142=CARTESIAN_POINT('Ctrl Pts',(-58.9158341632416,-5.68000001947823,
-56.5172160817437));
#139143=CARTESIAN_POINT('Ctrl Pts',(-58.8953629897436,-5.68000001981915,
-56.4927761874893));
#139144=CARTESIAN_POINT('Ctrl Pts',(-58.8744667885101,-5.68000001977524,
-56.468763578303));
#139145=CARTESIAN_POINT('Ctrl Pts',(-58.8531845723455,-5.68000001964656,
-56.4452355795564));
#139146=CARTESIAN_POINT('Ctrl Pts',(-58.8093620434502,-5.68000001938158,
-56.396788726233));
#139147=CARTESIAN_POINT('Ctrl Pts',(-58.7638692855098,-5.6800000177515,
-56.3502656276834));
#139148=CARTESIAN_POINT('Ctrl Pts',(-58.7166522079594,-5.68000001767937,
-56.3056325667689));
#139149=CARTESIAN_POINT('Ctrl Pts',(-58.6815782873768,-5.68000001762579,
-56.2724781125951));
#139150=CARTESIAN_POINT('Ctrl Pts',(-58.6455688559318,-5.680000018255,-56.2403749966795));
#139151=CARTESIAN_POINT('Ctrl Pts',(-58.6086287388195,-5.68000001901365,
-56.2093177964104));
#139152=CARTESIAN_POINT('Ctrl Pts',(-58.6017994579946,-5.68000001915391,
-56.203576116122));
#139153=CARTESIAN_POINT('Ctrl Pts',(-58.5949404401232,-5.68000001924633,
-56.1978709269311));
#139154=CARTESIAN_POINT('Ctrl Pts',(-58.5880516973688,-5.68000001929971,
-56.1922018795935));
#139155=CARTESIAN_POINT('Ctrl Pts',(-58.5576786887571,-5.68000001953509,
-56.1672066040054));
#139156=CARTESIAN_POINT('Ctrl Pts',(-58.5266453103076,-5.68000002035884,
-56.1428933547174));
#139157=CARTESIAN_POINT('Ctrl Pts',(-58.4950211556753,-5.68000001545765,
-56.119278519931));
#139158=CARTESIAN_POINT('',(-59.5,-5.68000001999999,-174.511260182693));
#139159=CARTESIAN_POINT('',(-59.5,-5.68000001999999,-58.1042606444049));
#139160=CARTESIAN_POINT('',(-58.6082745331212,-5.68000001999999,-176.427328712824));
#139161=CARTESIAN_POINT('Ctrl Pts',(-58.6082745331212,-5.6800000199515,
-176.427328712824));
#139162=CARTESIAN_POINT('Ctrl Pts',(-58.6185667882716,-5.68000001995871,
-176.418676244678));
#139163=CARTESIAN_POINT('Ctrl Pts',(-58.628783204882,-5.68000001996413,
-176.409943629197));
#139164=CARTESIAN_POINT('Ctrl Pts',(-58.6389210444463,-5.68000001996836,
-176.401132572172));
#139165=CARTESIAN_POINT('Ctrl Pts',(-58.7108573560278,-5.68000001999836,
-176.338610874187));
#139166=CARTESIAN_POINT('Ctrl Pts',(-58.7792948136848,-5.68000001999946,
-176.271947442152));
#139167=CARTESIAN_POINT('Ctrl Pts',(-58.8440583693357,-5.68000001994282,
-176.201117847417));
#139168=CARTESIAN_POINT('Ctrl Pts',(-58.8596678064677,-5.68000001992916,
-176.184046361841));
#139169=CARTESIAN_POINT('Ctrl Pts',(-58.875063977428,-5.6800000199106,-176.166733035301));
#139170=CARTESIAN_POINT('Ctrl Pts',(-58.8902447330317,-5.68000001988414,
-176.149177868712));
#139171=CARTESIAN_POINT('Ctrl Pts',(-58.9227212058659,-5.68000001982754,
-176.111621774291));
#139172=CARTESIAN_POINT('Ctrl Pts',(-58.9541409398416,-5.68000001973543,
-176.072997877296));
#139173=CARTESIAN_POINT('Ctrl Pts',(-58.984359985497,-5.68000001956971,
-176.033520885199));
#139174=CARTESIAN_POINT('Ctrl Pts',(-59.0268866354123,-5.6800000193365,
-175.977965715067));
#139175=CARTESIAN_POINT('Ctrl Pts',(-59.0670052242284,-5.68000001940972,
-175.920749643185));
#139176=CARTESIAN_POINT('Ctrl Pts',(-59.1043833915299,-5.68000001957814,
-175.862401050087));
#139177=CARTESIAN_POINT('Ctrl Pts',(-59.1540049590066,-5.68000001980172,
-175.784940092029));
#139178=CARTESIAN_POINT('Ctrl Pts',(-59.199181192514,-5.68000001997512,
-175.70506448782));
#139179=CARTESIAN_POINT('Ctrl Pts',(-59.239965893642,-5.68000001998963,
-175.622670099363));
#139180=CARTESIAN_POINT('Ctrl Pts',(-59.2487993257315,-5.68000001999278,
-175.604824553978));
#139181=CARTESIAN_POINT('Ctrl Pts',(-59.2574265918444,-5.6800000199934,
-175.586860742585));
#139182=CARTESIAN_POINT('Ctrl Pts',(-59.2658479718429,-5.68000001999155,
-175.568777423473));
#139183=CARTESIAN_POINT('Ctrl Pts',(-59.2686911708562,-5.68000001999092,
-175.5626721919));
#139184=CARTESIAN_POINT('Ctrl Pts',(-59.2715106588893,-5.68000001999007,
-175.556553812533));
#139185=CARTESIAN_POINT('Ctrl Pts',(-59.2743064287832,-5.68000001998893,
-175.550422281673));
#139186=CARTESIAN_POINT('Ctrl Pts',(-59.3235845105522,-5.68000001996885,
-175.44234826609));
#139187=CARTESIAN_POINT('Ctrl Pts',(-59.3657187337311,-5.68000001965404,
-175.32923562655));
#139188=CARTESIAN_POINT('Ctrl Pts',(-59.3992004790972,-5.68000001961977,
-175.214817860028));
#139189=CARTESIAN_POINT('Ctrl Pts',(-59.4149912346775,-5.68000001960361,
-175.160855828914));
#139190=CARTESIAN_POINT('Ctrl Pts',(-59.4289384514506,-5.68000001972945,
-175.106577823109));
#139191=CARTESIAN_POINT('Ctrl Pts',(-59.441030144846,-5.68000001987896,
-175.051984501471));
#139192=CARTESIAN_POINT('Ctrl Pts',(-59.4606225263251,-5.68000002012122,
-174.963525991253));
#139193=CARTESIAN_POINT('Ctrl Pts',(-59.4753677357896,-5.68000001999999,
-174.874236789973));
#139194=CARTESIAN_POINT('Ctrl Pts',(-59.485211909548,-5.68000001999999,
-174.784118621956));
#139195=CARTESIAN_POINT('Ctrl Pts',(-59.4950560833064,-5.68000001999999,
-174.694000453939));
#139196=CARTESIAN_POINT('Ctrl Pts',(-59.5,-5.68000001999999,-174.603053692373));
#139197=CARTESIAN_POINT('Ctrl Pts',(-59.5,-5.68000001999999,-174.511260182694));
#139198=CARTESIAN_POINT('',(-58.6082745331205,-5.68000001999999,-171.871644662643));
#139199=CARTESIAN_POINT('',(-58.6082745331205,-5.68000001999999,-176.785131631246));
#139200=CARTESIAN_POINT('',(-58.4667946194619,-5.68000001999999,-171.237717270032));
#139201=CARTESIAN_POINT('Origin',(-56.431269633621,-5.68000001999999,-172.018134872838));
#139202=CARTESIAN_POINT('',(-39.9791515366304,-5.68000001999998,-131.975599874271));
#139203=CARTESIAN_POINT('Ctrl Pts',(-39.9791515366304,-5.68000001999998,
-131.975599874271));
#139204=CARTESIAN_POINT('Ctrl Pts',(-46.164205183661,-5.68000001999998,
-145.052367414711));
#139205=CARTESIAN_POINT('Ctrl Pts',(-52.3196619691199,-5.68000001999999,
-158.143093167052));
#139206=CARTESIAN_POINT('Ctrl Pts',(-58.4667946194619,-5.68000001999999,
-171.237717270032));
#139207=CARTESIAN_POINT('',(-39.5,-5.68000001999998,-129.839692850412));
#139208=CARTESIAN_POINT('Ctrl Pts',(-39.5,-5.68000001999998,-129.839692850412));
#139209=CARTESIAN_POINT('Ctrl Pts',(-39.5,-5.68000001999998,-130.0740119535));
#139210=CARTESIAN_POINT('Ctrl Pts',(-39.516697911888,-5.68000001999998,
-130.308218863705));
#139211=CARTESIAN_POINT('Ctrl Pts',(-39.5492808611242,-5.68000001999998,
-130.539004174614));
#139212=CARTESIAN_POINT('Ctrl Pts',(-39.568225357989,-5.68000001999998,
-130.673188209559));
#139213=CARTESIAN_POINT('Ctrl Pts',(-39.5925388156195,-5.68000001999998,
-130.806215404499));
#139214=CARTESIAN_POINT('Ctrl Pts',(-39.6220534778078,-5.68000001999998,
-130.937436349817));
#139215=CARTESIAN_POINT('Ctrl Pts',(-39.6907803864263,-5.68000001999998,
-131.242993291658));
#139216=CARTESIAN_POINT('Ctrl Pts',(-39.7874256609414,-5.68000001999998,
-131.540730203477));
#139217=CARTESIAN_POINT('Ctrl Pts',(-39.913239336921,-5.68000001999998,
-131.830296953197));
#139218=CARTESIAN_POINT('Ctrl Pts',(-39.9343840562227,-5.68000001999998,
-131.878962629596));
#139219=CARTESIAN_POINT('Ctrl Pts',(-39.9563527642831,-5.68000001999998,
-131.927397503975));
#139220=CARTESIAN_POINT('Ctrl Pts',(-39.9791515366304,-5.68000001999998,
-131.975599874271));
#139221=CARTESIAN_POINT('',(-39.5,-5.68000001999998,-102.218950121094));
#139222=CARTESIAN_POINT('',(-39.5,-5.68000001999998,-55.24995));
#139223=CARTESIAN_POINT('',(-39.9791515366304,-5.68000001999998,-100.083043097235));
#139224=CARTESIAN_POINT('Ctrl Pts',(-39.9791515366304,-5.68000001999998,
-100.083043097235));
#139225=CARTESIAN_POINT('Ctrl Pts',(-39.88674512358,-5.68000001999998,-100.278413622971));
#139226=CARTESIAN_POINT('Ctrl Pts',(-39.8073027352616,-5.68000001999998,
-100.479790373907));
#139227=CARTESIAN_POINT('Ctrl Pts',(-39.7413121766313,-5.68000001999998,
-100.684533556796));
#139228=CARTESIAN_POINT('Ctrl Pts',(-39.694147898587,-5.68000001999998,
-100.830866071718));
#139229=CARTESIAN_POINT('Ctrl Pts',(-39.6538540641004,-5.68000001999998,
-100.978917355179));
#139230=CARTESIAN_POINT('Ctrl Pts',(-39.620593360194,-5.68000001999998,
-101.127718496005));
#139231=CARTESIAN_POINT('Ctrl Pts',(-39.5515828956696,-5.68000001999998,
-101.436456274949));
#139232=CARTESIAN_POINT('Ctrl Pts',(-39.5117440272004,-5.68000001999998,
-101.750163184452));
#139233=CARTESIAN_POINT('Ctrl Pts',(-39.502232472568,-5.68000001999998,
-102.069036097455));
#139234=CARTESIAN_POINT('Ctrl Pts',(-39.5007456673965,-5.68000001999998,
-102.118880935069));
#139235=CARTESIAN_POINT('Ctrl Pts',(-39.5,-5.68000001999998,-102.16885201916));
#139236=CARTESIAN_POINT('Ctrl Pts',(-39.5,-5.68000001999998,-102.218950121094));
#139237=CARTESIAN_POINT('Ctrl Pts',(-58.3535376001277,-5.68000001999999,
-61.0621827299711));
#139238=CARTESIAN_POINT('Ctrl Pts',(-52.2440275184664,-5.68000001999999,
-74.0763270103718));
#139239=CARTESIAN_POINT('Ctrl Pts',(-46.1262203434603,-5.68000001999998,
-87.0865851147193));
#139240=CARTESIAN_POINT('Ctrl Pts',(-39.9791515366304,-5.68000001999998,
-100.083043097235));
#139241=CARTESIAN_POINT('Ctrl Pts',(-59.5,-5.68000001999999,-58.1246434856214));
#139242=CARTESIAN_POINT('Ctrl Pts',(-60.,-5.68000001999998,-58.1246434856214));
#139243=CARTESIAN_POINT('Ctrl Pts',(-60.,-5.18000001999999,-58.1246434856214));
#139244=CARTESIAN_POINT('Ctrl Pts',(-59.4999999932887,-5.68000001999999,
-57.8769929082306));
#139245=CARTESIAN_POINT('Ctrl Pts',(-60.0020017947382,-5.68000001999912,
-57.8269512006129));
#139246=CARTESIAN_POINT('Ctrl Pts',(-60.,-5.17800220042073,-57.8275435066813));
#139247=CARTESIAN_POINT('Ctrl Pts',(-59.4640366407682,-5.68000001999999,
-57.6353667913546));
#139248=CARTESIAN_POINT('Ctrl Pts',(-59.9606548869199,-5.68000002000021,
-57.5365322236183));
#139249=CARTESIAN_POINT('Ctrl Pts',(-59.9568439660775,-5.17605025203681,
-57.5376710843709));
#139250=CARTESIAN_POINT('Ctrl Pts',(-59.3571704209101,-5.68000001999999,
-57.2820131603569));
#139251=CARTESIAN_POINT('Ctrl Pts',(-59.8350835786331,-5.68000001999988,
-57.1113495469635));
#139252=CARTESIAN_POINT('Ctrl Pts',(-59.8286045065143,-5.17319230589712,
-57.1137623423983));
#139253=CARTESIAN_POINT('Ctrl Pts',(-59.3124762512969,-5.68000001999999,
-57.1660493315578));
#139254=CARTESIAN_POINT('Ctrl Pts',(-59.7822107642191,-5.68000001999999,
-56.971551755675));
#139255=CARTESIAN_POINT('Ctrl Pts',(-59.7749715022372,-5.17225378701852,
-56.9746437275083));
#139256=CARTESIAN_POINT('Ctrl Pts',(-59.2079771855437,-5.68000001999999,
-56.9447878986704));
#139257=CARTESIAN_POINT('Ctrl Pts',(-59.6581215271118,-5.68000001999999,
-56.7045411154571));
#139258=CARTESIAN_POINT('Ctrl Pts',(-59.6495726219715,-5.17046209438582,
-56.7092025345767));
#139259=CARTESIAN_POINT('Ctrl Pts',(-59.1479068869942,-5.68000001999999,
-56.8384914380986));
#139260=CARTESIAN_POINT('Ctrl Pts',(-59.5865663613646,-5.68000001999988,
-56.5761588403972));
#139261=CARTESIAN_POINT('Ctrl Pts',(-59.5774882635866,-5.16960084340769,
-56.5816816551612));
#139262=CARTESIAN_POINT('Ctrl Pts',(-59.0120618664304,-5.68000001999999,
-56.6346018834074));
#139263=CARTESIAN_POINT('Ctrl Pts',(-59.4243672282747,-5.6800000200001,
-56.3296643856923));
#139264=CARTESIAN_POINT('Ctrl Pts',(-59.4144742405229,-5.16794806289525,
-56.3370811282929));
#139265=CARTESIAN_POINT('Ctrl Pts',(-58.9355640571429,-5.68000001999999,
-56.5363163451986));
#139266=CARTESIAN_POINT('Ctrl Pts',(-59.332837232209,-5.68000002000004,
-56.210751177698));
#139267=CARTESIAN_POINT('Ctrl Pts',(-59.3226768695123,-5.16715091135939,
-56.219170776799));
#139268=CARTESIAN_POINT('Ctrl Pts',(-58.770777205737,-5.68000001999999,
-56.3541800398345));
#139269=CARTESIAN_POINT('Ctrl Pts',(-59.1353297626326,-5.68000001999993,
-55.9901841613723));
#139270=CARTESIAN_POINT('Ctrl Pts',(-59.1249326459437,-5.16567306852165,
-56.0006670964121));
#139271=CARTESIAN_POINT('Ctrl Pts',(-58.6823687426766,-5.68000001999999,
-56.2698716578318));
#139272=CARTESIAN_POINT('Ctrl Pts',(-59.0292080232237,-5.68000001999941,
-55.8880220414999));
#139273=CARTESIAN_POINT('Ctrl Pts',(-59.0188424909195,-5.16498867365063,
-55.8995247770565));
#139274=CARTESIAN_POINT('Ctrl Pts',(-58.3993671534221,-5.68000001999999,
-56.0369236173554));
#139275=CARTESIAN_POINT('Ctrl Pts',(-58.6888368836822,-5.68000002000116,
-55.6053191370779));
#139276=CARTESIAN_POINT('Ctrl Pts',(-58.6792405846915,-5.16309702763064,
-55.6200638122352));
#139277=CARTESIAN_POINT('Ctrl Pts',(-58.1837972805939,-5.68000001999999,
-55.907468794294));
#139278=CARTESIAN_POINT('Ctrl Pts',(-58.42924178916,-5.68000002000209,-55.448215858158));
#139279=CARTESIAN_POINT('Ctrl Pts',(-58.4205568275121,-5.16204487752377,
-55.4647607356853));
#139280=CARTESIAN_POINT('Ctrl Pts',(-57.9591100572707,-5.68000001999999,
-55.8140496618682));
#139281=CARTESIAN_POINT('Ctrl Pts',(-58.1583910096328,-5.68000001999999,
-55.3347486595489));
#139282=CARTESIAN_POINT('Ctrl Pts',(-58.1509320687249,-5.16128538415681,
-55.3526885469843));
#139283=CARTESIAN_POINT('',(-60.,-5.18000001999999,-58.1246434856214));
#139284=CARTESIAN_POINT('Ctrl Pts',(-58.1702690071152,-5.16134039100008,
-55.3608055405081));
#139285=CARTESIAN_POINT('Ctrl Pts',(-58.4329181295403,-5.16209542477378,
-55.4722107983731));
#139286=CARTESIAN_POINT('Ctrl Pts',(-58.6846580097054,-5.16312727866648,
-55.6245218487779));
#139287=CARTESIAN_POINT('Ctrl Pts',(-59.018842492426,-5.16498874849922,
-55.8995247753848));
#139288=CARTESIAN_POINT('Ctrl Pts',(-59.1249326474558,-5.1656731433235,
-56.0006670948875));
#139289=CARTESIAN_POINT('Ctrl Pts',(-59.3226768709922,-5.16715098605971,
-56.2191707755726));
#139290=CARTESIAN_POINT('Ctrl Pts',(-59.414474241965,-5.16794813754046,
-56.3370811272117));
#139291=CARTESIAN_POINT('Ctrl Pts',(-59.5774882649122,-5.16960091793786,
-56.5816816543548));
#139292=CARTESIAN_POINT('Ctrl Pts',(-59.6495726232209,-5.17046216885565,
-56.7092025338954));
#139293=CARTESIAN_POINT('Ctrl Pts',(-59.7749715032972,-5.17225386136191,
-56.9746437270556));
#139294=CARTESIAN_POINT('Ctrl Pts',(-59.8286045074639,-5.1731923801738,
-57.1137623420447));
#139295=CARTESIAN_POINT('Ctrl Pts',(-59.9568439666376,-5.17605032610843,
-57.5376710842035));
#139296=CARTESIAN_POINT('Ctrl Pts',(-60.0000000002948,-5.17800227435048,
-57.8275435065941));
#139297=CARTESIAN_POINT('Ctrl Pts',(-60.,-5.18000001999999,-58.1246434856214));
#139298=CARTESIAN_POINT('Origin',(-59.5,-5.18000001999999,-58.1246434856214));
#139299=CARTESIAN_POINT('Ctrl Pts',(-58.1516269266116,-5.16456703757977,
-55.3528444275805));
#139300=CARTESIAN_POINT('Ctrl Pts',(-60.,-5.19571559048276,-56.1206307397359));
#139301=CARTESIAN_POINT('Ctrl Pts',(-60.,-5.2768578914742,-58.1207219873789));
#139302=CARTESIAN_POINT('Ctrl Pts',(-58.1275061007746,-4.96483231244508,
-55.3509116092303));
#139303=CARTESIAN_POINT('Ctrl Pts',(-60.0000000000005,-4.99483472640263,
-56.1098379052425));
#139304=CARTESIAN_POINT('Ctrl Pts',(-60.,-5.07672217607537,-58.12884135333));
#139305=CARTESIAN_POINT('Ctrl Pts',(-58.1024667524284,-4.76557632116298,
-55.3488500157616));
#139306=CARTESIAN_POINT('Ctrl Pts',(-60.0000000000001,-4.79479350163006,
-56.0981738677439));
#139307=CARTESIAN_POINT('Ctrl Pts',(-60.,-4.87658373874773,-58.1368637570314));
#139308=CARTESIAN_POINT('Ctrl Pts',(-58.0765164643631,-4.56684999234778,
-55.3466493905885));
#139309=CARTESIAN_POINT('Ctrl Pts',(-60.,-4.59579029342123,-56.0855524411383));
#139310=CARTESIAN_POINT('Ctrl Pts',(-60.,-4.67644015442612,-58.1447026957153));
#139311=CARTESIAN_POINT('',(-60.,-4.68000002001403,-58.1445632485962));
#139312=CARTESIAN_POINT('Ctrl Pts',(-60.,-4.68000002001403,-58.1445632485962));
#139313=CARTESIAN_POINT('Ctrl Pts',(-60.,-4.67801447919764,-57.8400901274889));
#139314=CARTESIAN_POINT('Ctrl Pts',(-59.9547202743521,-4.67607375656258,
-57.5431941162335));
#139315=CARTESIAN_POINT('Ctrl Pts',(-59.819980312157,-4.67323178879642,
-57.1093239470213));
#139316=CARTESIAN_POINT('Ctrl Pts',(-59.7637842928231,-4.67230172637259,
-56.9674919122442));
#139317=CARTESIAN_POINT('Ctrl Pts',(-59.6323866477998,-4.67052667748359,
-56.6970587190125));
#139318=CARTESIAN_POINT('Ctrl Pts',(-59.5568525046157,-4.66967405412828,
-56.567291481448));
#139319=CARTESIAN_POINT('Ctrl Pts',(-59.385918342594,-4.66803974391678,
-56.318763868979));
#139320=CARTESIAN_POINT('Ctrl Pts',(-59.289776717509,-4.6672543224009,-56.1994379500303));
#139321=CARTESIAN_POINT('Ctrl Pts',(-59.0834337883813,-4.66580663221926,
-55.9796562580523));
#139322=CARTESIAN_POINT('Ctrl Pts',(-58.9727240508436,-4.66513801841297,
-55.8782346380825));
#139323=CARTESIAN_POINT('Ctrl Pts',(-58.6298042492702,-4.66335817424259,
-55.6084094028642));
#139324=CARTESIAN_POINT('Ctrl Pts',(-58.3750448694008,-4.66239047068315,
-55.4619202173471));
#139325=CARTESIAN_POINT('Ctrl Pts',(-58.1110275345658,-4.6616933513699,
-55.3564444847807));
#139326=CARTESIAN_POINT('Ctrl Pts',(-60.,-4.68000002001403,-58.1445632485962));
#139327=CARTESIAN_POINT('Ctrl Pts',(-60.,-4.84666977904325,-58.1380335512985));
#139328=CARTESIAN_POINT('Ctrl Pts',(-60.,-5.01333597711292,-58.1313769278999));
#139329=CARTESIAN_POINT('Ctrl Pts',(-60.,-5.18000001999999,-58.1246434856214));
#139330=CARTESIAN_POINT('Ctrl Pts',(-60.,-4.68000001999999,-58.1445632485961));
#139331=CARTESIAN_POINT('Ctrl Pts',(-59.9999999999999,-4.18000001999999,
-58.144563248596));
#139332=CARTESIAN_POINT('Ctrl Pts',(-59.5,-4.18000001999999,-58.1445632485962));
#139333=CARTESIAN_POINT('Ctrl Pts',(-60.,-4.67801447919764,-57.8400901274889));
#139334=CARTESIAN_POINT('Ctrl Pts',(-59.9980183704624,-4.18000001999736,
-57.8406912127677));
#139335=CARTESIAN_POINT('Ctrl Pts',(-59.4999999931196,-4.18000001999999,
-57.8907708245007));
#139336=CARTESIAN_POINT('Ctrl Pts',(-59.9547202743521,-4.67607375656258,
-57.5431941162335));
#139337=CARTESIAN_POINT('Ctrl Pts',(-59.9509926566885,-4.18000002000109,
-57.5443378186833));
#139338=CARTESIAN_POINT('Ctrl Pts',(-59.4622668978632,-4.18000001999999,
-57.6432940448109));
#139339=CARTESIAN_POINT('Ctrl Pts',(-59.819980312157,-4.67323178879642,
-57.1093239470213));
#139340=CARTESIAN_POINT('Ctrl Pts',(-59.8137304682065,-4.18000001999945,
-57.1117161950833));
#139341=CARTESIAN_POINT('Ctrl Pts',(-59.3499835921793,-4.18000001999999,
-57.2816425794726));
#139342=CARTESIAN_POINT('Ctrl Pts',(-59.7637842928231,-4.67230172637259,
-56.9674919122442));
#139343=CARTESIAN_POINT('Ctrl Pts',(-59.756837410337,-4.18000002,-56.9705421764153));
#139344=CARTESIAN_POINT('Ctrl Pts',(-59.3031535768727,-4.18000001999999,
-57.163418767372));
#139345=CARTESIAN_POINT('Ctrl Pts',(-59.6323866477998,-4.67052667748359,
-56.6970587190125));
#139346=CARTESIAN_POINT('Ctrl Pts',(-59.6242664035215,-4.18000001999999,
-56.7016181941089));
#139347=CARTESIAN_POINT('Ctrl Pts',(-59.1936555403131,-4.18000001999999,
-56.9379996304409));
#139348=CARTESIAN_POINT('Ctrl Pts',(-59.5568525046157,-4.66967405412828,
-56.567291481448));
#139349=CARTESIAN_POINT('Ctrl Pts',(-59.5482752170826,-4.18000001999972,
-56.5726707527956));
#139350=CARTESIAN_POINT('Ctrl Pts',(-59.130710421318,-4.18000001999999,
-56.8298323231333));
#139351=CARTESIAN_POINT('Ctrl Pts',(-59.385918342594,-4.66803974391678,
-56.318763868979));
#139352=CARTESIAN_POINT('Ctrl Pts',(-59.3766737402574,-4.18000002000027,
-56.3259306460082));
#139353=CARTESIAN_POINT('Ctrl Pts',(-58.9882652846901,-4.18000001999999,
-56.622672397275));
#139354=CARTESIAN_POINT('Ctrl Pts',(-59.289776717509,-4.6672543224009,-56.1994379500303));
#139355=CARTESIAN_POINT('Ctrl Pts',(-59.280338735327,-4.18000002000033,
-56.2075385111788));
#139356=CARTESIAN_POINT('Ctrl Pts',(-58.9081472639374,-4.18000001999999,
-56.5232083679403));
#139357=CARTESIAN_POINT('Ctrl Pts',(-59.0834337883813,-4.66580663221926,
-55.9796562580523));
#139358=CARTESIAN_POINT('Ctrl Pts',(-59.0738973083079,-4.18000001999967,
-55.9896554831564));
#139359=CARTESIAN_POINT('Ctrl Pts',(-58.7361948243045,-4.18000001999999,
-56.3400094513659));
#139360=CARTESIAN_POINT('Ctrl Pts',(-58.9727240508436,-4.66513801841297,
-55.8782346380825));
#139361=CARTESIAN_POINT('Ctrl Pts',(-58.9632803249174,-4.18000001999956,
-55.889161374227));
#139362=CARTESIAN_POINT('Ctrl Pts',(-58.6439367094154,-4.18000001999999,
-56.2554694851693));
#139363=CARTESIAN_POINT('Ctrl Pts',(-58.6181223301711,-4.66329754200289,
-55.5992175260631));
#139364=CARTESIAN_POINT('Ctrl Pts',(-58.6095926714098,-4.18000002000086,
-55.6130627249839));
#139365=CARTESIAN_POINT('Ctrl Pts',(-58.3484352743845,-4.18000001999999,
-56.0228947878735));
#139366=CARTESIAN_POINT('Ctrl Pts',(-58.3484766058291,-4.66229039631671,
-55.4467718445047));
#139367=CARTESIAN_POINT('Ctrl Pts',(-58.3409094947055,-4.18000001999966,
-55.4621795466313));
#139368=CARTESIAN_POINT('Ctrl Pts',(-58.1237304207495,-4.18000001999999,
-55.8958235878219));
#139369=CARTESIAN_POINT('Ctrl Pts',(-58.0697760887706,-4.66158691772347,
-55.3403413730918));
#139370=CARTESIAN_POINT('Ctrl Pts',(-58.0634433345606,-4.18000001999999,
-55.3569201007255));
#139371=CARTESIAN_POINT('Ctrl Pts',(-57.8914800739755,-4.18000001999999,
-55.8071084335971));
#139372=CARTESIAN_POINT('',(-59.5,-4.18000001999999,-58.1445632485962));
#139373=CARTESIAN_POINT('Ctrl Pts',(-58.1504944089168,-4.18000007585629,
-55.9233081330324));
#139374=CARTESIAN_POINT('Ctrl Pts',(-58.2011234110634,-4.1800000934009,
-55.9495719668715));
#139375=CARTESIAN_POINT('Ctrl Pts',(-58.2508802238442,-4.18000007907268,
-55.9776159745792));
#139376=CARTESIAN_POINT('Ctrl Pts',(-58.2996228616342,-4.18000005788132,
-56.007327702339));
#139377=CARTESIAN_POINT('Ctrl Pts',(-58.3611066386641,-4.18000003115063,
-56.0448059621867));
#139378=CARTESIAN_POINT('Ctrl Pts',(-58.4211714230485,-4.18000002563093,
-56.0849815311993));
#139379=CARTESIAN_POINT('Ctrl Pts',(-58.4791990630186,-4.18000002261545,
-56.1275622952346));
#139380=CARTESIAN_POINT('Ctrl Pts',(-58.5015978396008,-4.18000002145147,
-56.1439985490753));
#139381=CARTESIAN_POINT('Ctrl Pts',(-58.5236932870565,-4.18000002089499,
-56.1607926562338));
#139382=CARTESIAN_POINT('Ctrl Pts',(-58.5454508633043,-4.18000002055973,
-56.1779259948581));
#139383=CARTESIAN_POINT('Ctrl Pts',(-58.601384203271,-4.18000001969785,
-56.2219715651515));
#139384=CARTESIAN_POINT('Ctrl Pts',(-58.6553029072665,-4.18000001999999,
-56.2682684120419));
#139385=CARTESIAN_POINT('Ctrl Pts',(-58.7070968429494,-4.18000001999999,
-56.3167184080419));
#139386=CARTESIAN_POINT('Ctrl Pts',(-58.7466278917693,-4.18000001999999,
-56.3536972383227));
#139387=CARTESIAN_POINT('Ctrl Pts',(-58.7849870908598,-4.18000001999997,
-56.3919927767765));
#139388=CARTESIAN_POINT('Ctrl Pts',(-58.8221712586797,-4.18000002000008,
-56.4316087082659));
#139389=CARTESIAN_POINT('Ctrl Pts',(-58.9081478861484,-4.18000002000031,
-56.5232080201017));
#139390=CARTESIAN_POINT('Ctrl Pts',(-58.9882663096845,-4.18000002000183,
-56.6226714971191));
#139391=CARTESIAN_POINT('Ctrl Pts',(-59.059488987448,-4.18000002000189,
-56.7262515801497));
#139392=CARTESIAN_POINT('Ctrl Pts',(-59.0864350865984,-4.18000002000191,
-56.7654396488238));
#139393=CARTESIAN_POINT('Ctrl Pts',(-59.1121963184049,-4.18000002000164,
-56.8052844356691));
#139394=CARTESIAN_POINT('Ctrl Pts',(-59.1367770480425,-4.18000002000115,
-56.845783548759));
#139395=CARTESIAN_POINT('Ctrl Pts',(-59.1771662439534,-4.18000002000036,
-56.9123286284587));
#139396=CARTESIAN_POINT('Ctrl Pts',(-59.2143783070055,-4.1800000199807,
-56.9806361125577));
#139397=CARTESIAN_POINT('Ctrl Pts',(-59.2484246951019,-4.18000002050115,
-57.0506994175354));
#139398=CARTESIAN_POINT('Ctrl Pts',(-59.3031923634925,-4.18000002133835,
-57.1634045844535));
#139399=CARTESIAN_POINT('Ctrl Pts',(-59.3500454603234,-4.18000002397293,
-57.2816264448194));
#139400=CARTESIAN_POINT('Ctrl Pts',(-59.3874625053509,-4.18000002286791,
-57.4021771888577));
#139401=CARTESIAN_POINT('Ctrl Pts',(-59.3945407287637,-4.18000002265887,
-57.4249819052179));
#139402=CARTESIAN_POINT('Ctrl Pts',(-59.4012856253719,-4.18000002232778,
-57.4478436795316));
#139403=CARTESIAN_POINT('Ctrl Pts',(-59.4076964194497,-4.18000002192605,
-57.4707623700245));
#139404=CARTESIAN_POINT('Ctrl Pts',(-59.4578200392951,-4.18000001878511,
-57.6499551058506));
#139405=CARTESIAN_POINT('Ctrl Pts',(-59.4876405140701,-4.18000002000073,
-57.8326096057389));
#139406=CARTESIAN_POINT('Ctrl Pts',(-59.4968871656945,-4.18000002000007,
-58.0187658449342));
#139407=CARTESIAN_POINT('Ctrl Pts',(-59.4989612576684,-4.18000001999992,
-58.0605220586746));
#139408=CARTESIAN_POINT('Ctrl Pts',(-59.5,-4.18000001999999,-58.1024544069462));
#139409=CARTESIAN_POINT('Ctrl Pts',(-59.5,-4.18000001999999,-58.1445632485962));
#139410=CARTESIAN_POINT('Origin',(-59.5,-4.68000001999999,-58.1445632485962));
#139411=CARTESIAN_POINT('Ctrl Pts',(-57.5408897718184,-3.75014666797429,
-60.8901206419019));
#139412=CARTESIAN_POINT('Ctrl Pts',(-57.5947641336391,-4.18011275636206,
-60.9185429056887));
#139413=CARTESIAN_POINT('Ctrl Pts',(-57.9789048525842,-4.18000000314622,
-61.1211158812058));
#139414=CARTESIAN_POINT('Ctrl Pts',(-57.6237851397972,-3.75639532415342,
-60.7345335560658));
#139415=CARTESIAN_POINT('Ctrl Pts',(-57.68640755168,-4.1801105122733,-60.7564968901202));
#139416=CARTESIAN_POINT('Ctrl Pts',(-58.1017608867774,-4.18000000339119,
-60.8877040749259));
#139417=CARTESIAN_POINT('Ctrl Pts',(-57.6637036934156,-3.75937776709444,
-60.5618009361651));
#139418=CARTESIAN_POINT('Ctrl Pts',(-57.7319155584136,-4.18010945496984,
-60.5708624589659));
#139419=CARTESIAN_POINT('Ctrl Pts',(-58.1609260730227,-4.18000000350811,
-60.6285977191473));
#139420=CARTESIAN_POINT('Ctrl Pts',(-57.6557606890352,-3.75878386386294,
-60.3838931293299));
#139421=CARTESIAN_POINT('Ctrl Pts',(-57.7229085994607,-4.18010966305883,
-60.3808564105654));
#139422=CARTESIAN_POINT('Ctrl Pts',(-58.14915342597,-4.18000000348483,-60.3617046583731));
#139423=CARTESIAN_POINT('',(-58.0081705490647,-4.18000001999999,-61.0621827299711));
#139424=CARTESIAN_POINT('Origin',(-58.0081705490647,-3.68000001999999,-61.0621827299711));
#139425=CARTESIAN_POINT('Origin',(-56.7672600194274,-4.18000063577663,-60.4581517878592));
#139426=CARTESIAN_POINT('Origin',(83.2809572255632,-4.18000001999993,-55.24995));
#139427=CARTESIAN_POINT('',(-40.0271577790679,-4.18000001999998,-98.926539349744));
#139428=CARTESIAN_POINT('Ctrl Pts',(-40.0271577790679,-4.18000001999998,
-98.926539349744));
#139429=CARTESIAN_POINT('Ctrl Pts',(-46.0600710189762,-4.18000001999998,
-86.3237225210772));
#139430=CARTESIAN_POINT('Ctrl Pts',(-52.0416455898407,-4.18000001999999,
-73.6965260027483));
#139431=CARTESIAN_POINT('Ctrl Pts',(-58.0081705490647,-4.18000001999999,
-61.0621827299711));
#139432=CARTESIAN_POINT('',(-39.5,-4.18000001999998,-101.255910620448));
#139433=CARTESIAN_POINT('Ctrl Pts',(-39.5,-4.18000001999998,-101.255910620448));
#139434=CARTESIAN_POINT('Ctrl Pts',(-39.5,-4.18000001999998,-100.974485528874));
#139435=CARTESIAN_POINT('Ctrl Pts',(-39.5222808837211,-4.18000001999998,
-100.693150422383));
#139436=CARTESIAN_POINT('Ctrl Pts',(-39.5655905129044,-4.18000001999998,
-100.416810780316));
#139437=CARTESIAN_POINT('Ctrl Pts',(-39.5844991866037,-4.18000001999998,
-100.296162873128));
#139438=CARTESIAN_POINT('Ctrl Pts',(-39.6074169109197,-4.18000001999998,
-100.17646712623));
#139439=CARTESIAN_POINT('Ctrl Pts',(-39.6342425380314,-4.18000001999998,
-100.058132231812));
#139440=CARTESIAN_POINT('Ctrl Pts',(-39.705309269373,-4.18000001999998,
-99.7446381943797));
#139441=CARTESIAN_POINT('Ctrl Pts',(-39.8034555232829,-4.18000001999998,
-99.4388673313459));
#139442=CARTESIAN_POINT('Ctrl Pts',(-39.9301327648642,-4.18000001999998,
-99.1412335947868));
#139443=CARTESIAN_POINT('Ctrl Pts',(-39.9607955551634,-4.18000001999998,
-99.0691900237701));
#139444=CARTESIAN_POINT('Ctrl Pts',(-39.9931302150587,-4.18000001999999,
-98.997623275415));
#139445=CARTESIAN_POINT('Ctrl Pts',(-40.0271577790679,-4.18000001999999,
-98.926539349744));
#139446=CARTESIAN_POINT('',(-39.5,-4.18000001999998,-130.802732351058));
#139447=CARTESIAN_POINT('',(-39.5,-4.18000001999998,-55.24995));
#139448=CARTESIAN_POINT('',(-40.0271577790634,-4.18000001999998,-133.132103621752));
#139449=CARTESIAN_POINT('Ctrl Pts',(-40.0271577790634,-4.18000001999998,
-133.132103621752));
#139450=CARTESIAN_POINT('Ctrl Pts',(-39.9035045934269,-4.18000001999998,
-132.873790865235));
#139451=CARTESIAN_POINT('Ctrl Pts',(-39.8011022473414,-4.18000001999999,
-132.605500495508));
#139452=CARTESIAN_POINT('Ctrl Pts',(-39.7207150267769,-4.18000001999999,
-132.332596829933));
#139453=CARTESIAN_POINT('Ctrl Pts',(-39.6875913562998,-4.18000001999999,
-132.220146479902));
#139454=CARTESIAN_POINT('Ctrl Pts',(-39.658204991549,-4.18000001999999,
-132.106913147232));
#139455=CARTESIAN_POINT('Ctrl Pts',(-39.6326069664648,-4.18000001999999,
-131.993272849631));
#139456=CARTESIAN_POINT('Ctrl Pts',(-39.5604708508339,-4.18000001999999,
-131.673030580114));
#139457=CARTESIAN_POINT('Ctrl Pts',(-39.5173036683714,-4.18000001999998,
-131.347852435241));
#139458=CARTESIAN_POINT('Ctrl Pts',(-39.5042396692621,-4.18000001999998,
-131.017545146585));
#139459=CARTESIAN_POINT('Ctrl Pts',(-39.5014171427719,-4.18000001999998,
-130.946181005764));
#139460=CARTESIAN_POINT('Ctrl Pts',(-39.5,-4.18000001999998,-130.874577408243));
#139461=CARTESIAN_POINT('Ctrl Pts',(-39.5,-4.18000001999998,-130.802732351058));
#139462=CARTESIAN_POINT('',(-58.1221005562789,-4.18000001999999,-171.237717270032));
#139463=CARTESIAN_POINT('Ctrl Pts',(-58.1221005562789,-4.18000001999999,
-171.237717270032));
#139464=CARTESIAN_POINT('Ctrl Pts',(-52.1178384024439,-4.18000001999999,
-158.522841724749));
#139465=CARTESIAN_POINT('Ctrl Pts',(-46.0984712740486,-4.18000001999998,
-145.815138971718));
#139466=CARTESIAN_POINT('Ctrl Pts',(-40.0271577790634,-4.18000001999998,
-133.132103621752));
#139467=CARTESIAN_POINT('',(-58.2644174754153,-4.18000001999999,-171.871644662643));
#139468=CARTESIAN_POINT('Origin',(-56.1314697890424,-4.18000001999999,-172.0066931789));
#139469=CARTESIAN_POINT('',(-58.2644174754116,-4.18000003136422,-176.647241333317));
#139470=CARTESIAN_POINT('',(-58.2644174754153,-4.18000001999999,-171.871644662643));
#139471=CARTESIAN_POINT('',(-59.5,-4.18000001999999,-174.488343624884));
#139472=CARTESIAN_POINT('Ctrl Pts',(-59.5,-4.18000001999999,-174.488343624884));
#139473=CARTESIAN_POINT('Ctrl Pts',(-59.5,-4.18000001999999,-174.676432184924));
#139474=CARTESIAN_POINT('Ctrl Pts',(-59.4792627601893,-4.18000001935391,
-174.860994953506));
#139475=CARTESIAN_POINT('Ctrl Pts',(-59.4381337746335,-4.18000002064829,
-175.042081103098));
#139476=CARTESIAN_POINT('Ctrl Pts',(-59.431381263521,-4.18000002086079,
-175.071811625767));
#139477=CARTESIAN_POINT('Ctrl Pts',(-59.4240789892461,-4.18000002115769,
-175.101448468679));
#139478=CARTESIAN_POINT('Ctrl Pts',(-59.4162283471532,-4.18000002161129,
-175.130991885445));
#139479=CARTESIAN_POINT('Ctrl Pts',(-59.4092933860371,-4.18000002201199,
-175.157089425504));
#139480=CARTESIAN_POINT('Ctrl Pts',(-59.4019280344311,-4.18000002232545,
-175.183113688583));
#139481=CARTESIAN_POINT('Ctrl Pts',(-59.3941336392735,-4.18000002248887,
-175.209064512545));
#139482=CARTESIAN_POINT('Ctrl Pts',(-59.3589528015432,-4.18000002322649,
-175.326196337184));
#139483=CARTESIAN_POINT('Ctrl Pts',(-59.3147522563139,-4.18000002089879,
-175.441619139941));
#139484=CARTESIAN_POINT('Ctrl Pts',(-59.2630854722639,-4.18000002030225,
-175.551758766342));
#139485=CARTESIAN_POINT('Ctrl Pts',(-59.2343127518865,-4.18000001997004,
-175.613094433564));
#139486=CARTESIAN_POINT('Ctrl Pts',(-59.2031440665131,-4.18000001999999,
-175.673101168879));
#139487=CARTESIAN_POINT('Ctrl Pts',(-59.1695814056726,-4.18000001999999,
-175.731779921994));
#139488=CARTESIAN_POINT('Ctrl Pts',(-59.1428767576963,-4.18000001999999,
-175.778468575586));
#139489=CARTESIAN_POINT('Ctrl Pts',(-59.1146521957298,-4.18000001999991,
-175.824314777934));
#139490=CARTESIAN_POINT('Ctrl Pts',(-59.0849057084902,-4.18000002000059,
-175.869317498238));
#139491=CARTESIAN_POINT('Ctrl Pts',(-59.0177729179323,-4.18000002000213,
-175.970881026476));
#139492=CARTESIAN_POINT('Ctrl Pts',(-58.9421638152095,-4.18000002001086,
-176.068866658213));
#139493=CARTESIAN_POINT('Ctrl Pts',(-58.8606254499681,-4.18000002000853,
-176.15981892266));
#139494=CARTESIAN_POINT('Ctrl Pts',(-58.8332817762446,-4.18000002000775,
-176.190319522422));
#139495=CARTESIAN_POINT('Ctrl Pts',(-58.8052684934467,-4.18000002000547,
-176.220067577769));
#139496=CARTESIAN_POINT('Ctrl Pts',(-58.7765893403539,-4.18000002000312,
-176.2490672712));
#139497=CARTESIAN_POINT('Ctrl Pts',(-58.7334919025214,-4.18000001999957,
-176.292646399243));
#139498=CARTESIAN_POINT('Ctrl Pts',(-58.6887854216316,-4.1800000198565,
-176.334637716938));
#139499=CARTESIAN_POINT('Ctrl Pts',(-58.6426104314479,-4.18000002015176,
-176.374934331063));
#139500=CARTESIAN_POINT('Ctrl Pts',(-58.6279756118792,-4.18000002024535,
-176.387706043078));
#139501=CARTESIAN_POINT('Ctrl Pts',(-58.6131935185628,-4.18000002040339,
-176.400307828981));
#139502=CARTESIAN_POINT('Ctrl Pts',(-58.5982692931781,-4.18000002077447,
-176.412737145101));
#139503=CARTESIAN_POINT('Ctrl Pts',(-58.5771929061033,-4.18000002129852,
-176.430290155116));
#139504=CARTESIAN_POINT('Ctrl Pts',(-58.5557921166901,-4.18000002220248,
-176.447510765875));
#139505=CARTESIAN_POINT('Ctrl Pts',(-58.5341058949341,-4.18000002446768,
-176.464377473526));
#139506=CARTESIAN_POINT('Ctrl Pts',(-58.4881980669411,-4.18000002926289,
-176.500082813181));
#139507=CARTESIAN_POINT('Ctrl Pts',(-58.4409815652462,-4.18000004169373,
-176.534222750276));
#139508=CARTESIAN_POINT('Ctrl Pts',(-58.3925215548524,-4.18000005349381,
-176.566751049323));
#139509=CARTESIAN_POINT('Ctrl Pts',(-58.3507358574755,-4.18000006366869,
-176.59479928227));
#139510=CARTESIAN_POINT('Ctrl Pts',(-58.3080246526018,-4.18000007127262,
-176.621648795663));
#139511=CARTESIAN_POINT('Ctrl Pts',(-58.2644174754055,-4.18000006545692,
-176.647241333307));
#139512=CARTESIAN_POINT('',(-59.5,-4.18000001999999,-174.466077711105));
#139513=CARTESIAN_POINT('Origin',(0.,-12.9675000200281,-60.64995));
#139514=CARTESIAN_POINT('',(-39.585730865575,-3.78242429077387,-98.7152302188469));
#139515=CARTESIAN_POINT('',(-39.7525219239569,1.81208306810639,-94.9115092130908));
#139516=CARTESIAN_POINT('Ctrl Pts',(-39.585730865631,-3.78242429107081,
-98.7152302188737));
#139517=CARTESIAN_POINT('Ctrl Pts',(-39.5925554021339,-3.50286551329097,
-98.5654740436898));
#139518=CARTESIAN_POINT('Ctrl Pts',(-39.5995949827268,-3.22506435949984,
-98.4103062973797));
#139519=CARTESIAN_POINT('Ctrl Pts',(-39.6215565252267,-2.38668519024414,
-97.9237506811802));
#139520=CARTESIAN_POINT('Ctrl Pts',(-39.6371406048982,-1.82970860306462,
-97.5751506494424));
#139521=CARTESIAN_POINT('Ctrl Pts',(-39.6847862724127,-0.212218467036257,
-96.496949566391));
#139522=CARTESIAN_POINT('Ctrl Pts',(-39.7182100340316,0.816234902512257,
-95.7247235977679));
#139523=CARTESIAN_POINT('Ctrl Pts',(-39.7525219240432,1.8120830678168,-94.9115092131337));
#139524=CARTESIAN_POINT('Ctrl Pts',(-57.5607154366947,-3.75164060643487,
-60.8508735991007));
#139525=CARTESIAN_POINT('Ctrl Pts',(-51.5953561753878,-3.75882514278712,
-73.4851842515103));
#139526=CARTESIAN_POINT('Ctrl Pts',(-45.6152480050635,-3.76777552135149,
-86.1124074293824));
#139527=CARTESIAN_POINT('Ctrl Pts',(-39.585730865631,-3.78242429107081,
-98.7152302188737));
#139528=CARTESIAN_POINT('Ctrl Pts',(-39.7525219240432,1.8120830678168,-94.9115092131337));
#139529=CARTESIAN_POINT('Ctrl Pts',(-42.5630938966427,1.82180095215014,
-89.2547782578028));
#139530=CARTESIAN_POINT('Ctrl Pts',(-45.3466144966382,1.82978958392238,
-83.5843555039947));
#139531=CARTESIAN_POINT('Ctrl Pts',(-50.8828928487858,1.84368306852047,
-72.2280037103762));
#139532=CARTESIAN_POINT('Ctrl Pts',(-53.6353179962474,1.84957228639408,
-66.5419044818115));
#139533=CARTESIAN_POINT('Ctrl Pts',(-56.377904566775,1.85477723331148,-60.8508735991007));
#139534=CARTESIAN_POINT('Ctrl Pts',(-56.4768060379592,1.84328648456651,
-60.3843526253219));
#139535=CARTESIAN_POINT('Ctrl Pts',(-56.3127916612335,2.47013219497058,
-60.3918959659146));
#139536=CARTESIAN_POINT('Ctrl Pts',(-56.9600934028813,2.46999996959074,
-60.3623927486908));
#139537=CARTESIAN_POINT('Ctrl Pts',(-56.4849292473983,1.84234741764349,
-60.5602093497011));
#139538=CARTESIAN_POINT('Ctrl Pts',(-56.3176950849992,2.47013256123686,
-60.5376645429823));
#139539=CARTESIAN_POINT('Ctrl Pts',(-56.9719086646404,2.46999996957514,
-60.6262162467223));
#139540=CARTESIAN_POINT('Ctrl Pts',(-56.4442115172646,1.84705094373349,
-60.7334982606779));
#139541=CARTESIAN_POINT('Ctrl Pts',(-56.2937114156122,2.47013073129433,
-60.6793039133547));
#139542=CARTESIAN_POINT('Ctrl Pts',(-56.9126832861354,2.46999996965326,
-60.8861329835762));
#139543=CARTESIAN_POINT('Ctrl Pts',(-56.3570930423877,1.85720121361396,
-60.8904421107847));
#139544=CARTESIAN_POINT('Ctrl Pts',(-56.232192761867,2.4701269151012,-60.8230951160809));
#139545=CARTESIAN_POINT('Ctrl Pts',(-56.7859903733787,2.46999996982182,
-61.1215882796171));
#139546=CARTESIAN_POINT('',(-56.8161649572467,2.46999998000001,-61.0621827299711));
#139547=CARTESIAN_POINT('Origin',(-55.5227769329964,2.47000037335106,-60.4517448637277));
#139548=CARTESIAN_POINT('Origin',(-56.8161649572467,1.96999998000001,-61.0621827299711));
#139549=CARTESIAN_POINT('Origin',(83.2809572255632,2.46999998000007,-55.24995));
#139550=CARTESIAN_POINT('',(-57.,2.46999998000001,-55.74995));
#139551=CARTESIAN_POINT('',(83.2809572255632,2.46999998000007,-55.74995));
#139552=CARTESIAN_POINT('',(-59.5,2.46999998000001,-58.24995));
#139553=CARTESIAN_POINT('Origin',(-57.,2.46999998000001,-58.24995));
#139554=CARTESIAN_POINT('',(-59.5,2.46999998000001,-174.34995));
#139555=CARTESIAN_POINT('',(-59.5,2.46999998000001,-58.24995));
#139556=CARTESIAN_POINT('',(-57.077763566464,2.46999998000001,-176.848740272858));
#139557=CARTESIAN_POINT('Origin',(-57.,2.46999998000001,-174.34995));
#139558=CARTESIAN_POINT('',(-57.077763566464,2.46999998000001,-171.871644662643));
#139559=CARTESIAN_POINT('',(-57.077763566464,2.46999998000001,-176.84995));
#139560=CARTESIAN_POINT('',(-56.9324803875071,2.46999998000001,-171.237717270032));
#139561=CARTESIAN_POINT('Origin',(-55.639113972473,2.47000037313163,-171.847693895992));
#139562=CARTESIAN_POINT('',(-40.1772697316389,2.46999998000002,-136.935824627502));
#139563=CARTESIAN_POINT('Ctrl Pts',(-40.1772697316389,2.46999998000002,
-136.935824627502));
#139564=CARTESIAN_POINT('Ctrl Pts',(-43.0113367121144,2.46999998000002,
-142.632519945825));
#139565=CARTESIAN_POINT('Ctrl Pts',(-45.8169723643453,2.46999998000002,
-148.343102920405));
#139566=CARTESIAN_POINT('Ctrl Pts',(-48.6065865655743,2.46999998000001,
-154.061511783466));
#139567=CARTESIAN_POINT('Ctrl Pts',(-51.3962007668033,2.46999998000001,
-159.779920646528));
#139568=CARTESIAN_POINT('Ctrl Pts',(-54.1694328122146,2.46999998000001,
-165.506331589084));
#139569=CARTESIAN_POINT('Ctrl Pts',(-56.9324803874897,2.46999998000001,
-171.23771727004));
#139570=CARTESIAN_POINT('',(-39.5,2.46999998000002,-134.012863078852));
#139571=CARTESIAN_POINT('Ctrl Pts',(-39.5,2.46999998000002,-134.012863078852));
#139572=CARTESIAN_POINT('Ctrl Pts',(-39.5,2.46999998000002,-134.194202123598));
#139573=CARTESIAN_POINT('Ctrl Pts',(-39.5074991738613,2.46999998000002,
-134.375559257497));
#139574=CARTESIAN_POINT('Ctrl Pts',(-39.5222608830472,2.46999998000002,
-134.556078177935));
#139575=CARTESIAN_POINT('Ctrl Pts',(-39.5372803972933,2.46999998000002,
-134.739749761156));
#139576=CARTESIAN_POINT('Ctrl Pts',(-39.5598184209784,2.46999998000002,
-134.922554775989));
#139577=CARTESIAN_POINT('Ctrl Pts',(-39.5896791401062,2.46999998000002,
-135.103595442119));
#139578=CARTESIAN_POINT('Ctrl Pts',(-39.6126641240195,2.46999998000002,
-135.242949647918));
#139579=CARTESIAN_POINT('Ctrl Pts',(-39.6399889131325,2.46999998000002,
-135.381258722716));
#139580=CARTESIAN_POINT('Ctrl Pts',(-39.671584618531,2.46999998000002,-135.518108079287));
#139581=CARTESIAN_POINT('Ctrl Pts',(-39.7480265101501,2.46999998000002,
-135.849198129379));
#139582=CARTESIAN_POINT('Ctrl Pts',(-39.8488754308751,2.46999998000002,
-136.172910839316));
#139583=CARTESIAN_POINT('Ctrl Pts',(-39.976224515067,2.46999998000002,-136.488613556871));
#139584=CARTESIAN_POINT('Ctrl Pts',(-40.0371049338932,2.46999998000002,
-136.639538188887));
#139585=CARTESIAN_POINT('Ctrl Pts',(-40.1040424074824,2.46999998000002,
-136.788632003769));
#139586=CARTESIAN_POINT('Ctrl Pts',(-40.1772697316389,2.46999998000002,
-136.935824627502));
#139587=CARTESIAN_POINT('',(-39.5,2.46999998000002,-98.0457798926543));
#139588=CARTESIAN_POINT('',(-39.5,2.46999998000002,-55.24995));
#139589=CARTESIAN_POINT('',(-40.177269731639,2.46999998000002,-95.1228183440042));
#139590=CARTESIAN_POINT('Ctrl Pts',(-40.1772697316388,2.46999998000002,
-95.1228183440041));
#139591=CARTESIAN_POINT('Ctrl Pts',(-40.0557143101432,2.46999998000002,
-95.367154206676));
#139592=CARTESIAN_POINT('Ctrl Pts',(-39.9506490904769,2.46999998000002,
-95.6194942161999));
#139593=CARTESIAN_POINT('Ctrl Pts',(-39.862036785698,2.46999998000002,-95.876484568063));
#139594=CARTESIAN_POINT('Ctrl Pts',(-39.785571796048,2.46999998000002,-96.0982456953059));
#139595=CARTESIAN_POINT('Ctrl Pts',(-39.721358807228,2.46999998000002,-96.3234708895919));
#139596=CARTESIAN_POINT('Ctrl Pts',(-39.6694028678065,2.46999998000002,
-96.5500162443606));
#139597=CARTESIAN_POINT('Ctrl Pts',(-39.5883957972392,2.46999998000002,
-96.9032342930522));
#139598=CARTESIAN_POINT('Ctrl Pts',(-39.5360425809491,2.46999998000002,
-97.2613436845053));
#139599=CARTESIAN_POINT('Ctrl Pts',(-39.5132030141796,2.46999998000002,
-97.6244912071908));
#139600=CARTESIAN_POINT('Ctrl Pts',(-39.5044179952616,2.46999998000002,
-97.7641723968128));
#139601=CARTESIAN_POINT('Ctrl Pts',(-39.5,2.46999998000002,-97.9045990595778));
#139602=CARTESIAN_POINT('Ctrl Pts',(-39.5,2.46999998000002,-98.0457798926543));
#139603=CARTESIAN_POINT('Ctrl Pts',(-56.8161649572467,2.46999998000001,
-61.0621827299711));
#139604=CARTESIAN_POINT('Ctrl Pts',(-54.0722086604215,2.46999998000001,
-66.7532163030615));
#139605=CARTESIAN_POINT('Ctrl Pts',(-51.3181460106093,2.46999998000001,
-72.4393128412015));
#139606=CARTESIAN_POINT('Ctrl Pts',(-48.5478694191173,2.46999998000001,
-78.1174887380514));
#139607=CARTESIAN_POINT('Ctrl Pts',(-45.7775928276252,2.46999998000002,
-83.7956646349013));
#139608=CARTESIAN_POINT('Ctrl Pts',(-42.9914528488282,2.46999998000002,
-89.4660911391003));
#139609=CARTESIAN_POINT('Ctrl Pts',(-40.1772697316389,2.46999998000002,
-95.1228183440041));
#139610=CARTESIAN_POINT('Origin',(-60.,2.96999998000001,-55.74995));
#139611=CARTESIAN_POINT('',(-57.,2.96999998000001,-55.24995));
#139612=CARTESIAN_POINT('',(-60.,2.96999998000001,-55.24995));
#139613=CARTESIAN_POINT('Origin',(-57.,2.96999998000001,-55.74995));
#139614=CARTESIAN_POINT('Origin',(-60.,28.41999998,-55.24995));
#139615=CARTESIAN_POINT('',(-57.,3.46999998000001,-55.24995));
#139616=CARTESIAN_POINT('',(-60.,3.46999998000001,-55.24995));
#139617=CARTESIAN_POINT('',(-57.,28.41999998,-55.24995));
#139618=CARTESIAN_POINT('Origin',(83.2809572255632,3.46999998000007,-55.74995));
#139619=CARTESIAN_POINT('',(-57.,3.96999998000001,-55.74995));
#139620=CARTESIAN_POINT('',(83.2809572255632,3.96999998000007,-55.74995));
#139621=CARTESIAN_POINT('Origin',(-57.,3.46999998000001,-55.74995));
#139622=CARTESIAN_POINT('Ctrl Pts',(-55.6456300835169,4.33828227850038,
-60.8898982295148));
#139623=CARTESIAN_POINT('Ctrl Pts',(-55.7339281824781,3.96993431898625,
-60.9380383069126));
#139624=CARTESIAN_POINT('Ctrl Pts',(-56.0692321081993,3.96999998739438,
-61.1207654305588));
#139625=CARTESIAN_POINT('Ctrl Pts',(-55.7334016533014,4.32662458144452,
-60.7353258635364));
#139626=CARTESIAN_POINT('Ctrl Pts',(-55.8351750163154,3.96993697857447,
-60.7722679906112));
#139627=CARTESIAN_POINT('Ctrl Pts',(-56.1954681966718,3.96999998716033,
-60.8888693966731));
#139628=CARTESIAN_POINT('Ctrl Pts',(-55.7764277962604,4.32095586851412,
-60.5620589091497));
#139629=CARTESIAN_POINT('Ctrl Pts',(-55.8870156345094,3.96993824711686,
-60.5772788420628));
#139630=CARTESIAN_POINT('Ctrl Pts',(-56.2573698974905,3.96999998704652,
-60.6289874486285));
#139631=CARTESIAN_POINT('Ctrl Pts',(-55.7678794768586,4.32208288640323,
-60.3838032961762));
#139632=CARTESIAN_POINT('Ctrl Pts',(-55.8768003135833,3.96993799744087,
-60.3787010736661));
#139633=CARTESIAN_POINT('Ctrl Pts',(-56.2450717652166,3.96999998706915,
-60.3615697395426));
#139634=CARTESIAN_POINT('',(-56.0993680931338,3.96999998000001,-61.0621827299711));
#139635=CARTESIAN_POINT('Origin',(-56.0993680931338,4.46999998000001,-61.0621827299711));
#139636=CARTESIAN_POINT('Origin',(-54.7700863539085,3.96999970901095,-60.4480774066313));
#139637=CARTESIAN_POINT('Origin',(83.2809572255632,3.96999998000007,-55.24995));
#139638=CARTESIAN_POINT('',(-40.2576018765703,3.96999998000001,-92.9619213022396));
#139639=CARTESIAN_POINT('Ctrl Pts',(-40.2576018765703,3.96999998000001,
-92.9619213022396));
#139640=CARTESIAN_POINT('Ctrl Pts',(-42.9469753996782,3.96999998000001,
-87.669671462365));
#139641=CARTESIAN_POINT('Ctrl Pts',(-45.6032617662994,3.96999998000001,
-82.3609901712845));
#139642=CARTESIAN_POINT('Ctrl Pts',(-48.2402535232915,3.96999998000001,
-77.0427269617097));
#139643=CARTESIAN_POINT('Ctrl Pts',(-50.8772452802836,3.96999998000001,
-71.724463752135));
#139644=CARTESIAN_POINT('Ctrl Pts',(-53.4945730592583,3.96999998000001,
-66.3964351916018));
#139645=CARTESIAN_POINT('Ctrl Pts',(-56.0993680931338,3.96999998000001,
-61.0621827299711));
#139646=CARTESIAN_POINT('',(-39.5,3.96999998000002,-96.1952589849652));
#139647=CARTESIAN_POINT('Ctrl Pts',(-39.5,3.96999998000002,-96.1952589849652));
#139648=CARTESIAN_POINT('Ctrl Pts',(-39.5,3.96999998000001,-95.9142103380175));
#139649=CARTESIAN_POINT('Ctrl Pts',(-39.5161227273835,3.96999998000002,
-95.6343109988079));
#139650=CARTESIAN_POINT('Ctrl Pts',(-39.5801128567305,3.96999998000002,
-95.0767752377766));
#139651=CARTESIAN_POINT('Ctrl Pts',(-39.6280462441481,3.96999998000002,
-94.7999095964395));
#139652=CARTESIAN_POINT('Ctrl Pts',(-39.81711425019,3.96999998000002,-93.9870091546851));
#139653=CARTESIAN_POINT('Ctrl Pts',(-40.0026450649981,3.96999998000001,
-93.4636348550876));
#139654=CARTESIAN_POINT('Ctrl Pts',(-40.2576018765703,3.96999998000001,
-92.9619213022396));
#139655=CARTESIAN_POINT('',(-39.5,3.96999998000002,-135.863383986541));
#139656=CARTESIAN_POINT('',(-39.5,3.96999998000002,-55.24995));
#139657=CARTESIAN_POINT('',(-40.2576018765703,3.96999998000001,-139.096721669266));
#139658=CARTESIAN_POINT('Ctrl Pts',(-40.2576018765703,3.96999998000001,
-139.096721669266));
#139659=CARTESIAN_POINT('Ctrl Pts',(-40.1422232489776,3.96999998000001,
-138.869675289076));
#139660=CARTESIAN_POINT('Ctrl Pts',(-40.0403932052765,3.96999998000002,
-138.635953665709));
#139661=CARTESIAN_POINT('Ctrl Pts',(-39.9518763029248,3.96999998000002,
-138.39795690135));
#139662=CARTESIAN_POINT('Ctrl Pts',(-39.8589569884594,3.96999998000002,
-138.148123303454));
#139663=CARTESIAN_POINT('Ctrl Pts',(-39.7807077156224,3.96999998000002,
-137.893577344799));
#139664=CARTESIAN_POINT('Ctrl Pts',(-39.716907177829,3.96999998000002,-137.637072537678));
#139665=CARTESIAN_POINT('Ctrl Pts',(-39.7071356404147,3.96999998000002,
-137.597786876358));
#139666=CARTESIAN_POINT('Ctrl Pts',(-39.6977031285481,3.96999998000002,
-137.55845524907));
#139667=CARTESIAN_POINT('Ctrl Pts',(-39.6886089528968,3.96999998000002,
-137.519087538285));
#139668=CARTESIAN_POINT('Ctrl Pts',(-39.6032792176026,3.96999998000002,
-137.149704268237));
#139669=CARTESIAN_POINT('Ctrl Pts',(-39.5465796834614,3.96999998000002,
-136.775425176638));
#139670=CARTESIAN_POINT('Ctrl Pts',(-39.5191682987985,3.96999998000002,
-136.396137730949));
#139671=CARTESIAN_POINT('Ctrl Pts',(-39.5064128043265,3.96999998000002,
-136.219641761254));
#139672=CARTESIAN_POINT('Ctrl Pts',(-39.5000000000002,3.96999998000002,
-136.042061173864));
#139673=CARTESIAN_POINT('Ctrl Pts',(-39.5,3.96999998000002,-135.863383986541));
#139674=CARTESIAN_POINT('',(-56.217166622605,3.96999998000001,-171.237717270032));
#139675=CARTESIAN_POINT('Ctrl Pts',(-56.217166622605,3.96999998000001,-171.237717270032));
#139676=CARTESIAN_POINT('Ctrl Pts',(-53.5931275135095,3.96999998000001,
-165.863064362473));
#139677=CARTESIAN_POINT('Ctrl Pts',(-50.9564483006798,3.96999998000001,
-160.49468788009));
#139678=CARTESIAN_POINT('Ctrl Pts',(-48.2998833897147,3.96999998000001,
-155.136185612272));
#139679=CARTESIAN_POINT('Ctrl Pts',(-45.6433184787496,3.96999998000001,
-149.777683344454));
#139680=CARTESIAN_POINT('Ctrl Pts',(-42.9672487496428,3.96999998000001,
-144.428866165794));
#139681=CARTESIAN_POINT('Ctrl Pts',(-40.2576018765703,3.96999998000001,
-139.096721669266));
#139682=CARTESIAN_POINT('',(-56.3642936064049,3.96999998000001,-171.871644662643));
#139683=CARTESIAN_POINT('Origin',(-54.8887873789865,3.96999970486963,-171.85218621454));
#139684=CARTESIAN_POINT('',(-56.3642936064049,3.96999998000001,-176.84995));
#139685=CARTESIAN_POINT('',(-56.3642936064049,3.96999998000001,-171.871644662643));
#139686=CARTESIAN_POINT('',(-57.,3.96999998000001,-176.84995));
#139687=CARTESIAN_POINT('',(83.2809572255632,3.96999998000007,-176.84995));
#139688=CARTESIAN_POINT('',(-59.5,3.96999998000001,-174.34995));
#139689=CARTESIAN_POINT('Origin',(-57.,3.96999998000001,-174.34995));
#139690=CARTESIAN_POINT('',(-59.5,3.96999998000001,-58.24995));
#139691=CARTESIAN_POINT('',(-59.5,3.96999998000001,-174.34995));
#139692=CARTESIAN_POINT('Origin',(-57.,3.96999998000001,-58.24995));
#139693=CARTESIAN_POINT('Origin',(0.,-12.9675000200281,-60.64995));
#139694=CARTESIAN_POINT('',(-39.8417798628559,4.28988750369335,-92.7506121713693));
#139695=CARTESIAN_POINT('',(-40.0642139580843,9.89540189669765,-86.9391114694665));
#139696=CARTESIAN_POINT('Ctrl Pts',(-39.8417723428251,4.289984134881,-92.7507162230213));
#139697=CARTESIAN_POINT('Ctrl Pts',(-39.8692662103635,5.02430264837445,
-92.0707528204852));
#139698=CARTESIAN_POINT('Ctrl Pts',(-39.8971213137832,5.74554162158512,
-91.3685155609789));
#139699=CARTESIAN_POINT('Ctrl Pts',(-39.9251065221777,6.45615586467189,
-90.6478697442548));
#139700=CARTESIAN_POINT('Ctrl Pts',(-39.9717823825843,7.64137238140021,
-89.4459218055498));
#139701=CARTESIAN_POINT('Ctrl Pts',(-40.0183482409369,8.78465889880687,
-88.2051541708012));
#139702=CARTESIAN_POINT('Ctrl Pts',(-40.0642139729082,9.89540198625494,
-86.9391115876706));
#139703=CARTESIAN_POINT('Ctrl Pts',(-55.6666368275827,4.33549309160633,
-60.8508735991007));
#139704=CARTESIAN_POINT('Ctrl Pts',(-53.0636135602343,4.32979793687723,
-66.1851229317376));
#139705=CARTESIAN_POINT('Ctrl Pts',(-50.4483866480001,4.32340038871991,
-71.5131546215955));
#139706=CARTESIAN_POINT('Ctrl Pts',(-45.179787381339,4.30850505134695,-82.1496810408829));
#139707=CARTESIAN_POINT('Ctrl Pts',(-42.5267665530282,4.30001892806028,
-87.4583592350843));
#139708=CARTESIAN_POINT('Ctrl Pts',(-39.8417798628559,4.28988750369335,
-92.7506121713693));
#139709=CARTESIAN_POINT('Ctrl Pts',(-40.064213984323,9.89540181527278,-86.9391114268059));
#139710=CARTESIAN_POINT('Ctrl Pts',(-42.3769453355832,9.90511004939769,
-82.6211625585897));
#139711=CARTESIAN_POINT('Ctrl Pts',(-44.6533124708726,9.91361722903472,
-78.283718841389));
#139712=CARTESIAN_POINT('Ctrl Pts',(-49.1597584393762,9.92893028193935,
-69.5840753777615));
#139713=CARTESIAN_POINT('Ctrl Pts',(-51.3895604060249,9.93573233905146,
-65.2217230121251));
#139714=CARTESIAN_POINT('Ctrl Pts',(-53.6034226162473,9.94191093135268,
-60.8508735991007));
#139715=CARTESIAN_POINT('Ctrl Pts',(-53.7125918503832,9.92402752715881,
-60.40351858218));
#139716=CARTESIAN_POINT('Ctrl Pts',(-53.4161966316591,10.6200463510678,
-60.411613444258));
#139717=CARTESIAN_POINT('Ctrl Pts',(-54.1724511599881,10.6199999790608,
-60.3911473089805));
#139718=CARTESIAN_POINT('Ctrl Pts',(-53.7172936685689,9.92326040045936,
-60.5668141071178));
#139719=CARTESIAN_POINT('Ctrl Pts',(-53.4174513698505,10.620046463598,-60.5214955398562));
#139720=CARTESIAN_POINT('Ctrl Pts',(-54.1790134480646,10.6199999790597,
-60.6361119980643));
#139721=CARTESIAN_POINT('Ctrl Pts',(-53.6753724344268,9.93009784663695,
-60.7276561184828));
#139722=CARTESIAN_POINT('Ctrl Pts',(-53.4068684094031,10.6200454844905,
-60.6288932216019));
#139723=CARTESIAN_POINT('Ctrl Pts',(-54.1205022571196,10.6199999790689,
-60.8773492053566));
#139724=CARTESIAN_POINT('Ctrl Pts',(-53.5909494181271,9.94395845212128,
-60.8730306626157));
#139725=CARTESIAN_POINT('Ctrl Pts',(-53.3671997002977,10.6200436156875,
-60.752177389371));
#139726=CARTESIAN_POINT('Ctrl Pts',(-54.0027434996135,10.6199999790877,
-61.095435351044));
#139727=CARTESIAN_POINT('',(-54.0201152391274,10.61999998,-61.0621827299711));
#139728=CARTESIAN_POINT('Origin',(-52.5839997447372,10.6200000169309,-60.4356500018395));
#139729=CARTESIAN_POINT('Origin',(-54.0201152391274,10.11999998,-61.0621827299711));
#139730=CARTESIAN_POINT('Origin',(83.2809572255632,10.6199999800001,-55.24995));
#139731=CARTESIAN_POINT('',(-54.1424378198232,10.61999998,-171.237717270032));
#139732=CARTESIAN_POINT('',(-54.2951871140408,10.61999998,-171.871644662643));
#139733=CARTESIAN_POINT('Origin',(-52.7058336009045,10.6200000150414,-171.86389522969));
#139734=CARTESIAN_POINT('',(-40.4577925858907,10.61999998,-144.90822241383));
#139735=CARTESIAN_POINT('Ctrl Pts',(-40.4577925858907,10.61999998,-144.90822241383));
#139736=CARTESIAN_POINT('Ctrl Pts',(-42.7973924930771,10.61999998,-149.265897143292));
#139737=CARTESIAN_POINT('Ctrl Pts',(-45.0988060523871,10.61999998,-153.643419067936));
#139738=CARTESIAN_POINT('Ctrl Pts',(-47.3760737205893,10.61999998,-158.033490718866));
#139739=CARTESIAN_POINT('Ctrl Pts',(-49.6533413887914,10.61999998,-162.423562369795));
#139740=CARTESIAN_POINT('Ctrl Pts',(-51.9061626796858,10.61999998,-166.826339923461));
#139741=CARTESIAN_POINT('Ctrl Pts',(-54.1424378198232,10.61999998,-171.237717270032));
#139742=CARTESIAN_POINT('',(-39.5,10.61999998,-140.924467062102));
#139743=CARTESIAN_POINT('Ctrl Pts',(-39.5,10.61999998,-140.924467062102));
#139744=CARTESIAN_POINT('Ctrl Pts',(-39.5,10.61999998,-141.064641740712));
#139745=CARTESIAN_POINT('Ctrl Pts',(-39.503286113677,10.619999980029,-141.204536867587));
#139746=CARTESIAN_POINT('Ctrl Pts',(-39.5098002370266,10.6199999796907,
-141.344151254401));
#139747=CARTESIAN_POINT('Ctrl Pts',(-39.5163738758532,10.6199999793493,
-141.48504121068));
#139748=CARTESIAN_POINT('Ctrl Pts',(-39.5262347839855,10.6199999785395,
-141.625645980314));
#139749=CARTESIAN_POINT('Ctrl Pts',(-39.5393758471116,10.6199999780094,
-141.765968909085));
#139750=CARTESIAN_POINT('Ctrl Pts',(-39.5454296177965,10.6199999777652,
-141.830612296341));
#139751=CARTESIAN_POINT('Ctrl Pts',(-39.5521802385778,10.6199999776063,
-141.895195868192));
#139752=CARTESIAN_POINT('Ctrl Pts',(-39.5596307210412,10.6199999776383,
-141.959719632822));
#139753=CARTESIAN_POINT('Ctrl Pts',(-39.5766960195726,10.6199999777115,
-142.107511042464));
#139754=CARTESIAN_POINT('Ctrl Pts',(-39.5974615300863,10.6199999785835,
-142.255205307));
#139755=CARTESIAN_POINT('Ctrl Pts',(-39.6219007996117,10.6199999791661,
-142.402216894674));
#139756=CARTESIAN_POINT('Ctrl Pts',(-39.6461342711765,10.6199999797438,
-142.547990528615));
#139757=CARTESIAN_POINT('Ctrl Pts',(-39.6739797737404,10.6199999799661,
-142.693092202937));
#139758=CARTESIAN_POINT('Ctrl Pts',(-39.7053613936664,10.6199999799929,
-142.836960501119));
#139759=CARTESIAN_POINT('Ctrl Pts',(-39.7158636782078,10.6199999800019,
-142.885107977494));
#139760=CARTESIAN_POINT('Ctrl Pts',(-39.7267615964739,10.61999998,-142.933117442992));
#139761=CARTESIAN_POINT('Ctrl Pts',(-39.7380510717141,10.61999998,-142.980968310073));
#139762=CARTESIAN_POINT('Ctrl Pts',(-39.8192390703692,10.61999998,-143.32508670792));
#139763=CARTESIAN_POINT('Ctrl Pts',(-39.9201606061929,10.61999998,-143.66253928893));
#139764=CARTESIAN_POINT('Ctrl Pts',(-40.0436577688856,10.61999998,-143.992366080452));
#139765=CARTESIAN_POINT('Ctrl Pts',(-40.1606310196878,10.61999998,-144.304769306281));
#139766=CARTESIAN_POINT('Ctrl Pts',(-40.2978572937945,10.61999998,-144.61033131776));
#139767=CARTESIAN_POINT('Ctrl Pts',(-40.4577925858907,10.61999998,-144.90822241383));
#139768=CARTESIAN_POINT('',(-39.5,10.61999998,-91.1341759094044));
#139769=CARTESIAN_POINT('',(-39.5,10.61999998,-55.24995));
#139770=CARTESIAN_POINT('',(-40.4577925858907,10.61999998,-87.1504205576762));
#139771=CARTESIAN_POINT('Ctrl Pts',(-40.4577925858907,10.61999998,-87.1504205576762));
#139772=CARTESIAN_POINT('Ctrl Pts',(-40.3970580365439,10.61999998,-87.2635430663928));
#139773=CARTESIAN_POINT('Ctrl Pts',(-40.3395672151842,10.61999998,-87.3780682227962));
#139774=CARTESIAN_POINT('Ctrl Pts',(-40.2851314284313,10.61999998,-87.4939105062412));
#139775=CARTESIAN_POINT('Ctrl Pts',(-40.228662932352,10.61999998,-87.6140785045144));
#139776=CARTESIAN_POINT('Ctrl Pts',(-40.1754817433885,10.61999998,-87.7356644050421));
#139777=CARTESIAN_POINT('Ctrl Pts',(-40.1254267036636,10.61999998,-87.8586004744554));
#139778=CARTESIAN_POINT('Ctrl Pts',(-40.0931586145966,10.61999998,-87.9378514761361));
#139779=CARTESIAN_POINT('Ctrl Pts',(-40.0621906903527,10.61999998,-88.0176641176432));
#139780=CARTESIAN_POINT('Ctrl Pts',(-40.0324904304423,10.61999998,-88.0980242245577));
#139781=CARTESIAN_POINT('Ctrl Pts',(-39.9448659684135,10.61999998,-88.3351100668433));
#139782=CARTESIAN_POINT('Ctrl Pts',(-39.8685902579997,10.61999998,-88.5761404610461));
#139783=CARTESIAN_POINT('Ctrl Pts',(-39.8033297324296,10.61999998,-88.8189034289914));
#139784=CARTESIAN_POINT('Ctrl Pts',(-39.779079208429,10.61999998,-88.9091130791463));
#139785=CARTESIAN_POINT('Ctrl Pts',(-39.7563491787977,10.61999998,-88.9995618473627));
#139786=CARTESIAN_POINT('Ctrl Pts',(-39.735120734996,10.61999998,-89.090136059728));
#139787=CARTESIAN_POINT('Ctrl Pts',(-39.6384824206275,10.61999998,-89.5024573438502));
#139788=CARTESIAN_POINT('Ctrl Pts',(-39.5716278198207,10.61999998,-89.9196108763344));
#139789=CARTESIAN_POINT('Ctrl Pts',(-39.5345653063048,10.61999998,-90.3415980465025));
#139790=CARTESIAN_POINT('Ctrl Pts',(-39.5115257817286,10.61999998,-90.6039219650835));
#139791=CARTESIAN_POINT('Ctrl Pts',(-39.500000000001,10.61999998,-90.8681139415185));
#139792=CARTESIAN_POINT('Ctrl Pts',(-39.5,10.61999998,-91.1341759094044));
#139793=CARTESIAN_POINT('Ctrl Pts',(-54.0201152391274,10.61999998,-61.0621827299711));
#139794=CARTESIAN_POINT('Ctrl Pts',(-51.8036107556176,10.61999998,-65.4330353431782));
#139795=CARTESIAN_POINT('Ctrl Pts',(-49.570749196272,10.61999998,-69.7953845096745));
#139796=CARTESIAN_POINT('Ctrl Pts',(-47.313790090977,10.61999998,-74.1452062415669));
#139797=CARTESIAN_POINT('Ctrl Pts',(-45.056830985682,10.61999998,-78.4950279734592));
#139798=CARTESIAN_POINT('Ctrl Pts',(-42.7760635123042,10.61999998,-82.8324726037656));
#139799=CARTESIAN_POINT('Ctrl Pts',(-40.4577925858907,10.61999998,-87.1504205576762));
#139800=CARTESIAN_POINT('',(-59.5,10.61999998,-58.24995));
#139801=CARTESIAN_POINT('Origin',(-57.,10.61999998,-58.24995));
#139802=CARTESIAN_POINT('',(-59.5,10.61999998,-174.34995));
#139803=CARTESIAN_POINT('',(-59.5,10.61999998,-58.24995));
#139804=CARTESIAN_POINT('',(-57.,10.61999998,-176.84995));
#139805=CARTESIAN_POINT('Origin',(-57.,10.61999998,-174.34995));
#139806=CARTESIAN_POINT('',(-54.2951871140408,10.61999998,-176.84995));
#139807=CARTESIAN_POINT('',(83.2809572255632,10.6199999800001,-176.84995));
#139808=CARTESIAN_POINT('',(-54.2951871140408,10.61999998,-176.84995));
#139809=CARTESIAN_POINT('Origin',(0.,-12.9675000200281,-60.64995));
#139810=CARTESIAN_POINT('',(-39.4379155619868,-56.882767417621,-60.64995));
#139811=CARTESIAN_POINT('',(-39.4999994911539,-56.8280450701514,-60.6499500000002));
#139812=CARTESIAN_POINT('Ctrl Pts',(-39.4379155619868,-56.882767417621,
-60.64995));
#139813=CARTESIAN_POINT('Ctrl Pts',(-39.4584539679692,-56.8643229911399,
-60.64995));
#139814=CARTESIAN_POINT('Ctrl Pts',(-39.4791489724441,-56.8460828416128,
-60.64995));
#139815=CARTESIAN_POINT('Ctrl Pts',(-39.4999988314732,-56.8280445593217,
-60.64995));
#139816=CARTESIAN_POINT('',(-33.85,-61.3211699373828,-60.64995));
#139817=CARTESIAN_POINT('Origin',(0.,-12.9675000200281,-60.64995));
#139818=CARTESIAN_POINT('',(-33.85,-12.9675000200281,-60.64995));
#139819=CARTESIAN_POINT('',(-39.5,-12.9675000200281,-60.64995));
#139820=CARTESIAN_POINT('Ctrl Pts',(-39.4564221286262,-64.6472412200127,
-59.64995));
#139821=CARTESIAN_POINT('Ctrl Pts',(-39.9999999999999,-64.599684318524,
-59.64995));
#139822=CARTESIAN_POINT('Ctrl Pts',(-40.,-65.1453385690586,-59.64995));
#139823=CARTESIAN_POINT('Ctrl Pts',(-39.4564221286269,-64.6472412200127,
-59.7808732880376));
#139824=CARTESIAN_POINT('Ctrl Pts',(-39.9999999999999,-64.5996843185171,
-59.7746029379318));
#139825=CARTESIAN_POINT('Ctrl Pts',(-40.,-65.1453385690423,-59.8463349320561));
#139826=CARTESIAN_POINT('Ctrl Pts',(-39.4575563441365,-64.6210152418146,
-59.9116978933072));
#139827=CARTESIAN_POINT('Ctrl Pts',(-40.,-64.5762635801886,-59.898971233264));
#139828=CARTESIAN_POINT('Ctrl Pts',(-40.,-65.1061484482599,-60.0425718399612));
#139829=CARTESIAN_POINT('Ctrl Pts',(-39.4619222489981,-64.5200642984147,
-60.153568971423));
#139830=CARTESIAN_POINT('Ctrl Pts',(-39.9999999999999,-64.4844350369598,
-60.1322291512609));
#139831=CARTESIAN_POINT('Ctrl Pts',(-40.,-64.9552949839326,-60.4053784571341));
#139832=CARTESIAN_POINT('Ctrl Pts',(-39.4651522214972,-64.4453790312801,
-60.2644967268053));
#139833=CARTESIAN_POINT('Ctrl Pts',(-39.9999999999999,-64.4163683849594,
-60.2406767152616));
#139834=CARTESIAN_POINT('Ctrl Pts',(-40.,-64.8436909621967,-60.5717700902076));
#139835=CARTESIAN_POINT('Ctrl Pts',(-39.4732193617865,-64.2588460104538,
-60.4496168355678));
#139836=CARTESIAN_POINT('Ctrl Pts',(-39.9999999999999,-64.2423415370877,
-60.4261994932778));
#139837=CARTESIAN_POINT('Ctrl Pts',(-40.,-64.5649501059399,-60.8494502533521));
#139838=CARTESIAN_POINT('Ctrl Pts',(-39.4780533572402,-64.1470716093135,
-60.5237363920406));
#139839=CARTESIAN_POINT('Ctrl Pts',(-39.9999999999993,-64.1369109528056,
-60.5031527166045));
#139840=CARTESIAN_POINT('Ctrl Pts',(-40.,-64.3979228839314,-60.9606295880612));
#139841=CARTESIAN_POINT('Ctrl Pts',(-39.4885935839748,-63.9033544725257,
-60.623922672982));
#139842=CARTESIAN_POINT('Ctrl Pts',(-40.0000000000006,-63.9016439800941,
-60.6120353079401));
#139843=CARTESIAN_POINT('Ctrl Pts',(-40.,-64.0337304042775,-61.1109090094727));
#139844=CARTESIAN_POINT('Ctrl Pts',(-39.4942946417933,-63.771531360673,
-60.64995));
#139845=CARTESIAN_POINT('Ctrl Pts',(-39.9999999999999,-63.7723272342478,
-60.6442102195365));
#139846=CARTESIAN_POINT('Ctrl Pts',(-40.,-63.8367439033901,-61.149949999985));
#139847=CARTESIAN_POINT('Ctrl Pts',(-39.5,-63.6396088127436,-60.64995));
#139848=CARTESIAN_POINT('Ctrl Pts',(-39.9999999999999,-63.6396088127435,
-60.64995));
#139849=CARTESIAN_POINT('Ctrl Pts',(-40.,-63.6396088127436,-61.14995));
#139850=CARTESIAN_POINT('',(-40.,-63.6396088127436,-61.14995));
#139851=CARTESIAN_POINT('Origin',(-39.5,-63.6396088127436,-61.14995));
#139852=CARTESIAN_POINT('Ctrl Pts',(-40.,-65.1453385690586,-59.64995));
#139853=CARTESIAN_POINT('Ctrl Pts',(-40.,-65.1453385690423,-59.8463349320561));
#139854=CARTESIAN_POINT('Ctrl Pts',(-40.,-65.1061484482599,-60.0425718399612));
#139855=CARTESIAN_POINT('Ctrl Pts',(-40.,-64.9552949839326,-60.4053784571341));
#139856=CARTESIAN_POINT('Ctrl Pts',(-40.,-64.8436909621967,-60.5717700902076));
#139857=CARTESIAN_POINT('Ctrl Pts',(-40.,-64.5649501059399,-60.8494502533521));
#139858=CARTESIAN_POINT('Ctrl Pts',(-40.,-64.3979228839314,-60.9606295880612));
#139859=CARTESIAN_POINT('Ctrl Pts',(-40.,-64.0337304042775,-61.1109090094727));
#139860=CARTESIAN_POINT('Ctrl Pts',(-40.,-63.8367439033901,-61.149949999985));
#139861=CARTESIAN_POINT('Ctrl Pts',(-40.,-63.6396088127436,-61.14995));
#139862=CARTESIAN_POINT('Ctrl Pts',(-33.85,-64.133919761665,-60.64995));
#139863=CARTESIAN_POINT('Ctrl Pts',(-33.35,-64.1339197616649,-60.64995));
#139864=CARTESIAN_POINT('Ctrl Pts',(-33.35,-64.133919761665,-61.14995));
#139865=CARTESIAN_POINT('Ctrl Pts',(-33.8442946417933,-64.2658423095942,
-60.64995));
#139866=CARTESIAN_POINT('Ctrl Pts',(-33.35,-64.265066231498,-60.6556217969808));
#139867=CARTESIAN_POINT('Ctrl Pts',(-33.35,-64.3310548523114,-61.149949999985));
#139868=CARTESIAN_POINT('Ctrl Pts',(-33.8385935839748,-64.3976654214474,
-60.6239226729819));
#139869=CARTESIAN_POINT('Ctrl Pts',(-33.3499999999993,-64.399347719172,
-60.6353187454038));
#139870=CARTESIAN_POINT('Ctrl Pts',(-33.35,-64.5280413531989,-61.1109090094727));
#139871=CARTESIAN_POINT('Ctrl Pts',(-33.8280533572402,-64.6413825582346,
-60.5237363920407));
#139872=CARTESIAN_POINT('Ctrl Pts',(-33.3500000000007,-64.6507229380173,
-60.5426326522465));
#139873=CARTESIAN_POINT('Ctrl Pts',(-33.35,-64.8922338328527,-60.9606295880612));
#139874=CARTESIAN_POINT('Ctrl Pts',(-33.8232193617858,-64.7531569593752,
-60.4496168355678));
#139875=CARTESIAN_POINT('Ctrl Pts',(-33.35,-64.7680300213717,-60.4706504746468));
#139876=CARTESIAN_POINT('Ctrl Pts',(-33.35,-65.0592610548614,-60.849450253352));
#139877=CARTESIAN_POINT('Ctrl Pts',(-33.8151522214979,-64.9396899802014,
-60.2644967268053));
#139878=CARTESIAN_POINT('Ctrl Pts',(-33.35,-64.9649606354368,-60.2852157712117));
#139879=CARTESIAN_POINT('Ctrl Pts',(-33.35,-65.338001911118,-60.5717700902076));
#139880=CARTESIAN_POINT('Ctrl Pts',(-33.8119222489988,-65.0143752473362,
-60.1535689714224));
#139881=CARTESIAN_POINT('Ctrl Pts',(-33.35,-65.0449787669832,-60.1718710142623));
#139882=CARTESIAN_POINT('Ctrl Pts',(-33.35,-65.4496059328539,-60.4053784571335));
#139883=CARTESIAN_POINT('Ctrl Pts',(-33.8075563441358,-65.1153261907357,
-59.9116978933078));
#139884=CARTESIAN_POINT('Ctrl Pts',(-33.35,-65.1530905830856,-59.9224177216081));
#139885=CARTESIAN_POINT('Ctrl Pts',(-33.35,-65.6004593971813,-60.0425718399618));
#139886=CARTESIAN_POINT('Ctrl Pts',(-33.8064221286289,-65.1415521689339,
-59.7808732880372));
#139887=CARTESIAN_POINT('Ctrl Pts',(-33.35,-65.1814839309564,-59.7861314644984));
#139888=CARTESIAN_POINT('Ctrl Pts',(-33.35,-65.6396495179636,-59.8463349320557));
#139889=CARTESIAN_POINT('Ctrl Pts',(-33.8064221286261,-65.1415521689341,
-59.64995));
#139890=CARTESIAN_POINT('Ctrl Pts',(-33.3499999999999,-65.1814839309712,
-59.64995));
#139891=CARTESIAN_POINT('Ctrl Pts',(-33.35,-65.63964951798,-59.64995));
#139892=CARTESIAN_POINT('',(-33.35,-64.133919761665,-61.14995));
#139893=CARTESIAN_POINT('Origin',(-33.85,-64.133919761665,-61.14995));
#139894=CARTESIAN_POINT('Ctrl Pts',(-33.35,-64.133919761665,-61.14995));
#139895=CARTESIAN_POINT('Ctrl Pts',(-33.35,-64.3310548523114,-61.149949999985));
#139896=CARTESIAN_POINT('Ctrl Pts',(-33.35,-64.5280413531989,-61.1109090094727));
#139897=CARTESIAN_POINT('Ctrl Pts',(-33.35,-64.8922338328527,-60.9606295880612));
#139898=CARTESIAN_POINT('Ctrl Pts',(-33.35,-65.0592610548614,-60.849450253352));
#139899=CARTESIAN_POINT('Ctrl Pts',(-33.35,-65.338001911118,-60.5717700902076));
#139900=CARTESIAN_POINT('Ctrl Pts',(-33.35,-65.4496059328539,-60.4053784571335));
#139901=CARTESIAN_POINT('Ctrl Pts',(-33.35,-65.6004593971813,-60.0425718399618));
#139902=CARTESIAN_POINT('Ctrl Pts',(-33.35,-65.6396495179636,-59.8463349320557));
#139903=CARTESIAN_POINT('Ctrl Pts',(-33.35,-65.63964951798,-59.64995));
#139904=CARTESIAN_POINT('Origin',(-40.,67.7009572055632,-55.24995));
#139905=CARTESIAN_POINT('',(-40.,-62.6133861954129,-171.14995));
#139906=CARTESIAN_POINT('',(-40.,-64.1281275541908,-172.64995));
#139907=CARTESIAN_POINT('Ctrl Pts',(-40.,-62.6133861954129,-171.14995));
#139908=CARTESIAN_POINT('Ctrl Pts',(-40.,-62.8117011147884,-171.149950000016));
#139909=CARTESIAN_POINT('Ctrl Pts',(-40.,-63.0098665547682,-171.18899099047));
#139910=CARTESIAN_POINT('Ctrl Pts',(-40.,-63.3762386807026,-171.339270411997));
#139911=CARTESIAN_POINT('Ctrl Pts',(-40.,-63.5442655393439,-171.450449746589));
#139912=CARTESIAN_POINT('Ctrl Pts',(-40.,-63.8246746245531,-171.728129909852));
#139913=CARTESIAN_POINT('Ctrl Pts',(-40.,-63.9369465821947,-171.894521542842));
#139914=CARTESIAN_POINT('Ctrl Pts',(-40.,-64.0887028854776,-172.257328160063));
#139915=CARTESIAN_POINT('Ctrl Pts',(-40.,-64.1281275541786,-172.453565067926));
#139916=CARTESIAN_POINT('Ctrl Pts',(-40.,-64.1281275541908,-172.64995));
#139917=CARTESIAN_POINT('',(-40.,-56.978215522411,-171.14995));
#139918=CARTESIAN_POINT('',(-40.,-62.5431157780617,-171.14995));
#139919=CARTESIAN_POINT('',(-40.,-56.7758867300388,-171.126786878085));
#139920=CARTESIAN_POINT('Ctrl Pts',(-40.,-56.7758867300388,-171.126786878085));
#139921=CARTESIAN_POINT('Ctrl Pts',(-40.,-56.8424288281835,-171.142376649979));
#139922=CARTESIAN_POINT('Ctrl Pts',(-40.,-56.909888666977,-171.14995));
#139923=CARTESIAN_POINT('Ctrl Pts',(-40.,-56.978215522411,-171.14995));
#139924=CARTESIAN_POINT('',(-40.,-56.3715344108516,-170.85018387548));
#139925=CARTESIAN_POINT('Ctrl Pts',(-40.,-56.3715344108516,-170.85018387548));
#139926=CARTESIAN_POINT('Ctrl Pts',(-40.,-56.3837583326098,-170.871947332769));
#139927=CARTESIAN_POINT('Ctrl Pts',(-40.,-56.3977040563913,-170.892479579619));
#139928=CARTESIAN_POINT('Ctrl Pts',(-39.9999999999999,-56.4130583083895,
-170.911803741317));
#139929=CARTESIAN_POINT('Ctrl Pts',(-39.9999999999997,-56.4292409786976,
-170.93217051254));
#139930=CARTESIAN_POINT('Ctrl Pts',(-39.9999999999994,-56.4469891868559,
-170.951195798845));
#139931=CARTESIAN_POINT('Ctrl Pts',(-39.9999999999991,-56.4659895184401,
-170.968879578563));
#139932=CARTESIAN_POINT('Ctrl Pts',(-39.9999999999989,-56.4862759122404,
-170.987760307968));
#139933=CARTESIAN_POINT('Ctrl Pts',(-39.9999999999988,-56.5079910115924,
-171.00511257564));
#139934=CARTESIAN_POINT('Ctrl Pts',(-39.9999999999991,-56.5307948409902,
-171.020896071165));
#139935=CARTESIAN_POINT('Ctrl Pts',(-39.9999999999992,-56.5352406042463,
-171.023973172086));
#139936=CARTESIAN_POINT('Ctrl Pts',(-39.9999999999993,-56.5397278285604,
-171.026990509393));
#139937=CARTESIAN_POINT('Ctrl Pts',(-39.9999999999994,-56.5442540887154,
-171.029947579459));
#139938=CARTESIAN_POINT('Ctrl Pts',(-39.9999999999994,-56.5444049748233,
-171.030046155497));
#139939=CARTESIAN_POINT('Ctrl Pts',(-39.9999999999994,-56.5445558983641,
-171.030144660686));
#139940=CARTESIAN_POINT('Ctrl Pts',(-39.9999999999994,-56.5447068592425,
-171.030243095025));
#139941=CARTESIAN_POINT('Ctrl Pts',(-39.9999999999998,-56.5677583970532,
-171.045273895852));
#139942=CARTESIAN_POINT('Ctrl Pts',(-39.9999999999999,-56.5918056322567,
-171.058759052615));
#139943=CARTESIAN_POINT('Ctrl Pts',(-39.9999999999999,-56.6166148891246,
-171.070798762234));
#139944=CARTESIAN_POINT('Ctrl Pts',(-40.,-56.6425070267785,-171.083363984176));
#139945=CARTESIAN_POINT('Ctrl Pts',(-40.,-56.6692310020628,-171.094354961296));
#139946=CARTESIAN_POINT('Ctrl Pts',(-40.,-56.6965412231962,-171.103832593434));
#139947=CARTESIAN_POINT('Ctrl Pts',(-40.,-56.7225306079871,-171.112851847704));
#139948=CARTESIAN_POINT('Ctrl Pts',(-40.,-56.7490526547635,-171.120500083882));
#139949=CARTESIAN_POINT('Ctrl Pts',(-40.,-56.7758867300388,-171.126786878085));
#139950=CARTESIAN_POINT('',(-40.,-55.08000002,-165.390538702986));
#139951=CARTESIAN_POINT('Ctrl Pts',(-40.,-55.08000002,-165.390538702986));
#139952=CARTESIAN_POINT('Ctrl Pts',(-40.,-55.08000002,-165.865206657822));
#139953=CARTESIAN_POINT('Ctrl Pts',(-40.,-55.1054794225748,-166.33732512172));
#139954=CARTESIAN_POINT('Ctrl Pts',(-40.,-55.1564354838473,-166.806894369245));
#139955=CARTESIAN_POINT('Ctrl Pts',(-40.,-55.2073915451197,-167.27646361677));
#139956=CARTESIAN_POINT('Ctrl Pts',(-40.,-55.2841712278673,-167.745175405874));
#139957=CARTESIAN_POINT('Ctrl Pts',(-40.,-55.3883950832632,-168.207118124506));
#139958=CARTESIAN_POINT('Ctrl Pts',(-40.,-55.4926189386592,-168.669060843138));
#139959=CARTESIAN_POINT('Ctrl Pts',(-40.,-55.6233617621228,-169.121472747749));
#139960=CARTESIAN_POINT('Ctrl Pts',(-40.,-55.7848473238897,-169.562835831867));
#139961=CARTESIAN_POINT('Ctrl Pts',(-40.,-55.9143897222723,-169.916893692202));
#139962=CARTESIAN_POINT('Ctrl Pts',(-40.,-56.0634514911903,-170.263936360591));
#139963=CARTESIAN_POINT('Ctrl Pts',(-40.,-56.2378305482492,-170.601880104106));
#139964=CARTESIAN_POINT('Ctrl Pts',(-40.,-56.2808297421808,-170.685211834478));
#139965=CARTESIAN_POINT('Ctrl Pts',(-40.,-56.3253685536862,-170.767990232518));
#139966=CARTESIAN_POINT('Ctrl Pts',(-40.,-56.3715344108516,-170.85018387548));
#139967=CARTESIAN_POINT('',(-40.,-55.08000002,-66.6681042685293));
#139968=CARTESIAN_POINT('',(-40.,-55.08000002,-166.086292363451));
#139969=CARTESIAN_POINT('',(-40.,-56.2369767507657,-61.4585861992193));
#139970=CARTESIAN_POINT('Ctrl Pts',(-40.,-56.2369767507657,-61.4585861992193));
#139971=CARTESIAN_POINT('Ctrl Pts',(-40.,-56.0300621110256,-61.860218211459));
#139972=CARTESIAN_POINT('Ctrl Pts',(-40.,-55.8576823937473,-62.2755058381188));
#139973=CARTESIAN_POINT('Ctrl Pts',(-40.,-55.7121267698271,-62.7014001044593));
#139974=CARTESIAN_POINT('Ctrl Pts',(-40.,-55.566571145907,-63.1272943707998));
#139975=CARTESIAN_POINT('Ctrl Pts',(-40.,-55.4484096188021,-63.563870007102));
#139976=CARTESIAN_POINT('Ctrl Pts',(-40.,-55.355528959088,-64.0016972473019));
#139977=CARTESIAN_POINT('Ctrl Pts',(-40.,-55.2432744366403,-64.5308503337945));
#139978=CARTESIAN_POINT('Ctrl Pts',(-40.,-55.1660815895365,-65.0649117752177));
#139979=CARTESIAN_POINT('Ctrl Pts',(-40.,-55.1225595401112,-65.6036868919965));
#139980=CARTESIAN_POINT('Ctrl Pts',(-40.,-55.0940603190416,-65.9564890086839));
#139981=CARTESIAN_POINT('Ctrl Pts',(-40.,-55.0800000199998,-66.3113124768414));
#139982=CARTESIAN_POINT('Ctrl Pts',(-40.,-55.08000002,-66.6681042685293));
#139983=CARTESIAN_POINT('',(-40.,-56.8280459100727,-61.14995));
#139984=CARTESIAN_POINT('Ctrl Pts',(-40.,-56.8280459100727,-61.14995));
#139985=CARTESIAN_POINT('Ctrl Pts',(-40.,-56.777525746988,-61.1499499958728));
#139986=CARTESIAN_POINT('Ctrl Pts',(-40.,-56.7268325166736,-61.15437366761));
#139987=CARTESIAN_POINT('Ctrl Pts',(-40.,-56.6774814901222,-61.1633382145165));
#139988=CARTESIAN_POINT('Ctrl Pts',(-40.,-56.6695344165963,-61.1647817896226));
#139989=CARTESIAN_POINT('Ctrl Pts',(-40.,-56.6616221088453,-61.1663432172135));
#139990=CARTESIAN_POINT('Ctrl Pts',(-40.,-56.6537508667182,-61.1680231060305));
#139991=CARTESIAN_POINT('Ctrl Pts',(-40.,-56.6068413991694,-61.1780345741923));
#139992=CARTESIAN_POINT('Ctrl Pts',(-40.,-56.5611509800557,-61.1921536886353));
#139993=CARTESIAN_POINT('Ctrl Pts',(-40.,-56.5168370445324,-61.2111466189146));
#139994=CARTESIAN_POINT('Ctrl Pts',(-40.,-56.5074712817997,-61.2151607800694));
#139995=CARTESIAN_POINT('Ctrl Pts',(-40.,-56.4981670562375,-61.2193928254494));
#139996=CARTESIAN_POINT('Ctrl Pts',(-40.,-56.4889259423713,-61.2238502921498));
#139997=CARTESIAN_POINT('Ctrl Pts',(-40.,-56.4359851254178,-61.2493863835866));
#139998=CARTESIAN_POINT('Ctrl Pts',(-40.,-56.3871673636495,-61.2813158980448));
#139999=CARTESIAN_POINT('Ctrl Pts',(-40.,-56.3436555786936,-61.3209915546623));
#140000=CARTESIAN_POINT('Ctrl Pts',(-40.,-56.3001590827628,-61.3606532701805));
#140001=CARTESIAN_POINT('Ctrl Pts',(-40.,-56.2640024859216,-61.4061278501816));
#140002=CARTESIAN_POINT('Ctrl Pts',(-40.,-56.2369767507657,-61.4585861992193));
#140003=CARTESIAN_POINT('',(-40.,67.7009572055632,-61.14995));
#140004=CARTESIAN_POINT('',(-40.,-70.08000002,-55.74995));
#140005=CARTESIAN_POINT('',(-40.,67.7009572055632,-55.74995));
#140006=CARTESIAN_POINT('',(-40.,-72.58000002,-58.24995));
#140007=CARTESIAN_POINT('Origin',(-40.,-70.08000002,-58.24995));
#140008=CARTESIAN_POINT('',(-40.,-72.58000002,-174.34995));
#140009=CARTESIAN_POINT('',(-40.,-72.58000002,-58.24995));
#140010=CARTESIAN_POINT('',(-40.,-70.08000002,-176.84995));
#140011=CARTESIAN_POINT('Origin',(-40.,-70.08000002,-174.34995));
#140012=CARTESIAN_POINT('',(-40.,-64.1281275541909,-176.84995));
#140013=CARTESIAN_POINT('',(-40.,67.7009572055632,-176.84995));
#140014=CARTESIAN_POINT('',(-40.,-64.1281275541909,-55.24995));
#140015=CARTESIAN_POINT('Origin',(-40.5,-73.08000002,-55.74995));
#140016=CARTESIAN_POINT('',(-40.5,-70.08000002,-55.24995));
#140017=CARTESIAN_POINT('',(-40.5,-73.08000002,-55.24995));
#140018=CARTESIAN_POINT('Origin',(-40.5,-70.08000002,-55.74995));
#140019=CARTESIAN_POINT('Origin',(-41.5,-73.08000002,-55.24995));
#140020=CARTESIAN_POINT('',(-41.,-70.08000002,-55.24995));
#140021=CARTESIAN_POINT('',(-41.,-73.08000002,-55.24995));
#140022=CARTESIAN_POINT('',(-41.5,-70.08000002,-55.24995));
#140023=CARTESIAN_POINT('Origin',(-41.,-73.08000002,-55.74995));
#140024=CARTESIAN_POINT('',(-41.5,-70.08000002,-55.74995));
#140025=CARTESIAN_POINT('',(-41.5,-73.08000002,-55.74995));
#140026=CARTESIAN_POINT('Origin',(-41.,-70.08000002,-55.74995));
#140027=CARTESIAN_POINT('Origin',(-41.5,-73.08000002,-177.34995));
#140028=CARTESIAN_POINT('',(-41.5,-58.6035812240168,-171.14995));
#140029=CARTESIAN_POINT('',(-41.5,-56.3473237326807,-171.14995));
#140030=CARTESIAN_POINT('Ctrl Pts',(-41.5,-58.6035812240168,-171.14995));
#140031=CARTESIAN_POINT('Ctrl Pts',(-41.5,-58.4156574039305,-171.149950044596));
#140032=CARTESIAN_POINT('Ctrl Pts',(-41.4999999999992,-58.2278101348557,
-171.167358426711));
#140033=CARTESIAN_POINT('Ctrl Pts',(-41.5000000000009,-58.0399262281501,
-171.183208448531));
#140034=CARTESIAN_POINT('Ctrl Pts',(-41.5000000000009,-58.0397839854562,
-171.183220448228));
#140035=CARTESIAN_POINT('Ctrl Pts',(-41.5000000000009,-58.039641742701,
-171.183232446501));
#140036=CARTESIAN_POINT('Ctrl Pts',(-41.5000000000009,-58.0394994998845,
-171.183244443348));
#140037=CARTESIAN_POINT('Ctrl Pts',(-41.5000000000023,-57.8789705149886,
-171.196783556842));
#140038=CARTESIAN_POINT('Ctrl Pts',(-41.4999999999993,-57.7184422672608,
-171.208492413784));
#140039=CARTESIAN_POINT('Ctrl Pts',(-41.500000000002,-57.5579169091739,
-171.211623701818));
#140040=CARTESIAN_POINT('Ctrl Pts',(-41.5000000000025,-57.5306624002507,
-171.212155341919));
#140041=CARTESIAN_POINT('Ctrl Pts',(-41.5000000000032,-57.5034079726239,
-171.212439843791));
#140042=CARTESIAN_POINT('Ctrl Pts',(-41.5000000000045,-57.4761536342535,
-171.212444366369));
#140043=CARTESIAN_POINT('Ctrl Pts',(-41.5000000000045,-57.4759114394356,
-171.212444406558));
#140044=CARTESIAN_POINT('Ctrl Pts',(-41.5000000000045,-57.4756692446243,
-171.212444424596));
#140045=CARTESIAN_POINT('Ctrl Pts',(-41.5000000000045,-57.4754270498201,
-171.212444420506));
#140046=CARTESIAN_POINT('Ctrl Pts',(-41.5000000000123,-57.314176726691,
-171.21244169735));
#140047=CARTESIAN_POINT('Ctrl Pts',(-41.5000000000007,-57.1529297994809,
-171.202628065338));
#140048=CARTESIAN_POINT('Ctrl Pts',(-41.5000000000001,-56.9916840158814,
-171.189830777412));
#140049=CARTESIAN_POINT('Ctrl Pts',(-41.5,-56.9650429028844,-171.187716402784));
#140050=CARTESIAN_POINT('Ctrl Pts',(-41.5,-56.9384018138948,-171.185520466727));
#140051=CARTESIAN_POINT('Ctrl Pts',(-41.5,-56.9117607329796,-171.183273657174));
#140052=CARTESIAN_POINT('Ctrl Pts',(-41.5,-56.9116320467988,-171.18326280426));
#140053=CARTESIAN_POINT('Ctrl Pts',(-41.5,-56.9115033606235,-171.183251950612));
#140054=CARTESIAN_POINT('Ctrl Pts',(-41.5,-56.9113746744539,-171.183241096235));
#140055=CARTESIAN_POINT('Ctrl Pts',(-41.5000000000001,-56.7724125203318,
-171.171519963661));
#140056=CARTESIAN_POINT('Ctrl Pts',(-41.5,-56.6334506983164,-171.158942972401));
#140057=CARTESIAN_POINT('Ctrl Pts',(-41.5,-56.494486471775,-171.153174108112));
#140058=CARTESIAN_POINT('Ctrl Pts',(-41.5,-56.4454325541915,-171.151137717881));
#140059=CARTESIAN_POINT('Ctrl Pts',(-41.5,-56.3963783401894,-171.149950012104));
#140060=CARTESIAN_POINT('Ctrl Pts',(-41.5,-56.3473237326807,-171.14995));
#140061=CARTESIAN_POINT('',(-41.5,-62.2620341086569,-171.14995));
#140062=CARTESIAN_POINT('',(-41.5,-55.58000002,-171.14995));
#140063=CARTESIAN_POINT('',(-41.5,-63.7767754674349,-172.64995));
#140064=CARTESIAN_POINT('Ctrl Pts',(-41.5,-63.7767754674349,-172.64995));
#140065=CARTESIAN_POINT('Ctrl Pts',(-41.5,-63.7767754674226,-172.453565067926));
#140066=CARTESIAN_POINT('Ctrl Pts',(-41.5,-63.7373507987217,-172.257328160063));
#140067=CARTESIAN_POINT('Ctrl Pts',(-41.5,-63.5855944954388,-171.894521542842));
#140068=CARTESIAN_POINT('Ctrl Pts',(-41.5,-63.4733225377971,-171.728129909852));
#140069=CARTESIAN_POINT('Ctrl Pts',(-41.5,-63.192913452588,-171.450449746589));
#140070=CARTESIAN_POINT('Ctrl Pts',(-41.5,-63.0248865939453,-171.339270411997));
#140071=CARTESIAN_POINT('Ctrl Pts',(-41.5,-62.6585144680136,-171.18899099047));
#140072=CARTESIAN_POINT('Ctrl Pts',(-41.5,-62.4603490280314,-171.149950000016));
#140073=CARTESIAN_POINT('Ctrl Pts',(-41.5,-62.2620341086569,-171.14995));
#140074=CARTESIAN_POINT('',(-41.5,-63.7767754674349,-176.84995));
#140075=CARTESIAN_POINT('',(-41.5,-63.7767754674349,-177.34995));
#140076=CARTESIAN_POINT('',(-41.5,-70.08000002,-176.84995));
#140077=CARTESIAN_POINT('',(-41.5,-73.08000002,-176.84995));
#140078=CARTESIAN_POINT('',(-41.5,-72.58000002,-174.34995));
#140079=CARTESIAN_POINT('Origin',(-41.5,-70.08000002,-174.34995));
#140080=CARTESIAN_POINT('',(-41.5,-72.58000002,-58.24995));
#140081=CARTESIAN_POINT('',(-41.5,-72.58000002,-174.34995));
#140082=CARTESIAN_POINT('Origin',(-41.5,-70.08000002,-58.24995));
#140083=CARTESIAN_POINT('',(-41.5,-63.4208871539288,-61.14995));
#140084=CARTESIAN_POINT('Ctrl Pts',(-41.5,-63.4208871539288,-61.14995));
#140085=CARTESIAN_POINT('Ctrl Pts',(-41.5,-63.6180222445752,-61.149949999985));
#140086=CARTESIAN_POINT('Ctrl Pts',(-41.5,-63.8150087454628,-61.1109090094727));
#140087=CARTESIAN_POINT('Ctrl Pts',(-41.5,-64.1792012251166,-60.9606295880612));
#140088=CARTESIAN_POINT('Ctrl Pts',(-41.5,-64.3462284471252,-60.849450253352));
#140089=CARTESIAN_POINT('Ctrl Pts',(-41.5,-64.6249693033818,-60.5717700902076));
#140090=CARTESIAN_POINT('Ctrl Pts',(-41.5,-64.7365733251178,-60.4053784571342));
#140091=CARTESIAN_POINT('Ctrl Pts',(-41.5,-64.8874267894451,-60.0425718399611));
#140092=CARTESIAN_POINT('Ctrl Pts',(-41.5,-64.9266169102275,-59.8463349320562));
#140093=CARTESIAN_POINT('Ctrl Pts',(-41.5,-64.9266169102438,-59.64995));
#140094=CARTESIAN_POINT('',(-41.5,-58.6035812240174,-61.14995));
#140095=CARTESIAN_POINT('',(-41.5,-73.08000002,-61.14995));
#140096=CARTESIAN_POINT('',(-41.5,-56.3473237326805,-61.14995));
#140097=CARTESIAN_POINT('Ctrl Pts',(-41.5,-56.3473237326805,-61.14995));
#140098=CARTESIAN_POINT('Ctrl Pts',(-41.5,-56.4247882486865,-61.1499499808859));
#140099=CARTESIAN_POINT('Ctrl Pts',(-41.5,-56.5020743317105,-61.146992865599));
#140100=CARTESIAN_POINT('Ctrl Pts',(-41.5,-56.5792618257269,-61.1424262748502));
#140101=CARTESIAN_POINT('Ctrl Pts',(-41.5,-56.6823474618058,-61.1363274900916));
#140102=CARTESIAN_POINT('Ctrl Pts',(-41.5,-56.7852572696789,-61.1273561280416));
#140103=CARTESIAN_POINT('Ctrl Pts',(-41.5000000000002,-56.8881825068214,
-61.1186215077308));
#140104=CARTESIAN_POINT('Ctrl Pts',(-41.5000000000002,-56.8960417889417,
-61.1179545396757));
#140105=CARTESIAN_POINT('Ctrl Pts',(-41.5000000000002,-56.9039011612638,
-61.1172889307083));
#140106=CARTESIAN_POINT('Ctrl Pts',(-41.5000000000002,-56.9117607090172,
-61.1166260587005));
#140107=CARTESIAN_POINT('Ctrl Pts',(-41.5000000000002,-56.9118309970963,
-61.116620130624));
#140108=CARTESIAN_POINT('Ctrl Pts',(-41.5000000000002,-56.9119012851879,
-61.1166142029013));
#140109=CARTESIAN_POINT('Ctrl Pts',(-41.5000000000002,-56.9119715732919,
-61.1166082755328));
#140110=CARTESIAN_POINT('Ctrl Pts',(-41.5000000000007,-57.0997257526663,
-61.1007750386643));
#140111=CARTESIAN_POINT('Ctrl Pts',(-41.4999999999977,-57.2880101287523,
-61.0874286525006));
#140112=CARTESIAN_POINT('Ctrl Pts',(-41.5000000000023,-57.4761536341595,
-61.0874562423818));
#140113=CARTESIAN_POINT('Ctrl Pts',(-41.5000000000023,-57.476328431569,
-61.0874562680146));
#140114=CARTESIAN_POINT('Ctrl Pts',(-41.5000000000023,-57.4765032288573,
-61.087456305165));
#140115=CARTESIAN_POINT('Ctrl Pts',(-41.5000000000023,-57.4766780260241,
-61.0874563538243));
#140116=CARTESIAN_POINT('Ctrl Pts',(-41.500000000005,-57.5875579724858,
-61.0874872201067));
#140117=CARTESIAN_POINT('Ctrl Pts',(-41.5000000000027,-57.698214536846,
-61.0921466646789));
#140118=CARTESIAN_POINT('Ctrl Pts',(-41.5000000000012,-57.808755193549,
-61.099196348861));
#140119=CARTESIAN_POINT('Ctrl Pts',(-41.5000000000001,-57.8858564168486,
-61.1041134471534));
#140120=CARTESIAN_POINT('Ctrl Pts',(-41.5,-57.9629012529634,-61.1101948863673));
#140121=CARTESIAN_POINT('Ctrl Pts',(-41.5,-58.039926161923,-61.1166923365635));
#140122=CARTESIAN_POINT('Ctrl Pts',(-41.5,-58.0400259760022,-61.1167007563983));
#140123=CARTESIAN_POINT('Ctrl Pts',(-41.5,-58.0401257900677,-61.1167091766712));
#140124=CARTESIAN_POINT('Ctrl Pts',(-41.5,-58.0402256041196,-61.1167175973794));
#140125=CARTESIAN_POINT('Ctrl Pts',(-41.5000000000001,-58.1358345616333,
-61.1247835471793));
#140126=CARTESIAN_POINT('Ctrl Pts',(-41.5,-58.2314235934514,-61.1332503625508));
#140127=CARTESIAN_POINT('Ctrl Pts',(-41.5,-58.3271142909714,-61.1396237955236));
#140128=CARTESIAN_POINT('Ctrl Pts',(-41.5,-58.4115316341018,-61.145246372139));
#140129=CARTESIAN_POINT('Ctrl Pts',(-41.5,-58.4960281098014,-61.149241951551));
#140130=CARTESIAN_POINT('Ctrl Pts',(-41.5,-58.5806871719333,-61.1498651031254));
#140131=CARTESIAN_POINT('Ctrl Pts',(-41.5,-58.5883171817095,-61.149921265484));
#140132=CARTESIAN_POINT('Ctrl Pts',(-41.5,-58.5959485120575,-61.1499499981887));
#140133=CARTESIAN_POINT('Ctrl Pts',(-41.5,-58.6035812240174,-61.14995));
#140134=CARTESIAN_POINT('',(-41.5,-55.58000002,-61.14995));
#140135=CARTESIAN_POINT('',(-41.5,-73.08000002,-61.14995));
#140136=CARTESIAN_POINT('',(-41.5,-55.58000002,-171.14995));
#140137=CARTESIAN_POINT('',(-41.5,-55.58000002,-60.64995));
#140138=CARTESIAN_POINT('',(-41.5,-55.58000002,-171.14995));
#140139=CARTESIAN_POINT('Ctrl Pts',(-42.,-63.4208871539288,-60.64995));
#140140=CARTESIAN_POINT('Ctrl Pts',(-41.4999999999999,-63.4208871539288,
-60.64995));
#140141=CARTESIAN_POINT('Ctrl Pts',(-41.5,-63.4208871539288,-61.14995));
#140142=CARTESIAN_POINT('Ctrl Pts',(-41.9942946417934,-63.5528097018572,
-60.64995));
#140143=CARTESIAN_POINT('Ctrl Pts',(-41.5,-63.5520336237608,-60.6556217969809));
#140144=CARTESIAN_POINT('Ctrl Pts',(-41.5,-63.6180222445752,-61.149949999985));
#140145=CARTESIAN_POINT('Ctrl Pts',(-41.9885935839755,-63.6846328137124,
-60.6239226729814));
#140146=CARTESIAN_POINT('Ctrl Pts',(-41.4999999999993,-63.6863151114373,
-60.6353187454032));
#140147=CARTESIAN_POINT('Ctrl Pts',(-41.5,-63.8150087454628,-61.1109090094727));
#140148=CARTESIAN_POINT('Ctrl Pts',(-41.9780533572395,-63.9283499504973,
-60.5237363920413));
#140149=CARTESIAN_POINT('Ctrl Pts',(-41.5000000000007,-63.9376903302796,
-60.5426326522472));
#140150=CARTESIAN_POINT('Ctrl Pts',(-41.5,-64.1792012251166,-60.9606295880612));
#140151=CARTESIAN_POINT('Ctrl Pts',(-41.9732193617859,-64.0401243516391,
-60.4496168355678));
#140152=CARTESIAN_POINT('Ctrl Pts',(-41.5,-64.0549974136357,-60.4706504746468));
#140153=CARTESIAN_POINT('Ctrl Pts',(-41.5,-64.3462284471252,-60.849450253352));
#140154=CARTESIAN_POINT('Ctrl Pts',(-41.9651522214979,-64.2266573724653,
-60.2644967268053));
#140155=CARTESIAN_POINT('Ctrl Pts',(-41.4999999999999,-64.2519280277007,
-60.2852157712117));
#140156=CARTESIAN_POINT('Ctrl Pts',(-41.5,-64.6249693033818,-60.5717700902076));
#140157=CARTESIAN_POINT('Ctrl Pts',(-41.9619222489988,-64.3013426395998,
-60.153568971423));
#140158=CARTESIAN_POINT('Ctrl Pts',(-41.5,-64.3319461592471,-60.1718710142637));
#140159=CARTESIAN_POINT('Ctrl Pts',(-41.5,-64.7365733251178,-60.4053784571342));
#140160=CARTESIAN_POINT('Ctrl Pts',(-41.9575563441358,-64.4022935829999,
-59.9116978933072));
#140161=CARTESIAN_POINT('Ctrl Pts',(-41.5,-64.4400579753494,-59.9224177216068));
#140162=CARTESIAN_POINT('Ctrl Pts',(-41.5,-64.8874267894451,-60.0425718399611));
#140163=CARTESIAN_POINT('Ctrl Pts',(-41.9564221286289,-64.4285195611977,
-59.7808732880376));
#140164=CARTESIAN_POINT('Ctrl Pts',(-41.5,-64.4684513232201,-59.7861314644994));
#140165=CARTESIAN_POINT('Ctrl Pts',(-41.5,-64.9266169102275,-59.8463349320562));
#140166=CARTESIAN_POINT('Ctrl Pts',(-41.9564221286262,-64.428519561198,
-59.64995));
#140167=CARTESIAN_POINT('Ctrl Pts',(-41.5,-64.4684513232351,-59.64995));
#140168=CARTESIAN_POINT('Ctrl Pts',(-41.5,-64.9266169102438,-59.64995));
#140169=CARTESIAN_POINT('Origin',(-42.,-63.4208871539288,-61.14995));
#140170=CARTESIAN_POINT('Ctrl Pts',(-25.559825688233,-65.4594929016656,
-60.8818893816927));
#140171=CARTESIAN_POINT('Ctrl Pts',(-25.2,-65.5225267460509,-60.9659777046599));
#140172=CARTESIAN_POINT('Ctrl Pts',(-25.2,-65.7473676730038,-61.2659196908451));
#140173=CARTESIAN_POINT('Ctrl Pts',(-25.5689423412454,-65.58489046904,-60.7845618642934));
#140174=CARTESIAN_POINT('Ctrl Pts',(-25.2,-65.6598013792258,-60.8537298337023));
#140175=CARTESIAN_POINT('Ctrl Pts',(-25.2,-65.9366774304564,-61.1240102848084));
#140176=CARTESIAN_POINT('Ctrl Pts',(-25.5836282597575,-65.6869336598766,
-60.6533188274199));
#140177=CARTESIAN_POINT('Ctrl Pts',(-25.2,-65.7653321407853,-60.7026110037421));
#140178=CARTESIAN_POINT('Ctrl Pts',(-25.2,-66.0916524900825,-60.9336707597463));
#140179=CARTESIAN_POINT('Ctrl Pts',(-25.6175094928883,-65.8217787894205,
-60.3603674876955));
#140180=CARTESIAN_POINT('Ctrl Pts',(-25.2,-65.8913484330066,-60.3775874746364));
#140181=CARTESIAN_POINT('Ctrl Pts',(-25.2,-66.2983665260919,-60.5086792251106));
#140182=CARTESIAN_POINT('Ctrl Pts',(-25.6369719721911,-65.8562864448621,
-60.1960022731895));
#140183=CARTESIAN_POINT('Ctrl Pts',(-25.2,-65.9121534157352,-60.1989021139916));
#140184=CARTESIAN_POINT('Ctrl Pts',(-25.2,-66.3526821146748,-60.2701831868566));
#140185=CARTESIAN_POINT('Ctrl Pts',(-25.6564221286262,-65.8545847766702,
-60.0322609860583));
#140186=CARTESIAN_POINT('Ctrl Pts',(-25.2,-65.8945165387074,-60.0322609860583));
#140187=CARTESIAN_POINT('Ctrl Pts',(-25.2,-66.3526821257161,-60.0322609860583));
#140188=CARTESIAN_POINT('',(-25.2,-65.7473676730073,-61.2659196908498));
#140189=CARTESIAN_POINT('Origin',(-25.7,-65.7473676730073,-61.2659196908498));
#140190=CARTESIAN_POINT('Ctrl Pts',(-25.2,-65.7473676730038,-61.2659196908451));
#140191=CARTESIAN_POINT('Ctrl Pts',(-25.2,-65.7793674058565,-61.2419322158012));
#140192=CARTESIAN_POINT('Ctrl Pts',(-25.2,-65.8101247224078,-61.2167624788248));
#140193=CARTESIAN_POINT('Ctrl Pts',(-25.2,-65.8397093268158,-61.1904934725279));
#140194=CARTESIAN_POINT('Ctrl Pts',(-25.2,-65.8701731473597,-61.163443785378));
#140195=CARTESIAN_POINT('Ctrl Pts',(-25.2,-65.8993940496695,-61.1352280130908));
#140196=CARTESIAN_POINT('Ctrl Pts',(-25.2,-65.9274189899595,-61.105888948837));
#140197=CARTESIAN_POINT('Ctrl Pts',(-25.2,-65.953675127919,-61.0784016282334));
#140198=CARTESIAN_POINT('Ctrl Pts',(-25.2,-65.9788815373659,-61.0499274395304));
#140199=CARTESIAN_POINT('Ctrl Pts',(-25.2,-66.003048363658,-61.0204714365432));
#140200=CARTESIAN_POINT('Ctrl Pts',(-25.2,-66.0310884832222,-60.9862944272966));
#140201=CARTESIAN_POINT('Ctrl Pts',(-25.2,-66.0577887607432,-60.9507091443297));
#140202=CARTESIAN_POINT('Ctrl Pts',(-25.2,-66.0829136816528,-60.9139799086674));
#140203=CARTESIAN_POINT('Ctrl Pts',(-25.2,-66.1080535088014,-60.8772288821003));
#140204=CARTESIAN_POINT('Ctrl Pts',(-25.2,-66.1316155749469,-60.8393332860743));
#140205=CARTESIAN_POINT('Ctrl Pts',(-25.2,-66.1534043153279,-60.8005903814081));
#140206=CARTESIAN_POINT('Ctrl Pts',(-25.2,-66.1680937996861,-60.7744707764132));
#140207=CARTESIAN_POINT('Ctrl Pts',(-25.2,-66.1819781266407,-60.7479667213004));
#140208=CARTESIAN_POINT('Ctrl Pts',(-25.2,-66.1950095070847,-60.7211749919409));
#140209=CARTESIAN_POINT('Ctrl Pts',(-25.2,-66.2246788862505,-60.6601765443636));
#140210=CARTESIAN_POINT('Ctrl Pts',(-25.2,-66.2502610540319,-60.5971407841896));
#140211=CARTESIAN_POINT('Ctrl Pts',(-25.2,-66.2716923178953,-60.5326135007196));
#140212=CARTESIAN_POINT('Ctrl Pts',(-25.2,-66.2932651285445,-60.4676600347516));
#140213=CARTESIAN_POINT('Ctrl Pts',(-25.2,-66.3106323191261,-60.4011940591385));
#140214=CARTESIAN_POINT('Ctrl Pts',(-25.2,-66.3236799285786,-60.3337525435423));
#140215=CARTESIAN_POINT('Ctrl Pts',(-25.2,-66.3364083912035,-60.2679606593083));
#140216=CARTESIAN_POINT('Ctrl Pts',(-25.2,-66.345026048704,-60.2012392210405));
#140217=CARTESIAN_POINT('Ctrl Pts',(-25.2,-66.3493785138956,-60.1340856776664));
#140218=CARTESIAN_POINT('Ctrl Pts',(-25.2,-66.3515726828295,-60.1002321688644));
#140219=CARTESIAN_POINT('Ctrl Pts',(-25.2,-66.3526821241379,-60.0662689342246));
#140220=CARTESIAN_POINT('Ctrl Pts',(-25.2,-66.3526821257161,-60.0322609860583));
#140221=CARTESIAN_POINT('Origin',(-25.2,67.7009572055632,-55.24995));
#140222=CARTESIAN_POINT('',(-25.2,-70.08000002,-176.84995));
#140223=CARTESIAN_POINT('',(-25.2,-66.1031295107182,-176.84995));
#140224=CARTESIAN_POINT('',(-25.2,67.7009572055632,-176.84995));
#140225=CARTESIAN_POINT('',(-25.2,-72.58000002,-174.34995));
#140226=CARTESIAN_POINT('Origin',(-25.2,-70.08000002,-174.34995));
#140227=CARTESIAN_POINT('',(-25.2,-72.58000002,-58.24995));
#140228=CARTESIAN_POINT('',(-25.2,-72.58000002,-174.34995));
#140229=CARTESIAN_POINT('Origin',(-25.2,-70.08000002,-58.24995));
#140230=CARTESIAN_POINT('',(-25.2,-65.5994372375942,-61.4386408691297));
#140231=CARTESIAN_POINT('Origin',(-25.2,-66.2733246929871,-61.7660459272207));
#140232=CARTESIAN_POINT('',(-25.2,-56.0768896606488,-79.4153515046414));
#140233=CARTESIAN_POINT('Ctrl Pts',(-25.2,-56.0768896606488,-79.4153515046414));
#140234=CARTESIAN_POINT('Ctrl Pts',(-25.2,-59.3123551324919,-73.4555771707379));
#140235=CARTESIAN_POINT('Ctrl Pts',(-25.2,-62.4759494901776,-67.4577315724186));
#140236=CARTESIAN_POINT('Ctrl Pts',(-25.2,-65.5994372375941,-61.4386408691297));
#140237=CARTESIAN_POINT('',(-25.2,-55.08000002,-83.5456386250819));
#140238=CARTESIAN_POINT('Ctrl Pts',(-25.2,-55.08000002,-83.5456386250819));
#140239=CARTESIAN_POINT('Ctrl Pts',(-25.2,-55.08000002,-83.1859931739116));
#140240=CARTESIAN_POINT('Ctrl Pts',(-25.2,-55.1006621337637,-82.8281867002424));
#140241=CARTESIAN_POINT('Ctrl Pts',(-25.2,-55.1417030348395,-82.4721939873444));
#140242=CARTESIAN_POINT('Ctrl Pts',(-25.2,-55.1827439359154,-82.1162012744465));
#140243=CARTESIAN_POINT('Ctrl Pts',(-25.2,-55.2446154752335,-81.7605756924467));
#140244=CARTESIAN_POINT('Ctrl Pts',(-25.2,-55.3267103680732,-81.412917955686));
#140245=CARTESIAN_POINT('Ctrl Pts',(-25.2,-55.4088052609129,-81.0652602189252));
#140246=CARTESIAN_POINT('Ctrl Pts',(-25.2,-55.5103655940696,-80.7242806574902));
#140247=CARTESIAN_POINT('Ctrl Pts',(-25.2,-55.6343884585548,-80.3910074402699));
#140248=CARTESIAN_POINT('Ctrl Pts',(-25.2,-55.75841132304,-80.0577342230495));
#140249=CARTESIAN_POINT('Ctrl Pts',(-25.2,-55.9048956589413,-79.7321669507792));
#140250=CARTESIAN_POINT('Ctrl Pts',(-25.2,-56.0768896606488,-79.4153515046414));
#140251=CARTESIAN_POINT('',(-25.2,-55.08000002,-148.513004346424));
#140252=CARTESIAN_POINT('',(-25.2,-55.08000002,-84.0594740639255));
#140253=CARTESIAN_POINT('',(-25.2,-56.0768896606488,-152.643291466864));
#140254=CARTESIAN_POINT('Ctrl Pts',(-25.2,-56.0768896606487,-152.643291466864));
#140255=CARTESIAN_POINT('Ctrl Pts',(-25.2,-56.0149669290359,-152.529228896965));
#140256=CARTESIAN_POINT('Ctrl Pts',(-25.2,-55.9563289964362,-152.41374598058));
#140257=CARTESIAN_POINT('Ctrl Pts',(-25.2,-55.9007756544416,-152.296934067097));
#140258=CARTESIAN_POINT('Ctrl Pts',(-25.2,-55.8430042328458,-152.175458201578));
#140259=CARTESIAN_POINT('Ctrl Pts',(-25.2,-55.788568493397,-152.052544547971));
#140260=CARTESIAN_POINT('Ctrl Pts',(-25.2,-55.737292667624,-151.928266900594));
#140261=CARTESIAN_POINT('Ctrl Pts',(-25.2,-55.7009775154013,-151.840249562709));
#140262=CARTESIAN_POINT('Ctrl Pts',(-25.2,-55.6662483997962,-151.751547420779));
#140263=CARTESIAN_POINT('Ctrl Pts',(-25.2,-55.6330574644204,-151.662180878469));
#140264=CARTESIAN_POINT('Ctrl Pts',(-25.2,-55.5638026420096,-151.475712375937));
#140265=CARTESIAN_POINT('Ctrl Pts',(-25.2,-55.5013746560306,-151.2866750003));
#140266=CARTESIAN_POINT('Ctrl Pts',(-25.2,-55.445644045516,-151.096220906455));
#140267=CARTESIAN_POINT('Ctrl Pts',(-25.2,-55.400687777676,-150.942587110322));
#140268=CARTESIAN_POINT('Ctrl Pts',(-25.2,-55.3600885309565,-150.788032233726));
#140269=CARTESIAN_POINT('Ctrl Pts',(-25.2,-55.323754356376,-150.633166383806));
#140270=CARTESIAN_POINT('Ctrl Pts',(-25.2,-55.2248092846637,-150.21143635132));
#140271=CARTESIAN_POINT('Ctrl Pts',(-25.2,-55.1560866851002,-149.784875950083));
#140272=CARTESIAN_POINT('Ctrl Pts',(-25.2,-55.1174016248561,-149.353514705421));
#140273=CARTESIAN_POINT('Ctrl Pts',(-25.2,-55.0924544716303,-149.075339228934));
#140274=CARTESIAN_POINT('Ctrl Pts',(-25.2,-55.0800000200004,-148.795167064059));
#140275=CARTESIAN_POINT('Ctrl Pts',(-25.2,-55.08000002,-148.513004346424));
#140276=CARTESIAN_POINT('',(-25.2,-65.7246041881209,-170.861259130871));
#140277=CARTESIAN_POINT('Ctrl Pts',(-25.2,-65.7246041881209,-170.861259130871));
#140278=CARTESIAN_POINT('Ctrl Pts',(-25.2,-62.5605227754587,-164.761159036905));
#140279=CARTESIAN_POINT('Ctrl Pts',(-25.2,-59.3555847723563,-158.682695424483));
#140280=CARTESIAN_POINT('Ctrl Pts',(-25.2,-56.0768896606488,-152.643291466864));
#140281=CARTESIAN_POINT('',(-25.2,-65.7816577220592,-170.947457636992));
#140282=CARTESIAN_POINT('Ctrl Pts',(-25.2,-65.7816577220592,-170.947457636992));
#140283=CARTESIAN_POINT('Ctrl Pts',(-25.2,-65.759637326036,-170.920712146581));
#140284=CARTESIAN_POINT('Ctrl Pts',(-25.2,-65.7405592277015,-170.892019192244));
#140285=CARTESIAN_POINT('Ctrl Pts',(-25.2,-65.7246041881209,-170.861259130871));
#140286=CARTESIAN_POINT('',(-25.2,-66.1031295107175,-171.854014632589));
#140287=CARTESIAN_POINT('Ctrl Pts',(-25.2,-66.1031295107175,-171.854014632589));
#140288=CARTESIAN_POINT('Ctrl Pts',(-25.2,-66.1031295063964,-171.725572055906));
#140289=CARTESIAN_POINT('Ctrl Pts',(-25.2,-66.0871173562522,-171.599865253241));
#140290=CARTESIAN_POINT('Ctrl Pts',(-25.2,-66.0541497294316,-171.477055409759));
#140291=CARTESIAN_POINT('Ctrl Pts',(-25.2,-66.0447396524368,-171.442001322026));
#140292=CARTESIAN_POINT('Ctrl Pts',(-25.2,-66.0339478541515,-171.407183310008));
#140293=CARTESIAN_POINT('Ctrl Pts',(-25.2,-66.0217516132152,-171.372605255459));
#140294=CARTESIAN_POINT('Ctrl Pts',(-25.2,-65.9940406295851,-171.294040728194));
#140295=CARTESIAN_POINT('Ctrl Pts',(-25.2,-65.9598967243513,-171.219005811917));
#140296=CARTESIAN_POINT('Ctrl Pts',(-25.2,-65.9193893860812,-171.147550497268));
#140297=CARTESIAN_POINT('Ctrl Pts',(-25.2,-65.8796084720189,-171.077376601556));
#140298=CARTESIAN_POINT('Ctrl Pts',(-25.2,-65.8336900811277,-171.010655009755));
#140299=CARTESIAN_POINT('Ctrl Pts',(-25.2,-65.7816577220592,-170.947457636992));
#140300=CARTESIAN_POINT('',(-25.2,-66.1031295107182,-171.799329694116));
#140301=CARTESIAN_POINT('Origin',(0.,-12.9675000200281,-61.64995));
#140302=CARTESIAN_POINT('',(-31.1074520910898,-62.0598503138784,-61.2273317382593));
#140303=CARTESIAN_POINT('',(-25.5011648721215,-65.1922357602732,-61.2273317382593));
#140304=CARTESIAN_POINT('Origin',(0.,-12.9675000200281,-61.2273317382593));
#140305=CARTESIAN_POINT('Origin',(-25.767032515919,-66.4122774533306,-61.8843165123376));
#140306=CARTESIAN_POINT('',(-31.35,-62.9782728042642,-60.64995));
#140307=CARTESIAN_POINT('Origin',(0.,-12.9675000200281,-60.64995));
#140308=CARTESIAN_POINT('Ctrl Pts',(-31.1074520910898,-62.0598503138784,
-61.2273317382593));
#140309=CARTESIAN_POINT('Ctrl Pts',(-31.1192593280084,-62.1041984096607,
-61.1334442002736));
#140310=CARTESIAN_POINT('Ctrl Pts',(-31.1342845229578,-62.1606836378221,
-61.0509981549565));
#140311=CARTESIAN_POINT('Ctrl Pts',(-31.1697097530512,-62.2941363459118,
-60.9056817830676));
#140312=CARTESIAN_POINT('Ctrl Pts',(-31.1896892584046,-62.369523292851,
-60.8449704353912));
#140313=CARTESIAN_POINT('Ctrl Pts',(-31.2539016024624,-62.6123775685824,
-60.6987791235328));
#140314=CARTESIAN_POINT('Ctrl Pts',(-31.3019361194217,-62.7947963971694,
-60.64995));
#140315=CARTESIAN_POINT('Ctrl Pts',(-31.35,-62.9782728042642,-60.64995));
#140316=CARTESIAN_POINT('Origin',(0.,-12.9675000200281,-60.64995));
#140317=CARTESIAN_POINT('',(-31.35,-12.9675000200281,-60.64995));
#140318=CARTESIAN_POINT('Ctrl Pts',(-31.3064221286262,-65.3602738277489,
-59.64995));
#140319=CARTESIAN_POINT('Ctrl Pts',(-31.8499999999999,-65.3127169262601,
-59.64995));
#140320=CARTESIAN_POINT('Ctrl Pts',(-31.85,-65.8583711767947,-59.64995));
#140321=CARTESIAN_POINT('Ctrl Pts',(-31.3064221286269,-65.3602738277488,
-59.7808732880376));
#140322=CARTESIAN_POINT('Ctrl Pts',(-31.8499999999999,-65.3127169262533,
-59.7746029379323));
#140323=CARTESIAN_POINT('Ctrl Pts',(-31.85,-65.8583711767784,-59.8463349320561));
#140324=CARTESIAN_POINT('Ctrl Pts',(-31.3075563441358,-65.3340478495507,
-59.9116978933073));
#140325=CARTESIAN_POINT('Ctrl Pts',(-31.8499999999999,-65.2892961879233,
-59.8989712332632));
#140326=CARTESIAN_POINT('Ctrl Pts',(-31.85,-65.819181055996,-60.0425718399612));
#140327=CARTESIAN_POINT('Ctrl Pts',(-31.3119222489988,-65.2330969061508,
-60.1535689714229));
#140328=CARTESIAN_POINT('Ctrl Pts',(-31.8499999999999,-65.1974676446973,
-60.1322291512615));
#140329=CARTESIAN_POINT('Ctrl Pts',(-31.85,-65.6683275916687,-60.4053784571341));
#140330=CARTESIAN_POINT('Ctrl Pts',(-31.3151522214972,-65.1584116390162,
-60.2644967268053));
#140331=CARTESIAN_POINT('Ctrl Pts',(-31.8499999999999,-65.1294009926956,
-60.2406767152616));
#140332=CARTESIAN_POINT('Ctrl Pts',(-31.85,-65.5567235699328,-60.5717700902076));
#140333=CARTESIAN_POINT('Ctrl Pts',(-31.3232193617865,-64.9718786181899,
-60.4496168355678));
#140334=CARTESIAN_POINT('Ctrl Pts',(-31.8499999999999,-64.9553741448238,
-60.4261994932778));
#140335=CARTESIAN_POINT('Ctrl Pts',(-31.85,-65.2779827136761,-60.8494502533521));
#140336=CARTESIAN_POINT('Ctrl Pts',(-31.3280533572402,-64.8601042170482,
-60.5237363920412));
#140337=CARTESIAN_POINT('Ctrl Pts',(-31.8499999999993,-64.8499435605403,
-60.5031527166052));
#140338=CARTESIAN_POINT('Ctrl Pts',(-31.85,-65.1109554916676,-60.9606295880612));
#140339=CARTESIAN_POINT('Ctrl Pts',(-31.3385935839747,-64.6163870802633,
-60.6239226729814));
#140340=CARTESIAN_POINT('Ctrl Pts',(-31.8500000000006,-64.6146765878316,
-60.6120353079394));
#140341=CARTESIAN_POINT('Ctrl Pts',(-31.85,-64.7467630120136,-61.1109090094727));
#140342=CARTESIAN_POINT('Ctrl Pts',(-31.3442946417934,-64.4845639684081,
-60.64995));
#140343=CARTESIAN_POINT('Ctrl Pts',(-31.85,-64.4853598419829,-60.6442102195366));
#140344=CARTESIAN_POINT('Ctrl Pts',(-31.85,-64.5497765111262,-61.149949999985));
#140345=CARTESIAN_POINT('Ctrl Pts',(-31.35,-64.3526414204797,-60.64995));
#140346=CARTESIAN_POINT('Ctrl Pts',(-31.8499999999999,-64.3526414204797,
-60.64995));
#140347=CARTESIAN_POINT('Ctrl Pts',(-31.85,-64.3526414204797,-61.14995));
#140348=CARTESIAN_POINT('',(-31.85,-64.3526414204797,-61.14995));
#140349=CARTESIAN_POINT('Origin',(-31.35,-64.3526414204797,-61.14995));
#140350=CARTESIAN_POINT('Ctrl Pts',(-31.85,-65.8583711767947,-59.64995));
#140351=CARTESIAN_POINT('Ctrl Pts',(-31.85,-65.8583711767784,-59.8463349320561));
#140352=CARTESIAN_POINT('Ctrl Pts',(-31.85,-65.819181055996,-60.0425718399612));
#140353=CARTESIAN_POINT('Ctrl Pts',(-31.85,-65.6683275916687,-60.4053784571341));
#140354=CARTESIAN_POINT('Ctrl Pts',(-31.85,-65.5567235699328,-60.5717700902076));
#140355=CARTESIAN_POINT('Ctrl Pts',(-31.85,-65.2779827136761,-60.8494502533521));
#140356=CARTESIAN_POINT('Ctrl Pts',(-31.85,-65.1109554916676,-60.9606295880612));
#140357=CARTESIAN_POINT('Ctrl Pts',(-31.85,-64.7467630120136,-61.1109090094727));
#140358=CARTESIAN_POINT('Ctrl Pts',(-31.85,-64.5497765111262,-61.149949999985));
#140359=CARTESIAN_POINT('Ctrl Pts',(-31.85,-64.3526414204797,-61.14995));
#140360=CARTESIAN_POINT('Origin',(-31.85,67.7009572055632,-55.24995));
#140361=CARTESIAN_POINT('',(-31.85,-70.08000002,-55.74995));
#140362=CARTESIAN_POINT('',(-31.85,67.7009572055632,-55.74995));
#140363=CARTESIAN_POINT('',(-31.85,-72.58000002,-58.24995));
#140364=CARTESIAN_POINT('Origin',(-31.85,-70.08000002,-58.24995));
#140365=CARTESIAN_POINT('',(-31.85,-72.58000002,-174.34995));
#140366=CARTESIAN_POINT('',(-31.85,-72.58000002,-58.24995));
#140367=CARTESIAN_POINT('',(-31.85,-70.08000002,-176.84995));
#140368=CARTESIAN_POINT('Origin',(-31.85,-70.08000002,-174.34995));
#140369=CARTESIAN_POINT('',(-31.85,-65.2735353570153,-176.84995));
#140370=CARTESIAN_POINT('',(-31.85,67.7009572055632,-176.84995));
#140371=CARTESIAN_POINT('',(-31.85,-65.2735353570153,-172.64995));
#140372=CARTESIAN_POINT('',(-31.85,-65.2735353570153,-55.24995));
#140373=CARTESIAN_POINT('',(-31.85,-63.7587939982373,-171.14995));
#140374=CARTESIAN_POINT('Ctrl Pts',(-31.85,-63.7587939982373,-171.14995));
#140375=CARTESIAN_POINT('Ctrl Pts',(-31.85,-63.9571089176128,-171.149950000016));
#140376=CARTESIAN_POINT('Ctrl Pts',(-31.85,-64.1552743575927,-171.18899099047));
#140377=CARTESIAN_POINT('Ctrl Pts',(-31.85,-64.521646483527,-171.339270411997));
#140378=CARTESIAN_POINT('Ctrl Pts',(-31.85,-64.6896733421684,-171.450449746589));
#140379=CARTESIAN_POINT('Ctrl Pts',(-31.85,-64.9700824273775,-171.728129909852));
#140380=CARTESIAN_POINT('Ctrl Pts',(-31.85,-65.0823543850191,-171.894521542842));
#140381=CARTESIAN_POINT('Ctrl Pts',(-31.85,-65.2341106883021,-172.257328160063));
#140382=CARTESIAN_POINT('Ctrl Pts',(-31.85,-65.273535357003,-172.453565067926));
#140383=CARTESIAN_POINT('Ctrl Pts',(-31.85,-65.2735353570153,-172.64995));
#140384=CARTESIAN_POINT('',(-31.85,-63.1109998882233,-171.14995));
#140385=CARTESIAN_POINT('',(-31.85,-63.6885235808861,-171.14995));
#140386=CARTESIAN_POINT('',(-31.85,-62.5757608260974,-170.861259130871));
#140387=CARTESIAN_POINT('Ctrl Pts',(-31.85,-62.5757608260974,-170.861259130871));
#140388=CARTESIAN_POINT('Ctrl Pts',(-31.85,-62.5934214847795,-170.893275292324));
#140389=CARTESIAN_POINT('Ctrl Pts',(-31.85,-62.6145900881586,-170.922872024471));
#140390=CARTESIAN_POINT('Ctrl Pts',(-31.85,-62.6386464997607,-170.949982960699));
#140391=CARTESIAN_POINT('Ctrl Pts',(-31.85,-62.6499713199276,-170.962745731906));
#140392=CARTESIAN_POINT('Ctrl Pts',(-31.85,-62.6619368642693,-170.974957283073));
#140393=CARTESIAN_POINT('Ctrl Pts',(-31.85,-62.6744818503514,-170.986608828398));
#140394=CARTESIAN_POINT('Ctrl Pts',(-31.85,-62.703885288123,-171.013918184157));
#140395=CARTESIAN_POINT('Ctrl Pts',(-31.85,-62.7356294724133,-171.037482725823));
#140396=CARTESIAN_POINT('Ctrl Pts',(-31.85,-62.7694892975011,-171.057780531265));
#140397=CARTESIAN_POINT('Ctrl Pts',(-31.85,-62.7808526179145,-171.064592452659));
#140398=CARTESIAN_POINT('Ctrl Pts',(-31.85,-62.7924544589391,-171.071036069574));
#140399=CARTESIAN_POINT('Ctrl Pts',(-31.85,-62.8042869861286,-171.077128390385));
#140400=CARTESIAN_POINT('Ctrl Pts',(-31.85,-62.8513324723594,-171.10135112744));
#140401=CARTESIAN_POINT('Ctrl Pts',(-31.85,-62.9022833426441,-171.119790824143));
#140402=CARTESIAN_POINT('Ctrl Pts',(-31.85,-62.9536152465698,-171.131828583671));
#140403=CARTESIAN_POINT('Ctrl Pts',(-31.85,-63.0049433927144,-171.143865461968));
#140404=CARTESIAN_POINT('Ctrl Pts',(-31.85,-63.0574025248319,-171.14995));
#140405=CARTESIAN_POINT('Ctrl Pts',(-31.85,-63.1109998882233,-171.14995));
#140406=CARTESIAN_POINT('',(-31.85,-56.2763252281792,-159.66866755714));
#140407=CARTESIAN_POINT('Ctrl Pts',(-31.85,-56.2763252281792,-159.66866755714));
#140408=CARTESIAN_POINT('Ctrl Pts',(-31.85,-58.4123038607033,-163.37917596697));
#140409=CARTESIAN_POINT('Ctrl Pts',(-31.85,-60.5078491316876,-167.112441157955));
#140410=CARTESIAN_POINT('Ctrl Pts',(-31.85,-62.5757608260974,-170.86125913087));
#140411=CARTESIAN_POINT('',(-31.85,-55.08000002,-154.831379798159));
#140412=CARTESIAN_POINT('Ctrl Pts',(-31.85,-55.08000002,-154.831379798159));
#140413=CARTESIAN_POINT('Ctrl Pts',(-31.85,-55.08000002,-155.253410854053));
#140414=CARTESIAN_POINT('Ctrl Pts',(-31.85,-55.1042084466772,-155.6729366979));
#140415=CARTESIAN_POINT('Ctrl Pts',(-31.85,-55.1523697302198,-156.089983777379));
#140416=CARTESIAN_POINT('Ctrl Pts',(-31.85,-55.2005310137623,-156.507030856859));
#140417=CARTESIAN_POINT('Ctrl Pts',(-31.85,-55.2730856890926,-156.92345630647));
#140418=CARTESIAN_POINT('Ctrl Pts',(-31.85,-55.3707143450195,-157.332589580255));
#140419=CARTESIAN_POINT('Ctrl Pts',(-31.85,-55.4683430009464,-157.74172285404));
#140420=CARTESIAN_POINT('Ctrl Pts',(-31.85,-55.5903137943579,-158.141820520543));
#140421=CARTESIAN_POINT('Ctrl Pts',(-31.85,-55.7395613131142,-158.531793284255));
#140422=CARTESIAN_POINT('Ctrl Pts',(-31.85,-55.8729496111693,-158.880327073445));
#140423=CARTESIAN_POINT('Ctrl Pts',(-31.85,-56.0279262451313,-159.220847442033));
#140424=CARTESIAN_POINT('Ctrl Pts',(-31.85,-56.2101595915589,-159.551250340992));
#140425=CARTESIAN_POINT('Ctrl Pts',(-31.85,-56.2318262512452,-159.590533640737));
#140426=CARTESIAN_POINT('Ctrl Pts',(-31.85,-56.2538782710724,-159.629673897819));
#140427=CARTESIAN_POINT('Ctrl Pts',(-31.85,-56.2763252281792,-159.668667557141));
#140428=CARTESIAN_POINT('',(-31.85,-55.08000002,-77.227263173365));
#140429=CARTESIAN_POINT('',(-31.85,-55.08000002,-155.433057559267));
#140430=CARTESIAN_POINT('',(-31.85,-56.2763252281792,-72.3899754143654));
#140431=CARTESIAN_POINT('Ctrl Pts',(-31.85,-56.2763252281792,-72.3899754143654));
#140432=CARTESIAN_POINT('Ctrl Pts',(-31.85,-56.0652560607924,-72.7566335394409));
#140433=CARTESIAN_POINT('Ctrl Pts',(-31.85,-55.8881616822718,-73.1379857966025));
#140434=CARTESIAN_POINT('Ctrl Pts',(-31.85,-55.737982230652,-73.5309787881812));
#140435=CARTESIAN_POINT('Ctrl Pts',(-31.85,-55.5878027790321,-73.9239717797599));
#140436=CARTESIAN_POINT('Ctrl Pts',(-31.85,-55.4647382249676,-74.3299545387688));
#140437=CARTESIAN_POINT('Ctrl Pts',(-31.85,-55.367968034963,-74.7375921331689));
#140438=CARTESIAN_POINT('Ctrl Pts',(-31.85,-55.2585018339702,-75.1987107776474));
#140439=CARTESIAN_POINT('Ctrl Pts',(-31.85,-55.1807511519297,-75.6645810411795));
#140440=CARTESIAN_POINT('Ctrl Pts',(-31.85,-55.1338484059997,-76.1350729813869));
#140441=CARTESIAN_POINT('Ctrl Pts',(-31.85,-55.0978253247023,-76.4964285710389));
#140442=CARTESIAN_POINT('Ctrl Pts',(-31.85,-55.0800000199994,-76.8605105831145));
#140443=CARTESIAN_POINT('Ctrl Pts',(-31.85,-55.08000002,-77.227263173365));
#140444=CARTESIAN_POINT('',(-31.85,-62.4426282692182,-61.4386408691297));
#140445=CARTESIAN_POINT('Ctrl Pts',(-31.85,-62.4426282692182,-61.4386408691297));
#140446=CARTESIAN_POINT('Ctrl Pts',(-31.85,-60.41789121461,-65.1063702600533));
#140447=CARTESIAN_POINT('Ctrl Pts',(-31.85,-58.3664753860175,-68.7590777918155));
#140448=CARTESIAN_POINT('Ctrl Pts',(-31.85,-56.2763252281792,-72.3899754143654));
#140449=CARTESIAN_POINT('',(-31.85,-62.9782728042642,-61.14995));
#140450=CARTESIAN_POINT('Ctrl Pts',(-31.85,-62.9782728042642,-61.14995));
#140451=CARTESIAN_POINT('Ctrl Pts',(-31.85,-62.9222361461974,-61.14995));
#140452=CARTESIAN_POINT('Ctrl Pts',(-31.85,-62.8664016141262,-61.1566668506656));
#140453=CARTESIAN_POINT('Ctrl Pts',(-31.85,-62.8123519766725,-61.1700628877868));
#140454=CARTESIAN_POINT('Ctrl Pts',(-31.85,-62.763267528681,-61.1822283179052));
#140455=CARTESIAN_POINT('Ctrl Pts',(-31.85,-62.7156536890974,-61.1999027909623));
#140456=CARTESIAN_POINT('Ctrl Pts',(-31.85,-62.6707013203275,-61.2230949953743));
#140457=CARTESIAN_POINT('Ctrl Pts',(-31.85,-62.6234720220053,-61.2474619324434));
#140458=CARTESIAN_POINT('Ctrl Pts',(-31.85,-62.5794710795978,-61.2778158553603));
#140459=CARTESIAN_POINT('Ctrl Pts',(-31.85,-62.5405071542091,-61.3141449414402));
#140460=CARTESIAN_POINT('Ctrl Pts',(-31.85,-62.5015487187516,-61.350468908832));
#140461=CARTESIAN_POINT('Ctrl Pts',(-31.85,-62.4685524875291,-61.3916801947947));
#140462=CARTESIAN_POINT('Ctrl Pts',(-31.85,-62.4426282692182,-61.4386408691297));
#140463=CARTESIAN_POINT('',(-31.85,67.7009572055632,-61.14995));
#140464=CARTESIAN_POINT('Origin',(-32.35,-73.08000002,-55.74995));
#140465=CARTESIAN_POINT('',(-32.35,-70.08000002,-55.24995));
#140466=CARTESIAN_POINT('',(-32.35,-73.08000002,-55.24995));
#140467=CARTESIAN_POINT('Origin',(-32.35,-70.08000002,-55.74995));
#140468=CARTESIAN_POINT('Origin',(-41.5,-73.08000002,-55.24995));
#140469=CARTESIAN_POINT('',(-32.85,-70.08000002,-55.24995));
#140470=CARTESIAN_POINT('',(-32.85,-73.08000002,-55.24995));
#140471=CARTESIAN_POINT('',(-41.5,-70.08000002,-55.24995));
#140472=CARTESIAN_POINT('Origin',(-32.85,67.7009572055632,-55.74995));
#140473=CARTESIAN_POINT('',(-33.35,-70.08000002,-55.74995));
#140474=CARTESIAN_POINT('',(-33.35,67.7009572055632,-55.74995));
#140475=CARTESIAN_POINT('Origin',(-32.85,-70.08000002,-55.74995));
#140476=CARTESIAN_POINT('Origin',(-33.35,67.7009572055632,-55.24995));
#140477=CARTESIAN_POINT('',(-33.35,-70.08000002,-176.84995));
#140478=CARTESIAN_POINT('',(-33.35,-64.9221832702593,-176.84995));
#140479=CARTESIAN_POINT('',(-33.35,67.7009572055632,-176.84995));
#140480=CARTESIAN_POINT('',(-33.35,-72.58000002,-174.34995));
#140481=CARTESIAN_POINT('Origin',(-33.35,-70.08000002,-174.34995));
#140482=CARTESIAN_POINT('',(-33.35,-72.58000002,-58.24995));
#140483=CARTESIAN_POINT('',(-33.35,-72.58000002,-174.34995));
#140484=CARTESIAN_POINT('Origin',(-33.35,-70.08000002,-58.24995));
#140485=CARTESIAN_POINT('',(-33.35,-61.3211699373828,-61.14995));
#140486=CARTESIAN_POINT('',(-33.35,67.7009572055632,-61.14995));
#140487=CARTESIAN_POINT('',(-33.35,-60.7669593817595,-61.4386408691297));
#140488=CARTESIAN_POINT('Ctrl Pts',(-33.35,-60.7669593817595,-61.4386408691297));
#140489=CARTESIAN_POINT('Ctrl Pts',(-33.35,-60.7854255655573,-61.4063230635265));
#140490=CARTESIAN_POINT('Ctrl Pts',(-33.35,-60.8074669942764,-61.3766005831693));
#140491=CARTESIAN_POINT('Ctrl Pts',(-33.35,-60.8323159282117,-61.349574172408));
#140492=CARTESIAN_POINT('Ctrl Pts',(-33.35,-60.8598479301244,-61.3196295802292));
#140493=CARTESIAN_POINT('Ctrl Pts',(-33.35,-60.8908254879513,-61.2929954345222));
#140494=CARTESIAN_POINT('Ctrl Pts',(-33.35,-60.9241484264025,-61.2697698227383));
#140495=CARTESIAN_POINT('Ctrl Pts',(-33.35,-60.9500168068528,-61.2517399313259));
#140496=CARTESIAN_POINT('Ctrl Pts',(-33.35,-60.9772970763435,-61.2357633244769));
#140497=CARTESIAN_POINT('Ctrl Pts',(-33.35,-61.0054624679791,-61.2218683128494));
#140498=CARTESIAN_POINT('Ctrl Pts',(-33.35,-61.0316582964252,-61.2089449583455));
#140499=CARTESIAN_POINT('Ctrl Pts',(-33.35,-61.0586931044519,-61.1978139207404));
#140500=CARTESIAN_POINT('Ctrl Pts',(-33.35,-61.0863521110361,-61.1884108897488));
#140501=CARTESIAN_POINT('Ctrl Pts',(-33.35,-61.1146264284013,-61.1787986760331));
#140502=CARTESIAN_POINT('Ctrl Pts',(-33.35,-61.1435543947086,-61.1709920371076));
#140503=CARTESIAN_POINT('Ctrl Pts',(-33.35,-61.1729286914005,-61.1649732421567));
#140504=CARTESIAN_POINT('Ctrl Pts',(-33.35,-61.2017965294041,-61.1590582206179));
#140505=CARTESIAN_POINT('Ctrl Pts',(-33.35,-61.2310968493206,-61.1548700235783));
#140506=CARTESIAN_POINT('Ctrl Pts',(-33.35,-61.2606330881675,-61.1524405238988));
#140507=CARTESIAN_POINT('Ctrl Pts',(-33.35,-61.2807251508685,-61.1507878537622));
#140508=CARTESIAN_POINT('Ctrl Pts',(-33.35,-61.3009263849488,-61.14995));
#140509=CARTESIAN_POINT('Ctrl Pts',(-33.35,-61.3211699373828,-61.14995));
#140510=CARTESIAN_POINT('',(-33.35,-56.3642045114132,-69.0177323827589));
#140511=CARTESIAN_POINT('Ctrl Pts',(-33.35,-56.3642045114132,-69.0177323827589));
#140512=CARTESIAN_POINT('Ctrl Pts',(-33.35,-57.8514954063616,-66.5028158819518));
#140513=CARTESIAN_POINT('Ctrl Pts',(-33.35,-59.3174212852614,-63.975488272466));
#140514=CARTESIAN_POINT('Ctrl Pts',(-33.35,-60.7669593817595,-61.4386408691297));
#140515=CARTESIAN_POINT('',(-33.35,-55.08000002,-74.155095361993));
#140516=CARTESIAN_POINT('Ctrl Pts',(-33.35,-55.08000002,-74.155095361993));
#140517=CARTESIAN_POINT('Ctrl Pts',(-33.35,-55.0800000199996,-73.9307666441726));
#140518=CARTESIAN_POINT('Ctrl Pts',(-33.35,-55.0863156531016,-73.7071338026571));
#140519=CARTESIAN_POINT('Ctrl Pts',(-33.35,-55.099013419779,-73.4842001164092));
#140520=CARTESIAN_POINT('Ctrl Pts',(-33.35,-55.1117111864564,-73.2612664301613));
#140521=CARTESIAN_POINT('Ctrl Pts',(-33.35,-55.1307909278358,-73.0390315071252));
#140522=CARTESIAN_POINT('Ctrl Pts',(-33.35,-55.1563760274665,-72.8175000855932));
#140523=CARTESIAN_POINT('Ctrl Pts',(-33.35,-55.1806216024912,-72.6075670863636));
#140524=CARTESIAN_POINT('Ctrl Pts',(-33.35,-55.210750014218,-72.3979880684058));
#140525=CARTESIAN_POINT('Ctrl Pts',(-33.35,-55.2468600350687,-72.1892231805709));
#140526=CARTESIAN_POINT('Ctrl Pts',(-33.35,-55.2824608236509,-71.9834023457969));
#140527=CARTESIAN_POINT('Ctrl Pts',(-33.35,-55.3238757306228,-71.7783731405196));
#140528=CARTESIAN_POINT('Ctrl Pts',(-33.35,-55.3711489449082,-71.5745698720716));
#140529=CARTESIAN_POINT('Ctrl Pts',(-33.35,-55.3771233770109,-71.5488130284117));
#140530=CARTESIAN_POINT('Ctrl Pts',(-33.35,-55.3831913115131,-71.5230757533204));
#140531=CARTESIAN_POINT('Ctrl Pts',(-33.35,-55.3893527788883,-71.4973589120773));
#140532=CARTESIAN_POINT('Ctrl Pts',(-33.35,-55.49371790368,-71.061757912807));
#140533=CARTESIAN_POINT('Ctrl Pts',(-33.35,-55.62429768467,-70.6362303826932));
#140534=CARTESIAN_POINT('Ctrl Pts',(-33.35,-55.7846973533805,-70.2221616988514));
#140535=CARTESIAN_POINT('Ctrl Pts',(-33.35,-55.9170285274408,-69.8805512983134));
#140536=CARTESIAN_POINT('Ctrl Pts',(-33.35,-56.0694235888807,-69.5466508245293));
#140537=CARTESIAN_POINT('Ctrl Pts',(-33.35,-56.2474267877794,-69.2225907454076));
#140538=CARTESIAN_POINT('Ctrl Pts',(-33.35,-56.2851826821973,-69.1538550248807));
#140539=CARTESIAN_POINT('Ctrl Pts',(-33.35,-56.3240908525374,-69.0855620877321));
#140540=CARTESIAN_POINT('Ctrl Pts',(-33.35,-56.3642045114132,-69.0177323827589));
#140541=CARTESIAN_POINT('',(-33.35,-55.08000002,-157.903547609535));
#140542=CARTESIAN_POINT('',(-33.35,-55.08000002,-74.7820934264633));
#140543=CARTESIAN_POINT('',(-33.35,-56.3642045114216,-163.040910588762));
#140544=CARTESIAN_POINT('Ctrl Pts',(-33.35,-56.3642045114216,-163.040910588761));
#140545=CARTESIAN_POINT('Ctrl Pts',(-33.35,-56.15744649645,-162.69129563093));
#140546=CARTESIAN_POINT('Ctrl Pts',(-33.35,-55.9820013313226,-162.328090330091));
#140547=CARTESIAN_POINT('Ctrl Pts',(-33.35,-55.8312183864901,-161.954181181917));
#140548=CARTESIAN_POINT('Ctrl Pts',(-33.35,-55.8149691191711,-161.913886507288));
#140549=CARTESIAN_POINT('Ctrl Pts',(-33.35,-55.7990063112135,-161.873467504085));
#140550=CARTESIAN_POINT('Ctrl Pts',(-33.35,-55.7833216689026,-161.832927771927));
#140551=CARTESIAN_POINT('Ctrl Pts',(-33.35,-55.6220934454647,-161.4162049124));
#140552=CARTESIAN_POINT('Ctrl Pts',(-33.35,-55.4903395808871,-160.984647645305));
#140553=CARTESIAN_POINT('Ctrl Pts',(-33.35,-55.3869054679322,-160.551047169605));
#140554=CARTESIAN_POINT('Ctrl Pts',(-33.35,-55.2731785652171,-160.074298854097));
#140555=CARTESIAN_POINT('Ctrl Pts',(-33.35,-55.1917492545593,-159.592825164627));
#140556=CARTESIAN_POINT('Ctrl Pts',(-33.35,-55.1414674766992,-159.106794321394));
#140557=CARTESIAN_POINT('Ctrl Pts',(-33.35,-55.1002871472375,-158.708739377742));
#140558=CARTESIAN_POINT('Ctrl Pts',(-33.35,-55.08000002,-158.307627565795));
#140559=CARTESIAN_POINT('Ctrl Pts',(-33.35,-55.08000002,-157.903547609535));
#140560=CARTESIAN_POINT('',(-33.35,-60.9047458754482,-170.861259130871));
#140561=CARTESIAN_POINT('Ctrl Pts',(-33.35,-60.9047458754482,-170.861259130871));
#140562=CARTESIAN_POINT('Ctrl Pts',(-33.35,-59.4103419837617,-168.243380962845));
#140563=CARTESIAN_POINT('Ctrl Pts',(-33.35,-57.8986402212887,-165.635546042559));
#140564=CARTESIAN_POINT('Ctrl Pts',(-33.35,-56.3642045114219,-163.040910588762));
#140565=CARTESIAN_POINT('',(-33.35,-61.4584329769396,-171.14995));
#140566=CARTESIAN_POINT('Ctrl Pts',(-33.35,-61.4584329769396,-171.14995));
#140567=CARTESIAN_POINT('Ctrl Pts',(-33.35,-61.3933512658327,-171.14995));
#140568=CARTESIAN_POINT('Ctrl Pts',(-33.35,-61.3285261814765,-171.141518537402));
#140569=CARTESIAN_POINT('Ctrl Pts',(-33.35,-61.2661398376586,-171.124539608288));
#140570=CARTESIAN_POINT('Ctrl Pts',(-33.35,-61.2235444953616,-171.112946954301));
#140571=CARTESIAN_POINT('Ctrl Pts',(-33.35,-61.1820855819977,-171.09736868316));
#140572=CARTESIAN_POINT('Ctrl Pts',(-33.35,-61.1424600695407,-171.077754003862));
#140573=CARTESIAN_POINT('Ctrl Pts',(-33.35,-61.107639036433,-171.06051754798));
#140574=CARTESIAN_POINT('Ctrl Pts',(-33.35,-61.0743836755045,-171.040165282673));
#140575=CARTESIAN_POINT('Ctrl Pts',(-33.35,-61.0435144499431,-171.016803427716));
#140576=CARTESIAN_POINT('Ctrl Pts',(-33.35,-61.0154640589469,-170.995574869045));
#140577=CARTESIAN_POINT('Ctrl Pts',(-33.35,-60.9893827952823,-170.971860522156));
#140578=CARTESIAN_POINT('Ctrl Pts',(-33.35,-60.9659114268331,-170.945708806781));
#140579=CARTESIAN_POINT('Ctrl Pts',(-33.35,-60.9427675971716,-170.91992203396));
#140580=CARTESIAN_POINT('Ctrl Pts',(-33.35,-60.9221601342065,-170.891765212974));
#140581=CARTESIAN_POINT('Ctrl Pts',(-33.35,-60.9047458754482,-170.861259130871));
#140582=CARTESIAN_POINT('',(-33.35,-63.4074419114814,-171.14995));
#140583=CARTESIAN_POINT('',(-33.35,-61.8036605881122,-171.14995));
#140584=CARTESIAN_POINT('',(-33.35,-64.9221832702593,-172.64995));
#140585=CARTESIAN_POINT('Ctrl Pts',(-33.35,-64.9221832702593,-172.64995));
#140586=CARTESIAN_POINT('Ctrl Pts',(-33.35,-64.922183270247,-172.453565067926));
#140587=CARTESIAN_POINT('Ctrl Pts',(-33.35,-64.8827586015461,-172.257328160063));
#140588=CARTESIAN_POINT('Ctrl Pts',(-33.35,-64.7310022982632,-171.894521542842));
#140589=CARTESIAN_POINT('Ctrl Pts',(-33.35,-64.6187303406215,-171.728129909852));
#140590=CARTESIAN_POINT('Ctrl Pts',(-33.35,-64.3383212554124,-171.450449746589));
#140591=CARTESIAN_POINT('Ctrl Pts',(-33.35,-64.1702943967697,-171.339270411997));
#140592=CARTESIAN_POINT('Ctrl Pts',(-33.35,-63.8039222708381,-171.18899099047));
#140593=CARTESIAN_POINT('Ctrl Pts',(-33.35,-63.6057568308558,-171.149950000016));
#140594=CARTESIAN_POINT('Ctrl Pts',(-33.35,-63.4074419114814,-171.14995));
#140595=CARTESIAN_POINT('',(-33.35,-64.9221832702593,-55.24995));
#140596=CARTESIAN_POINT('Origin',(0.,-12.9675000200281,-60.64995));
#140597=CARTESIAN_POINT('',(-37.,33.02054075664,-60.64995));
#140598=CARTESIAN_POINT('',(-31.,37.2609769076718,-60.64995));
#140599=CARTESIAN_POINT('Origin',(0.,-12.9675000200281,-60.64995));
#140600=CARTESIAN_POINT('',(-37.,-12.9675000200281,-60.64995));
#140601=CARTESIAN_POINT('',(-31.,-12.9675000200281,-60.64995));
#140602=CARTESIAN_POINT('Ctrl Pts',(-30.9564221286262,39.4558948199267,
-59.64995));
#140603=CARTESIAN_POINT('Ctrl Pts',(-30.5,39.4958265819639,-59.64995));
#140604=CARTESIAN_POINT('Ctrl Pts',(-30.5,39.9539921689726,-59.64995));
#140605=CARTESIAN_POINT('Ctrl Pts',(-30.9564221286278,39.4558948199266,
-59.7808732880376));
#140606=CARTESIAN_POINT('Ctrl Pts',(-30.5,39.4958265819509,-59.7861314644993));
#140607=CARTESIAN_POINT('Ctrl Pts',(-30.5,39.9539921689583,-59.8463349320561));
#140608=CARTESIAN_POINT('Ctrl Pts',(-30.9575563441362,39.4296688417285,
-59.9116978933072));
#140609=CARTESIAN_POINT('Ctrl Pts',(-30.4999999999997,39.4674332340768,
-59.9224177216067));
#140610=CARTESIAN_POINT('Ctrl Pts',(-30.5,39.9148020481738,-60.0425718399611));
#140611=CARTESIAN_POINT('Ctrl Pts',(-30.9619222489984,39.3287178983286,
-60.153568971423));
#140612=CARTESIAN_POINT('Ctrl Pts',(-30.5000000000003,39.3593214179772,
-60.1718710142636));
#140613=CARTESIAN_POINT('Ctrl Pts',(-30.5,39.7639485838465,-60.4053784571342));
#140614=CARTESIAN_POINT('Ctrl Pts',(-30.9651522214976,39.2540326311941,
-60.2644967268053));
#140615=CARTESIAN_POINT('Ctrl Pts',(-30.5000000000001,39.2793032864295,
-60.2852157712117));
#140616=CARTESIAN_POINT('Ctrl Pts',(-30.5,39.65234456211,-60.5717700902076));
#140617=CARTESIAN_POINT('Ctrl Pts',(-30.9732193617862,39.0674996103677,
-60.4496168355678));
#140618=CARTESIAN_POINT('Ctrl Pts',(-30.5,39.0823726723643,-60.4706504746469));
#140619=CARTESIAN_POINT('Ctrl Pts',(-30.5,39.3736037058546,-60.8494502533521));
#140620=CARTESIAN_POINT('Ctrl Pts',(-30.9780533572398,38.9557252092273,
-60.5237363920407));
#140621=CARTESIAN_POINT('Ctrl Pts',(-30.5,38.9650655890091,-60.5426326522477));
#140622=CARTESIAN_POINT('Ctrl Pts',(-30.5,39.206576483846,-60.9606295880612));
#140623=CARTESIAN_POINT('Ctrl Pts',(-30.9885935839752,38.71200807244,-60.6239226729818));
#140624=CARTESIAN_POINT('Ctrl Pts',(-30.5,38.7136903701654,-60.6353187454024));
#140625=CARTESIAN_POINT('Ctrl Pts',(-30.5,38.8423840041908,-61.1109090094727));
#140626=CARTESIAN_POINT('Ctrl Pts',(-30.994294641792,38.5801849605867,-60.64995));
#140627=CARTESIAN_POINT('Ctrl Pts',(-30.4999999999973,38.5794088824901,
-60.655621796981));
#140628=CARTESIAN_POINT('Ctrl Pts',(-30.5,38.6453975033045,-61.149949999985));
#140629=CARTESIAN_POINT('Ctrl Pts',(-31.,38.4482624126576,-60.64995));
#140630=CARTESIAN_POINT('Ctrl Pts',(-30.5,38.4482624126575,-60.64995));
#140631=CARTESIAN_POINT('Ctrl Pts',(-30.5,38.4482624126576,-61.14995));
#140632=CARTESIAN_POINT('',(-30.5,38.4482624126576,-61.14995));
#140633=CARTESIAN_POINT('Ctrl Pts',(-30.5,39.9539921689726,-59.64995));
#140634=CARTESIAN_POINT('Ctrl Pts',(-30.5,39.9539921689583,-59.8463349320561));
#140635=CARTESIAN_POINT('Ctrl Pts',(-30.5,39.9148020481738,-60.0425718399611));
#140636=CARTESIAN_POINT('Ctrl Pts',(-30.5,39.7639485838465,-60.4053784571342));
#140637=CARTESIAN_POINT('Ctrl Pts',(-30.5,39.65234456211,-60.5717700902076));
#140638=CARTESIAN_POINT('Ctrl Pts',(-30.5,39.3736037058546,-60.8494502533521));
#140639=CARTESIAN_POINT('Ctrl Pts',(-30.5,39.206576483846,-60.9606295880612));
#140640=CARTESIAN_POINT('Ctrl Pts',(-30.5,38.8423840041908,-61.1109090094727));
#140641=CARTESIAN_POINT('Ctrl Pts',(-30.5,38.6453975033045,-61.149949999985));
#140642=CARTESIAN_POINT('Ctrl Pts',(-30.5,38.4482624126576,-61.14995));
#140643=CARTESIAN_POINT('Origin',(-31.,38.4482624126576,-61.14995));
#140644=CARTESIAN_POINT('Ctrl Pts',(-37.,37.923330431502,-60.64995));
#140645=CARTESIAN_POINT('Ctrl Pts',(-37.5,37.923330431502,-60.64995));
#140646=CARTESIAN_POINT('Ctrl Pts',(-37.5,37.923330431502,-61.14995));
#140647=CARTESIAN_POINT('Ctrl Pts',(-36.9942946417934,38.0552529794313,
-60.64995));
#140648=CARTESIAN_POINT('Ctrl Pts',(-37.5000000000028,38.0560488530063,
-60.6442102195364));
#140649=CARTESIAN_POINT('Ctrl Pts',(-37.5,38.1204655221491,-61.149949999985));
#140650=CARTESIAN_POINT('Ctrl Pts',(-36.9885935839748,38.1870760912844,
-60.6239226729819));
#140651=CARTESIAN_POINT('Ctrl Pts',(-37.5,38.1853655988526,-60.6120353079393));
#140652=CARTESIAN_POINT('Ctrl Pts',(-37.5,38.3174520230353,-61.1109090094727));
#140653=CARTESIAN_POINT('Ctrl Pts',(-36.9780533572402,38.4307932280718,
-60.5237363920407));
#140654=CARTESIAN_POINT('Ctrl Pts',(-37.5,38.4206325715641,-60.5031527166052));
#140655=CARTESIAN_POINT('Ctrl Pts',(-37.5,38.6816445026906,-60.9606295880611));
#140656=CARTESIAN_POINT('Ctrl Pts',(-36.9732193617859,38.5425676292119,
-60.4496168355682));
#140657=CARTESIAN_POINT('Ctrl Pts',(-37.4999999999993,38.5260631558441,
-60.4261994932771));
#140658=CARTESIAN_POINT('Ctrl Pts',(-37.5,38.8486717246983,-60.8494502533514));
#140659=CARTESIAN_POINT('Ctrl Pts',(-36.9651522214979,38.7291006500388,
-60.2644967268049));
#140660=CARTESIAN_POINT('Ctrl Pts',(-37.5000000000007,38.70009000372,-60.2406767152623));
#140661=CARTESIAN_POINT('Ctrl Pts',(-37.5,39.1274125809551,-60.5717700902082));
#140662=CARTESIAN_POINT('Ctrl Pts',(-36.9619222489981,38.8037859171731,
-60.153568971423));
#140663=CARTESIAN_POINT('Ctrl Pts',(-37.4999999999994,38.768156655719,-60.1322291512603));
#140664=CARTESIAN_POINT('Ctrl Pts',(-37.5,39.239016602691,-60.4053784571342));
#140665=CARTESIAN_POINT('Ctrl Pts',(-36.9575563441365,38.904736860573,-59.9116978933072));
#140666=CARTESIAN_POINT('Ctrl Pts',(-37.5000000000007,38.8599851989463,
-59.8989712332646));
#140667=CARTESIAN_POINT('Ctrl Pts',(-37.5,39.3898700670183,-60.0425718399611));
#140668=CARTESIAN_POINT('Ctrl Pts',(-36.9564221286271,38.9309628387711,
-59.7808732880376));
#140669=CARTESIAN_POINT('Ctrl Pts',(-37.5,38.8834059372763,-59.7746029379313));
#140670=CARTESIAN_POINT('Ctrl Pts',(-37.5,39.4290601878028,-59.8463349320561));
#140671=CARTESIAN_POINT('Ctrl Pts',(-36.9564221286262,38.9309628387712,
-59.64995));
#140672=CARTESIAN_POINT('Ctrl Pts',(-37.5,38.8834059372825,-59.64995));
#140673=CARTESIAN_POINT('Ctrl Pts',(-37.5,39.4290601878171,-59.64995));
#140674=CARTESIAN_POINT('',(-37.5,37.923330431502,-61.14995));
#140675=CARTESIAN_POINT('Origin',(-37.,37.923330431502,-61.14995));
#140676=CARTESIAN_POINT('Ctrl Pts',(-37.5,37.923330431502,-61.14995));
#140677=CARTESIAN_POINT('Ctrl Pts',(-37.5,38.1204655221491,-61.149949999985));
#140678=CARTESIAN_POINT('Ctrl Pts',(-37.5,38.3174520230353,-61.1109090094727));
#140679=CARTESIAN_POINT('Ctrl Pts',(-37.5,38.6816445026906,-60.9606295880611));
#140680=CARTESIAN_POINT('Ctrl Pts',(-37.5,38.8486717246983,-60.8494502533514));
#140681=CARTESIAN_POINT('Ctrl Pts',(-37.5,39.1274125809551,-60.5717700902082));
#140682=CARTESIAN_POINT('Ctrl Pts',(-37.5,39.239016602691,-60.4053784571342));
#140683=CARTESIAN_POINT('Ctrl Pts',(-37.5,39.3898700670183,-60.0425718399611));
#140684=CARTESIAN_POINT('Ctrl Pts',(-37.5,39.4290601878028,-59.8463349320561));
#140685=CARTESIAN_POINT('Ctrl Pts',(-37.5,39.4290601878171,-59.64995));
#140686=CARTESIAN_POINT('Origin',(-30.5,-9.33460238845303,-92.34995));
#140687=CARTESIAN_POINT('',(-30.5,43.91999998,-55.74995));
#140688=CARTESIAN_POINT('',(-30.5,39.4958265819638,-55.74995));
#140689=CARTESIAN_POINT('',(-30.5,46.41999998,-58.24995));
#140690=CARTESIAN_POINT('Origin',(-30.5,43.91999998,-58.24995));
#140691=CARTESIAN_POINT('',(-30.5,46.41999998,-58.24995));
#140692=CARTESIAN_POINT('',(-30.5,28.91999998,-91.34995));
#140693=CARTESIAN_POINT('Origin',(-30.5,29.41999998,-91.34995));
#140694=CARTESIAN_POINT('',(-30.5,28.91999998,-78.0460091084363));
#140695=CARTESIAN_POINT('',(-30.5,28.91999998,-91.34995));
#140696=CARTESIAN_POINT('',(-30.5,30.1096831288108,-73.2320455176344));
#140697=CARTESIAN_POINT('Ctrl Pts',(-30.5,30.1096831288108,-73.2320455176344));
#140698=CARTESIAN_POINT('Ctrl Pts',(-30.5,29.8999686314803,-73.5970828192481));
#140699=CARTESIAN_POINT('Ctrl Pts',(-30.5,29.7239010511178,-73.976669190304));
#140700=CARTESIAN_POINT('Ctrl Pts',(-30.5,29.5745597864535,-74.3678121335876));
#140701=CARTESIAN_POINT('Ctrl Pts',(-30.5,29.4252185217892,-74.7589550768711));
#140702=CARTESIAN_POINT('Ctrl Pts',(-30.5,29.3028136262495,-75.1629449137757));
#140703=CARTESIAN_POINT('Ctrl Pts',(-30.5,29.2065461283391,-75.5685697596184));
#140704=CARTESIAN_POINT('Ctrl Pts',(-30.5,29.0974180990884,-76.0283826871663));
#140705=CARTESIAN_POINT('Ctrl Pts',(-30.5,29.0199506911356,-76.4929481091058));
#140706=CARTESIAN_POINT('Ctrl Pts',(-30.5,28.9733024240056,-76.9621397516273));
#140707=CARTESIAN_POINT('Ctrl Pts',(-30.5,28.9376489765478,-77.3207447031833));
#140708=CARTESIAN_POINT('Ctrl Pts',(-30.5,28.91999998,-77.6820522875113));
#140709=CARTESIAN_POINT('Ctrl Pts',(-30.5,28.91999998,-78.0460091084363));
#140710=CARTESIAN_POINT('',(-30.5,36.7276789742547,-61.4386408691296));
#140711=CARTESIAN_POINT('Ctrl Pts',(-30.5,36.7276789742547,-61.4386408691296));
#140712=CARTESIAN_POINT('Ctrl Pts',(-30.5,34.5564250420216,-65.3892731044285));
#140713=CARTESIAN_POINT('Ctrl Pts',(-30.5,32.355340677558,-69.3231656718822));
#140714=CARTESIAN_POINT('Ctrl Pts',(-30.5,30.1096831288108,-73.2320455176344));
#140715=CARTESIAN_POINT('',(-30.5,37.2609769076718,-61.14995));
#140716=CARTESIAN_POINT('Ctrl Pts',(-30.5,37.2609769076718,-61.14995));
#140717=CARTESIAN_POINT('Ctrl Pts',(-30.5,37.2057964810295,-61.14995));
#140718=CARTESIAN_POINT('Ctrl Pts',(-30.5,37.1508139868679,-61.1565255904659));
#140719=CARTESIAN_POINT('Ctrl Pts',(-30.5,37.0975659565504,-61.1696247206415));
#140720=CARTESIAN_POINT('Ctrl Pts',(-30.5,37.0479567714751,-61.1818286870479));
#140721=CARTESIAN_POINT('Ctrl Pts',(-30.5,36.9998515275003,-61.199695577265));
#140722=CARTESIAN_POINT('Ctrl Pts',(-30.5,36.9544986327132,-61.223223625875));
#140723=CARTESIAN_POINT('Ctrl Pts',(-30.5,36.9220640062061,-61.2400499711985));
#140724=CARTESIAN_POINT('Ctrl Pts',(-30.5,36.8911731746044,-61.2597722334507));
#140725=CARTESIAN_POINT('Ctrl Pts',(-30.5,36.8624864317523,-61.2822151380555));
#140726=CARTESIAN_POINT('Ctrl Pts',(-30.5,36.8352464003271,-61.3035262164814));
#140727=CARTESIAN_POINT('Ctrl Pts',(-30.5,36.8099924249354,-61.3272911886642));
#140728=CARTESIAN_POINT('Ctrl Pts',(-30.5,36.7873187400316,-61.3533954059167));
#140729=CARTESIAN_POINT('Ctrl Pts',(-30.5,36.7660341218411,-61.3779003904282));
#140730=CARTESIAN_POINT('Ctrl Pts',(-30.5,36.7470225594144,-61.4044673363619));
#140731=CARTESIAN_POINT('Ctrl Pts',(-30.5,36.730815934666,-61.4330244036176));
#140732=CARTESIAN_POINT('Ctrl Pts',(-30.5,36.7297582655658,-61.4348880814715));
#140733=CARTESIAN_POINT('Ctrl Pts',(-30.5,36.728712560285,-61.4367602423504));
#140734=CARTESIAN_POINT('Ctrl Pts',(-30.5,36.7276789742547,-61.4386408691296));
#140735=CARTESIAN_POINT('',(-30.5,-9.33460238845303,-61.14995));
#140736=CARTESIAN_POINT('Origin',(-30.,0.,-55.74995));
#140737=CARTESIAN_POINT('',(-30.,43.91999998,-55.24995));
#140738=CARTESIAN_POINT('',(-30.,43.91999998,-55.24995));
#140739=CARTESIAN_POINT('Origin',(-30.,43.91999998,-55.74995));
#140740=CARTESIAN_POINT('Origin',(0.,0.,-55.24995));
#140741=CARTESIAN_POINT('',(-29.5,43.91999998,-55.24995));
#140742=CARTESIAN_POINT('',(-29.5,39.6270595772528,-55.24995));
#140743=CARTESIAN_POINT('',(0.,43.91999998,-55.24995));
#140744=CARTESIAN_POINT('Origin',(-29.5,-9.33460238845303,-55.74995));
#140745=CARTESIAN_POINT('',(-29.,43.91999998,-55.74995));
#140746=CARTESIAN_POINT('',(-29.,43.91999998,-55.74995));
#140747=CARTESIAN_POINT('Origin',(-29.5,43.91999998,-55.74995));
#140748=CARTESIAN_POINT('Origin',(-29.,-9.33460238845303,-92.34995));
#140749=CARTESIAN_POINT('',(-29.,38.7048160259599,-61.150138786574));
#140750=CARTESIAN_POINT('Ctrl Pts',(-29.,38.7048160259599,-61.150138786574));
#140751=CARTESIAN_POINT('Ctrl Pts',(-29.,38.7587438294333,-61.1488407776134));
#140752=CARTESIAN_POINT('Ctrl Pts',(-29.0000000000001,38.8125135208643,
-61.1445744929232));
#140753=CARTESIAN_POINT('Ctrl Pts',(-28.9999999999995,38.86581213546,-61.1374999313473));
#140754=CARTESIAN_POINT('Ctrl Pts',(-28.999999999999,38.9206199981767,-61.1302250405725));
#140755=CARTESIAN_POINT('Ctrl Pts',(-28.9999999999976,38.9749308760979,
-61.1199805166188));
#140756=CARTESIAN_POINT('Ctrl Pts',(-28.9999999999961,39.0284204191823,
-61.106886234665));
#140757=CARTESIAN_POINT('Ctrl Pts',(-28.9999999999946,39.0824266406301,
-61.0936654694441));
#140758=CARTESIAN_POINT('Ctrl Pts',(-28.9999999999932,39.135596867869,-61.0775394193));
#140759=CARTESIAN_POINT('Ctrl Pts',(-28.9999999999937,39.1875946577402,
-61.058579376025));
#140760=CARTESIAN_POINT('Ctrl Pts',(-28.999999999994,39.214574559218,-61.04874164829));
#140761=CARTESIAN_POINT('Ctrl Pts',(-28.9999999999949,39.2412386526437,
-61.0381401159529));
#140762=CARTESIAN_POINT('Ctrl Pts',(-28.999999999996,39.2675379042626,-61.0267795633669));
#140763=CARTESIAN_POINT('Ctrl Pts',(-28.999999999996,39.2679181300168,-61.02661531631));
#140764=CARTESIAN_POINT('Ctrl Pts',(-28.9999999999961,39.268298302465,-61.026450901664));
#140765=CARTESIAN_POINT('Ctrl Pts',(-28.9999999999961,39.268678421493,-61.0262863194886));
#140766=CARTESIAN_POINT('Ctrl Pts',(-29.0000000000039,39.4448840602191,
-60.9499936185261));
#140767=CARTESIAN_POINT('Ctrl Pts',(-29.,39.6087415856579,-60.8380654560188));
#140768=CARTESIAN_POINT('Ctrl Pts',(-29.,39.7446514854509,-60.6995134053984));
#140769=CARTESIAN_POINT('Ctrl Pts',(-29.,39.7447518137561,-60.6994111266649));
#140770=CARTESIAN_POINT('Ctrl Pts',(-29.,39.744852125437,-60.6993088358292));
#140771=CARTESIAN_POINT('Ctrl Pts',(-29.,39.7449524204946,-60.6992065328918));
#140772=CARTESIAN_POINT('Ctrl Pts',(-28.9999999999999,39.812931097784,-60.6298669408688));
#140773=CARTESIAN_POINT('Ctrl Pts',(-29.,39.8732750955302,-60.554966232983));
#140774=CARTESIAN_POINT('Ctrl Pts',(-29.,39.9261853767363,-60.4746513000797));
#140775=CARTESIAN_POINT('Ctrl Pts',(-29.,39.9261884127568,-60.4746466915656));
#140776=CARTESIAN_POINT('Ctrl Pts',(-29.,39.9261914487538,-60.4746420830303));
#140777=CARTESIAN_POINT('Ctrl Pts',(-29.,39.9261944847274,-60.4746374744739));
#140778=CARTESIAN_POINT('Ctrl Pts',(-29.,39.9791069872138,-60.3943171935884));
#140779=CARTESIAN_POINT('Ctrl Pts',(-29.0000000000001,40.0249202649622,
-60.3075521828599));
#140780=CARTESIAN_POINT('Ctrl Pts',(-28.9999999999999,40.0614666645048,
-60.2182183202257));
#140781=CARTESIAN_POINT('Ctrl Pts',(-28.9999999999999,40.0615163877946,
-60.218096776829));
#140782=CARTESIAN_POINT('Ctrl Pts',(-28.9999999999999,40.0615660940304,
-60.2179752284374));
#140783=CARTESIAN_POINT('Ctrl Pts',(-28.9999999999999,40.0616157832065,
-60.2178536750606));
#140784=CARTESIAN_POINT('Ctrl Pts',(-28.9999999999996,40.0995205469999,
-60.1251282086843));
#140785=CARTESIAN_POINT('Ctrl Pts',(-28.9999999999997,40.1280273344111,
-60.0287688634752));
#140786=CARTESIAN_POINT('Ctrl Pts',(-28.9999999999998,40.1466650082864,
-59.9302710126536));
#140787=CARTESIAN_POINT('Ctrl Pts',(-29.,40.1639177847726,-59.8390921769273));
#140788=CARTESIAN_POINT('Ctrl Pts',(-29.,40.1727138277874,-59.746082025009));
#140789=CARTESIAN_POINT('Ctrl Pts',(-29.,40.1727138277873,-59.6524466674074));
#140790=CARTESIAN_POINT('',(-29.,38.2024209812184,-61.4386408691297));
#140791=CARTESIAN_POINT('Ctrl Pts',(-29.,38.2024209812184,-61.4386408691297));
#140792=CARTESIAN_POINT('Ctrl Pts',(-29.,38.2265260808242,-61.3934796764616));
#140793=CARTESIAN_POINT('Ctrl Pts',(-29.,38.2570947542809,-61.3534209131338));
#140794=CARTESIAN_POINT('Ctrl Pts',(-29.,38.293280667393,-61.3178293882391));
#140795=CARTESIAN_POINT('Ctrl Pts',(-29.,38.3294709547425,-61.2822335609581));
#140796=CARTESIAN_POINT('Ctrl Pts',(-29.,38.3706505444737,-61.2520122466304));
#140797=CARTESIAN_POINT('Ctrl Pts',(-29.,38.4145916132166,-61.2276531730517));
#140798=CARTESIAN_POINT('Ctrl Pts',(-29.,38.4390337855644,-61.2141034645061));
#140799=CARTESIAN_POINT('Ctrl Pts',(-29.,38.4644512947928,-61.2023317240158));
#140800=CARTESIAN_POINT('Ctrl Pts',(-29.,38.490593259323,-61.1923093713145));
#140801=CARTESIAN_POINT('Ctrl Pts',(-29.,38.5172131854938,-61.1821037768321));
#140802=CARTESIAN_POINT('Ctrl Pts',(-29.,38.5445857496398,-61.1737118246007));
#140803=CARTESIAN_POINT('Ctrl Pts',(-29.,38.5724697430453,-61.1671525783509));
#140804=CARTESIAN_POINT('Ctrl Pts',(-29.,38.5996144829857,-61.1607672291985));
#140805=CARTESIAN_POINT('Ctrl Pts',(-29.,38.6272453201521,-61.1561187181941));
#140806=CARTESIAN_POINT('Ctrl Pts',(-29.,38.6551404973774,-61.1532723608215));
#140807=CARTESIAN_POINT('Ctrl Pts',(-29.,38.6716230181358,-61.1515905237032));
#140808=CARTESIAN_POINT('Ctrl Pts',(-29.,38.688197742811,-61.1505387782063));
#140809=CARTESIAN_POINT('Ctrl Pts',(-29.,38.7048160259599,-61.150138786574));
#140810=CARTESIAN_POINT('',(-29.,30.0207919771236,-76.4370443259982));
#140811=CARTESIAN_POINT('Ctrl Pts',(-29.,30.0207919771236,-76.4370443259982));
#140812=CARTESIAN_POINT('Ctrl Pts',(-29.,32.8015436034469,-71.4667836449984));
#140813=CARTESIAN_POINT('Ctrl Pts',(-29.,35.5206811754595,-66.4629124977081));
#140814=CARTESIAN_POINT('Ctrl Pts',(-29.,38.2024209812184,-61.4386408691297));
#140815=CARTESIAN_POINT('',(-29.,28.91999998,-80.9397703408579));
#140816=CARTESIAN_POINT('Ctrl Pts',(-29.,28.91999998,-80.9397703408579));
#140817=CARTESIAN_POINT('Ctrl Pts',(-29.,28.9199999800001,-80.5473141158908));
#140818=CARTESIAN_POINT('Ctrl Pts',(-29.,28.9425413961516,-80.1570353641503));
#140819=CARTESIAN_POINT('Ctrl Pts',(-29.,28.98734507234,-79.7689071194953));
#140820=CARTESIAN_POINT('Ctrl Pts',(-29.,29.0321487485283,-79.3807788748402));
#140821=CARTESIAN_POINT('Ctrl Pts',(-29.,29.0997153099482,-78.9928975232084));
#140822=CARTESIAN_POINT('Ctrl Pts',(-29.,29.1899491656343,-78.6129950217198));
#140823=CARTESIAN_POINT('Ctrl Pts',(-29.,29.2801830213205,-78.2330925202312));
#140824=CARTESIAN_POINT('Ctrl Pts',(-29.,29.3927364426023,-77.8611684636915));
#140825=CARTESIAN_POINT('Ctrl Pts',(-29.,29.5298914474149,-77.498038591685));
#140826=CARTESIAN_POINT('Ctrl Pts',(-29.,29.6670464522275,-77.1349087196785));
#140827=CARTESIAN_POINT('Ctrl Pts',(-29.,29.8286298518252,-76.7805111234986));
#140828=CARTESIAN_POINT('Ctrl Pts',(-29.,30.0207919771235,-76.4370443259982));
#140829=CARTESIAN_POINT('',(-29.,28.91999998,-91.34995));
#140830=CARTESIAN_POINT('',(-29.,28.91999998,-80.3749072158811));
#140831=CARTESIAN_POINT('Origin',(-29.,29.41999998,-91.34995));
#140832=CARTESIAN_POINT('',(-29.,46.41999998,-58.24995));
#140833=CARTESIAN_POINT('',(-29.,46.41999998,-92.34995));
#140834=CARTESIAN_POINT('Origin',(-29.,43.91999998,-58.24995));
#140835=CARTESIAN_POINT('Ctrl Pts',(-28.4933647440612,38.6927858841383,
-60.650327573148));
#140836=CARTESIAN_POINT('Ctrl Pts',(-29.,38.6926240909195,-60.6436056187277));
#140837=CARTESIAN_POINT('Ctrl Pts',(-29.,38.7048160259599,-61.150138786574));
#140838=CARTESIAN_POINT('Ctrl Pts',(-28.4870505338491,38.8213938162437,
-60.647315885492));
#140839=CARTESIAN_POINT('Ctrl Pts',(-29.0000000000007,38.8211017330502,
-60.6340675708554));
#140840=CARTESIAN_POINT('Ctrl Pts',(-29.,38.8968977730653,-61.1455154974199));
#140841=CARTESIAN_POINT('Ctrl Pts',(-28.4808526630789,38.9512642676271,
-60.6191174333591));
#140842=CARTESIAN_POINT('Ctrl Pts',(-28.9999999999993,38.9470356871939,
-60.5993042062512));
#140843=CARTESIAN_POINT('Ctrl Pts',(-29.,39.0908916037092,-61.103090199825));
#140844=CARTESIAN_POINT('Ctrl Pts',(-28.4702284641343,39.1877232210837,
-60.5175376561534));
#140845=CARTESIAN_POINT('Ctrl Pts',(-29.0000000000007,39.1728401027082,
-60.4895768580073));
#140846=CARTESIAN_POINT('Ctrl Pts',(-29.,39.4441857876827,-60.9504725910835));
#140847=CARTESIAN_POINT('Ctrl Pts',(-28.465656656414,39.2976315760154,-60.4428805969007));
#140848=CARTESIAN_POINT('Ctrl Pts',(-29.0000000000007,39.2753871003781,
-60.4130391624567));
#140849=CARTESIAN_POINT('Ctrl Pts',(-29.,39.6084483440092,-60.8383643971029));
#140850=CARTESIAN_POINT('Ctrl Pts',(-28.4606134496588,39.434276061177,-60.3041245704241));
#140851=CARTESIAN_POINT('Ctrl Pts',(-28.9999999999996,39.4020840949312,
-60.2760820218603));
#140852=CARTESIAN_POINT('Ctrl Pts',(-29.,39.8127532432739,-60.6300880930806));
#140853=CARTESIAN_POINT('Ctrl Pts',(-28.4592438293891,39.4746917169037,
-60.2541491598715));
#140854=CARTESIAN_POINT('Ctrl Pts',(-29.,39.439411822071,-60.2273142826608));
#140855=CARTESIAN_POINT('Ctrl Pts',(-29.,39.8731969861748,-60.5550848424531));
#140856=CARTESIAN_POINT('Ctrl Pts',(-28.4570887248156,39.5455314661108,
-60.1469471546371));
#140857=CARTESIAN_POINT('Ctrl Pts',(-29.,39.5049075987374,-60.1236050817051));
#140858=CARTESIAN_POINT('Ctrl Pts',(-29.,39.9791737873547,-60.3942177709194));
#140859=CARTESIAN_POINT('Ctrl Pts',(-28.4563005932054,39.5761796095201,
-60.0890325252997));
#140860=CARTESIAN_POINT('Ctrl Pts',(-29.0000000000002,39.5332188379146,
-60.0680634823705));
#140861=CARTESIAN_POINT('Ctrl Pts',(-29.,40.025042572592,-60.3073218018945));
#140862=CARTESIAN_POINT('Ctrl Pts',(-28.4548707416055,39.6494517959669,
-59.9101257001469));
#140863=CARTESIAN_POINT('Ctrl Pts',(-28.9999999999997,39.6014080499751,
-59.8970923098554));
#140864=CARTESIAN_POINT('Ctrl Pts',(-29.,40.1347632142717,-60.0389178342029));
#140865=CARTESIAN_POINT('Ctrl Pts',(-28.4551199545093,39.6747304042147,
-59.7821590925224));
#140866=CARTESIAN_POINT('Ctrl Pts',(-29.,39.6256255569264,-59.7761492712348));
#140867=CARTESIAN_POINT('Ctrl Pts',(-29.,40.1727138319509,-59.8469756744913));
#140868=CARTESIAN_POINT('Ctrl Pts',(-28.4564221286262,39.6746164787415,
-59.6524466674074));
#140869=CARTESIAN_POINT('Ctrl Pts',(-29.,39.6270595772528,-59.6524466674074));
#140870=CARTESIAN_POINT('Ctrl Pts',(-29.,40.1727138277874,-59.6524466674074));
#140871=CARTESIAN_POINT('Origin',(-28.5,38.7048160259599,-61.150138786574));
#140872=CARTESIAN_POINT('Ctrl Pts',(-39.,37.7046087726872,-61.14995));
#140873=CARTESIAN_POINT('Ctrl Pts',(-39.,37.7046087726872,-60.64995));
#140874=CARTESIAN_POINT('Ctrl Pts',(-39.5,37.7046087726872,-60.64995));
#140875=CARTESIAN_POINT('Ctrl Pts',(-39.,37.9017438633342,-61.149949999985));
#140876=CARTESIAN_POINT('Ctrl Pts',(-38.9999999999973,37.8357552425198,
-60.655621796981));
#140877=CARTESIAN_POINT('Ctrl Pts',(-39.4942946417934,37.8365313206165,
-60.64995));
#140878=CARTESIAN_POINT('Ctrl Pts',(-39.,38.0987303642205,-61.110909009472));
#140879=CARTESIAN_POINT('Ctrl Pts',(-39.,37.9700367301949,-60.6353187454024));
#140880=CARTESIAN_POINT('Ctrl Pts',(-39.4885935839755,37.9683544324696,
-60.6239226729818));
#140881=CARTESIAN_POINT('Ctrl Pts',(-39.,38.4629228438758,-60.9606295880618));
#140882=CARTESIAN_POINT('Ctrl Pts',(-39.,38.2214119490388,-60.5426326522478));
#140883=CARTESIAN_POINT('Ctrl Pts',(-39.4780533572395,38.2120715692569,
-60.5237363920407));
#140884=CARTESIAN_POINT('Ctrl Pts',(-39.,38.6299500658835,-60.8494502533514));
#140885=CARTESIAN_POINT('Ctrl Pts',(-39.,38.3387190323947,-60.4706504746467));
#140886=CARTESIAN_POINT('Ctrl Pts',(-39.4732193617859,38.3238459703974,
-60.4496168355678));
#140887=CARTESIAN_POINT('Ctrl Pts',(-39.,38.9086909221403,-60.5717700902082));
#140888=CARTESIAN_POINT('Ctrl Pts',(-39.,38.5356496464585,-60.2852157712116));
#140889=CARTESIAN_POINT('Ctrl Pts',(-39.4651522214979,38.5103789912237,
-60.2644967268053));
#140890=CARTESIAN_POINT('Ctrl Pts',(-39.,39.0202949438762,-60.4053784571342));
#140891=CARTESIAN_POINT('Ctrl Pts',(-39.,38.6156677780068,-60.1718710142637));
#140892=CARTESIAN_POINT('Ctrl Pts',(-39.4619222489988,38.5850642583582,
-60.153568971423));
#140893=CARTESIAN_POINT('Ctrl Pts',(-39.,39.1711484082035,-60.0425718399611));
#140894=CARTESIAN_POINT('Ctrl Pts',(-39.,38.7237795941064,-59.9224177216067));
#140895=CARTESIAN_POINT('Ctrl Pts',(-39.4575563441359,38.6860152017583,
-59.9116978933072));
#140896=CARTESIAN_POINT('Ctrl Pts',(-39.,39.2103385289879,-59.8463349320561));
#140897=CARTESIAN_POINT('Ctrl Pts',(-39.,38.7521729419779,-59.7861314644994));
#140898=CARTESIAN_POINT('Ctrl Pts',(-39.4564221286291,38.7122411799561,
-59.7808732880376));
#140899=CARTESIAN_POINT('Ctrl Pts',(-39.,39.2103385290023,-59.64995));
#140900=CARTESIAN_POINT('Ctrl Pts',(-39.,38.7521729419935,-59.64995));
#140901=CARTESIAN_POINT('Ctrl Pts',(-39.4564221286262,38.7122411799564,
-59.64995));
#140902=CARTESIAN_POINT('',(-39.,37.7046087726872,-61.14995));
#140903=CARTESIAN_POINT('Origin',(-39.5,37.7046087726872,-61.14995));
#140904=CARTESIAN_POINT('Ctrl Pts',(-39.,39.2103385290022,-59.64995));
#140905=CARTESIAN_POINT('Ctrl Pts',(-39.,39.2103385289878,-59.8463349320561));
#140906=CARTESIAN_POINT('Ctrl Pts',(-39.,39.1711484082035,-60.0425718399611));
#140907=CARTESIAN_POINT('Ctrl Pts',(-39.,39.0957216760398,-60.2239751485477));
#140908=CARTESIAN_POINT('Ctrl Pts',(-39.,39.0202949438762,-60.4053784571342));
#140909=CARTESIAN_POINT('Ctrl Pts',(-39.,38.9086909221403,-60.5717700902082));
#140910=CARTESIAN_POINT('Ctrl Pts',(-39.,38.7693204940119,-60.7106101717798));
#140911=CARTESIAN_POINT('Ctrl Pts',(-39.,38.6299500658835,-60.8494502533514));
#140912=CARTESIAN_POINT('Ctrl Pts',(-39.,38.4629228438757,-60.9606295880618));
#140913=CARTESIAN_POINT('Ctrl Pts',(-39.,38.2808266040481,-61.0357692987669));
#140914=CARTESIAN_POINT('Ctrl Pts',(-39.,38.0987303642205,-61.110909009472));
#140915=CARTESIAN_POINT('Ctrl Pts',(-39.,37.9017438633342,-61.149949999985));
#140916=CARTESIAN_POINT('Ctrl Pts',(-39.,37.7046087726872,-61.14995));
#140917=CARTESIAN_POINT('Origin',(-39.,46.91999998,-129.34995));
#140918=CARTESIAN_POINT('',(-39.,31.080768958446,-61.14995));
#140919=CARTESIAN_POINT('',(-39.,31.080768958446,-91.9958480337503));
#140920=CARTESIAN_POINT('',(-39.,31.080768958446,-129.34995));
#140921=CARTESIAN_POINT('',(-39.,31.080768958446,-61.14995));
#140922=CARTESIAN_POINT('',(-39.,43.91999998,-55.74995));
#140923=CARTESIAN_POINT('',(-39.,46.91999998,-55.74995));
#140924=CARTESIAN_POINT('',(-39.,46.41999998,-58.24995));
#140925=CARTESIAN_POINT('Origin',(-39.,43.91999998,-58.24995));
#140926=CARTESIAN_POINT('',(-39.,46.41999998,-91.9958480337503));
#140927=CARTESIAN_POINT('',(-39.,46.41999998,-129.34995));
#140928=CARTESIAN_POINT('',(-39.,46.41999998,-91.9958480337503));
#140929=CARTESIAN_POINT('Origin',(-38.5,-1.68631645800828E-14,-55.74995));
#140930=CARTESIAN_POINT('',(-38.5,43.91999998,-55.24995));
#140931=CARTESIAN_POINT('',(-38.5,-1.68631645800828E-14,-55.24995));
#140932=CARTESIAN_POINT('Origin',(-38.5,43.91999998,-55.74995));
#140933=CARTESIAN_POINT('Origin',(0.,0.,-55.24995));
#140934=CARTESIAN_POINT('',(-38.,43.91999998,-55.24995));
#140935=CARTESIAN_POINT('',(-38.,38.8834059372824,-55.24995));
#140936=CARTESIAN_POINT('',(0.,43.91999998,-55.24995));
#140937=CARTESIAN_POINT('Origin',(-38.,-9.33460238845303,-55.74995));
#140938=CARTESIAN_POINT('',(-37.5,43.91999998,-55.74995));
#140939=CARTESIAN_POINT('',(-37.5,43.91999998,-55.74995));
#140940=CARTESIAN_POINT('Origin',(-38.,43.91999998,-55.74995));
#140941=CARTESIAN_POINT('Origin',(-37.5,-9.33460238845303,-92.34995));
#140942=CARTESIAN_POINT('',(-37.5,46.41999998,-58.24995));
#140943=CARTESIAN_POINT('',(-37.5,46.41999998,-92.34995));
#140944=CARTESIAN_POINT('Origin',(-37.5,43.91999998,-58.24995));
#140945=CARTESIAN_POINT('',(-37.5,33.02054075664,-61.14995));
#140946=CARTESIAN_POINT('',(-37.5,-9.33460238845303,-61.14995));
#140947=CARTESIAN_POINT('',(-37.5,32.4374646344434,-61.4386408691296));
#140948=CARTESIAN_POINT('Ctrl Pts',(-37.5,32.4374646344434,-61.4386408691296));
#140949=CARTESIAN_POINT('Ctrl Pts',(-37.5,32.4670379954265,-61.3894770341505));
#140950=CARTESIAN_POINT('Ctrl Pts',(-37.5,32.5044515673201,-61.3474771045912));
#140951=CARTESIAN_POINT('Ctrl Pts',(-37.5,32.5478217582305,-61.3109844882787));
#140952=CARTESIAN_POINT('Ctrl Pts',(-37.5,32.5912010725173,-61.2744841953601));
#140953=CARTESIAN_POINT('Ctrl Pts',(-37.5,32.6399569706336,-61.2443658937749));
#140954=CARTESIAN_POINT('Ctrl Pts',(-37.5,32.6911307205588,-61.2206312870705));
#140955=CARTESIAN_POINT('Ctrl Pts',(-37.5,32.7200261312687,-61.2072294705187));
#140956=CARTESIAN_POINT('Ctrl Pts',(-37.5,32.7497820420349,-61.1958060470671));
#140957=CARTESIAN_POINT('Ctrl Pts',(-37.5,32.7801663767934,-61.1862777806123));
#140958=CARTESIAN_POINT('Ctrl Pts',(-37.5,32.8113193812834,-61.1765084659306));
#140959=CARTESIAN_POINT('Ctrl Pts',(-37.5,32.8431343593207,-61.168731309436));
#140960=CARTESIAN_POINT('Ctrl Pts',(-37.5,32.8753810744804,-61.1629086143648));
#140961=CARTESIAN_POINT('Ctrl Pts',(-37.5,32.9073189135581,-61.1571416921447));
#140962=CARTESIAN_POINT('Ctrl Pts',(-37.5,32.9396816981554,-61.1532921099755));
#140963=CARTESIAN_POINT('Ctrl Pts',(-37.5,32.9722439056897,-61.1513728702169));
#140964=CARTESIAN_POINT('Ctrl Pts',(-37.5,32.9883041294272,-61.1504262691642));
#140965=CARTESIAN_POINT('Ctrl Pts',(-37.5,33.0044127038511,-61.14995));
#140966=CARTESIAN_POINT('Ctrl Pts',(-37.5,33.02054075664,-61.14995));
#140967=CARTESIAN_POINT('',(-37.5,30.3198029183596,-64.9254179945056));
#140968=CARTESIAN_POINT('Ctrl Pts',(-37.5,30.3198029183591,-64.9254179945063));
#140969=CARTESIAN_POINT('Ctrl Pts',(-37.5,31.0308541172825,-63.7662953234662));
#140970=CARTESIAN_POINT('Ctrl Pts',(-37.5,31.7365266751429,-62.6039057229559));
#140971=CARTESIAN_POINT('Ctrl Pts',(-37.5,32.4374646344434,-61.4386408691296));
#140972=CARTESIAN_POINT('',(-37.5,28.91999998,-70.4461836365688));
#140973=CARTESIAN_POINT('Ctrl Pts',(-37.5,28.91999998,-70.4461836365688));
#140974=CARTESIAN_POINT('Ctrl Pts',(-37.5,28.91999998,-69.9121746574189));
#140975=CARTESIAN_POINT('Ctrl Pts',(-37.5,28.9527491161432,-69.3820227305135));
#140976=CARTESIAN_POINT('Ctrl Pts',(-37.5,29.0202545273688,-68.8559643077599));
#140977=CARTESIAN_POINT('Ctrl Pts',(-37.5,29.0748216912419,-68.4307314910118));
#140978=CARTESIAN_POINT('Ctrl Pts',(-37.5,29.1520996751857,-68.0081734812099));
#140979=CARTESIAN_POINT('Ctrl Pts',(-37.5,29.2531734731887,-67.5884180460506));
#140980=CARTESIAN_POINT('Ctrl Pts',(-37.5,29.3662299152087,-67.1188991701864));
#140981=CARTESIAN_POINT('Ctrl Pts',(-37.5,29.5081290337322,-66.6603034853492));
#140982=CARTESIAN_POINT('Ctrl Pts',(-37.5,29.6832395831696,-66.2153982561153));
#140983=CARTESIAN_POINT('Ctrl Pts',(-37.5,29.813724236086,-65.883874515234));
#140984=CARTESIAN_POINT('Ctrl Pts',(-37.5,29.9624113407314,-65.5596714884752));
#140985=CARTESIAN_POINT('Ctrl Pts',(-37.5,30.1346313217948,-65.2449329573506));
#140986=CARTESIAN_POINT('Ctrl Pts',(-37.5,30.1935307469916,-65.137292029416));
#140987=CARTESIAN_POINT('Ctrl Pts',(-37.5,30.2551830721499,-65.0307582682135));
#140988=CARTESIAN_POINT('Ctrl Pts',(-37.5,30.3198029183595,-64.9254179945056));
#140989=CARTESIAN_POINT('',(-37.5,28.91999998,-91.34995));
#140990=CARTESIAN_POINT('',(-37.5,28.91999998,-69.7748183683767));
#140991=CARTESIAN_POINT('Origin',(-37.5,29.41999998,-91.34995));
#140992=CARTESIAN_POINT('Origin',(0.,-12.9675000200281,-60.64995));
#140993=CARTESIAN_POINT('',(-48.4322308821779,20.76999998,-60.64995));
#140994=CARTESIAN_POINT('',(-43.9604906504041,26.41999998,-60.64995));
#140995=CARTESIAN_POINT('Origin',(0.,-12.9675000200281,-60.64995));
#140996=CARTESIAN_POINT('',(-1.41024658483895E-14,20.76999998,-60.64995));
#140997=CARTESIAN_POINT('',(-1.64641978096591E-14,26.4199999800001,-60.64995));
#140998=CARTESIAN_POINT('Ctrl Pts',(-51.6895836746289,26.3764221086262,
-59.64995));
#140999=CARTESIAN_POINT('Ctrl Pts',(-51.6420267731401,26.91999998,-59.64995));
#141000=CARTESIAN_POINT('Ctrl Pts',(-52.1876810236747,26.91999998,-59.64995));
#141001=CARTESIAN_POINT('Ctrl Pts',(-51.6895836746287,26.3764221086278,
-59.7808732880375));
#141002=CARTESIAN_POINT('Ctrl Pts',(-51.6420267731333,26.919999980002,-59.7746029379318));
#141003=CARTESIAN_POINT('Ctrl Pts',(-52.1876810236604,26.91999998,-59.8463349320561));
#141004=CARTESIAN_POINT('Ctrl Pts',(-51.6633576964307,26.3775563241358,
-59.9116978933072));
#141005=CARTESIAN_POINT('Ctrl Pts',(-51.6186060348034,26.9199999800004,
-59.8989712332639));
#141006=CARTESIAN_POINT('Ctrl Pts',(-52.148490902876,26.91999998,-60.0425718399612));
#141007=CARTESIAN_POINT('Ctrl Pts',(-51.5624067530308,26.3819222289988,
-60.1535689714229));
#141008=CARTESIAN_POINT('Ctrl Pts',(-51.5267774915774,26.9199999799997,
-60.1322291512607));
#141009=CARTESIAN_POINT('Ctrl Pts',(-51.9976374385487,26.91999998,-60.4053784571341));
#141010=CARTESIAN_POINT('Ctrl Pts',(-51.4877214858962,26.3851522014976,
-60.2644967268053));
#141011=CARTESIAN_POINT('Ctrl Pts',(-51.4587108395762,26.9199999799996,
-60.2406767152617));
#141012=CARTESIAN_POINT('Ctrl Pts',(-51.8860334168128,26.91999998,-60.5717700902076));
#141013=CARTESIAN_POINT('Ctrl Pts',(-51.3011884650699,26.3932193417862,
-60.4496168355678));
#141014=CARTESIAN_POINT('Ctrl Pts',(-51.2846839917031,26.9199999800004,
-60.4261994932779));
#141015=CARTESIAN_POINT('Ctrl Pts',(-51.6072925605561,26.91999998,-60.8494502533521));
#141016=CARTESIAN_POINT('Ctrl Pts',(-51.1894140639292,26.3980533372399,
-60.5237363920408));
#141017=CARTESIAN_POINT('Ctrl Pts',(-51.1792534074218,26.9199999799993,
-60.5031527166058));
#141018=CARTESIAN_POINT('Ctrl Pts',(-51.4402653385482,26.91999998,-60.9606295880611));
#141019=CARTESIAN_POINT('Ctrl Pts',(-50.9456969271423,26.4085935639752,
-60.6239226729817));
#141020=CARTESIAN_POINT('Ctrl Pts',(-50.9439864347103,26.9199999800007,
-60.6120353079387));
#141021=CARTESIAN_POINT('Ctrl Pts',(-51.0760728588929,26.91999998,-61.1109090094727));
#141022=CARTESIAN_POINT('Ctrl Pts',(-50.8138738152888,26.4142946217921,
-60.64995));
#141023=CARTESIAN_POINT('Ctrl Pts',(-50.8146696888639,26.9199999800028,
-60.6442102195338));
#141024=CARTESIAN_POINT('Ctrl Pts',(-50.8790863580067,26.91999998,-61.149949999985));
#141025=CARTESIAN_POINT('Ctrl Pts',(-50.6819512673597,26.41999998,-60.64995));
#141026=CARTESIAN_POINT('Ctrl Pts',(-50.6819512673597,26.91999998,-60.64995));
#141027=CARTESIAN_POINT('Ctrl Pts',(-50.6819512673597,26.91999998,-61.14995));
#141028=CARTESIAN_POINT('',(-50.6819512673597,26.91999998,-61.14995));
#141029=CARTESIAN_POINT('Ctrl Pts',(-52.1876810236747,26.91999998,-59.64995));
#141030=CARTESIAN_POINT('Ctrl Pts',(-52.1876810236604,26.91999998,-59.8463349320561));
#141031=CARTESIAN_POINT('Ctrl Pts',(-52.148490902876,26.91999998,-60.0425718399612));
#141032=CARTESIAN_POINT('Ctrl Pts',(-51.9976374385487,26.91999998,-60.4053784571341));
#141033=CARTESIAN_POINT('Ctrl Pts',(-51.8860334168128,26.91999998,-60.5717700902076));
#141034=CARTESIAN_POINT('Ctrl Pts',(-51.6072925605561,26.91999998,-60.8494502533521));
#141035=CARTESIAN_POINT('Ctrl Pts',(-51.4402653385482,26.91999998,-60.9606295880611));
#141036=CARTESIAN_POINT('Ctrl Pts',(-51.0760728588929,26.91999998,-61.1109090094727));
#141037=CARTESIAN_POINT('Ctrl Pts',(-50.8790863580067,26.91999998,-61.149949999985));
#141038=CARTESIAN_POINT('Ctrl Pts',(-50.6819512673597,26.91999998,-61.14995));
#141039=CARTESIAN_POINT('Origin',(-50.6819512673597,26.41999998,-61.14995));
#141040=CARTESIAN_POINT('Ctrl Pts',(-51.1762622162812,20.76999998,-60.64995));
#141041=CARTESIAN_POINT('Ctrl Pts',(-51.1762622162812,20.26999998,-60.64995));
#141042=CARTESIAN_POINT('Ctrl Pts',(-51.1762622162812,20.26999998,-61.14995));
#141043=CARTESIAN_POINT('Ctrl Pts',(-51.3081847642104,20.764294621792,-60.64995));
#141044=CARTESIAN_POINT('Ctrl Pts',(-51.3074086861135,20.2699999799973,
-60.6556217969837));
#141045=CARTESIAN_POINT('Ctrl Pts',(-51.3733973069281,20.26999998,-61.149949999985));
#141046=CARTESIAN_POINT('Ctrl Pts',(-51.4400078760636,20.7585935639752,
-60.6239226729818));
#141047=CARTESIAN_POINT('Ctrl Pts',(-51.4416901737888,20.2699999799993,
-60.6353187454032));
#141048=CARTESIAN_POINT('Ctrl Pts',(-51.5703838078145,20.26999998,-61.1109090094727));
#141049=CARTESIAN_POINT('Ctrl Pts',(-51.6837250128509,20.7480533372398,
-60.5237363920407));
#141050=CARTESIAN_POINT('Ctrl Pts',(-51.6930653926326,20.2699999800007,
-60.5426326522471));
#141051=CARTESIAN_POINT('Ctrl Pts',(-51.9345762874696,20.26999998,-60.9606295880612));
#141052=CARTESIAN_POINT('Ctrl Pts',(-51.7954994139911,20.7432193417859,
-60.4496168355681));
#141053=CARTESIAN_POINT('Ctrl Pts',(-51.810372475988,20.2699999799993,-60.4706504746462));
#141054=CARTESIAN_POINT('Ctrl Pts',(-52.1016035094776,20.26999998,-60.849450253352));
#141055=CARTESIAN_POINT('Ctrl Pts',(-51.9820324348179,20.7351522014979,
-60.264496726805));
#141056=CARTESIAN_POINT('Ctrl Pts',(-52.007303090053,20.2699999800007,-60.2852157712124));
#141057=CARTESIAN_POINT('Ctrl Pts',(-52.3803443657342,20.26999998,-60.5717700902076));
#141058=CARTESIAN_POINT('Ctrl Pts',(-52.0567177019522,20.7319222289985,
-60.153568971423));
#141059=CARTESIAN_POINT('Ctrl Pts',(-52.0873212216015,20.2699999800003,
-60.1718710142637));
#141060=CARTESIAN_POINT('Ctrl Pts',(-52.4919483874702,20.26999998,-60.4053784571342));
#141061=CARTESIAN_POINT('Ctrl Pts',(-52.1576686453522,20.7275563241362,
-59.9116978933072));
#141062=CARTESIAN_POINT('Ctrl Pts',(-52.1954330376997,20.2699999799997,
-59.9224177216067));
#141063=CARTESIAN_POINT('Ctrl Pts',(-52.6428018517975,20.26999998,-60.0425718399611));
#141064=CARTESIAN_POINT('Ctrl Pts',(-52.1838946235501,20.7264221086281,
-59.7808732880376));
#141065=CARTESIAN_POINT('Ctrl Pts',(-52.2238263855712,20.2699999800007,
-59.7861314644994));
#141066=CARTESIAN_POINT('Ctrl Pts',(-52.6819919725819,20.26999998,-59.8463349320562));
#141067=CARTESIAN_POINT('Ctrl Pts',(-52.1838946235503,20.7264221086262,
-59.64995));
#141068=CARTESIAN_POINT('Ctrl Pts',(-52.2238263855875,20.26999998,-59.6499499999999));
#141069=CARTESIAN_POINT('Ctrl Pts',(-52.6819919725962,20.26999998,-59.64995));
#141070=CARTESIAN_POINT('',(-51.1762622162812,20.26999998,-61.14995));
#141071=CARTESIAN_POINT('Origin',(-51.1762622162812,20.76999998,-61.14995));
#141072=CARTESIAN_POINT('Ctrl Pts',(-51.1762622162812,20.26999998,-61.14995));
#141073=CARTESIAN_POINT('Ctrl Pts',(-51.3733973069281,20.26999998,-61.149949999985));
#141074=CARTESIAN_POINT('Ctrl Pts',(-51.5703838078145,20.26999998,-61.1109090094727));
#141075=CARTESIAN_POINT('Ctrl Pts',(-51.9345762874696,20.26999998,-60.9606295880612));
#141076=CARTESIAN_POINT('Ctrl Pts',(-52.1016035094776,20.26999998,-60.849450253352));
#141077=CARTESIAN_POINT('Ctrl Pts',(-52.3803443657342,20.26999998,-60.5717700902076));
#141078=CARTESIAN_POINT('Ctrl Pts',(-52.4919483874702,20.26999998,-60.4053784571342));
#141079=CARTESIAN_POINT('Ctrl Pts',(-52.6428018517975,20.26999998,-60.0425718399611));
#141080=CARTESIAN_POINT('Ctrl Pts',(-52.6819919725819,20.26999998,-59.8463349320562));
#141081=CARTESIAN_POINT('Ctrl Pts',(-52.6819919725962,20.26999998,-59.64995));
#141082=CARTESIAN_POINT('Origin',(83.2809572255632,26.9199999800001,-55.24995));
#141083=CARTESIAN_POINT('',(-49.6616970192851,26.91999998,-171.14995));
#141084=CARTESIAN_POINT('',(-51.176438378063,26.91999998,-172.64995));
#141085=CARTESIAN_POINT('Ctrl Pts',(-49.6616970192851,26.91999998,-171.14995));
#141086=CARTESIAN_POINT('Ctrl Pts',(-49.8600119386601,26.91999998,-171.149950000016));
#141087=CARTESIAN_POINT('Ctrl Pts',(-50.058177378641,26.91999998,-171.18899099047));
#141088=CARTESIAN_POINT('Ctrl Pts',(-50.4245495045741,26.91999998,-171.339270411997));
#141089=CARTESIAN_POINT('Ctrl Pts',(-50.5925763632168,26.91999998,-171.450449746589));
#141090=CARTESIAN_POINT('Ctrl Pts',(-50.8729854484245,26.91999998,-171.728129909852));
#141091=CARTESIAN_POINT('Ctrl Pts',(-50.9852574060669,26.91999998,-171.894521542842));
#141092=CARTESIAN_POINT('Ctrl Pts',(-51.1370137093498,26.91999998,-172.257328160063));
#141093=CARTESIAN_POINT('Ctrl Pts',(-51.176438378046,26.91999998,-172.453565067926));
#141094=CARTESIAN_POINT('Ctrl Pts',(-51.176438378063,26.91999998,-172.64995));
#141095=CARTESIAN_POINT('',(-44.1114262156583,26.91999998,-171.14995));
#141096=CARTESIAN_POINT('',(-49.5914266019339,26.91999998,-171.14995));
#141097=CARTESIAN_POINT('',(-43.5020331013479,26.91999998,-170.861259130871));
#141098=CARTESIAN_POINT('Ctrl Pts',(-43.5020331013479,26.91999998,-170.861259130871));
#141099=CARTESIAN_POINT('Ctrl Pts',(-43.5336466193108,26.91999998,-170.911515457779));
#141100=CARTESIAN_POINT('Ctrl Pts',(-43.5734840835972,26.91999998,-170.953836204196));
#141101=CARTESIAN_POINT('Ctrl Pts',(-43.61923735557,26.91999998,-170.99036760152));
#141102=CARTESIAN_POINT('Ctrl Pts',(-43.6650022527906,26.91999998,-171.026908280947));
#141103=CARTESIAN_POINT('Ctrl Pts',(-43.7162207484477,26.91999998,-171.056845311872));
#141104=CARTESIAN_POINT('Ctrl Pts',(-43.7696000450754,26.91999998,-171.080313003677));
#141105=CARTESIAN_POINT('Ctrl Pts',(-43.8006630727512,26.91999998,-171.093969563544));
#141106=CARTESIAN_POINT('Ctrl Pts',(-43.8326179990562,26.91999998,-171.105532778688));
#141107=CARTESIAN_POINT('Ctrl Pts',(-43.8652115257657,26.91999998,-171.115097339925));
#141108=CARTESIAN_POINT('Ctrl Pts',(-43.8987093663282,26.91999998,-171.124927271807));
#141109=CARTESIAN_POINT('Ctrl Pts',(-43.9328831236168,26.91999998,-171.132646173148));
#141110=CARTESIAN_POINT('Ctrl Pts',(-43.9674767132984,26.91999998,-171.138304320373));
#141111=CARTESIAN_POINT('Ctrl Pts',(-44.0018197383425,26.91999998,-171.143921485104));
#141112=CARTESIAN_POINT('Ctrl Pts',(-44.0365780353935,26.91999998,-171.147507459409));
#141113=CARTESIAN_POINT('Ctrl Pts',(-44.0714975023722,26.91999998,-171.149061689887));
#141114=CARTESIAN_POINT('Ctrl Pts',(-44.0847888272127,26.91999998,-171.149653273435));
#141115=CARTESIAN_POINT('Ctrl Pts',(-44.0981033481738,26.91999998,-171.14995));
#141116=CARTESIAN_POINT('Ctrl Pts',(-44.1114262156583,26.91999998,-171.14995));
#141117=CARTESIAN_POINT('',(-41.0569324495328,26.91999998,-167.025025538602));
#141118=CARTESIAN_POINT('Ctrl Pts',(-41.0569324495328,26.91999998,-167.025025538602));
#141119=CARTESIAN_POINT('Ctrl Pts',(-41.879954591083,26.91999998,-168.29867810854));
#141120=CARTESIAN_POINT('Ctrl Pts',(-42.6945981803054,26.91999998,-169.577671730211));
#141121=CARTESIAN_POINT('Ctrl Pts',(-43.502033101348,26.91999998,-170.861259130871));
#141122=CARTESIAN_POINT('',(-39.5,26.91999998,-161.0070032805));
#141123=CARTESIAN_POINT('Ctrl Pts',(-39.5,26.91999998,-161.0070032805));
#141124=CARTESIAN_POINT('Ctrl Pts',(-39.5,26.91999998,-161.534495292789));
#141125=CARTESIAN_POINT('Ctrl Pts',(-39.5301402469972,26.91999998,-162.058113878039));
#141126=CARTESIAN_POINT('Ctrl Pts',(-39.5903041384792,26.91999998,-162.577874021264));
#141127=CARTESIAN_POINT('Ctrl Pts',(-39.6504680299611,26.91999998,-163.097634164489));
#141128=CARTESIAN_POINT('Ctrl Pts',(-39.7405665669947,26.91999998,-163.613547303305));
#141129=CARTESIAN_POINT('Ctrl Pts',(-39.864660766352,26.91999998,-164.12509154227));
#141130=CARTESIAN_POINT('Ctrl Pts',(-39.9267078660346,26.91999998,-164.380863661769));
#141131=CARTESIAN_POINT('Ctrl Pts',(-39.997456507107,26.91999998,-164.6357182099));
#141132=CARTESIAN_POINT('Ctrl Pts',(-40.0767145462179,26.91999998,-164.886071972517));
#141133=CARTESIAN_POINT('Ctrl Pts',(-40.1559725853186,26.91999998,-165.136425735101));
#141134=CARTESIAN_POINT('Ctrl Pts',(-40.2438971237555,26.91999998,-165.383070268404));
#141135=CARTESIAN_POINT('Ctrl Pts',(-40.3414754155803,26.91999998,-165.625583031388));
#141136=CARTESIAN_POINT('Ctrl Pts',(-40.4688793539746,26.91999998,-165.942221912202));
#141137=CARTESIAN_POINT('Ctrl Pts',(-40.6122052010756,26.91999998,-166.252046258618));
#141138=CARTESIAN_POINT('Ctrl Pts',(-40.7764339005815,26.91999998,-166.552924284045));
#141139=CARTESIAN_POINT('Ctrl Pts',(-40.8637697314878,26.91999998,-166.712929401488));
#141140=CARTESIAN_POINT('Ctrl Pts',(-40.9570176103092,26.91999998,-166.870404192079));
#141141=CARTESIAN_POINT('Ctrl Pts',(-41.0569324495327,26.91999998,-167.025025538601));
#141142=CARTESIAN_POINT('',(-39.5,26.91999998,-71.0516396909898));
#141143=CARTESIAN_POINT('',(-39.5,26.91999998,-55.24995));
#141144=CARTESIAN_POINT('',(-41.0569324495432,26.91999998,-65.0336174328882));
#141145=CARTESIAN_POINT('Ctrl Pts',(-41.0569324495432,26.91999998,-65.0336174328882));
#141146=CARTESIAN_POINT('Ctrl Pts',(-40.8648408575281,26.91999998,-65.3308851945513));
#141147=CARTESIAN_POINT('Ctrl Pts',(-40.6972294070533,26.91999998,-65.6389714709844));
#141148=CARTESIAN_POINT('Ctrl Pts',(-40.5488568184254,26.91999998,-65.9555599509487));
#141149=CARTESIAN_POINT('Ctrl Pts',(-40.4750173837546,26.91999998,-66.1131140827463));
#141150=CARTESIAN_POINT('Ctrl Pts',(-40.4059436807373,26.91999998,-66.2727743327574));
#141151=CARTESIAN_POINT('Ctrl Pts',(-40.3409938376608,26.91999998,-66.4342570423367));
#141152=CARTESIAN_POINT('Ctrl Pts',(-40.1455341065928,26.91999998,-66.9202222963147));
#141153=CARTESIAN_POINT('Ctrl Pts',(-39.9875645491708,26.91999998,-67.4263054005813));
#141154=CARTESIAN_POINT('Ctrl Pts',(-39.8638827946265,26.91999998,-67.936760324224));
#141155=CARTESIAN_POINT('Ctrl Pts',(-39.7402010400822,26.91999998,-68.4472152478667));
#141156=CARTESIAN_POINT('Ctrl Pts',(-39.6502847003092,26.91999998,-68.9623259739815));
#141157=CARTESIAN_POINT('Ctrl Pts',(-39.5902135268069,26.91999998,-69.4815519521983));
#141158=CARTESIAN_POINT('Ctrl Pts',(-39.5301423533046,26.91999998,-70.0007779304151));
#141159=CARTESIAN_POINT('Ctrl Pts',(-39.5000000000007,26.91999998,-70.5241306955437));
#141160=CARTESIAN_POINT('Ctrl Pts',(-39.5,26.91999998,-71.0516396909898));
#141161=CARTESIAN_POINT('',(-43.3501517762232,26.91999998,-61.4386408691297));
#141162=CARTESIAN_POINT('Ctrl Pts',(-43.3501517762232,26.91999998,-61.4386408691297));
#141163=CARTESIAN_POINT('Ctrl Pts',(-42.5924607769204,26.91999998,-62.641249943458));
#141164=CARTESIAN_POINT('Ctrl Pts',(-41.828377509759,26.91999998,-63.839782013441));
#141165=CARTESIAN_POINT('Ctrl Pts',(-41.0569324495432,26.91999998,-65.0336174328882));
#141166=CARTESIAN_POINT('',(-43.9604906504041,26.91999998,-61.14995));
#141167=CARTESIAN_POINT('Ctrl Pts',(-43.9604906504041,26.91999998,-61.14995));
#141168=CARTESIAN_POINT('Ctrl Pts',(-43.9014853731981,26.91999998,-61.14995));
#141169=CARTESIAN_POINT('Ctrl Pts',(-43.8433879790802,26.91999998,-61.1556451738328));
#141170=CARTESIAN_POINT('Ctrl Pts',(-43.7862158462631,26.91999998,-61.1670601882964));
#141171=CARTESIAN_POINT('Ctrl Pts',(-43.7290408237003,26.91999998,-61.178475779728));
#141172=CARTESIAN_POINT('Ctrl Pts',(-43.6721412316922,26.91999998,-61.1959228882129));
#141173=CARTESIAN_POINT('Ctrl Pts',(-43.6185804531072,26.91999998,-61.2193930049692));
#141174=CARTESIAN_POINT('Ctrl Pts',(-43.5650151406998,26.91999998,-61.2428651084281));
#141175=CARTESIAN_POINT('Ctrl Pts',(-43.5142347717189,26.91999998,-61.2723879193617));
#141176=CARTESIAN_POINT('Ctrl Pts',(-43.4680362753946,26.91999998,-61.3091376491944));
#141177=CARTESIAN_POINT('Ctrl Pts',(-43.4218479344169,26.91999998,-61.345879300707));
#141178=CARTESIAN_POINT('Ctrl Pts',(-43.3818141153598,26.91999998,-61.3883863242137));
#141179=CARTESIAN_POINT('Ctrl Pts',(-43.3501517762232,26.91999998,-61.4386408691297));
#141180=CARTESIAN_POINT('',(83.2809572255632,26.9199999800001,-61.14995));
#141181=CARTESIAN_POINT('',(-57.,26.91999998,-55.74995));
#141182=CARTESIAN_POINT('',(83.2809572255632,26.9199999800001,-55.74995));
#141183=CARTESIAN_POINT('',(-59.5,26.91999998,-58.24995));
#141184=CARTESIAN_POINT('Origin',(-57.,26.91999998,-58.24995));
#141185=CARTESIAN_POINT('',(-59.5,26.91999998,-174.34995));
#141186=CARTESIAN_POINT('',(-59.5,26.91999998,-58.24995));
#141187=CARTESIAN_POINT('',(-57.,26.91999998,-176.84995));
#141188=CARTESIAN_POINT('Origin',(-57.,26.91999998,-174.34995));
#141189=CARTESIAN_POINT('',(-51.176438378063,26.91999998,-176.84995));
#141190=CARTESIAN_POINT('',(83.2809572255632,26.9199999800001,-176.84995));
#141191=CARTESIAN_POINT('',(-51.176438378063,26.91999998,-55.24995));
#141192=CARTESIAN_POINT('Origin',(-60.,27.41999998,-55.74995));
#141193=CARTESIAN_POINT('',(-57.,27.41999998,-55.24995));
#141194=CARTESIAN_POINT('',(-60.,27.41999998,-55.24995));
#141195=CARTESIAN_POINT('Origin',(-57.,27.41999998,-55.74995));
#141196=CARTESIAN_POINT('Origin',(-60.,28.41999998,-55.24995));
#141197=CARTESIAN_POINT('',(-57.,27.91999998,-55.24995));
#141198=CARTESIAN_POINT('',(-60.,27.91999998,-55.24995));
#141199=CARTESIAN_POINT('',(-57.,28.41999998,-55.24995));
#141200=CARTESIAN_POINT('Origin',(-60.,27.91999998,-55.74995));
#141201=CARTESIAN_POINT('',(-57.,28.41999998,-55.74995));
#141202=CARTESIAN_POINT('',(-60.,28.41999998,-55.74995));
#141203=CARTESIAN_POINT('Origin',(-57.,27.91999998,-55.74995));
#141204=CARTESIAN_POINT('Ctrl Pts',(-50.4632296085449,28.91999998,-60.64995));
#141205=CARTESIAN_POINT('Ctrl Pts',(-50.4632296085449,28.41999998,-60.64995));
#141206=CARTESIAN_POINT('Ctrl Pts',(-50.4632296085449,28.41999998,-61.14995));
#141207=CARTESIAN_POINT('Ctrl Pts',(-50.5951521564739,28.9142946217921,
-60.64995));
#141208=CARTESIAN_POINT('Ctrl Pts',(-50.5943760783778,28.4199999799973,
-60.6556217969837));
#141209=CARTESIAN_POINT('Ctrl Pts',(-50.6603646991919,28.41999998,-61.149949999985));
#141210=CARTESIAN_POINT('Ctrl Pts',(-50.7269752683276,28.9085935639752,
-60.6239226729817));
#141211=CARTESIAN_POINT('Ctrl Pts',(-50.728657566052,28.4199999799997,-60.6353187454025));
#141212=CARTESIAN_POINT('Ctrl Pts',(-50.8573512000782,28.41999998,-61.1109090094727));
#141213=CARTESIAN_POINT('Ctrl Pts',(-50.9706924051143,28.8980533372399,
-60.5237363920408));
#141214=CARTESIAN_POINT('Ctrl Pts',(-50.9800327848971,28.4199999800004,
-60.5426326522478));
#141215=CARTESIAN_POINT('Ctrl Pts',(-51.2215436797334,28.41999998,-60.9606295880612));
#141216=CARTESIAN_POINT('Ctrl Pts',(-51.0824668062551,28.8932193417862,
-60.4496168355678));
#141217=CARTESIAN_POINT('Ctrl Pts',(-51.0973398682523,28.4199999799993,
-60.4706504746461));
#141218=CARTESIAN_POINT('Ctrl Pts',(-51.3885709017413,28.41999998,-60.849450253352));
#141219=CARTESIAN_POINT('Ctrl Pts',(-51.2689998270813,28.8851522014976,
-60.2644967268053));
#141220=CARTESIAN_POINT('Ctrl Pts',(-51.294270482316,28.4199999800007,-60.2852157712125));
#141221=CARTESIAN_POINT('Ctrl Pts',(-51.6673117579979,28.41999998,-60.5717700902076));
#141222=CARTESIAN_POINT('Ctrl Pts',(-51.343685094216,28.8819222289984,-60.153568971423));
#141223=CARTESIAN_POINT('Ctrl Pts',(-51.3742886138646,28.4199999800003,
-60.1718710142637));
#141224=CARTESIAN_POINT('Ctrl Pts',(-51.7789157797339,28.41999998,-60.4053784571342));
#141225=CARTESIAN_POINT('Ctrl Pts',(-51.4446360376159,28.8775563241362,
-59.9116978933072));
#141226=CARTESIAN_POINT('Ctrl Pts',(-51.4824004299641,28.4199999799996,
-59.9224177216067));
#141227=CARTESIAN_POINT('Ctrl Pts',(-51.9297692440612,28.41999998,-60.0425718399611));
#141228=CARTESIAN_POINT('Ctrl Pts',(-51.4708620158139,28.8764221086278,
-59.7808732880376));
#141229=CARTESIAN_POINT('Ctrl Pts',(-51.5107937778383,28.4199999799973,
-59.7861314644994));
#141230=CARTESIAN_POINT('Ctrl Pts',(-51.9689593648456,28.41999998,-59.8463349320562));
#141231=CARTESIAN_POINT('Ctrl Pts',(-51.4708620158141,28.8764221086262,
-59.64995));
#141232=CARTESIAN_POINT('Ctrl Pts',(-51.5107937778512,28.41999998,-59.6499499999999));
#141233=CARTESIAN_POINT('Ctrl Pts',(-51.9689593648599,28.41999998,-59.64995));
#141234=CARTESIAN_POINT('',(-50.4632296085449,28.41999998,-61.14995));
#141235=CARTESIAN_POINT('Origin',(-50.4632296085449,28.91999998,-61.14995));
#141236=CARTESIAN_POINT('Ctrl Pts',(-50.4632296085449,28.41999998,-61.14995));
#141237=CARTESIAN_POINT('Ctrl Pts',(-50.6603646991919,28.41999998,-61.149949999985));
#141238=CARTESIAN_POINT('Ctrl Pts',(-50.8573512000782,28.41999998,-61.1109090094727));
#141239=CARTESIAN_POINT('Ctrl Pts',(-51.2215436797334,28.41999998,-60.9606295880612));
#141240=CARTESIAN_POINT('Ctrl Pts',(-51.3885709017413,28.41999998,-60.849450253352));
#141241=CARTESIAN_POINT('Ctrl Pts',(-51.6673117579979,28.41999998,-60.5717700902076));
#141242=CARTESIAN_POINT('Ctrl Pts',(-51.7789157797339,28.41999998,-60.4053784571342));
#141243=CARTESIAN_POINT('Ctrl Pts',(-51.9297692440612,28.41999998,-60.0425718399611));
#141244=CARTESIAN_POINT('Ctrl Pts',(-51.9689593648456,28.41999998,-59.8463349320562));
#141245=CARTESIAN_POINT('Ctrl Pts',(-51.9689593648599,28.41999998,-59.64995));
#141246=CARTESIAN_POINT('Origin',(-60.,28.41999998,-55.24995));
#141247=CARTESIAN_POINT('',(-42.,28.41999998,-171.14995));
#141248=CARTESIAN_POINT('',(-42.,28.41999998,-95.34995));
#141249=CARTESIAN_POINT('',(-42.,28.41999998,-95.34995));
#141250=CARTESIAN_POINT('',(-43.6738487993976,28.41999998,-171.14995));
#141251=CARTESIAN_POINT('',(-41.7558360441701,28.41999998,-171.14995));
#141252=CARTESIAN_POINT('',(-45.342056117244,28.41999998,-171.14995));
#141253=CARTESIAN_POINT('Ctrl Pts',(-45.342056117244,28.41999998,-171.14995));
#141254=CARTESIAN_POINT('Ctrl Pts',(-45.2224947881419,28.41999998,-171.149950023642));
#141255=CARTESIAN_POINT('Ctrl Pts',(-45.1028907122947,28.41999998,-171.153734801587));
#141256=CARTESIAN_POINT('Ctrl Pts',(-44.9833706553313,28.41999998,-171.157527071728));
#141257=CARTESIAN_POINT('Ctrl Pts',(-44.9639944908913,28.41999998,-171.158141861008));
#141258=CARTESIAN_POINT('Ctrl Pts',(-44.9446205282351,28.41999998,-171.158756957286));
#141259=CARTESIAN_POINT('Ctrl Pts',(-44.9252493015934,28.41999998,-171.15935636922));
#141260=CARTESIAN_POINT('Ctrl Pts',(-44.7862513546676,28.41999998,-171.163657440581));
#141261=CARTESIAN_POINT('Ctrl Pts',(-44.6473090850418,28.41999998,-171.167020207454));
#141262=CARTESIAN_POINT('Ctrl Pts',(-44.5082302458003,28.41999998,-171.167024238765));
#141263=CARTESIAN_POINT('Ctrl Pts',(-44.5082032664897,28.41999998,-171.167024239547));
#141264=CARTESIAN_POINT('Ctrl Pts',(-44.5081762871737,28.41999998,-171.167024240203));
#141265=CARTESIAN_POINT('Ctrl Pts',(-44.5081493078523,28.41999998,-171.167024240732));
#141266=CARTESIAN_POINT('Ctrl Pts',(-44.3691292618367,28.41999998,-171.16702696589));
#141267=CARTESIAN_POINT('Ctrl Pts',(-44.2300667116137,28.41999998,-171.163669289098));
#141268=CARTESIAN_POINT('Ctrl Pts',(-44.0910473224682,28.41999998,-171.159368608161));
#141269=CARTESIAN_POINT('Ctrl Pts',(-43.9520204566156,28.41999998,-171.155067695926));
#141270=CARTESIAN_POINT('Ctrl Pts',(-43.8129841111527,28.41999998,-171.149950027538));
#141271=CARTESIAN_POINT('Ctrl Pts',(-43.6738487993976,28.41999998,-171.14995));
#141272=CARTESIAN_POINT('',(-49.3103449325291,28.41999998,-171.14995));
#141273=CARTESIAN_POINT('',(-41.7558360441701,28.41999998,-171.14995));
#141274=CARTESIAN_POINT('',(-50.825086291307,28.41999998,-172.64995));
#141275=CARTESIAN_POINT('Ctrl Pts',(-50.825086291307,28.41999998,-172.64995));
#141276=CARTESIAN_POINT('Ctrl Pts',(-50.82508629129,28.41999998,-172.453565067926));
#141277=CARTESIAN_POINT('Ctrl Pts',(-50.7856616225938,28.41999998,-172.257328160063));
#141278=CARTESIAN_POINT('Ctrl Pts',(-50.6339053193109,28.41999998,-171.894521542842));
#141279=CARTESIAN_POINT('Ctrl Pts',(-50.5216333616693,28.41999998,-171.728129909852));
#141280=CARTESIAN_POINT('Ctrl Pts',(-50.2412242764601,28.41999998,-171.450449746589));
#141281=CARTESIAN_POINT('Ctrl Pts',(-50.0731974178181,28.41999998,-171.339270411997));
#141282=CARTESIAN_POINT('Ctrl Pts',(-49.7068252918851,28.41999998,-171.18899099047));
#141283=CARTESIAN_POINT('Ctrl Pts',(-49.5086598519041,28.41999998,-171.149950000016));
#141284=CARTESIAN_POINT('Ctrl Pts',(-49.3103449325291,28.41999998,-171.14995));
#141285=CARTESIAN_POINT('',(-50.825086291307,28.41999998,-176.84995));
#141286=CARTESIAN_POINT('',(-50.825086291307,28.41999998,-55.24995));
#141287=CARTESIAN_POINT('',(-57.,28.41999998,-176.84995));
#141288=CARTESIAN_POINT('',(-60.,28.41999998,-176.84995));
#141289=CARTESIAN_POINT('',(-59.5,28.41999998,-174.34995));
#141290=CARTESIAN_POINT('Origin',(-57.,28.41999998,-174.34995));
#141291=CARTESIAN_POINT('',(-59.5,28.41999998,-58.24995));
#141292=CARTESIAN_POINT('',(-59.5,28.41999998,-174.34995));
#141293=CARTESIAN_POINT('Origin',(-57.,28.41999998,-58.24995));
#141294=CARTESIAN_POINT('',(-45.342056117244,28.41999998,-61.14995));
#141295=CARTESIAN_POINT('',(-60.,28.41999998,-61.14995));
#141296=CARTESIAN_POINT('',(-43.6738487993976,28.41999998,-61.14995));
#141297=CARTESIAN_POINT('Ctrl Pts',(-43.6738487993976,28.41999998,-61.14995));
#141298=CARTESIAN_POINT('Ctrl Pts',(-43.8129691638245,28.41999998,-61.1499499724651));
#141299=CARTESIAN_POINT('Ctrl Pts',(-43.9520102350777,28.41999998,-61.1448326154154));
#141300=CARTESIAN_POINT('Ctrl Pts',(-44.0910473222173,28.41999998,-61.1405313837273));
#141301=CARTESIAN_POINT('Ctrl Pts',(-44.2300643593017,28.41999998,-61.1362307723049));
#141302=CARTESIAN_POINT('Ctrl Pts',(-44.3691300592233,28.4199999800001,
-61.1328730966358));
#141303=CARTESIAN_POINT('Ctrl Pts',(-44.5081446038248,28.41999998,-61.1328757503144));
#141304=CARTESIAN_POINT('Ctrl Pts',(-44.5081731511562,28.41999998,-61.1328757508594));
#141305=CARTESIAN_POINT('Ctrl Pts',(-44.5082016984814,28.41999998,-61.132875751546));
#141306=CARTESIAN_POINT('Ctrl Pts',(-44.5082302458005,28.41999998,-61.1328757523744));
#141307=CARTESIAN_POINT('Ctrl Pts',(-44.6473090834153,28.41999998,-61.1328797881197));
#141308=CARTESIAN_POINT('Ctrl Pts',(-44.7862513535664,28.41999998,-61.1362425571023));
#141309=CARTESIAN_POINT('Ctrl Pts',(-44.9252493016292,28.41999998,-61.140543629625));
#141310=CARTESIAN_POINT('Ctrl Pts',(-45.0447391053953,28.41999998,-61.144241053356));
#141311=CARTESIAN_POINT('Ctrl Pts',(-45.1643332045556,28.41999998,-61.1485385900917));
#141312=CARTESIAN_POINT('Ctrl Pts',(-45.2839053205809,28.41999998,-61.1496673946892));
#141313=CARTESIAN_POINT('Ctrl Pts',(-45.3032896860482,28.41999998,-61.1498503902034));
#141314=CARTESIAN_POINT('Ctrl Pts',(-45.3226734672922,28.41999998,-61.1499499961673));
#141315=CARTESIAN_POINT('Ctrl Pts',(-45.342056117244,28.41999998,-61.14995));
#141316=CARTESIAN_POINT('',(-41.7558360441701,28.41999998,-61.14995));
#141317=CARTESIAN_POINT('',(-60.,28.41999998,-61.14995));
#141318=CARTESIAN_POINT('',(-41.7558360441701,28.41999998,-94.0656090587062));
#141319=CARTESIAN_POINT('',(-41.7558360441701,28.41999998,-60.64995));
#141320=CARTESIAN_POINT('Origin',(-38.5,28.41999998,-95.34995));
#141321=CARTESIAN_POINT('Origin',(83.2809572255632,12.1199999800001,-55.24995));
#141322=CARTESIAN_POINT('',(-57.,12.11999998,-176.84995));
#141323=CARTESIAN_POINT('',(-53.1963133798215,12.11999998,-176.84995));
#141324=CARTESIAN_POINT('',(83.2809572255632,12.1199999800001,-176.84995));
#141325=CARTESIAN_POINT('',(-59.5,12.11999998,-174.34995));
#141326=CARTESIAN_POINT('Origin',(-57.,12.11999998,-174.34995));
#141327=CARTESIAN_POINT('',(-59.5,12.11999998,-58.24995));
#141328=CARTESIAN_POINT('',(-59.5,12.11999998,-174.34995));
#141329=CARTESIAN_POINT('Origin',(-57.,12.11999998,-58.24995));
#141330=CARTESIAN_POINT('',(-53.2607580814926,12.11999998,-60.7033966151602));
#141331=CARTESIAN_POINT('Origin',(-50.5588767647388,12.11999998,-59.7245163413739));
#141332=CARTESIAN_POINT('',(-52.8224784153176,12.11999998,-61.275204160084));
#141333=CARTESIAN_POINT('Origin',(-52.0615368275148,12.11999998,-60.1416270042289));
#141334=CARTESIAN_POINT('',(-52.6867218473722,12.11999998,-61.4386408691297));
#141335=CARTESIAN_POINT('Origin',(-53.5608834560611,12.11999998,-61.8978040915907));
#141336=CARTESIAN_POINT('',(-40.5508657493525,12.11999998,-84.2187933558389));
#141337=CARTESIAN_POINT('Ctrl Pts',(-40.5508657493525,12.11999998,-84.2187933558389));
#141338=CARTESIAN_POINT('Ctrl Pts',(-42.6282147356021,12.11999998,-80.4512454090371));
#141339=CARTESIAN_POINT('Ctrl Pts',(-44.6709958246292,12.11999998,-76.6652818249174));
#141340=CARTESIAN_POINT('Ctrl Pts',(-46.6906839910419,12.11999998,-72.8670157601218));
#141341=CARTESIAN_POINT('Ctrl Pts',(-48.7103721574547,12.11999998,-69.0687496953263));
#141342=CARTESIAN_POINT('Ctrl Pts',(-50.7067642663818,12.11999998,-65.2580729321624));
#141343=CARTESIAN_POINT('Ctrl Pts',(-52.6867218473722,12.11999998,-61.4386408691297));
#141344=CARTESIAN_POINT('',(-39.5,12.11999998,-88.5398461374725));
#141345=CARTESIAN_POINT('Ctrl Pts',(-39.5,12.11999998,-88.5398461374725));
#141346=CARTESIAN_POINT('Ctrl Pts',(-39.5,12.11999998,-88.1633801721072));
#141347=CARTESIAN_POINT('Ctrl Pts',(-39.5216886477936,12.11999998,-87.7889298981599));
#141348=CARTESIAN_POINT('Ctrl Pts',(-39.5647508040475,12.11999998,-87.4164660273289));
#141349=CARTESIAN_POINT('Ctrl Pts',(-39.6078129603014,12.11999998,-87.0440021564979));
#141350=CARTESIAN_POINT('Ctrl Pts',(-39.672739619198,12.11999998,-86.6717926677294));
#141351=CARTESIAN_POINT('Ctrl Pts',(-39.7591103506482,12.11999998,-86.3076691214426));
#141352=CARTESIAN_POINT('Ctrl Pts',(-39.8454810820984,12.11999998,-85.9435455751558));
#141353=CARTESIAN_POINT('Ctrl Pts',(-39.9523131981843,12.11999998,-85.5865932598646));
#141354=CARTESIAN_POINT('Ctrl Pts',(-40.0830988504763,12.11999998,-85.2380360010512));
#141355=CARTESIAN_POINT('Ctrl Pts',(-40.2020523584857,12.11999998,-84.9210126276812));
#141356=CARTESIAN_POINT('Ctrl Pts',(-40.340821045384,12.11999998,-84.6109338990986));
#141357=CARTESIAN_POINT('Ctrl Pts',(-40.5020760733022,12.11999998,-84.3087360817072));
#141358=CARTESIAN_POINT('Ctrl Pts',(-40.5181158924597,12.11999998,-84.2786768742311));
#141359=CARTESIAN_POINT('Ctrl Pts',(-40.5343782322712,12.11999998,-84.2486956551327));
#141360=CARTESIAN_POINT('Ctrl Pts',(-40.5508657493525,12.11999998,-84.2187933558389));
#141361=CARTESIAN_POINT('',(-39.5,12.11999998,-143.518796834034));
#141362=CARTESIAN_POINT('',(-39.5,12.11999998,-55.24995));
#141363=CARTESIAN_POINT('',(-40.5508657493446,12.11999998,-147.839849615653));
#141364=CARTESIAN_POINT('Ctrl Pts',(-40.5508657493446,12.11999998,-147.839849615653));
#141365=CARTESIAN_POINT('Ctrl Pts',(-40.4872051775685,12.11999998,-147.72439272417));
#141366=CARTESIAN_POINT('Ctrl Pts',(-40.4268911487417,12.11999998,-147.607488691345));
#141367=CARTESIAN_POINT('Ctrl Pts',(-40.369709660312,12.11999998,-147.489235888513));
#141368=CARTESIAN_POINT('Ctrl Pts',(-40.3100900049245,12.11999998,-147.365940893103));
#141369=CARTESIAN_POINT('Ctrl Pts',(-40.2538755845828,12.11999998,-147.241179143609));
#141370=CARTESIAN_POINT('Ctrl Pts',(-40.2008730860127,12.11999998,-147.115031779943));
#141371=CARTESIAN_POINT('Ctrl Pts',(-40.1592698126768,12.11999998,-147.016014877103));
#141372=CARTESIAN_POINT('Ctrl Pts',(-40.119646471931,12.11999998,-146.916143544358));
#141373=CARTESIAN_POINT('Ctrl Pts',(-40.0819301037035,12.11999998,-146.815448147357));
#141374=CARTESIAN_POINT('Ctrl Pts',(-40.0215352750629,12.11999998,-146.654205654174));
#141375=CARTESIAN_POINT('Ctrl Pts',(-39.9660661346646,12.11999998,-146.490922340265));
#141376=CARTESIAN_POINT('Ctrl Pts',(-39.9154672964458,12.11999998,-146.32638803891));
#141377=CARTESIAN_POINT('Ctrl Pts',(-39.8629240743822,12.11999998,-146.15553110548));
#141378=CARTESIAN_POINT('Ctrl Pts',(-39.8156327203447,12.11999998,-145.983326186388));
#141379=CARTESIAN_POINT('Ctrl Pts',(-39.7734780737249,12.11999998,-145.81067296635));
#141380=CARTESIAN_POINT('Ctrl Pts',(-39.7676020779481,12.11999998,-145.786606589968));
#141381=CARTESIAN_POINT('Ctrl Pts',(-39.7618258061274,12.11999998,-145.762531511883));
#141382=CARTESIAN_POINT('Ctrl Pts',(-39.7561488675992,12.11999998,-145.738450173272));
#141383=CARTESIAN_POINT('Ctrl Pts',(-39.6543246883751,12.11999998,-145.306516213354));
#141384=CARTESIAN_POINT('Ctrl Pts',(-39.5830357134849,12.11999998,-144.869793515198));
#141385=CARTESIAN_POINT('Ctrl Pts',(-39.5419615359823,12.11999998,-144.428332293186));
#141386=CARTESIAN_POINT('Ctrl Pts',(-39.5139579007162,12.11999998,-144.127351974236));
#141387=CARTESIAN_POINT('Ctrl Pts',(-39.5,12.11999998,-143.824168887332));
#141388=CARTESIAN_POINT('Ctrl Pts',(-39.5,12.11999998,-143.518796834034));
#141389=CARTESIAN_POINT('',(-52.811758955289,12.11999998,-170.861259130871));
#141390=CARTESIAN_POINT('Ctrl Pts',(-52.811758955289,12.11999998,-170.861259130871));
#141391=CARTESIAN_POINT('Ctrl Pts',(-50.8116686437173,12.11999998,-167.001247608061));
#141392=CARTESIAN_POINT('Ctrl Pts',(-48.794913685955,12.11999998,-163.150111451771));
#141393=CARTESIAN_POINT('Ctrl Pts',(-46.7544651237368,12.11999998,-159.311594190676));
#141394=CARTESIAN_POINT('Ctrl Pts',(-44.7140165615186,12.11999998,-155.47307692958));
#141395=CARTESIAN_POINT('Ctrl Pts',(-42.6500867945137,12.11999998,-151.647065442471));
#141396=CARTESIAN_POINT('Ctrl Pts',(-40.5508657493446,12.11999998,-147.839849615653));
#141397=CARTESIAN_POINT('',(-52.8706140943225,12.11999998,-170.949706593448));
#141398=CARTESIAN_POINT('Ctrl Pts',(-52.8706140943225,12.11999998,-170.949706593448));
#141399=CARTESIAN_POINT('Ctrl Pts',(-52.8478318703964,12.11999998,-170.92232940649));
#141400=CARTESIAN_POINT('Ctrl Pts',(-52.8281487108054,12.11999998,-170.892890025127));
#141401=CARTESIAN_POINT('Ctrl Pts',(-52.811758955289,12.11999998,-170.861259130871));
#141402=CARTESIAN_POINT('',(-53.1963133798215,12.11999998,-171.855638188259));
#141403=CARTESIAN_POINT('Ctrl Pts',(-53.1963133798215,12.11999998,-171.855638188259));
#141404=CARTESIAN_POINT('Ctrl Pts',(-53.196313374732,12.11999998,-171.73372692869));
#141405=CARTESIAN_POINT('Ctrl Pts',(-53.1815021190177,12.11999998,-171.614382981042));
#141406=CARTESIAN_POINT('Ctrl Pts',(-53.1513539481864,12.11999998,-171.497697478252));
#141407=CARTESIAN_POINT('Ctrl Pts',(-53.1406117769373,12.11999998,-171.456120970666));
#141408=CARTESIAN_POINT('Ctrl Pts',(-53.1279219841079,12.11999998,-171.414882055034));
#141409=CARTESIAN_POINT('Ctrl Pts',(-53.1132591959952,12.11999998,-171.373985128688));
#141410=CARTESIAN_POINT('Ctrl Pts',(-53.0817091112288,12.11999998,-171.285986756006));
#141411=CARTESIAN_POINT('Ctrl Pts',(-53.0420949559112,12.11999998,-171.202535400955));
#141412=CARTESIAN_POINT('Ctrl Pts',(-52.9945125852814,12.11999998,-171.123638976918));
#141413=CARTESIAN_POINT('Ctrl Pts',(-52.9579184729698,12.11999998,-171.062962206006));
#141414=CARTESIAN_POINT('Ctrl Pts',(-52.9166104754484,12.11999998,-171.00498002573));
#141415=CARTESIAN_POINT('Ctrl Pts',(-52.8706140943225,12.11999998,-170.949706593449));
#141416=CARTESIAN_POINT('',(-53.1963133798215,12.11999998,-171.806096612245));
#141417=CARTESIAN_POINT('Ctrl Pts',(-52.81219032515,12.5218539749099,-60.5055220850798));
#141418=CARTESIAN_POINT('Ctrl Pts',(-52.8857929788877,12.11999998,-60.5379900686009));
#141419=CARTESIAN_POINT('Ctrl Pts',(-53.2607580814926,12.11999998,-60.7033966151602));
#141420=CARTESIAN_POINT('Ctrl Pts',(-52.8700875991767,12.5389561241882,
-60.3657903170377));
#141421=CARTESIAN_POINT('Ctrl Pts',(-52.9388615253298,12.1199999799981,
-60.3810288628603));
#141422=CARTESIAN_POINT('Ctrl Pts',(-53.3498368505456,12.11999998,-60.5014612122216));
#141423=CARTESIAN_POINT('Ctrl Pts',(-52.8985874779024,12.5574454029709,
-60.2163866339305));
#141424=CARTESIAN_POINT('Ctrl Pts',(-52.9540808994585,12.1199999800015,
-60.2191862528169));
#141425=CARTESIAN_POINT('Ctrl Pts',(-53.3950245780495,12.11999998,-60.2853240337268));
#141426=CARTESIAN_POINT('Ctrl Pts',(-52.8969272312866,12.5764221086261,
-60.0627241236309));
#141427=CARTESIAN_POINT('Ctrl Pts',(-52.9368589933238,12.11999998,-60.0627241236309));
#141428=CARTESIAN_POINT('Ctrl Pts',(-53.3950245803325,12.11999998,-60.0627241236311));
#141429=CARTESIAN_POINT('Origin',(-53.2607580814926,12.61999998,-60.7033966151602));
#141430=CARTESIAN_POINT('Ctrl Pts',(-52.4885489491165,12.6049688303995,
-60.8798615124595));
#141431=CARTESIAN_POINT('Ctrl Pts',(-52.7011006011713,12.5792267001133,
-60.7309116189004));
#141432=CARTESIAN_POINT('Ctrl Pts',(-52.8135194149171,12.5211707144541,
-60.5028360925954));
#141433=CARTESIAN_POINT('Ctrl Pts',(-52.5003487858574,12.5616578171005,
-60.8867883233088));
#141434=CARTESIAN_POINT('Ctrl Pts',(-52.7083699494148,12.5371106789483,
-60.7374192211268));
#141435=CARTESIAN_POINT('Ctrl Pts',(-52.8184252363688,12.4804454574502,
-60.5118893693287));
#141436=CARTESIAN_POINT('Ctrl Pts',(-52.5124335500125,12.5183120391401,
-60.8937038544239));
#141437=CARTESIAN_POINT('Ctrl Pts',(-52.7160214096145,12.4948853110753,
-60.7440415583411));
#141438=CARTESIAN_POINT('Ctrl Pts',(-52.823766550455,12.4396518133592,-60.5210243207318));
#141439=CARTESIAN_POINT('Ctrl Pts',(-52.5248032674767,12.4749209213966,
-60.9005813814078));
#141440=CARTESIAN_POINT('Ctrl Pts',(-52.7240626356492,12.4525613978151,
-60.750736804912));
#141441=CARTESIAN_POINT('Ctrl Pts',(-52.8295491865184,12.3987982841401,
-60.5301925771521));
#141442=CARTESIAN_POINT('',(-52.5245819708686,12.4756972986232,-60.9004583201709));
#141443=CARTESIAN_POINT('Ctrl Pts',(-52.4885489491165,12.6049688303995,
-60.8798615124595));
#141444=CARTESIAN_POINT('Ctrl Pts',(-52.5003074888079,12.5618093982546,
-60.8867640803813));
#141445=CARTESIAN_POINT('Ctrl Pts',(-52.5123202735365,12.518720787882,-60.8936385283445));
#141446=CARTESIAN_POINT('Ctrl Pts',(-52.5245819708709,12.4756972986243,
-60.9004583201737));
#141447=CARTESIAN_POINT('Ctrl Pts',(-52.81219032515,12.5218539749099,-60.5055220850798));
#141448=CARTESIAN_POINT('Ctrl Pts',(-52.7486445377005,12.4996864767879,
-60.660571058145));
#141449=CARTESIAN_POINT('Ctrl Pts',(-52.6505629615106,12.4839221309077,
-60.7971452199062));
#141450=CARTESIAN_POINT('Ctrl Pts',(-52.5245819708686,12.4756972986232,
-60.9004583201709));
#141451=CARTESIAN_POINT('Origin',(0.,-12.9675000200281,-61.64995));
#141452=CARTESIAN_POINT('',(-49.1629069712534,18.0283224583225,-61.2273317382593));
#141453=CARTESIAN_POINT('',(-52.2790965136749,12.4220352393542,-61.2273317382593));
#141454=CARTESIAN_POINT('Origin',(0.,-12.9675000200281,-61.2273317382593));
#141455=CARTESIAN_POINT('Origin',(-53.868230923887,12.7669411850502,-62.1522526801527));
#141456=CARTESIAN_POINT('',(-50.0811190791972,18.26999998,-60.64995));
#141457=CARTESIAN_POINT('Origin',(0.,-12.9675000200281,-60.64995));
#141458=CARTESIAN_POINT('Ctrl Pts',(-49.1629069712534,18.0283224583225,
-61.2273317382593));
#141459=CARTESIAN_POINT('Ctrl Pts',(-49.2072136788996,18.0400790290492,
-61.1335104039183));
#141460=CARTESIAN_POINT('Ctrl Pts',(-49.2636489250068,18.0550404895701,
-61.0510932718963));
#141461=CARTESIAN_POINT('Ctrl Pts',(-49.3970153298707,18.0903238932961,
-60.9057963508575));
#141462=CARTESIAN_POINT('Ctrl Pts',(-49.4723725947842,18.1102284712985,
-60.8450701877959));
#141463=CARTESIAN_POINT('Ctrl Pts',(-49.7151670266325,18.1742094267258,
-60.6988289354793));
#141464=CARTESIAN_POINT('Ctrl Pts',(-49.897617121419,18.2220908968247,-60.64995));
#141465=CARTESIAN_POINT('Ctrl Pts',(-50.0811190791972,18.26999998,-60.64995));
#141466=CARTESIAN_POINT('Origin',(0.,-12.9675000200281,-60.64995));
#141467=CARTESIAN_POINT('',(-1.30574517062348E-14,18.26999998,-60.64995));
#141468=CARTESIAN_POINT('Ctrl Pts',(-52.4026162823651,18.2264221086262,
-59.64995));
#141469=CARTESIAN_POINT('Ctrl Pts',(-52.3550593808763,18.76999998,-59.64995));
#141470=CARTESIAN_POINT('Ctrl Pts',(-52.900713631411,18.76999998,-59.64995));
#141471=CARTESIAN_POINT('Ctrl Pts',(-52.402616282365,18.2264221086281,-59.7808732880371));
#141472=CARTESIAN_POINT('Ctrl Pts',(-52.3550593808723,18.76999998,-59.7746029379313));
#141473=CARTESIAN_POINT('Ctrl Pts',(-52.9007136313967,18.76999998,-59.8463349320561));
#141474=CARTESIAN_POINT('Ctrl Pts',(-52.3763903041667,18.2275563241362,
-59.9116978933078));
#141475=CARTESIAN_POINT('Ctrl Pts',(-52.3316386425403,18.76999998,-59.8989712332646));
#141476=CARTESIAN_POINT('Ctrl Pts',(-52.8615235106123,18.76999998,-60.0425718399612));
#141477=CARTESIAN_POINT('Ctrl Pts',(-52.2754393607673,18.2319222289985,
-60.1535689714224));
#141478=CARTESIAN_POINT('Ctrl Pts',(-52.239810099313,18.76999998,-60.1322291512602));
#141479=CARTESIAN_POINT('Ctrl Pts',(-52.710670046285,18.76999998,-60.4053784571341));
#141480=CARTESIAN_POINT('Ctrl Pts',(-52.2007540936325,18.2351522014976,
-60.2644967268053));
#141481=CARTESIAN_POINT('Ctrl Pts',(-52.1717434473124,18.7699999799997,
-60.2406767152624));
#141482=CARTESIAN_POINT('Ctrl Pts',(-52.5990660245491,18.76999998,-60.5717700902076));
#141483=CARTESIAN_POINT('Ctrl Pts',(-52.0142210728062,18.2432193417862,
-60.4496168355678));
#141484=CARTESIAN_POINT('Ctrl Pts',(-51.9977165994394,18.7699999800003,
-60.4261994932772));
#141485=CARTESIAN_POINT('Ctrl Pts',(-52.3203251682923,18.76999998,-60.8494502533521));
#141486=CARTESIAN_POINT('Ctrl Pts',(-51.9024466716657,18.2480533372399,
-60.5237363920407));
#141487=CARTESIAN_POINT('Ctrl Pts',(-51.8922860151588,18.7699999800003,
-60.5031527166051));
#141488=CARTESIAN_POINT('Ctrl Pts',(-52.1532979462845,18.76999998,-60.9606295880612));
#141489=CARTESIAN_POINT('Ctrl Pts',(-51.6587295348784,18.2585935639752,
-60.6239226729819));
#141490=CARTESIAN_POINT('Ctrl Pts',(-51.657019042446,18.7699999799997,-60.6120353079393));
#141491=CARTESIAN_POINT('Ctrl Pts',(-51.7891054666292,18.76999998,-61.1109090094727));
#141492=CARTESIAN_POINT('Ctrl Pts',(-51.5269064230252,18.264294621793,-60.64995));
#141493=CARTESIAN_POINT('Ctrl Pts',(-51.5277022966008,18.7699999800007,
-60.6442102195358));
#141494=CARTESIAN_POINT('Ctrl Pts',(-51.592118965743,18.76999998,-61.149949999985));
#141495=CARTESIAN_POINT('Ctrl Pts',(-51.394983875096,18.26999998,-60.64995));
#141496=CARTESIAN_POINT('Ctrl Pts',(-51.394983875096,18.76999998,-60.64995));
#141497=CARTESIAN_POINT('Ctrl Pts',(-51.394983875096,18.76999998,-61.14995));
#141498=CARTESIAN_POINT('',(-51.394983875096,18.76999998,-61.14995));
#141499=CARTESIAN_POINT('Origin',(-51.394983875096,18.26999998,-61.14995));
#141500=CARTESIAN_POINT('Ctrl Pts',(-52.900713631411,18.76999998,-59.64995));
#141501=CARTESIAN_POINT('Ctrl Pts',(-52.9007136313967,18.76999998,-59.8463349320561));
#141502=CARTESIAN_POINT('Ctrl Pts',(-52.8615235106123,18.76999998,-60.0425718399612));
#141503=CARTESIAN_POINT('Ctrl Pts',(-52.710670046285,18.76999998,-60.4053784571341));
#141504=CARTESIAN_POINT('Ctrl Pts',(-52.5990660245491,18.76999998,-60.5717700902076));
#141505=CARTESIAN_POINT('Ctrl Pts',(-52.3203251682923,18.76999998,-60.8494502533521));
#141506=CARTESIAN_POINT('Ctrl Pts',(-52.1532979462845,18.76999998,-60.9606295880612));
#141507=CARTESIAN_POINT('Ctrl Pts',(-51.7891054666292,18.76999998,-61.1109090094727));
#141508=CARTESIAN_POINT('Ctrl Pts',(-51.592118965743,18.76999998,-61.149949999985));
#141509=CARTESIAN_POINT('Ctrl Pts',(-51.394983875096,18.76999998,-61.14995));
#141510=CARTESIAN_POINT('Origin',(83.2809572255632,18.7699999800001,-55.24995));
#141511=CARTESIAN_POINT('',(-57.,18.76999998,-55.74995));
#141512=CARTESIAN_POINT('',(83.2809572255632,18.7699999800001,-55.74995));
#141513=CARTESIAN_POINT('',(-59.5,18.76999998,-58.24995));
#141514=CARTESIAN_POINT('Origin',(-57.,18.76999998,-58.24995));
#141515=CARTESIAN_POINT('',(-59.5,18.76999998,-174.34995));
#141516=CARTESIAN_POINT('',(-59.5,18.76999998,-58.24995));
#141517=CARTESIAN_POINT('',(-57.,18.76999998,-176.84995));
#141518=CARTESIAN_POINT('Origin',(-57.,18.76999998,-174.34995));
#141519=CARTESIAN_POINT('',(-52.3218461808875,18.76999998,-176.84995));
#141520=CARTESIAN_POINT('',(83.2809572255632,18.7699999800001,-176.84995));
#141521=CARTESIAN_POINT('',(-52.3218461808875,18.76999998,-172.64995));
#141522=CARTESIAN_POINT('',(-52.3218461808875,18.76999998,-55.24995));
#141523=CARTESIAN_POINT('',(-50.8071048221096,18.76999998,-171.14995));
#141524=CARTESIAN_POINT('Ctrl Pts',(-50.8071048221096,18.76999998,-171.14995));
#141525=CARTESIAN_POINT('Ctrl Pts',(-51.0054197414846,18.76999998,-171.149950000016));
#141526=CARTESIAN_POINT('Ctrl Pts',(-51.2035851814656,18.76999998,-171.18899099047));
#141527=CARTESIAN_POINT('Ctrl Pts',(-51.5699573073986,18.76999998,-171.339270411997));
#141528=CARTESIAN_POINT('Ctrl Pts',(-51.7379841660413,18.76999998,-171.450449746589));
#141529=CARTESIAN_POINT('Ctrl Pts',(-52.0183932512491,18.76999998,-171.728129909852));
#141530=CARTESIAN_POINT('Ctrl Pts',(-52.1306652088914,18.76999998,-171.894521542842));
#141531=CARTESIAN_POINT('Ctrl Pts',(-52.2824215121743,18.76999998,-172.257328160063));
#141532=CARTESIAN_POINT('Ctrl Pts',(-52.3218461808705,18.76999998,-172.453565067926));
#141533=CARTESIAN_POINT('Ctrl Pts',(-52.3218461808875,18.76999998,-172.64995));
#141534=CARTESIAN_POINT('',(-50.2136602208993,18.76999998,-171.14995));
#141535=CARTESIAN_POINT('',(-50.7368344047584,18.76999998,-171.14995));
#141536=CARTESIAN_POINT('',(-49.6791770659623,18.76999998,-170.861259130871));
#141537=CARTESIAN_POINT('Ctrl Pts',(-49.6791770659623,18.76999998,-170.861259130871));
#141538=CARTESIAN_POINT('Ctrl Pts',(-49.6968576580123,18.76999998,-170.89335724814));
#141539=CARTESIAN_POINT('Ctrl Pts',(-49.7180606234586,18.76999998,-170.923027065572));
#141540=CARTESIAN_POINT('Ctrl Pts',(-49.742166968171,18.76999998,-170.95020183613));
#141541=CARTESIAN_POINT('Ctrl Pts',(-49.7534002577179,18.76999998,-170.962864978123));
#141542=CARTESIAN_POINT('Ctrl Pts',(-49.7652647303595,18.76999998,-170.974986007307));
#141543=CARTESIAN_POINT('Ctrl Pts',(-49.7777010515148,18.76999998,-170.986556367076));
#141544=CARTESIAN_POINT('Ctrl Pts',(-49.8071230954838,18.76999998,-171.013929705992));
#141545=CARTESIAN_POINT('Ctrl Pts',(-49.8388986066917,18.76999998,-171.037546210365));
#141546=CARTESIAN_POINT('Ctrl Pts',(-49.8728019101419,18.76999998,-171.057883544606));
#141547=CARTESIAN_POINT('Ctrl Pts',(-49.8840707206927,18.76999998,-171.064643286087));
#141548=CARTESIAN_POINT('Ctrl Pts',(-49.8955748425991,18.76999998,-171.071040378572));
#141549=CARTESIAN_POINT('Ctrl Pts',(-49.9073066431081,18.76999998,-171.07709133376));
#141550=CARTESIAN_POINT('Ctrl Pts',(-49.9542902216173,18.76999998,-171.101324232019));
#141551=CARTESIAN_POINT('Ctrl Pts',(-50.0051782135404,18.76999998,-171.119773228097));
#141552=CARTESIAN_POINT('Ctrl Pts',(-50.0564485939595,18.76999998,-171.131817408419));
#141553=CARTESIAN_POINT('Ctrl Pts',(-50.1077152012182,18.76999998,-171.143860702368));
#141554=CARTESIAN_POINT('Ctrl Pts',(-50.1601164670163,18.76999998,-171.14995));
#141555=CARTESIAN_POINT('Ctrl Pts',(-50.2136602208993,18.76999998,-171.14995));
#141556=CARTESIAN_POINT('',(-40.7628307834967,18.76999998,-155.145469613787));
#141557=CARTESIAN_POINT('Ctrl Pts',(-40.7628307834967,18.76999998,-155.145469613787));
#141558=CARTESIAN_POINT('Ctrl Pts',(-43.8140512781903,18.76999998,-160.339185894338));
#141559=CARTESIAN_POINT('Ctrl Pts',(-46.7729974319751,18.76999998,-165.585253981682));
#141560=CARTESIAN_POINT('Ctrl Pts',(-49.6791770659623,18.76999998,-170.861259130871));
#141561=CARTESIAN_POINT('',(-39.5,18.76999998,-150.084863924608));
#141562=CARTESIAN_POINT('Ctrl Pts',(-39.5,18.76999998,-150.084863924608));
#141563=CARTESIAN_POINT('Ctrl Pts',(-39.5,18.76999998,-150.526736484781));
#141564=CARTESIAN_POINT('Ctrl Pts',(-39.5253915082895,18.76999998,-150.965860868514));
#141565=CARTESIAN_POINT('Ctrl Pts',(-39.5759031870658,18.76999998,-151.402266443275));
#141566=CARTESIAN_POINT('Ctrl Pts',(-39.6264148658422,18.76999998,-151.838672018036));
#141567=CARTESIAN_POINT('Ctrl Pts',(-39.7023798052339,18.76999998,-152.273874561637));
#141568=CARTESIAN_POINT('Ctrl Pts',(-39.8051549665992,18.76999998,-152.702666397218));
#141569=CARTESIAN_POINT('Ctrl Pts',(-39.9079301279644,18.76999998,-153.131458232799));
#141570=CARTESIAN_POINT('Ctrl Pts',(-40.0364383090913,18.76999998,-153.550444480149));
#141571=CARTESIAN_POINT('Ctrl Pts',(-40.1940856267786,18.76999998,-153.958327235804));
#141572=CARTESIAN_POINT('Ctrl Pts',(-40.3268328904701,18.76999998,-154.301785789457));
#141573=CARTESIAN_POINT('Ctrl Pts',(-40.4800174576556,18.76999998,-154.637456687643));
#141574=CARTESIAN_POINT('Ctrl Pts',(-40.6592112617779,18.76999998,-154.963216752245));
#141575=CARTESIAN_POINT('Ctrl Pts',(-40.6928235206997,18.76999998,-155.024321162029));
#141576=CARTESIAN_POINT('Ctrl Pts',(-40.727351034357,18.76999998,-155.085076813253));
#141577=CARTESIAN_POINT('Ctrl Pts',(-40.7628307834967,18.76999998,-155.145469613787));
#141578=CARTESIAN_POINT('',(-39.5,18.76999998,-81.9737790469184));
#141579=CARTESIAN_POINT('',(-39.5,18.76999998,-55.24995));
#141580=CARTESIAN_POINT('',(-40.7628307834967,18.76999998,-76.9131733577189));
#141581=CARTESIAN_POINT('Ctrl Pts',(-40.7628307834967,18.76999998,-76.913173357719));
#141582=CARTESIAN_POINT('Ctrl Pts',(-40.5548564785642,18.76999998,-77.2671823633761));
#141583=CARTESIAN_POINT('Ctrl Pts',(-40.3788354530891,18.76999998,-77.6350438334276));
#141584=CARTESIAN_POINT('Ctrl Pts',(-40.2280138947791,18.76999998,-78.0138298371173));
#141585=CARTESIAN_POINT('Ctrl Pts',(-40.2160748553596,18.76999998,-78.0438145493842));
#141586=CARTESIAN_POINT('Ctrl Pts',(-40.2042937476386,18.76999998,-78.0738677286071));
#141587=CARTESIAN_POINT('Ctrl Pts',(-40.1926672329271,18.76999998,-78.1039879273901));
#141588=CARTESIAN_POINT('Ctrl Pts',(-40.0341671712826,18.76999998,-78.5146056819203));
#141589=CARTESIAN_POINT('Ctrl Pts',(-39.9044907334798,18.76999998,-78.9396134648084));
#141590=CARTESIAN_POINT('Ctrl Pts',(-39.802619647733,18.76999998,-79.366578420212));
#141591=CARTESIAN_POINT('Ctrl Pts',(-39.689990788524,18.76999998,-79.8386316578583));
#141592=CARTESIAN_POINT('Ctrl Pts',(-39.6094172115555,18.76999998,-80.315401745757));
#141593=CARTESIAN_POINT('Ctrl Pts',(-39.5598665237953,18.76999998,-80.7967368113115));
#141594=CARTESIAN_POINT('Ctrl Pts',(-39.5197815285328,18.76999998,-81.1861222001843));
#141595=CARTESIAN_POINT('Ctrl Pts',(-39.4999999999993,18.76999998,-81.57849522885));
#141596=CARTESIAN_POINT('Ctrl Pts',(-39.5,18.76999998,-81.9737790469184));
#141597=CARTESIAN_POINT('',(-49.5462350640495,18.76999998,-61.4386408691297));
#141598=CARTESIAN_POINT('Ctrl Pts',(-49.5462350640495,18.76999998,-61.4386408691297));
#141599=CARTESIAN_POINT('Ctrl Pts',(-46.6826907236407,18.76999998,-66.6332909352423));
#141600=CARTESIAN_POINT('Ctrl Pts',(-43.7675305143725,18.76999998,-71.7986436352564));
#141601=CARTESIAN_POINT('Ctrl Pts',(-40.7628307834967,18.76999998,-76.9131733577189));
#141602=CARTESIAN_POINT('',(-50.0811190791972,18.76999998,-61.14995));
#141603=CARTESIAN_POINT('Ctrl Pts',(-50.0811190791972,18.76999998,-61.14995));
#141604=CARTESIAN_POINT('Ctrl Pts',(-50.0253653304666,18.76999998,-61.14995));
#141605=CARTESIAN_POINT('Ctrl Pts',(-49.9698122997694,18.76999998,-61.156619759286));
#141606=CARTESIAN_POINT('Ctrl Pts',(-49.9160272892489,18.76999998,-61.1699168656485));
#141607=CARTESIAN_POINT('Ctrl Pts',(-49.8667673647605,18.76999998,-61.182095248603));
#141608=CARTESIAN_POINT('Ctrl Pts',(-49.8189890147707,18.76999998,-61.1998333372795));
#141609=CARTESIAN_POINT('Ctrl Pts',(-49.7739018815406,18.76999998,-61.2231365482226));
#141610=CARTESIAN_POINT('Ctrl Pts',(-49.7267405569306,18.76999998,-61.2475118015822));
#141611=CARTESIAN_POINT('Ctrl Pts',(-49.6828095888518,18.76999998,-61.2778731395778));
#141612=CARTESIAN_POINT('Ctrl Pts',(-49.6439176192587,18.76999998,-61.3141973629269));
#141613=CARTESIAN_POINT('Ctrl Pts',(-49.6050311049514,18.76999998,-61.3505164911619));
#141614=CARTESIAN_POINT('Ctrl Pts',(-49.572103750808,18.76999998,-61.391713439551));
#141615=CARTESIAN_POINT('Ctrl Pts',(-49.5462350640495,18.76999998,-61.4386408691297));
#141616=CARTESIAN_POINT('',(83.2809572255632,18.7699999800001,-61.14995));
#141617=CARTESIAN_POINT('Origin',(-60.,19.26999998,-55.74995));
#141618=CARTESIAN_POINT('',(-57.,19.26999998,-55.24995));
#141619=CARTESIAN_POINT('',(-60.,19.26999998,-55.24995));
#141620=CARTESIAN_POINT('Origin',(-57.,19.26999998,-55.74995));
#141621=CARTESIAN_POINT('Origin',(-60.,28.41999998,-55.24995));
#141622=CARTESIAN_POINT('',(-57.,19.76999998,-55.24995));
#141623=CARTESIAN_POINT('',(-60.,19.76999998,-55.24995));
#141624=CARTESIAN_POINT('',(-57.,28.41999998,-55.24995));
#141625=CARTESIAN_POINT('Origin',(83.2809572255632,19.7699999800001,-55.74995));
#141626=CARTESIAN_POINT('',(-57.,20.26999998,-55.74995));
#141627=CARTESIAN_POINT('',(83.2809572255632,20.2699999800001,-55.74995));
#141628=CARTESIAN_POINT('Origin',(-57.,19.76999998,-55.74995));
#141629=CARTESIAN_POINT('Origin',(83.2809572255632,20.2699999800001,-55.24995));
#141630=CARTESIAN_POINT('',(-57.,20.26999998,-176.84995));
#141631=CARTESIAN_POINT('',(-51.9704940941315,20.26999998,-176.84995));
#141632=CARTESIAN_POINT('',(83.2809572255632,20.2699999800001,-176.84995));
#141633=CARTESIAN_POINT('',(-59.5,20.26999998,-174.34995));
#141634=CARTESIAN_POINT('Origin',(-57.,20.26999998,-174.34995));
#141635=CARTESIAN_POINT('',(-59.5,20.26999998,-58.24995));
#141636=CARTESIAN_POINT('',(-59.5,20.26999998,-174.34995));
#141637=CARTESIAN_POINT('Origin',(-57.,20.26999998,-58.24995));
#141638=CARTESIAN_POINT('',(-48.4322308821779,20.26999998,-61.14995));
#141639=CARTESIAN_POINT('',(83.2809572255632,20.2699999800001,-61.14995));
#141640=CARTESIAN_POINT('',(-47.878929697957,20.26999998,-61.4386408691297));
#141641=CARTESIAN_POINT('Ctrl Pts',(-47.878929697957,20.26999998,-61.4386408691297));
#141642=CARTESIAN_POINT('Ctrl Pts',(-47.8974331987387,20.26999998,-61.4062039153375));
#141643=CARTESIAN_POINT('Ctrl Pts',(-47.9195379615588,20.26999998,-61.3763755387995));
#141644=CARTESIAN_POINT('Ctrl Pts',(-47.9444691614869,20.26999998,-61.3492604871258));
#141645=CARTESIAN_POINT('Ctrl Pts',(-47.9720805388406,20.26999998,-61.3192304875314));
#141646=CARTESIAN_POINT('Ctrl Pts',(-48.0031577468356,20.26999998,-61.2925292835123));
#141647=CARTESIAN_POINT('Ctrl Pts',(-48.0365924563163,20.26999998,-61.2692603439468));
#141648=CARTESIAN_POINT('Ctrl Pts',(-48.0621704908693,20.26999998,-61.2514592698696));
#141649=CARTESIAN_POINT('Ctrl Pts',(-48.089126771587,20.26999998,-61.2356661036976));
#141650=CARTESIAN_POINT('Ctrl Pts',(-48.1169536143029,20.26999998,-61.2219104511051));
#141651=CARTESIAN_POINT('Ctrl Pts',(-48.1430951909369,20.26999998,-61.2089878766662));
#141652=CARTESIAN_POINT('Ctrl Pts',(-48.1700747212765,20.26999998,-61.1978560977682));
#141653=CARTESIAN_POINT('Ctrl Pts',(-48.1976781569078,20.26999998,-61.1884510370574));
#141654=CARTESIAN_POINT('Ctrl Pts',(-48.2258927336205,20.26999998,-61.1788377479562));
#141655=CARTESIAN_POINT('Ctrl Pts',(-48.2547605141934,20.26999998,-61.171028311645));
#141656=CARTESIAN_POINT('Ctrl Pts',(-48.284075038586,20.26999998,-61.1650052516751));
#141657=CARTESIAN_POINT('Ctrl Pts',(-48.3128848180532,20.26999998,-61.1590858982813));
#141658=CARTESIAN_POINT('Ctrl Pts',(-48.3421274958272,20.26999998,-61.1548920321836));
#141659=CARTESIAN_POINT('Ctrl Pts',(-48.3716073656787,20.26999998,-61.1524557732793));
#141660=CARTESIAN_POINT('Ctrl Pts',(-48.3917271240067,20.26999998,-61.1507930474726));
#141661=CARTESIAN_POINT('Ctrl Pts',(-48.4119573716394,20.26999998,-61.14995));
#141662=CARTESIAN_POINT('Ctrl Pts',(-48.4322308821779,20.26999998,-61.14995));
#141663=CARTESIAN_POINT('',(-40.8552491802306,20.26999998,-73.4195575571114));
#141664=CARTESIAN_POINT('Ctrl Pts',(-40.8552491802306,20.26999998,-73.4195575571114));
#141665=CARTESIAN_POINT('Ctrl Pts',(-43.2510477030711,20.26999998,-69.4579107098797));
#141666=CARTESIAN_POINT('Ctrl Pts',(-45.5849708137067,20.26999998,-65.4599900833935));
#141667=CARTESIAN_POINT('Ctrl Pts',(-47.878929697957,20.26999998,-61.4386408691297));
#141668=CARTESIAN_POINT('',(-39.5,20.26999998,-78.7897987614789));
#141669=CARTESIAN_POINT('Ctrl Pts',(-39.5,20.26999998,-78.7897987614789));
#141670=CARTESIAN_POINT('Ctrl Pts',(-39.4999999999996,20.26999998,-78.4276754534817));
#141671=CARTESIAN_POINT('Ctrl Pts',(-39.5156108303728,20.26999998,-78.0671937952878));
#141672=CARTESIAN_POINT('Ctrl Pts',(-39.5473687221685,20.26999998,-77.7085899056884));
#141673=CARTESIAN_POINT('Ctrl Pts',(-39.5782679790921,20.26999998,-77.3596815527725));
#141674=CARTESIAN_POINT('Ctrl Pts',(-39.6244528955629,20.26999998,-77.0125506150128));
#141675=CARTESIAN_POINT('Ctrl Pts',(-39.686466172093,20.26999998,-76.6674187362246));
#141676=CARTESIAN_POINT('Ctrl Pts',(-39.7259630317165,20.26999998,-76.447600882196));
#141677=CARTESIAN_POINT('Ctrl Pts',(-39.7718817094826,20.26999998,-76.2285940465893));
#141678=CARTESIAN_POINT('Ctrl Pts',(-39.8243734219799,20.26999998,-76.0104569305838));
#141679=CARTESIAN_POINT('Ctrl Pts',(-39.9341806286948,20.26999998,-75.5541367564111));
#141680=CARTESIAN_POINT('Ctrl Pts',(-40.0717001000673,20.26999998,-75.1087680536983));
#141681=CARTESIAN_POINT('Ctrl Pts',(-40.2410990749131,20.26999998,-74.6759976525381));
#141682=CARTESIAN_POINT('Ctrl Pts',(-40.3724674808339,20.26999998,-74.3403854814384));
#141683=CARTESIAN_POINT('Ctrl Pts',(-40.5227478579483,20.26999998,-74.0122470450345));
#141684=CARTESIAN_POINT('Ctrl Pts',(-40.6973553853198,20.26999998,-73.6937223220025));
#141685=CARTESIAN_POINT('Ctrl Pts',(-40.747903487491,20.26999998,-73.6015108321186));
#141686=CARTESIAN_POINT('Ctrl Pts',(-40.8004906856034,20.26999998,-73.5101051618135));
#141687=CARTESIAN_POINT('Ctrl Pts',(-40.8552491802306,20.26999998,-73.4195575571114));
#141688=CARTESIAN_POINT('',(-39.5,20.26999998,-153.26884421004));
#141689=CARTESIAN_POINT('',(-39.5,20.26999998,-55.24995));
#141690=CARTESIAN_POINT('',(-40.8552491802207,20.26999998,-158.639085414378));
#141691=CARTESIAN_POINT('Ctrl Pts',(-40.8552491802207,20.26999998,-158.639085414378));
#141692=CARTESIAN_POINT('Ctrl Pts',(-40.6523563182981,20.26999998,-158.303585638801));
#141693=CARTESIAN_POINT('Ctrl Pts',(-40.4787269326741,20.26999998,-157.955339387341));
#141694=CARTESIAN_POINT('Ctrl Pts',(-40.3280973119502,20.26999998,-157.59707498981));
#141695=CARTESIAN_POINT('Ctrl Pts',(-40.2977909470182,20.26999998,-157.52499294166));
#141696=CARTESIAN_POINT('Ctrl Pts',(-40.2684157827682,20.26999998,-157.452505284515));
#141697=CARTESIAN_POINT('Ctrl Pts',(-40.2399210161217,20.26999998,-157.379634146926));
#141698=CARTESIAN_POINT('Ctrl Pts',(-40.0698006898873,20.26999998,-156.944576655372));
#141699=CARTESIAN_POINT('Ctrl Pts',(-39.9310881570986,20.26999998,-156.493265246319));
#141700=CARTESIAN_POINT('Ctrl Pts',(-39.8222693035353,20.26999998,-156.039426370008));
#141701=CARTESIAN_POINT('Ctrl Pts',(-39.7053251420368,20.26999998,-155.551700161656));
#141702=CARTESIAN_POINT('Ctrl Pts',(-39.6210196491341,20.26999998,-155.059280307642));
#141703=CARTESIAN_POINT('Ctrl Pts',(-39.5680311845015,20.26999998,-154.562356823708));
#141704=CARTESIAN_POINT('Ctrl Pts',(-39.5224060219208,20.26999998,-154.134486061611));
#141705=CARTESIAN_POINT('Ctrl Pts',(-39.5,20.26999998,-153.703276192992));
#141706=CARTESIAN_POINT('Ctrl Pts',(-39.5,20.26999998,-153.26884421004));
#141707=CARTESIAN_POINT('',(-48.0164881467928,20.26999998,-170.861259130871));
#141708=CARTESIAN_POINT('Ctrl Pts',(-48.0164881467928,20.26999998,-170.861259130871));
#141709=CARTESIAN_POINT('Ctrl Pts',(-45.678332174125,20.26999998,-166.758535769278));
#141710=CARTESIAN_POINT('Ctrl Pts',(-43.29896123138,20.26999998,-162.67996116032));
#141711=CARTESIAN_POINT('Ctrl Pts',(-40.8552491802207,20.26999998,-158.639085414378));
#141712=CARTESIAN_POINT('',(-48.5692718988023,20.26999998,-171.14995));
#141713=CARTESIAN_POINT('Ctrl Pts',(-48.5692718988023,20.26999998,-171.14995));
#141714=CARTESIAN_POINT('Ctrl Pts',(-48.5047948684865,20.26999998,-171.14995));
#141715=CARTESIAN_POINT('Ctrl Pts',(-48.4405703346684,20.26999998,-171.141645130581));
#141716=CARTESIAN_POINT('Ctrl Pts',(-48.3787338163772,20.26999998,-171.124930042695));
#141717=CARTESIAN_POINT('Ctrl Pts',(-48.3356628951272,20.26999998,-171.113287501137));
#141718=CARTESIAN_POINT('Ctrl Pts',(-48.2937500450322,20.26999998,-171.097563680328));
#141719=CARTESIAN_POINT('Ctrl Pts',(-48.2537194844918,20.26999998,-171.077708139862));
#141720=CARTESIAN_POINT('Ctrl Pts',(-48.2190067257619,20.26999998,-171.060490279898));
#141721=CARTESIAN_POINT('Ctrl Pts',(-48.1858587814808,20.26999998,-171.04016650214));
#141722=CARTESIAN_POINT('Ctrl Pts',(-48.1550885346334,20.26999998,-171.016846515546));
#141723=CARTESIAN_POINT('Ctrl Pts',(-48.1271078573602,20.26999998,-170.995640672703));
#141724=CARTESIAN_POINT('Ctrl Pts',(-48.1010921834767,20.26999998,-170.971956505702));
#141725=CARTESIAN_POINT('Ctrl Pts',(-48.0776779540561,20.26999998,-170.945845192498));
#141726=CARTESIAN_POINT('Ctrl Pts',(-48.0545175809105,20.26999998,-170.920016977258));
#141727=CARTESIAN_POINT('Ctrl Pts',(-48.033901319099,20.26999998,-170.891813734436));
#141728=CARTESIAN_POINT('Ctrl Pts',(-48.0164881467928,20.26999998,-170.861259130871));
#141729=CARTESIAN_POINT('',(-50.4557527353536,20.26999998,-171.14995));
#141730=CARTESIAN_POINT('',(-48.9127966158122,20.26999998,-171.14995));
#141731=CARTESIAN_POINT('',(-51.9704940941315,20.26999998,-172.64995));
#141732=CARTESIAN_POINT('Ctrl Pts',(-51.9704940941315,20.26999998,-172.64995));
#141733=CARTESIAN_POINT('Ctrl Pts',(-51.9704940941145,20.26999998,-172.453565067926));
#141734=CARTESIAN_POINT('Ctrl Pts',(-51.9310694254183,20.26999998,-172.257328160063));
#141735=CARTESIAN_POINT('Ctrl Pts',(-51.7793131221354,20.26999998,-171.894521542842));
#141736=CARTESIAN_POINT('Ctrl Pts',(-51.6670411644938,20.26999998,-171.728129909852));
#141737=CARTESIAN_POINT('Ctrl Pts',(-51.3866320792846,20.26999998,-171.450449746589));
#141738=CARTESIAN_POINT('Ctrl Pts',(-51.2186052206426,20.26999998,-171.339270411997));
#141739=CARTESIAN_POINT('Ctrl Pts',(-50.8522330947096,20.26999998,-171.18899099047));
#141740=CARTESIAN_POINT('Ctrl Pts',(-50.6540676547286,20.26999998,-171.149950000016));
#141741=CARTESIAN_POINT('Ctrl Pts',(-50.4557527353536,20.26999998,-171.14995));
#141742=CARTESIAN_POINT('',(-51.9704940941315,20.26999998,-55.24995));
#141743=CARTESIAN_POINT('Origin',(0.,-12.9675000200281,-61.64995));
#141744=CARTESIAN_POINT('',(-52.1700794675439,-38.5802945048887,-61.2273317382593));
#141745=CARTESIAN_POINT('',(-49.0214378669496,-44.1865817238571,-61.2273317382593));
#141746=CARTESIAN_POINT('Origin',(0.,-12.9675000200281,-61.2273317382593));
#141747=CARTESIAN_POINT('',(-49.940073970993,-44.43000002,-60.64995));
#141748=CARTESIAN_POINT('Ctrl Pts',(-49.940073970993,-44.43000002,-60.64995));
#141749=CARTESIAN_POINT('Ctrl Pts',(-49.847975325787,-44.405792727464,-60.64995));
#141750=CARTESIAN_POINT('Ctrl Pts',(-49.7578576522452,-44.382047471718,
-60.6621027778979));
#141751=CARTESIAN_POINT('Ctrl Pts',(-49.581571905815,-44.3354917333839,
-60.7102142267434));
#141752=CARTESIAN_POINT('Ctrl Pts',(-49.494126795535,-44.312341612126,-60.7470666030416));
#141753=CARTESIAN_POINT('Ctrl Pts',(-49.3327124735647,-44.2695203114938,
-60.8438912527599));
#141754=CARTESIAN_POINT('Ctrl Pts',(-49.2581152115204,-44.2496846870305,
-60.9035137960622));
#141755=CARTESIAN_POINT('Ctrl Pts',(-49.1234012768228,-44.2138057335947,
-61.0494267271759));
#141756=CARTESIAN_POINT('Ctrl Pts',(-49.0658454246046,-44.1984444719328,
-61.1333401037095));
#141757=CARTESIAN_POINT('Ctrl Pts',(-49.0214378669496,-44.1865817238571,
-61.2273317382593));
#141758=CARTESIAN_POINT('Origin',(0.,-12.9675000200281,-60.64995));
#141759=CARTESIAN_POINT('Origin',(-53.021204175293,-38.7665567539115,-61.6005868751704));
#141760=CARTESIAN_POINT('Ctrl Pts',(-52.877242281998,-38.7364221486262,
-60.0032396521562));
#141761=CARTESIAN_POINT('Ctrl Pts',(-52.9171740440352,-38.28000002,-60.0032396521562));
#141762=CARTESIAN_POINT('Ctrl Pts',(-53.3753396310439,-38.28000002,-60.0032396521563));
#141763=CARTESIAN_POINT('Ctrl Pts',(-52.8788986395818,-38.7174898948119,
-60.1690974501184));
#141764=CARTESIAN_POINT('Ctrl Pts',(-52.9343465054118,-38.28000002,-60.1721379135101));
#141765=CARTESIAN_POINT('Ctrl Pts',(-53.3753396328414,-38.28000002,-60.244893556147));
#141766=CARTESIAN_POINT('Ctrl Pts',(-52.8422535332614,-38.6982739394415,
-60.3389622441799));
#141767=CARTESIAN_POINT('Ctrl Pts',(-52.9111776732915,-38.28000002,-60.3567456822519));
#141768=CARTESIAN_POINT('Ctrl Pts',(-53.317850201657,-38.28000002,-60.4921247747839));
#141769=CARTESIAN_POINT('Ctrl Pts',(-52.6988044737759,-38.6656865171052,
-60.6372698562504));
#141770=CARTESIAN_POINT('Ctrl Pts',(-52.7751833670329,-38.28000002,-60.6874729542071));
#141771=CARTESIAN_POINT('Ctrl Pts',(-53.0984000724383,-38.28000002,-60.9263821015509));
#141772=CARTESIAN_POINT('Ctrl Pts',(-52.5917711956707,-38.6521075044106,
-60.7679496692827));
#141773=CARTESIAN_POINT('Ctrl Pts',(-52.6635868839933,-38.28000002,-60.8378349680257));
#141774=CARTESIAN_POINT('Ctrl Pts',(-52.9360725977236,-38.28000002,-61.1166772774171));
#141775=CARTESIAN_POINT('Ctrl Pts',(-52.4601060488526,-38.6442121687577,
-60.8635779995784));
#141776=CARTESIAN_POINT('Ctrl Pts',(-52.5193575501106,-38.28000002,-60.9475523661896));
#141777=CARTESIAN_POINT('Ctrl Pts',(-52.7375342894721,-38.28000002,-61.2567639997892));
#141778=CARTESIAN_POINT('',(-52.7375342894721,-38.28000002,-61.2567639997892));
#141779=CARTESIAN_POINT('Ctrl Pts',(-53.3753396310439,-38.28000002,-60.0032396521563));
#141780=CARTESIAN_POINT('Ctrl Pts',(-53.3753396310439,-38.28000002,-60.0589758767835));
#141781=CARTESIAN_POINT('Ctrl Pts',(-53.3722852139107,-38.28000002,-60.1146939077158));
#141782=CARTESIAN_POINT('Ctrl Pts',(-53.3663204826485,-38.28000002,-60.1700562792009));
#141783=CARTESIAN_POINT('Ctrl Pts',(-53.3600346473475,-38.28000002,-60.2283990164901));
#141784=CARTESIAN_POINT('Ctrl Pts',(-53.3505169273235,-38.28000002,-60.2863478004802));
#141785=CARTESIAN_POINT('Ctrl Pts',(-53.3378827651207,-38.28000002,-60.3435292248105));
#141786=CARTESIAN_POINT('Ctrl Pts',(-53.3251015247972,-38.28000002,-60.4013763154742));
#141787=CARTESIAN_POINT('Ctrl Pts',(-53.3091307297629,-38.28000002,-60.458439390228));
#141788=CARTESIAN_POINT('Ctrl Pts',(-53.2900367865638,-38.2800000200001,
-60.514335009952));
#141789=CARTESIAN_POINT('Ctrl Pts',(-53.2713085336432,-38.2800000200001,
-60.5691601077553));
#141790=CARTESIAN_POINT('Ctrl Pts',(-53.2495752764748,-38.2800000200002,
-60.6228632354968));
#141791=CARTESIAN_POINT('Ctrl Pts',(-53.2248527900284,-38.2800000200003,
-60.6750669890667));
#141792=CARTESIAN_POINT('Ctrl Pts',(-53.2194501346316,-38.2800000200003,
-60.6864751818296));
#141793=CARTESIAN_POINT('Ctrl Pts',(-53.2139045547126,-38.2800000200004,
-60.6978116715983));
#141794=CARTESIAN_POINT('Ctrl Pts',(-53.2082159323665,-38.2800000200004,
-60.7090723322489));
#141795=CARTESIAN_POINT('Ctrl Pts',(-53.2081854825349,-38.2800000200004,
-60.7091326078656));
#141796=CARTESIAN_POINT('Ctrl Pts',(-53.2081550286956,-38.2800000200004,
-60.7091928811299));
#141797=CARTESIAN_POINT('Ctrl Pts',(-53.2081245708486,-38.2800000200004,
-60.7092531520411));
#141798=CARTESIAN_POINT('Ctrl Pts',(-53.1761754390121,-38.2800000200006,
-60.7724750628699));
#141799=CARTESIAN_POINT('Ctrl Pts',(-53.1397892479681,-38.2800000200007,
-60.833387133241));
#141800=CARTESIAN_POINT('Ctrl Pts',(-53.0993211720575,-38.2800000200006,
-60.8914909948822));
#141801=CARTESIAN_POINT('Ctrl Pts',(-53.0593989894049,-38.2800000200005,
-60.948811065705));
#141802=CARTESIAN_POINT('Ctrl Pts',(-53.0155035526423,-38.2800000200003,
-61.003399073172));
#141803=CARTESIAN_POINT('Ctrl Pts',(-52.9679386190619,-38.2800000200002,
-61.0547432417688));
#141804=CARTESIAN_POINT('Ctrl Pts',(-52.9223553337123,-38.2800000200001,
-61.103948311807));
#141805=CARTESIAN_POINT('Ctrl Pts',(-52.8734012103222,-38.28000002,-61.1501747492911));
#141806=CARTESIAN_POINT('Ctrl Pts',(-52.8213200539946,-38.28000002,-61.1929312639283));
#141807=CARTESIAN_POINT('Ctrl Pts',(-52.7942271507162,-38.28000002,-61.2151734374372));
#141808=CARTESIAN_POINT('Ctrl Pts',(-52.7662877001538,-38.28000002,-61.2364758695292));
#141809=CARTESIAN_POINT('Ctrl Pts',(-52.7375342894721,-38.28000002,-61.2567639997892));
#141810=CARTESIAN_POINT('Origin',(-52.7375342894721,-38.78000002,-61.2567639997892));
#141811=CARTESIAN_POINT('Origin',(83.2809572255632,-38.28000002,-55.2499500000007));
#141812=CARTESIAN_POINT('',(-52.7704579175045,-38.28000002,-170.960578619515));
#141813=CARTESIAN_POINT('',(-53.1262583325313,-38.28000002,-171.916267709546));
#141814=CARTESIAN_POINT('Ctrl Pts',(-52.7704579175044,-38.28000002,-170.960578619515));
#141815=CARTESIAN_POINT('Ctrl Pts',(-52.8285971612714,-38.28000002,-171.026452630405));
#141816=CARTESIAN_POINT('Ctrl Pts',(-52.8797920295936,-38.28000002,-171.096554170654));
#141817=CARTESIAN_POINT('Ctrl Pts',(-52.9240704508372,-38.28000002,-171.170767761981));
#141818=CARTESIAN_POINT('Ctrl Pts',(-52.9683488720808,-38.28000002,-171.244981353309));
#141819=CARTESIAN_POINT('Ctrl Pts',(-53.0057109090821,-38.28000002,-171.323307205357));
#141820=CARTESIAN_POINT('Ctrl Pts',(-53.0361319037073,-38.28000002,-171.405662091087));
#141821=CARTESIAN_POINT('Ctrl Pts',(-53.0782642785414,-38.28000002,-171.519721705435));
#141822=CARTESIAN_POINT('Ctrl Pts',(-53.1052589026233,-38.28000002,-171.636480608475));
#141823=CARTESIAN_POINT('Ctrl Pts',(-53.1178820115772,-38.28000002,-171.755802197905));
#141824=CARTESIAN_POINT('Ctrl Pts',(-53.1234875228305,-38.28000002,-171.808789026646));
#141825=CARTESIAN_POINT('Ctrl Pts',(-53.126258330058,-38.28000002,-171.862281331533));
#141826=CARTESIAN_POINT('Ctrl Pts',(-53.1262583325313,-38.28000002,-171.916267709546));
#141827=CARTESIAN_POINT('',(-52.7021525552272,-38.28000002,-170.861259130871));
#141828=CARTESIAN_POINT('Ctrl Pts',(-52.7021525552272,-38.28000002,-170.861259130871));
#141829=CARTESIAN_POINT('Ctrl Pts',(-52.7208104423973,-38.28000002,-170.897192602603));
#141830=CARTESIAN_POINT('Ctrl Pts',(-52.7436752534113,-38.28000002,-170.930232830913));
#141831=CARTESIAN_POINT('Ctrl Pts',(-52.7704579175045,-38.28000002,-170.960578619515));
#141832=CARTESIAN_POINT('',(-40.5593018105246,-38.28000002,-148.113408860656));
#141833=CARTESIAN_POINT('Ctrl Pts',(-40.5593018105246,-38.28000002,-148.113408860656));
#141834=CARTESIAN_POINT('Ctrl Pts',(-42.6385266988695,-38.28000002,-151.875135830624));
#141835=CARTESIAN_POINT('Ctrl Pts',(-44.6827387638261,-38.28000002,-155.655552720007));
#141836=CARTESIAN_POINT('Ctrl Pts',(-46.7035558598462,-38.28000002,-159.448457893456));
#141837=CARTESIAN_POINT('Ctrl Pts',(-48.7243729558662,-38.28000002,-163.241363066904));
#141838=CARTESIAN_POINT('Ctrl Pts',(-50.7215893876843,-38.28000002,-167.046866324983));
#141839=CARTESIAN_POINT('Ctrl Pts',(-52.7021525552272,-38.28000002,-170.86125913087));
#141840=CARTESIAN_POINT('',(-39.5,-38.28000002,-143.762156710948));
#141841=CARTESIAN_POINT('Ctrl Pts',(-39.5,-38.28000002,-143.762156710948));
#141842=CARTESIAN_POINT('Ctrl Pts',(-39.5,-38.28000002,-144.141283590664));
#141843=CARTESIAN_POINT('Ctrl Pts',(-39.5218408888636,-38.28000002,-144.518367123251));
#141844=CARTESIAN_POINT('Ctrl Pts',(-39.5652079410422,-38.28000002,-144.893436753186));
#141845=CARTESIAN_POINT('Ctrl Pts',(-39.6085749932207,-38.28000002,-145.26850638312));
#141846=CARTESIAN_POINT('Ctrl Pts',(-39.6739630147302,-38.28000002,-145.643330762739));
#141847=CARTESIAN_POINT('Ctrl Pts',(-39.7609941006785,-38.28000002,-146.010070025021));
#141848=CARTESIAN_POINT('Ctrl Pts',(-39.8480251866268,-38.28000002,-146.376809287303));
#141849=CARTESIAN_POINT('Ctrl Pts',(-39.9556757536423,-38.28000002,-146.736297755287));
#141850=CARTESIAN_POINT('Ctrl Pts',(-40.0875243805731,-38.28000002,-147.087277124802));
#141851=CARTESIAN_POINT('Ctrl Pts',(-40.2065170359403,-38.28000002,-147.404034061373));
#141852=CARTESIAN_POINT('Ctrl Pts',(-40.3452186968574,-38.28000002,-147.713860479167));
#141853=CARTESIAN_POINT('Ctrl Pts',(-40.5063035885313,-38.28000002,-148.015815905667));
#141854=CARTESIAN_POINT('Ctrl Pts',(-40.5237072071016,-38.28000002,-148.048439182831));
#141855=CARTESIAN_POINT('Ctrl Pts',(-40.5413721449694,-38.28000002,-148.080970567495));
#141856=CARTESIAN_POINT('Ctrl Pts',(-40.5593018105246,-38.28000002,-148.113408860656));
#141857=CARTESIAN_POINT('',(-39.5,-38.28000002,-88.296486260558));
#141858=CARTESIAN_POINT('',(-39.5,-38.28000002,-55.2499500000007));
#141859=CARTESIAN_POINT('',(-40.5593018105246,-38.28000002,-83.9452341108497));
#141860=CARTESIAN_POINT('Ctrl Pts',(-40.5593018105246,-38.28000002,-83.9452341108497));
#141861=CARTESIAN_POINT('Ctrl Pts',(-40.495353484328,-38.28000002,-84.0609292165928));
#141862=CARTESIAN_POINT('Ctrl Pts',(-40.4347639681505,-38.28000002,-84.1780768945295));
#141863=CARTESIAN_POINT('Ctrl Pts',(-40.3773169004728,-38.28000002,-84.2965776208556));
#141864=CARTESIAN_POINT('Ctrl Pts',(-40.3173964789325,-38.28000002,-84.4201803348204));
#141865=CARTESIAN_POINT('Ctrl Pts',(-40.2608947873255,-38.28000002,-84.5452556205675));
#141866=CARTESIAN_POINT('Ctrl Pts',(-40.207615546208,-38.28000002,-84.6717210755968));
#141867=CARTESIAN_POINT('Ctrl Pts',(-40.1651845073098,-38.28000002,-84.7724368615028));
#141868=CARTESIAN_POINT('Ctrl Pts',(-40.1247982681521,-38.28000002,-84.8740350854922));
#141869=CARTESIAN_POINT('Ctrl Pts',(-40.086379235959,-38.28000002,-84.9764835369928));
#141870=CARTESIAN_POINT('Ctrl Pts',(-40.0265153547945,-38.28000002,-85.1361169680306));
#141871=CARTESIAN_POINT('Ctrl Pts',(-39.971455536752,-38.28000002,-85.2977643783894));
#141872=CARTESIAN_POINT('Ctrl Pts',(-39.9211479365401,-38.28000002,-85.4606561619592));
#141873=CARTESIAN_POINT('Ctrl Pts',(-39.8688810993164,-38.28000002,-85.6298917903944));
#141874=CARTESIAN_POINT('Ctrl Pts',(-39.821743908823,-38.28000002,-85.8004696290636));
#141875=CARTESIAN_POINT('Ctrl Pts',(-39.7796250224717,-38.28000002,-85.9715109372541));
#141876=CARTESIAN_POINT('Ctrl Pts',(-39.7722762919974,-38.28000002,-86.0013535229144));
#141877=CARTESIAN_POINT('Ctrl Pts',(-39.7650802005722,-38.28000002,-86.0312102022423));
#141878=CARTESIAN_POINT('Ctrl Pts',(-39.758035997616,-38.28000002,-86.0610762975502));
#141879=CARTESIAN_POINT('Ctrl Pts',(-39.6557558157212,-38.28000002,-86.4947250268103));
#141880=CARTESIAN_POINT('Ctrl Pts',(-39.5840763701735,-38.28000002,-86.933158987616));
#141881=CARTESIAN_POINT('Ctrl Pts',(-39.5426478307198,-38.28000002,-87.3763235090948));
#141882=CARTESIAN_POINT('Ctrl Pts',(-39.5141828100106,-38.28000002,-87.6808161957276));
#141883=CARTESIAN_POINT('Ctrl Pts',(-39.5,-38.28000002,-87.9875423033807));
#141884=CARTESIAN_POINT('Ctrl Pts',(-39.5,-38.28000002,-88.296486260558));
#141885=CARTESIAN_POINT('',(-52.5768547844511,-38.28000002,-61.4386408691297));
#141886=CARTESIAN_POINT('Ctrl Pts',(-52.5768547844511,-38.28000002,-61.4386408691297));
#141887=CARTESIAN_POINT('Ctrl Pts',(-50.6164600523975,-38.28000002,-65.2124493416261));
#141888=CARTESIAN_POINT('Ctrl Pts',(-48.6396458371541,-38.28000002,-68.9774905161615));
#141889=CARTESIAN_POINT('Ctrl Pts',(-46.6396326262455,-38.28000002,-72.7301444246032));
#141890=CARTESIAN_POINT('Ctrl Pts',(-44.6396194153369,-38.28000002,-76.4827983330448));
#141891=CARTESIAN_POINT('Ctrl Pts',(-42.6166038138442,-38.28000002,-80.2231699540513));
#141892=CARTESIAN_POINT('Ctrl Pts',(-40.5593018105246,-38.28000002,-83.9452341108497));
#141893=CARTESIAN_POINT('Origin',(-53.0468858550318,-38.28000002,-61.6241485284586));
#141894=CARTESIAN_POINT('',(-59.5,-38.28000002,-58.24995));
#141895=CARTESIAN_POINT('Origin',(-57.,-38.28000002,-58.24995));
#141896=CARTESIAN_POINT('',(-59.5,-38.28000002,-174.34995));
#141897=CARTESIAN_POINT('',(-59.5,-38.28000002,-58.24995));
#141898=CARTESIAN_POINT('',(-57.,-38.28000002,-176.84995));
#141899=CARTESIAN_POINT('Origin',(-57.,-38.28000002,-174.34995));
#141900=CARTESIAN_POINT('',(-53.1262583325313,-38.28000002,-176.84995));
#141901=CARTESIAN_POINT('',(83.2809572255632,-38.28000002,-176.84995));
#141902=CARTESIAN_POINT('',(-53.1262583325313,-38.28000002,-176.84995));
#141903=CARTESIAN_POINT('Ctrl Pts',(-51.4511770665258,-55.0364221486262,
-59.64995));
#141904=CARTESIAN_POINT('Ctrl Pts',(-51.491108828563,-54.58000002,-59.64995));
#141905=CARTESIAN_POINT('Ctrl Pts',(-51.9492744155716,-54.58000002,-59.64995));
#141906=CARTESIAN_POINT('Ctrl Pts',(-51.4511770665255,-55.0364221486294,
-59.7808732880376));
#141907=CARTESIAN_POINT('Ctrl Pts',(-51.4911088285445,-54.58000002,-59.7861314644994));
#141908=CARTESIAN_POINT('Ctrl Pts',(-51.9492744155546,-54.58000002,-59.8463349320562));
#141909=CARTESIAN_POINT('Ctrl Pts',(-51.4249510883276,-55.0375563641359,
-59.9116978933072));
#141910=CARTESIAN_POINT('Ctrl Pts',(-51.4627154806765,-54.58000002,-59.9224177216068));
#141911=CARTESIAN_POINT('Ctrl Pts',(-51.9100842947729,-54.58000002,-60.0425718399611));
#141912=CARTESIAN_POINT('Ctrl Pts',(-51.3240001449277,-55.0419222689988,
-60.153568971423));
#141913=CARTESIAN_POINT('Ctrl Pts',(-51.3546036645756,-54.58000002,-60.1718710142638));
#141914=CARTESIAN_POINT('Ctrl Pts',(-51.7592308304456,-54.58000002,-60.4053784571342));
#141915=CARTESIAN_POINT('Ctrl Pts',(-51.2493148777934,-55.0451522414979,
-60.2644967268049));
#141916=CARTESIAN_POINT('Ctrl Pts',(-51.2745855330292,-54.58000002,-60.2852157712116));
#141917=CARTESIAN_POINT('Ctrl Pts',(-51.6476268087097,-54.58000002,-60.5717700902076));
#141918=CARTESIAN_POINT('Ctrl Pts',(-51.0627818569665,-55.0532193817859,
-60.4496168355682));
#141919=CARTESIAN_POINT('Ctrl Pts',(-51.0776549189628,-54.58000002,-60.4706504746468));
#141920=CARTESIAN_POINT('Ctrl Pts',(-51.3688859524529,-54.58000002,-60.8494502533521));
#141921=CARTESIAN_POINT('Ctrl Pts',(-50.9510074558263,-55.0580533772402,
-60.5237363920407));
#141922=CARTESIAN_POINT('Ctrl Pts',(-50.9603478356083,-54.5800000199993,
-60.5426326522464));
#141923=CARTESIAN_POINT('Ctrl Pts',(-51.2018587304451,-54.58000002,-60.9606295880612));
#141924=CARTESIAN_POINT('Ctrl Pts',(-50.707290319039,-55.0685936039748,
-60.6239226729819));
#141925=CARTESIAN_POINT('Ctrl Pts',(-50.7089726167645,-54.5800000200007,
-60.6353187454038));
#141926=CARTESIAN_POINT('Ctrl Pts',(-50.8376662507899,-54.58000002,-61.1109090094727));
#141927=CARTESIAN_POINT('Ctrl Pts',(-50.5754672071858,-55.0742946617933,
-60.64995));
#141928=CARTESIAN_POINT('Ctrl Pts',(-50.5746911290892,-54.58000002,-60.6556217969812));
#141929=CARTESIAN_POINT('Ctrl Pts',(-50.6406797499036,-54.58000002,-61.149949999985));
#141930=CARTESIAN_POINT('Ctrl Pts',(-50.4435446592566,-55.08000002,-60.64995));
#141931=CARTESIAN_POINT('Ctrl Pts',(-50.4435446592566,-54.58000002,-60.64995));
#141932=CARTESIAN_POINT('Ctrl Pts',(-50.4435446592566,-54.58000002,-61.14995));
#141933=CARTESIAN_POINT('',(-50.4435446592566,-54.58000002,-61.14995));
#141934=CARTESIAN_POINT('Origin',(-50.4435446592566,-55.08000002,-61.14995));
#141935=CARTESIAN_POINT('Ctrl Pts',(-51.9492744155716,-54.58000002,-59.64995));
#141936=CARTESIAN_POINT('Ctrl Pts',(-51.9492744155546,-54.58000002,-59.8463349320562));
#141937=CARTESIAN_POINT('Ctrl Pts',(-51.9100842947729,-54.58000002,-60.0425718399611));
#141938=CARTESIAN_POINT('Ctrl Pts',(-51.7592308304456,-54.58000002,-60.4053784571342));
#141939=CARTESIAN_POINT('Ctrl Pts',(-51.6476268087097,-54.58000002,-60.5717700902076));
#141940=CARTESIAN_POINT('Ctrl Pts',(-51.3688859524529,-54.58000002,-60.8494502533521));
#141941=CARTESIAN_POINT('Ctrl Pts',(-51.2018587304451,-54.58000002,-60.9606295880612));
#141942=CARTESIAN_POINT('Ctrl Pts',(-50.8376662507899,-54.58000002,-61.1109090094727));
#141943=CARTESIAN_POINT('Ctrl Pts',(-50.6406797499036,-54.58000002,-61.149949999985));
#141944=CARTESIAN_POINT('Ctrl Pts',(-50.4435446592566,-54.58000002,-61.14995));
#141945=CARTESIAN_POINT('Origin',(-60.,-54.58000002,-55.24995));
#141946=CARTESIAN_POINT('',(-49.2787232447289,-54.58000002,-171.14995));
#141947=CARTESIAN_POINT('',(-50.7934646035069,-54.58000002,-172.64995));
#141948=CARTESIAN_POINT('Ctrl Pts',(-49.2787232447289,-54.58000002,-171.14995));
#141949=CARTESIAN_POINT('Ctrl Pts',(-49.477038164104,-54.58000002,-171.149950000016));
#141950=CARTESIAN_POINT('Ctrl Pts',(-49.6752036040849,-54.58000002,-171.18899099047));
#141951=CARTESIAN_POINT('Ctrl Pts',(-50.0415757300179,-54.58000002,-171.339270411997));
#141952=CARTESIAN_POINT('Ctrl Pts',(-50.2096025886599,-54.58000002,-171.450449746589));
#141953=CARTESIAN_POINT('Ctrl Pts',(-50.4900116738692,-54.58000002,-171.728129909852));
#141954=CARTESIAN_POINT('Ctrl Pts',(-50.6022836315107,-54.58000002,-171.894521542842));
#141955=CARTESIAN_POINT('Ctrl Pts',(-50.7540399347937,-54.58000002,-172.257328160063));
#141956=CARTESIAN_POINT('Ctrl Pts',(-50.7934646034919,-54.58000002,-172.453565067926));
#141957=CARTESIAN_POINT('Ctrl Pts',(-50.7934646035069,-54.58000002,-172.64995));
#141958=CARTESIAN_POINT('',(-45.8586217441902,-54.58000002,-171.14995));
#141959=CARTESIAN_POINT('',(-49.3489936620801,-54.58000002,-171.14995));
#141960=CARTESIAN_POINT('',(-43.1572831724514,-54.58000002,-171.14995));
#141961=CARTESIAN_POINT('Ctrl Pts',(-43.1572831724514,-54.58000002,-171.14995));
#141962=CARTESIAN_POINT('Ctrl Pts',(-43.279524411259,-54.58000002,-171.149950030568));
#141963=CARTESIAN_POINT('Ctrl Pts',(-43.4015975649118,-54.58000002,-171.160610139864));
#141964=CARTESIAN_POINT('Ctrl Pts',(-43.5235528170126,-54.58000002,-171.176313109177));
#141965=CARTESIAN_POINT('Ctrl Pts',(-43.6257700730144,-54.5800000200001,
-171.189474612323));
#141966=CARTESIAN_POINT('Ctrl Pts',(-43.7279044984664,-54.5800000200001,
-171.206180488419));
#141967=CARTESIAN_POINT('Ctrl Pts',(-43.829985527596,-54.5800000200001,
-171.223144870208));
#141968=CARTESIAN_POINT('Ctrl Pts',(-43.9984923413766,-54.5800000200002,
-171.251148250928));
#141969=CARTESIAN_POINT('Ctrl Pts',(-44.1669616089445,-54.5800000200002,
-171.278751491316));
#141970=CARTESIAN_POINT('Ctrl Pts',(-44.3358012503232,-54.5800000200001,
-171.290923113047));
#141971=CARTESIAN_POINT('Ctrl Pts',(-44.3914319971545,-54.5800000200001,
-171.294933524355));
#141972=CARTESIAN_POINT('Ctrl Pts',(-44.4471029574849,-54.5800000200001,
-171.297268373358));
#141973=CARTESIAN_POINT('Ctrl Pts',(-44.5028287572164,-54.58000002,-171.297388261734));
#141974=CARTESIAN_POINT('Ctrl Pts',(-44.5028370935956,-54.58000002,-171.297388279669));
#141975=CARTESIAN_POINT('Ctrl Pts',(-44.5028454299759,-54.58000002,-171.297388297554));
#141976=CARTESIAN_POINT('Ctrl Pts',(-44.5028537663573,-54.58000002,-171.29738831539));
#141977=CARTESIAN_POINT('Ctrl Pts',(-44.7276220562719,-54.58000002,-171.297869208197));
#141978=CARTESIAN_POINT('Ctrl Pts',(-44.9531763212381,-54.5800000200004,
-171.261837296445));
#141979=CARTESIAN_POINT('Ctrl Pts',(-45.1787623634369,-54.5800000200001,
-171.22433455003));
#141980=CARTESIAN_POINT('Ctrl Pts',(-45.1788060542272,-54.5800000200001,
-171.224327286617));
#141981=CARTESIAN_POINT('Ctrl Pts',(-45.178849745033,-54.5800000200001,
-171.224320023146));
#141982=CARTESIAN_POINT('Ctrl Pts',(-45.1788934358544,-54.5800000200001,
-171.224312759618));
#141983=CARTESIAN_POINT('Ctrl Pts',(-45.2946034848909,-54.58000002,-171.205076152327));
#141984=CARTESIAN_POINT('Ctrl Pts',(-45.4103612459202,-54.58000002,-171.185995253716));
#141985=CARTESIAN_POINT('Ctrl Pts',(-45.5265088418228,-54.58000002,-171.171982248345));
#141986=CARTESIAN_POINT('Ctrl Pts',(-45.6241378685024,-54.58000002,-171.160203476132));
#141987=CARTESIAN_POINT('Ctrl Pts',(-45.7220426205362,-54.58000002,-171.152008348194));
#141988=CARTESIAN_POINT('Ctrl Pts',(-45.8204240164945,-54.58000002,-171.150287040904));
#141989=CARTESIAN_POINT('Ctrl Pts',(-45.8331484827184,-54.58000002,-171.150064410231));
#141990=CARTESIAN_POINT('Ctrl Pts',(-45.8458809158945,-54.58000002,-171.149950003086));
#141991=CARTESIAN_POINT('Ctrl Pts',(-45.8586217441902,-54.58000002,-171.14995));
#141992=CARTESIAN_POINT('',(-42.5,-54.58000002,-171.14995));
#141993=CARTESIAN_POINT('',(-49.3489936620801,-54.58000002,-171.14995));
#141994=CARTESIAN_POINT('',(-42.5,-54.58000002,-61.14995));
#141995=CARTESIAN_POINT('',(-42.5,-54.58000002,-171.64995));
#141996=CARTESIAN_POINT('',(-43.1572831724516,-54.58000002,-61.14995));
#141997=CARTESIAN_POINT('',(-60.,-54.58000002,-61.14995));
#141998=CARTESIAN_POINT('',(-45.8586217441897,-54.58000002,-61.14995));
#141999=CARTESIAN_POINT('Ctrl Pts',(-45.8586217441897,-54.58000002,-61.14995));
#142000=CARTESIAN_POINT('Ctrl Pts',(-45.7594843223745,-54.58000002,-61.1499499759911));
#142001=CARTESIAN_POINT('Ctrl Pts',(-45.660855613418,-54.58000002,-61.1430183938606));
#142002=CARTESIAN_POINT('Ctrl Pts',(-45.5625314448157,-54.58000002,-61.1320945152429));
#142003=CARTESIAN_POINT('Ctrl Pts',(-45.4342876572931,-54.58000002,-61.1178465476446));
#142004=CARTESIAN_POINT('Ctrl Pts',(-45.3065614560445,-54.58000002,-61.0968118490375));
#142005=CARTESIAN_POINT('Ctrl Pts',(-45.1788934332666,-54.5800000200001,
-61.075587255946));
#142006=CARTESIAN_POINT('Ctrl Pts',(-45.1788516209101,-54.5800000200001,
-61.0755803047123));
#142007=CARTESIAN_POINT('Ctrl Pts',(-45.1788098085678,-54.5800000200001,
-61.0755733535312));
#142008=CARTESIAN_POINT('Ctrl Pts',(-45.1787679962398,-54.5800000200001,
-61.0755664024026));
#142009=CARTESIAN_POINT('Ctrl Pts',(-44.9531807615356,-54.5800000200004,
-61.0380634472604));
#142010=CARTESIAN_POINT('Ctrl Pts',(-44.7276252028241,-54.58000002,-61.0020307849363));
#142011=CARTESIAN_POINT('Ctrl Pts',(-44.5028537665277,-54.58000002,-61.0025117642945));
#142012=CARTESIAN_POINT('Ctrl Pts',(-44.502848607531,-54.58000002,-61.002511775334));
#142013=CARTESIAN_POINT('Ctrl Pts',(-44.5028434485348,-54.58000002,-61.0025117863925));
#142014=CARTESIAN_POINT('Ctrl Pts',(-44.502838289539,-54.58000002,-61.00251179747));
#142015=CARTESIAN_POINT('Ctrl Pts',(-44.3506760857117,-54.58000002,-61.0028385232137));
#142016=CARTESIAN_POINT('Ctrl Pts',(-44.1989241833619,-54.5800000200001,
-61.0196754576617));
#142017=CARTESIAN_POINT('Ctrl Pts',(-44.0472833113151,-54.5800000200001,
-61.0420612980709));
#142018=CARTESIAN_POINT('Ctrl Pts',(-43.9748362264978,-54.5800000200001,
-61.0527562304921));
#142019=CARTESIAN_POINT('Ctrl Pts',(-43.9024145037625,-54.58000002,-61.0647186315171));
#142020=CARTESIAN_POINT('Ctrl Pts',(-43.8299855489727,-54.58000002,-61.0767552584245));
#142021=CARTESIAN_POINT('Ctrl Pts',(-43.7015244308365,-54.58000002,-61.0981036066867));
#142022=CARTESIAN_POINT('Ctrl Pts',(-43.5729778197523,-54.58000002,-61.1190439724879));
#142023=CARTESIAN_POINT('Ctrl Pts',(-43.4442858805813,-54.58000002,-61.1330238652824));
#142024=CARTESIAN_POINT('Ctrl Pts',(-43.348706683562,-54.58000002,-61.1434066983979));
#142025=CARTESIAN_POINT('Ctrl Pts',(-43.2530473192986,-54.58000002,-61.1499499760532));
#142026=CARTESIAN_POINT('Ctrl Pts',(-43.1572831724516,-54.58000002,-61.14995));
#142027=CARTESIAN_POINT('',(-60.,-54.58000002,-61.14995));
#142028=CARTESIAN_POINT('',(-57.,-54.58000002,-55.74995));
#142029=CARTESIAN_POINT('',(-60.,-54.58000002,-55.74995));
#142030=CARTESIAN_POINT('',(-59.5,-54.58000002,-58.24995));
#142031=CARTESIAN_POINT('Origin',(-57.,-54.58000002,-58.24995));
#142032=CARTESIAN_POINT('',(-59.5,-54.58000002,-174.34995));
#142033=CARTESIAN_POINT('',(-59.5,-54.58000002,-58.24995));
#142034=CARTESIAN_POINT('',(-57.,-54.58000002,-176.84995));
#142035=CARTESIAN_POINT('Origin',(-57.,-54.58000002,-174.34995));
#142036=CARTESIAN_POINT('',(-50.7934646035069,-54.58000002,-176.84995));
#142037=CARTESIAN_POINT('',(-60.,-54.58000002,-176.84995));
#142038=CARTESIAN_POINT('',(-50.7934646035069,-54.58000002,-55.24995));
#142039=CARTESIAN_POINT('Origin',(-60.,-54.08000002,-55.74995));
#142040=CARTESIAN_POINT('',(-57.,-54.08000002,-55.24995));
#142041=CARTESIAN_POINT('',(-60.,-54.08000002,-55.24995));
#142042=CARTESIAN_POINT('Origin',(-57.,-54.08000002,-55.74995));
#142043=CARTESIAN_POINT('Origin',(-60.,28.41999998,-55.24995));
#142044=CARTESIAN_POINT('',(-57.,-53.58000002,-55.24995));
#142045=CARTESIAN_POINT('',(-60.,-53.58000002,-55.24995));
#142046=CARTESIAN_POINT('',(-57.,28.41999998,-55.24995));
#142047=CARTESIAN_POINT('Origin',(83.2809572255632,-53.5800000199999,-55.74995));
#142048=CARTESIAN_POINT('',(-57.,-53.08000002,-55.74995));
#142049=CARTESIAN_POINT('',(83.2809572255632,-53.0800000199999,-55.74995));
#142050=CARTESIAN_POINT('Origin',(-57.,-53.58000002,-55.74995));
#142051=CARTESIAN_POINT('Origin',(83.2809572255632,-53.0800000199999,-55.2499500000008));
#142052=CARTESIAN_POINT('',(-57.,-53.08000002,-176.84995));
#142053=CARTESIAN_POINT('',(-51.1448166902628,-53.08000002,-176.84995));
#142054=CARTESIAN_POINT('',(83.2809572255632,-53.0800000199999,-176.84995));
#142055=CARTESIAN_POINT('',(-59.5,-53.08000002,-174.34995));
#142056=CARTESIAN_POINT('Origin',(-57.,-53.08000002,-174.34995));
#142057=CARTESIAN_POINT('',(-59.5,-53.08000002,-58.24995));
#142058=CARTESIAN_POINT('',(-59.5,-53.08000002,-174.34995));
#142059=CARTESIAN_POINT('Origin',(-57.,-53.08000002,-58.24995));
#142060=CARTESIAN_POINT('',(-50.6622663180714,-53.08000002,-61.14995));
#142061=CARTESIAN_POINT('Ctrl Pts',(-50.6622663180714,-53.08000002,-61.14995));
#142062=CARTESIAN_POINT('Ctrl Pts',(-50.8594014087184,-53.08000002,-61.149949999985));
#142063=CARTESIAN_POINT('Ctrl Pts',(-51.0563879096046,-53.08000002,-61.1109090094727));
#142064=CARTESIAN_POINT('Ctrl Pts',(-51.4205803892599,-53.08000002,-60.9606295880612));
#142065=CARTESIAN_POINT('Ctrl Pts',(-51.5876076112677,-53.08000002,-60.8494502533514));
#142066=CARTESIAN_POINT('Ctrl Pts',(-51.8663484675245,-53.08000002,-60.5717700902082));
#142067=CARTESIAN_POINT('Ctrl Pts',(-51.9779524892604,-53.08000002,-60.4053784571342));
#142068=CARTESIAN_POINT('Ctrl Pts',(-52.1288059535877,-53.08000002,-60.0425718399611));
#142069=CARTESIAN_POINT('Ctrl Pts',(-52.1679960743694,-53.08000002,-59.8463349320561));
#142070=CARTESIAN_POINT('Ctrl Pts',(-52.1679960743864,-53.08000002,-59.64995));
#142071=CARTESIAN_POINT('',(-43.7578534463097,-53.08000002,-61.14995));
#142072=CARTESIAN_POINT('',(83.2809572255632,-53.0800000199999,-61.14995));
#142073=CARTESIAN_POINT('',(-43.1446480925044,-53.08000002,-61.4386408691297));
#142074=CARTESIAN_POINT('Ctrl Pts',(-43.1446480925044,-53.08000002,-61.4386408691297));
#142075=CARTESIAN_POINT('Ctrl Pts',(-43.1765609373872,-53.08000002,-61.3882288400421));
#142076=CARTESIAN_POINT('Ctrl Pts',(-43.2167516388878,-53.08000002,-61.3458652617053));
#142077=CARTESIAN_POINT('Ctrl Pts',(-43.2628503174202,-53.08000002,-61.3093295271296));
#142078=CARTESIAN_POINT('Ctrl Pts',(-43.3089610210815,-53.08000002,-61.2727842619789));
#142079=CARTESIAN_POINT('Ctrl Pts',(-43.3605330051288,-53.08000002,-61.2428744748388));
#142080=CARTESIAN_POINT('Ctrl Pts',(-43.414231413078,-53.08000002,-61.2194436041558));
#142081=CARTESIAN_POINT('Ctrl Pts',(-43.4456262415641,-53.08000002,-61.205744721927));
#142082=CARTESIAN_POINT('Ctrl Pts',(-43.477917759742,-53.08000002,-61.1941576093824));
#142083=CARTESIAN_POINT('Ctrl Pts',(-43.5108494925037,-53.08000002,-61.1845858141908));
#142084=CARTESIAN_POINT('Ctrl Pts',(-43.5447058226298,-53.08000002,-61.1747452795231));
#142085=CARTESIAN_POINT('Ctrl Pts',(-43.5792402145375,-53.08000002,-61.1670347524206));
#142086=CARTESIAN_POINT('Ctrl Pts',(-43.6141927055652,-53.08000002,-61.1614020099222));
#142087=CARTESIAN_POINT('Ctrl Pts',(-43.6489049458008,-53.08000002,-61.1558079848602));
#142088=CARTESIAN_POINT('Ctrl Pts',(-43.6840310643501,-53.08000002,-61.1522634649488));
#142089=CARTESIAN_POINT('Ctrl Pts',(-43.7193126347007,-53.08000002,-61.1507670586125));
#142090=CARTESIAN_POINT('Ctrl Pts',(-43.7321435462893,-53.08000002,-61.1502228578524));
#142091=CARTESIAN_POINT('Ctrl Pts',(-43.7449948697401,-53.08000002,-61.14995));
#142092=CARTESIAN_POINT('Ctrl Pts',(-43.7578534463097,-53.08000002,-61.14995));
#142093=CARTESIAN_POINT('',(-41.0647116264214,-53.08000002,-64.687079328241));
#142094=CARTESIAN_POINT('Ctrl Pts',(-41.0647116264215,-53.08000002,-64.6870793282409));
#142095=CARTESIAN_POINT('Ctrl Pts',(-41.7638515954828,-53.08000002,-63.6079981134234));
#142096=CARTESIAN_POINT('Ctrl Pts',(-42.4569204735311,-53.08000002,-62.5250292766735));
#142097=CARTESIAN_POINT('Ctrl Pts',(-43.1446480925044,-53.08000002,-61.4386408691297));
#142098=CARTESIAN_POINT('',(-39.5,-53.08000002,-70.7293062304687));
#142099=CARTESIAN_POINT('Ctrl Pts',(-39.5,-53.08000002,-70.7293062304687));
#142100=CARTESIAN_POINT('Ctrl Pts',(-39.5,-53.08000002,-70.1996325547074));
#142101=CARTESIAN_POINT('Ctrl Pts',(-39.5302602116353,-53.08000002,-69.6738635266889));
#142102=CARTESIAN_POINT('Ctrl Pts',(-39.5906692531643,-53.08000002,-69.1519847741694));
#142103=CARTESIAN_POINT('Ctrl Pts',(-39.6510782946932,-53.08000002,-68.6301060216499));
#142104=CARTESIAN_POINT('Ctrl Pts',(-39.7415458248093,-53.08000002,-68.1121058873189));
#142105=CARTESIAN_POINT('Ctrl Pts',(-39.8661752652165,-53.08000002,-67.5985138592656));
#142106=CARTESIAN_POINT('Ctrl Pts',(-39.9284899854243,-53.08000002,-67.3417178452216));
#142107=CARTESIAN_POINT('Ctrl Pts',(-39.9995673120589,-53.08000002,-67.0857801566515));
#142108=CARTESIAN_POINT('Ctrl Pts',(-40.0792084204325,-53.08000002,-66.8343727800802));
#142109=CARTESIAN_POINT('Ctrl Pts',(-40.1588495287955,-53.08000002,-66.5829654035428));
#142110=CARTESIAN_POINT('Ctrl Pts',(-40.2472081235396,-53.08000002,-66.3353006307905));
#142111=CARTESIAN_POINT('Ctrl Pts',(-40.3452847184366,-53.08000002,-66.0918080038346));
#142112=CARTESIAN_POINT('Ctrl Pts',(-40.4725149961156,-53.08000002,-65.7759361633318));
#142113=CARTESIAN_POINT('Ctrl Pts',(-40.6155606032241,-53.08000002,-65.4668542003385));
#142114=CARTESIAN_POINT('Ctrl Pts',(-40.7793840759704,-53.08000002,-65.1666925984838));
#142115=CARTESIAN_POINT('Ctrl Pts',(-40.8681301749544,-53.08000002,-65.0040897017021));
#142116=CARTESIAN_POINT('Ctrl Pts',(-40.9629743342391,-53.08000002,-64.8441048248421));
#142117=CARTESIAN_POINT('Ctrl Pts',(-41.0647116264214,-53.08000002,-64.687079328241));
#142118=CARTESIAN_POINT('',(-39.5,-53.08000002,-161.329336741015));
#142119=CARTESIAN_POINT('',(-39.5,-53.08000002,-55.2499500000008));
#142120=CARTESIAN_POINT('',(-41.0647116264263,-53.08000002,-167.371563643272));
#142121=CARTESIAN_POINT('Ctrl Pts',(-41.0647116264263,-53.08000002,-167.371563643272));
#142122=CARTESIAN_POINT('Ctrl Pts',(-40.8730279274754,-53.08000002,-167.075711184725));
#142123=CARTESIAN_POINT('Ctrl Pts',(-40.7056641754826,-53.08000002,-166.769103901981));
#142124=CARTESIAN_POINT('Ctrl Pts',(-40.5574162968198,-53.08000002,-166.454043185635));
#142125=CARTESIAN_POINT('Ctrl Pts',(-40.4818120706005,-53.08000002,-166.293366878586));
#142126=CARTESIAN_POINT('Ctrl Pts',(-40.4111805199785,-53.08000002,-166.130491546332));
#142127=CARTESIAN_POINT('Ctrl Pts',(-40.3448358791345,-53.08000002,-165.965720445509));
#142128=CARTESIAN_POINT('Ctrl Pts',(-40.1483999357586,-53.08000002,-165.477859388165));
#142129=CARTESIAN_POINT('Ctrl Pts',(-39.9897001835278,-53.08000002,-164.969734884954));
#142130=CARTESIAN_POINT('Ctrl Pts',(-39.8654535116526,-53.08000002,-164.457153153597));
#142131=CARTESIAN_POINT('Ctrl Pts',(-39.7412068397774,-53.08000002,-163.94457142224));
#142132=CARTESIAN_POINT('Ctrl Pts',(-39.6509082568844,-53.08000002,-163.427315362986));
#142133=CARTESIAN_POINT('Ctrl Pts',(-39.5905852088212,-53.08000002,-162.905931958774));
#142134=CARTESIAN_POINT('Ctrl Pts',(-39.530262160758,-53.08000002,-162.384548554563));
#142135=CARTESIAN_POINT('Ctrl Pts',(-39.4999999999991,-53.08000002,-161.85902605313));
#142136=CARTESIAN_POINT('Ctrl Pts',(-39.5,-53.08000002,-161.329336741015));
#142137=CARTESIAN_POINT('',(-43.2972503047852,-53.08000002,-170.861259130871));
#142138=CARTESIAN_POINT('Ctrl Pts',(-43.2972503047852,-53.08000002,-170.861259130871));
#142139=CARTESIAN_POINT('Ctrl Pts',(-42.5594745131554,-53.08000002,-169.693930655453));
#142140=CARTESIAN_POINT('Ctrl Pts',(-41.8155944388483,-53.08000002,-168.530506878352));
#142141=CARTESIAN_POINT('Ctrl Pts',(-41.0647116264263,-53.08000002,-167.371563643272));
#142142=CARTESIAN_POINT('',(-43.9094855672884,-53.08000002,-171.14995));
#142143=CARTESIAN_POINT('Ctrl Pts',(-43.9094855672884,-53.08000002,-171.14995));
#142144=CARTESIAN_POINT('Ctrl Pts',(-43.8503415173364,-53.08000002,-171.14995));
#142145=CARTESIAN_POINT('Ctrl Pts',(-43.7921001974326,-53.08000002,-171.144262868806));
#142146=CARTESIAN_POINT('Ctrl Pts',(-43.7347793831646,-53.08000002,-171.132860793684));
#142147=CARTESIAN_POINT('Ctrl Pts',(-43.6774556974662,-53.08000002,-171.121458147386));
#142148=CARTESIAN_POINT('Ctrl Pts',(-43.6204048981063,-53.08000002,-171.104031177905));
#142149=CARTESIAN_POINT('Ctrl Pts',(-43.5666850153843,-53.08000002,-171.080579637536));
#142150=CARTESIAN_POINT('Ctrl Pts',(-43.5129605101707,-53.08000002,-171.057126079209));
#142151=CARTESIAN_POINT('Ctrl Pts',(-43.4620141840633,-53.08000002,-171.02762282191));
#142152=CARTESIAN_POINT('Ctrl Pts',(-43.4156376346715,-53.08000002,-170.990867761886));
#142153=CARTESIAN_POINT('Ctrl Pts',(-43.3692713886891,-53.08000002,-170.95412086768));
#142154=CARTESIAN_POINT('Ctrl Pts',(-43.3290601923967,-53.08000002,-170.911589580894));
#142155=CARTESIAN_POINT('Ctrl Pts',(-43.2972503047852,-53.08000002,-170.861259130871));
#142156=CARTESIAN_POINT('',(-49.6300753314849,-53.08000002,-171.14995));
#142157=CARTESIAN_POINT('',(-43.4531980731446,-53.08000002,-171.14995));
#142158=CARTESIAN_POINT('',(-51.1448166902628,-53.08000002,-172.64995));
#142159=CARTESIAN_POINT('Ctrl Pts',(-51.1448166902628,-53.08000002,-172.64995));
#142160=CARTESIAN_POINT('Ctrl Pts',(-51.1448166902479,-53.08000002,-172.453565067926));
#142161=CARTESIAN_POINT('Ctrl Pts',(-51.1053920215496,-53.08000002,-172.257328160063));
#142162=CARTESIAN_POINT('Ctrl Pts',(-50.9536357182667,-53.08000002,-171.894521542842));
#142163=CARTESIAN_POINT('Ctrl Pts',(-50.8413637606251,-53.08000002,-171.728129909852));
#142164=CARTESIAN_POINT('Ctrl Pts',(-50.5609546754159,-53.08000002,-171.450449746589));
#142165=CARTESIAN_POINT('Ctrl Pts',(-50.3929278167739,-53.08000002,-171.339270411997));
#142166=CARTESIAN_POINT('Ctrl Pts',(-50.0265556908409,-53.08000002,-171.18899099047));
#142167=CARTESIAN_POINT('Ctrl Pts',(-49.8283902508599,-53.08000002,-171.149950000016));
#142168=CARTESIAN_POINT('Ctrl Pts',(-49.6300753314849,-53.08000002,-171.14995));
#142169=CARTESIAN_POINT('',(-51.1448166902628,-53.08000002,-55.2499500000008));
#142170=CARTESIAN_POINT('Ctrl Pts',(-50.6622663180714,-52.58000002,-60.64995));
#142171=CARTESIAN_POINT('Ctrl Pts',(-50.6622663180714,-53.0800000199999,
-60.64995));
#142172=CARTESIAN_POINT('Ctrl Pts',(-50.6622663180714,-53.08000002,-61.14995));
#142173=CARTESIAN_POINT('Ctrl Pts',(-50.7941888660007,-52.5742946617934,
-60.64995));
#142174=CARTESIAN_POINT('Ctrl Pts',(-50.7949847395758,-53.08000002,-60.6442102195366));
#142175=CARTESIAN_POINT('Ctrl Pts',(-50.8594014087184,-53.08000002,-61.149949999985));
#142176=CARTESIAN_POINT('Ctrl Pts',(-50.9260119778537,-52.5685936039755,
-60.6239226729819));
#142177=CARTESIAN_POINT('Ctrl Pts',(-50.9243014854221,-53.08000002,-60.61203530794));
#142178=CARTESIAN_POINT('Ctrl Pts',(-51.0563879096046,-53.08000002,-61.1109090094727));
#142179=CARTESIAN_POINT('Ctrl Pts',(-51.1697291146411,-52.5580533772395,
-60.5237363920407));
#142180=CARTESIAN_POINT('Ctrl Pts',(-51.1595684581335,-53.08000002,-60.5031527166044));
#142181=CARTESIAN_POINT('Ctrl Pts',(-51.4205803892599,-53.08000002,-60.9606295880612));
#142182=CARTESIAN_POINT('Ctrl Pts',(-51.2815035157812,-52.5532193817859,
-60.4496168355682));
#142183=CARTESIAN_POINT('Ctrl Pts',(-51.2649990424134,-53.0800000200007,
-60.4261994932773));
#142184=CARTESIAN_POINT('Ctrl Pts',(-51.5876076112677,-53.08000002,-60.8494502533514));
#142185=CARTESIAN_POINT('Ctrl Pts',(-51.4680365366082,-52.5451522414979,
-60.2644967268049));
#142186=CARTESIAN_POINT('Ctrl Pts',(-51.4390258902891,-53.0800000199993,
-60.2406767152623));
#142187=CARTESIAN_POINT('Ctrl Pts',(-51.8663484675245,-53.08000002,-60.5717700902082));
#142188=CARTESIAN_POINT('Ctrl Pts',(-51.5427218037424,-52.5419222689988,
-60.153568971423));
#142189=CARTESIAN_POINT('Ctrl Pts',(-51.507092542289,-53.08000002,-60.1322291512615));
#142190=CARTESIAN_POINT('Ctrl Pts',(-51.9779524892604,-53.08000002,-60.4053784571342));
#142191=CARTESIAN_POINT('Ctrl Pts',(-51.6436727471424,-52.5375563641358,
-59.9116978933072));
#142192=CARTESIAN_POINT('Ctrl Pts',(-51.598921085515,-53.08000002,-59.8989712332631));
#142193=CARTESIAN_POINT('Ctrl Pts',(-52.1288059535877,-53.08000002,-60.0425718399611));
#142194=CARTESIAN_POINT('Ctrl Pts',(-51.6698987253403,-52.5364221486294,
-59.7808732880376));
#142195=CARTESIAN_POINT('Ctrl Pts',(-51.6223418238443,-53.0800000200021,
-59.7746029379323));
#142196=CARTESIAN_POINT('Ctrl Pts',(-52.1679960743694,-53.08000002,-59.8463349320561));
#142197=CARTESIAN_POINT('Ctrl Pts',(-51.6698987253405,-52.5364221486262,
-59.64995));
#142198=CARTESIAN_POINT('Ctrl Pts',(-51.6223418238518,-53.08000002,-59.64995));
#142199=CARTESIAN_POINT('Ctrl Pts',(-52.1679960743864,-53.08000002,-59.64995));
#142200=CARTESIAN_POINT('Origin',(-50.6622663180714,-52.58000002,-61.14995));
#142201=CARTESIAN_POINT('Origin',(0.,-12.9675000200281,-60.64995));
#142202=CARTESIAN_POINT('',(-43.7578534463097,-52.58000002,-60.64995));
#142203=CARTESIAN_POINT('',(-48.2747189347426,-46.93000002,-60.64995));
#142204=CARTESIAN_POINT('Origin',(0.,-12.9675000200281,-60.64995));
#142205=CARTESIAN_POINT('',(1.65582490824295E-14,-52.58000002,-60.64995));
#142206=CARTESIAN_POINT('',(1.41965171211599E-14,-46.93000002,-60.64995));
#142207=CARTESIAN_POINT('Ctrl Pts',(-52.1642096742619,-46.8864221486262,
-59.64995));
#142208=CARTESIAN_POINT('Ctrl Pts',(-52.2041414362991,-46.43000002,-59.64995));
#142209=CARTESIAN_POINT('Ctrl Pts',(-52.6623070233078,-46.43000002,-59.64995));
#142210=CARTESIAN_POINT('Ctrl Pts',(-52.1642096742618,-46.8864221486274,
-59.7808732880376));
#142211=CARTESIAN_POINT('Ctrl Pts',(-52.2041414362827,-46.4300000200027,
-59.7861314645));
#142212=CARTESIAN_POINT('Ctrl Pts',(-52.6623070232907,-46.43000002,-59.8463349320562));
#142213=CARTESIAN_POINT('Ctrl Pts',(-52.1379836960638,-46.8875563641358,
-59.9116978933072));
#142214=CARTESIAN_POINT('Ctrl Pts',(-52.175748088412,-46.43000002,-59.9224177216061));
#142215=CARTESIAN_POINT('Ctrl Pts',(-52.6231169025091,-46.43000002,-60.0425718399611));
#142216=CARTESIAN_POINT('Ctrl Pts',(-52.0370327526638,-46.8919222689988,
-60.153568971423));
#142217=CARTESIAN_POINT('Ctrl Pts',(-52.0676362723124,-46.43000002,-60.1718710142644));
#142218=CARTESIAN_POINT('Ctrl Pts',(-52.4722634381817,-46.43000002,-60.4053784571342));
#142219=CARTESIAN_POINT('Ctrl Pts',(-51.9623474855296,-46.8951522414972,
-60.264496726805));
#142220=CARTESIAN_POINT('Ctrl Pts',(-51.9876181407653,-46.43000002,-60.2852157712123));
#142221=CARTESIAN_POINT('Ctrl Pts',(-52.3606594164458,-46.43000002,-60.5717700902076));
#142222=CARTESIAN_POINT('Ctrl Pts',(-51.7758144647026,-46.9032193817865,
-60.4496168355682));
#142223=CARTESIAN_POINT('Ctrl Pts',(-51.7906875266988,-46.43000002,-60.4706504746462));
#142224=CARTESIAN_POINT('Ctrl Pts',(-52.0819185601891,-46.43000002,-60.8494502533521));
#142225=CARTESIAN_POINT('Ctrl Pts',(-51.6640400635624,-46.9080533772402,
-60.5237363920407));
#142226=CARTESIAN_POINT('Ctrl Pts',(-51.6733804433437,-46.4300000200007,
-60.5426326522478));
#142227=CARTESIAN_POINT('Ctrl Pts',(-51.9148913381812,-46.43000002,-60.9606295880612));
#142228=CARTESIAN_POINT('Ctrl Pts',(-51.4203229267752,-46.9185936039748,
-60.6239226729819));
#142229=CARTESIAN_POINT('Ctrl Pts',(-51.4220052245013,-46.4300000199993,
-60.6353187454025));
#142230=CARTESIAN_POINT('Ctrl Pts',(-51.550698858526,-46.43000002,-61.1109090094727));
#142231=CARTESIAN_POINT('Ctrl Pts',(-51.288499814922,-46.9242946617933,
-60.64995));
#142232=CARTESIAN_POINT('Ctrl Pts',(-51.2877237368248,-46.4300000199999,
-60.6556217969811));
#142233=CARTESIAN_POINT('Ctrl Pts',(-51.3537123576397,-46.43000002,-61.149949999985));
#142234=CARTESIAN_POINT('Ctrl Pts',(-51.1565772669927,-46.93000002,-60.64995));
#142235=CARTESIAN_POINT('Ctrl Pts',(-51.1565772669928,-46.43000002,-60.64995));
#142236=CARTESIAN_POINT('Ctrl Pts',(-51.1565772669927,-46.43000002,-61.14995));
#142237=CARTESIAN_POINT('',(-51.1565772669927,-46.43000002,-61.14995));
#142238=CARTESIAN_POINT('Origin',(-51.1565772669927,-46.93000002,-61.14995));
#142239=CARTESIAN_POINT('Ctrl Pts',(-52.6623070233077,-46.43000002,-59.64995));
#142240=CARTESIAN_POINT('Ctrl Pts',(-52.6623070232906,-46.43000002,-59.8463349320562));
#142241=CARTESIAN_POINT('Ctrl Pts',(-52.623116902509,-46.43000002,-60.0425718399611));
#142242=CARTESIAN_POINT('Ctrl Pts',(-52.5476901703453,-46.43000002,-60.2239751485476));
#142243=CARTESIAN_POINT('Ctrl Pts',(-52.4722634381816,-46.43000002,-60.4053784571342));
#142244=CARTESIAN_POINT('Ctrl Pts',(-52.3606594164458,-46.43000002,-60.5717700902076));
#142245=CARTESIAN_POINT('Ctrl Pts',(-52.2212889883174,-46.43000002,-60.7106101717798));
#142246=CARTESIAN_POINT('Ctrl Pts',(-52.0819185601891,-46.43000002,-60.8494502533521));
#142247=CARTESIAN_POINT('Ctrl Pts',(-51.9148913381812,-46.43000002,-60.9606295880612));
#142248=CARTESIAN_POINT('Ctrl Pts',(-51.7327950983536,-46.43000002,-61.0357692987669));
#142249=CARTESIAN_POINT('Ctrl Pts',(-51.550698858526,-46.43000002,-61.1109090094727));
#142250=CARTESIAN_POINT('Ctrl Pts',(-51.3537123576397,-46.43000002,-61.149949999985));
#142251=CARTESIAN_POINT('Ctrl Pts',(-51.1565772669927,-46.43000002,-61.14995));
#142252=CARTESIAN_POINT('Origin',(83.2809572255632,-46.4300000199999,-55.2499500000008));
#142253=CARTESIAN_POINT('',(-57.,-46.43000002,-55.74995));
#142254=CARTESIAN_POINT('',(83.2809572255632,-46.4300000199999,-55.74995));
#142255=CARTESIAN_POINT('',(-59.5,-46.43000002,-58.24995));
#142256=CARTESIAN_POINT('Origin',(-57.,-46.43000002,-58.24995));
#142257=CARTESIAN_POINT('',(-59.5,-46.43000002,-174.34995));
#142258=CARTESIAN_POINT('',(-59.5,-46.43000002,-58.24995));
#142259=CARTESIAN_POINT('',(-57.,-46.43000002,-176.84995));
#142260=CARTESIAN_POINT('Origin',(-57.,-46.43000002,-174.34995));
#142261=CARTESIAN_POINT('',(-51.9388724063314,-46.43000002,-176.84995));
#142262=CARTESIAN_POINT('',(83.2809572255632,-46.4300000199999,-176.84995));
#142263=CARTESIAN_POINT('',(-51.9388724063314,-46.43000002,-172.64995));
#142264=CARTESIAN_POINT('',(-51.9388724063314,-46.43000002,-55.2499500000008));
#142265=CARTESIAN_POINT('',(-50.4241310475534,-46.43000002,-171.14995));
#142266=CARTESIAN_POINT('Ctrl Pts',(-50.4241310475534,-46.43000002,-171.14995));
#142267=CARTESIAN_POINT('Ctrl Pts',(-50.6224459669284,-46.43000002,-171.149950000016));
#142268=CARTESIAN_POINT('Ctrl Pts',(-50.8206114069094,-46.43000002,-171.18899099047));
#142269=CARTESIAN_POINT('Ctrl Pts',(-51.1869835328424,-46.43000002,-171.339270411997));
#142270=CARTESIAN_POINT('Ctrl Pts',(-51.3550103914843,-46.43000002,-171.450449746589));
#142271=CARTESIAN_POINT('Ctrl Pts',(-51.6354194766937,-46.43000002,-171.728129909852));
#142272=CARTESIAN_POINT('Ctrl Pts',(-51.7476914343352,-46.43000002,-171.894521542842));
#142273=CARTESIAN_POINT('Ctrl Pts',(-51.8994477376182,-46.43000002,-172.257328160063));
#142274=CARTESIAN_POINT('Ctrl Pts',(-51.9388724063164,-46.43000002,-172.453565067926));
#142275=CARTESIAN_POINT('Ctrl Pts',(-51.9388724063314,-46.43000002,-172.64995));
#142276=CARTESIAN_POINT('',(-48.4122058243951,-46.43000002,-171.14995));
#142277=CARTESIAN_POINT('',(-50.4944014649046,-46.43000002,-171.14995));
#142278=CARTESIAN_POINT('',(-47.8576079004676,-46.43000002,-170.861259130871));
#142279=CARTESIAN_POINT('Ctrl Pts',(-47.8576079004676,-46.43000002,-170.861259130871));
#142280=CARTESIAN_POINT('Ctrl Pts',(-47.8760580377295,-46.43000002,-170.89352615778));
#142281=CARTESIAN_POINT('Ctrl Pts',(-47.8980723549741,-46.43000002,-170.923203523829));
#142282=CARTESIAN_POINT('Ctrl Pts',(-47.9228861329636,-46.43000002,-170.950192158739));
#142283=CARTESIAN_POINT('Ctrl Pts',(-47.9503841163788,-46.43000002,-170.98010026203));
#142284=CARTESIAN_POINT('Ctrl Pts',(-47.981319017648,-46.43000002,-171.00670574507));
#142285=CARTESIAN_POINT('Ctrl Pts',(-48.0145941519157,-46.43000002,-171.02991277546));
#142286=CARTESIAN_POINT('Ctrl Pts',(-48.0405863852474,-46.43000002,-171.048040502428));
#142287=CARTESIAN_POINT('Ctrl Pts',(-48.0680050205668,-46.43000002,-171.06409541242));
#142288=CARTESIAN_POINT('Ctrl Pts',(-48.0963149978629,-46.43000002,-171.078049783599));
#142289=CARTESIAN_POINT('Ctrl Pts',(-48.1225339813698,-46.43000002,-171.090973475624));
#142290=CARTESIAN_POINT('Ctrl Pts',(-48.1495923840829,-46.43000002,-171.102104191555));
#142291=CARTESIAN_POINT('Ctrl Pts',(-48.177275111639,-46.43000002,-171.111506345608));
#142292=CARTESIAN_POINT('Ctrl Pts',(-48.2055749629089,-46.43000002,-171.121118099391));
#142293=CARTESIAN_POINT('Ctrl Pts',(-48.234528655658,-46.43000002,-171.128923533851));
#142294=CARTESIAN_POINT('Ctrl Pts',(-48.2639285033285,-46.43000002,-171.134940493274));
#142295=CARTESIAN_POINT('Ctrl Pts',(-48.2928212065521,-46.43000002,-171.140853660745));
#142296=CARTESIAN_POINT('Ctrl Pts',(-48.3221462163591,-46.43000002,-171.145039422868));
#142297=CARTESIAN_POINT('Ctrl Pts',(-48.3517066016403,-46.43000002,-171.147466016794));
#142298=CARTESIAN_POINT('Ctrl Pts',(-48.3717866301037,-46.43000002,-171.149114374034));
#142299=CARTESIAN_POINT('Ctrl Pts',(-48.3919752683816,-46.43000002,-171.14995));
#142300=CARTESIAN_POINT('Ctrl Pts',(-48.4122058243951,-46.43000002,-171.14995));
#142301=CARTESIAN_POINT('',(-40.8634877666247,-46.43000002,-158.96051646616));
#142302=CARTESIAN_POINT('Ctrl Pts',(-40.8634877666247,-46.43000002,-158.96051646616));
#142303=CARTESIAN_POINT('Ctrl Pts',(-43.2493545263947,-46.43000002,-162.895404681481));
#142304=CARTESIAN_POINT('Ctrl Pts',(-45.5734709768386,-46.43000002,-166.866583832071));
#142305=CARTESIAN_POINT('Ctrl Pts',(-47.8576079004676,-46.43000002,-170.861259130871));
#142306=CARTESIAN_POINT('',(-39.5,-46.43000002,-153.563058845195));
#142307=CARTESIAN_POINT('Ctrl Pts',(-39.5,-46.43000002,-153.563058845195));
#142308=CARTESIAN_POINT('Ctrl Pts',(-39.4999999999995,-46.43000002,-153.949465551028));
#142309=CARTESIAN_POINT('Ctrl Pts',(-39.5176594219082,-46.43000002,-154.333958533364));
#142310=CARTESIAN_POINT('Ctrl Pts',(-39.5536573145523,-46.43000002,-154.716308049412));
#142311=CARTESIAN_POINT('Ctrl Pts',(-39.5886363261013,-46.43000002,-155.087835579366));
#142312=CARTESIAN_POINT('Ctrl Pts',(-39.6409303087516,-46.43000002,-155.457339415589));
#142313=CARTESIAN_POINT('Ctrl Pts',(-39.711211141592,-46.43000002,-155.824604113663));
#142314=CARTESIAN_POINT('Ctrl Pts',(-39.7452479661607,-46.43000002,-156.002469451813));
#142315=CARTESIAN_POINT('Ctrl Pts',(-39.7835042486637,-46.43000002,-156.179809528778));
#142316=CARTESIAN_POINT('Ctrl Pts',(-39.8260607087683,-46.43000002,-156.356599303471));
#142317=CARTESIAN_POINT('Ctrl Pts',(-39.9364913068056,-46.43000002,-156.815354578187));
#142318=CARTESIAN_POINT('Ctrl Pts',(-40.0748112905465,-46.43000002,-157.263052526106));
#142319=CARTESIAN_POINT('Ctrl Pts',(-40.2452594329879,-46.43000002,-157.698012597756));
#142320=CARTESIAN_POINT('Ctrl Pts',(-40.3764895639192,-46.43000002,-158.032893731307));
#142321=CARTESIAN_POINT('Ctrl Pts',(-40.5265005956173,-46.43000002,-158.360328778722));
#142322=CARTESIAN_POINT('Ctrl Pts',(-40.7006921181746,-46.43000002,-158.678176979839));
#142323=CARTESIAN_POINT('Ctrl Pts',(-40.7527491045398,-46.43000002,-158.773165640762));
#142324=CARTESIAN_POINT('Ctrl Pts',(-40.8069659798529,-46.43000002,-158.867297969463));
#142325=CARTESIAN_POINT('Ctrl Pts',(-40.8634877666247,-46.43000002,-158.960516466159));
#142326=CARTESIAN_POINT('',(-39.5,-46.43000002,-78.4955841262963));
#142327=CARTESIAN_POINT('',(-39.5,-46.43000002,-55.2499500000008));
#142328=CARTESIAN_POINT('',(-40.8634877666247,-46.43000002,-73.0981265053466));
#142329=CARTESIAN_POINT('Ctrl Pts',(-40.8634877666247,-46.43000002,-73.0981265053466));
#142330=CARTESIAN_POINT('Ctrl Pts',(-40.661044199348,-46.43000002,-73.4320063432862));
#142331=CARTESIAN_POINT('Ctrl Pts',(-40.4876415800298,-46.43000002,-73.7785418551243));
#142332=CARTESIAN_POINT('Ctrl Pts',(-40.3370596438449,-46.43000002,-74.1350223226556));
#142333=CARTESIAN_POINT('Ctrl Pts',(-40.305064047112,-46.43000002,-74.210767166767));
#142334=CARTESIAN_POINT('Ctrl Pts',(-40.2740989238678,-46.43000002,-74.2869610781288));
#142335=CARTESIAN_POINT('Ctrl Pts',(-40.2441048562922,-46.43000002,-74.3635781632946));
#142336=CARTESIAN_POINT('Ctrl Pts',(-40.0729487154701,-46.43000002,-74.8007807729435));
#142337=CARTESIAN_POINT('Ctrl Pts',(-39.9334371777348,-46.43000002,-75.2543998579721));
#142338=CARTESIAN_POINT('Ctrl Pts',(-39.8240030986842,-46.43000002,-75.7106064091747));
#142339=CARTESIAN_POINT('Ctrl Pts',(-39.7066850117819,-46.43000002,-76.1996796511091));
#142340=CARTESIAN_POINT('Ctrl Pts',(-39.6220553949032,-46.43000002,-76.6934446581353));
#142341=CARTESIAN_POINT('Ctrl Pts',(-39.5687675179992,-46.43000002,-77.1917081792648));
#142342=CARTESIAN_POINT('Ctrl Pts',(-39.5226417428819,-46.43000002,-77.6230031089943));
#142343=CARTESIAN_POINT('Ctrl Pts',(-39.5,-46.43000002,-78.0576687430938));
#142344=CARTESIAN_POINT('Ctrl Pts',(-39.5,-46.43000002,-78.4955841262963));
#142345=CARTESIAN_POINT('',(-47.7195914591242,-46.43000002,-61.4386408691297));
#142346=CARTESIAN_POINT('Ctrl Pts',(-47.7195914591242,-46.43000002,-61.4386408691297));
#142347=CARTESIAN_POINT('Ctrl Pts',(-45.4798130845491,-46.43000002,-65.351943995909));
#142348=CARTESIAN_POINT('Ctrl Pts',(-43.2013098945494,-46.43000002,-69.2424758480089));
#142349=CARTESIAN_POINT('Ctrl Pts',(-40.8634877666247,-46.43000002,-73.0981265053466));
#142350=CARTESIAN_POINT('',(-48.2747189347426,-46.43000002,-61.14995));
#142351=CARTESIAN_POINT('Ctrl Pts',(-48.2747189347426,-46.43000002,-61.14995));
#142352=CARTESIAN_POINT('Ctrl Pts',(-48.2086234136051,-46.43000002,-61.14995));
#142353=CARTESIAN_POINT('Ctrl Pts',(-48.1427915915172,-46.43000002,-61.1585974051143));
#142354=CARTESIAN_POINT('Ctrl Pts',(-48.0794858636046,-46.43000002,-61.1760262255644));
#142355=CARTESIAN_POINT('Ctrl Pts',(-48.0376978539717,-46.43000002,-61.1875309620373));
#142356=CARTESIAN_POINT('Ctrl Pts',(-47.9970101587091,-46.43000002,-61.2028630486499));
#142357=CARTESIAN_POINT('Ctrl Pts',(-47.9580757097656,-46.43000002,-61.2220733995985));
#142358=CARTESIAN_POINT('Ctrl Pts',(-47.9230818282115,-46.43000002,-61.2393394650997));
#142359=CARTESIAN_POINT('Ctrl Pts',(-47.8896549296879,-46.43000002,-61.2597370764849));
#142360=CARTESIAN_POINT('Ctrl Pts',(-47.8586276391547,-46.43000002,-61.2831656716456));
#142361=CARTESIAN_POINT('Ctrl Pts',(-47.8304660966181,-46.43000002,-61.3044303508313));
#142362=CARTESIAN_POINT('Ctrl Pts',(-47.8042802405272,-46.43000002,-61.3281927143748));
#142363=CARTESIAN_POINT('Ctrl Pts',(-47.7807177502455,-46.43000002,-61.3544087872413));
#142364=CARTESIAN_POINT('Ctrl Pts',(-47.7576005025357,-46.43000002,-61.3801294747912));
#142365=CARTESIAN_POINT('Ctrl Pts',(-47.7370072711932,-46.43000002,-61.4082122550317));
#142366=CARTESIAN_POINT('Ctrl Pts',(-47.7195914591242,-46.43000002,-61.4386408691297));
#142367=CARTESIAN_POINT('',(83.2809572255632,-46.4300000199999,-61.14995));
#142368=CARTESIAN_POINT('Origin',(-60.,-45.93000002,-55.74995));
#142369=CARTESIAN_POINT('',(-57.,-45.93000002,-55.24995));
#142370=CARTESIAN_POINT('',(-60.,-45.93000002,-55.24995));
#142371=CARTESIAN_POINT('Origin',(-57.,-45.93000002,-55.74995));
#142372=CARTESIAN_POINT('Origin',(-60.,28.41999998,-55.24995));
#142373=CARTESIAN_POINT('',(-57.,-45.43000002,-55.24995));
#142374=CARTESIAN_POINT('',(-60.,-45.43000002,-55.24995));
#142375=CARTESIAN_POINT('',(-57.,28.41999998,-55.24995));
#142376=CARTESIAN_POINT('Origin',(83.2809572255632,-45.4300000199999,-55.74995));
#142377=CARTESIAN_POINT('',(-57.,-44.93000002,-55.74995));
#142378=CARTESIAN_POINT('',(83.2809572255632,-44.93000002,-55.74995));
#142379=CARTESIAN_POINT('Origin',(-57.,-45.43000002,-55.74995));
#142380=CARTESIAN_POINT('Ctrl Pts',(-51.3752989258075,-44.43000002,-60.64995));
#142381=CARTESIAN_POINT('Ctrl Pts',(-51.3752989258075,-44.93000002,-60.64995));
#142382=CARTESIAN_POINT('Ctrl Pts',(-51.3752989258075,-44.93000002,-61.14995));
#142383=CARTESIAN_POINT('Ctrl Pts',(-51.5072214737368,-44.4242946617934,
-60.64995));
#142384=CARTESIAN_POINT('Ctrl Pts',(-51.5080173473124,-44.9300000200007,
-60.6442102195364));
#142385=CARTESIAN_POINT('Ctrl Pts',(-51.5724340164545,-44.93000002,-61.149949999985));
#142386=CARTESIAN_POINT('Ctrl Pts',(-51.6390445855899,-44.4185936039755,
-60.6239226729819));
#142387=CARTESIAN_POINT('Ctrl Pts',(-51.6373340931575,-44.9300000200007,
-60.61203530794));
#142388=CARTESIAN_POINT('Ctrl Pts',(-51.7694205173407,-44.93000002,-61.1109090094727));
#142389=CARTESIAN_POINT('Ctrl Pts',(-51.8827617223772,-44.4080533772395,
-60.5237363920407));
#142390=CARTESIAN_POINT('Ctrl Pts',(-51.8726010658704,-44.9300000199993,
-60.5031527166044));
#142391=CARTESIAN_POINT('Ctrl Pts',(-52.1336129969961,-44.93000002,-60.9606295880612));
#142392=CARTESIAN_POINT('Ctrl Pts',(-51.9945361235173,-44.4032193817859,
-60.4496168355682));
#142393=CARTESIAN_POINT('Ctrl Pts',(-51.9780316501496,-44.93000002,-60.4261994932779));
#142394=CARTESIAN_POINT('Ctrl Pts',(-52.3006402190038,-44.93000002,-60.8494502533521));
#142395=CARTESIAN_POINT('Ctrl Pts',(-52.1810691443443,-44.3951522414979,
-60.2644967268049));
#142396=CARTESIAN_POINT('Ctrl Pts',(-52.1520584980253,-44.93000002,-60.2406767152616));
#142397=CARTESIAN_POINT('Ctrl Pts',(-52.5793810752606,-44.93000002,-60.5717700902076));
#142398=CARTESIAN_POINT('Ctrl Pts',(-52.2557544114786,-44.3919222689988,
-60.153568971423));
#142399=CARTESIAN_POINT('Ctrl Pts',(-52.2201251500251,-44.93000002,-60.1322291512615));
#142400=CARTESIAN_POINT('Ctrl Pts',(-52.6909850969965,-44.93000002,-60.4053784571342));
#142401=CARTESIAN_POINT('Ctrl Pts',(-52.3567053548786,-44.3875563641358,
-59.9116978933072));
#142402=CARTESIAN_POINT('Ctrl Pts',(-52.3119536932511,-44.93000002,-59.8989712332631));
#142403=CARTESIAN_POINT('Ctrl Pts',(-52.8418385613238,-44.93000002,-60.0425718399611));
#142404=CARTESIAN_POINT('Ctrl Pts',(-52.3829313330764,-44.3864221486294,
-59.7808732880376));
#142405=CARTESIAN_POINT('Ctrl Pts',(-52.3353744315805,-44.9300000200007,
-59.7746029379323));
#142406=CARTESIAN_POINT('Ctrl Pts',(-52.8810286821055,-44.93000002,-59.8463349320562));
#142407=CARTESIAN_POINT('Ctrl Pts',(-52.3829313330767,-44.3864221486262,
-59.64995));
#142408=CARTESIAN_POINT('Ctrl Pts',(-52.3353744315879,-44.93000002,-59.64995));
#142409=CARTESIAN_POINT('Ctrl Pts',(-52.8810286821225,-44.93000002,-59.64995));
#142410=CARTESIAN_POINT('',(-51.3752989258075,-44.93000002,-61.14995));
#142411=CARTESIAN_POINT('Origin',(-51.3752989258075,-44.43000002,-61.14995));
#142412=CARTESIAN_POINT('Ctrl Pts',(-51.3752989258075,-44.93000002,-61.14995));
#142413=CARTESIAN_POINT('Ctrl Pts',(-51.5724340164545,-44.93000002,-61.149949999985));
#142414=CARTESIAN_POINT('Ctrl Pts',(-51.7694205173407,-44.93000002,-61.1109090094727));
#142415=CARTESIAN_POINT('Ctrl Pts',(-52.1336129969961,-44.93000002,-60.9606295880612));
#142416=CARTESIAN_POINT('Ctrl Pts',(-52.3006402190038,-44.93000002,-60.8494502533521));
#142417=CARTESIAN_POINT('Ctrl Pts',(-52.5793810752606,-44.93000002,-60.5717700902076));
#142418=CARTESIAN_POINT('Ctrl Pts',(-52.6909850969965,-44.93000002,-60.4053784571342));
#142419=CARTESIAN_POINT('Ctrl Pts',(-52.8418385613238,-44.93000002,-60.0425718399611));
#142420=CARTESIAN_POINT('Ctrl Pts',(-52.8810286821055,-44.93000002,-59.8463349320562));
#142421=CARTESIAN_POINT('Ctrl Pts',(-52.8810286821225,-44.93000002,-59.64995));
#142422=CARTESIAN_POINT('Origin',(83.2809572255632,-44.93000002,-55.2499500000007));
#142423=CARTESIAN_POINT('',(-57.,-44.93000002,-176.84995));
#142424=CARTESIAN_POINT('',(-52.2902244930873,-44.93000002,-176.84995));
#142425=CARTESIAN_POINT('',(83.2809572255632,-44.93000002,-176.84995));
#142426=CARTESIAN_POINT('',(-59.5,-44.93000002,-174.34995));
#142427=CARTESIAN_POINT('Origin',(-57.,-44.93000002,-174.34995));
#142428=CARTESIAN_POINT('',(-59.5,-44.93000002,-58.24995));
#142429=CARTESIAN_POINT('',(-59.5,-44.93000002,-174.34995));
#142430=CARTESIAN_POINT('Origin',(-57.,-44.93000002,-58.24995));
#142431=CARTESIAN_POINT('',(-49.940073970993,-44.93000002,-61.14995));
#142432=CARTESIAN_POINT('',(83.2809572255632,-44.93000002,-61.14995));
#142433=CARTESIAN_POINT('',(-49.4036629110189,-44.93000002,-61.4386408691297));
#142434=CARTESIAN_POINT('Ctrl Pts',(-49.4036629110189,-44.93000002,-61.4386408691297));
#142435=CARTESIAN_POINT('Ctrl Pts',(-49.421292954971,-44.93000002,-61.4067508873822));
#142436=CARTESIAN_POINT('Ctrl Pts',(-49.4424088019262,-44.93000002,-61.3772666862022));
#142437=CARTESIAN_POINT('Ctrl Pts',(-49.4663885772136,-44.93000002,-61.3502540659087));
#142438=CARTESIAN_POINT('Ctrl Pts',(-49.4778548596159,-44.93000002,-61.33733758404));
#142439=CARTESIAN_POINT('Ctrl Pts',(-49.4899767151878,-44.93000002,-61.3249865422104));
#142440=CARTESIAN_POINT('Ctrl Pts',(-49.5026897554816,-44.93000002,-61.3132100906898));
#142441=CARTESIAN_POINT('Ctrl Pts',(-49.5320647115447,-44.93000002,-61.2859992317605));
#142442=CARTESIAN_POINT('Ctrl Pts',(-49.5637608854771,-44.93000002,-61.2625146831493));
#142443=CARTESIAN_POINT('Ctrl Pts',(-49.597554081752,-44.93000002,-61.2422777750133));
#142444=CARTESIAN_POINT('Ctrl Pts',(-49.6090633503044,-44.93000002,-61.2353854997602));
#142445=CARTESIAN_POINT('Ctrl Pts',(-49.6208161109919,-44.93000002,-61.2288703265774));
#142446=CARTESIAN_POINT('Ctrl Pts',(-49.6328042123455,-44.93000002,-61.2227144603287));
#142447=CARTESIAN_POINT('Ctrl Pts',(-49.679945666351,-44.93000002,-61.1985074172725));
#142448=CARTESIAN_POINT('Ctrl Pts',(-49.7309938530465,-44.93000002,-61.1800821085049));
#142449=CARTESIAN_POINT('Ctrl Pts',(-49.7824210964939,-44.93000002,-61.1680542343897));
#142450=CARTESIAN_POINT('Ctrl Pts',(-49.833844605741,-44.93000002,-61.1560272336343));
#142451=CARTESIAN_POINT('Ctrl Pts',(-49.8863934436428,-44.93000002,-61.14995));
#142452=CARTESIAN_POINT('Ctrl Pts',(-49.940073970993,-44.93000002,-61.14995));
#142453=CARTESIAN_POINT('',(-40.7712064624936,-44.93000002,-76.6047958451324));
#142454=CARTESIAN_POINT('Ctrl Pts',(-40.7712064624935,-44.93000002,-76.6047958451324));
#142455=CARTESIAN_POINT('Ctrl Pts',(-43.723712605206,-44.93000002,-71.5921120242627));
#142456=CARTESIAN_POINT('Ctrl Pts',(-46.5890589653218,-44.93000002,-66.5298175388285));
#142457=CARTESIAN_POINT('Ctrl Pts',(-49.4036629110189,-44.93000002,-61.4386408691297));
#142458=CARTESIAN_POINT('',(-39.5,-44.93000002,-81.6937887068282));
#142459=CARTESIAN_POINT('Ctrl Pts',(-39.5,-44.93000002,-81.6937887068282));
#142460=CARTESIAN_POINT('Ctrl Pts',(-39.5,-44.93000002,-81.4715915443627));
#142461=CARTESIAN_POINT('Ctrl Pts',(-39.5062851881924,-44.93000002,-81.2500804744028));
#142462=CARTESIAN_POINT('Ctrl Pts',(-39.5189031887286,-44.93000002,-81.0292580402078));
#142463=CARTESIAN_POINT('Ctrl Pts',(-39.5308326200065,-44.93000002,-80.820485973209));
#142464=CARTESIAN_POINT('Ctrl Pts',(-39.5484229321411,-44.93000002,-80.6123290364163));
#142465=CARTESIAN_POINT('Ctrl Pts',(-39.5717668549559,-44.93000002,-80.4047900585203));
#142466=CARTESIAN_POINT('Ctrl Pts',(-39.5731142710435,-44.93000002,-80.392810865484));
#142467=CARTESIAN_POINT('Ctrl Pts',(-39.5744808704139,-44.93000002,-80.3808337323845));
#142468=CARTESIAN_POINT('Ctrl Pts',(-39.5758666762242,-44.93000002,-80.3688586602483));
#142469=CARTESIAN_POINT('Ctrl Pts',(-39.5992261762147,-44.93000002,-80.167003757221));
#142470=CARTESIAN_POINT('Ctrl Pts',(-39.6280811656786,-44.93000002,-79.9654411052776));
#142471=CARTESIAN_POINT('Ctrl Pts',(-39.6625124125991,-44.93000002,-79.7646415180465));
#142472=CARTESIAN_POINT('Ctrl Pts',(-39.6964841131887,-44.93000002,-79.5665219590392));
#142473=CARTESIAN_POINT('Ctrl Pts',(-39.735884231964,-44.93000002,-79.3691455608356));
#142474=CARTESIAN_POINT('Ctrl Pts',(-39.7807398869814,-44.93000002,-79.1729578992683));
#142475=CARTESIAN_POINT('Ctrl Pts',(-39.7892690083245,-44.93000002,-79.1356536090762));
#142476=CARTESIAN_POINT('Ctrl Pts',(-39.7979952284868,-44.93000002,-79.0983922704894));
#142477=CARTESIAN_POINT('Ctrl Pts',(-39.8069185231454,-44.93000002,-79.0611769040833));
#142478=CARTESIAN_POINT('Ctrl Pts',(-39.9103339550991,-44.93000002,-78.6298739672843));
#142479=CARTESIAN_POINT('Ctrl Pts',(-40.0396611959927,-44.93000002,-78.2084773864585));
#142480=CARTESIAN_POINT('Ctrl Pts',(-40.1983721980467,-44.93000002,-77.7983145251762));
#142481=CARTESIAN_POINT('Ctrl Pts',(-40.3310078543919,-44.93000002,-77.455539168644));
#142482=CARTESIAN_POINT('Ctrl Pts',(-40.4839381620924,-44.93000002,-77.1205226744026));
#142483=CARTESIAN_POINT('Ctrl Pts',(-40.6627223002475,-44.93000002,-76.7953903625546));
#142484=CARTESIAN_POINT('Ctrl Pts',(-40.6978701506679,-44.93000002,-76.7314713707381));
#142485=CARTESIAN_POINT('Ctrl Pts',(-40.7340173780027,-44.93000002,-76.6679344511564));
#142486=CARTESIAN_POINT('Ctrl Pts',(-40.7712064624936,-44.93000002,-76.6047958451324));
#142487=CARTESIAN_POINT('',(-39.5,-44.93000002,-150.364854264666));
#142488=CARTESIAN_POINT('',(-39.5,-44.93000002,-55.2499500000007));
#142489=CARTESIAN_POINT('',(-40.7712064624936,-44.93000002,-155.453847126373));
#142490=CARTESIAN_POINT('Ctrl Pts',(-40.7712064624936,-44.93000002,-155.453847126373));
#142491=CARTESIAN_POINT('Ctrl Pts',(-40.5636969173457,-44.93000002,-155.101543121134));
#142492=CARTESIAN_POINT('Ctrl Pts',(-40.3878808277004,-44.93000002,-154.735494168741));
#142493=CARTESIAN_POINT('Ctrl Pts',(-40.2370488760485,-44.93000002,-154.358609995095));
#142494=CARTESIAN_POINT('Ctrl Pts',(-40.2234902738441,-44.93000002,-154.324731081963));
#142495=CARTESIAN_POINT('Ctrl Pts',(-40.2101335892538,-44.93000002,-154.290764600354));
#142496=CARTESIAN_POINT('Ctrl Pts',(-40.1969739657515,-44.93000002,-154.256712656464));
#142497=CARTESIAN_POINT('Ctrl Pts',(-40.0374208080236,-44.93000002,-153.843851667435));
#142498=CARTESIAN_POINT('Ctrl Pts',(-39.9069198944888,-44.93000002,-153.416428338648));
#142499=CARTESIAN_POINT('Ctrl Pts',(-39.8044156663649,-44.93000002,-152.987004278786));
#142500=CARTESIAN_POINT('Ctrl Pts',(-39.6913863431124,-44.93000002,-152.513487119906));
#142501=CARTESIAN_POINT('Ctrl Pts',(-39.6104670975055,-44.93000002,-152.035255380817));
#142502=CARTESIAN_POINT('Ctrl Pts',(-39.560598744179,-44.93000002,-151.552464535407));
#142503=CARTESIAN_POINT('Ctrl Pts',(-39.5200177005092,-44.93000002,-151.159586987341));
#142504=CARTESIAN_POINT('Ctrl Pts',(-39.4999999999997,-44.93000002,-150.763690175803));
#142505=CARTESIAN_POINT('Ctrl Pts',(-39.5,-44.93000002,-150.364854264666));
#142506=CARTESIAN_POINT('',(-49.5369875341119,-44.93000002,-170.861259130871));
#142507=CARTESIAN_POINT('Ctrl Pts',(-49.5369875341119,-44.93000002,-170.861259130871));
#142508=CARTESIAN_POINT('Ctrl Pts',(-46.6796235355215,-44.93000002,-165.688723110732));
#142509=CARTESIAN_POINT('Ctrl Pts',(-43.770354187064,-44.93000002,-160.545717743323));
#142510=CARTESIAN_POINT('Ctrl Pts',(-40.7712064624936,-44.93000002,-155.453847126373));
#142511=CARTESIAN_POINT('',(-50.0729884546894,-44.93000002,-171.14995));
#142512=CARTESIAN_POINT('Ctrl Pts',(-50.0729884546894,-44.93000002,-171.14995));
#142513=CARTESIAN_POINT('Ctrl Pts',(-50.0168171487332,-44.93000002,-171.14995));
#142514=CARTESIAN_POINT('Ctrl Pts',(-49.9608486377765,-44.93000002,-171.143210614633));
#142515=CARTESIAN_POINT('Ctrl Pts',(-49.9066731284723,-44.93000002,-171.129767219263));
#142516=CARTESIAN_POINT('Ctrl Pts',(-49.8576729639807,-44.93000002,-171.117608061131));
#142517=CARTESIAN_POINT('Ctrl Pts',(-49.8101382025066,-44.93000002,-171.099963916562));
#142518=CARTESIAN_POINT('Ctrl Pts',(-49.7652508518366,-44.93000002,-171.076824577701));
#142519=CARTESIAN_POINT('Ctrl Pts',(-49.7179896877752,-44.93000002,-171.052461542819));
#142520=CARTESIAN_POINT('Ctrl Pts',(-49.6739559670876,-44.93000002,-171.022111093102));
#142521=CARTESIAN_POINT('Ctrl Pts',(-49.6349583346168,-44.93000002,-170.985779705428));
#142522=CARTESIAN_POINT('Ctrl Pts',(-49.5959662083459,-44.93000002,-170.949453447498));
#142523=CARTESIAN_POINT('Ctrl Pts',(-49.5629377334322,-44.93000002,-170.908235414179));
#142524=CARTESIAN_POINT('Ctrl Pts',(-49.5369875341119,-44.93000002,-170.861259130871));
#142525=CARTESIAN_POINT('',(-50.7754831343094,-44.93000002,-171.14995));
#142526=CARTESIAN_POINT('',(-49.7553180351958,-44.93000002,-171.14995));
#142527=CARTESIAN_POINT('',(-52.2902244930873,-44.93000002,-172.64995));
#142528=CARTESIAN_POINT('Ctrl Pts',(-52.2902244930873,-44.93000002,-172.64995));
#142529=CARTESIAN_POINT('Ctrl Pts',(-52.2902244930723,-44.93000002,-172.453565067926));
#142530=CARTESIAN_POINT('Ctrl Pts',(-52.2507998243741,-44.93000002,-172.257328160063));
#142531=CARTESIAN_POINT('Ctrl Pts',(-52.0990435210912,-44.93000002,-171.894521542842));
#142532=CARTESIAN_POINT('Ctrl Pts',(-51.9867715634496,-44.93000002,-171.728129909852));
#142533=CARTESIAN_POINT('Ctrl Pts',(-51.7063624782404,-44.93000002,-171.450449746589));
#142534=CARTESIAN_POINT('Ctrl Pts',(-51.5383356195984,-44.93000002,-171.339270411997));
#142535=CARTESIAN_POINT('Ctrl Pts',(-51.1719634936654,-44.93000002,-171.18899099047));
#142536=CARTESIAN_POINT('Ctrl Pts',(-50.9737980536844,-44.93000002,-171.149950000016));
#142537=CARTESIAN_POINT('Ctrl Pts',(-50.7754831343094,-44.93000002,-171.14995));
#142538=CARTESIAN_POINT('',(-52.2902244930873,-44.93000002,-55.2499500000007));
#142539=CARTESIAN_POINT('Origin',(0.,-12.9675000200281,-60.64995));
#142540=CARTESIAN_POINT('',(1.31515029790052E-14,-44.43000002,-60.64995));
#142541=CARTESIAN_POINT('Origin',(-1.8346904061005E-14,28.9199999800001,
-61.14995));
#142542=CARTESIAN_POINT('Origin',(-45.342056117244,28.91999998,-61.14995));
#142543=CARTESIAN_POINT('Origin',(-44.5079524583208,31.5404524382925,235.35105));
#142544=CARTESIAN_POINT('',(-44.5079524583208,29.5404524382925,-52.64995));
#142545=CARTESIAN_POINT('Origin',(-44.5079524583208,31.5404524382925,-52.64995));
#142546=CARTESIAN_POINT('',(-44.5079524583208,29.5404524382925,-55.24995));
#142547=CARTESIAN_POINT('',(-44.5079524583208,29.5404524382925,235.35105));
#142548=CARTESIAN_POINT('Origin',(-44.5079524583208,31.5404524382925,-55.24995));
#142549=CARTESIAN_POINT('Origin',(0.,45.41999998,-55.24995));
#142550=CARTESIAN_POINT('',(-44.5079524583208,28.7904524382925,-55.24995));
#142551=CARTESIAN_POINT('Origin',(-44.5079524583208,31.5404524382925,-55.24995));
#142552=CARTESIAN_POINT('Origin',(-44.5079524583208,31.5404524382925,-52.64995));
#142553=CARTESIAN_POINT('',(-44.5079524583208,28.7904524382925,-60.649950000076));
#142554=CARTESIAN_POINT('',(-44.5079524583208,28.7904524382925,-52.64995));
#142555=CARTESIAN_POINT('Ctrl Pts',(-44.5079556015694,28.7904524382943,
-60.6499500000744));
#142556=CARTESIAN_POINT('Ctrl Pts',(-44.5807764535743,28.7904525215285,
-60.6499499625289));
#142557=CARTESIAN_POINT('Ctrl Pts',(-44.6535686798933,28.7933450738462,
-60.6499600881128));
#142558=CARTESIAN_POINT('Ctrl Pts',(-44.8330889160976,28.807634767527,-60.6499589648009));
#142559=CARTESIAN_POINT('Ctrl Pts',(-44.9394280112978,28.8223952301239,
-60.6499497576228));
#142560=CARTESIAN_POINT('Ctrl Pts',(-45.1451244228601,28.8633251672665,
-60.6499554517945));
#142561=CARTESIAN_POINT('Ctrl Pts',(-45.2444206001228,28.8889220866332,
-60.64995));
#142562=CARTESIAN_POINT('Ctrl Pts',(-45.342056117244,28.91999998,-60.64995));
#142563=CARTESIAN_POINT('Ctrl Pts',(-43.6738487993976,28.91999998,-60.64995));
#142564=CARTESIAN_POINT('Ctrl Pts',(-43.7715308492441,28.8889072750245,
-60.64995));
#142565=CARTESIAN_POINT('Ctrl Pts',(-43.8708751019496,28.8633007826373,
-60.6499548134291));
#142566=CARTESIAN_POINT('Ctrl Pts',(-44.0766026663055,28.8223760301817,
-60.6499497945332));
#142567=CARTESIAN_POINT('Ctrl Pts',(-44.1829231968646,28.8076227744794,
-60.6499592870445));
#142568=CARTESIAN_POINT('Ctrl Pts',(-44.3623973025031,28.7933425641166,
-60.6499605225574));
#142569=CARTESIAN_POINT('Ctrl Pts',(-44.4351590053701,28.7904524382924,
-60.6499500380157));
#142570=CARTESIAN_POINT('Ctrl Pts',(-44.5079524583208,28.7904524382924,
-60.6499500000761));
#142571=CARTESIAN_POINT('Origin',(-1.8346904061005E-14,28.9199999800001,
-61.14995));
#142572=CARTESIAN_POINT('Origin',(-43.6738487993998,28.91999998,-61.1499500000012));
#142573=CARTESIAN_POINT('Origin',(-41.7558360441701,28.91999998,-61.14995));
#142574=CARTESIAN_POINT('Ctrl Pts',(-41.4049466656477,29.0638025010082,
-60.64995));
#142575=CARTESIAN_POINT('Ctrl Pts',(-41.5509245680609,28.91999998,-60.64995));
#142576=CARTESIAN_POINT('Ctrl Pts',(-41.7558360441701,28.91999998,-60.64995));
#142577=CARTESIAN_POINT('Ctrl Pts',(-41.0540572871252,28.7076050220163,
-60.64995));
#142578=CARTESIAN_POINT('Ctrl Pts',(-41.3460130919516,28.41999998,-60.64995));
#142579=CARTESIAN_POINT('Ctrl Pts',(-41.7558360441701,28.41999998,-60.64995));
#142580=CARTESIAN_POINT('Ctrl Pts',(-41.0540572871252,28.7076050220163,
-61.14995));
#142581=CARTESIAN_POINT('Ctrl Pts',(-41.3460130919516,28.41999998,-61.14995));
#142582=CARTESIAN_POINT('Ctrl Pts',(-41.7558360441701,28.41999998,-61.14995));
#142583=CARTESIAN_POINT('',(-41.0540572871253,28.7076050220164,-61.14995));
#142584=CARTESIAN_POINT('Origin',(-41.4049466656476,29.0638025010082,-61.14995));
#142585=CARTESIAN_POINT('Origin',(-41.7558360441701,29.41999998,-61.14995));
#142586=CARTESIAN_POINT('Origin',(0.,-12.9675000200281,-61.14995));
#142587=CARTESIAN_POINT('',(-39.3277310924369,30.3404619167909,-61.14995));
#142588=CARTESIAN_POINT('Origin',(-39.6638655462185,30.7106154376184,-61.14995));
#142589=CARTESIAN_POINT('Origin',(0.,-12.9675000200281,-61.14995));
#142590=CARTESIAN_POINT('Ctrl Pts',(-39.5,31.080768958446,-60.64995));
#142591=CARTESIAN_POINT('Ctrl Pts',(-39.5,30.859420873127,-60.64995));
#142592=CARTESIAN_POINT('Ctrl Pts',(-39.6638655462185,30.7106154376184,
-60.64995));
#142593=CARTESIAN_POINT('Ctrl Pts',(-39.,31.080768958446,-60.64995));
#142594=CARTESIAN_POINT('Ctrl Pts',(-39.,30.638072787808,-60.64995));
#142595=CARTESIAN_POINT('Ctrl Pts',(-39.327731092437,30.3404619167909,-60.64995));
#142596=CARTESIAN_POINT('Ctrl Pts',(-39.,31.080768958446,-61.14995));
#142597=CARTESIAN_POINT('Ctrl Pts',(-39.,30.638072787808,-61.14995));
#142598=CARTESIAN_POINT('Ctrl Pts',(-39.327731092437,30.3404619167909,-61.14995));
#142599=CARTESIAN_POINT('Origin',(-39.5,31.080768958446,-61.14995));
#142600=CARTESIAN_POINT('Origin',(-40.,31.080768958446,-61.14995));
#142601=CARTESIAN_POINT('Origin',(-39.5,46.91999998,-61.14995));
#142602=CARTESIAN_POINT('Origin',(-42.,-12.9675000200281,-61.14995));
#142603=CARTESIAN_POINT('Origin',(-42.,-58.6035812240174,-61.14995));
#142604=CARTESIAN_POINT('Origin',(-44.5079524583206,-57.475452478349,235.35105));
#142605=CARTESIAN_POINT('',(-44.5079524583206,-59.475452478349,-52.64995));
#142606=CARTESIAN_POINT('Origin',(-44.5079524583206,-57.4754524783489,-52.64995));
#142607=CARTESIAN_POINT('',(-44.5079524583206,-59.475452478349,-55.24995));
#142608=CARTESIAN_POINT('',(-44.5079524583206,-59.475452478349,235.35105));
#142609=CARTESIAN_POINT('Origin',(-44.5079524583206,-57.4754524783489,-55.24995));
#142610=CARTESIAN_POINT('Origin',(0.,45.41999998,-55.24995));
#142611=CARTESIAN_POINT('',(-44.5079524583206,-60.2254524783489,-55.24995));
#142612=CARTESIAN_POINT('Origin',(-44.5079524583206,-57.4754524783489,-55.24995));
#142613=CARTESIAN_POINT('Origin',(-44.5079524583206,-57.4754524783489,-52.64995));
#142614=CARTESIAN_POINT('',(-44.5079524583206,-60.2254524783489,-52.64995));
#142615=CARTESIAN_POINT('',(-43.1572831724516,-55.08000002,-60.64995));
#142616=CARTESIAN_POINT('Ctrl Pts',(-43.1572831724516,-55.08000002,-60.64995));
#142617=CARTESIAN_POINT('Ctrl Pts',(-43.2591939625004,-55.0225379010846,
-60.64995));
#142618=CARTESIAN_POINT('Ctrl Pts',(-43.3646678477756,-54.9716377963979,
-60.6499762002035));
#142619=CARTESIAN_POINT('Ctrl Pts',(-43.5936897926153,-54.8786129298137,
-60.6499834450286));
#142620=CARTESIAN_POINT('Ctrl Pts',(-43.7176454367697,-54.8382440852848,
-60.6498840207772));
#142621=CARTESIAN_POINT('Ctrl Pts',(-43.9338902925228,-54.7844427443954,
-60.6500640176676));
#142622=CARTESIAN_POINT('Ctrl Pts',(-44.0248533307545,-54.7666339585926,
-60.6502067882311));
#142623=CARTESIAN_POINT('Ctrl Pts',(-44.1415243890079,-54.7498576856671,
-60.6502317877326));
#142624=CARTESIAN_POINT('Ctrl Pts',(-44.1665445877625,-54.7466107515332,
-60.6502292561755));
#142625=CARTESIAN_POINT('Ctrl Pts',(-44.2185163631109,-54.74059222261,-60.6502076153997));
#142626=CARTESIAN_POINT('Ctrl Pts',(-44.2454709099202,-54.7378737484825,
-60.6501872468532));
#142627=CARTESIAN_POINT('Ctrl Pts',(-44.3345799963878,-54.7302149256925,
-60.6500997974043));
#142628=CARTESIAN_POINT('Ctrl Pts',(-44.3968571027281,-54.7269903094689,
-60.6500013450001));
#142629=CARTESIAN_POINT('Ctrl Pts',(-44.4753229318579,-54.7255987179309,
-60.6499540212932));
#142630=CARTESIAN_POINT('Ctrl Pts',(-44.4914595252895,-54.7254545924531,
-60.6499486298046));
#142631=CARTESIAN_POINT('Ctrl Pts',(-44.5716245853561,-54.7254442044781,
-60.6499568462188));
#142632=CARTESIAN_POINT('Ctrl Pts',(-44.635636337937,-54.7276720035774,
-60.6500693941759));
#142633=CARTESIAN_POINT('Ctrl Pts',(-44.8100535271152,-54.7398514986511,
-60.6502928314114));
#142634=CARTESIAN_POINT('Ctrl Pts',(-44.9200103914693,-54.7542422074975,
-60.6502860595425));
#142635=CARTESIAN_POINT('Ctrl Pts',(-45.1075048885113,-54.7904085846981,
-60.650061577148));
#142636=CARTESIAN_POINT('Ctrl Pts',(-45.1854986877238,-54.8090210757263,
-60.6499482199387));
#142637=CARTESIAN_POINT('Ctrl Pts',(-45.3711482014312,-54.8619988092867,
-60.6499529098674));
#142638=CARTESIAN_POINT('Ctrl Pts',(-45.4777060174319,-54.8996370242669,
-60.6499736151979));
#142639=CARTESIAN_POINT('Ctrl Pts',(-45.6764516340763,-54.9839240727125,
-60.6499624365077));
#142640=CARTESIAN_POINT('Ctrl Pts',(-45.7689217186581,-55.0294229071022,
-60.64995));
#142641=CARTESIAN_POINT('Ctrl Pts',(-45.8586217441897,-55.08000002,-60.64995));
#142642=CARTESIAN_POINT('',(-42.,-56.3473237326805,-60.64995));
#142643=CARTESIAN_POINT('Origin',(-44.5079524583206,-57.4754524783489,-60.64995));
#142644=CARTESIAN_POINT('Ctrl Pts',(-42.,-58.6035812240174,-60.64995));
#142645=CARTESIAN_POINT('Ctrl Pts',(-41.9586127577213,-58.5115728992456,
-60.64995));
#142646=CARTESIAN_POINT('Ctrl Pts',(-41.9223200866006,-58.4173567491329,
-60.6499639595534));
#142647=CARTESIAN_POINT('Ctrl Pts',(-41.8579031946497,-58.2180944893023,
-60.6499671932779));
#142648=CARTESIAN_POINT('Ctrl Pts',(-41.8306620008004,-58.1129431414189,
-60.6499312309338));
#142649=CARTESIAN_POINT('Ctrl Pts',(-41.7951274186657,-57.9323775711289,
-60.6499828894708));
#142650=CARTESIAN_POINT('Ctrl Pts',(-41.7836058362703,-57.8577298063975,
-60.6500200799918));
#142651=CARTESIAN_POINT('Ctrl Pts',(-41.763699988371,-57.6806798505207,
-60.6500271654877));
#142652=CARTESIAN_POINT('Ctrl Pts',(-41.7579524619679,-57.5781054625679,
-60.6499494618776));
#142653=CARTESIAN_POINT('Ctrl Pts',(-41.7579524619679,-57.3728595819394,
-60.6499505378071));
#142654=CARTESIAN_POINT('Ctrl Pts',(-41.7636932451375,-57.2703453579396,
-60.6500300767565));
#142655=CARTESIAN_POINT('Ctrl Pts',(-41.7835828980496,-57.0933348984399,
-60.6500220919564));
#142656=CARTESIAN_POINT('Ctrl Pts',(-41.795103251114,-57.0186677636544,
-60.6499835586185));
#142657=CARTESIAN_POINT('Ctrl Pts',(-41.8306429216694,-56.8380335332052,
-60.6499306306421));
#142658=CARTESIAN_POINT('Ctrl Pts',(-41.8578946341288,-56.732833798761,
-60.6499676698703));
#142659=CARTESIAN_POINT('Ctrl Pts',(-41.9223259722371,-56.5335329279262,
-60.6499642647307));
#142660=CARTESIAN_POINT('Ctrl Pts',(-41.9586161144824,-56.4393245950086,
-60.64995));
#142661=CARTESIAN_POINT('Ctrl Pts',(-42.,-56.3473237326805,-60.64995));
#142662=CARTESIAN_POINT('Origin',(1.8445455022812E-14,-55.08000002,-61.14995));
#142663=CARTESIAN_POINT('Origin',(-45.8586217441897,-55.08000002,-61.14995));
#142664=CARTESIAN_POINT('Origin',(3.3975957231091E-14,-70.08000002,-58.24995));
#142665=CARTESIAN_POINT('',(-24.7,-73.08000002,-58.24995));
#142666=CARTESIAN_POINT('Origin',(-24.7,-70.08000002,-58.24995));
#142667=CARTESIAN_POINT('',(-24.2,-73.08000002,-58.24995));
#142668=CARTESIAN_POINT('',(41.5,-73.0800000199999,-58.24995));
#142669=CARTESIAN_POINT('Origin',(-24.2,-70.08000002,-58.24995));
#142670=CARTESIAN_POINT('Origin',(-24.7,-70.08000002,-58.24995));
#142671=CARTESIAN_POINT('Origin',(-24.7,-72.58000002,-58.24995));
#142672=CARTESIAN_POINT('Origin',(-38.,46.41999998,-92.34995));
#142673=CARTESIAN_POINT('',(-38.,46.91999998,-58.24995));
#142674=CARTESIAN_POINT('',(-38.,46.91999998,-58.24995));
#142675=CARTESIAN_POINT('Origin',(-38.,46.41999998,-58.24995));
#142676=CARTESIAN_POINT('Origin',(39.,46.91999998,-129.34995));
#142677=CARTESIAN_POINT('',(-38.5,46.91999998,-58.24995));
#142678=CARTESIAN_POINT('',(-38.5,46.91999998,-129.34995));
#142679=CARTESIAN_POINT('',(39.,46.91999998,-58.24995));
#142680=CARTESIAN_POINT('Ctrl Pts',(-39.3571428571429,46.41999998,-92.4750054575003));
#142681=CARTESIAN_POINT('Ctrl Pts',(-39.,46.41999998,-92.3685260300003));
#142682=CARTESIAN_POINT('Ctrl Pts',(-39.,46.41999998,-91.9958480337503));
#142683=CARTESIAN_POINT('Ctrl Pts',(-39.3571428368889,46.5515558031783,
-92.4750054514617));
#142684=CARTESIAN_POINT('Ctrl Pts',(-38.9999999828818,46.5004721093605,
-92.3685260276219));
#142685=CARTESIAN_POINT('Ctrl Pts',(-39.,46.4857778904494,-91.9958480266757));
#142686=CARTESIAN_POINT('Ctrl Pts',(-39.3344873999803,46.6833015096169,
-92.4680006788624));
#142687=CARTESIAN_POINT('Ctrl Pts',(-38.9800988943412,46.5814616819635,
-92.3656111964877));
#142688=CARTESIAN_POINT('Ctrl Pts',(-38.9867843211749,46.5516507463266,
-91.9876757856315));
#142689=CARTESIAN_POINT('Ctrl Pts',(-39.2481885236226,46.925205464765,-92.444400991043));
#142690=CARTESIAN_POINT('Ctrl Pts',(-38.9110717002523,46.7195168934596,
-92.3578064732695));
#142691=CARTESIAN_POINT('Ctrl Pts',(-38.9364433009268,46.6726027208644,
-91.9601428292582));
#142692=CARTESIAN_POINT('Ctrl Pts',(-39.1845108402481,47.0356954006484,
-92.4279818041452));
#142693=CARTESIAN_POINT('Ctrl Pts',(-38.8613908761224,46.7770047607051,
-92.3532077914066));
#142694=CARTESIAN_POINT('Ctrl Pts',(-38.8992979918264,46.7278476911263,
-91.9409870962964));
#142695=CARTESIAN_POINT('Ctrl Pts',(-39.0271570378558,47.2191189043121,
-92.3955365750638));
#142696=CARTESIAN_POINT('Ctrl Pts',(-38.7552585438029,46.8601105768582,
-92.347890765886));
#142697=CARTESIAN_POINT('Ctrl Pts',(-38.8075082704007,46.819559441354,-91.903134346114));
#142698=CARTESIAN_POINT('Ctrl Pts',(-38.9319509445986,47.2935007246494,
-92.3793987064332));
#142699=CARTESIAN_POINT('Ctrl Pts',(-38.6983937732817,46.8857748070212,
-92.3473559512381));
#142700=CARTESIAN_POINT('Ctrl Pts',(-38.7519713842669,46.8567503512399,
-91.884306817494));
#142701=CARTESIAN_POINT('Ctrl Pts',(-38.7257728904125,47.3934379073013,
-92.3566603033275));
#142702=CARTESIAN_POINT('Ctrl Pts',(-38.5942499321354,46.9153405921297,
-92.3486011659899));
#142703=CARTESIAN_POINT('Ctrl Pts',(-38.631700852823,46.9067189447356,-91.8577786938935));
#142704=CARTESIAN_POINT('Ctrl Pts',(-38.6117163199788,47.4199999701223,
-92.34995));
#142705=CARTESIAN_POINT('Ctrl Pts',(-38.5461650349159,46.9199999780196,
-92.3499499995552));
#142706=CARTESIAN_POINT('Ctrl Pts',(-38.5651678532719,46.91999998,-91.849950002847));
#142707=CARTESIAN_POINT('Ctrl Pts',(-38.5,47.41999998,-92.34995));
#142708=CARTESIAN_POINT('Ctrl Pts',(-38.5,46.91999998,-92.34995));
#142709=CARTESIAN_POINT('Ctrl Pts',(-38.5,46.91999998,-91.84995));
#142710=CARTESIAN_POINT('Origin',(-39.5,46.41999998,-91.9958480337503));
#142711=CARTESIAN_POINT('Ctrl Pts',(-39.,46.41999998,-91.9958480337503));
#142712=CARTESIAN_POINT('Ctrl Pts',(-39.,46.4857778904494,-91.9958480266757));
#142713=CARTESIAN_POINT('Ctrl Pts',(-38.9867843211749,46.5516507463266,
-91.9876757856315));
#142714=CARTESIAN_POINT('Ctrl Pts',(-38.9364433009268,46.6726027208644,
-91.9601428292582));
#142715=CARTESIAN_POINT('Ctrl Pts',(-38.8992979918264,46.7278476911263,
-91.9409870962964));
#142716=CARTESIAN_POINT('Ctrl Pts',(-38.8075082704007,46.819559441354,-91.903134346114));
#142717=CARTESIAN_POINT('Ctrl Pts',(-38.7519713842669,46.8567503512399,
-91.884306817494));
#142718=CARTESIAN_POINT('Ctrl Pts',(-38.631700852823,46.9067189447356,-91.8577786938935));
#142719=CARTESIAN_POINT('Ctrl Pts',(-38.5651678532719,46.91999998,-91.849950002847));
#142720=CARTESIAN_POINT('Ctrl Pts',(-38.5,46.91999998,-91.84995));
#142721=CARTESIAN_POINT('Ctrl Pts',(-41.0540572871253,28.7076050220164,
-93.3976987687948));
#142722=CARTESIAN_POINT('Ctrl Pts',(-40.9209666515892,28.8387123238495,
-93.5739383154377));
#142723=CARTESIAN_POINT('Ctrl Pts',(-40.9899542848408,29.0638025010082,
-93.6765918018241));
#142724=CARTESIAN_POINT('Ctrl Pts',(-41.181465342889,28.5820956174237,-93.4924903917862));
#142725=CARTESIAN_POINT('Ctrl Pts',(-40.9927653037546,28.7197223139655,
-93.6733291751567));
#142726=CARTESIAN_POINT('Ctrl Pts',(-41.0445777715999,29.0010249744694,
-93.7578714615268));
#142727=CARTESIAN_POINT('Ctrl Pts',(-41.3136336664734,28.5141965951637,
-93.601569918277));
#142728=CARTESIAN_POINT('Ctrl Pts',(-41.064373682842,28.640994986895,-93.7860557549848));
#142729=CARTESIAN_POINT('Ctrl Pts',(-41.1012013116007,28.9670983124193,
-93.8513385014916));
#142730=CARTESIAN_POINT('Ctrl Pts',(-41.5532792074141,28.4325824175145,
-93.828366995811));
#142731=CARTESIAN_POINT('Ctrl Pts',(-41.1909352247283,28.5106646509549,
-94.0164009875504));
#142732=CARTESIAN_POINT('Ctrl Pts',(-41.203906529354,28.9262911739198,-94.0457359962981));
#142733=CARTESIAN_POINT('Ctrl Pts',(-41.6609761593771,28.4199999800001,
-93.9453729847263));
#142734=CARTESIAN_POINT('Ctrl Pts',(-41.245616944193,28.4623003387481,-94.1347575623882));
#142735=CARTESIAN_POINT('Ctrl Pts',(-41.2500626594833,28.9199999557335,
-94.1460275680244));
#142736=CARTESIAN_POINT('Ctrl Pts',(-41.7558360441699,28.41999998,-94.0656090587062));
#142737=CARTESIAN_POINT('Ctrl Pts',(-41.2907166092886,28.4199999800001,
-94.2490863360339));
#142738=CARTESIAN_POINT('Ctrl Pts',(-41.2907166092886,28.91999998,-94.2490863360339));
#142739=CARTESIAN_POINT('',(-41.0540572871253,28.7076050220164,-93.3976987687948));
#142740=CARTESIAN_POINT('Origin',(-41.4049466656476,29.0638025010082,-93.3976987687947));
#142741=CARTESIAN_POINT('Origin',(-41.75583604417,28.91999998,-94.0656090587062));
#142742=CARTESIAN_POINT('Ctrl Pts',(-41.7558360441701,28.41999998,-94.0656090587062));
#142743=CARTESIAN_POINT('Ctrl Pts',(-41.6609761593771,28.4199999800001,
-93.9453729847263));
#142744=CARTESIAN_POINT('Ctrl Pts',(-41.5532792074141,28.4325824175145,
-93.828366995811));
#142745=CARTESIAN_POINT('Ctrl Pts',(-41.3136336664734,28.5141965951637,
-93.601569918277));
#142746=CARTESIAN_POINT('Ctrl Pts',(-41.181465342889,28.5820956174237,-93.4924903917862));
#142747=CARTESIAN_POINT('Ctrl Pts',(-41.0540572871253,28.7076050220164,
-93.3976987687948));
#142748=CARTESIAN_POINT('Origin',(-38.5,28.91999998,-95.34995));
#142749=CARTESIAN_POINT('Origin',(-42.,28.91999998,-95.34995));
#142750=CARTESIAN_POINT('Origin',(-39.5,58.91999998,-91.9958480337503));
#142751=CARTESIAN_POINT('Origin',(-39.5,31.080768958446,-91.9958480337503));
#142752=CARTESIAN_POINT('Ctrl Pts',(-39.,31.080768958446,-91.9958480337503));
#142753=CARTESIAN_POINT('Ctrl Pts',(-39.,31.080768958446,-92.3685260300003));
#142754=CARTESIAN_POINT('Ctrl Pts',(-39.3571428571429,31.080768958446,-92.4750054575003));
#142755=CARTESIAN_POINT('Ctrl Pts',(-39.,30.7973529986378,-91.9958480635187));
#142756=CARTESIAN_POINT('Ctrl Pts',(-39.0000001561187,30.8288322275033,
-92.3685260646169));
#142757=CARTESIAN_POINT('Ctrl Pts',(-39.3571429430277,30.9391538899445,
-92.4750054831062));
#142758=CARTESIAN_POINT('Ctrl Pts',(-39.1237015311635,30.5257400818631,
-92.0131591004063));
#142759=CARTESIAN_POINT('Ctrl Pts',(-39.0995023767794,30.5843250255347,
-92.3886066067861));
#142760=CARTESIAN_POINT('Ctrl Pts',(-39.410274588038,30.8031308123719,-92.4898846529936));
#142761=CARTESIAN_POINT('Ctrl Pts',(-39.3277310924369,30.3404619167909,
-92.0491293459315));
#142762=CARTESIAN_POINT('Ctrl Pts',(-39.2532568247562,30.4080916052285,
-92.4345203712043));
#142763=CARTESIAN_POINT('Ctrl Pts',(-39.4975990396159,30.7106154376184,
-92.5206751536556));
#142764=CARTESIAN_POINT('',(-39.3277310924369,30.3404619167909,-92.0491293459315));
#142765=CARTESIAN_POINT('Origin',(-39.6638655462185,30.7106154376184,-92.0491293459315));
#142766=CARTESIAN_POINT('Ctrl Pts',(-39.3277310924369,30.3404619167909,
-92.0491293459315));
#142767=CARTESIAN_POINT('Ctrl Pts',(-39.1237015311635,30.5257400818631,
-92.0131591004063));
#142768=CARTESIAN_POINT('Ctrl Pts',(-39.,30.7973529986378,-91.9958480635187));
#142769=CARTESIAN_POINT('Ctrl Pts',(-39.,31.080768958446,-91.9958480337503));
#142770=CARTESIAN_POINT('Ctrl Pts',(-40.9899542848408,29.0638025010082,
-93.6765918018241));
#142771=CARTESIAN_POINT('Ctrl Pts',(-40.9209666515892,28.8387123238495,
-93.5739383154377));
#142772=CARTESIAN_POINT('Ctrl Pts',(-41.0540572871253,28.7076050220164,
-93.3976987687948));
#142773=CARTESIAN_POINT('Ctrl Pts',(-40.7930602005308,29.2900891143653,
-93.3836137237161));
#142774=CARTESIAN_POINT('Ctrl Pts',(-40.6946394065552,29.0602110175707,
-93.2636650794047));
#142775=CARTESIAN_POINT('Ctrl Pts',(-40.8263518506557,28.931917162897,-93.0559775318146));
#142776=CARTESIAN_POINT('Ctrl Pts',(-40.5646325235533,29.548843193136,-93.1505624120075));
#142777=CARTESIAN_POINT('Ctrl Pts',(-40.4345448959912,29.3109818121476,
-93.0268336432776));
#142778=CARTESIAN_POINT('Ctrl Pts',(-40.5620537232219,29.1885351995273,
-92.7839978150636));
#142779=CARTESIAN_POINT('Ctrl Pts',(-40.0606440851126,30.1068692044787,
-92.7683994467215));
#142780=CARTESIAN_POINT('Ctrl Pts',(-39.8699190705461,29.8439046252157,
-92.6499647524336));
#142781=CARTESIAN_POINT('Ctrl Pts',(-39.979050150362,29.7418321774292,-92.3381410201203));
#142782=CARTESIAN_POINT('Ctrl Pts',(-39.7830757934441,30.4081688522969,
-92.6213339269874));
#142783=CARTESIAN_POINT('Ctrl Pts',(-39.5589873293178,30.1314683688792,
-92.5153277294035));
#142784=CARTESIAN_POINT('Ctrl Pts',(-39.6579655806366,30.0405777253273,
-92.1665648604216));
#142785=CARTESIAN_POINT('Ctrl Pts',(-39.4975990396159,30.7106154376184,
-92.5206751536556));
#142786=CARTESIAN_POINT('Ctrl Pts',(-39.2532568247562,30.4080916052286,
-92.4345203712043));
#142787=CARTESIAN_POINT('Ctrl Pts',(-39.3277310924369,30.3404619167909,
-92.0491293459315));
#142788=CARTESIAN_POINT('Ctrl Pts',(-41.0540572871253,28.7076050220164,
-93.3976987687948));
#142789=CARTESIAN_POINT('Ctrl Pts',(-40.8263518506557,28.931917162897,-93.0559775318146));
#142790=CARTESIAN_POINT('Ctrl Pts',(-40.5620537232219,29.1885351995273,
-92.7839978150636));
#142791=CARTESIAN_POINT('Ctrl Pts',(-39.979050150362,29.7418321774292,-92.3381410201203));
#142792=CARTESIAN_POINT('Ctrl Pts',(-39.6579655806366,30.0405777253273,
-92.1665648604216));
#142793=CARTESIAN_POINT('Ctrl Pts',(-39.3277310924369,30.3404619167909,
-92.0491293459315));
#142794=CARTESIAN_POINT('Origin',(-4.,46.41999998,-92.34995));
#142795=CARTESIAN_POINT('',(-4.,46.91999998,-57.9072287192657));
#142796=CARTESIAN_POINT('Origin',(39.,46.91999998,-129.34995));
#142797=CARTESIAN_POINT('',(-4.5,46.91999998,-92.34995));
#142798=CARTESIAN_POINT('Origin',(-4.5,46.41999998,-92.34995));
#142799=CARTESIAN_POINT('Ctrl Pts',(-5.00000098575356,31.8716754827171,
-91.8489571492625));
#142800=CARTESIAN_POINT('Ctrl Pts',(-4.99900616154964,31.8716754827171,
-92.34995));
#142801=CARTESIAN_POINT('Ctrl Pts',(-5.5,31.8716754827171,-92.34995));
#142802=CARTESIAN_POINT('Ctrl Pts',(-5.00000096584847,31.7882063435841,
-91.8489671288812));
#142803=CARTESIAN_POINT('Ctrl Pts',(-4.99903601393703,31.7072113826353,
-92.3399186475543));
#142804=CARTESIAN_POINT('Ctrl Pts',(-5.48989377680063,31.7056523166615,
-92.34995));
#142805=CARTESIAN_POINT('Ctrl Pts',(-5.0000009456393,31.7039607739183,-91.8276307576481));
#142806=CARTESIAN_POINT('Ctrl Pts',(-4.99906555653788,31.5446619586649,
-92.2883582792096));
#142807=CARTESIAN_POINT('Ctrl Pts',(-5.47963373781052,31.538103809625,-92.3071746231476));
#142808=CARTESIAN_POINT('Ctrl Pts',(-5.00000091915851,31.5940866659345,
-91.7681041344864));
#142809=CARTESIAN_POINT('Ctrl Pts',(-4.99910325428599,31.3370094182925,
-92.161272810455));
#142810=CARTESIAN_POINT('Ctrl Pts',(-5.46619042199875,31.3196047327668,
-92.1878686007335));
#142811=CARTESIAN_POINT('Ctrl Pts',(-5.00000091080218,31.559505537537,-91.7433851154801));
#142812=CARTESIAN_POINT('Ctrl Pts',(-4.99911492812357,31.2726858878274,
-92.1103972204605));
#142813=CARTESIAN_POINT('Ctrl Pts',(-5.46194839019336,31.2508398250121,
-92.1383294170381));
#142814=CARTESIAN_POINT('Ctrl Pts',(-5.00000089592572,31.4980571027819,
-91.6865378587354));
#142815=CARTESIAN_POINT('Ctrl Pts',(-4.99913545432373,31.1595480268538,
-91.9961676804234));
#142816=CARTESIAN_POINT('Ctrl Pts',(-5.45439667136824,31.1286541135227,
-92.0244078521253));
#142817=CARTESIAN_POINT('Ctrl Pts',(-5.00000088941156,31.4712115049486,
-91.6546739801726));
#142818=CARTESIAN_POINT('Ctrl Pts',(-4.99914433728297,31.1105664451877,
-91.9333048742068));
#142819=CARTESIAN_POINT('Ctrl Pts',(-5.45108997919633,31.0752759499814,
-91.9605552262364));
#142820=CARTESIAN_POINT('Ctrl Pts',(-5.00000087274503,31.4026135113337,
-91.5484928091743));
#142821=CARTESIAN_POINT('Ctrl Pts',(-4.99916680129901,30.9866628751625,
-91.7272955383522));
#142822=CARTESIAN_POINT('Ctrl Pts',(-5.44262999595016,30.938884482232,-91.7477840212027));
#142823=CARTESIAN_POINT('Ctrl Pts',(-5.00000086614597,31.3755689941199,
-91.4665221319677));
#142824=CARTESIAN_POINT('Ctrl Pts',(-4.99917557417014,30.9382275273277,
-91.5708670061703));
#142825=CARTESIAN_POINT('Ctrl Pts',(-5.43928039898085,30.8851161679224,
-91.5835323055617));
#142826=CARTESIAN_POINT('Ctrl Pts',(-5.00000086340344,31.3643200540024,
-91.3002194649783));
#142827=CARTESIAN_POINT('Ctrl Pts',(-4.99917920690221,30.9181743619019,
-91.2558237036598));
#142828=CARTESIAN_POINT('Ctrl Pts',(-5.43788833142316,30.8627516985332,
-91.2503023235849));
#142829=CARTESIAN_POINT('Ctrl Pts',(-5.00000086731321,31.3803302826731,
-91.214808683899));
#142830=CARTESIAN_POINT('Ctrl Pts',(-4.99917405374185,30.946764229838,-91.0936720204704));
#142831=CARTESIAN_POINT('Ctrl Pts',(-5.4398728408893,30.894582824155,-91.0791566847487));
#142832=CARTESIAN_POINT('Ctrl Pts',(-5.0000008759766,31.4159376038031,-91.1390388927801));
#142833=CARTESIAN_POINT('Ctrl Pts',(-4.99916246706242,31.0105597677355,
-90.9485621815415));
#142834=CARTESIAN_POINT('Ctrl Pts',(-5.44427033638568,30.9653765476951,
-90.9273317382594));
#142835=CARTESIAN_POINT('Origin',(-5.5,31.415090518797,-91.1386408691297));
#142836=CARTESIAN_POINT('Ctrl Pts',(-12.,30.2507177004773,-91.1386408691297));
#142837=CARTESIAN_POINT('Ctrl Pts',(-12.,29.679733250215,-90.8631216114042));
#142838=CARTESIAN_POINT('Ctrl Pts',(-11.3834743397155,29.812801930373,-90.9273317382593));
#142839=CARTESIAN_POINT('Ctrl Pts',(-12.,30.2139234693476,-91.2148931255634));
#142840=CARTESIAN_POINT('Ctrl Pts',(-11.9999999999987,29.5832417343753,
-91.0342442171839));
#142841=CARTESIAN_POINT('Ctrl Pts',(-11.3742392183232,29.741677094381,-91.0798230944648));
#142842=CARTESIAN_POINT('Ctrl Pts',(-12.,30.1973151560885,-91.3015254072135));
#142843=CARTESIAN_POINT('Ctrl Pts',(-11.9999999999999,29.5383067623994,
-91.2361587739122));
#142844=CARTESIAN_POINT('Ctrl Pts',(-11.3700547859617,29.7095698537212,
-91.2531008141058));
#142845=CARTESIAN_POINT('Ctrl Pts',(-12.,30.2066913195442,-91.427825927492));
#142846=CARTESIAN_POINT('Ctrl Pts',(-12.0000000000001,29.5635939180596,
-91.5323968928992));
#142847=CARTESIAN_POINT('Ctrl Pts',(-11.3724129716406,29.7276939951996,
-91.5057018551446));
#142848=CARTESIAN_POINT('Ctrl Pts',(-12.,30.2155293203062,-91.4701692696895));
#142849=CARTESIAN_POINT('Ctrl Pts',(-11.9999999999998,29.5872932859939,
-91.6306703852657));
#142850=CARTESIAN_POINT('Ctrl Pts',(-11.374636075473,29.7447777509884,-91.5903885436157));
#142851=CARTESIAN_POINT('Ctrl Pts',(-12.,30.2434629903521,-91.5500105484349));
#142852=CARTESIAN_POINT('Ctrl Pts',(-12.0000000000001,29.6609253730622,
-91.812155424579));
#142853=CARTESIAN_POINT('Ctrl Pts',(-11.3816540502047,29.7987767762788,
-91.7500710926331));
#142854=CARTESIAN_POINT('Ctrl Pts',(-12.,30.2626690028682,-91.5881956385046));
#142855=CARTESIAN_POINT('Ctrl Pts',(-11.9999999999999,29.7106471563183,
-91.8964616250679));
#142856=CARTESIAN_POINT('Ctrl Pts',(-11.3864765114273,29.8359053318054,
-91.8264412916623));
#142857=CARTESIAN_POINT('Ctrl Pts',(-12.,30.3342288077533,-91.6940226905849));
#142858=CARTESIAN_POINT('Ctrl Pts',(-12.0000000000001,29.8895113426933,
-92.1195167159054));
#142859=CARTESIAN_POINT('Ctrl Pts',(-11.4044123087811,29.9742563988052,
-92.0380953518635));
#142860=CARTESIAN_POINT('Ctrl Pts',(-12.,30.3998197343385,-91.7515247512526));
#142861=CARTESIAN_POINT('Ctrl Pts',(-11.9999999999989,30.0452979686933,
-92.2283418495211));
#142862=CARTESIAN_POINT('Ctrl Pts',(-11.4208142717207,30.101082992511,-92.1530994985312));
#142863=CARTESIAN_POINT('Ctrl Pts',(-12.,30.5498659135928,-91.8294071489743));
#142864=CARTESIAN_POINT('Ctrl Pts',(-12.0000000000011,30.3770555999401,
-92.3523349137576));
#142865=CARTESIAN_POINT('Ctrl Pts',(-11.458128525139,30.3912975665021,-92.3088643019226));
#142866=CARTESIAN_POINT('Ctrl Pts',(-12.,30.635088667613,-91.8499499468525));
#142867=CARTESIAN_POINT('Ctrl Pts',(-12.,30.5530678891822,-92.3711185577562));
#142868=CARTESIAN_POINT('Ctrl Pts',(-11.4792261802719,30.5561711606282,
-92.34995));
#142869=CARTESIAN_POINT('Ctrl Pts',(-12.,30.7194735506599,-91.84995));
#142870=CARTESIAN_POINT('Ctrl Pts',(-12.,30.7194735506598,-92.34995));
#142871=CARTESIAN_POINT('Ctrl Pts',(-11.5,30.7194735506599,-92.34995));
#142872=CARTESIAN_POINT('Origin',(-11.5,30.2507177004773,-91.1386408691297));
#142873=CARTESIAN_POINT('Origin',(-12.5,46.41999998,-92.34995));
#142874=CARTESIAN_POINT('',(-12.5,46.91999998,-58.2396719107252));
#142875=CARTESIAN_POINT('Origin',(39.,46.91999998,-129.34995));
#142876=CARTESIAN_POINT('',(-13.,46.91999998,-92.34995));
#142877=CARTESIAN_POINT('Origin',(-13.,46.41999998,-92.34995));
#142878=CARTESIAN_POINT('Ctrl Pts',(-13.5,29.9836543272765,-91.84995));
#142879=CARTESIAN_POINT('Ctrl Pts',(-13.5,29.9836543272765,-92.34995));
#142880=CARTESIAN_POINT('Ctrl Pts',(-14.,29.9836543272765,-92.34995));
#142881=CARTESIAN_POINT('Ctrl Pts',(-13.5,29.9498130224307,-91.8499499813658));
#142882=CARTESIAN_POINT('Ctrl Pts',(-13.5,29.9198591164476,-92.340077310875));
#142883=CARTESIAN_POINT('Ctrl Pts',(-13.9900288285115,29.9192223045234,
-92.34995));
#142884=CARTESIAN_POINT('Ctrl Pts',(-13.5,29.9164799575816,-91.8468718299503));
#142885=CARTESIAN_POINT('Ctrl Pts',(-13.4999999999992,29.8581345500688,
-92.3247747757233));
#142886=CARTESIAN_POINT('Ctrl Pts',(-13.9801870069313,29.8557668849998,
-92.3437935523175));
#142887=CARTESIAN_POINT('Ctrl Pts',(-13.5,29.8836583509375,-91.8408299848543));
#142888=CARTESIAN_POINT('Ctrl Pts',(-13.5,29.7983343836869,-92.3043420473086));
#142889=CARTESIAN_POINT('Ctrl Pts',(-13.9704776589253,29.7932964571608,
-92.3317099697086));
#142890=CARTESIAN_POINT('Origin',(-14.,29.8836583509375,-91.8408299848543));
#142891=CARTESIAN_POINT('Ctrl Pts',(-13.5,29.8836583509376,-91.8408299848543));
#142892=CARTESIAN_POINT('Ctrl Pts',(-13.5,29.798334383687,-92.3043420473087));
#142893=CARTESIAN_POINT('Ctrl Pts',(-13.9704776589254,29.793296457161,-92.3317099697086));
#142894=CARTESIAN_POINT('Ctrl Pts',(-13.5,29.8088158028921,-91.8270528245268));
#142895=CARTESIAN_POINT('Ctrl Pts',(-13.5,29.6658016093476,-92.2593052595342));
#142896=CARTESIAN_POINT('Ctrl Pts',(-13.9485824763266,29.6507732526529,
-92.3041572803908));
#142897=CARTESIAN_POINT('Ctrl Pts',(-13.5,29.7360856593875,-91.7971835648529));
#142898=CARTESIAN_POINT('Ctrl Pts',(-13.5,29.5406281722262,-92.1878683704653));
#142899=CARTESIAN_POINT('Ctrl Pts',(-13.9277414892694,29.5120300570818,
-92.2444171371624));
#142900=CARTESIAN_POINT('Ctrl Pts',(-13.5,29.6110266364568,-91.7101609842055));
#142901=CARTESIAN_POINT('Ctrl Pts',(-13.5,29.3333704157687,-92.0065554596633));
#142902=CARTESIAN_POINT('Ctrl Pts',(-13.8924131672203,29.2732201982241,
-92.0703719609639));
#142903=CARTESIAN_POINT('Ctrl Pts',(-13.5,29.5578590401594,-91.6523482016898));
#142904=CARTESIAN_POINT('Ctrl Pts',(-13.4999999999999,29.2476129207544,
-91.895386283959));
#142905=CARTESIAN_POINT('Ctrl Pts',(-13.8776710606793,29.1715523493698,
-91.9547463954628));
#142906=CARTESIAN_POINT('Ctrl Pts',(-13.5,29.4834479217461,-91.5199437062307));
#142907=CARTESIAN_POINT('Ctrl Pts',(-13.5000000000001,29.1302566914018,
-91.6522607622863));
#142908=CARTESIAN_POINT('Ctrl Pts',(-13.8571693529918,29.0291974882966,
-91.6899374203782));
#142909=CARTESIAN_POINT('Ctrl Pts',(-13.5,29.4617011701904,-91.4445487431295));
#142910=CARTESIAN_POINT('Ctrl Pts',(-13.5000000000001,29.0962692564556,
-91.5174684103174));
#142911=CARTESIAN_POINT('Ctrl Pts',(-13.851254772454,28.9875557647693,-91.5391474846049));
#142912=CARTESIAN_POINT('Ctrl Pts',(-13.5,29.4559384360516,-91.2911813034188));
#142913=CARTESIAN_POINT('Ctrl Pts',(-13.4999999999999,29.0873381907095,
-91.2460073456115));
#142914=CARTESIAN_POINT('Ctrl Pts',(-13.8496827900737,28.9765232161018,
-91.2324126084916));
#142915=CARTESIAN_POINT('Ctrl Pts',(-13.5,29.4717444256829,-91.2146593048585));
#142916=CARTESIAN_POINT('Ctrl Pts',(-13.4999999999996,29.1119956223332,
-91.1098405101534));
#142917=CARTESIAN_POINT('Ctrl Pts',(-13.8539744318671,29.0067940350096,
-91.0793665022882));
#142918=CARTESIAN_POINT('Ctrl Pts',(-13.5,29.5044693674792,-91.1451435916293));
#142919=CARTESIAN_POINT('Ctrl Pts',(-13.5,29.162996502681,-90.984393353347));
#142920=CARTESIAN_POINT('Ctrl Pts',(-13.8629670146647,29.0694104105324,
-90.9403371832566));
#142921=CARTESIAN_POINT('Origin',(-14.,29.5044693674792,-91.1451435916293));
#142922=CARTESIAN_POINT('Ctrl Pts',(-21.7666112105514,28.41999998,-87.8078183592076));
#142923=CARTESIAN_POINT('Ctrl Pts',(-20.7092106783515,28.41999998,-86.6470800003654));
#142924=CARTESIAN_POINT('Ctrl Pts',(-19.8416434885933,29.3176415862829,
-85.6947270505041));
#142925=CARTESIAN_POINT('Ctrl Pts',(-20.7402388551495,28.41999998,-88.7428151801658));
#142926=CARTESIAN_POINT('Ctrl Pts',(-19.7296405475835,28.4199999799976,
-87.5847244149266));
#142927=CARTESIAN_POINT('Ctrl Pts',(-18.8896716409139,29.2827357288726,
-86.6297133466452));
#142928=CARTESIAN_POINT('Ctrl Pts',(-19.6830654074503,28.4199999800001,
-89.6522445020127));
#142929=CARTESIAN_POINT('Ctrl Pts',(-18.7197222668567,28.41999998,-88.4987039616193));
#142930=CARTESIAN_POINT('Ctrl Pts',(-17.9119477871191,29.2478866829953,
-87.5391531932496));
#142931=CARTESIAN_POINT('Ctrl Pts',(-17.4871574021565,28.4199999800001,
-91.4036210595759));
#142932=CARTESIAN_POINT('Ctrl Pts',(-16.6238286994528,28.41999998,-90.2586559409325));
#142933=CARTESIAN_POINT('Ctrl Pts',(-15.8876250911483,29.1791411788287,
-89.290529750932));
#142934=CARTESIAN_POINT('Ctrl Pts',(-16.353131902533,28.4199999800001,-92.2410073071712));
#142935=CARTESIAN_POINT('Ctrl Pts',(-15.5423832476573,28.4199999800097,
-91.1005048403699));
#142936=CARTESIAN_POINT('Ctrl Pts',(-14.8453850851454,29.1454134093176,
-90.1279271408305));
#142937=CARTESIAN_POINT('Ctrl Pts',(-15.1919283151595,28.4199999800001,
-93.0160464292372));
#142938=CARTESIAN_POINT('Ctrl Pts',(-14.4341913591531,28.41999998,-91.8807658383619));
#142939=CARTESIAN_POINT('Ctrl Pts',(-13.781556827362,29.1135284095041,-90.9029551205337));
#142940=CARTESIAN_POINT('',(-20.,28.4199999800001,-89.3628471840451));
#142941=CARTESIAN_POINT('Origin',(-20.0888710624269,28.4200000295341,-83.1773333845304));
#142942=CARTESIAN_POINT('Ctrl Pts',(-19.8077681778583,29.3163999071086,
-85.7279764688716));
#142943=CARTESIAN_POINT('Ctrl Pts',(-19.8136574212126,29.2576540355216,
-85.8367033527245));
#142944=CARTESIAN_POINT('Ctrl Pts',(-19.8196451473997,29.202108371412,-85.946486159213));
#142945=CARTESIAN_POINT('Ctrl Pts',(-19.8256705338347,29.1496220282844,
-86.0572294761739));
#142946=CARTESIAN_POINT('Ctrl Pts',(-19.831938355614,29.0950238629849,-86.1724286225603));
#142947=CARTESIAN_POINT('Ctrl Pts',(-19.8382471186921,29.0437352856753,
-86.288667271822));
#142948=CARTESIAN_POINT('Ctrl Pts',(-19.8445663866126,28.9956132814831,
-86.4058785872911));
#142949=CARTESIAN_POINT('Ctrl Pts',(-19.8509287374279,28.9471631957372,
-86.5238890147492));
#142950=CARTESIAN_POINT('Ctrl Pts',(-19.8573022294804,28.9019223155722,
-86.6428858945738));
#142951=CARTESIAN_POINT('Ctrl Pts',(-19.863688044158,28.8597720721441,-86.7628362248108));
#142952=CARTESIAN_POINT('Ctrl Pts',(-19.870186584175,28.8168777732216,-86.884903973478));
#142953=CARTESIAN_POINT('Ctrl Pts',(-19.8766984153534,28.7771835491368,
-87.0079596644619));
#142954=CARTESIAN_POINT('Ctrl Pts',(-19.8832503422814,28.7406029640851,
-87.1319972358868));
#142955=CARTESIAN_POINT('Ctrl Pts',(-19.8894441753394,28.7060216814381,
-87.2492555659603));
#142956=CARTESIAN_POINT('Ctrl Pts',(-19.8956744956213,28.6742230445864,
-87.3673920903953));
#142957=CARTESIAN_POINT('Ctrl Pts',(-19.9019775505939,28.6451714612775,
-87.486417589477));
#142958=CARTESIAN_POINT('Ctrl Pts',(-19.9110636635093,28.6032924093798,
-87.6579977405552));
#142959=CARTESIAN_POINT('Ctrl Pts',(-19.9202391291903,28.5671050608127,
-87.8316012622964));
#142960=CARTESIAN_POINT('Ctrl Pts',(-19.9294481187907,28.5367577809419,
-88.0065835848011));
#142961=CARTESIAN_POINT('Ctrl Pts',(-19.9386272558149,28.5065088771713,
-88.180998671014));
#142962=CARTESIAN_POINT('Ctrl Pts',(-19.9478394433303,28.4820622096005,
-88.3567835651411));
#142963=CARTESIAN_POINT('Ctrl Pts',(-19.9570427327963,28.463517168047,-88.5332849397664));
#142964=CARTESIAN_POINT('Ctrl Pts',(-19.9661625657539,28.4451402951058,
-88.708185779221));
#142965=CARTESIAN_POINT('Ctrl Pts',(-19.9752734569136,28.4325584744372,
-88.883790083378));
#142966=CARTESIAN_POINT('Ctrl Pts',(-19.9843510994179,28.4258221481163,
-89.0594484841297));
#142967=CARTESIAN_POINT('Ctrl Pts',(-19.989578681727,28.4219428699572,-89.1606056675928));
#142968=CARTESIAN_POINT('Ctrl Pts',(-19.9947955600196,28.420001288699,-89.2617805437457));
#142969=CARTESIAN_POINT('Ctrl Pts',(-20.,28.4199999806615,-89.3628471840451));
#142970=CARTESIAN_POINT('Origin',(-13.9259921622961,31.8088924073546,-92.6508709683574));
#142971=CARTESIAN_POINT('Origin',(-60.,28.41999998,-55.24995));
#142972=CARTESIAN_POINT('',(-20.,28.4199999800001,-91.34995));
#142973=CARTESIAN_POINT('Ctrl Pts',(-20.,29.41999998,-92.34995));
#142974=CARTESIAN_POINT('Ctrl Pts',(-20.,28.41999998,-92.34995));
#142975=CARTESIAN_POINT('Ctrl Pts',(-20.,28.41999998,-91.34995));
#142976=CARTESIAN_POINT('Ctrl Pts',(-20.5,29.41999998,-92.34995));
#142977=CARTESIAN_POINT('Ctrl Pts',(-20.5,28.41999998,-92.34995));
#142978=CARTESIAN_POINT('Ctrl Pts',(-20.5,28.41999998,-91.34995));
#142979=CARTESIAN_POINT('Ctrl Pts',(-20.5,29.41999998,-91.84995));
#142980=CARTESIAN_POINT('Ctrl Pts',(-20.5,28.91999998,-91.84995));
#142981=CARTESIAN_POINT('Ctrl Pts',(-20.5,28.91999998,-91.34995));
#142982=CARTESIAN_POINT('Origin',(-20.,28.9199999800001,-91.34995));
#142983=CARTESIAN_POINT('Origin',(-21.,46.41999998,-92.34995));
#142984=CARTESIAN_POINT('',(-21.,46.91999998,-58.24995));
#142985=CARTESIAN_POINT('',(-21.,46.91999998,-58.24995));
#142986=CARTESIAN_POINT('Origin',(-21.,46.41999998,-58.24995));
#142987=CARTESIAN_POINT('Origin',(39.,46.91999998,-129.34995));
#142988=CARTESIAN_POINT('',(-21.5,46.91999998,-58.24995));
#142989=CARTESIAN_POINT('',(-21.5,46.91999998,-92.34995));
#142990=CARTESIAN_POINT('',(39.,46.91999998,-58.24995));
#142991=CARTESIAN_POINT('Origin',(-21.5,46.41999998,-92.34995));
#142992=CARTESIAN_POINT('Origin',(-21.5,46.41999998,-58.24995));
#142993=CARTESIAN_POINT('Ctrl Pts',(-22.5,28.41999998,-91.34995));
#142994=CARTESIAN_POINT('Ctrl Pts',(-22.5,28.41999998,-92.34995));
#142995=CARTESIAN_POINT('Ctrl Pts',(-22.5,29.41999998,-92.34995));
#142996=CARTESIAN_POINT('Ctrl Pts',(-22.,28.41999998,-91.34995));
#142997=CARTESIAN_POINT('Ctrl Pts',(-22.,28.41999998,-92.34995));
#142998=CARTESIAN_POINT('Ctrl Pts',(-22.,29.41999998,-92.34995));
#142999=CARTESIAN_POINT('Ctrl Pts',(-22.,28.91999998,-91.34995));
#143000=CARTESIAN_POINT('Ctrl Pts',(-22.,28.91999998,-91.84995));
#143001=CARTESIAN_POINT('Ctrl Pts',(-22.,29.41999998,-91.84995));
#143002=CARTESIAN_POINT('Origin',(-22.5,28.9199999800001,-91.34995));
#143003=CARTESIAN_POINT('Origin',(-60.,28.41999998,-55.24995));
#143004=CARTESIAN_POINT('',(-28.5,28.41999998,-80.9397703408579));
#143005=CARTESIAN_POINT('',(-28.5,28.41999998,-91.34995));
#143006=CARTESIAN_POINT('',(-22.5,28.41999998,-87.1305533863517));
#143007=CARTESIAN_POINT('Ctrl Pts',(-22.5,28.41999998,-87.1305533863517));
#143008=CARTESIAN_POINT('Ctrl Pts',(-22.9996306884463,28.4199999800004,
-86.6629501694543));
#143009=CARTESIAN_POINT('Ctrl Pts',(-23.4925641465851,28.4199999800118,
-86.1891300413705));
#143010=CARTESIAN_POINT('Ctrl Pts',(-23.9796464830031,28.4199999800316,
-85.7094996089126));
#143011=CARTESIAN_POINT('Ctrl Pts',(-24.4984981224756,28.4199999800526,
-85.1985859140088));
#143012=CARTESIAN_POINT('Ctrl Pts',(-25.0107103809229,28.4199999800828,
-84.6810791338099));
#143013=CARTESIAN_POINT('Ctrl Pts',(-25.5172665601457,28.4199999801285,
-84.15742328956));
#143014=CARTESIAN_POINT('Ctrl Pts',(-25.9324040800905,28.419999980166,-83.7282720968532));
#143015=CARTESIAN_POINT('Ctrl Pts',(-26.3437419377233,28.4199999802138,
-83.2949899596838));
#143016=CARTESIAN_POINT('Ctrl Pts',(-26.7518048403012,28.4199999802818,
-82.85780136844));
#143017=CARTESIAN_POINT('Ctrl Pts',(-27.3023421757726,28.4199999803735,
-82.2679691621764));
#143018=CARTESIAN_POINT('Ctrl Pts',(-27.8456527104533,28.4199999804996,
-81.6723376117165));
#143019=CARTESIAN_POINT('Ctrl Pts',(-28.3826963466553,28.4199999807123,
-81.0712589143804));
#143020=CARTESIAN_POINT('Ctrl Pts',(-28.4218307391328,28.4199999807278,
-81.0274582842905));
#143021=CARTESIAN_POINT('Ctrl Pts',(-28.460931835895,28.4199999807438,-80.9836287163303));
#143022=CARTESIAN_POINT('Ctrl Pts',(-28.5,28.4199999807603,-80.9397703408579));
#143023=CARTESIAN_POINT('',(-22.5,28.4199999800001,-87.5942752792638));
#143024=CARTESIAN_POINT('Ctrl Pts',(-28.5,29.41999998,-92.34995));
#143025=CARTESIAN_POINT('Ctrl Pts',(-28.5,28.41999998,-92.34995));
#143026=CARTESIAN_POINT('Ctrl Pts',(-28.5,28.41999998,-91.34995));
#143027=CARTESIAN_POINT('Ctrl Pts',(-29.,29.41999998,-92.34995));
#143028=CARTESIAN_POINT('Ctrl Pts',(-29.,28.41999998,-92.34995));
#143029=CARTESIAN_POINT('Ctrl Pts',(-29.,28.41999998,-91.34995));
#143030=CARTESIAN_POINT('Ctrl Pts',(-29.,29.41999998,-91.84995));
#143031=CARTESIAN_POINT('Ctrl Pts',(-29.,28.91999998,-91.84995));
#143032=CARTESIAN_POINT('Ctrl Pts',(-29.,28.91999998,-91.34995));
#143033=CARTESIAN_POINT('Origin',(-28.5,28.91999998,-91.34995));
#143034=CARTESIAN_POINT('Origin',(-29.5,46.41999998,-92.34995));
#143035=CARTESIAN_POINT('',(-29.5,46.91999998,-58.24995));
#143036=CARTESIAN_POINT('',(-29.5,46.91999998,-58.24995));
#143037=CARTESIAN_POINT('Origin',(-29.5,46.41999998,-58.24995));
#143038=CARTESIAN_POINT('Origin',(39.,46.91999998,-129.34995));
#143039=CARTESIAN_POINT('',(-30.,46.91999998,-58.24995));
#143040=CARTESIAN_POINT('',(-30.,46.91999998,-92.34995));
#143041=CARTESIAN_POINT('',(39.,46.91999998,-58.24995));
#143042=CARTESIAN_POINT('Origin',(-30.,46.41999998,-92.34995));
#143043=CARTESIAN_POINT('Origin',(-30.,46.41999998,-58.24995));
#143044=CARTESIAN_POINT('Ctrl Pts',(-31.,28.41999998,-91.34995));
#143045=CARTESIAN_POINT('Ctrl Pts',(-31.,28.41999998,-92.34995));
#143046=CARTESIAN_POINT('Ctrl Pts',(-31.,29.41999998,-92.34995));
#143047=CARTESIAN_POINT('Ctrl Pts',(-30.5,28.41999998,-91.34995));
#143048=CARTESIAN_POINT('Ctrl Pts',(-30.5,28.41999998,-92.34995));
#143049=CARTESIAN_POINT('Ctrl Pts',(-30.5,29.41999998,-92.34995));
#143050=CARTESIAN_POINT('Ctrl Pts',(-30.5,28.91999998,-91.34995));
#143051=CARTESIAN_POINT('Ctrl Pts',(-30.5,28.91999998,-91.84995));
#143052=CARTESIAN_POINT('Ctrl Pts',(-30.5,29.41999998,-91.84995));
#143053=CARTESIAN_POINT('Origin',(-31.,28.91999998,-91.34995));
#143054=CARTESIAN_POINT('Origin',(-60.,28.41999998,-55.24995));
#143055=CARTESIAN_POINT('',(-37.,28.41999998,-70.4461836365688));
#143056=CARTESIAN_POINT('',(-37.,28.41999998,-91.34995));
#143057=CARTESIAN_POINT('',(-31.,28.41999998,-78.0460091084363));
#143058=CARTESIAN_POINT('Ctrl Pts',(-31.,28.41999998,-78.0460091084363));
#143059=CARTESIAN_POINT('Ctrl Pts',(-31.6054626504327,28.4199999800001,
-77.3245680023291));
#143060=CARTESIAN_POINT('Ctrl Pts',(-32.2037002325589,28.4199999800031,
-76.5972335154354));
#143061=CARTESIAN_POINT('Ctrl Pts',(-32.7954596657072,28.4199999800058,
-75.8646586780361));
#143062=CARTESIAN_POINT('Ctrl Pts',(-33.4345463106021,28.4199999800088,
-75.0734946192274));
#143063=CARTESIAN_POINT('Ctrl Pts',(-34.0660773010423,28.4199999800106,
-74.2762178948229));
#143064=CARTESIAN_POINT('Ctrl Pts',(-34.6909510193196,28.4199999800288,
-73.4736062556181));
#143065=CARTESIAN_POINT('Ctrl Pts',(-34.9391029883029,28.4199999800361,
-73.1548704010415));
#143066=CARTESIAN_POINT('Ctrl Pts',(-35.1862046047006,28.4199999800463,
-72.8352927773724));
#143067=CARTESIAN_POINT('Ctrl Pts',(-35.4323104279066,28.4199999800634,
-72.5149207187905));
#143068=CARTESIAN_POINT('Ctrl Pts',(-35.9594751118247,28.4199999801002,
-71.8286759449022));
#143069=CARTESIAN_POINT('Ctrl Pts',(-36.4818085017622,28.4199999801598,
-71.1391285306312));
#143070=CARTESIAN_POINT('Ctrl Pts',(-37.,28.4199999803545,-70.4461836365688));
#143071=CARTESIAN_POINT('',(-31.,28.41999998,-78.6384479219785));
#143072=CARTESIAN_POINT('Ctrl Pts',(-37.,29.41999998,-92.34995));
#143073=CARTESIAN_POINT('Ctrl Pts',(-37.,28.41999998,-92.34995));
#143074=CARTESIAN_POINT('Ctrl Pts',(-37.,28.41999998,-91.34995));
#143075=CARTESIAN_POINT('Ctrl Pts',(-37.5,29.41999998,-92.34995));
#143076=CARTESIAN_POINT('Ctrl Pts',(-37.5,28.41999998,-92.34995));
#143077=CARTESIAN_POINT('Ctrl Pts',(-37.5,28.41999998,-91.34995));
#143078=CARTESIAN_POINT('Ctrl Pts',(-37.5,29.41999998,-91.84995));
#143079=CARTESIAN_POINT('Ctrl Pts',(-37.5,28.91999998,-91.84995));
#143080=CARTESIAN_POINT('Ctrl Pts',(-37.5,28.91999998,-91.34995));
#143081=CARTESIAN_POINT('Origin',(-37.,28.91999998,-91.34995));
#143082=CARTESIAN_POINT('Origin',(-42.,28.91999998,-92.34995));
#143083=CARTESIAN_POINT('Origin',(-42.,28.91999998,-171.14995));
#143084=CARTESIAN_POINT('Origin',(-42.,58.91999998,-171.14995));
#143085=CARTESIAN_POINT('',(-42.,28.91999998,-171.64995));
#143086=CARTESIAN_POINT('Origin',(-42.,28.91999998,-171.14995));
#143087=CARTESIAN_POINT('Origin',(-42.,30.4123236926243,-171.14995));
#143088=CARTESIAN_POINT('',(-42.,28.91999998,-171.64995));
#143089=CARTESIAN_POINT('Ctrl Pts',(-42.0000617764046,30.4123236926243,
-171.649949996184));
#143090=CARTESIAN_POINT('Ctrl Pts',(-41.5,30.4123236926243,-171.650011780222));
#143091=CARTESIAN_POINT('Ctrl Pts',(-41.5,30.4123236926243,-171.14995));
#143092=CARTESIAN_POINT('Ctrl Pts',(-41.929864311704,30.5683704599569,-171.649958724212));
#143093=CARTESIAN_POINT('Ctrl Pts',(-41.5000000000006,30.5590517401679,
-171.583996757915));
#143094=CARTESIAN_POINT('Ctrl Pts',(-41.5,30.6002163674433,-171.149950044589));
#143095=CARTESIAN_POINT('Ctrl Pts',(-41.8681695534321,30.7453325953812,
-171.649964230513));
#143096=CARTESIAN_POINT('Ctrl Pts',(-41.5,30.7482244616852,-171.547558090571));
#143097=CARTESIAN_POINT('Ctrl Pts',(-41.5,30.7881194136978,-171.167360442076));
#143098=CARTESIAN_POINT('Ctrl Pts',(-41.782059127798,31.1278785851814,-171.649970496006));
#143099=CARTESIAN_POINT('Ctrl Pts',(-41.5,31.1331148272644,-171.511616746684));
#143100=CARTESIAN_POINT('Ctrl Pts',(-41.5,31.1638381213445,-171.199054581264));
#143101=CARTESIAN_POINT('Ctrl Pts',(-41.7580490411456,31.3335084853296,
-171.649971475853));
#143102=CARTESIAN_POINT('Ctrl Pts',(-41.5000000000007,31.3394417200798,
-171.507283264433));
#143103=CARTESIAN_POINT('Ctrl Pts',(-41.5,31.3517239082014,-171.212413163406));
#143104=CARTESIAN_POINT('Ctrl Pts',(-41.7579337455091,31.7458587360553,
-171.649971481651));
#143105=CARTESIAN_POINT('Ctrl Pts',(-41.4999999999994,31.739954085554,-171.507256427626));
#143106=CARTESIAN_POINT('Ctrl Pts',(-41.5,31.72777865723,-171.212471328128));
#143107=CARTESIAN_POINT('Ctrl Pts',(-41.7818539242555,31.9518486363857,
-171.649970508384));
#143108=CARTESIAN_POINT('Ctrl Pts',(-41.5000000000001,31.9466344699074,
-171.511552982749));
#143109=CARTESIAN_POINT('Ctrl Pts',(-41.5,31.9159478899749,-171.199145438258));
#143110=CARTESIAN_POINT('Ctrl Pts',(-41.8680165447745,32.3351574715402,
-171.649964244171));
#143111=CARTESIAN_POINT('Ctrl Pts',(-41.5,32.3322632068598,-171.547472271891));
#143112=CARTESIAN_POINT('Ctrl Pts',(-41.5,32.2923404450921,-171.167401493624));
#143113=CARTESIAN_POINT('Ctrl Pts',(-41.9298158029953,32.5124265790917,
-171.649958730482));
#143114=CARTESIAN_POINT('Ctrl Pts',(-41.5,32.5217552106974,-171.583952704406));
#143115=CARTESIAN_POINT('Ctrl Pts',(-41.5,32.4805522169437,-171.149950046396));
#143116=CARTESIAN_POINT('Ctrl Pts',(-42.0000617764046,32.6685811839606,
-171.649949996184));
#143117=CARTESIAN_POINT('Ctrl Pts',(-41.5,32.6685811839606,-171.650011780222));
#143118=CARTESIAN_POINT('Ctrl Pts',(-41.5,32.6685811839606,-171.14995));
#143119=CARTESIAN_POINT('Origin',(-42.,32.6685811839606,-171.14995));
#143120=CARTESIAN_POINT('Origin',(-42.,58.91999998,-171.14995));
#143121=CARTESIAN_POINT('',(-42.,36.3270340686007,-171.64995));
#143122=CARTESIAN_POINT('Origin',(-42.,36.3270340686007,-171.14995));
#143123=CARTESIAN_POINT('',(-42.,28.91999998,-171.64995));
#143124=CARTESIAN_POINT('Ctrl Pts',(-42.,36.3270340686007,-171.64995));
#143125=CARTESIAN_POINT('Ctrl Pts',(-41.5,36.3270340686007,-171.64995));
#143126=CARTESIAN_POINT('Ctrl Pts',(-41.5,36.3270340686007,-171.14995));
#143127=CARTESIAN_POINT('Ctrl Pts',(-41.9908895000013,36.460524412126,-171.64995));
#143128=CARTESIAN_POINT('Ctrl Pts',(-41.5,36.4592824973649,-171.640924254979));
#143129=CARTESIAN_POINT('Ctrl Pts',(-41.5,36.5253489879757,-171.149950000016));
#143130=CARTESIAN_POINT('Ctrl Pts',(-41.9817858670191,36.5939141376228,
-171.675977326981));
#143131=CARTESIAN_POINT('Ctrl Pts',(-41.5,36.5965520755147,-171.658003579003));
#143132=CARTESIAN_POINT('Ctrl Pts',(-41.5,36.7235144279567,-171.18899099047));
#143133=CARTESIAN_POINT('Ctrl Pts',(-41.9649548930127,36.840527660716,-171.776163607997));
#143134=CARTESIAN_POINT('Ctrl Pts',(-41.5,36.8549873364184,-171.746711574348));
#143135=CARTESIAN_POINT('Ctrl Pts',(-41.5,37.0898865538897,-171.339270411997));
#143136=CARTESIAN_POINT('Ctrl Pts',(-41.9572358131754,36.9536304124011,
-171.850283164392));
#143137=CARTESIAN_POINT('Ctrl Pts',(-41.4999999999986,36.9765510525756,
-171.817687494207));
#143138=CARTESIAN_POINT('Ctrl Pts',(-41.5,37.2579134125323,-171.450449746589));
#143139=CARTESIAN_POINT('Ctrl Pts',(-41.9443539433771,37.1423802312719,
-172.035403273234));
#143140=CARTESIAN_POINT('Ctrl Pts',(-41.5000000000014,37.1809962719461,
-172.003556970024));
#143141=CARTESIAN_POINT('Ctrl Pts',(-41.5,37.5383224977403,-171.728129909852));
#143142=CARTESIAN_POINT('Ctrl Pts',(-41.9391962191204,37.2179530739059,
-172.146331028561));
#143143=CARTESIAN_POINT('Ctrl Pts',(-41.5,37.2645653642152,-172.118296873734));
#143144=CARTESIAN_POINT('Ctrl Pts',(-41.5,37.6505944553831,-171.894521542842));
#143145=CARTESIAN_POINT('Ctrl Pts',(-41.9322246014265,37.3201037397322,
-172.388202106709));
#143146=CARTESIAN_POINT('Ctrl Pts',(-41.5,37.3773763733446,-172.371853931892));
#143147=CARTESIAN_POINT('Ctrl Pts',(-41.5,37.8023507586648,-172.257328160063));
#143148=CARTESIAN_POINT('Ctrl Pts',(-41.9304134495219,37.3466413930076,
-172.51902671195));
#143149=CARTESIAN_POINT('Ctrl Pts',(-41.5,37.4071320584576,-172.511015867074));
#143150=CARTESIAN_POINT('Ctrl Pts',(-41.5,37.8417754273637,-172.453565067926));
#143151=CARTESIAN_POINT('Ctrl Pts',(-41.93041344952,37.3466413930079,-172.64995));
#143152=CARTESIAN_POINT('Ctrl Pts',(-41.5,37.4071320584705,-172.64995));
#143153=CARTESIAN_POINT('Ctrl Pts',(-41.5,37.8417754273786,-172.64995));
#143154=CARTESIAN_POINT('',(-41.93041344952,37.3466413930079,-172.64995));
#143155=CARTESIAN_POINT('Origin',(-42.,37.8417754273786,-172.64995));
#143156=CARTESIAN_POINT('Ctrl Pts',(-41.93041344952,37.3466413930079,-172.64995));
#143157=CARTESIAN_POINT('Ctrl Pts',(-41.9304134495219,37.3466413930076,
-172.51902671195));
#143158=CARTESIAN_POINT('Ctrl Pts',(-41.9322246014265,37.3201037397322,
-172.388202106709));
#143159=CARTESIAN_POINT('Ctrl Pts',(-41.9391962191204,37.2179530739059,
-172.146331028561));
#143160=CARTESIAN_POINT('Ctrl Pts',(-41.9443539433771,37.1423802312719,
-172.035403273234));
#143161=CARTESIAN_POINT('Ctrl Pts',(-41.9572358131754,36.9536304124011,
-171.850283164392));
#143162=CARTESIAN_POINT('Ctrl Pts',(-41.9649548930127,36.840527660716,-171.776163607997));
#143163=CARTESIAN_POINT('Ctrl Pts',(-41.9817858670191,36.5939141376228,
-171.675977326981));
#143164=CARTESIAN_POINT('Ctrl Pts',(-41.9908895000013,36.460524412126,-171.64995));
#143165=CARTESIAN_POINT('Ctrl Pts',(-42.,36.3270340686007,-171.64995));
#143166=CARTESIAN_POINT('Origin',(-42.,37.8417754273786,-171.64995));
#143167=CARTESIAN_POINT('',(-41.93041344952,37.3466413930079,-174.34995));
#143168=CARTESIAN_POINT('Origin',(-42.,37.8417754273786,-174.34995));
#143169=CARTESIAN_POINT('',(-41.93041344952,37.3466413930079,-171.64995));
#143170=CARTESIAN_POINT('Ctrl Pts',(-41.93041344952,37.3466413930079,-174.34995));
#143171=CARTESIAN_POINT('Ctrl Pts',(-41.5,37.4071320584705,-174.34995));
#143172=CARTESIAN_POINT('Ctrl Pts',(-41.5,37.8417754273786,-174.34995));
#143173=CARTESIAN_POINT('Ctrl Pts',(-41.9304134495165,37.3466413930083,
-174.808181527339));
#143174=CARTESIAN_POINT('Ctrl Pts',(-41.4999999999921,37.4071320584705,
-174.750729116851));
#143175=CARTESIAN_POINT('Ctrl Pts',(-41.5,37.8417754273818,-174.742719880575));
#143176=CARTESIAN_POINT('Ctrl Pts',(-41.8393178154807,37.3594440494534,
-175.266067601));
#143177=CARTESIAN_POINT('Ctrl Pts',(-41.418170761701,37.4186324079233,-175.152286591264));
#143178=CARTESIAN_POINT('Ctrl Pts',(-41.4219180279654,37.8545780838243,
-175.135193658002));
#143179=CARTESIAN_POINT('Ctrl Pts',(-41.4886658111382,37.4087249748338,
-176.112616425556));
#143180=CARTESIAN_POINT('Ctrl Pts',(-41.1060831277358,37.4624934645027,
-175.889590467068));
#143181=CARTESIAN_POINT('Ctrl Pts',(-41.1213591671024,37.9038590092046,
-175.860806936189));
#143182=CARTESIAN_POINT('Ctrl Pts',(-41.2292473935486,37.445183855779,-176.500863524274));
#143183=CARTESIAN_POINT('Ctrl Pts',(-40.8743194488686,37.4950657253844,
-176.226515658809));
#143184=CARTESIAN_POINT('Ctrl Pts',(-40.8990005234543,37.9403178901501,
-176.193590163665));
#143185=CARTESIAN_POINT('Ctrl Pts',(-40.5813269737971,37.5362431323916,
-177.148783944032));
#143186=CARTESIAN_POINT('Ctrl Pts',(-40.3016108905592,37.5755546642088,
-176.782638117262));
#143187=CARTESIAN_POINT('Ctrl Pts',(-40.343640163665,38.0313771667621,-176.748950523454));
#143188=CARTESIAN_POINT('Ctrl Pts',(-40.193079875155,37.5908077037056,-177.408202361589));
#143189=CARTESIAN_POINT('Ctrl Pts',(-39.9585494594759,37.6237688040866,
-177.001555340038));
#143190=CARTESIAN_POINT('Ctrl Pts',(-40.0108569362568,38.0859417380754,
-176.971309167074));
#143191=CARTESIAN_POINT('Ctrl Pts',(-39.3465310504406,37.7097823821472,
-177.758854365991));
#143192=CARTESIAN_POINT('Ctrl Pts',(-39.218856185771,37.7277259142,-177.290648705564));
#143193=CARTESIAN_POINT('Ctrl Pts',(-39.2852436579338,38.204916416519,-177.271868027993));
#143194=CARTESIAN_POINT('Ctrl Pts',(-38.8886449769195,37.7741340731185,
-177.849949999987));
#143195=CARTESIAN_POINT('Ctrl Pts',(-38.8208550398785,37.7836613274466,
-177.358977353131));
#143196=CARTESIAN_POINT('Ctrl Pts',(-38.8927698806272,38.2692681074913,
-177.34995));
#143197=CARTESIAN_POINT('Ctrl Pts',(-38.43041344952,37.8385343144662,-177.84995));
#143198=CARTESIAN_POINT('Ctrl Pts',(-38.43041344952,37.8385343144661,-177.34995));
#143199=CARTESIAN_POINT('Ctrl Pts',(-38.5,38.333668348837,-177.34995));
#143200=CARTESIAN_POINT('Ctrl Pts',(-38.43041344952,37.8385343144662,-177.84995));
#143201=CARTESIAN_POINT('Ctrl Pts',(-38.8886449769195,37.7741340731185,
-177.849949999987));
#143202=CARTESIAN_POINT('Ctrl Pts',(-39.3465310504406,37.7097823821472,
-177.758854365991));
#143203=CARTESIAN_POINT('Ctrl Pts',(-39.7698054627978,37.6502950429264,
-177.58352836379));
#143204=CARTESIAN_POINT('Ctrl Pts',(-40.193079875155,37.5908077037056,-177.408202361589));
#143205=CARTESIAN_POINT('Ctrl Pts',(-40.5813269737971,37.5362431323916,
-177.148783944032));
#143206=CARTESIAN_POINT('Ctrl Pts',(-40.9052871836729,37.4907134940853,
-176.824823734153));
#143207=CARTESIAN_POINT('Ctrl Pts',(-41.2292473935486,37.445183855779,-176.500863524274));
#143208=CARTESIAN_POINT('Ctrl Pts',(-41.4886658111382,37.4087249748338,
-176.112616425556));
#143209=CARTESIAN_POINT('Ctrl Pts',(-41.6639918133095,37.3840845121436,
-175.689342013278));
#143210=CARTESIAN_POINT('Ctrl Pts',(-41.8393178154807,37.3594440494534,
-175.266067601));
#143211=CARTESIAN_POINT('Ctrl Pts',(-41.9304134495165,37.3466413930083,
-174.808181527339));
#143212=CARTESIAN_POINT('Ctrl Pts',(-41.93041344952,37.3466413930079,-174.34995));
#143213=CARTESIAN_POINT('Origin',(-45.5612236321975,36.8363642992885,-171.64995));
#143214=CARTESIAN_POINT('',(-44.628608857647,36.9674347581595,-172.64995));
#143215=CARTESIAN_POINT('',(-44.628608857647,36.9674347581595,-171.64995));
#143216=CARTESIAN_POINT('',(-44.628608857647,36.9674347581595,-172.64995));
#143217=CARTESIAN_POINT('Origin',(-44.2110895547669,33.9966305519348,-171.64995));
#143218=CARTESIAN_POINT('',(-46.2674193015002,36.1810087180727,-172.64995));
#143219=CARTESIAN_POINT('',(-46.2674193015002,36.1810087180727,-171.64995));
#143220=CARTESIAN_POINT('Origin',(-44.2110895547669,33.9966305519348,-172.64995));
#143221=CARTESIAN_POINT('Origin',(0.,-12.9675000200281,-171.64995));
#143222=CARTESIAN_POINT('',(-49.1485087381009,33.2999192814719,-172.64995));
#143223=CARTESIAN_POINT('',(-49.1485087381009,33.2999192814719,-171.64995));
#143224=CARTESIAN_POINT('Origin',(0.,-12.9675000200281,-172.64995));
#143225=CARTESIAN_POINT('Origin',(-46.9641305719631,31.2435895347386,-171.64995));
#143226=CARTESIAN_POINT('',(-49.9349347781878,31.6611088376188,-172.64995));
#143227=CARTESIAN_POINT('',(-49.9349347781878,31.6611088376188,-171.64995));
#143228=CARTESIAN_POINT('Origin',(-46.9641305719631,31.2435895347386,-172.64995));
#143229=CARTESIAN_POINT('Origin',(-52.6124803109502,12.6093824234965,-171.64995));
#143230=CARTESIAN_POINT('',(-50.3299522569362,28.85041342952,-172.64995));
#143231=CARTESIAN_POINT('',(-50.3904429223989,28.41999998,-172.64995));
#143232=CARTESIAN_POINT('',(-52.5050296388285,13.3739336825608,-172.133326251627));
#143233=CARTESIAN_POINT('',(-52.5050296388285,13.3739336825608,-171.64995));
#143234=CARTESIAN_POINT('',(-51.9770573602378,17.1306516479033,-172.64995));
#143235=CARTESIAN_POINT('Ctrl Pts',(-51.9770573602378,17.1306516479033,
-172.64995));
#143236=CARTESIAN_POINT('Ctrl Pts',(-52.0505828082768,16.6074909011023,
-172.64994999816));
#143237=CARTESIAN_POINT('Ctrl Pts',(-52.1235483667,16.0883139759212,-172.620408747532));
#143238=CARTESIAN_POINT('Ctrl Pts',(-52.1959928599554,15.5728446220577,
-172.563374785654));
#143239=CARTESIAN_POINT('Ctrl Pts',(-52.2118579788214,15.4599584356367,
-172.550884525264));
#143240=CARTESIAN_POINT('Ctrl Pts',(-52.2276981039084,15.3472500891943,
-172.537075526609));
#143241=CARTESIAN_POINT('Ctrl Pts',(-52.2435136369168,15.2347167244825,
-172.521968983896));
#143242=CARTESIAN_POINT('Ctrl Pts',(-52.2955483171873,14.8644707359723,
-172.472266952379));
#143243=CARTESIAN_POINT('Ctrl Pts',(-52.347327733492,14.4960410449546,-172.409096799907));
#143244=CARTESIAN_POINT('Ctrl Pts',(-52.3987708154505,14.1300044971607,
-172.328180486668));
#143245=CARTESIAN_POINT('Ctrl Pts',(-52.4343604559392,13.8767710467971,
-172.272200510581));
#143246=CARTESIAN_POINT('Ctrl Pts',(-52.4697891103107,13.6246830721773,
-172.207726272012));
#143247=CARTESIAN_POINT('Ctrl Pts',(-52.5050296388285,13.3739336825608,
-172.133326251627));
#143248=CARTESIAN_POINT('',(-51.8267121465167,18.20041342952,-172.64995));
#143249=CARTESIAN_POINT('',(-52.3378926620474,14.5631750666398,-172.64995));
#143250=CARTESIAN_POINT('',(-51.8267121465167,18.20041342952,-176.84995));
#143251=CARTESIAN_POINT('',(-51.8267121465167,18.20041342952,-171.64995));
#143252=CARTESIAN_POINT('',(-51.6861713118143,19.20041342952,-177.84995));
#143253=CARTESIAN_POINT('Ctrl Pts',(-51.6861713118143,19.20041342952,-177.84995));
#143254=CARTESIAN_POINT('Ctrl Pts',(-51.7230681564996,18.9378787379949,
-177.849949999941));
#143255=CARTESIAN_POINT('Ctrl Pts',(-51.7595317568342,18.6784267402051,
-177.742176873059));
#143256=CARTESIAN_POINT('Ctrl Pts',(-51.7855486890661,18.4933066483335,
-177.557056781187));
#143257=CARTESIAN_POINT('Ctrl Pts',(-51.8115656212979,18.3081865564618,
-177.371936689315));
#143258=CARTESIAN_POINT('Ctrl Pts',(-51.8267121465076,18.2004134295853,
-177.112484691526));
#143259=CARTESIAN_POINT('Ctrl Pts',(-51.8267121465167,18.20041342952,-176.84995));
#143260=CARTESIAN_POINT('',(-51.6159008944631,19.70041342952,-177.84995));
#143261=CARTESIAN_POINT('',(-52.6124803109502,12.6093824234965,-177.84995));
#143262=CARTESIAN_POINT('',(-51.4753600597607,20.70041342952,-176.84995));
#143263=CARTESIAN_POINT('Ctrl Pts',(-51.4753600597607,20.70041342952,-176.84995));
#143264=CARTESIAN_POINT('Ctrl Pts',(-51.4753600597699,20.7004134294547,
-177.112484691526));
#143265=CARTESIAN_POINT('Ctrl Pts',(-51.4905065849796,20.5926403025782,
-177.371936689315));
#143266=CARTESIAN_POINT('Ctrl Pts',(-51.5165235172115,20.4075202107065,
-177.557056781187));
#143267=CARTESIAN_POINT('Ctrl Pts',(-51.5425404494433,20.2224001188348,
-177.742176873059));
#143268=CARTESIAN_POINT('Ctrl Pts',(-51.5790040497779,19.9629481210451,
-177.849949999941));
#143269=CARTESIAN_POINT('Ctrl Pts',(-51.6159008944631,19.70041342952,-177.84995));
#143270=CARTESIAN_POINT('',(-51.4753600597607,20.70041342952,-172.64995));
#143271=CARTESIAN_POINT('',(-51.4753600597607,20.70041342952,-171.64995));
#143272=CARTESIAN_POINT('',(-50.6813043436922,26.35041342952,-172.64995));
#143273=CARTESIAN_POINT('',(-51.5358507252234,20.26999998,-172.64995));
#143274=CARTESIAN_POINT('',(-50.6813043436922,26.35041342952,-176.84995));
#143275=CARTESIAN_POINT('',(-50.6813043436922,26.35041342952,-171.64995));
#143276=CARTESIAN_POINT('',(-50.5407635089898,27.3504134295199,-177.84995));
#143277=CARTESIAN_POINT('Ctrl Pts',(-50.5407635089898,27.3504134295199,
-177.84995));
#143278=CARTESIAN_POINT('Ctrl Pts',(-50.5776603536751,27.0878787379949,
-177.849949999941));
#143279=CARTESIAN_POINT('Ctrl Pts',(-50.6141239540097,26.8284267402052,
-177.742176873059));
#143280=CARTESIAN_POINT('Ctrl Pts',(-50.6401408862415,26.6433066483335,
-177.557056781187));
#143281=CARTESIAN_POINT('Ctrl Pts',(-50.6661578184733,26.4581865564618,
-177.371936689315));
#143282=CARTESIAN_POINT('Ctrl Pts',(-50.681304343683,26.3504134295853,-177.112484691526));
#143283=CARTESIAN_POINT('Ctrl Pts',(-50.6813043436922,26.35041342952,-176.84995));
#143284=CARTESIAN_POINT('',(-50.4704930916386,27.85041342952,-177.84995));
#143285=CARTESIAN_POINT('',(-52.6124803109502,12.6093824234965,-177.84995));
#143286=CARTESIAN_POINT('',(-50.3299522569362,28.85041342952,-176.84995));
#143287=CARTESIAN_POINT('Ctrl Pts',(-50.3299522569362,28.85041342952,-176.84995));
#143288=CARTESIAN_POINT('Ctrl Pts',(-50.3299522569454,28.8504134294547,
-177.112484691526));
#143289=CARTESIAN_POINT('Ctrl Pts',(-50.3450987821552,28.7426403025778,
-177.371936689315));
#143290=CARTESIAN_POINT('Ctrl Pts',(-50.3711157143869,28.5575202107065,
-177.557056781187));
#143291=CARTESIAN_POINT('Ctrl Pts',(-50.3971326466187,28.3724001188352,
-177.742176873059));
#143292=CARTESIAN_POINT('Ctrl Pts',(-50.4335962469534,28.1129481210447,
-177.849949999941));
#143293=CARTESIAN_POINT('Ctrl Pts',(-50.4704930916386,27.85041342952,-177.84995));
#143294=CARTESIAN_POINT('',(-50.3299522569362,28.85041342952,-171.64995));
#143295=CARTESIAN_POINT('Origin',(-57.4563699825364,14.0697991873612,-179.64995));
#143296=CARTESIAN_POINT('',(-52.7229737572976,12.4589111791821,-171.855631767295));
#143297=CARTESIAN_POINT('',(-52.7229737572976,12.4589111791821,-176.84995));
#143298=CARTESIAN_POINT('',(-52.7229737572976,12.4589111791821,-179.64995));
#143299=CARTESIAN_POINT('Ctrl Pts',(-52.5050296388285,13.3739336825608,
-172.133326251627));
#143300=CARTESIAN_POINT('Ctrl Pts',(-52.5484527228769,13.0649623850707,
-172.023316132141));
#143301=CARTESIAN_POINT('Ctrl Pts',(-52.6198951421523,12.7615490364788,
-171.918010656511));
#143302=CARTESIAN_POINT('Ctrl Pts',(-52.7229737572976,12.4589111791821,
-171.855638188259));
#143303=CARTESIAN_POINT('',(-52.9322463618642,11.9408779899289,-177.695579616717));
#143304=CARTESIAN_POINT('',(-52.9322463618642,11.9408779899289,-179.64995));
#143305=CARTESIAN_POINT('Ctrl Pts',(-52.7229737572976,12.4589111791821,
-176.84995));
#143306=CARTESIAN_POINT('Ctrl Pts',(-52.7229737689762,12.4589111448658,
-177.021627393075));
#143307=CARTESIAN_POINT('Ctrl Pts',(-52.7396382131267,12.4078638336875,
-177.193608615338));
#143308=CARTESIAN_POINT('Ctrl Pts',(-52.8083222549725,12.2244699412272,
-177.486975267512));
#143309=CARTESIAN_POINT('Ctrl Pts',(-52.8614762873877,12.0912699189313,
-177.610143591528));
#143310=CARTESIAN_POINT('Ctrl Pts',(-52.9322463618642,11.9408779899289,
-177.695579616717));
#143311=CARTESIAN_POINT('Origin',(0.,-12.9675000200281,-179.64995));
#143312=CARTESIAN_POINT('',(-52.9322463618642,-37.8758780299853,-177.801086692062));
#143313=CARTESIAN_POINT('',(-52.9322463618642,-37.8758780299853,-179.64995));
#143314=CARTESIAN_POINT('',(-53.0752347700893,-37.5697245962714,-177.84995));
#143315=CARTESIAN_POINT('Origin',(-53.46537255433,-36.3098838506748,-168.829790838513));
#143316=CARTESIAN_POINT('',(-53.3022372549338,-37.073961884407,-177.84995));
#143317=CARTESIAN_POINT('Origin',(0.,-12.9675000200281,-177.84995));
#143318=CARTESIAN_POINT('',(-53.7396474992599,-36.0824364606782,-176.84995));
#143319=CARTESIAN_POINT('Ctrl Pts',(-53.7396474992599,-36.0824364606782,
-176.84995));
#143320=CARTESIAN_POINT('Ctrl Pts',(-53.7396474962954,-36.0824364675704,
-176.886929243848));
#143321=CARTESIAN_POINT('Ctrl Pts',(-53.7387474700292,-36.084532659728,
-176.923734373979));
#143322=CARTESIAN_POINT('Ctrl Pts',(-53.7370043459075,-36.0885863209691,
-176.960178957691));
#143323=CARTESIAN_POINT('Ctrl Pts',(-53.7352184275947,-36.0927395007421,
-176.997518266259));
#143324=CARTESIAN_POINT('Ctrl Pts',(-53.7325474396826,-36.0989476220765,
-177.034480202452));
#143325=CARTESIAN_POINT('Ctrl Pts',(-53.7290307937802,-36.1071124473775,
-177.070872685112));
#143326=CARTESIAN_POINT('Ctrl Pts',(-53.7254987744608,-36.1153129661398,
-177.107424261644));
#143327=CARTESIAN_POINT('Ctrl Pts',(-53.7211135624651,-36.1254876499985,
-177.143402563608));
#143328=CARTESIAN_POINT('Ctrl Pts',(-53.7158949175065,-36.1375837241684,
-177.178604159826));
#143329=CARTESIAN_POINT('Ctrl Pts',(-53.7124883567771,-36.145479645729,
-177.201582610407));
#143330=CARTESIAN_POINT('Ctrl Pts',(-53.7087262603452,-36.1541952209921,
-177.224229886336));
#143331=CARTESIAN_POINT('Ctrl Pts',(-53.7046098856868,-36.1637255131277,
-177.246483747673));
#143332=CARTESIAN_POINT('Ctrl Pts',(-53.7045192628111,-36.1639353245641,
-177.246973671229));
#143333=CARTESIAN_POINT('Ctrl Pts',(-53.7044284725267,-36.1641455209115,
-177.247463380496));
#143334=CARTESIAN_POINT('Ctrl Pts',(-53.7043375149313,-36.1643561019227,
-177.247952874551));
#143335=CARTESIAN_POINT('Ctrl Pts',(-53.6892733519036,-36.1992319874256,
-177.329021620969));
#143336=CARTESIAN_POINT('Ctrl Pts',(-53.6695548792039,-36.2447904442786,
-177.404845363428));
#143337=CARTESIAN_POINT('Ctrl Pts',(-53.6462229783026,-36.2984391069735,
-177.472877385954));
#143338=CARTESIAN_POINT('Ctrl Pts',(-53.63420658674,-36.3260692319461,-177.507915226417));
#143339=CARTESIAN_POINT('Ctrl Pts',(-53.621231984313,-36.3558446669857,
-177.540885760614));
#143340=CARTESIAN_POINT('Ctrl Pts',(-53.6074429005481,-36.3874074842064,
-177.571437587764));
#143341=CARTESIAN_POINT('Ctrl Pts',(-53.6072249340652,-36.3879064032337,
-177.571920525892));
#143342=CARTESIAN_POINT('Ctrl Pts',(-53.6070067635404,-36.3884057700779,
-177.572402861668));
#143343=CARTESIAN_POINT('Ctrl Pts',(-53.6067883895477,-36.3889055833105,
-177.572884593669));
#143344=CARTESIAN_POINT('Ctrl Pts',(-53.5821747509554,-36.4452411483472,
-177.627182164609));
#143345=CARTESIAN_POINT('Ctrl Pts',(-53.5548118941679,-36.5076136010266,
-177.674313675415));
#143346=CARTESIAN_POINT('Ctrl Pts',(-53.525557578149,-36.573947440761,-177.713411209491));
#143347=CARTESIAN_POINT('Ctrl Pts',(-53.5065780536932,-36.6169833036631,
-177.738776786443));
#143348=CARTESIAN_POINT('Ctrl Pts',(-53.4868028977425,-36.6616853915001,
-177.760761117544));
#143349=CARTESIAN_POINT('Ctrl Pts',(-53.4664703600909,-36.7074778455205,
-177.779132991661));
#143350=CARTESIAN_POINT('Ctrl Pts',(-53.4662816165212,-36.7079029292647,
-177.779303534716));
#143351=CARTESIAN_POINT('Ctrl Pts',(-53.4660928305315,-36.7083280943329,
-177.779473761639));
#143352=CARTESIAN_POINT('Ctrl Pts',(-53.4659040022552,-36.7087533403953,
-177.77964367236));
#143353=CARTESIAN_POINT('Ctrl Pts',(-53.449183813925,-36.7464076281519,
-177.794688766856));
#143354=CARTESIAN_POINT('Ctrl Pts',(-53.4320805422693,-36.7848119006861,
-177.807311664152));
#143355=CARTESIAN_POINT('Ctrl Pts',(-53.414687406387,-36.8237527438975,
-177.817537516946));
#143356=CARTESIAN_POINT('Ctrl Pts',(-53.3964494296165,-36.8645850698633,
-177.828260072498));
#143357=CARTESIAN_POINT('Ctrl Pts',(-53.3778922436238,-36.9060085268256,
-177.836347616446));
#143358=CARTESIAN_POINT('Ctrl Pts',(-53.3591168326372,-36.9477888085125,
-177.841770056554));
#143359=CARTESIAN_POINT('Ctrl Pts',(-53.3414627191038,-36.9870739052215,
-177.846868659901));
#143360=CARTESIAN_POINT('Ctrl Pts',(-53.32361520173,-37.0266755174969,-177.84961057998));
#143361=CARTESIAN_POINT('Ctrl Pts',(-53.3056598276501,-37.0663926738602,
-177.849920463284));
#143362=CARTESIAN_POINT('Ctrl Pts',(-53.3045193956941,-37.0689153010198,
-177.84994014546));
#143363=CARTESIAN_POINT('Ctrl Pts',(-53.3033785305218,-37.0714383891504,
-177.84994999975));
#143364=CARTESIAN_POINT('Ctrl Pts',(-53.3022372549337,-37.073961884407,
-177.84995));
#143365=CARTESIAN_POINT('',(-53.7396474992599,-36.0824364606782,-171.871644662643));
#143366=CARTESIAN_POINT('',(-53.7396474992599,-36.0824364606782,-179.64995));
#143367=CARTESIAN_POINT('',(-55.8171229357418,-30.4803178166104,-171.871644662643));
#143368=CARTESIAN_POINT('Origin',(0.,-12.9675000200281,-171.871644662643));
#143369=CARTESIAN_POINT('',(-55.8171229357418,-30.4803178166104,-176.84995));
#143370=CARTESIAN_POINT('',(-55.8171229357418,-30.4803178166104,-179.64995));
#143371=CARTESIAN_POINT('',(-56.1185967245324,-29.4887923928816,-177.84995));
#143372=CARTESIAN_POINT('Ctrl Pts',(-56.1185967245324,-29.4887923928816,
-177.84995));
#143373=CARTESIAN_POINT('Ctrl Pts',(-56.0810569766533,-29.6163052971279,
-177.849949980253));
#143374=CARTESIAN_POINT('Ctrl Pts',(-56.04332441336,-29.7428150883777,-177.825190994024));
#143375=CARTESIAN_POINT('Ctrl Pts',(-55.9716327345056,-29.9804872937887,
-177.727911302019));
#143376=CARTESIAN_POINT('Ctrl Pts',(-55.9382985315747,-30.0895950523083,
-177.656111307255));
#143377=CARTESIAN_POINT('Ctrl Pts',(-55.8527945813582,-30.367294876883,
-177.382125514336));
#143378=CARTESIAN_POINT('Ctrl Pts',(-55.8171229439391,-30.4803177904842,
-177.121808892945));
#143379=CARTESIAN_POINT('Ctrl Pts',(-55.8171229357418,-30.4803178166104,
-176.84995));
#143380=CARTESIAN_POINT('',(-56.262175563026,-28.9930296810172,-177.84995));
#143381=CARTESIAN_POINT('Origin',(0.,-12.9675000200281,-177.84995));
#143382=CARTESIAN_POINT('',(-56.5169491525423,-28.0699653316567,-177.215087021068));
#143383=CARTESIAN_POINT('Ctrl Pts',(-56.5169491525423,-28.0699653316567,
-177.215087021068));
#143384=CARTESIAN_POINT('Ctrl Pts',(-56.4972682976465,-28.1436156829388,
-177.404470992826));
#143385=CARTESIAN_POINT('Ctrl Pts',(-56.4617523202342,-28.2759697513382,
-177.568612620023));
#143386=CARTESIAN_POINT('Ctrl Pts',(-56.3721096851181,-28.6028436438479,
-177.790491903933));
#143387=CARTESIAN_POINT('Ctrl Pts',(-56.3176963010821,-28.7981083537361,
-177.849949971516));
#143388=CARTESIAN_POINT('Ctrl Pts',(-56.262175563026,-28.9930296810172,
-177.84995));
#143389=CARTESIAN_POINT('',(-56.5351989170821,-28.0015042572884,-176.849882244789));
#143390=CARTESIAN_POINT('Origin',(-55.1126545812022,-33.3251112519863,-176.014041861122));
#143391=CARTESIAN_POINT('',(-56.5351989170821,-28.0015042572884,-171.871644662643));
#143392=CARTESIAN_POINT('',(-56.5351989170821,-28.0015042572884,-179.64995));
#143393=CARTESIAN_POINT('',(-57.7346476057222,-22.3993856132206,-171.871644662643));
#143394=CARTESIAN_POINT('Origin',(0.,-12.9675000200281,-171.871644662643));
#143395=CARTESIAN_POINT('',(-57.7346476057222,-22.3993856132206,-176.657965001855));
#143396=CARTESIAN_POINT('',(-57.7346476057223,-22.3993856132206,-179.64995));
#143397=CARTESIAN_POINT('',(-57.8819282087167,-21.4487963148736,-177.697497252237));
#143398=CARTESIAN_POINT('Ctrl Pts',(-57.8819282087167,-21.4487963148736,
-177.697497252237));
#143399=CARTESIAN_POINT('Ctrl Pts',(-57.8765896421257,-21.4852301944858,
-177.698151252249));
#143400=CARTESIAN_POINT('Ctrl Pts',(-57.8712308062151,-21.5215461998529,
-177.696528688191));
#143401=CARTESIAN_POINT('Ctrl Pts',(-57.8658871784514,-21.5575327106499,
-177.692745867402));
#143402=CARTESIAN_POINT('Ctrl Pts',(-57.8604287549616,-21.5942923100333,
-177.688881781285));
#143403=CARTESIAN_POINT('Ctrl Pts',(-57.8549860188209,-21.630709268616,
-177.682763561799));
#143404=CARTESIAN_POINT('Ctrl Pts',(-57.849594035819,-21.6665701891049,
-177.674461317079));
#143405=CARTESIAN_POINT('Ctrl Pts',(-57.8442188129476,-21.7023196415672,
-177.66618487858));
#143406=CARTESIAN_POINT('Ctrl Pts',(-57.8388938392211,-21.7375177024571,
-177.655737740554));
#143407=CARTESIAN_POINT('Ctrl Pts',(-57.8336539589831,-21.7719470718028,
-177.643138949619));
#143408=CARTESIAN_POINT('Ctrl Pts',(-57.8307658910941,-21.7909235276623,
-177.63619486657));
#143409=CARTESIAN_POINT('Ctrl Pts',(-57.8279036918339,-21.8096662565538,
-177.62859626689));
#143410=CARTESIAN_POINT('Ctrl Pts',(-57.8250735265724,-21.8281360946975,
-177.620340114691));
#143411=CARTESIAN_POINT('Ctrl Pts',(-57.825000507433,-21.8286126222366,
-177.62012710341));
#143412=CARTESIAN_POINT('Ctrl Pts',(-57.8249275065196,-21.8290889901148,
-177.619913645942));
#143413=CARTESIAN_POINT('Ctrl Pts',(-57.8248545239147,-21.8295651979082,
-177.619699742645));
#143414=CARTESIAN_POINT('Ctrl Pts',(-57.8134041423527,-21.9042783566095,
-177.586140042007));
#143415=CARTESIAN_POINT('Ctrl Pts',(-57.8024908179666,-21.9744875656957,
-177.5418492558));
#143416=CARTESIAN_POINT('Ctrl Pts',(-57.7925715206908,-22.0376966071899,
-177.489169880456));
#143417=CARTESIAN_POINT('Ctrl Pts',(-57.7867917707696,-22.074527084434,
-177.458474801256));
#143418=CARTESIAN_POINT('Ctrl Pts',(-57.7813493744914,-22.1089817246166,
-177.424931754286));
#143419=CARTESIAN_POINT('Ctrl Pts',(-57.776333363324,-22.1405749184086,
-177.389003065334));
#143420=CARTESIAN_POINT('Ctrl Pts',(-57.7762581999322,-22.1410483327462,
-177.388464684929));
#143421=CARTESIAN_POINT('Ctrl Pts',(-57.7761831269835,-22.141521141353,
-177.387925738145));
#143422=CARTESIAN_POINT('Ctrl Pts',(-57.7761081445995,-22.1419933437069,
-177.387386226876));
#143423=CARTESIAN_POINT('Ctrl Pts',(-57.7675362470183,-22.1959749590623,
-177.325709935863));
#143424=CARTESIAN_POINT('Ctrl Pts',(-57.7601479409379,-22.2420339156224,
-177.256653403117));
#143425=CARTESIAN_POINT('Ctrl Pts',(-57.7541200519868,-22.2794160573285,
-177.182965839539));
#143426=CARTESIAN_POINT('Ctrl Pts',(-57.7505729125353,-22.3014137534883,
-177.139604048044));
#143427=CARTESIAN_POINT('Ctrl Pts',(-57.7474968850876,-22.3204065587794,
-177.094637483863));
#143428=CARTESIAN_POINT('Ctrl Pts',(-57.7449284196372,-22.3362374915981,
-177.048618868861));
#143429=CARTESIAN_POINT('Ctrl Pts',(-57.7449026192307,-22.3363965143727,
-177.048156608808));
#143430=CARTESIAN_POINT('Ctrl Pts',(-57.7448768691533,-22.3365552239542,
-177.047694236815));
#143431=CARTESIAN_POINT('Ctrl Pts',(-57.7448511693847,-22.3367136204909,
-177.04723175335));
#143432=CARTESIAN_POINT('Ctrl Pts',(-57.7426315058001,-22.3503941726404,
-177.007287514071));
#143433=CARTESIAN_POINT('Ctrl Pts',(-57.740792620676,-22.3617057222206,
-176.966623027288));
#143434=CARTESIAN_POINT('Ctrl Pts',(-57.7393137106679,-22.3707907309251,
-176.925440939058));
#143435=CARTESIAN_POINT('Ctrl Pts',(-57.7377438892451,-22.3804342124164,
-176.881727309435));
#143436=CARTESIAN_POINT('Ctrl Pts',(-57.7365796223128,-22.3875691725098,
-176.837429305389));
#143437=CARTESIAN_POINT('Ctrl Pts',(-57.7358055387825,-22.3923071177908,
-176.792774052489));
#143438=CARTESIAN_POINT('Ctrl Pts',(-57.7350314552522,-22.3970450630717,
-176.748118799589));
#143439=CARTESIAN_POINT('Ctrl Pts',(-57.7346476057222,-22.3993856132206,
-176.703104836952));
#143440=CARTESIAN_POINT('Ctrl Pts',(-57.7346476057222,-22.3993856132206,
-176.657965001855));
#143441=CARTESIAN_POINT('',(-57.9523179894071,-20.9536655363849,-177.688917160843));
#143442=CARTESIAN_POINT('Origin',(-1.12335876835565,-12.9875583193149,-185.751570786959));
#143443=CARTESIAN_POINT('',(-58.0853233553176,-19.9205720538986,-176.438901946458));
#143444=CARTESIAN_POINT('Ctrl Pts',(-58.0853233553176,-19.9205720538986,
-176.438901946458));
#143445=CARTESIAN_POINT('Ctrl Pts',(-58.0853233563387,-19.9205720453688,
-176.739635437133));
#143446=CARTESIAN_POINT('Ctrl Pts',(-58.0755566427899,-20.0041330036795,
-177.044575565272));
#143447=CARTESIAN_POINT('Ctrl Pts',(-58.0411746905458,-20.2805473548039,
-177.404658872083));
#143448=CARTESIAN_POINT('Ctrl Pts',(-58.0268899075637,-20.3936565135702,
-177.503861519498));
#143449=CARTESIAN_POINT('Ctrl Pts',(-57.9924606110737,-20.6579008473032,
-177.646467205152));
#143450=CARTESIAN_POINT('Ctrl Pts',(-57.9732407850675,-20.8018374150098,
-177.686379114698));
#143451=CARTESIAN_POINT('Ctrl Pts',(-57.9523179894071,-20.9536655363849,
-177.688917160843));
#143452=CARTESIAN_POINT('',(-58.0853233553176,-19.9205720538986,-171.871644662643));
#143453=CARTESIAN_POINT('',(-58.0853233553177,-19.9205720538986,-179.64995));
#143454=CARTESIAN_POINT('',(-58.4843989875811,-14.3184534098307,-171.871644662643));
#143455=CARTESIAN_POINT('Origin',(0.,-12.9675000200281,-171.871644662643));
#143456=CARTESIAN_POINT('',(-58.4843989875811,-14.3184534098307,-176.2719717603));
#143457=CARTESIAN_POINT('',(-58.4843989875811,-14.3184534098307,-179.64995));
#143458=CARTESIAN_POINT('',(-58.4988777713114,-13.3298527448197,-177.624285947696));
#143459=CARTESIAN_POINT('Ctrl Pts',(-58.4988777713114,-13.3298527448197,
-177.624285947696));
#143460=CARTESIAN_POINT('Ctrl Pts',(-58.4979165468949,-13.4850345491919,
-177.624397973596));
#143461=CARTESIAN_POINT('Ctrl Pts',(-58.4962883484962,-13.6395668470119,
-177.578389493351));
#143462=CARTESIAN_POINT('Ctrl Pts',(-58.4926597506031,-13.9035447147552,
-177.415964369801));
#143463=CARTESIAN_POINT('Ctrl Pts',(-58.4906864354198,-14.0146226773921,
-177.299459860577));
#143464=CARTESIAN_POINT('Ctrl Pts',(-58.4858850316409,-14.2631520760781,
-176.90254004861));
#143465=CARTESIAN_POINT('Ctrl Pts',(-58.4843989865928,-14.3184534526179,
-176.580946374937));
#143466=CARTESIAN_POINT('Ctrl Pts',(-58.4843989875811,-14.3184534098307,
-176.2719717603));
#143467=CARTESIAN_POINT('',(-58.4998385375645,-12.8300551987823,-177.624173936067));
#143468=CARTESIAN_POINT('Origin',(-0.784469541075961,-12.9675000162872,
-184.352939511374));
#143469=CARTESIAN_POINT('',(-58.48912660861,-11.8396398505087,-176.26629097911));
#143470=CARTESIAN_POINT('Ctrl Pts',(-58.48912660861,-11.8396398505087,-176.26629097911));
#143471=CARTESIAN_POINT('Ctrl Pts',(-58.48912660861,-11.8396398505087,-176.409811534267));
#143472=CARTESIAN_POINT('Ctrl Pts',(-58.4893483896326,-11.8507761032368,
-176.551488494009));
#143473=CARTESIAN_POINT('Ctrl Pts',(-58.4898674690037,-11.8787272918338,
-176.69038150372));
#143474=CARTESIAN_POINT('Ctrl Pts',(-58.4899146582257,-11.8812683191139,
-176.703008191328));
#143475=CARTESIAN_POINT('Ctrl Pts',(-58.4899643050979,-11.8839483504645,
-176.715611866643));
#143476=CARTESIAN_POINT('Ctrl Pts',(-58.4900164667572,-11.8867716762097,
-176.728191820333));
#143477=CARTESIAN_POINT('Ctrl Pts',(-58.4900183886416,-11.8868757010012,
-176.72865532585));
#143478=CARTESIAN_POINT('Ctrl Pts',(-58.4900203139396,-11.886979920305,
-176.72911879896));
#143479=CARTESIAN_POINT('Ctrl Pts',(-58.4900222426542,-11.8870843343361,
-176.729582239632));
#143480=CARTESIAN_POINT('Ctrl Pts',(-58.4904143757935,-11.9083130858161,
-176.82380584864));
#143481=CARTESIAN_POINT('Ctrl Pts',(-58.4909611779826,-11.9381550632,-176.917576442102));
#143482=CARTESIAN_POINT('Ctrl Pts',(-58.491628008076,-11.977637278452,-177.007000513354));
#143483=CARTESIAN_POINT('Ctrl Pts',(-58.4920261001825,-12.0012078377274,
-177.060385951801));
#143484=CARTESIAN_POINT('Ctrl Pts',(-58.4924669768134,-12.0282147910085,
-177.11222193254));
#143485=CARTESIAN_POINT('Ctrl Pts',(-58.4929432955759,-12.0588830464209,
-177.16167335862));
#143486=CARTESIAN_POINT('Ctrl Pts',(-58.4929498715258,-12.0593064454722,
-177.162356073909));
#143487=CARTESIAN_POINT('Ctrl Pts',(-58.4929564542504,-12.0597305436947,
-177.163038337516));
#143488=CARTESIAN_POINT('Ctrl Pts',(-58.4929630437302,-12.0601553416844,
-177.163720147168));
#143489=CARTESIAN_POINT('Ctrl Pts',(-58.4935968230333,-12.1010126145907,
-177.229296924179));
#143490=CARTESIAN_POINT('Ctrl Pts',(-58.4943004033954,-12.1491458631888,
-177.291840545738));
#143491=CARTESIAN_POINT('Ctrl Pts',(-58.4950024041184,-12.2028473374637,
-177.347256942163));
#143492=CARTESIAN_POINT('Ctrl Pts',(-58.4950097920195,-12.203412495261,
-177.347840147912));
#143493=CARTESIAN_POINT('Ctrl Pts',(-58.4950171797681,-12.2039782717463,
-177.348422567924));
#143494=CARTESIAN_POINT('Ctrl Pts',(-58.4950245672806,-12.2045446649403,
-177.349004197405));
#143495=CARTESIAN_POINT('Ctrl Pts',(-58.4957264419677,-12.2583566950054,
-177.404263800622));
#143496=CARTESIAN_POINT('Ctrl Pts',(-58.4964292592559,-12.3178002283294,
-177.452938198818));
#143497=CARTESIAN_POINT('Ctrl Pts',(-58.4970868450185,-12.3836929510146,
-177.494029767074));
#143498=CARTESIAN_POINT('Ctrl Pts',(-58.497092582954,-12.3842679150954,
-177.494388322234));
#143499=CARTESIAN_POINT('Ctrl Pts',(-58.4970983175096,-12.3848433769923,
-177.494746304328));
#143500=CARTESIAN_POINT('Ctrl Pts',(-58.4971040486531,-12.3854193371859,
-177.495103712595));
#143501=CARTESIAN_POINT('Ctrl Pts',(-58.4975789393164,-12.4331442135926,
-177.524719067176));
#143502=CARTESIAN_POINT('Ctrl Pts',(-58.4980179792098,-12.4835732801599,
-177.549749276793));
#143503=CARTESIAN_POINT('Ctrl Pts',(-58.4984026087067,-12.5359391559795,
-177.569640300895));
#143504=CARTESIAN_POINT('Ctrl Pts',(-58.4987756724468,-12.586730397031,
-177.588933204606));
#143505=CARTESIAN_POINT('Ctrl Pts',(-58.4990975247219,-12.6393425576089,
-177.603390836224));
#143506=CARTESIAN_POINT('Ctrl Pts',(-58.4993516232983,-12.6930550657785,
-177.612550490896));
#143507=CARTESIAN_POINT('Ctrl Pts',(-58.4995646774467,-12.7380914168376,
-177.620230590698));
#143508=CARTESIAN_POINT('Ctrl Pts',(-58.4997300980035,-12.7839007001903,
-177.624186575413));
#143509=CARTESIAN_POINT('Ctrl Pts',(-58.4998385375645,-12.8300551987823,
-177.624173936067));
#143510=CARTESIAN_POINT('',(-58.48912660861,-11.8396398505087,-171.871644662643));
#143511=CARTESIAN_POINT('',(-58.48912660861,-11.8396398505087,-179.64995));
#143512=CARTESIAN_POINT('',(-58.1115942404669,-6.23752120644091,-171.871644662643));
#143513=CARTESIAN_POINT('Origin',(0.,-12.9675000200281,-171.871644662643));
#143514=CARTESIAN_POINT('',(-58.1115942404669,-6.2375212064409,-176.427328712824));
#143515=CARTESIAN_POINT('',(-58.1115942404669,-6.2375212064409,-179.64995));
#143516=CARTESIAN_POINT('',(-57.9826110754301,-5.20432973493148,-177.68524973918));
#143517=CARTESIAN_POINT('Ctrl Pts',(-57.9826110754301,-5.20432973493148,
-177.68524973918));
#143518=CARTESIAN_POINT('Ctrl Pts',(-57.9864133803307,-5.2327289015275,
-177.684790303892));
#143519=CARTESIAN_POINT('Ctrl Pts',(-57.9901585317882,-5.26087114190315,
-177.682937908873));
#143520=CARTESIAN_POINT('Ctrl Pts',(-57.9938499513602,-5.28876235919762,
-177.679797008529));
#143521=CARTESIAN_POINT('Ctrl Pts',(-57.9976152499095,-5.31721178304887,
-177.676593247137));
#143522=CARTESIAN_POINT('Ctrl Pts',(-58.0013246616446,-5.34540021247655,
-177.672048874718));
#143523=CARTESIAN_POINT('Ctrl Pts',(-58.0049820412409,-5.37334248086361,
-177.666219172833));
#143524=CARTESIAN_POINT('Ctrl Pts',(-58.007100919411,-5.38953064535377,
-177.662841774415));
#143525=CARTESIAN_POINT('Ctrl Pts',(-58.0092023028963,-5.40563608053654,
-177.659031970271));
#143526=CARTESIAN_POINT('Ctrl Pts',(-58.0112866328471,-5.42166024630091,
-177.654792733909));
#143527=CARTESIAN_POINT('Ctrl Pts',(-58.0127082279004,-5.43258935796885,
-177.651901407879));
#143528=CARTESIAN_POINT('Ctrl Pts',(-58.0141227858996,-5.44348757569482,
-177.648808284626));
#143529=CARTESIAN_POINT('Ctrl Pts',(-58.0155294925106,-5.45434822190654,
-177.64551435811));
#143530=CARTESIAN_POINT('Ctrl Pts',(-58.0189462259725,-5.48072752022011,
-177.637513777987));
#143531=CARTESIAN_POINT('Ctrl Pts',(-58.0223147701654,-5.50687103546867,
-177.628330087141));
#143532=CARTESIAN_POINT('Ctrl Pts',(-58.0256102732283,-5.5325791664003,
-177.618027059099));
#143533=CARTESIAN_POINT('Ctrl Pts',(-58.0292381208968,-5.5608799086786,
-177.606684992183));
#143534=CARTESIAN_POINT('Ctrl Pts',(-58.0327774052011,-5.58865274716566,
-177.593984257917));
#143535=CARTESIAN_POINT('Ctrl Pts',(-58.0361953413916,-5.61562914495262,
-177.580061370298));
#143536=CARTESIAN_POINT('Ctrl Pts',(-58.0369297082255,-5.62142520746788,
-177.577069943211));
#143537=CARTESIAN_POINT('Ctrl Pts',(-58.0376584880584,-5.62718459987921,
-177.574022261851));
#143538=CARTESIAN_POINT('Ctrl Pts',(-58.0383813818279,-5.63290483163266,
-177.570919942798));
#143539=CARTESIAN_POINT('Ctrl Pts',(-58.0384493306635,-5.63344250826457,
-177.570628338449));
#143540=CARTESIAN_POINT('Ctrl Pts',(-58.0385172322329,-5.63397987194777,
-177.570336244847));
#143541=CARTESIAN_POINT('Ctrl Pts',(-58.0385850863885,-5.63451692127423,
-177.570043663697));
#143542=CARTESIAN_POINT('Ctrl Pts',(-58.0490694432021,-5.71749808455882,
-177.524836039379));
#143543=CARTESIAN_POINT('Ctrl Pts',(-58.0585606908555,-5.79407235500368,
-177.467381876561));
#143544=CARTESIAN_POINT('Ctrl Pts',(-58.0668921625487,-5.86215495271816,
-177.400951487675));
#143545=CARTESIAN_POINT('Ctrl Pts',(-58.0716810779971,-5.90128871155089,
-177.362767415605));
#143546=CARTESIAN_POINT('Ctrl Pts',(-58.0760868293938,-5.93761722714578,
-177.321616651462));
#143547=CARTESIAN_POINT('Ctrl Pts',(-58.0800778613687,-5.97074680033053,
-177.278112939551));
#143548=CARTESIAN_POINT('Ctrl Pts',(-58.0801358840197,-5.97122844660027,
-177.27748047138));
#143549=CARTESIAN_POINT('Ctrl Pts',(-58.0801938210413,-5.97170942905892,
-177.276847523818));
#143550=CARTESIAN_POINT('Ctrl Pts',(-58.0802516724784,-5.97218974777175,
-177.276214098177));
#143551=CARTESIAN_POINT('Ctrl Pts',(-58.086346247512,-6.0227907108724,-177.209483515685));
#143552=CARTESIAN_POINT('Ctrl Pts',(-58.0914882451368,-6.06600199005215,
-177.137485615197));
#143553=CARTESIAN_POINT('Ctrl Pts',(-58.0957336562472,-6.10193041985869,
-177.061710183546));
#143554=CARTESIAN_POINT('Ctrl Pts',(-58.0990967930801,-6.1303922631263,
-177.001682276099));
#143555=CARTESIAN_POINT('Ctrl Pts',(-58.1018971540568,-6.15428295037259,
-176.939282520675));
#143556=CARTESIAN_POINT('Ctrl Pts',(-58.1041602520257,-6.17363798086331,
-176.875236987128));
#143557=CARTESIAN_POINT('Ctrl Pts',(-58.1041777800786,-6.17378788864586,
-176.874740944307));
#143558=CARTESIAN_POINT('Ctrl Pts',(-58.1041952749008,-6.1739375157485,
-176.874244853752));
#143559=CARTESIAN_POINT('Ctrl Pts',(-58.104212736516,-6.1740868623495,-176.873748715522));
#143560=CARTESIAN_POINT('Ctrl Pts',(-58.1067717090136,-6.19597337403407,
-176.801040431038));
#143561=CARTESIAN_POINT('Ctrl Pts',(-58.1086155525892,-6.2118188643998,
-176.72738700765));
#143562=CARTESIAN_POINT('Ctrl Pts',(-58.1098212142835,-6.22220604020927,
-176.652935850911));
#143563=CARTESIAN_POINT('Ctrl Pts',(-58.1110268759779,-6.23259321601874,
-176.578484694172));
#143564=CARTESIAN_POINT('Ctrl Pts',(-58.1115942404669,-6.23752120644093,
-176.50323543809));
#143565=CARTESIAN_POINT('Ctrl Pts',(-58.1115942404669,-6.2375212064409,
-176.427328712824));
#143566=CARTESIAN_POINT('',(-57.914127722791,-4.70894021166827,-177.693561815623));
#143567=CARTESIAN_POINT('Origin',(-1.08549480256543,-12.950394379074,-185.613342531869));
#143568=CARTESIAN_POINT('',(-57.7706512256236,-3.75870764711888,-176.647241333324));
#143569=CARTESIAN_POINT('Ctrl Pts',(-57.7706512256236,-3.75870764711888,
-176.647241333324));
#143570=CARTESIAN_POINT('Ctrl Pts',(-57.7706512234859,-3.7587076337082,
-176.91349018761));
#143571=CARTESIAN_POINT('Ctrl Pts',(-57.7839302828914,-3.84070116554495,
-177.179630564281));
#143572=CARTESIAN_POINT('Ctrl Pts',(-57.8378689508709,-4.18900518947036,
-177.581280960616));
#143573=CARTESIAN_POINT('Ctrl Pts',(-57.8761547096863,-4.44264996470081,
-177.698192218067));
#143574=CARTESIAN_POINT('Ctrl Pts',(-57.914127722791,-4.70894021166827,
-177.693561815623));
#143575=CARTESIAN_POINT('',(-57.7706512256236,-3.75870764711888,-171.871644662643));
#143576=CARTESIAN_POINT('',(-57.7706512256236,-3.75870764711888,-179.64995));
#143577=CARTESIAN_POINT('',(-56.5940537057312,1.84341099694893,-171.871644662643));
#143578=CARTESIAN_POINT('Origin',(0.,-12.9675000200281,-171.871644662643));
#143579=CARTESIAN_POINT('',(-56.5940537057312,1.84341099694892,-176.848740272858));
#143580=CARTESIAN_POINT('',(-56.5940537057312,1.84341099694893,-179.64995));
#143581=CARTESIAN_POINT('',(-56.5169491525423,2.13496529160038,-177.558207897086));
#143582=CARTESIAN_POINT('Ctrl Pts',(-56.5169491525423,2.13496529160038,
-177.558207897086));
#143583=CARTESIAN_POINT('Ctrl Pts',(-56.5659347005564,1.95164994081541,
-177.37392715461));
#143584=CARTESIAN_POINT('Ctrl Pts',(-56.5940537017931,1.84341101199667,
-177.116606872607));
#143585=CARTESIAN_POINT('Ctrl Pts',(-56.5940537057312,1.84341099694892,
-176.848740272858));
#143586=CARTESIAN_POINT('',(-56.3252430313217,2.83493642067774,-177.84995));
#143587=CARTESIAN_POINT('Ctrl Pts',(-56.3252430313217,2.83493642067774,
-177.84995));
#143588=CARTESIAN_POINT('Ctrl Pts',(-56.3976379760506,2.57689628418379,
-177.849949962148));
#143589=CARTESIAN_POINT('Ctrl Pts',(-56.4669147992933,2.32220551629932,
-177.746434148089));
#143590=CARTESIAN_POINT('Ctrl Pts',(-56.5169491525423,2.13496529160038,
-177.558207897086));
#143591=CARTESIAN_POINT('',(-56.1837939657261,3.33069913254215,-177.84995));
#143592=CARTESIAN_POINT('Origin',(0.,-12.9675000200281,-177.84995));
#143593=CARTESIAN_POINT('',(-55.8866301012659,4.32222455627096,-176.84995));
#143594=CARTESIAN_POINT('Ctrl Pts',(-55.8866301012659,4.32222455627096,
-176.84995));
#143595=CARTESIAN_POINT('Ctrl Pts',(-55.8866301033422,4.3222245495596,-176.887711783017));
#143596=CARTESIAN_POINT('Ctrl Pts',(-55.8873019941254,4.32005750494367,
-176.925285001291));
#143597=CARTESIAN_POINT('Ctrl Pts',(-55.8886053322676,4.31584578460431,
-176.962497615251));
#143598=CARTESIAN_POINT('Ctrl Pts',(-55.8899346297675,4.31155017693619,
-177.000451414885));
#143599=CARTESIAN_POINT('Ctrl Pts',(-55.8919208352951,4.30512748218138,
-177.038031169975));
#143600=CARTESIAN_POINT('Ctrl Pts',(-55.8945372498695,4.2966554166734,-177.075061157623));
#143601=CARTESIAN_POINT('Ctrl Pts',(-55.8971529093906,4.28818579606139,
-177.112080459038));
#143602=CARTESIAN_POINT('Ctrl Pts',(-55.9003985106906,4.27766770883152,
-177.148551411106));
#143603=CARTESIAN_POINT('Ctrl Pts',(-55.9042621819464,4.26513074059418,
-177.184288779349));
#143604=CARTESIAN_POINT('Ctrl Pts',(-55.9062291959159,4.25874810862931,
-177.202482848646));
#143605=CARTESIAN_POINT('Ctrl Pts',(-55.9083566338582,4.25184146461301,
-177.22048652526));
#143606=CARTESIAN_POINT('Ctrl Pts',(-55.9106442880651,4.24441025685161,
-177.238272995257));
#143607=CARTESIAN_POINT('Ctrl Pts',(-55.9107052688196,4.24421216718633,
-177.238747119518));
#143608=CARTESIAN_POINT('Ctrl Pts',(-55.9107663607186,4.2440137135512,-177.239221068301));
#143609=CARTESIAN_POINT('Ctrl Pts',(-55.9108275637053,4.24381489610749,
-177.239694840879));
#143610=CARTESIAN_POINT('Ctrl Pts',(-55.921455868223,4.20928892853543,-177.321968590922));
#143611=CARTESIAN_POINT('Ctrl Pts',(-55.9354579988732,4.16369334127097,
-177.399293819938));
#143612=CARTESIAN_POINT('Ctrl Pts',(-55.9520401750182,4.10936168614069,
-177.468909678496));
#143613=CARTESIAN_POINT('Ctrl Pts',(-55.9599200188453,4.08354330418918,
-177.50199110813));
#143614=CARTESIAN_POINT('Ctrl Pts',(-55.9683824151876,4.05575233687861,
-177.533330971158));
#143615=CARTESIAN_POINT('Ctrl Pts',(-55.977341715845,4.02624042822255,-177.562628970791));
#143616=CARTESIAN_POINT('Ctrl Pts',(-55.9774917411594,4.02574624530113,
-177.563119571762));
#143617=CARTESIAN_POINT('Ctrl Pts',(-55.9776419059241,4.025251579432,-177.563609601226));
#143618=CARTESIAN_POINT('Ctrl Pts',(-55.9777922097306,4.02475643181778,
-177.564099057738));
#143619=CARTESIAN_POINT('Ctrl Pts',(-55.9952457911948,3.96725889117992,
-177.620935736128));
#143620=CARTESIAN_POINT('Ctrl Pts',(-56.0147502621915,3.90266672703055,
-177.670629519414));
#143621=CARTESIAN_POINT('Ctrl Pts',(-56.035495980374,3.83347839358597,-177.711737746819));
#143622=CARTESIAN_POINT('Ctrl Pts',(-56.0478214929272,3.79237199924909,
-177.73616109859));
#143623=CARTESIAN_POINT('Ctrl Pts',(-56.0605847921298,3.74964437876968,
-177.757554032043));
#143624=CARTESIAN_POINT('Ctrl Pts',(-56.0736137591996,3.70582717944109,
-177.775616713981));
#143625=CARTESIAN_POINT('Ctrl Pts',(-56.0737452759341,3.7053848807584,-177.775799041938));
#143626=CARTESIAN_POINT('Ctrl Pts',(-56.0738768160358,3.70494248350759,
-177.775981025699));
#143627=CARTESIAN_POINT('Ctrl Pts',(-56.0740083793673,3.70449998810519,
-177.776162665075));
#143628=CARTESIAN_POINT('Ctrl Pts',(-56.0854652800848,3.6659662581182,-177.791980326975));
#143629=CARTESIAN_POINT('Ctrl Pts',(-56.0971863579254,3.62638912180277,
-177.805308764985));
#143630=CARTESIAN_POINT('Ctrl Pts',(-56.1090759206044,3.58608423515432,
-177.816113161796));
#143631=CARTESIAN_POINT('Ctrl Pts',(-56.1213067753348,3.54462238943047,
-177.827227700776));
#143632=CARTESIAN_POINT('Ctrl Pts',(-56.1337163559748,3.50238900930299,
-177.835671763787));
#143633=CARTESIAN_POINT('Ctrl Pts',(-56.1462034955942,3.45971409454013,
-177.841352247251));
#143634=CARTESIAN_POINT('Ctrl Pts',(-56.1579134207247,3.41969531745779,
-177.846679170638));
#143635=CARTESIAN_POINT('Ctrl Pts',(-56.1696918925471,3.37928709608612,
-177.849575574952));
#143636=CARTESIAN_POINT('Ctrl Pts',(-56.181452499676,3.33876843673331,-177.849916077404));
#143637=CARTESIAN_POINT('Ctrl Pts',(-56.1822330780449,3.33607912072425,
-177.84993867733));
#143638=CARTESIAN_POINT('Ctrl Pts',(-56.1830135754984,3.33338932446783,
-177.849949999684));
#143639=CARTESIAN_POINT('Ctrl Pts',(-56.1837939657261,3.33069913254215,
-177.84995));
#143640=CARTESIAN_POINT('',(-55.8866301012659,4.32222455627096,-171.871644662643));
#143641=CARTESIAN_POINT('',(-55.8866301012659,4.32222455627096,-179.64995));
#143642=CARTESIAN_POINT('',(-53.8350584096845,9.92434320033876,-171.871644662643));
#143643=CARTESIAN_POINT('Origin',(0.,-12.9675000200281,-171.871644662643));
#143644=CARTESIAN_POINT('',(-53.8350584096845,9.92434320033876,-176.84995));
#143645=CARTESIAN_POINT('',(-53.8350584096845,9.92434320033876,-179.64995));
#143646=CARTESIAN_POINT('',(-53.4025720561307,10.9158686240676,-177.84995));
#143647=CARTESIAN_POINT('Ctrl Pts',(-53.4025720561307,10.9158686240675,
-177.84995));
#143648=CARTESIAN_POINT('Ctrl Pts',(-53.4256992941538,10.8641567398107,
-177.849949993739));
#143649=CARTESIAN_POINT('Ctrl Pts',(-53.4485179803107,10.8129304526923,
-177.845955353724));
#143650=CARTESIAN_POINT('Ctrl Pts',(-53.4709798749292,10.7623159210355,
-177.837971298851));
#143651=CARTESIAN_POINT('Ctrl Pts',(-53.4932283385007,10.7121823244318,
-177.8300631078));
#143652=CARTESIAN_POINT('Ctrl Pts',(-53.5151269426185,10.6626484619086,
-177.818240932981));
#143653=CARTESIAN_POINT('Ctrl Pts',(-53.5366259143442,10.6138407725573,
-177.80245915115));
#143654=CARTESIAN_POINT('Ctrl Pts',(-53.5459258227763,10.5927278073634,
-177.795632353673));
#143655=CARTESIAN_POINT('Ctrl Pts',(-53.5551508985509,10.5717508130022,
-177.788063986787));
#143656=CARTESIAN_POINT('Ctrl Pts',(-53.5642968110718,10.5509205718341,
-177.77974738364));
#143657=CARTESIAN_POINT('Ctrl Pts',(-53.5644850520156,10.5504918443291,
-177.779576211522));
#143658=CARTESIAN_POINT('Ctrl Pts',(-53.5646732319863,10.5500632415521,
-177.779404746864));
#143659=CARTESIAN_POINT('Ctrl Pts',(-53.5648613509312,10.5496347636521,
-177.779232989633));
#143660=CARTESIAN_POINT('Ctrl Pts',(-53.5997722939231,10.4701182239962,
-177.747358438588));
#143661=CARTESIAN_POINT('Ctrl Pts',(-53.6324973478398,10.3950941639657,
-177.70548367066));
#143662=CARTESIAN_POINT('Ctrl Pts',(-53.6625657515364,10.3258245179381,
-177.65369711681));
#143663=CARTESIAN_POINT('Ctrl Pts',(-53.6768635990427,10.2928860604893,
-177.629072056654));
#143664=CARTESIAN_POINT('Ctrl Pts',(-53.6905609342834,10.2612483121633,
-177.602206386714));
#143665=CARTESIAN_POINT('Ctrl Pts',(-53.7036082895117,10.2310442594454,
-177.573112646646));
#143666=CARTESIAN_POINT('Ctrl Pts',(-53.7038266840866,10.2305386856232,
-177.572625657913));
#143667=CARTESIAN_POINT('Ctrl Pts',(-53.7040448535835,10.2300336133805,
-177.572138119876));
#143668=CARTESIAN_POINT('Ctrl Pts',(-53.7042627976345,10.2295290436849,
-177.571650033405));
#143669=CARTESIAN_POINT('Ctrl Pts',(-53.7326736221947,10.1637541760739,
-177.508023891499));
#143670=CARTESIAN_POINT('Ctrl Pts',(-53.757265528039,10.106491327388,-177.435049789273));
#143671=CARTESIAN_POINT('Ctrl Pts',(-53.777230163758,10.059865738004,-177.354607724318));
#143672=CARTESIAN_POINT('Ctrl Pts',(-53.7856960958566,10.0400943242234,
-177.320496555482));
#143673=CARTESIAN_POINT('Ctrl Pts',(-53.7933301997471,10.0222350963628,
-177.28504246554));
#143674=CARTESIAN_POINT('Ctrl Pts',(-53.8000719149495,10.0064474410941,
-177.248388344963));
#143675=CARTESIAN_POINT('Ctrl Pts',(-53.8001626051629,10.0062350640087,
-177.247895270142));
#143676=CARTESIAN_POINT('Ctrl Pts',(-53.8002531267728,10.0060230790139,
-177.247402027608));
#143677=CARTESIAN_POINT('Ctrl Pts',(-53.800343479687,10.0058114863479,-177.246908617746));
#143678=CARTESIAN_POINT('Ctrl Pts',(-53.8073717082883,9.989352453007,-177.208528037134));
#143679=CARTESIAN_POINT('Ctrl Pts',(-53.8133972227366,9.97522506645285,
-177.169027476767));
#143680=CARTESIAN_POINT('Ctrl Pts',(-53.8183528652338,9.96359686430567,
-177.128668162154));
#143681=CARTESIAN_POINT('Ctrl Pts',(-53.8232487909443,9.95210878503223,
-177.088795187826));
#143682=CARTESIAN_POINT('Ctrl Pts',(-53.8271003741327,9.9430602856234,-177.048084581928));
#143683=CARTESIAN_POINT('Ctrl Pts',(-53.829861825915,9.93656859429005,-177.006803377711));
#143684=CARTESIAN_POINT('Ctrl Pts',(-53.8325710248907,9.93019974018784,
-176.966303305646));
#143685=CARTESIAN_POINT('Ctrl Pts',(-53.8342309082794,9.92629199069107,
-176.925254528035));
#143686=CARTESIAN_POINT('Ctrl Pts',(-53.8348176649726,9.92491022336673,
-176.883916088102));
#143687=CARTESIAN_POINT('Ctrl Pts',(-53.8349780875801,9.9245324403442,-176.872613924192));
#143688=CARTESIAN_POINT('Ctrl Pts',(-53.8350584093113,9.92434320121651,
-176.861290124361));
#143689=CARTESIAN_POINT('Ctrl Pts',(-53.8350584096845,9.92434320033876,
-176.84995));
#143690=CARTESIAN_POINT('',(-53.1780777607544,11.411631335932,-177.84995));
#143691=CARTESIAN_POINT('Origin',(0.,-12.9675000200281,-177.84995));
#143692=CARTESIAN_POINT('Ctrl Pts',(-52.9322463618642,11.9408779899289,
-177.695579616717));
#143693=CARTESIAN_POINT('Ctrl Pts',(-53.0073952368163,11.7811807683279,
-177.797243661242));
#143694=CARTESIAN_POINT('Ctrl Pts',(-53.092575147757,11.598137759657,-177.849949986084));
#143695=CARTESIAN_POINT('Ctrl Pts',(-53.1780777607544,11.411631335932,-177.84995));
#143696=CARTESIAN_POINT('Origin',(-57.4563699825363,-40.0047992274175,-179.64995));
#143697=CARTESIAN_POINT('',(-52.5050296388285,-39.3089337226171,-172.133326251627));
#143698=CARTESIAN_POINT('',(-52.5050296388285,-39.3089337226171,-171.64995));
#143699=CARTESIAN_POINT('',(-52.6451348158797,-38.6439112191206,-171.916267709118));
#143700=CARTESIAN_POINT('Ctrl Pts',(-52.6451348158641,-38.6439112191758,
-171.916267709546));
#143701=CARTESIAN_POINT('Ctrl Pts',(-52.5828776664721,-38.8638072188231,
-171.976552511458));
#143702=CARTESIAN_POINT('Ctrl Pts',(-52.5365289707088,-39.0848043302806,
-172.053524336593));
#143703=CARTESIAN_POINT('Ctrl Pts',(-52.5050296388285,-39.3089337226171,
-172.133326251627));
#143704=CARTESIAN_POINT('',(-52.6451348158641,-38.6439112191758,-176.84995));
#143705=CARTESIAN_POINT('',(-52.6451348158641,-38.6439112191758,-179.64995));
#143706=CARTESIAN_POINT('Ctrl Pts',(-52.9322463618642,-37.8758780299853,
-177.801086692062));
#143707=CARTESIAN_POINT('Ctrl Pts',(-52.8342434317084,-38.0841419017282,
-177.740238340822));
#143708=CARTESIAN_POINT('Ctrl Pts',(-52.7606534316743,-38.2807615372527,
-177.619039957031));
#143709=CARTESIAN_POINT('Ctrl Pts',(-52.6665978216312,-38.5625293047724,
-177.280964618108));
#143710=CARTESIAN_POINT('Ctrl Pts',(-52.6451348250506,-38.6439111866979,
-177.06710203648));
#143711=CARTESIAN_POINT('Ctrl Pts',(-52.6451348158641,-38.6439112191758,
-176.84995));
#143712=CARTESIAN_POINT('Origin',(-52.6124803109501,-38.5443824635529,-171.64995));
#143713=CARTESIAN_POINT('',(-51.4437383719606,-46.86041346952,-172.64995));
#143714=CARTESIAN_POINT('',(-50.6496826558921,-52.51041346952,-172.64995));
#143715=CARTESIAN_POINT('',(-50.5696324866523,-53.08000002,-172.64995));
#143716=CARTESIAN_POINT('',(-51.4437383719606,-46.86041346952,-176.84995));
#143717=CARTESIAN_POINT('',(-51.4437383719606,-46.86041346952,-171.64995));
#143718=CARTESIAN_POINT('',(-51.584279206663,-45.86041346952,-177.84995));
#143719=CARTESIAN_POINT('Ctrl Pts',(-51.584279206663,-45.86041346952,-177.84995));
#143720=CARTESIAN_POINT('Ctrl Pts',(-51.5473823619777,-46.1229481610447,
-177.849949999941));
#143721=CARTESIAN_POINT('Ctrl Pts',(-51.5109187616431,-46.3824001588352,
-177.742176873059));
#143722=CARTESIAN_POINT('Ctrl Pts',(-51.4849018294113,-46.5675202507065,
-177.557056781187));
#143723=CARTESIAN_POINT('Ctrl Pts',(-51.4588848971795,-46.7526403425778,
-177.371936689315));
#143724=CARTESIAN_POINT('Ctrl Pts',(-51.4437383719698,-46.8604134694541,
-177.112484691526));
#143725=CARTESIAN_POINT('Ctrl Pts',(-51.4437383719606,-46.86041346952,-176.84995));
#143726=CARTESIAN_POINT('',(-51.6545496240141,-45.3604134695199,-177.84995));
#143727=CARTESIAN_POINT('',(-52.6124803109501,-38.5443824635529,-177.84995));
#143728=CARTESIAN_POINT('',(-51.7950904587165,-44.36041346952,-176.84995));
#143729=CARTESIAN_POINT('Ctrl Pts',(-51.7950904587165,-44.36041346952,-176.84995));
#143730=CARTESIAN_POINT('Ctrl Pts',(-51.7950904587073,-44.3604134695857,
-177.112484691526));
#143731=CARTESIAN_POINT('Ctrl Pts',(-51.7799439334977,-44.4681865964612,
-177.371936689315));
#143732=CARTESIAN_POINT('Ctrl Pts',(-51.7539270012658,-44.6533066883334,
-177.557056781187));
#143733=CARTESIAN_POINT('Ctrl Pts',(-51.7279100690339,-44.8384267802056,
-177.742176873059));
#143734=CARTESIAN_POINT('Ctrl Pts',(-51.6914464686995,-45.0978787779945,
-177.849949999941));
#143735=CARTESIAN_POINT('Ctrl Pts',(-51.6545496240141,-45.3604134695199,
-177.84995));
#143736=CARTESIAN_POINT('',(-51.7950904587165,-44.36041346952,-172.64995));
#143737=CARTESIAN_POINT('',(-51.7950904587165,-44.36041346952,-171.64995));
#143738=CARTESIAN_POINT('',(-51.9770573602378,-43.0656516879596,-172.64995));
#143739=CARTESIAN_POINT('',(-51.7150402894768,-44.93000002,-172.64995));
#143740=CARTESIAN_POINT('Ctrl Pts',(-52.5050296388285,-39.3089337226171,
-172.133326251627));
#143741=CARTESIAN_POINT('Ctrl Pts',(-52.4540911811657,-39.671379681976,
-172.240867836498));
#143742=CARTESIAN_POINT('Ctrl Pts',(-52.4027597205576,-40.0366220025921,
-172.327673864957));
#143743=CARTESIAN_POINT('Ctrl Pts',(-52.3511170282707,-40.4040788516728,
-172.398058085082));
#143744=CARTESIAN_POINT('Ctrl Pts',(-52.3153892921749,-40.6582949033385,
-172.446751689745));
#143745=CARTESIAN_POINT('Ctrl Pts',(-52.2795125603002,-40.913571115058,
-172.487583846607));
#143746=CARTESIAN_POINT('Ctrl Pts',(-52.2435136369167,-41.1697167645394,
-172.521968983892));
#143747=CARTESIAN_POINT('Ctrl Pts',(-52.1712955694628,-41.6835750151102,
-172.590949606935));
#143748=CARTESIAN_POINT('Ctrl Pts',(-52.0985648108884,-42.2010812525561,
-172.632879273597));
#143749=CARTESIAN_POINT('Ctrl Pts',(-52.0252827479205,-42.7225102245918,
-172.645720761145));
#143750=CARTESIAN_POINT('Ctrl Pts',(-52.0092341999975,-42.8367015765715,
-172.648533007688));
#143751=CARTESIAN_POINT('Ctrl Pts',(-51.9931592080461,-42.9510810875898,
-172.649949999597));
#143752=CARTESIAN_POINT('Ctrl Pts',(-51.9770573602378,-43.0656516879596,
-172.64995));
#143753=CARTESIAN_POINT('',(-49.9349347781878,-57.596108877675,-172.64995));
#143754=CARTESIAN_POINT('',(-49.9349347781878,-57.596108877675,-171.64995));
#143755=CARTESIAN_POINT('',(-50.2983305691361,-55.0104134695199,-172.64995));
#143756=CARTESIAN_POINT('',(-49.9349347781878,-57.596108877675,-172.64995));
#143757=CARTESIAN_POINT('',(-50.2983305691361,-55.0104134695199,-176.84995));
#143758=CARTESIAN_POINT('',(-50.2983305691361,-55.0104134695199,-171.64995));
#143759=CARTESIAN_POINT('',(-50.4388714038385,-54.0104134695199,-177.84995));
#143760=CARTESIAN_POINT('Ctrl Pts',(-50.4388714038385,-54.0104134695199,
-177.84995));
#143761=CARTESIAN_POINT('Ctrl Pts',(-50.4019745591532,-54.2729481610447,
-177.849949999941));
#143762=CARTESIAN_POINT('Ctrl Pts',(-50.3655109588186,-54.5324001588352,
-177.742176873059));
#143763=CARTESIAN_POINT('Ctrl Pts',(-50.3394940265868,-54.7175202507064,
-177.557056781187));
#143764=CARTESIAN_POINT('Ctrl Pts',(-50.313477094355,-54.9026403425777,
-177.371936689315));
#143765=CARTESIAN_POINT('Ctrl Pts',(-50.2983305691453,-55.0104134694541,
-177.112484691526));
#143766=CARTESIAN_POINT('Ctrl Pts',(-50.2983305691361,-55.0104134695199,
-176.84995));
#143767=CARTESIAN_POINT('',(-50.5091418211897,-53.5104134695199,-177.84995));
#143768=CARTESIAN_POINT('',(-52.6124803109501,-38.5443824635529,-177.84995));
#143769=CARTESIAN_POINT('',(-50.6496826558921,-52.51041346952,-176.84995));
#143770=CARTESIAN_POINT('Ctrl Pts',(-50.6496826558921,-52.51041346952,-176.84995));
#143771=CARTESIAN_POINT('Ctrl Pts',(-50.6496826558828,-52.5104134695858,
-177.112484691526));
#143772=CARTESIAN_POINT('Ctrl Pts',(-50.6345361306733,-52.6181865964613,
-177.371936689314));
#143773=CARTESIAN_POINT('Ctrl Pts',(-50.6085191984413,-52.8033066883334,
-177.557056781187));
#143774=CARTESIAN_POINT('Ctrl Pts',(-50.5825022662094,-52.9884267802056,
-177.742176873059));
#143775=CARTESIAN_POINT('Ctrl Pts',(-50.546038665875,-53.2478787779945,
-177.849949999941));
#143776=CARTESIAN_POINT('Ctrl Pts',(-50.5091418211897,-53.5104134695199,
-177.84995));
#143777=CARTESIAN_POINT('',(-50.6496826558921,-52.51041346952,-171.64995));
#143778=CARTESIAN_POINT('Origin',(-46.9641305719631,-57.1785895747948,-171.64995));
#143779=CARTESIAN_POINT('',(-49.148508738101,-59.2349193215281,-172.64995));
#143780=CARTESIAN_POINT('',(-49.148508738101,-59.2349193215281,-171.64995));
#143781=CARTESIAN_POINT('Origin',(-46.9641305719631,-57.1785895747948,-172.64995));
#143782=CARTESIAN_POINT('Origin',(0.,-12.9675000200281,-171.64995));
#143783=CARTESIAN_POINT('',(-46.2674193015002,-62.1160087581289,-172.64995));
#143784=CARTESIAN_POINT('',(-46.2674193015002,-62.1160087581289,-171.64995));
#143785=CARTESIAN_POINT('Origin',(0.,-12.9675000200281,-172.64995));
#143786=CARTESIAN_POINT('Origin',(-44.2110895547669,-59.9316305919911,-171.64995));
#143787=CARTESIAN_POINT('',(-44.628608857647,-62.9024347982158,-172.64995));
#143788=CARTESIAN_POINT('',(-44.628608857647,-62.9024347982158,-171.64995));
#143789=CARTESIAN_POINT('Origin',(-44.2110895547669,-59.9316305919911,-172.64995));
#143790=CARTESIAN_POINT('Origin',(-45.5612236321975,-62.7713643393447,-171.64995));
#143791=CARTESIAN_POINT('',(-41.9304134495199,-63.2816414330641,-172.64995));
#143792=CARTESIAN_POINT('',(-41.5,-63.3421320985267,-172.64995));
#143793=CARTESIAN_POINT('',(-30.098151667932,-64.9445573802656,-172.64995));
#143794=CARTESIAN_POINT('Ctrl Pts',(-30.098151667932,-64.9445573802656,
-172.64995));
#143795=CARTESIAN_POINT('Ctrl Pts',(-29.5972390118835,-65.0149560630596,
-172.649949998196));
#143796=CARTESIAN_POINT('Ctrl Pts',(-29.1003075629514,-65.0847952236824,
-172.623020954979));
#143797=CARTESIAN_POINT('Ctrl Pts',(-28.6071269714123,-65.1541072356763,
-172.570721117616));
#143798=CARTESIAN_POINT('Ctrl Pts',(-28.4194541760847,-65.1804829269826,
-172.550819165184));
#143799=CARTESIAN_POINT('Ctrl Pts',(-28.2323246108402,-65.2067822722795,
-172.527242787946));
#143800=CARTESIAN_POINT('Ctrl Pts',(-28.0457258647366,-65.2330070158113,
-172.500075926044));
#143801=CARTESIAN_POINT('Ctrl Pts',(-27.7072474293089,-65.2805770576551,
-172.450796940499));
#143802=CARTESIAN_POINT('Ctrl Pts',(-27.3705571686055,-65.3278957879305,
-172.389422697018));
#143803=CARTESIAN_POINT('Ctrl Pts',(-27.0359780488069,-65.3749178167011,
-172.313768645042));
#143804=CARTESIAN_POINT('Ctrl Pts',(-26.7013989290084,-65.4219398454716,
-172.238114593065));
#143805=CARTESIAN_POINT('Ctrl Pts',(-26.3688785032062,-65.4686725436693,
-172.14853549193));
#143806=CARTESIAN_POINT('Ctrl Pts',(-26.0394480946395,-65.5149709682656,
-172.038055421481));
#143807=CARTESIAN_POINT('',(-31.28041344952,-64.7784013226445,-172.64995));
#143808=CARTESIAN_POINT('',(-27.530675086669,-65.3053926820751,-172.64995));
#143809=CARTESIAN_POINT('',(-31.28041344952,-64.7784013226445,-176.84995));
#143810=CARTESIAN_POINT('',(-31.28041344952,-64.7784013226445,-171.64995));
#143811=CARTESIAN_POINT('',(-32.28041344952,-64.6378604879421,-177.84995));
#143812=CARTESIAN_POINT('Ctrl Pts',(-32.28041344952,-64.6378604879421,-177.84995));
#143813=CARTESIAN_POINT('Ctrl Pts',(-32.0178787579952,-64.6747573326273,
-177.849949999941));
#143814=CARTESIAN_POINT('Ctrl Pts',(-31.7584267602047,-64.711220932962,
-177.742176873059));
#143815=CARTESIAN_POINT('Ctrl Pts',(-31.5733066683334,-64.7372378651937,
-177.557056781187));
#143816=CARTESIAN_POINT('Ctrl Pts',(-31.3881865764622,-64.7632547974255,
-177.371936689315));
#143817=CARTESIAN_POINT('Ctrl Pts',(-31.2804134495858,-64.7784013226352,
-177.112484691526));
#143818=CARTESIAN_POINT('Ctrl Pts',(-31.28041344952,-64.7784013226445,-176.84995));
#143819=CARTESIAN_POINT('',(-32.7804134495199,-64.5675900705909,-177.84995));
#143820=CARTESIAN_POINT('',(-45.5612236321975,-62.7713643393447,-177.84995));
#143821=CARTESIAN_POINT('',(-33.7804134495199,-64.4270492358885,-176.84995));
#143822=CARTESIAN_POINT('Ctrl Pts',(-33.7804134495199,-64.4270492358885,
-176.84995));
#143823=CARTESIAN_POINT('Ctrl Pts',(-33.7804134494542,-64.4270492358978,
-177.112484691526));
#143824=CARTESIAN_POINT('Ctrl Pts',(-33.6726403225778,-64.4421957611075,
-177.371936689315));
#143825=CARTESIAN_POINT('Ctrl Pts',(-33.4875202307065,-64.4682126933392,
-177.557056781187));
#143826=CARTESIAN_POINT('Ctrl Pts',(-33.3024001388352,-64.494229625571,
-177.742176873059));
#143827=CARTESIAN_POINT('Ctrl Pts',(-33.0429481410447,-64.5306932259057,
-177.849949999941));
#143828=CARTESIAN_POINT('Ctrl Pts',(-32.7804134495199,-64.5675900705909,
-177.84995));
#143829=CARTESIAN_POINT('',(-33.7804134495199,-64.4270492358885,-172.64995));
#143830=CARTESIAN_POINT('',(-33.7804134495199,-64.4270492358885,-171.64995));
#143831=CARTESIAN_POINT('',(-39.43041344952,-63.6329935198201,-172.64995));
#143832=CARTESIAN_POINT('',(-33.35,-64.4875399013512,-172.64995));
#143833=CARTESIAN_POINT('',(-39.43041344952,-63.63299351982,-176.84995));
#143834=CARTESIAN_POINT('',(-39.43041344952,-63.63299351982,-171.64995));
#143835=CARTESIAN_POINT('',(-40.4304134495199,-63.4924526851176,-177.84995));
#143836=CARTESIAN_POINT('Ctrl Pts',(-40.4304134495199,-63.4924526851176,
-177.84995));
#143837=CARTESIAN_POINT('Ctrl Pts',(-40.1678787579952,-63.5293495298029,
-177.849949999941));
#143838=CARTESIAN_POINT('Ctrl Pts',(-39.9084267602046,-63.5658131301376,
-177.742176873059));
#143839=CARTESIAN_POINT('Ctrl Pts',(-39.7233066683334,-63.5918300623693,
-177.557056781187));
#143840=CARTESIAN_POINT('Ctrl Pts',(-39.5381865764622,-63.6178469946011,
-177.371936689315));
#143841=CARTESIAN_POINT('Ctrl Pts',(-39.4304134495858,-63.6329935198108,
-177.112484691526));
#143842=CARTESIAN_POINT('Ctrl Pts',(-39.43041344952,-63.63299351982,-176.84995));
#143843=CARTESIAN_POINT('',(-40.9304134495199,-63.4221822677665,-177.84995));
#143844=CARTESIAN_POINT('',(-45.5612236321975,-62.7713643393447,-177.84995));
#143845=CARTESIAN_POINT('',(-41.9304134495199,-63.2816414330641,-176.84995));
#143846=CARTESIAN_POINT('Ctrl Pts',(-41.9304134495199,-63.2816414330641,
-176.84995));
#143847=CARTESIAN_POINT('Ctrl Pts',(-41.9304134494542,-63.2816414330733,
-177.112484691526));
#143848=CARTESIAN_POINT('Ctrl Pts',(-41.8226403225787,-63.2967879582829,
-177.371936689315));
#143849=CARTESIAN_POINT('Ctrl Pts',(-41.6375202307065,-63.3228048905148,
-177.557056781187));
#143850=CARTESIAN_POINT('Ctrl Pts',(-41.4524001388343,-63.3488218227467,
-177.742176873059));
#143851=CARTESIAN_POINT('Ctrl Pts',(-41.1929481410454,-63.3852854230811,
-177.849949999941));
#143852=CARTESIAN_POINT('Ctrl Pts',(-40.9304134495199,-63.4221822677665,
-177.84995));
#143853=CARTESIAN_POINT('',(-41.9304134495199,-63.2816414330641,-171.64995));
#143854=CARTESIAN_POINT('Ctrl Pts',(-42.0000617764046,-58.6035812240168,
-171.649949996184));
#143855=CARTESIAN_POINT('Ctrl Pts',(-41.5,-58.6035812240167,-171.650011780221));
#143856=CARTESIAN_POINT('Ctrl Pts',(-41.5,-58.6035812240168,-171.14995));
#143857=CARTESIAN_POINT('Ctrl Pts',(-41.9298643117037,-58.4475344566842,
-171.649958724212));
#143858=CARTESIAN_POINT('Ctrl Pts',(-41.5,-58.4568531764746,-171.583996757909));
#143859=CARTESIAN_POINT('Ctrl Pts',(-41.5,-58.415688549198,-171.149950044589));
#143860=CARTESIAN_POINT('Ctrl Pts',(-41.8681695534326,-58.2705723212599,
-171.649964230513));
#143861=CARTESIAN_POINT('Ctrl Pts',(-41.5,-58.2676804549564,-171.547558090573));
#143862=CARTESIAN_POINT('Ctrl Pts',(-41.5,-58.227785502943,-171.167360442076));
#143863=CARTESIAN_POINT('Ctrl Pts',(-41.7820591277973,-57.8880263314597,
-171.649970496006));
#143864=CARTESIAN_POINT('Ctrl Pts',(-41.5,-57.8827900893765,-171.511616746682));
#143865=CARTESIAN_POINT('Ctrl Pts',(-41.5,-57.8520667952971,-171.199054581264));
#143866=CARTESIAN_POINT('Ctrl Pts',(-41.7580490411456,-57.6823964313123,
-171.649971475853));
#143867=CARTESIAN_POINT('Ctrl Pts',(-41.4999999999974,-57.6764631965623,
-171.507283264427));
#143868=CARTESIAN_POINT('Ctrl Pts',(-41.5,-57.6641810084405,-171.212413163406));
#143869=CARTESIAN_POINT('Ctrl Pts',(-41.7579337455091,-57.2700461805852,
-171.649971481651));
#143870=CARTESIAN_POINT('Ctrl Pts',(-41.5000000000026,-57.275950831087,
-171.507256427632));
#143871=CARTESIAN_POINT('Ctrl Pts',(-41.5,-57.2881262594105,-171.212471328128));
#143872=CARTESIAN_POINT('Ctrl Pts',(-41.7818539242554,-57.0640562802561,
-171.649970508384));
#143873=CARTESIAN_POINT('Ctrl Pts',(-41.5,-57.0692704467351,-171.511552982749));
#143874=CARTESIAN_POINT('Ctrl Pts',(-41.5,-57.0999570266663,-171.199145438258));
#143875=CARTESIAN_POINT('Ctrl Pts',(-41.8680165447745,-56.6807474451005,
-171.649964244171));
#143876=CARTESIAN_POINT('Ctrl Pts',(-41.5,-56.6836417097802,-171.547472271891));
#143877=CARTESIAN_POINT('Ctrl Pts',(-41.5,-56.7235644715492,-171.167401493624));
#143878=CARTESIAN_POINT('Ctrl Pts',(-41.929815802996,-56.5034783375505,
-171.649958730482));
#143879=CARTESIAN_POINT('Ctrl Pts',(-41.4999999999999,-56.494149705945,
-171.583952704407));
#143880=CARTESIAN_POINT('Ctrl Pts',(-41.5,-56.5353526996975,-171.149950046396));
#143881=CARTESIAN_POINT('Ctrl Pts',(-42.0000617764046,-56.3473237326807,
-171.649949996184));
#143882=CARTESIAN_POINT('Ctrl Pts',(-41.5,-56.3473237326807,-171.650011780221));
#143883=CARTESIAN_POINT('Ctrl Pts',(-41.5,-56.3473237326807,-171.14995));
#143884=CARTESIAN_POINT('Origin',(-42.,-58.6035812240168,-171.14995));
#143885=CARTESIAN_POINT('Origin',(-42.,-56.3473237326807,-171.14995));
#143886=CARTESIAN_POINT('Origin',(0.,-12.9675000200281,-171.64995));
#143887=CARTESIAN_POINT('',(-48.9446667094463,-57.4569357767149,-171.64995));
#143888=CARTESIAN_POINT('',(-49.2787232447289,-55.08000002,-171.64995));
#143889=CARTESIAN_POINT('',(-49.3685531658572,-54.4408269190399,-171.64995));
#143890=CARTESIAN_POINT('',(-48.4203826827217,-58.549476072617,-171.64995));
#143891=CARTESIAN_POINT('Origin',(-46.9641305719631,-57.1785895747948,-171.64995));
#143892=CARTESIAN_POINT('',(-45.5819760525891,-61.3878827027496,-171.64995));
#143893=CARTESIAN_POINT('Origin',(0.,-12.9675000200281,-171.64995));
#143894=CARTESIAN_POINT('',(-44.489435756687,-61.9121667294742,-171.64995));
#143895=CARTESIAN_POINT('Origin',(-44.2110895547669,-59.9316305919911,-171.64995));
#143896=CARTESIAN_POINT('',(-42.,-62.2620341086569,-171.64995));
#143897=CARTESIAN_POINT('',(-44.489435756687,-61.9121667294742,-171.64995));
#143898=CARTESIAN_POINT('',(-42.,-62.3323045260081,-171.64995));
#143899=CARTESIAN_POINT('',(-42.5,-55.08000002,-171.64995));
#143900=CARTESIAN_POINT('Ctrl Pts',(-43.1572831724514,-55.0801481215059,
-171.649949978066));
#143901=CARTESIAN_POINT('Ctrl Pts',(-43.1572831724515,-54.58000002,-171.650098123446));
#143902=CARTESIAN_POINT('Ctrl Pts',(-43.1572831724514,-54.58000002,-171.14995));
#143903=CARTESIAN_POINT('Ctrl Pts',(-43.3271185292342,-54.9843723315205,
-171.649978738968));
#143904=CARTESIAN_POINT('Ctrl Pts',(-43.3143913613982,-54.5800000199971,
-171.56146605948));
#143905=CARTESIAN_POINT('Ctrl Pts',(-43.3817682803707,-54.58000002,-171.149950056136));
#143906=CARTESIAN_POINT('Ctrl Pts',(-43.529947173783,-54.8943395876967,
-171.649995064611));
#143907=CARTESIAN_POINT('Ctrl Pts',(-43.5407821982002,-54.5800000200016,
-171.520211742113));
#143908=CARTESIAN_POINT('Ctrl Pts',(-43.6059648750607,-54.58000002,-171.185915645006));
#143909=CARTESIAN_POINT('Ctrl Pts',(-43.9881565230544,-54.7646161135083,
-171.65000835312));
#143910=CARTESIAN_POINT('Ctrl Pts',(-44.0046317151095,-54.5800000199985,
-171.495876387334));
#143911=CARTESIAN_POINT('Ctrl Pts',(-44.0540062919344,-54.58000002,-171.260373422648));
#143912=CARTESIAN_POINT('Ctrl Pts',(-44.2440095987557,-54.7260645641701,
-171.650006647719));
#143913=CARTESIAN_POINT('Ctrl Pts',(-44.2580491347888,-54.58000002,-171.503655116484));
#143914=CARTESIAN_POINT('Ctrl Pts',(-44.2780419706102,-54.58000002,-171.296906912307));
#143915=CARTESIAN_POINT('Ctrl Pts',(-44.7601884828714,-54.7249655177493,
-171.65000663285));
#143916=CARTESIAN_POINT('Ctrl Pts',(-44.7466180387422,-54.58000002,-171.503788967852));
#143917=CARTESIAN_POINT('Ctrl Pts',(-44.7276655629966,-54.58000002,-171.297869301671));
#143918=CARTESIAN_POINT('Ctrl Pts',(-45.0183788445838,-54.7626525929476,
-171.650008425802));
#143919=CARTESIAN_POINT('Ctrl Pts',(-45.00211408603,-54.58000002,-171.49586884709));
#143920=CARTESIAN_POINT('Ctrl Pts',(-44.9532637149971,-54.58000002,-171.261822611311));
#143921=CARTESIAN_POINT('Ctrl Pts',(-45.4809398893321,-54.8922510295823,
-171.649995402787));
#143922=CARTESIAN_POINT('Ctrl Pts',(-45.4698465063652,-54.58000002,-171.519435241711));
#143923=CARTESIAN_POINT('Ctrl Pts',(-45.4045230317323,-54.58000002,-171.186802156157));
#143924=CARTESIAN_POINT('Ctrl Pts',(-45.6855420836464,-54.9825427397827,
-171.649979290157));
#143925=CARTESIAN_POINT('Ctrl Pts',(-45.6987517183234,-54.5800000199883,
-171.559908009068));
#143926=CARTESIAN_POINT('Ctrl Pts',(-45.6299507757146,-54.58000002,-171.149950055386));
#143927=CARTESIAN_POINT('Ctrl Pts',(-45.8586217441902,-55.0801481215059,
-171.649949978066));
#143928=CARTESIAN_POINT('Ctrl Pts',(-45.8586217441902,-54.58000002,-171.650098123446));
#143929=CARTESIAN_POINT('Ctrl Pts',(-45.8586217441902,-54.58000002,-171.14995));
#143930=CARTESIAN_POINT('Origin',(-43.1572831724514,-55.08000002,-171.14995));
#143931=CARTESIAN_POINT('Origin',(-45.8586217441902,-55.08000002,-171.14995));
#143932=CARTESIAN_POINT('Origin',(0.,-12.9675000200281,-171.64995));
#143933=CARTESIAN_POINT('',(-42.,-55.58000002,-171.64995));
#143934=CARTESIAN_POINT('',(-42.,-62.3323045260081,-171.64995));
#143935=CARTESIAN_POINT('',(-42.5,-55.08000002,-171.64995));
#143936=CARTESIAN_POINT('Origin',(-42.5,-55.58000002,-171.64995));
#143937=CARTESIAN_POINT('',(-42.5,-55.08000002,-171.64995));
#143938=CARTESIAN_POINT('Ctrl Pts',(-45.342056117244,28.9200050678815,-171.649949999974));
#143939=CARTESIAN_POINT('Ctrl Pts',(-45.342056117244,28.41999998,-171.649955087908));
#143940=CARTESIAN_POINT('Ctrl Pts',(-45.342056117244,28.41999998,-171.14995));
#143941=CARTESIAN_POINT('Ctrl Pts',(-45.2161093325492,28.8799153348106,
-171.649950408626));
#143942=CARTESIAN_POINT('Ctrl Pts',(-45.2207546457863,28.4199999799926,
-171.611343620546));
#143943=CARTESIAN_POINT('Ctrl Pts',(-45.2032855852167,28.41999998,-171.149950027441));
#143944=CARTESIAN_POINT('Ctrl Pts',(-45.0809055449373,28.8470468727513,
-171.649950690988));
#143945=CARTESIAN_POINT('Ctrl Pts',(-45.0814092233328,28.4199999800032,
-171.586474354512));
#143946=CARTESIAN_POINT('Ctrl Pts',(-45.0642313709306,28.41999998,-171.155055788632));
#143947=CARTESIAN_POINT('Ctrl Pts',(-44.7999542633241,28.8023061531436,
-171.649951053492));
#143948=CARTESIAN_POINT('Ctrl Pts',(-44.7998786663722,28.4199999799969,
-171.556875075933));
#143949=CARTESIAN_POINT('Ctrl Pts',(-44.7862672310248,28.41999998,-171.163656910012));
#143950=CARTESIAN_POINT('Ctrl Pts',(-44.6541596767004,28.7904721518725,
-171.64995113455));
#143951=CARTESIAN_POINT('Ctrl Pts',(-44.6527441767021,28.4199999799986,
-171.550586180072));
#143952=CARTESIAN_POINT('Ctrl Pts',(-44.6472721153249,28.41999998,-171.16702013224));
#143953=CARTESIAN_POINT('Ctrl Pts',(-44.36232828092,28.7904412154044,-171.649951134795));
#143954=CARTESIAN_POINT('Ctrl Pts',(-44.3637416796286,28.4199999800014,
-171.550568959217));
#143955=CARTESIAN_POINT('Ctrl Pts',(-44.3691883762669,28.41999998,-171.167028040093));
#143956=CARTESIAN_POINT('Ctrl Pts',(-44.2164190292983,28.802252604719,-171.649951053893));
#143957=CARTESIAN_POINT('Ctrl Pts',(-44.2164931090597,28.4199999799986,
-171.556843793952));
#143958=CARTESIAN_POINT('Ctrl Pts',(-44.2300913879779,28.41999998,-171.163669856825));
#143959=CARTESIAN_POINT('Ctrl Pts',(-43.9353228646307,28.846974377406,-171.649950691605));
#143960=CARTESIAN_POINT('Ctrl Pts',(-43.9348222136901,28.4199999800015,
-171.586421593668));
#143961=CARTESIAN_POINT('Ctrl Pts',(-43.9520032655911,28.41999998,-171.15506708045));
#143962=CARTESIAN_POINT('Ctrl Pts',(-43.8001087095933,28.8798156647999,
-171.649950409642));
#143963=CARTESIAN_POINT('Ctrl Pts',(-43.7954409326623,28.41999998,-171.611251100138));
#143964=CARTESIAN_POINT('Ctrl Pts',(-43.8129594627921,28.41999998,-171.149950027533));
#143965=CARTESIAN_POINT('Ctrl Pts',(-43.6738487993976,28.9200050678815,
-171.649949999974));
#143966=CARTESIAN_POINT('Ctrl Pts',(-43.6738487993976,28.41999998,-171.649955087908));
#143967=CARTESIAN_POINT('Ctrl Pts',(-43.6738487993976,28.41999998,-171.14995));
#143968=CARTESIAN_POINT('Origin',(-45.342056117244,28.91999998,-171.14995));
#143969=CARTESIAN_POINT('Origin',(-43.6738487993976,28.91999998,-171.14995));
#143970=CARTESIAN_POINT('Origin',(0.,-12.9675000200281,-171.64995));
#143971=CARTESIAN_POINT('',(-44.489435756687,35.9771666894179,-171.64995));
#143972=CARTESIAN_POINT('',(-41.3608268990399,36.416863989729,-171.64995));
#143973=CARTESIAN_POINT('',(-45.5819760525891,35.4528826626933,-171.64995));
#143974=CARTESIAN_POINT('Origin',(-44.2110895547669,33.9966305519348,-171.64995));
#143975=CARTESIAN_POINT('',(-48.4203826827217,32.6144760325608,-171.64995));
#143976=CARTESIAN_POINT('Origin',(0.,-12.9675000200281,-171.64995));
#143977=CARTESIAN_POINT('',(-48.9446667094463,31.5219357366587,-171.64995));
#143978=CARTESIAN_POINT('Origin',(-46.9641305719631,31.2435895347386,-171.64995));
#143979=CARTESIAN_POINT('',(-49.3103449325291,28.91999998,-171.64995));
#143980=CARTESIAN_POINT('',(-48.9446667094463,31.5219357366587,-171.64995));
#143981=CARTESIAN_POINT('',(-49.3806153498803,28.91999998,-171.64995));
#143982=CARTESIAN_POINT('Origin',(0.,-12.9675000200281,-171.64995));
#143983=CARTESIAN_POINT('',(-49.3806153498803,28.91999998,-171.64995));
#143984=CARTESIAN_POINT('Origin',(-24.2,67.7009572055632,-176.84995));
#143985=CARTESIAN_POINT('',(-24.2,-70.08000002,-177.34995));
#143986=CARTESIAN_POINT('Origin',(-24.2,-70.08000002,-176.84995));
#143987=CARTESIAN_POINT('',(-24.2,-73.08000002,-177.34995));
#143988=CARTESIAN_POINT('Ctrl Pts',(-23.0233258551573,-66.6335614680093,
-171.428053802042));
#143989=CARTESIAN_POINT('Ctrl Pts',(-23.7000418723672,-66.4085345904138,
-171.549239609537));
#143990=CARTESIAN_POINT('Ctrl Pts',(-23.6999999991623,-67.045403335443,
-171.20624326695));
#143991=CARTESIAN_POINT('Ctrl Pts',(-23.0096928629965,-66.7164302706428,
-171.571078901801));
#143992=CARTESIAN_POINT('Ctrl Pts',(-23.7000436385783,-66.4472919682874,
-171.670421709922));
#143993=CARTESIAN_POINT('Ctrl Pts',(-23.6999999991454,-67.1609416565799,
-171.420795636143));
#143994=CARTESIAN_POINT('Ctrl Pts',(-23.0026938228076,-66.7592463230786,
-171.731032985107));
#143995=CARTESIAN_POINT('Ctrl Pts',(-23.7000445959748,-66.4581897882961,
-171.777275420463));
#143996=CARTESIAN_POINT('Ctrl Pts',(-23.6999999991368,-67.220679933255,
-171.660715193487));
#143997=CARTESIAN_POINT('Ctrl Pts',(-23.0034444927493,-66.754655532928,
-171.89560645919));
#143998=CARTESIAN_POINT('Ctrl Pts',(-23.700044492639,-66.4569597257248,
-171.887725483309));
#143999=CARTESIAN_POINT('Ctrl Pts',(-23.6999999991377,-67.2142749444987,
-171.907589194352));
#144000=CARTESIAN_POINT('Origin',(-23.2,-67.0618271655313,-171.237717270032));
#144001=CARTESIAN_POINT('Origin',(0.,-12.9675000200281,-171.64995));
#144002=CARTESIAN_POINT('',(-17.3782102443554,-55.386710964082,-144.502505142985));
#144003=CARTESIAN_POINT('Ctrl Pts',(-17.3782102443554,-55.386710964082,
-144.502505142985));
#144004=CARTESIAN_POINT('Ctrl Pts',(-17.393698976901,-59.8910064811234,
-153.453571806853));
#144005=CARTESIAN_POINT('Ctrl Pts',(-17.4052435876731,-64.3204354194662,
-162.443049524475));
#144006=CARTESIAN_POINT('Ctrl Pts',(-17.4148840712405,-68.7171063154928,
-171.449026400902));
#144007=CARTESIAN_POINT('',(-22.9849163979996,-55.5914230987146,-150.046801024052));
#144008=CARTESIAN_POINT('Ctrl Pts',(-22.9849164538399,-55.5914231005407,
-150.046800950003));
#144009=CARTESIAN_POINT('Ctrl Pts',(-21.8819096287209,-55.5491926957159,
-148.844364427775));
#144010=CARTESIAN_POINT('Ctrl Pts',(-20.7471390543143,-55.506534730412,
-147.668247996036));
#144011=CARTESIAN_POINT('Ctrl Pts',(-19.5724972232793,-55.4640266335675,
-146.531662497644));
#144012=CARTESIAN_POINT('Ctrl Pts',(-18.8525414070574,-55.4379727754883,
-145.835031985619));
#144013=CARTESIAN_POINT('Ctrl Pts',(-18.1219084936406,-55.4121270272551,
-145.157368487698));
#144014=CARTESIAN_POINT('Ctrl Pts',(-17.3782871132615,-55.3867051178771,
-144.502418094041));
#144015=CARTESIAN_POINT('Ctrl Pts',(-23.0213852109847,-66.6453596297547,
-171.449026400902));
#144016=CARTESIAN_POINT('Ctrl Pts',(-23.0112491123844,-63.0152939322715,
-164.285990110815));
#144017=CARTESIAN_POINT('Ctrl Pts',(-22.9994804181366,-59.343937645489,
-157.144704426787));
#144018=CARTESIAN_POINT('Ctrl Pts',(-22.9849163103246,-55.591423110293,
-150.046801090999));
#144019=CARTESIAN_POINT('Ctrl Pts',(-17.4014093021639,-68.8184551193695,
-171.915576738158));
#144020=CARTESIAN_POINT('Ctrl Pts',(-17.0499387022882,-68.9277121722468,
-171.920632758432));
#144021=CARTESIAN_POINT('Ctrl Pts',(-17.0500000069342,-69.2954487057978,
-171.937551171933));
#144022=CARTESIAN_POINT('Ctrl Pts',(-17.4003036470898,-68.8268112548536,
-171.739609324912));
#144023=CARTESIAN_POINT('Ctrl Pts',(-17.0499389461697,-68.9377102872281,
-171.724562885898));
#144024=CARTESIAN_POINT('Ctrl Pts',(-17.0500000069124,-69.3074655181351,
-171.673561286109));
#144025=CARTESIAN_POINT('Ctrl Pts',(-17.4058449755969,-68.7849016359872,
-171.566109516219));
#144026=CARTESIAN_POINT('Ctrl Pts',(-17.0499377162343,-68.887140708855,
-171.529148195035));
#144027=CARTESIAN_POINT('Ctrl Pts',(-17.0500000070217,-69.2471945003534,
-171.413338787174));
#144028=CARTESIAN_POINT('Ctrl Pts',(-17.4177209010562,-68.6958205805999,
-171.409539580699));
#144029=CARTESIAN_POINT('Ctrl Pts',(-17.049935034885,-68.784349448281,-171.361182926232));
#144030=CARTESIAN_POINT('Ctrl Pts',(-17.050000007256,-69.1191208280442,
-171.178440426026));
#144031=CARTESIAN_POINT('Origin',(-17.55,-69.1496478013716,-171.237717270032));
#144032=CARTESIAN_POINT('Origin',(-16.55,-73.08000002,-176.84995));
#144033=CARTESIAN_POINT('',(-16.55,-70.08000002,-177.34995));
#144034=CARTESIAN_POINT('',(-16.55,-73.08000002,-177.34995));
#144035=CARTESIAN_POINT('Origin',(-16.55,-70.08000002,-176.84995));
#144036=CARTESIAN_POINT('Origin',(-41.5,-73.08000002,-177.34995));
#144037=CARTESIAN_POINT('',(-16.05,-70.08000002,-177.34995));
#144038=CARTESIAN_POINT('',(-16.05,-73.08000002,-177.34995));
#144039=CARTESIAN_POINT('',(41.5,-70.08000002,-177.34995));
#144040=CARTESIAN_POINT('Origin',(-16.05,67.7009572055632,-176.84995));
#144041=CARTESIAN_POINT('Origin',(-16.05,-70.08000002,-176.84995));
#144042=CARTESIAN_POINT('Ctrl Pts',(-14.9365391746094,-69.4116829512029,
-171.409919376296));
#144043=CARTESIAN_POINT('Ctrl Pts',(-15.5501264775731,-69.2858420378444,
-171.477695372047));
#144044=CARTESIAN_POINT('Ctrl Pts',(-15.5499999899231,-69.8405291599117,
-171.179005018994));
#144045=CARTESIAN_POINT('Ctrl Pts',(-14.9264726997877,-69.4976592258842,
-171.564867666237));
#144046=CARTESIAN_POINT('Ctrl Pts',(-15.5501302527645,-69.3463988305637,
-171.619616090566));
#144047=CARTESIAN_POINT('Ctrl Pts',(-15.5499999897578,-69.9655161046422,
-171.411462758814));
#144048=CARTESIAN_POINT('Ctrl Pts',(-14.9216112388798,-69.5395284795157,
-171.737936502975));
#144049=CARTESIAN_POINT('Ctrl Pts',(-15.5501321305785,-69.3710444733645,
-171.760987815194));
#144050=CARTESIAN_POINT('Ctrl Pts',(-15.5499999896779,-70.0263968022397,
-171.67105498688));
#144051=CARTESIAN_POINT('Ctrl Pts',(-14.9225783333433,-69.5312053406244,
-171.916063466645));
#144052=CARTESIAN_POINT('Ctrl Pts',(-15.550131758936,-69.3660274114058,
-171.908368448016));
#144053=CARTESIAN_POINT('Ctrl Pts',(-15.5499999896938,-70.0142946511941,
-171.938280796929));
#144054=CARTESIAN_POINT('Origin',(-15.05,-69.870344670579,-171.237717270032));
#144055=CARTESIAN_POINT('Origin',(0.,-12.9675000200281,-171.64995));
#144056=CARTESIAN_POINT('',(-9.30242220787652,-55.1547652726017,-138.840493482365));
#144057=CARTESIAN_POINT('Ctrl Pts',(-9.30242220787652,-55.1547652726017,
-138.840493482365));
#144058=CARTESIAN_POINT('Ctrl Pts',(-9.31373871873353,-60.3366136239018,
-149.697543382477));
#144059=CARTESIAN_POINT('Ctrl Pts',(-9.32139301854133,-65.4864258912612,
-160.57036601249));
#144060=CARTESIAN_POINT('Ctrl Pts',(-9.3276302147955,-70.6241744288951,
-171.449026400902));
#144061=CARTESIAN_POINT('',(-14.8995695352622,-55.3054345022359,-142.448537940653));
#144062=CARTESIAN_POINT('Ctrl Pts',(-14.8995694550282,-55.3054345175152,
-142.448537985759));
#144063=CARTESIAN_POINT('Ctrl Pts',(-13.8974507820956,-55.2740998389091,
-141.671728947382));
#144064=CARTESIAN_POINT('Ctrl Pts',(-12.8656304705197,-55.2438017962785,
-140.937883847407));
#144065=CARTESIAN_POINT('Ctrl Pts',(-10.9773541322587,-55.1936555815648,
-139.745510662921));
#144066=CARTESIAN_POINT('Ctrl Pts',(-10.1477730317694,-55.1733155860424,
-139.269609716656));
#144067=CARTESIAN_POINT('Ctrl Pts',(-9.30242220787652,-55.1547652726017,
-138.840493482365));
#144068=CARTESIAN_POINT('Ctrl Pts',(-14.9341313545396,-69.4322546019744,
-171.449026400902));
#144069=CARTESIAN_POINT('Ctrl Pts',(-14.9252396269456,-64.7624344426112,
-161.762591659591));
#144070=CARTESIAN_POINT('Ctrl Pts',(-14.9144862578123,-60.0660270491051,
-152.089344301479));
#144071=CARTESIAN_POINT('Ctrl Pts',(-14.8995694550282,-55.3054345175152,
-142.448537985759));
#144072=CARTESIAN_POINT('Ctrl Pts',(-9.32033898305081,-70.7202599648223,
-171.871644662643));
#144073=CARTESIAN_POINT('Ctrl Pts',(-8.89999999999996,-70.7880957152448,
-171.871644662643));
#144074=CARTESIAN_POINT('Ctrl Pts',(-8.9,-71.2138732976838,-171.871644662643));
#144075=CARTESIAN_POINT('Ctrl Pts',(-9.32033898569755,-70.7202599643952,
-171.725683074261));
#144076=CARTESIAN_POINT('Ctrl Pts',(-8.89999999999997,-70.7880957023883,
-171.715624308049));
#144077=CARTESIAN_POINT('Ctrl Pts',(-8.9,-71.2138732807092,-171.652697712588));
#144078=CARTESIAN_POINT('Ctrl Pts',(-9.32278024510803,-70.6879410017649,
-171.582358093922));
#144079=CARTESIAN_POINT('Ctrl Pts',(-8.90000000000455,-70.7514100828351,
-171.561941332422));
#144080=CARTESIAN_POINT('Ctrl Pts',(-8.9,-71.16598797688,-171.437720890984));
#144081=CARTESIAN_POINT('Ctrl Pts',(-9.3276302147955,-70.6241744288951,
-171.449026400902));
#144082=CARTESIAN_POINT('Ctrl Pts',(-8.89999999999997,-70.680735306053,
-171.422308714525));
#144083=CARTESIAN_POINT('Ctrl Pts',(-8.9,-71.0715121820529,-171.237717270032));
#144084=CARTESIAN_POINT('Origin',(-9.4,-71.0715121820529,-171.237717270032));
#144085=CARTESIAN_POINT('Ctrl Pts',(-8.9,-72.58000002,-174.451268889151));
#144086=CARTESIAN_POINT('Ctrl Pts',(-8.89999999999996,-73.0800000199999,
-174.45126888915));
#144087=CARTESIAN_POINT('Ctrl Pts',(-8.4,-73.08000002,-174.451268889151));
#144088=CARTESIAN_POINT('Ctrl Pts',(-8.9,-72.58000001309,-174.70608894667));
#144089=CARTESIAN_POINT('Ctrl Pts',(-8.89999999999997,-73.0780290434905,
-174.756376067791));
#144090=CARTESIAN_POINT('Ctrl Pts',(-8.40197484549326,-73.08000002,-174.75697631869));
#144091=CARTESIAN_POINT('Ctrl Pts',(-8.9,-72.5419664714886,-174.954543971783));
#144092=CARTESIAN_POINT('Ctrl Pts',(-8.89999999999997,-73.0306532835766,
-175.053905133681));
#144093=CARTESIAN_POINT('Ctrl Pts',(-8.40390532350201,-73.0343597586633,
-175.055047332367));
#144094=CARTESIAN_POINT('Ctrl Pts',(-8.9,-72.4287614956301,-175.317581230789));
#144095=CARTESIAN_POINT('Ctrl Pts',(-8.89999999999997,-72.892300013639,
-175.488192872161));
#144096=CARTESIAN_POINT('Ctrl Pts',(-8.40673247093662,-72.8985137923177,
-175.490582060873));
#144097=CARTESIAN_POINT('Ctrl Pts',(-8.9,-72.3815711902508,-175.436174718935));
#144098=CARTESIAN_POINT('Ctrl Pts',(-8.89999999999996,-72.8349801887897,
-175.629812439872));
#144099=CARTESIAN_POINT('Ctrl Pts',(-8.40765712457444,-72.8418854248583,
-175.632858253021));
#144100=CARTESIAN_POINT('Ctrl Pts',(-8.9,-72.2712246146549,-175.662282844729));
#144101=CARTESIAN_POINT('Ctrl Pts',(-8.89999999999995,-72.7014018648635,
-175.899567338683));
#144102=CARTESIAN_POINT('Ctrl Pts',(-8.40942187655549,-72.7094695330285,
-175.904119271778));
#144103=CARTESIAN_POINT('Ctrl Pts',(-8.9,-72.2077913051056,-175.770759223));
#144104=CARTESIAN_POINT('Ctrl Pts',(-8.90000000000094,-72.6248303464193,
-176.028888062411));
#144105=CARTESIAN_POINT('Ctrl Pts',(-8.41026946333178,-72.6333495611344,
-176.034257895752));
#144106=CARTESIAN_POINT('Ctrl Pts',(-8.9,-72.0642238201576,-175.978456398961));
#144107=CARTESIAN_POINT('Ctrl Pts',(-8.89999999999898,-72.4518932717193,
-176.276278393733));
#144108=CARTESIAN_POINT('Ctrl Pts',(-8.41189381664575,-72.4610685811814,
-176.283431179031));
#144109=CARTESIAN_POINT('Ctrl Pts',(-8.9,-71.9835055577593,-176.078093003191));
#144110=CARTESIAN_POINT('Ctrl Pts',(-8.89999999999997,-72.354843766023,
-176.394881486481));
#144111=CARTESIAN_POINT('Ctrl Pts',(-8.41267385193151,-72.3642066660697,
-176.402964676645));
#144112=CARTESIAN_POINT('Ctrl Pts',(-8.9,-71.8103399713904,-176.261453778625));
#144113=CARTESIAN_POINT('Ctrl Pts',(-8.89999999999996,-72.1469580486365,
-176.612968031678));
#144114=CARTESIAN_POINT('Ctrl Pts',(-8.41411048564612,-72.15640796091,-176.622941542856));
#144115=CARTESIAN_POINT('Ctrl Pts',(-8.9,-71.7174295924368,-176.34602338026));
#144116=CARTESIAN_POINT('Ctrl Pts',(-8.89999999999996,-72.0355638390553,
-176.713502881279));
#144117=CARTESIAN_POINT('Ctrl Pts',(-8.41477368991416,-72.0449155064423,
-176.724399172119));
#144118=CARTESIAN_POINT('Ctrl Pts',(-8.9,-71.4198068682475,-176.578502281526));
#144119=CARTESIAN_POINT('Ctrl Pts',(-8.89999999999996,-71.6793465425378,
-176.989505620533));
#144120=CARTESIAN_POINT('Ctrl Pts',(-8.4165979801388,-71.6877682388606,
-177.003302608065));
#144121=CARTESIAN_POINT('Ctrl Pts',(-8.9,-71.1936270830052,-176.705108386635));
#144122=CARTESIAN_POINT('Ctrl Pts',(-8.90000000001297,-71.4089014982389,
-177.139847092069));
#144123=CARTESIAN_POINT('Ctrl Pts',(-8.41759316850175,-71.4163525958445,
-177.155190995531));
#144124=CARTESIAN_POINT('Ctrl Pts',(-8.9,-70.9600741080247,-176.793015835821));
#144125=CARTESIAN_POINT('Ctrl Pts',(-8.89999999999996,-71.1298793121603,
-177.244155204947));
#144126=CARTESIAN_POINT('Ctrl Pts',(-8.41828452049191,-71.1360889256296,
-177.260652939026));
#144127=CARTESIAN_POINT('',(-8.4,-73.08000002,-174.451268889151));
#144128=CARTESIAN_POINT('Ctrl Pts',(-8.4181782717274,-71.1781985203566,
-177.244444626904));
#144129=CARTESIAN_POINT('Ctrl Pts',(-8.41749277252308,-71.4434978899076,
-177.139867487715));
#144130=CARTESIAN_POINT('Ctrl Pts',(-8.41653697428584,-71.6997115543464,
-176.993975834412));
#144131=CARTESIAN_POINT('Ctrl Pts',(-8.41477368991416,-72.0449155064423,
-176.724399172119));
#144132=CARTESIAN_POINT('Ctrl Pts',(-8.41411048564612,-72.15640796091,-176.622941542856));
#144133=CARTESIAN_POINT('Ctrl Pts',(-8.41267385193151,-72.3642066660697,
-176.402964676645));
#144134=CARTESIAN_POINT('Ctrl Pts',(-8.41189381664575,-72.4610685811814,
-176.283431179031));
#144135=CARTESIAN_POINT('Ctrl Pts',(-8.41026946333178,-72.6333495611344,
-176.034257895752));
#144136=CARTESIAN_POINT('Ctrl Pts',(-8.40942187655549,-72.7094695330285,
-175.904119271778));
#144137=CARTESIAN_POINT('Ctrl Pts',(-8.40765712457444,-72.8418854248583,
-175.632858253021));
#144138=CARTESIAN_POINT('Ctrl Pts',(-8.40673247093662,-72.8985137923177,
-175.490582060873));
#144139=CARTESIAN_POINT('Ctrl Pts',(-8.40390532350201,-73.0343597586633,
-175.055047332367));
#144140=CARTESIAN_POINT('Ctrl Pts',(-8.40197484549326,-73.08000002,-174.75697631869));
#144141=CARTESIAN_POINT('Ctrl Pts',(-8.4,-73.08000002,-174.451268889151));
#144142=CARTESIAN_POINT('Origin',(-8.4,-72.58000002,-174.451268889151));
#144143=CARTESIAN_POINT('Ctrl Pts',(-8.51230691249381,-71.1434663357063,
-177.254202907715));
#144144=CARTESIAN_POINT('Ctrl Pts',(-8.48384574056985,-73.08000002,-176.520599502442));
#144145=CARTESIAN_POINT('Ctrl Pts',(-8.40355780430818,-73.08000002,-174.451130838212));
#144146=CARTESIAN_POINT('Ctrl Pts',(-8.31384446654331,-71.169690780161,
-177.251953160255));
#144147=CARTESIAN_POINT('Ctrl Pts',(-8.285073768204,-73.0800000200061,-176.507651386999));
#144148=CARTESIAN_POINT('Ctrl Pts',(-8.20353011255175,-73.08000002,-174.458891192924));
#144149=CARTESIAN_POINT('Ctrl Pts',(-8.11484675268687,-71.1950080123697,
-177.249844108498));
#144150=CARTESIAN_POINT('Ctrl Pts',(-8.08524840860191,-73.0800000200063,
-176.495676023668));
#144151=CARTESIAN_POINT('Ctrl Pts',(-8.00350691066062,-73.08000002,-174.46684979476));
#144152=CARTESIAN_POINT('Ctrl Pts',(-7.91536503462484,-71.2194103886422,
-177.247865511992));
#144153=CARTESIAN_POINT('Ctrl Pts',(-7.88456937757999,-73.0800000199998,
-176.484587012089));
#144154=CARTESIAN_POINT('Ctrl Pts',(-7.80348623696872,-73.08000002,-174.474919939778));
#144155=CARTESIAN_POINT('',(-7.9,-73.08000002,-174.471034982976));
#144156=CARTESIAN_POINT('Ctrl Pts',(-7.9,-73.08000002,-174.471034982976));
#144157=CARTESIAN_POINT('Ctrl Pts',(-7.90199316078775,-73.08000002,-174.769251346187));
#144158=CARTESIAN_POINT('Ctrl Pts',(-7.90394076068631,-73.0365253516511,
-175.060187649793));
#144159=CARTESIAN_POINT('Ctrl Pts',(-7.90679252703161,-72.9073122055494,
-175.485606387024));
#144160=CARTESIAN_POINT('Ctrl Pts',(-7.90772857701081,-72.8532929465542,
-175.625142180141));
#144161=CARTESIAN_POINT('Ctrl Pts',(-7.90951546143904,-72.7269941355612,
-175.891343758978));
#144162=CARTESIAN_POINT('Ctrl Pts',(-7.9103743244834,-72.6543924247951,
-176.019207476496));
#144163=CARTESIAN_POINT('Ctrl Pts',(-7.9120222658245,-72.4901918790006,
-176.264409528534));
#144164=CARTESIAN_POINT('Ctrl Pts',(-7.91281676658892,-72.3977319011293,
-176.382553154925));
#144165=CARTESIAN_POINT('Ctrl Pts',(-7.91428825612723,-72.198695730848,
-176.6012613201));
#144166=CARTESIAN_POINT('Ctrl Pts',(-7.91496944868021,-72.0919119068452,
-176.702452310058));
#144167=CARTESIAN_POINT('Ctrl Pts',(-7.91682110979193,-71.7555164883556,
-176.977410112178));
#144168=CARTESIAN_POINT('Ctrl Pts',(-7.91784535584628,-71.5021289246249,
-177.129353672878));
#144169=CARTESIAN_POINT('Ctrl Pts',(-7.91859121655449,-71.2381488509313,
-177.239961484006));
#144170=CARTESIAN_POINT('Ctrl Pts',(-7.9,-73.08000002,-174.471034982976));
#144171=CARTESIAN_POINT('Ctrl Pts',(-8.06666381945983,-73.08000002,-174.464342510025));
#144172=CARTESIAN_POINT('Ctrl Pts',(-8.23333002609749,-73.08000002,-174.457737044943));
#144173=CARTESIAN_POINT('Ctrl Pts',(-8.4,-73.08000002,-174.451268889151));
#144174=CARTESIAN_POINT('Ctrl Pts',(-7.9,-73.08000002,-174.471034982976));
#144175=CARTESIAN_POINT('Ctrl Pts',(-7.39999999999995,-73.0800000199999,
-174.471034982977));
#144176=CARTESIAN_POINT('Ctrl Pts',(-7.4,-72.58000002,-174.471034982976));
#144177=CARTESIAN_POINT('Ctrl Pts',(-7.90199316078775,-73.08000002,-174.769251346187));
#144178=CARTESIAN_POINT('Ctrl Pts',(-7.39999999999996,-73.081997137201,
-174.769844466953));
#144179=CARTESIAN_POINT('Ctrl Pts',(-7.4,-72.5800000132661,-174.719615315523));
#144180=CARTESIAN_POINT('Ctrl Pts',(-7.90394076068631,-73.0365253516511,
-175.060187649793));
#144181=CARTESIAN_POINT('Ctrl Pts',(-7.39999999999996,-73.040326257465,
-175.061328113453));
#144182=CARTESIAN_POINT('Ctrl Pts',(-7.4,-72.5437711321103,-174.962127460747));
#144183=CARTESIAN_POINT('Ctrl Pts',(-7.90679252703161,-72.9073122055494,
-175.485606387024));
#144184=CARTESIAN_POINT('Ctrl Pts',(-7.39999999999996,-72.9137734508192,
-175.488022550208));
#144185=CARTESIAN_POINT('Ctrl Pts',(-7.4,-72.4360935067573,-175.316738645421));
#144186=CARTESIAN_POINT('Ctrl Pts',(-7.90772857701081,-72.8532929465542,
-175.625142180141));
#144187=CARTESIAN_POINT('Ctrl Pts',(-7.40000000000002,-72.8605108035235,
-175.628237972001));
#144188=CARTESIAN_POINT('Ctrl Pts',(-7.4,-72.3910774582401,-175.433049854657));
#144189=CARTESIAN_POINT('Ctrl Pts',(-7.90951546143904,-72.7269941355612,
-175.891343758978));
#144190=CARTESIAN_POINT('Ctrl Pts',(-7.39999999999993,-72.7355139213092,
-175.896009980972));
#144191=CARTESIAN_POINT('Ctrl Pts',(-7.4,-72.2858284501893,-175.654944429739));
#144192=CARTESIAN_POINT('Ctrl Pts',(-7.9103743244834,-72.6543924247951,
-176.019207476496));
#144193=CARTESIAN_POINT('Ctrl Pts',(-7.39999999999901,-72.6634371311262,
-176.024735407069));
#144194=CARTESIAN_POINT('Ctrl Pts',(-7.4,-72.2253270246874,-175.761526340889));
#144195=CARTESIAN_POINT('Ctrl Pts',(-7.9120222658245,-72.4901918790006,
-176.264409528534));
#144196=CARTESIAN_POINT('Ctrl Pts',(-7.40000000000093,-72.5000420015558,
-176.271831635453));
#144197=CARTESIAN_POINT('Ctrl Pts',(-7.4,-72.0884932351423,-175.96591668417));
#144198=CARTESIAN_POINT('Ctrl Pts',(-7.91281676658892,-72.3977319011293,
-176.382553154925));
#144199=CARTESIAN_POINT('Ctrl Pts',(-7.39999999999761,-72.4078441030974,
-176.390977561524));
#144200=CARTESIAN_POINT('Ctrl Pts',(-7.4,-72.0114432535103,-176.064396375895));
#144201=CARTESIAN_POINT('Ctrl Pts',(-7.91428825612723,-72.198695730848,
-176.6012613201));
#144202=CARTESIAN_POINT('Ctrl Pts',(-7.40000000000231,-72.2090331198025,
-176.611745838634));
#144203=CARTESIAN_POINT('Ctrl Pts',(-7.4,-71.8455797798041,-176.246702589259));
#144204=CARTESIAN_POINT('Ctrl Pts',(-7.91496944868021,-72.0919119068452,
-176.702452310058));
#144205=CARTESIAN_POINT('Ctrl Pts',(-7.40000000000137,-72.1022117673413,
-176.713954380549));
#144206=CARTESIAN_POINT('Ctrl Pts',(-7.4,-71.7565932593015,-176.331051292497));
#144207=CARTESIAN_POINT('Ctrl Pts',(-7.91685114292327,-71.7500603021656,
-176.981869807169));
#144208=CARTESIAN_POINT('Ctrl Pts',(-7.39999999999722,-71.7595719221786,
-176.996603847265));
#144209=CARTESIAN_POINT('Ctrl Pts',(-7.4,-71.4717169212771,-176.56396241752));
#144210=CARTESIAN_POINT('Ctrl Pts',(-7.91789548135802,-71.4896799957509,
-177.136789521634));
#144211=CARTESIAN_POINT('Ctrl Pts',(-7.39999999999657,-71.4982684775377,
-177.153312936568));
#144212=CARTESIAN_POINT('Ctrl Pts',(-7.4,-71.2547332556153,-176.693097313134));
#144213=CARTESIAN_POINT('Ctrl Pts',(-7.91864558019502,-71.2187040784628,
-177.248023282853));
#144214=CARTESIAN_POINT('Ctrl Pts',(-7.39999999999996,-71.2260554869631,
-177.265927135801));
#144215=CARTESIAN_POINT('Ctrl Pts',(-7.4,-71.028920068719,-176.785817298486));
#144216=CARTESIAN_POINT('Origin',(-7.9,-72.58000002,-174.471034982976));
#144217=CARTESIAN_POINT('Ctrl Pts',(-6.84687749809456,-70.9710952348089,
-171.449026400902));
#144218=CARTESIAN_POINT('Ctrl Pts',(-7.39999999999995,-70.9175980522952,
-171.474145745141));
#144219=CARTESIAN_POINT('Ctrl Pts',(-7.4,-71.4211246238516,-171.237717270032));
#144220=CARTESIAN_POINT('Ctrl Pts',(-6.84335093752903,-71.0335272731666,
-171.581102626116));
#144221=CARTESIAN_POINT('Ctrl Pts',(-7.40000000000424,-70.9726288200743,
-171.600718024433));
#144222=CARTESIAN_POINT('Ctrl Pts',(-7.4,-71.5141496698322,-171.435834655863));
#144223=CARTESIAN_POINT('Ctrl Pts',(-6.84152542419482,-71.0660673850682,
-171.724228262147));
#144224=CARTESIAN_POINT('Ctrl Pts',(-7.39999999999997,-71.0003029730699,
-171.734045906264));
#144225=CARTESIAN_POINT('Ctrl Pts',(-7.4,-71.5626363329153,-171.650517772678));
#144226=CARTESIAN_POINT('Ctrl Pts',(-6.84152542372878,-71.066067385123,
-171.871644662643));
#144227=CARTESIAN_POINT('Ctrl Pts',(-7.39999999999996,-71.0003029749948,
-171.871644662643));
#144228=CARTESIAN_POINT('Ctrl Pts',(-7.4,-71.5626363369615,-171.871644662643));
#144229=CARTESIAN_POINT('Origin',(-6.9,-71.4211246238516,-171.237717270032));
#144230=CARTESIAN_POINT('Origin',(0.,-12.9675000200281,-171.64995));
#144231=CARTESIAN_POINT('',(-1.23668893165473,-55.0504165218146,-136.482360813851));
#144232=CARTESIAN_POINT('Ctrl Pts',(-1.23668893165476,-55.0504165218146,
-136.482360813851));
#144233=CARTESIAN_POINT('Ctrl Pts',(-1.23673299366641,-55.1913381585796,
-136.784440607054));
#144234=CARTESIAN_POINT('Ctrl Pts',(-1.23677661819369,-55.3322593149882,
-137.08652062441));
#144235=CARTESIAN_POINT('Ctrl Pts',(-1.23699261729668,-56.0368627647092,
-138.596921799561));
#144236=CARTESIAN_POINT('Ctrl Pts',(-1.23715863033152,-56.6005380707885,
-139.805246217854));
#144237=CARTESIAN_POINT('Ctrl Pts',(-1.23731859936897,-57.1642067307399,
-141.01357373723));
#144238=CARTESIAN_POINT('Ctrl Pts',(-1.23795847551899,-59.4188813711729,
-145.84688381608));
#144239=CARTESIAN_POINT('Ctrl Pts',(-1.23850317159002,-61.6734513223852,
-150.68024274455));
#144240=CARTESIAN_POINT('Ctrl Pts',(-1.23898586311735,-63.927952799307,
-155.513633616344));
#144241=CARTESIAN_POINT('Ctrl Pts',(-1.23951632777425,-66.4055876545563,
-160.825396689281));
#144242=CARTESIAN_POINT('Ctrl Pts',(-1.23997137264739,-68.8831392394364,
-166.137198611174));
#144243=CARTESIAN_POINT('Ctrl Pts',(-1.24037635835043,-71.360635368318,
-171.449026400902));
#144244=CARTESIAN_POINT('',(-6.82752390438728,-55.1067946098355,-137.742762001241));
#144245=CARTESIAN_POINT('Ctrl Pts',(-6.82752390105444,-55.106794611208,
-137.742762010959));
#144246=CARTESIAN_POINT('Ctrl Pts',(-6.37447262318503,-55.0992223452637,
-137.571341088341));
#144247=CARTESIAN_POINT('Ctrl Pts',(-5.91551255237738,-55.0922385931689,
-137.414112752179));
#144248=CARTESIAN_POINT('Ctrl Pts',(-4.97306841018422,-55.0794633322322,
-137.127585972214));
#144249=CARTESIAN_POINT('Ctrl Pts',(-4.48820368733454,-55.0737025194561,
-136.999007240366));
#144250=CARTESIAN_POINT('Ctrl Pts',(-3.08479586460781,-55.0595407739023,
-136.68378809349));
#144251=CARTESIAN_POINT('Ctrl Pts',(-2.16238887065941,-55.0533427639956,
-136.546951183472));
#144252=CARTESIAN_POINT('Ctrl Pts',(-1.23668893165476,-55.0504165218146,
-136.482360813851));
#144253=CARTESIAN_POINT('Ctrl Pts',(-6.84687749809456,-70.9710952348089,
-171.449026400902));
#144254=CARTESIAN_POINT('Ctrl Pts',(-6.84214680864307,-65.6936814169362,
-160.208420694676));
#144255=CARTESIAN_POINT('Ctrl Pts',(-6.83631983013148,-60.409494445995,
-148.971070239119));
#144256=CARTESIAN_POINT('Ctrl Pts',(-6.82752390105444,-55.106794611208,
-137.742762010959));
#144257=CARTESIAN_POINT('Ctrl Pts',(-1.23940677966098,-71.4543692372681,
-171.871644662643));
#144258=CARTESIAN_POINT('Ctrl Pts',(-0.749999999999965,-71.4647403528508,
-171.871644662643));
#144259=CARTESIAN_POINT('Ctrl Pts',(-0.749999999999965,-71.9542570083556,
-171.871644662643));
#144260=CARTESIAN_POINT('Ctrl Pts',(-1.23940678000784,-71.4543692372607,
-171.725769781663));
#144261=CARTESIAN_POINT('Ctrl Pts',(-0.749999999999918,-71.4647403416089,
-171.724250912112));
#144262=CARTESIAN_POINT('Ctrl Pts',(-0.749999999999965,-71.9542569918424,
-171.652832243085));
#144263=CARTESIAN_POINT('Ctrl Pts',(-1.23973038817724,-71.4229357713421,
-171.582570495172));
#144264=CARTESIAN_POINT('Ctrl Pts',(-0.749999999994911,-71.432604194084,
-171.579497326419));
#144265=CARTESIAN_POINT('Ctrl Pts',(-0.749999999999965,-71.9071171402653,
-171.43803354201));
#144266=CARTESIAN_POINT('Ctrl Pts',(-1.24037635835043,-71.360635368318,
-171.449026400902));
#144267=CARTESIAN_POINT('Ctrl Pts',(-0.749999999999965,-71.3691907154173,
-171.445036077089));
#144268=CARTESIAN_POINT('Ctrl Pts',(-0.749999999999965,-71.813687061541,
-171.237717270032));
#144269=CARTESIAN_POINT('Origin',(-1.24999999999996,-71.813687061541,-171.237717270032));
#144270=CARTESIAN_POINT('Origin',(-25.7,-66.1031295107182,-179.64995));
#144271=CARTESIAN_POINT('Origin',(-25.7,-66.1031295107182,-176.84995));
#144272=CARTESIAN_POINT('Origin',(-25.7,-66.1031295107182,-171.854014632589));
#144273=CARTESIAN_POINT('Ctrl Pts',(-25.2,-66.1031295107182,-176.84995));
#144274=CARTESIAN_POINT('Ctrl Pts',(-25.2,-65.7373527968361,-176.84995));
#144275=CARTESIAN_POINT('Ctrl Pts',(-25.548606520496,-65.6266003779638,
-176.84995));
#144276=CARTESIAN_POINT('Ctrl Pts',(-25.2,-66.103129518477,-176.919185448026));
#144277=CARTESIAN_POINT('Ctrl Pts',(-25.1999999820547,-65.7373528064706,
-176.935176476617));
#144278=CARTESIAN_POINT('Ctrl Pts',(-25.5486064910184,-65.6266003873288,
-176.988420898571));
#144279=CARTESIAN_POINT('Ctrl Pts',(-25.1851215566574,-66.1120606092764,
-176.989079172076));
#144280=CARTESIAN_POINT('Ctrl Pts',(-25.1785584539962,-65.7486947399145,
-177.021615691098));
#144281=CARTESIAN_POINT('Ctrl Pts',(-25.5128982512925,-65.6373177084965,
-177.128208340634));
#144282=CARTESIAN_POINT('Ctrl Pts',(-25.1297698837022,-66.151663029906,
-177.114520781302));
#144283=CARTESIAN_POINT('Ctrl Pts',(-25.0944218125655,-65.7952388640609,
-177.17698788051));
#144284=CARTESIAN_POINT('Ctrl Pts',(-25.3800542465628,-65.6848405887261,
-177.37909156612));
#144285=CARTESIAN_POINT('Ctrl Pts',(-25.0892600555381,-66.1826911909829,
-177.170686801435));
#144286=CARTESIAN_POINT('Ctrl Pts',(-25.0308899200954,-65.8308593817032,
-177.246991922054));
#144287=CARTESIAN_POINT('Ctrl Pts',(-25.2828559308331,-65.7220623109706,
-177.491403988801));
#144288=CARTESIAN_POINT('Ctrl Pts',(-25.0407404589729,-66.228934721057,
-177.2158679411));
#144289=CARTESIAN_POINT('Ctrl Pts',(-24.9516549782085,-65.8798945343464,
-177.298823774072));
#144290=CARTESIAN_POINT('Ctrl Pts',(-25.166383622031,-65.7775666303703,
-177.581785882201));
#144291=CARTESIAN_POINT('Ctrl Pts',(-25.0407404589729,-66.228934721057,
-177.2158679411));
#144292=CARTESIAN_POINT('Ctrl Pts',(-25.0892600555381,-66.1826911909829,
-177.170686801435));
#144293=CARTESIAN_POINT('Ctrl Pts',(-25.1297698837022,-66.151663029906,
-177.114520781302));
#144294=CARTESIAN_POINT('Ctrl Pts',(-25.1851215566574,-66.1120606092764,
-176.989079172076));
#144295=CARTESIAN_POINT('Ctrl Pts',(-25.2,-66.103129518477,-176.919185448026));
#144296=CARTESIAN_POINT('Ctrl Pts',(-25.2,-66.1031295107182,-176.84995));
#144297=CARTESIAN_POINT('Ctrl Pts',(-26.0394480946395,-65.5149709682657,
-172.038055421481));
#144298=CARTESIAN_POINT('Ctrl Pts',(-26.1751497442534,-65.4958993451585,
-171.625426858395));
#144299=CARTESIAN_POINT('Ctrl Pts',(-26.2234488624093,-65.1680142434972,
-171.34400271074));
#144300=CARTESIAN_POINT('Ctrl Pts',(-25.8509081007284,-65.5414685363847,
-171.953748619745));
#144301=CARTESIAN_POINT('Ctrl Pts',(-25.9647846003821,-65.5168153550888,
-171.580148440091));
#144302=CARTESIAN_POINT('Ctrl Pts',(-25.9874436760592,-65.2410608891827,
-171.301817192477));
#144303=CARTESIAN_POINT('Ctrl Pts',(-25.6648820617275,-65.585552959265,
-171.879293448435));
#144304=CARTESIAN_POINT('Ctrl Pts',(-25.7473133163572,-65.5608787626348,
-171.533711217624));
#144305=CARTESIAN_POINT('Ctrl Pts',(-25.7492812072149,-65.3269811309762,
-171.264627955552));
#144306=CARTESIAN_POINT('Ctrl Pts',(-25.4789353138755,-65.6496769315936,
-171.836539704699));
#144307=CARTESIAN_POINT('Ctrl Pts',(-25.5297569849445,-65.6321510137328,
-171.506776385146));
#144308=CARTESIAN_POINT('Ctrl Pts',(-25.5048932192108,-65.4282717079069,
-171.24324485235));
#144309=CARTESIAN_POINT('',(-25.5241645957023,-65.4203114663316,-171.244965273982));
#144310=CARTESIAN_POINT('',(-26.2234488624093,-65.1680142434972,-171.34400271074));
#144311=CARTESIAN_POINT('Ctrl Pts',(-25.5241645957028,-65.4203114663335,
-171.244965273985));
#144312=CARTESIAN_POINT('Ctrl Pts',(-25.7618083043786,-65.3224706961895,
-171.266588348947));
#144313=CARTESIAN_POINT('Ctrl Pts',(-25.9936511816685,-65.2391401680605,
-171.302927382557));
#144314=CARTESIAN_POINT('Ctrl Pts',(-26.2234488624093,-65.1680142434972,
-171.34400271074));
#144315=CARTESIAN_POINT('Origin',(-25.9002749936795,-64.5247028995241,-172.038055421481));
#144316=CARTESIAN_POINT('Ctrl Pts',(-25.5241645957028,-65.4203114663335,
-171.244965273984));
#144317=CARTESIAN_POINT('Ctrl Pts',(-25.5204167023824,-65.4915081760158,
-171.329224126564));
#144318=CARTESIAN_POINT('Ctrl Pts',(-25.5190396326646,-65.5455021430107,
-171.42367336987));
#144319=CARTESIAN_POINT('Ctrl Pts',(-25.5254918386358,-65.6165368852731,
-171.632443841085));
#144320=CARTESIAN_POINT('Ctrl Pts',(-25.5332781069629,-65.6314702205409,
-171.740892625582));
#144321=CARTESIAN_POINT('Ctrl Pts',(-25.5486065204936,-65.6266003779646,
-171.854014632593));
#144322=CARTESIAN_POINT('Origin',(-24.7,-73.08000002,-176.84995));
#144323=CARTESIAN_POINT('',(-24.7,-70.08000002,-177.34995));
#144324=CARTESIAN_POINT('',(-24.7,-73.08000002,-177.34995));
#144325=CARTESIAN_POINT('Origin',(-24.7,-70.08000002,-176.84995));
#144326=CARTESIAN_POINT('Origin',(-41.5,-73.08000002,-177.34995));
#144327=CARTESIAN_POINT('',(41.5,-70.08000002,-177.34995));
#144328=CARTESIAN_POINT('Ctrl Pts',(-1.23668893165476,-55.0504165218147,
-95.5762821576554));
#144329=CARTESIAN_POINT('Ctrl Pts',(-0.749999999999964,-55.0621625368994,
-95.581761778993));
#144330=CARTESIAN_POINT('Ctrl Pts',(-0.749999999999971,-55.5033748716332,
-95.7875912885257));
#144331=CARTESIAN_POINT('Ctrl Pts',(-1.23837727019305,-60.4501569855996,
-84.0013918846235));
#144332=CARTESIAN_POINT('Ctrl Pts',(-0.750000000108156,-60.4692939396047,
-83.9872370540609));
#144333=CARTESIAN_POINT('Ctrl Pts',(-0.749999999999969,-60.9031648374056,
-84.2127012585751));
#144334=CARTESIAN_POINT('Ctrl Pts',(-1.23947201783252,-65.8492492116834,
-72.4261878753526));
#144335=CARTESIAN_POINT('Ctrl Pts',(-0.749999999981978,-65.8633206076967,
-72.4204079747872));
#144336=CARTESIAN_POINT('Ctrl Pts',(-0.749999999999967,-66.3022815738571,
-72.6374971882577));
#144337=CARTESIAN_POINT('Ctrl Pts',(-1.24035792914739,-71.2481103336038,
-60.8508735991007));
#144338=CARTESIAN_POINT('Ctrl Pts',(-0.749999999999965,-71.2566817467536,
-60.8548714197835));
#144339=CARTESIAN_POINT('Ctrl Pts',(-0.749999999999965,-71.701161634982,
-61.062182729971));
#144340=CARTESIAN_POINT('Origin',(-1.24999999999997,-55.5033748716332,-95.7875912885257));
#144341=CARTESIAN_POINT('Ctrl Pts',(-1.24037635835043,-71.360635368318,
-171.449026400902));
#144342=CARTESIAN_POINT('Ctrl Pts',(-0.749999999999976,-71.3691907154172,
-171.445036077089));
#144343=CARTESIAN_POINT('Ctrl Pts',(-0.749999999999965,-71.813687061541,
-171.237717270032));
#144344=CARTESIAN_POINT('Ctrl Pts',(-1.23948769887611,-65.9242696435089,
-159.793291324051));
#144345=CARTESIAN_POINT('Ctrl Pts',(-0.74999999977637,-65.9383759687714,
-159.799181671811));
#144346=CARTESIAN_POINT('Ctrl Pts',(-0.749999999999967,-66.3773023734559,
-159.58198200727));
#144347=CARTESIAN_POINT('Ctrl Pts',(-1.23838899982829,-60.4876714538986,
-148.137667147083));
#144348=CARTESIAN_POINT('Ctrl Pts',(-0.749999999843541,-60.5069208340151,
-148.152089356292));
#144349=CARTESIAN_POINT('Ctrl Pts',(-0.74999999999997,-60.9406796476674,
-147.926357767621));
#144350=CARTESIAN_POINT('Ctrl Pts',(-1.23668893165476,-55.0504165218146,
-136.482360813851));
#144351=CARTESIAN_POINT('Ctrl Pts',(-0.749999999999973,-55.0621625368995,
-136.476881192513));
#144352=CARTESIAN_POINT('Ctrl Pts',(-0.749999999999973,-55.5033748716332,
-136.27105168298));
#144353=CARTESIAN_POINT('Origin',(-1.24999999999997,-55.5033748716332,-136.27105168298));
#144354=CARTESIAN_POINT('Ctrl Pts',(-0.749999999999973,-55.08000002,-134.362052670054));
#144355=CARTESIAN_POINT('Ctrl Pts',(-0.749999999999966,-54.5800000199999,
-134.362052670054));
#144356=CARTESIAN_POINT('Ctrl Pts',(-1.24999999999997,-54.58000002,-134.362052670054));
#144357=CARTESIAN_POINT('Ctrl Pts',(-0.749999999999973,-55.0800000255278,
-135.020977206459));
#144358=CARTESIAN_POINT('Ctrl Pts',(-0.750000000006689,-54.5841777042435,
-135.09091556402));
#144359=CARTESIAN_POINT('Ctrl Pts',(-1.24580493030994,-54.58000002,-135.093949837831));
#144360=CARTESIAN_POINT('Ctrl Pts',(-0.749999999999973,-55.2219738253108,
-135.667845593964));
#144361=CARTESIAN_POINT('Ctrl Pts',(-0.74999999999389,-54.744924951658,
-135.807520949259));
#144362=CARTESIAN_POINT('Ctrl Pts',(-1.24129514745974,-54.7377489917927,
-135.812422632741));
#144363=CARTESIAN_POINT('Ctrl Pts',(-0.749999999999973,-55.5033748716332,
-136.27105168298));
#144364=CARTESIAN_POINT('Ctrl Pts',(-0.749999999999978,-55.0621625368994,
-136.476881192513));
#144365=CARTESIAN_POINT('Ctrl Pts',(-1.23668893165479,-55.0504165218146,
-136.482360813851));
#144366=CARTESIAN_POINT('',(-1.2499999994373,-54.58000002,-134.362052687297));
#144367=CARTESIAN_POINT('Origin',(-1.24999999999997,-55.08000002,-134.362052670054));
#144368=CARTESIAN_POINT('Origin',(-1.23487154781912,-62.0135240636403,-133.822664549727));
#144369=CARTESIAN_POINT('Origin',(-1.24999999999997,-55.08000002,-55.24995));
#144370=CARTESIAN_POINT('',(-1.24999998181205,-54.5800000199982,-97.6965897229033));
#144371=CARTESIAN_POINT('Origin',(-1.24999999999997,-55.08000002,-97.6965903014517));
#144372=CARTESIAN_POINT('',(-1.24999999999997,-54.58000002,-134.339054731985));
#144373=CARTESIAN_POINT('Ctrl Pts',(-0.749999999999973,-55.5033748716332,
-95.7875912885257));
#144374=CARTESIAN_POINT('Ctrl Pts',(-0.749999999999967,-55.0621625368995,
-95.5817617789931));
#144375=CARTESIAN_POINT('Ctrl Pts',(-1.23668893165476,-55.0504165218147,
-95.5762821576554));
#144376=CARTESIAN_POINT('Ctrl Pts',(-0.749999999999973,-55.2248025687359,
-96.3847337445855));
#144377=CARTESIAN_POINT('Ctrl Pts',(-0.750000000004237,-54.7481304442385,
-96.2443585547261));
#144378=CARTESIAN_POINT('Ctrl Pts',(-1.24124884403065,-54.7408920390033,
-96.2394858776278));
#144379=CARTESIAN_POINT('Ctrl Pts',(-0.749999999999973,-55.0800000216326,
-97.0309759697293));
#144380=CARTESIAN_POINT('Ctrl Pts',(-0.75000000000672,-54.5842199033567,
-96.9603643458105));
#144381=CARTESIAN_POINT('Ctrl Pts',(-1.24576233955167,-54.58000002,-96.9572624945429));
#144382=CARTESIAN_POINT('Ctrl Pts',(-0.749999999999973,-55.08000002,-97.6965903014517));
#144383=CARTESIAN_POINT('Ctrl Pts',(-0.749999999999965,-54.5800000199999,
-97.6965903014516));
#144384=CARTESIAN_POINT('Ctrl Pts',(-1.25,-54.58000002,-97.6965903014517));
#144385=CARTESIAN_POINT('Origin',(-1.23485323729605,-62.0131682900771,-98.2327688037691));
#144386=CARTESIAN_POINT('Ctrl Pts',(-6.8604212943599,-55.1073456615429,
-94.3034047511324));
#144387=CARTESIAN_POINT('Ctrl Pts',(-7.2042299691157,-54.58000002,-95.3011321772634));
#144388=CARTESIAN_POINT('Ctrl Pts',(-7.58857520038279,-54.58000002,-96.4164960598359));
#144389=CARTESIAN_POINT('Ctrl Pts',(-5.93585888223459,-55.0918247516195,
-94.6548535475511));
#144390=CARTESIAN_POINT('Ctrl Pts',(-6.23607825680947,-54.580000019985,
-95.6541184528592));
#144391=CARTESIAN_POINT('Ctrl Pts',(-6.56867789944001,-54.58000002,-96.7679442920248));
#144392=CARTESIAN_POINT('Ctrl Pts',(-4.99263467931988,-55.0788453329258,
-94.9451426129372));
#144393=CARTESIAN_POINT('Ctrl Pts',(-5.24614565799262,-54.58000002,-95.9461039187036));
#144394=CARTESIAN_POINT('Ctrl Pts',(-5.52653095835546,-54.58000002,-97.0582339217052));
#144395=CARTESIAN_POINT('Ctrl Pts',(-3.06075099962147,-55.0592467101081,
-95.3814216329573));
#144396=CARTESIAN_POINT('Ctrl Pts',(-3.21753929952213,-54.58000002,-96.3846721597723));
#144397=CARTESIAN_POINT('Ctrl Pts',(-3.38973164031852,-54.58000002,-97.4945129415963));
#144398=CARTESIAN_POINT('Ctrl Pts',(-2.0669285329079,-55.052711592208,-95.5256220795631));
#144399=CARTESIAN_POINT('Ctrl Pts',(-2.17279343333145,-54.5800000200112,
-96.5297363078781));
#144400=CARTESIAN_POINT('Ctrl Pts',(-2.28937244057036,-54.58000002,-97.638711952094));
#144401=CARTESIAN_POINT('Ctrl Pts',(-1.09375770007614,-55.0499908864773,
-95.5856784364438));
#144402=CARTESIAN_POINT('Ctrl Pts',(-1.14972373305894,-54.5800000199999,
-96.5901184946094));
#144403=CARTESIAN_POINT('Ctrl Pts',(-1.21149627184771,-54.58000002,-97.6987697451473));
#144404=CARTESIAN_POINT('',(-6.9,-54.58000002,-96.6432622057672));
#144405=CARTESIAN_POINT('Ctrl Pts',(-6.9,-54.5800000200288,-96.6432622057672));
#144406=CARTESIAN_POINT('Ctrl Pts',(-6.49061970139217,-54.5800000200775,
-96.7718187571058));
#144407=CARTESIAN_POINT('Ctrl Pts',(-6.07861873660027,-54.5800000205753,
-96.8899526380548));
#144408=CARTESIAN_POINT('Ctrl Pts',(-5.66396816650188,-54.5800000217474,
-96.9971605311361));
#144409=CARTESIAN_POINT('Ctrl Pts',(-5.26447645459909,-54.5800000228767,
-97.100449101863));
#144410=CARTESIAN_POINT('Ctrl Pts',(-4.86252531660949,-54.5800000241933,
-97.1935960044572));
#144411=CARTESIAN_POINT('Ctrl Pts',(-4.45809517257588,-54.5800000232613,
-97.2761964906685));
#144412=CARTESIAN_POINT('Ctrl Pts',(-4.34240961804981,-54.5800000229947,
-97.2998240149577));
#144413=CARTESIAN_POINT('Ctrl Pts',(-4.22645442245894,-54.5800000225654,
-97.3225679069059));
#144414=CARTESIAN_POINT('Ctrl Pts',(-4.1103033922506,-54.5800000220553,
-97.3444205163838));
#144415=CARTESIAN_POINT('Ctrl Pts',(-3.87438492650358,-54.5800000210192,
-97.3888061244265));
#144416=CARTESIAN_POINT('Ctrl Pts',(-3.63765702198839,-54.580000020604,
-97.4294862943975));
#144417=CARTESIAN_POINT('Ctrl Pts',(-3.4002729301617,-54.5800000203617,
-97.466451043988));
#144418=CARTESIAN_POINT('Ctrl Pts',(-3.16793216733923,-54.5800000201245,
-97.502630461283));
#144419=CARTESIAN_POINT('Ctrl Pts',(-2.93496148468305,-54.5800000200661,
-97.5352507112809));
#144420=CARTESIAN_POINT('Ctrl Pts',(-2.70149448625264,-54.5800000200335,
-97.5642527645727));
#144421=CARTESIAN_POINT('Ctrl Pts',(-2.47413670468755,-54.5800000200018,
-97.5924959104631));
#144422=CARTESIAN_POINT('Ctrl Pts',(-2.24630713852154,-54.580000020002,
-97.617307762456));
#144423=CARTESIAN_POINT('Ctrl Pts',(-2.01813705515799,-54.5800000200007,
-97.6385856637395));
#144424=CARTESIAN_POINT('Ctrl Pts',(-1.80087152563782,-54.5800000199995,
-97.6588466656259));
#144425=CARTESIAN_POINT('Ctrl Pts',(-1.5832964702307,-54.58000002,-97.6759032884734));
#144426=CARTESIAN_POINT('Ctrl Pts',(-1.36554569823268,-54.58000002,-97.6896238013577));
#144427=CARTESIAN_POINT('Ctrl Pts',(-1.32703559408406,-54.58000002,-97.6920503295178));
#144428=CARTESIAN_POINT('Ctrl Pts',(-1.28852006462875,-54.58000002,-97.6943724020827));
#144429=CARTESIAN_POINT('Ctrl Pts',(-1.24999994858807,-54.58000002,-97.6965891455738));
#144430=CARTESIAN_POINT('Ctrl Pts',(-6.9,-54.58000002,-96.6432622057672));
#144431=CARTESIAN_POINT('Ctrl Pts',(-6.8883412776675,-54.58000002,-96.2390470799649));
#144432=CARTESIAN_POINT('Ctrl Pts',(-6.87644795534686,-54.6248256750472,
-95.842546745885));
#144433=CARTESIAN_POINT('Ctrl Pts',(-6.86432673276943,-54.7125511587359,
-95.4535552447955));
#144434=CARTESIAN_POINT('Ctrl Pts',(-6.85220551051008,-54.8002766401224,
-95.0645637539141));
#144435=CARTESIAN_POINT('Ctrl Pts',(-6.83977061823003,-54.9324757175662,
-94.6806963775948));
#144436=CARTESIAN_POINT('Ctrl Pts',(-6.82752390201859,-55.1067945974843,
-94.3158809892684));
#144437=CARTESIAN_POINT('Ctrl Pts',(-6.84677576889373,-70.8578246683297,
-60.8508735991007));
#144438=CARTESIAN_POINT('Ctrl Pts',(-7.39999999999997,-70.8042142666047,
-60.8257004209668));
#144439=CARTESIAN_POINT('Ctrl Pts',(-7.4,-71.3078420373655,-61.0621827299711));
#144440=CARTESIAN_POINT('Ctrl Pts',(-6.84206094040904,-65.61805576689,-72.0110063808198));
#144441=CARTESIAN_POINT('Ctrl Pts',(-7.39999999999996,-65.5311408351844,
-72.0430210271706));
#144442=CARTESIAN_POINT('Ctrl Pts',(-7.4,-66.0675133276181,-72.2223201517098));
#144443=CARTESIAN_POINT('Ctrl Pts',(-6.83625690025051,-60.3715570323219,
-83.1679040708394));
#144444=CARTESIAN_POINT('Ctrl Pts',(-7.39999999995234,-60.2531402990131,
-83.2491486934777));
#144445=CARTESIAN_POINT('Ctrl Pts',(-7.4,-60.8202894597531,-83.3792196747323));
#144446=CARTESIAN_POINT('Ctrl Pts',(-6.82752390105444,-55.106794611208,
-94.3158809605474));
#144447=CARTESIAN_POINT('Ctrl Pts',(-7.39999999999997,-55.0309624818203,
-94.2800587259558));
#144448=CARTESIAN_POINT('Ctrl Pts',(-7.4,-55.5541151520872,-94.5271900914177));
#144449=CARTESIAN_POINT('Origin',(-6.9,-55.5541151520872,-94.5271900914178));
#144450=CARTESIAN_POINT('Ctrl Pts',(-7.4,-55.08000002,-96.6432622057672));
#144451=CARTESIAN_POINT('Ctrl Pts',(-7.39999999999996,-54.58000002,-96.6432622057672));
#144452=CARTESIAN_POINT('Ctrl Pts',(-6.9,-54.58000002,-96.6432622057672));
#144453=CARTESIAN_POINT('Ctrl Pts',(-7.4,-55.0800000228223,-96.276173584436));
#144454=CARTESIAN_POINT('Ctrl Pts',(-7.39999999999997,-54.5682037738145,
-96.2342789461818));
#144455=CARTESIAN_POINT('Ctrl Pts',(-6.8883412776675,-54.58000002,-96.2390470799649));
#144456=CARTESIAN_POINT('Ctrl Pts',(-7.4,-55.1203431091477,-95.9158883524807));
#144457=CARTESIAN_POINT('Ctrl Pts',(-7.39999999999997,-54.6014014206736,
-95.8348803330818));
#144458=CARTESIAN_POINT('Ctrl Pts',(-6.87644795534686,-54.6248256750472,
-95.842546745885));
#144459=CARTESIAN_POINT('Ctrl Pts',(-7.4,-55.2782489805768,-95.2085406483778));
#144460=CARTESIAN_POINT('Ctrl Pts',(-7.39999999999995,-54.7508604913788,
-95.0452270964761));
#144461=CARTESIAN_POINT('Ctrl Pts',(-6.85220551019199,-54.8002766424245,
-95.064563743706));
#144462=CARTESIAN_POINT('Ctrl Pts',(-7.4,-55.3972278356279,-94.8593050327909));
#144463=CARTESIAN_POINT('Ctrl Pts',(-7.39999999999369,-54.8709621105524,
-94.6521767160421));
#144464=CARTESIAN_POINT('Ctrl Pts',(-6.83977061757738,-54.9324757245047,
-94.6806963574476));
#144465=CARTESIAN_POINT('Ctrl Pts',(-7.4,-55.5541151520872,-94.5271900914177));
#144466=CARTESIAN_POINT('Ctrl Pts',(-7.39999999999997,-55.0309624818203,
-94.2800587259558));
#144467=CARTESIAN_POINT('Ctrl Pts',(-6.82752390105444,-55.106794611208,
-94.3158809605474));
#144468=CARTESIAN_POINT('Origin',(-6.9,-55.08000002,-96.6432622057672));
#144469=CARTESIAN_POINT('Origin',(-6.9,-55.08000002,-55.24995));
#144470=CARTESIAN_POINT('',(-6.9,-54.58000002,-135.415380765739));
#144471=CARTESIAN_POINT('Origin',(-6.9,-55.08000002,-135.415380765739));
#144472=CARTESIAN_POINT('',(-6.9,-54.58000002,-96.4806904787158));
#144473=CARTESIAN_POINT('Ctrl Pts',(-7.4,-55.569842315739,-137.564432008667));
#144474=CARTESIAN_POINT('Ctrl Pts',(-7.40000000000011,-55.0472163216404,
-137.816090401511));
#144475=CARTESIAN_POINT('Ctrl Pts',(-6.82627940990429,-55.1242727612674,
-137.778985645859));
#144476=CARTESIAN_POINT('Ctrl Pts',(-7.4,-55.4051297298433,-137.222270602494));
#144477=CARTESIAN_POINT('Ctrl Pts',(-7.39999999999862,-54.8790351803965,
-137.432659902946));
#144478=CARTESIAN_POINT('Ctrl Pts',(-6.8389262967378,-54.941259203202,-137.403152734529));
#144479=CARTESIAN_POINT('Ctrl Pts',(-7.4,-55.2827981883505,-136.868178474904));
#144480=CARTESIAN_POINT('Ctrl Pts',(-7.39999999999997,-54.7552910012621,
-137.033997183801));
#144481=CARTESIAN_POINT('Ctrl Pts',(-6.85155371766594,-54.805333739172,
-137.013956482872));
#144482=CARTESIAN_POINT('Ctrl Pts',(-7.4,-55.1186770997702,-136.137553696396));
#144483=CARTESIAN_POINT('Ctrl Pts',(-7.39999999999997,-54.5997930545306,
-136.218266932015));
#144484=CARTESIAN_POINT('Ctrl Pts',(-6.87660583005939,-54.6229757043942,
-136.210378498132));
#144485=CARTESIAN_POINT('Ctrl Pts',(-7.4,-55.0773024992163,-135.758275388548));
#144486=CARTESIAN_POINT('Ctrl Pts',(-7.40000000000133,-54.5659876123841,
-135.797876258651));
#144487=CARTESIAN_POINT('Ctrl Pts',(-6.88911403108312,-54.5770033281604,
-135.792971583838));
#144488=CARTESIAN_POINT('Ctrl Pts',(-7.4,-55.0801363807228,-135.378851871089));
#144489=CARTESIAN_POINT('Ctrl Pts',(-7.39999999999985,-54.581282028365,
-135.375165330398));
#144490=CARTESIAN_POINT('Ctrl Pts',(-6.90113321290139,-54.5801514737049,
-135.375156474088));
#144491=CARTESIAN_POINT('Origin',(-6.9,-55.5541151520872,-137.531452880088));
#144492=CARTESIAN_POINT('Ctrl Pts',(-6.82752391167578,-55.1067946098897,
-137.742761979991));
#144493=CARTESIAN_POINT('Ctrl Pts',(-6.83099153048951,-55.0574368043954,
-137.639465676912));
#144494=CARTESIAN_POINT('Ctrl Pts',(-6.83446840923335,-55.0116501943323,
-137.535137214437));
#144495=CARTESIAN_POINT('Ctrl Pts',(-6.83793753742844,-54.9693403128155,
-137.429833297904));
#144496=CARTESIAN_POINT('Ctrl Pts',(-6.84144322128202,-54.9265845943354,
-137.323419749845));
#144497=CARTESIAN_POINT('Ctrl Pts',(-6.84494129126791,-54.887378543277,
-137.216009330928));
#144498=CARTESIAN_POINT('Ctrl Pts',(-6.84842852672726,-54.851659632403,
-137.10762244633));
#144499=CARTESIAN_POINT('Ctrl Pts',(-6.85194224941648,-54.8156694192284,
-136.998412311235));
#144500=CARTESIAN_POINT('Ctrl Pts',(-6.85544530921929,-54.7832189819739,
-136.888209905991));
#144501=CARTESIAN_POINT('Ctrl Pts',(-6.85894403334902,-54.7542891926763,
-136.777010277306));
#144502=CARTESIAN_POINT('Ctrl Pts',(-6.86066524620696,-54.7400570544824,
-136.72230512663));
#144503=CARTESIAN_POINT('Ctrl Pts',(-6.86238552435822,-54.7266777157171,
-136.667358321512));
#144504=CARTESIAN_POINT('Ctrl Pts',(-6.86410608128596,-54.7141533541175,
-136.612168082043));
#144505=CARTESIAN_POINT('Ctrl Pts',(-6.86788574855968,-54.686640216424,
-136.490927837918));
#144506=CARTESIAN_POINT('Ctrl Pts',(-6.8716696820525,-54.6632062886195,
-136.368281734253));
#144507=CARTESIAN_POINT('Ctrl Pts',(-6.87543688800749,-54.6440113887563,
-136.244623751257));
#144508=CARTESIAN_POINT('Ctrl Pts',(-6.87918616660092,-54.6249078334902,
-136.121554231276));
#144509=CARTESIAN_POINT('Ctrl Pts',(-6.88291869407914,-54.6100032909578,
-135.997482854682));
#144510=CARTESIAN_POINT('Ctrl Pts',(-6.88662022495319,-54.5994096525472,
-135.872820988136));
#144511=CARTESIAN_POINT('Ctrl Pts',(-6.89030244377386,-54.5888712844875,
-135.748809521845));
#144512=CARTESIAN_POINT('Ctrl Pts',(-6.8939538237197,-54.5825991054037,
-135.624214165788));
#144513=CARTESIAN_POINT('Ctrl Pts',(-6.89756933233812,-54.5806551119451,
-135.499456180952));
#144514=CARTESIAN_POINT('Ctrl Pts',(-6.89838131639757,-54.5802185228322,
-135.471437579514));
#144515=CARTESIAN_POINT('Ctrl Pts',(-6.89919153278588,-54.580000040183,
-135.443410824955));
#144516=CARTESIAN_POINT('Ctrl Pts',(-6.9,-54.5800000200014,-135.415380765739));
#144517=CARTESIAN_POINT('Ctrl Pts',(-6.82752390105444,-55.106794611208,
-137.742762010959));
#144518=CARTESIAN_POINT('Ctrl Pts',(-7.39999999999997,-55.0309624818203,
-137.77858424555));
#144519=CARTESIAN_POINT('Ctrl Pts',(-7.4,-55.5541151520872,-137.531452880088));
#144520=CARTESIAN_POINT('Ctrl Pts',(-6.83631982946675,-60.4094944461354,
-148.971070239217));
#144521=CARTESIAN_POINT('Ctrl Pts',(-7.39999999999996,-60.2903951615484,
-148.888188464867));
#144522=CARTESIAN_POINT('Ctrl Pts',(-7.4,-60.858236996045,-148.759754479668));
#144523=CARTESIAN_POINT('Ctrl Pts',(-6.84214680798085,-65.6936814170396,
-160.208420694715));
#144524=CARTESIAN_POINT('Ctrl Pts',(-7.40000000024359,-65.6065688428949,
-160.175729571892));
#144525=CARTESIAN_POINT('Ctrl Pts',(-7.4,-66.1431501582269,-159.997106821727));
#144526=CARTESIAN_POINT('Ctrl Pts',(-6.84687749809456,-70.9710952348089,
-171.449026400902));
#144527=CARTESIAN_POINT('Ctrl Pts',(-7.39999999999995,-70.9175980522951,
-171.474145745141));
#144528=CARTESIAN_POINT('Ctrl Pts',(-7.4,-71.4211246238516,-171.237717270032));
#144529=CARTESIAN_POINT('Origin',(-7.9,-72.58000002,-55.24995));
#144530=CARTESIAN_POINT('',(-7.9,-73.08000002,-174.491325336599));
#144531=CARTESIAN_POINT('Origin',(3.54807775957937E-14,-73.08000002,3.11172719585489E-30));
#144532=CARTESIAN_POINT('',(-8.4,-73.08000002,-58.1922197332626));
#144533=CARTESIAN_POINT('Origin',(-8.4,-72.58000002,-55.24995));
#144534=CARTESIAN_POINT('Ctrl Pts',(-9.30242220787995,-55.1547652726018,
-93.2181494891395));
#144535=CARTESIAN_POINT('Ctrl Pts',(-8.89999999999997,-55.2270244231188,
-93.2526539147005));
#144536=CARTESIAN_POINT('Ctrl Pts',(-8.9,-55.5972887473416,-93.4294586200098));
#144537=CARTESIAN_POINT('Ctrl Pts',(-9.31365506854171,-60.298307210959,
-82.4413594877101));
#144538=CARTESIAN_POINT('Ctrl Pts',(-8.89999999981176,-60.4125449242165,
-82.3706902717217));
#144539=CARTESIAN_POINT('Ctrl Pts',(-8.9,-60.7433024895534,-82.6526792495127));
#144540=CARTESIAN_POINT('Ctrl Pts',(-9.32127686740287,-65.4102595335587,
-71.6490160146723));
#144541=CARTESIAN_POINT('Ctrl Pts',(-8.89999999999997,-65.4986935712713,
-71.6191417519029));
#144542=CARTESIAN_POINT('Ctrl Pts',(-8.9,-65.8565639782118,-71.8603324984455));
#144543=CARTESIAN_POINT('Ctrl Pts',(-9.32749162718857,-70.5102313269446,
-60.8508735991008));
#144544=CARTESIAN_POINT('Ctrl Pts',(-8.89999999999996,-70.5668839574465,
-60.8776359696917));
#144545=CARTESIAN_POINT('Ctrl Pts',(-8.9,-70.9575466375288,-61.0621827299711));
#144546=CARTESIAN_POINT('Origin',(-9.4,-55.5972887473416,-93.4294586200098));
#144547=CARTESIAN_POINT('Ctrl Pts',(-9.3276302147955,-70.6241744288951,
-171.449026400902));
#144548=CARTESIAN_POINT('Ctrl Pts',(-8.89999999999996,-70.6807353060531,
-171.422308714525));
#144549=CARTESIAN_POINT('Ctrl Pts',(-8.9,-71.0715121820529,-171.237717270032));
#144550=CARTESIAN_POINT('Ctrl Pts',(-9.32139302491482,-65.48642588992,-160.570366012028));
#144551=CARTESIAN_POINT('Ctrl Pts',(-8.89999999999997,-65.5751008964372,
-160.600947379136));
#144552=CARTESIAN_POINT('Ctrl Pts',(-8.9,-65.932751045448,-160.359049360718));
#144553=CARTESIAN_POINT('Ctrl Pts',(-9.31373872503275,-60.3366136221522,
-149.697543381378));
#144554=CARTESIAN_POINT('Ctrl Pts',(-8.89999999996837,-60.4515277778623,
-149.769759336176));
#144555=CARTESIAN_POINT('Ctrl Pts',(-8.9,-60.7816272203214,-149.486223352848));
#144556=CARTESIAN_POINT('Ctrl Pts',(-9.30242220787994,-55.1547652725975,
-138.840493482357));
#144557=CARTESIAN_POINT('Ctrl Pts',(-8.89999999999998,-55.2270244231145,
-138.805989056796));
#144558=CARTESIAN_POINT('Ctrl Pts',(-8.9,-55.5972887473373,-138.629184351487));
#144559=CARTESIAN_POINT('Origin',(-9.4,-55.5972887473373,-138.629184351487));
#144560=CARTESIAN_POINT('Ctrl Pts',(-8.9,-55.0800615856017,-136.31269455866));
#144561=CARTESIAN_POINT('Ctrl Pts',(-8.89999999999949,-54.5790205502306,
-136.310262631249));
#144562=CARTESIAN_POINT('Ctrl Pts',(-9.40104578491443,-54.580068463696,
-136.310267776416));
#144563=CARTESIAN_POINT('Ctrl Pts',(-8.9,-55.0781191191466,-136.719181715364));
#144564=CARTESIAN_POINT('Ctrl Pts',(-8.90000000000701,-54.5929085780248,
-136.748100743102));
#144565=CARTESIAN_POINT('Ctrl Pts',(-9.38483903200563,-54.5779095798998,
-136.755056625822));
#144566=CARTESIAN_POINT('Ctrl Pts',(-8.9,-55.1221566249649,-137.117922857594));
#144567=CARTESIAN_POINT('Ctrl Pts',(-8.90000000000104,-54.6552983120157,
-137.181065343466));
#144568=CARTESIAN_POINT('Ctrl Pts',(-9.36838029157539,-54.6268396387186,
-137.190977807678));
#144569=CARTESIAN_POINT('Ctrl Pts',(-8.9,-55.2980260549037,-137.900349863317));
#144570=CARTESIAN_POINT('Ctrl Pts',(-8.89999999999895,-54.8759793513846,
-138.023440966196));
#144571=CARTESIAN_POINT('Ctrl Pts',(-9.33501744196278,-54.8222491183721,
-138.045571332617));
#144572=CARTESIAN_POINT('Ctrl Pts',(-8.9,-55.4315173683664,-138.286573753949));
#144573=CARTESIAN_POINT('Ctrl Pts',(-8.89999999999893,-55.0334227401566,
-138.436762949154));
#144574=CARTESIAN_POINT('Ctrl Pts',(-9.31799140452363,-54.9705730458312,
-138.46700628841));
#144575=CARTESIAN_POINT('Ctrl Pts',(-8.9,-55.6084336906355,-138.652375441382));
#144576=CARTESIAN_POINT('Ctrl Pts',(-8.90000000000005,-55.2398419057005,
-138.830621016037));
#144577=CARTESIAN_POINT('Ctrl Pts',(-9.30138592606904,-55.1671456462707,
-138.865776623046));
#144578=CARTESIAN_POINT('',(-9.4,-54.58000002,-136.338455187671));
#144579=CARTESIAN_POINT('Origin',(-9.4,-55.08000002,-136.338455187671));
#144580=CARTESIAN_POINT('Ctrl Pts',(-9.4,-54.58000002,-136.338455187671));
#144581=CARTESIAN_POINT('Ctrl Pts',(-9.39568379879652,-54.5800000235886,
-136.456736569618));
#144582=CARTESIAN_POINT('Ctrl Pts',(-9.39134381256866,-54.5836651351887,
-136.574405163223));
#144583=CARTESIAN_POINT('Ctrl Pts',(-9.3869894402585,-54.5908887409915,
-136.691443516044));
#144584=CARTESIAN_POINT('Ctrl Pts',(-9.38259558962493,-54.5981778386323,
-136.809542981149));
#144585=CARTESIAN_POINT('Ctrl Pts',(-9.37818673013582,-54.6090898788391,
-136.927001658915));
#144586=CARTESIAN_POINT('Ctrl Pts',(-9.37376332616986,-54.6235628810459,
-137.043824528223));
#144587=CARTESIAN_POINT('Ctrl Pts',(-9.36931395071144,-54.6381208597708,
-137.161333309172));
#144588=CARTESIAN_POINT('Ctrl Pts',(-9.36484943919976,-54.6562815979561,
-137.278199798939));
#144589=CARTESIAN_POINT('Ctrl Pts',(-9.3603669253627,-54.6780337583374,
-137.394437436029));
#144590=CARTESIAN_POINT('Ctrl Pts',(-9.35747954189939,-54.6920452774223,
-137.469311188425));
#144591=CARTESIAN_POINT('Ctrl Pts',(-9.35458463586583,-54.7075480263028,
-137.543924144405));
#144592=CARTESIAN_POINT('Ctrl Pts',(-9.35168199702453,-54.7245503765222,
-137.618278743991));
#144593=CARTESIAN_POINT('Ctrl Pts',(-9.346722739198,-54.7535994739144,-137.745316122767));
#144594=CARTESIAN_POINT('Ctrl Pts',(-9.34174931509111,-54.7870830771536,
-137.871831855925));
#144595=CARTESIAN_POINT('Ctrl Pts',(-9.33675902757907,-54.8249939643255,
-137.997389579686));
#144596=CARTESIAN_POINT('Ctrl Pts',(-9.33180868381611,-54.8626014014535,
-138.121942301993));
#144597=CARTESIAN_POINT('Ctrl Pts',(-9.32684197484257,-54.9045657752775,
-138.245551915827));
#144598=CARTESIAN_POINT('Ctrl Pts',(-9.32187694789394,-54.9508338578952,
-138.36778554022));
#144599=CARTESIAN_POINT('Ctrl Pts',(-9.31696142496181,-54.9966406225888,
-138.48880042896));
#144600=CARTESIAN_POINT('Ctrl Pts',(-9.31204783361034,-55.0466658539161,
-138.608466213002));
#144601=CARTESIAN_POINT('Ctrl Pts',(-9.30717021919832,-55.1008095430556,
-138.726361914857));
#144602=CARTESIAN_POINT('Ctrl Pts',(-9.30558887632612,-55.1183631521896,
-138.764584191577));
#144603=CARTESIAN_POINT('Ctrl Pts',(-9.30401142729987,-55.1363492545961,
-138.802620437397));
#144604=CARTESIAN_POINT('Ctrl Pts',(-9.30243932966332,-55.1547633023018,
-138.840456402819));
#144605=CARTESIAN_POINT('Origin',(-9.4,-55.08000002,-55.24995));
#144606=CARTESIAN_POINT('',(-9.4,-54.58000002,-95.7201877838351));
#144607=CARTESIAN_POINT('Origin',(-9.4,-55.08000002,-95.7201877838351));
#144608=CARTESIAN_POINT('',(-9.4,-54.58000002,-136.131917111522));
#144609=CARTESIAN_POINT('Ctrl Pts',(-8.9,-55.5972887473416,-93.4294586200098));
#144610=CARTESIAN_POINT('Ctrl Pts',(-8.89999999999997,-55.2270244231188,
-93.2526539147005));
#144611=CARTESIAN_POINT('Ctrl Pts',(-9.30242220787995,-55.1547652726018,
-93.2181494891395));
#144612=CARTESIAN_POINT('Ctrl Pts',(-8.9,-55.4259676862915,-93.7882391070165));
#144613=CARTESIAN_POINT('Ctrl Pts',(-8.90000000000102,-55.0269773455407,
-93.6389456903403));
#144614=CARTESIAN_POINT('Ctrl Pts',(-9.31868748160984,-54.9644104418147,
-93.609279542603));
#144615=CARTESIAN_POINT('Ctrl Pts',(-8.9,-55.2983039792949,-94.15951472994));
#144616=CARTESIAN_POINT('Ctrl Pts',(-8.90000000000064,-54.8762991189121,
-94.036294307786));
#144617=CARTESIAN_POINT('Ctrl Pts',(-9.33504644279423,-54.8225599750811,
-94.0144115846847));
#144618=CARTESIAN_POINT('Ctrl Pts',(-8.9,-55.1250790215096,-94.9253056568412));
#144619=CARTESIAN_POINT('Ctrl Pts',(-8.89999999999928,-54.6591463230926,
-94.8606734038326));
#144620=CARTESIAN_POINT('Ctrl Pts',(-9.36771205478627,-54.6300877991462,
-94.8508246266895));
#144621=CARTESIAN_POINT('Ctrl Pts',(-8.9,-55.0800000205144,-95.3226944715878));
#144622=CARTESIAN_POINT('Ctrl Pts',(-8.89999999999998,-54.5956237519515,
-95.2920343273126));
#144623=CARTESIAN_POINT('Ctrl Pts',(-9.38412882836456,-54.58000002,-95.28525344501));
#144624=CARTESIAN_POINT('Ctrl Pts',(-8.9,-55.08000002,-95.7201877838351));
#144625=CARTESIAN_POINT('Ctrl Pts',(-8.89999999999996,-54.58000002,-95.720187783835));
#144626=CARTESIAN_POINT('Ctrl Pts',(-9.4,-54.58000002,-95.7201877838351));
#144627=CARTESIAN_POINT('Ctrl Pts',(-9.30242220787995,-55.1547652726018,
-93.2181494891395));
#144628=CARTESIAN_POINT('Ctrl Pts',(-9.31868748160984,-54.9644104418147,
-93.609279542603));
#144629=CARTESIAN_POINT('Ctrl Pts',(-9.33504644279423,-54.8225599750811,
-94.0144115846847));
#144630=CARTESIAN_POINT('Ctrl Pts',(-9.36771205478627,-54.6300877991462,
-94.8508246266895));
#144631=CARTESIAN_POINT('Ctrl Pts',(-9.38412882836456,-54.58000002,-95.28525344501));
#144632=CARTESIAN_POINT('Ctrl Pts',(-9.4,-54.58000002,-95.7201877838351));
#144633=CARTESIAN_POINT('Ctrl Pts',(-14.9356335973474,-55.3065630170304,
-89.5821211232313));
#144634=CARTESIAN_POINT('Ctrl Pts',(-15.6303319911964,-54.58000002,-90.5558876551412));
#144635=CARTESIAN_POINT('Ctrl Pts',(-16.4431419066885,-54.58000002,-91.6952124319348));
#144636=CARTESIAN_POINT('Ctrl Pts',(-13.9221964884044,-55.2748268726715,
-90.3693030445756));
#144637=CARTESIAN_POINT('Ctrl Pts',(-14.580009345269,-54.5800000199812,
-91.3456221401381));
#144638=CARTESIAN_POINT('Ctrl Pts',(-15.339723951503,-54.58000002,-92.4824059293848));
#144639=CARTESIAN_POINT('Ctrl Pts',(-12.878461314285,-55.2441424314898,
-91.1126600131971));
#144640=CARTESIAN_POINT('Ctrl Pts',(-13.4941774039103,-54.58000002,-92.0929943757894));
#144641=CARTESIAN_POINT('Ctrl Pts',(-14.2000751633255,-54.58000002,-93.2257513219804));
#144642=CARTESIAN_POINT('Ctrl Pts',(-10.7089431339248,-55.1865276043544,
-92.4826203625704));
#144643=CARTESIAN_POINT('Ctrl Pts',(-11.232462400793,-54.58000002,-93.4698992380895));
#144644=CARTESIAN_POINT('Ctrl Pts',(-11.824167023199,-54.58000002,-94.5957116711942));
#144645=CARTESIAN_POINT('Ctrl Pts',(-9.60108129664725,-55.1600911541447,
-93.0975581705506));
#144646=CARTESIAN_POINT('Ctrl Pts',(-10.0749231938442,-54.5800000200141,
-94.0883976981553));
#144647=CARTESIAN_POINT('Ctrl Pts',(-10.607529289827,-54.58000002,-95.2106503240539));
#144648=CARTESIAN_POINT('Ctrl Pts',(-8.4637455188182,-55.1370659786207,
-93.6259289312743));
#144649=CARTESIAN_POINT('Ctrl Pts',(-8.88330761013172,-54.58000002,-94.6201459052405));
#144650=CARTESIAN_POINT('Ctrl Pts',(-9.35547542469517,-54.58000002,-95.7390202399778));
#144651=CARTESIAN_POINT('',(-15.05,-54.5800000203361,-92.6513075005872));
#144652=CARTESIAN_POINT('Ctrl Pts',(-15.05,-54.5800000213444,-92.6513075005872));
#144653=CARTESIAN_POINT('Ctrl Pts',(-14.7116749748798,-54.5800000217462,
-92.8742343330668));
#144654=CARTESIAN_POINT('Ctrl Pts',(-14.3706840440903,-54.5800000214065,
-93.0921200800074));
#144655=CARTESIAN_POINT('Ctrl Pts',(-14.0263093380871,-54.580000021009,
-93.3049061919424));
#144656=CARTESIAN_POINT('Ctrl Pts',(-13.6916633339156,-54.5800000206227,
-93.5116810243007));
#144657=CARTESIAN_POINT('Ctrl Pts',(-13.3538223587274,-54.5800000202949,
-93.7136406704415));
#144658=CARTESIAN_POINT('Ctrl Pts',(-13.0120992871415,-54.5800000201906,
-93.9106936784565));
#144659=CARTESIAN_POINT('Ctrl Pts',(-12.7734325857321,-54.5800000201177,
-94.0483197135013));
#144660=CARTESIAN_POINT('Ctrl Pts',(-12.5336633488411,-54.5800000201,-94.1830804413658));
#144661=CARTESIAN_POINT('Ctrl Pts',(-12.2925916871682,-54.5800000202013,
-94.3149150255473));
#144662=CARTESIAN_POINT('Ctrl Pts',(-11.7801234903736,-54.5800000204166,
-94.5951679228056));
#144663=CARTESIAN_POINT('Ctrl Pts',(-11.2613422805828,-54.5800000202694,
-94.8625400042015));
#144664=CARTESIAN_POINT('Ctrl Pts',(-10.7355463256442,-54.580000020136,
-95.115608977548));
#144665=CARTESIAN_POINT('Ctrl Pts',(-10.2954190750505,-54.5800000200243,
-95.3274450527468));
#144666=CARTESIAN_POINT('Ctrl Pts',(-9.85037652345821,-54.5800000200001,
-95.529258479393));
#144667=CARTESIAN_POINT('Ctrl Pts',(-9.4,-54.58000002,-95.7201877838351));
#144668=CARTESIAN_POINT('Ctrl Pts',(-15.05,-54.58000002,-92.6513075005872));
#144669=CARTESIAN_POINT('Ctrl Pts',(-15.024892260307,-54.5800000199942,
-92.1213653817233));
#144670=CARTESIAN_POINT('Ctrl Pts',(-14.9996997962388,-54.6413287797313,
-91.6021394176372));
#144671=CARTESIAN_POINT('Ctrl Pts',(-14.9493011641311,-54.8817452975028,
-90.5846126994908));
#144672=CARTESIAN_POINT('Ctrl Pts',(-14.9239041921259,-55.0632253928883,
-90.0827451820339));
#144673=CARTESIAN_POINT('Ctrl Pts',(-14.8995694550283,-55.3054345175152,
-89.6101049857472));
#144674=CARTESIAN_POINT('Ctrl Pts',(-14.9339094669349,-69.3159372152924,
-60.8508735991008));
#144675=CARTESIAN_POINT('Ctrl Pts',(-15.55,-69.1834807533182,-60.7869757488078));
#144676=CARTESIAN_POINT('Ctrl Pts',(-15.55,-69.753968537624,-61.0621827299711));
#144677=CARTESIAN_POINT('Ctrl Pts',(-14.9250579803326,-64.6843968356381,
-70.4566455899725));
#144678=CARTESIAN_POINT('Ctrl Pts',(-15.5499999999812,-64.4850428243905,
-70.4989618700373));
#144679=CARTESIAN_POINT('Ctrl Pts',(-15.55,-65.1200769667078,-70.6679657074144));
#144680=CARTESIAN_POINT('Ctrl Pts',(-14.9143624117001,-60.0265024281888,
-80.0493410623047));
#144681=CARTESIAN_POINT('Ctrl Pts',(-15.5500000002265,-59.7682625842489,
-80.1682572157014));
#144682=CARTESIAN_POINT('Ctrl Pts',(-15.55,-60.4591562379615,-80.2606677496439));
#144683=CARTESIAN_POINT('Ctrl Pts',(-14.8995694550282,-55.3054345175152,
-89.6101049857472));
#144684=CARTESIAN_POINT('Ctrl Pts',(-15.55,-55.1214867472491,-89.519172133185));
#144685=CARTESIAN_POINT('Ctrl Pts',(-15.55,-55.7328910677637,-89.8214141166175));
#144686=CARTESIAN_POINT('Origin',(-15.05,-55.7328910677637,-89.8214141166176));
#144687=CARTESIAN_POINT('Ctrl Pts',(-15.55,-55.08000002,-92.6513075005872));
#144688=CARTESIAN_POINT('Ctrl Pts',(-15.55,-54.5800000199999,-92.6513075005872));
#144689=CARTESIAN_POINT('Ctrl Pts',(-15.05,-54.58000002,-92.6513075005872));
#144690=CARTESIAN_POINT('Ctrl Pts',(-15.55,-55.0800000226551,-92.1594703795246));
#144691=CARTESIAN_POINT('Ctrl Pts',(-15.5499999999999,-54.5542439251598,
-92.1076806752376));
#144692=CARTESIAN_POINT('Ctrl Pts',(-15.024892260188,-54.58000002,-92.1213653817264));
#144693=CARTESIAN_POINT('Ctrl Pts',(-15.55,-55.1351959031758,-91.676922782688));
#144694=CARTESIAN_POINT('Ctrl Pts',(-15.5499999999983,-54.5897383680245,
-91.5814692358521));
#144695=CARTESIAN_POINT('Ctrl Pts',(-14.9996997961174,-54.6413287797427,
-91.6021394176417));
#144696=CARTESIAN_POINT('Ctrl Pts',(-15.55,-55.3515707703666,-90.7300471126767));
#144697=CARTESIAN_POINT('Ctrl Pts',(-15.5500000000017,-54.7672056222625,
-90.5350573580561));
#144698=CARTESIAN_POINT('Ctrl Pts',(-14.9493011640063,-54.8817452975266,
-90.5846126995011));
#144699=CARTESIAN_POINT('Ctrl Pts',(-15.55,-55.5149014993407,-90.2623845064693));
#144700=CARTESIAN_POINT('Ctrl Pts',(-15.5499999999938,-54.9184989239094,
-90.0093785901182));
#144701=CARTESIAN_POINT('Ctrl Pts',(-14.923904192,-55.0632253929174,-90.0827451820487));
#144702=CARTESIAN_POINT('Ctrl Pts',(-15.55,-55.7328910677637,-89.8214141166176));
#144703=CARTESIAN_POINT('Ctrl Pts',(-15.55,-55.121486747249,-89.5191721331851));
#144704=CARTESIAN_POINT('Ctrl Pts',(-14.8995694550282,-55.3054345175152,
-89.6101049857472));
#144705=CARTESIAN_POINT('Origin',(-15.05,-55.08000002,-92.6513075005872));
#144706=CARTESIAN_POINT('Origin',(-15.05,-55.08000002,-55.24995));
#144707=CARTESIAN_POINT('',(-15.05,-54.580000020672,-139.407335470919));
#144708=CARTESIAN_POINT('Origin',(-15.05,-55.08000002,-139.407335470919));
#144709=CARTESIAN_POINT('',(-15.05,-54.58000002,-92.3169104578858));
#144710=CARTESIAN_POINT('Ctrl Pts',(-15.55,-55.784673861554,-142.339558479678));
#144711=CARTESIAN_POINT('Ctrl Pts',(-15.5500000000003,-55.1714603843291,
-142.657475116176));
#144712=CARTESIAN_POINT('Ctrl Pts',(-14.8938285640752,-55.3629945164905,
-142.558190130607));
#144713=CARTESIAN_POINT('Ctrl Pts',(-15.55,-55.5401271863377,-141.867316731602));
#144714=CARTESIAN_POINT('Ctrl Pts',(-15.5499999999988,-54.9426861434529,
-142.132025071305));
#144715=CARTESIAN_POINT('Ctrl Pts',(-14.9199544375999,-55.0912805253495,
-142.052148874024));
#144716=CARTESIAN_POINT('Ctrl Pts',(-15.55,-55.362894042524,-141.374710914757));
#144717=CARTESIAN_POINT('Ctrl Pts',(-15.5499999999981,-54.7770460479369,
-141.577324726442));
#144718=CARTESIAN_POINT('Ctrl Pts',(-14.946753914001,-54.8943433954032,
-141.523569141345));
#144719=CARTESIAN_POINT('Ctrl Pts',(-15.55,-55.1280599014707,-140.353868077711));
#144720=CARTESIAN_POINT('Ctrl Pts',(-15.5500000000017,-54.5840535900085,
-140.448758797019));
#144721=CARTESIAN_POINT('Ctrl Pts',(-15.001105737931,-54.6334073692214,
-140.426579139991));
#144722=CARTESIAN_POINT('Ctrl Pts',(-15.55,-55.0715453714938,-139.821424819443));
#144723=CARTESIAN_POINT('Ctrl Pts',(-15.5499999999997,-54.5490322450014,
-139.868468877722));
#144724=CARTESIAN_POINT('Ctrl Pts',(-15.0288653188588,-54.5706093318628,
-139.853620894103));
#144725=CARTESIAN_POINT('Ctrl Pts',(-15.55,-55.0810227214706,-139.29316520423));
#144726=CARTESIAN_POINT('Ctrl Pts',(-15.55,-54.5868072552659,-139.284387084));
#144727=CARTESIAN_POINT('Ctrl Pts',(-15.0557386144632,-54.5811354380133,
-139.284304796475));
#144728=CARTESIAN_POINT('Origin',(-15.05,-55.7328910677637,-142.237228854888));
#144729=CARTESIAN_POINT('Ctrl Pts',(-14.8995696008973,-55.3054345059085,
-142.448537780858));
#144730=CARTESIAN_POINT('Ctrl Pts',(-14.9050869560101,-55.2505199530171,
-142.341378389044));
#144731=CARTESIAN_POINT('Ctrl Pts',(-14.9106657820154,-55.1989345061021,
-142.233184634051));
#144732=CARTESIAN_POINT('Ctrl Pts',(-14.916264781587,-55.1505541483133,
-142.124033611185));
#144733=CARTESIAN_POINT('Ctrl Pts',(-14.9220196156331,-55.1008272414598,
-142.011844636256));
#144734=CARTESIAN_POINT('Ctrl Pts',(-14.9277960872094,-55.0544854940107,
-141.898643995188));
#144735=CARTESIAN_POINT('Ctrl Pts',(-14.933578643377,-55.0114188364469,
-141.784475897057));
#144736=CARTESIAN_POINT('Ctrl Pts',(-14.9394267629822,-54.9678638830437,
-141.669013344923));
#144737=CARTESIAN_POINT('Ctrl Pts',(-14.94528159598,-54.9276580556282,-141.552560655841));
#144738=CARTESIAN_POINT('Ctrl Pts',(-14.9511502353055,-54.8907235501576,
-141.435131421174));
#144739=CARTESIAN_POINT('Ctrl Pts',(-14.9570741056195,-54.8534414463534,
-141.31659703549));
#144740=CARTESIAN_POINT('Ctrl Pts',(-14.9630125985182,-54.8194920355816,
-141.19706689485));
#144741=CARTESIAN_POINT('Ctrl Pts',(-14.9689885366562,-54.7888405203331,
-141.076532755565));
#144742=CARTESIAN_POINT('Ctrl Pts',(-14.9706613173099,-54.7802605684443,
-141.042792918966));
#144743=CARTESIAN_POINT('Ctrl Pts',(-14.9723370964144,-54.7719393157975,
-141.0089743197));
#144744=CARTESIAN_POINT('Ctrl Pts',(-14.974016496481,-54.7638766966098,
-140.975076596103));
#144745=CARTESIAN_POINT('Ctrl Pts',(-14.9812183326244,-54.7293014554678,
-140.829711679284));
#144746=CARTESIAN_POINT('Ctrl Pts',(-14.9884710425149,-54.6994331689373,
-140.68264626882));
#144747=CARTESIAN_POINT('Ctrl Pts',(-14.9957348293262,-54.6744372616794,
-140.534379348079));
#144748=CARTESIAN_POINT('Ctrl Pts',(-15.0029606082856,-54.6495721458076,
-140.386888235788));
#144749=CARTESIAN_POINT('Ctrl Pts',(-15.0101970249367,-54.6295286679905,
-140.238208426256));
#144750=CARTESIAN_POINT('Ctrl Pts',(-15.0174130265094,-54.6144231957733,
-140.088851404552));
#144751=CARTESIAN_POINT('Ctrl Pts',(-15.0245747584206,-54.5994313278638,
-139.940617657963));
#144752=CARTESIAN_POINT('Ctrl Pts',(-15.0317160929112,-54.5893035220428,
-139.791717139304));
#144753=CARTESIAN_POINT('Ctrl Pts',(-15.0388192449019,-54.5841064305008,
-139.642665710458));
#144754=CARTESIAN_POINT('Ctrl Pts',(-15.0425567571479,-54.5813718426295,
-139.564238338876));
#144755=CARTESIAN_POINT('Ctrl Pts',(-15.0462839352885,-54.5800015872439,
-139.485769424767));
#144756=CARTESIAN_POINT('Ctrl Pts',(-15.05,-54.5800000213439,-139.407335470919));
#144757=CARTESIAN_POINT('Ctrl Pts',(-14.8995694550282,-55.3054345175152,
-142.448537985759));
#144758=CARTESIAN_POINT('Ctrl Pts',(-15.55,-55.1214867472491,-142.539470838321));
#144759=CARTESIAN_POINT('Ctrl Pts',(-15.55,-55.7328910677637,-142.237228854888));
#144760=CARTESIAN_POINT('Ctrl Pts',(-14.9144862578123,-60.0660270491051,
-152.089344301479));
#144761=CARTESIAN_POINT('Ctrl Pts',(-15.5500000000456,-59.8063638088322,
-151.967058554268));
#144762=CARTESIAN_POINT('Ctrl Pts',(-15.55,-60.4987241912205,-151.878017105041));
#144763=CARTESIAN_POINT('Ctrl Pts',(-14.9252396269456,-64.7624344426112,
-161.762591659591));
#144764=CARTESIAN_POINT('Ctrl Pts',(-15.549999999915,-64.5626692295554,
-161.718722395353));
#144765=CARTESIAN_POINT('Ctrl Pts',(-15.55,-65.1981673386922,-161.551271258869));
#144766=CARTESIAN_POINT('Ctrl Pts',(-14.9341313545396,-69.4322546019743,
-171.449026400902));
#144767=CARTESIAN_POINT('Ctrl Pts',(-15.5499999999999,-69.3001099534342,
-171.51276528209));
#144768=CARTESIAN_POINT('Ctrl Pts',(-15.55,-69.870344670579,-171.237717270032));
#144769=CARTESIAN_POINT('Origin',(-16.05,-70.08000002,-174.34995));
#144770=CARTESIAN_POINT('',(-16.05,-73.08000002,-174.34995));
#144771=CARTESIAN_POINT('Origin',(-16.05,-72.58000002,-174.34995));
#144772=CARTESIAN_POINT('Origin',(-16.05,-70.08000002,-174.34995));
#144773=CARTESIAN_POINT('Origin',(-16.05,-72.58000002,-55.24995));
#144774=CARTESIAN_POINT('',(-16.05,-73.08000002,-58.24995));
#144775=CARTESIAN_POINT('Origin',(-16.05,-72.58000002,-58.24995));
#144776=CARTESIAN_POINT('',(-16.05,-73.08000002,-174.34995));
#144777=CARTESIAN_POINT('Origin',(-16.05,-70.08000002,-58.24995));
#144778=CARTESIAN_POINT('Origin',(-16.05,-70.08000002,-58.24995));
#144779=CARTESIAN_POINT('Origin',(3.3975957231091E-14,-70.08000002,-58.24995));
#144780=CARTESIAN_POINT('',(-16.55,-73.08000002,-58.24995));
#144781=CARTESIAN_POINT('Origin',(-16.55,-70.08000002,-58.24995));
#144782=CARTESIAN_POINT('',(41.5,-73.0800000199999,-58.24995));
#144783=CARTESIAN_POINT('Origin',(-16.55,-70.08000002,-58.24995));
#144784=CARTESIAN_POINT('Origin',(-16.55,-72.58000002,-58.24995));
#144785=CARTESIAN_POINT('Ctrl Pts',(-17.3782102443508,-55.3867109640818,
-87.5561378285247));
#144786=CARTESIAN_POINT('Ctrl Pts',(-17.0499999999999,-55.4939415516614,
-87.6101736986065));
#144787=CARTESIAN_POINT('Ctrl Pts',(-17.05,-55.8060398696737,-87.7674469593951));
#144788=CARTESIAN_POINT('Ctrl Pts',(-17.3935607753682,-59.8507835488919,
-78.6850032603101));
#144789=CARTESIAN_POINT('Ctrl Pts',(-17.0499999998605,-60.0039146247672,
-78.6330864204663));
#144790=CARTESIAN_POINT('Ctrl Pts',(-17.05,-60.2763921316847,-78.8963304394585));
#144791=CARTESIAN_POINT('Ctrl Pts',(-17.4050347595683,-64.2412639062053,
-69.7761086016325));
#144792=CARTESIAN_POINT('Ctrl Pts',(-17.0499999999316,-64.3705933782976,
-69.756601957739));
#144793=CARTESIAN_POINT('Ctrl Pts',(-17.05,-64.6707170319981,-69.9874285386638));
#144794=CARTESIAN_POINT('Ctrl Pts',(-17.4146253252297,-68.5993151180197,
-60.8508735991007));
#144795=CARTESIAN_POINT('Ctrl Pts',(-17.05,-68.6914563568371,-60.8958957033858));
#144796=CARTESIAN_POINT('Ctrl Pts',(-17.05,-69.0317756926871,-61.0621827299711));
#144797=CARTESIAN_POINT('Origin',(-17.55,-55.8060398696737,-87.7674469593951));
#144798=CARTESIAN_POINT('Ctrl Pts',(-17.4148840712406,-68.7171063154928,
-171.449026400902));
#144799=CARTESIAN_POINT('Ctrl Pts',(-17.0499999999999,-68.809126121555,
-171.404072041895));
#144800=CARTESIAN_POINT('Ctrl Pts',(-17.05,-69.1496478013716,-171.237717270032));
#144801=CARTESIAN_POINT('Ctrl Pts',(-17.4052437025222,-64.32043537753,-162.443049517833));
#144802=CARTESIAN_POINT('Ctrl Pts',(-17.05,-64.4501495263083,-162.463595694273));
#144803=CARTESIAN_POINT('Ctrl Pts',(-17.05,-64.7499600097223,-162.23172927942));
#144804=CARTESIAN_POINT('Ctrl Pts',(-17.393699089013,-59.8910064308848,
-153.453571789302));
#144805=CARTESIAN_POINT('Ctrl Pts',(-17.0500000000351,-60.0450216003852,
-153.507379856851));
#144806=CARTESIAN_POINT('Ctrl Pts',(-17.05,-60.3166713897233,-153.242244037967));
#144807=CARTESIAN_POINT('Ctrl Pts',(-17.3782102443508,-55.3867109640869,
-144.502505142991));
#144808=CARTESIAN_POINT('Ctrl Pts',(-17.05,-55.4939415516665,-144.448469272909));
#144809=CARTESIAN_POINT('Ctrl Pts',(-17.05,-55.8060398696787,-144.291196012121));
#144810=CARTESIAN_POINT('Origin',(-17.55,-55.8060398696787,-144.291196012121));
#144811=CARTESIAN_POINT('Ctrl Pts',(-17.05,-55.0805074616842,-141.090900894366));
#144812=CARTESIAN_POINT('Ctrl Pts',(-17.0499999999999,-54.575891747757,
-141.084786328764));
#144813=CARTESIAN_POINT('Ctrl Pts',(-17.5546323543766,-54.5805643956983,
-141.084837323443));
#144814=CARTESIAN_POINT('Ctrl Pts',(-17.05,-55.0737407427313,-141.662277194932));
#144815=CARTESIAN_POINT('Ctrl Pts',(-17.05,-54.5986790821796,-141.679101787038));
#144816=CARTESIAN_POINT('Ctrl Pts',(-17.5241509980515,-54.5730421239016,
-141.696718195611));
#144817=CARTESIAN_POINT('Ctrl Pts',(-17.05,-55.1346896361868,-142.222271907188));
#144818=CARTESIAN_POINT('Ctrl Pts',(-17.05,-54.6883224645955,-142.274289971467));
#144819=CARTESIAN_POINT('Ctrl Pts',(-17.493703373038,-54.6407602724392,
-142.295501749987));
#144820=CARTESIAN_POINT('Ctrl Pts',(-17.05,-55.3871982275049,-143.319730865885));
#144821=CARTESIAN_POINT('Ctrl Pts',(-17.05,-55.007218915137,-143.426193042337));
#144822=CARTESIAN_POINT('Ctrl Pts',(-17.4330935790494,-54.9213199751476,
-143.467340431406));
#144823=CARTESIAN_POINT('Ctrl Pts',(-17.05,-55.5814626759696,-143.861508336615));
#144824=CARTESIAN_POINT('Ctrl Pts',(-17.05,-55.2333139511105,-143.992542009422));
#144825=CARTESIAN_POINT('Ctrl Pts',(-17.4026795826987,-55.1371704105482,
-144.044980325084));
#144826=CARTESIAN_POINT('Ctrl Pts',(-17.05,-55.8450287809867,-144.367275073454));
#144827=CARTESIAN_POINT('Ctrl Pts',(-17.05,-55.5380988270127,-144.527216600776));
#144828=CARTESIAN_POINT('Ctrl Pts',(-17.3739345303265,-55.4300165573977,
-144.583528621283));
#144829=CARTESIAN_POINT('',(-17.55,-54.58000002,-141.176536909659));
#144830=CARTESIAN_POINT('Origin',(-17.55,-55.08000002,-141.176536909659));
#144831=CARTESIAN_POINT('Ctrl Pts',(-17.55,-54.58000002,-141.176536909659));
#144832=CARTESIAN_POINT('Ctrl Pts',(-17.5434039653577,-54.5800000265972,
-141.308685646377));
#144833=CARTESIAN_POINT('Ctrl Pts',(-17.5367960353516,-54.5835879338551,
-141.440239551843));
#144834=CARTESIAN_POINT('Ctrl Pts',(-17.5301956955585,-54.5906604912783,
-141.571176756649));
#144835=CARTESIAN_POINT('Ctrl Pts',(-17.5234840454982,-54.5978523225997,
-141.70432212887));
#144836=CARTESIAN_POINT('Ctrl Pts',(-17.5167797303469,-54.6086468223138,
-141.836830569671));
#144837=CARTESIAN_POINT('Ctrl Pts',(-17.5100862770427,-54.622980971367,
-141.968701840416));
#144838=CARTESIAN_POINT('Ctrl Pts',(-17.503372066993,-54.6373595713593,
-142.100982050807));
#144839=CARTESIAN_POINT('Ctrl Pts',(-17.4966681563516,-54.6552995984296,
-142.232621988595));
#144840=CARTESIAN_POINT('Ctrl Pts',(-17.4899699068517,-54.6767881709156,
-142.363631902612));
#144841=CARTESIAN_POINT('Ctrl Pts',(-17.4832987536179,-54.6981898162009,
-142.494111845403));
#144842=CARTESIAN_POINT('Ctrl Pts',(-17.4766325502404,-54.7231114151653,
-142.623967706529));
#144843=CARTESIAN_POINT('Ctrl Pts',(-17.4699683223166,-54.7515915027105,
-142.753207159389));
#144844=CARTESIAN_POINT('Ctrl Pts',(-17.4677609485311,-54.7610248833477,
-142.796014785954));
#144845=CARTESIAN_POINT('Ctrl Pts',(-17.465553848176,-54.7708490838071,
-142.838754709885));
#144846=CARTESIAN_POINT('Ctrl Pts',(-17.4633471473699,-54.7810667130108,
-142.881426904301));
#144847=CARTESIAN_POINT('Ctrl Pts',(-17.4557628915023,-54.8161838951985,
-143.02808785625));
#144848=CARTESIAN_POINT('Ctrl Pts',(-17.4482142625559,-54.8560016932433,
-143.174199894099));
#144849=CARTESIAN_POINT('Ctrl Pts',(-17.440677260134,-54.9005823896015,
-143.31931656486));
#144850=CARTESIAN_POINT('Ctrl Pts',(-17.4333152627617,-54.9441279467171,
-143.461063706365));
#144851=CARTESIAN_POINT('Ctrl Pts',(-17.4259644460376,-54.9922184111824,
-143.601861162394));
#144852=CARTESIAN_POINT('Ctrl Pts',(-17.4186373285509,-55.0448895417837,
-143.741267924584));
#144853=CARTESIAN_POINT('Ctrl Pts',(-17.4115478748488,-55.0958522215165,
-143.876152862365));
#144854=CARTESIAN_POINT('Ctrl Pts',(-17.4044808446839,-55.1511037543352,
-144.009735693423));
#144855=CARTESIAN_POINT('Ctrl Pts',(-17.3974781607216,-55.2106471239,-144.141594677413));
#144856=CARTESIAN_POINT('Ctrl Pts',(-17.3910063762535,-55.2656762893459,
-144.263456941818));
#144857=CARTESIAN_POINT('Ctrl Pts',(-17.3845899846665,-55.3243713219084,
-144.383846491428));
#144858=CARTESIAN_POINT('Ctrl Pts',(-17.3782835568631,-55.3867049962959,
-144.502414961715));
#144859=CARTESIAN_POINT('Origin',(-17.55,-55.08000002,-55.24995));
#144860=CARTESIAN_POINT('',(-17.55,-54.58000002,-90.8821060618472));
#144861=CARTESIAN_POINT('Origin',(-17.55,-55.08000002,-90.8821060618472));
#144862=CARTESIAN_POINT('',(-17.55,-54.58000002,-140.803447286915));
#144863=CARTESIAN_POINT('Ctrl Pts',(-17.05,-55.8060398696737,-87.7674469593951));
#144864=CARTESIAN_POINT('Ctrl Pts',(-17.0499999999999,-55.4939415516614,
-87.6101736986065));
#144865=CARTESIAN_POINT('Ctrl Pts',(-17.3782102443508,-55.3867109640818,
-87.5561378285247));
#144866=CARTESIAN_POINT('Ctrl Pts',(-17.05,-55.5622216475024,-88.2512880043934));
#144867=CARTESIAN_POINT('Ctrl Pts',(-17.05,-55.2114257865401,-88.1214372575005));
#144868=CARTESIAN_POINT('Ctrl Pts',(-17.4056693808345,-55.1158123847072,
-88.0713943440392));
#144869=CARTESIAN_POINT('Ctrl Pts',(-17.05,-55.3841798573999,-88.7556128927223));
#144870=CARTESIAN_POINT('Ctrl Pts',(-17.05,-55.0036171481024,-88.6486574682591));
#144871=CARTESIAN_POINT('Ctrl Pts',(-17.4339593787444,-54.9179776170691,
-88.6091505606876));
#144872=CARTESIAN_POINT('Ctrl Pts',(-17.05,-55.1424163647715,-89.7992759203947));
#144873=CARTESIAN_POINT('Ctrl Pts',(-17.0499999999999,-54.6987064687868,
-89.7439019899564));
#144874=CARTESIAN_POINT('Ctrl Pts',(-17.4916046269366,-54.6493515142325,
-89.7235249939138));
#144875=CARTESIAN_POINT('Ctrl Pts',(-17.05,-55.0800000196891,-90.3423386098486));
#144876=CARTESIAN_POINT('Ctrl Pts',(-17.0500000000018,-54.6080382399387,
-90.3203722819605));
#144877=CARTESIAN_POINT('Ctrl Pts',(-17.5211522384036,-54.58000002,-90.3041534556916));
#144878=CARTESIAN_POINT('Ctrl Pts',(-17.05,-55.08000002,-90.8821060618472));
#144879=CARTESIAN_POINT('Ctrl Pts',(-17.0499999999999,-54.58000002,-90.8821060618472));
#144880=CARTESIAN_POINT('Ctrl Pts',(-17.55,-54.58000002,-90.8821060618472));
#144881=CARTESIAN_POINT('Ctrl Pts',(-17.3782123830793,-55.3866898645837,
-87.5561779606742));
#144882=CARTESIAN_POINT('Ctrl Pts',(-17.4056708497953,-55.1158021121638,
-88.0714222670871));
#144883=CARTESIAN_POINT('Ctrl Pts',(-17.4339601270529,-54.9179741299611,
-88.6091650266831));
#144884=CARTESIAN_POINT('Ctrl Pts',(-17.4916046269366,-54.6493515142325,
-89.7235249939138));
#144885=CARTESIAN_POINT('Ctrl Pts',(-17.5211522384036,-54.58000002,-90.3041534556916));
#144886=CARTESIAN_POINT('Ctrl Pts',(-17.55,-54.58000002,-90.8821060618472));
#144887=CARTESIAN_POINT('Origin',(-16.55,-72.58000002,-55.24995));
#144888=CARTESIAN_POINT('',(-16.55,-73.08000002,-174.34995));
#144889=CARTESIAN_POINT('Origin',(-16.55,-72.58000002,-174.34995));
#144890=CARTESIAN_POINT('',(-16.55,-73.08000002,-58.24995));
#144891=CARTESIAN_POINT('Origin',(-16.55,-70.08000002,-174.34995));
#144892=CARTESIAN_POINT('Origin',(-16.55,-70.08000002,-174.34995));
#144893=CARTESIAN_POINT('Ctrl Pts',(-23.0246352694011,-55.592944139339,
-81.9685164608053));
#144894=CARTESIAN_POINT('Ctrl Pts',(-23.9800920467566,-54.58000002,-82.9059773201362));
#144895=CARTESIAN_POINT('Ctrl Pts',(-25.1782904241482,-54.58000002,-84.0816077695088));
#144896=CARTESIAN_POINT('Ctrl Pts',(-21.9095359072908,-55.5502317234241,
-83.1856130754768));
#144897=CARTESIAN_POINT('Ctrl Pts',(-22.8383173576717,-54.5800000199764,
-84.1257656115259));
#144898=CARTESIAN_POINT('Ctrl Pts',(-23.9841110090257,-54.58000002,-85.2987111873827));
#144899=CARTESIAN_POINT('Ctrl Pts',(-20.7596485158525,-55.5069863868931,
-84.3783409260868));
#144900=CARTESIAN_POINT('Ctrl Pts',(-21.6556870958812,-54.5800000200059,
-85.3242347169187));
#144901=CARTESIAN_POINT('Ctrl Pts',(-22.7486109694941,-54.58000002,-86.4914322348344));
#144902=CARTESIAN_POINT('Ctrl Pts',(-18.3831304802005,-55.4209867081881,
-86.677763648685));
#144903=CARTESIAN_POINT('Ctrl Pts',(-19.2046498564005,-54.580000019994,
-87.6346041928195));
#144904=CARTESIAN_POINT('Ctrl Pts',(-20.1853568720873,-54.58000002,-88.7908549573443));
#144905=CARTESIAN_POINT('Ctrl Pts',(-17.1656615705366,-55.378552771758,
-87.7759223265742));
#144906=CARTESIAN_POINT('Ctrl Pts',(-17.9458952665752,-54.5800000199822,
-88.7385064703248));
#144907=CARTESIAN_POINT('Ctrl Pts',(-18.8674767865624,-54.58000002,-89.8890267533221));
#144908=CARTESIAN_POINT('Ctrl Pts',(-15.908562035693,-55.3376387148139,
-88.8056746987062));
#144909=CARTESIAN_POINT('Ctrl Pts',(-16.6397068497462,-54.58000002,-89.7756104658071));
#144910=CARTESIAN_POINT('Ctrl Pts',(-17.501426021519,-54.58000002,-90.9187660074097));
#144911=CARTESIAN_POINT('',(-23.2,-54.58000002,-86.035464915697));
#144912=CARTESIAN_POINT('Ctrl Pts',(-23.2,-54.5800000205323,-86.035464915697));
#144913=CARTESIAN_POINT('Ctrl Pts',(-22.7416005579447,-54.5800000204569,
-86.47348855531));
#144914=CARTESIAN_POINT('Ctrl Pts',(-22.2778852067935,-54.580000020382,
-86.9061566639853));
#144915=CARTESIAN_POINT('Ctrl Pts',(-21.8082168238936,-54.5800000203146,
-87.3329667341744));
#144916=CARTESIAN_POINT('Ctrl Pts',(-21.6948114072064,-54.5800000202983,
-87.4360236475592));
#144917=CARTESIAN_POINT('Ctrl Pts',(-21.5810587192231,-54.5800000202825,
-87.5387388947569));
#144918=CARTESIAN_POINT('Ctrl Pts',(-21.4669494079306,-54.5800000202671,
-87.6411051232897));
#144919=CARTESIAN_POINT('Ctrl Pts',(-21.0322856597371,-54.5800000202087,
-88.0310372688657));
#144920=CARTESIAN_POINT('Ctrl Pts',(-20.593585201871,-54.5800000201577,
-88.4149271477262));
#144921=CARTESIAN_POINT('Ctrl Pts',(-20.1500339722446,-54.580000020117,
-88.7924150855441));
#144922=CARTESIAN_POINT('Ctrl Pts',(-19.7265254012931,-54.5800000200782,
-89.1528455531393));
#144923=CARTESIAN_POINT('Ctrl Pts',(-19.2985947426906,-54.5800000200487,
-89.507439867046));
#144924=CARTESIAN_POINT('Ctrl Pts',(-18.86550622925,-54.5800000200292,-89.8558463488877));
#144925=CARTESIAN_POINT('Ctrl Pts',(-18.4324177158093,-54.5800000200098,
-90.2042528307294));
#144926=CARTESIAN_POINT('Ctrl Pts',(-17.9941717501709,-54.5800000200003,
-90.5464720515007));
#144927=CARTESIAN_POINT('Ctrl Pts',(-17.55,-54.58000002,-90.8821060618472));
#144928=CARTESIAN_POINT('Ctrl Pts',(-23.2,-54.58000002,-86.035464915697));
#144929=CARTESIAN_POINT('Ctrl Pts',(-23.1631558847544,-54.5800000199942,
-85.3330272043352));
#144930=CARTESIAN_POINT('Ctrl Pts',(-23.1266268845704,-54.6631759768875,
-84.6443771511168));
#144931=CARTESIAN_POINT('Ctrl Pts',(-23.0544213837377,-54.9946392601494,
-83.2949364329151));
#144932=CARTESIAN_POINT('Ctrl Pts',(-23.0184485783994,-55.2464820492743,
-82.6288060065001));
#144933=CARTESIAN_POINT('Ctrl Pts',(-22.9849163124812,-55.5914230881085,
-82.0118419201864));
#144934=CARTESIAN_POINT('Ctrl Pts',(-23.0210431649761,-66.5230748737403,
-60.8508735991007));
#144935=CARTESIAN_POINT('Ctrl Pts',(-23.6999999999999,-66.2910081673095,
-60.7330850354506));
#144936=CARTESIAN_POINT('Ctrl Pts',(-23.7,-66.9393955463102,-61.0621827299711));
#144937=CARTESIAN_POINT('Ctrl Pts',(-23.0109831737233,-62.9327835325611,
-67.9329755599233));
#144938=CARTESIAN_POINT('Ctrl Pts',(-23.7000000000839,-62.6252669058498,
-67.9176543808627));
#144939=CARTESIAN_POINT('Ctrl Pts',(-23.7,-63.3447762129971,-68.1442919238122));
#144940=CARTESIAN_POINT('Ctrl Pts',(-22.9993168926453,-59.3018045077389,
-74.9936336228867));
#144941=CARTESIAN_POINT('Ctrl Pts',(-23.7000000000403,-58.9382045046749,
-75.0250759674623));
#144942=CARTESIAN_POINT('Ctrl Pts',(-23.7,-59.7084208561779,-75.2049556739983));
#144943=CARTESIAN_POINT('Ctrl Pts',(-22.9849163103247,-55.591423110293,
-82.011841880507));
#144944=CARTESIAN_POINT('Ctrl Pts',(-23.7,-55.290324925596,-81.8523243454179));
#144945=CARTESIAN_POINT('Ctrl Pts',(-23.7,-55.9902808012637,-82.2231510113773));
#144946=CARTESIAN_POINT('Origin',(-23.2,-55.9902808012638,-82.2231510113773));
#144947=CARTESIAN_POINT('Ctrl Pts',(-23.7,-55.08000002,-86.035464915697));
#144948=CARTESIAN_POINT('Ctrl Pts',(-23.7,-54.58000002,-86.0354649156969));
#144949=CARTESIAN_POINT('Ctrl Pts',(-23.2,-54.58000002,-86.035464915697));
#144950=CARTESIAN_POINT('Ctrl Pts',(-23.7,-55.0800000221098,-85.3715851430748));
#144951=CARTESIAN_POINT('Ctrl Pts',(-23.7,-54.5417374496194,-85.3059841364058));
#144952=CARTESIAN_POINT('Ctrl Pts',(-23.163155884673,-54.58000002,-85.3330272043393));
#144953=CARTESIAN_POINT('Ctrl Pts',(-23.7,-55.1548583802702,-84.7198400663338));
#144954=CARTESIAN_POINT('Ctrl Pts',(-23.6999999999999,-54.5866204760292,
-84.6055144627376));
#144955=CARTESIAN_POINT('Ctrl Pts',(-23.1266268844869,-54.6631759768986,
-84.6443771511225));
#144956=CARTESIAN_POINT('Ctrl Pts',(-23.7,-55.4531753402921,-83.4411601721359));
#144957=CARTESIAN_POINT('Ctrl Pts',(-23.7,-54.8153941542428,-83.2070098309739));
#144958=CARTESIAN_POINT('Ctrl Pts',(-23.054421382878,-54.9946392637262,
-83.2949364184621));
#144959=CARTESIAN_POINT('Ctrl Pts',(-23.7,-55.6798282904624,-82.8091473369244));
#144960=CARTESIAN_POINT('Ctrl Pts',(-23.7000000000021,-55.01791265188,-82.4979478032362));
#144961=CARTESIAN_POINT('Ctrl Pts',(-23.0184485767712,-55.2464820601011,
-82.6288059779555));
#144962=CARTESIAN_POINT('Ctrl Pts',(-23.7,-55.9902808012637,-82.2231510113773));
#144963=CARTESIAN_POINT('Ctrl Pts',(-23.7,-55.290324925596,-81.8523243454179));
#144964=CARTESIAN_POINT('Ctrl Pts',(-22.9849163103247,-55.591423110293,
-82.011841880507));
#144965=CARTESIAN_POINT('Origin',(-23.2,-55.08000002,-86.035464915697));
#144966=CARTESIAN_POINT('Origin',(-23.2,-55.08000002,-55.24995));
#144967=CARTESIAN_POINT('',(-23.2,-54.5800000202568,-146.023178055809));
#144968=CARTESIAN_POINT('Origin',(-23.2,-55.08000002,-146.023178055809));
#144969=CARTESIAN_POINT('',(-23.2,-54.58000002,-85.5535812563546));
#144970=CARTESIAN_POINT('Ctrl Pts',(-23.7,-56.1877984637886,-150.184170074209));
#144971=CARTESIAN_POINT('Ctrl Pts',(-23.7000000000058,-55.4758653944209,
-150.617415324691));
#144972=CARTESIAN_POINT('Ctrl Pts',(-22.9645964648804,-55.8110221483383,
-150.413695161775));
#144973=CARTESIAN_POINT('Ctrl Pts',(-23.7,-55.770760534689,-149.494224653333));
#144974=CARTESIAN_POINT('Ctrl Pts',(-23.6999999999915,-55.104992262177,
-149.853316450234));
#144975=CARTESIAN_POINT('Ctrl Pts',(-23.0041504913057,-55.3476739653898,
-149.687711142526));
#144976=CARTESIAN_POINT('Ctrl Pts',(-23.7,-55.4874608362993,-148.759183505398));
#144977=CARTESIAN_POINT('Ctrl Pts',(-23.6999999999971,-54.84406999352,-149.022400495565));
#144978=CARTESIAN_POINT('Ctrl Pts',(-23.0460611054753,-55.0328364107862,
-148.913176733992));
#144979=CARTESIAN_POINT('Ctrl Pts',(-23.7,-55.126303632832,-147.221582957655));
#144980=CARTESIAN_POINT('Ctrl Pts',(-23.7000000000026,-54.5663401762214,
-147.338490969714));
#144981=CARTESIAN_POINT('Ctrl Pts',(-23.132906798941,-54.6314878274362,
-147.290542781339));
#144982=CARTESIAN_POINT('Ctrl Pts',(-23.7,-55.0524032880678,-146.416006958094));
#144983=CARTESIAN_POINT('Ctrl Pts',(-23.699999999999,-54.5265437589966,
-146.473947688457));
#144984=CARTESIAN_POINT('Ctrl Pts',(-23.1780014932925,-54.5493513836785,
-146.439171475211));
#144985=CARTESIAN_POINT('Ctrl Pts',(-23.7,-55.0891865678663,-145.627934484655));
#144986=CARTESIAN_POINT('Ctrl Pts',(-23.7000000000002,-54.6108701043512,
-145.605394331135));
#144987=CARTESIAN_POINT('Ctrl Pts',(-23.2215734466188,-54.5901934669506,
-145.604851313073));
#144988=CARTESIAN_POINT('Origin',(-23.2,-55.9902808012637,-149.835491960129));
#144989=CARTESIAN_POINT('Ctrl Pts',(-22.9849164538399,-55.5914231005407,
-150.046800950003));
#144990=CARTESIAN_POINT('Ctrl Pts',(-22.9908372008831,-55.5305186315594,
-149.937866229653));
#144991=CARTESIAN_POINT('Ctrl Pts',(-22.9968799288713,-55.472742437367,
-149.827854316054));
#144992=CARTESIAN_POINT('Ctrl Pts',(-23.0029707306892,-55.4179474788907,
-149.716871524626));
#144993=CARTESIAN_POINT('Ctrl Pts',(-23.0091875113402,-55.3620191712851,
-149.603593225481));
#144994=CARTESIAN_POINT('Ctrl Pts',(-23.0154546055321,-55.3091959345735,
-149.489303295622));
#144995=CARTESIAN_POINT('Ctrl Pts',(-23.0217323073057,-55.2593300727596,
-149.374077739874));
#144996=CARTESIAN_POINT('Ctrl Pts',(-23.0281927026225,-55.2080130156976,
-149.255498892459));
#144997=CARTESIAN_POINT('Ctrl Pts',(-23.0346646369944,-55.1598271938812,
-149.135928921938));
#144998=CARTESIAN_POINT('Ctrl Pts',(-23.0411415414134,-55.1146326815648,
-149.015415012526));
#144999=CARTESIAN_POINT('Ctrl Pts',(-23.0477026343699,-55.0688507188787,
-148.893334631057));
#145000=CARTESIAN_POINT('Ctrl Pts',(-23.0542693270987,-55.0261376966006,
-148.770285167514));
#145001=CARTESIAN_POINT('Ctrl Pts',(-23.0608656006907,-54.98638023854,-148.646285053031));
#145002=CARTESIAN_POINT('Ctrl Pts',(-23.0675533958685,-54.9460711560571,
-148.520564469111));
#145003=CARTESIAN_POINT('Ctrl Pts',(-23.074272175774,-54.9087996853551,
-148.393866137308));
#145004=CARTESIAN_POINT('Ctrl Pts',(-23.0810701888432,-54.8744894117583,
-148.266185449915));
#145005=CARTESIAN_POINT('Ctrl Pts',(-23.0839762476771,-54.8598222328834,
-148.211603679368));
#145006=CARTESIAN_POINT('Ctrl Pts',(-23.0868970210003,-54.8456967589052,
-148.156842142755));
#145007=CARTESIAN_POINT('Ctrl Pts',(-23.089837136435,-54.8321096326547,
-148.101899565739));
#145008=CARTESIAN_POINT('Ctrl Pts',(-23.1005386667511,-54.7826547569155,
-147.901917739631));
#145009=CARTESIAN_POINT('Ctrl Pts',(-23.1113627267195,-54.7403626997578,
-147.699512147701));
#145010=CARTESIAN_POINT('Ctrl Pts',(-23.1222318129805,-54.7053520485838,
-147.495526029615));
#145011=CARTESIAN_POINT('Ctrl Pts',(-23.1332194694889,-54.6699594681963,
-147.289314638505));
#145012=CARTESIAN_POINT('Ctrl Pts',(-23.1442532408192,-54.642007812508,
-147.081487627851));
#145013=CARTESIAN_POINT('Ctrl Pts',(-23.155279897433,-54.6215740728526,
-146.872924136455));
#145014=CARTESIAN_POINT('Ctrl Pts',(-23.1661946839301,-54.6013476421687,
-146.666476610302));
#145015=CARTESIAN_POINT('Ctrl Pts',(-23.1771027123396,-54.588487337632,
-146.459307075042));
#145016=CARTESIAN_POINT('Ctrl Pts',(-23.1879759364348,-54.5830254173653,
-146.25228214336));
#145017=CARTESIAN_POINT('Ctrl Pts',(-23.1919887037201,-54.5810096937153,
-146.175879517442));
#145018=CARTESIAN_POINT('Ctrl Pts',(-23.1959969478324,-54.5800011956741,
-146.099496753778));
#145019=CARTESIAN_POINT('Ctrl Pts',(-23.2,-54.5800000210274,-146.023178055809));
#145020=CARTESIAN_POINT('Ctrl Pts',(-22.9849163103247,-55.591423110293,
-150.046801090999));
#145021=CARTESIAN_POINT('Ctrl Pts',(-23.6999999999999,-55.2903249255959,
-150.206318626088));
#145022=CARTESIAN_POINT('Ctrl Pts',(-23.7,-55.9902808012637,-149.835491960129));
#145023=CARTESIAN_POINT('Ctrl Pts',(-22.9994804181366,-59.343937645489,
-157.144704426787));
#145024=CARTESIAN_POINT('Ctrl Pts',(-23.7,-58.9786022357095,-157.10917403496));
#145025=CARTESIAN_POINT('Ctrl Pts',(-23.7,-59.7506418899787,-156.933381838169));
#145026=CARTESIAN_POINT('Ctrl Pts',(-23.0112491123844,-63.0152939322715,
-164.285990110815));
#145027=CARTESIAN_POINT('Ctrl Pts',(-23.7000000003822,-62.707250125371,
-164.298966961939));
#145028=CARTESIAN_POINT('Ctrl Pts',(-23.7,-63.4274104915032,-164.074673486974));
#145029=CARTESIAN_POINT('Ctrl Pts',(-23.0213852109847,-66.6453596297547,
-171.449026400902));
#145030=CARTESIAN_POINT('Ctrl Pts',(-23.7,-66.413901371901,-171.56646471025));
#145031=CARTESIAN_POINT('Ctrl Pts',(-23.7,-67.0618271655313,-171.237717270032));
#145032=CARTESIAN_POINT('Origin',(-24.2,-70.08000002,-174.34995));
#145033=CARTESIAN_POINT('',(-24.2,-73.08000002,-174.34995));
#145034=CARTESIAN_POINT('Origin',(-24.2,-72.58000002,-174.34995));
#145035=CARTESIAN_POINT('Origin',(-24.2,-70.08000002,-174.34995));
#145036=CARTESIAN_POINT('Origin',(-24.2,-72.58000002,-55.24995));
#145037=CARTESIAN_POINT('Origin',(-24.2,-72.58000002,-58.24995));
#145038=CARTESIAN_POINT('',(-24.2,-73.08000002,-174.34995));
#145039=CARTESIAN_POINT('Origin',(-24.2,-70.08000002,-58.24995));
#145040=CARTESIAN_POINT('Origin',(0.,-12.9675000200281,-60.64995));
#145041=CARTESIAN_POINT('',(-28.2496026309167,29.643102187894,-76.2257352477989));
#145042=CARTESIAN_POINT('',(-22.2890532034791,29.4093902975657,-83.1809305852948));
#145043=CARTESIAN_POINT('Ctrl Pts',(-28.2496026843433,29.6431021904052,
-76.2257353081032));
#145044=CARTESIAN_POINT('Ctrl Pts',(-27.0281878838229,29.5945550182985,
-77.7598757997112));
#145045=CARTESIAN_POINT('Ctrl Pts',(-25.7765799171754,29.5448662110019,
-79.270584144585));
#145046=CARTESIAN_POINT('Ctrl Pts',(-24.4879779898396,29.4944735933695,
-80.7447462809204));
#145047=CARTESIAN_POINT('Ctrl Pts',(-23.7649962843928,29.4662003618423,
-81.5718382111928));
#145048=CARTESIAN_POINT('Ctrl Pts',(-23.0327081268011,29.4377909731413,
-82.3848464598177));
#145049=CARTESIAN_POINT('Ctrl Pts',(-22.2891503921926,29.4093838642151,
-83.1810211215431));
#145050=CARTESIAN_POINT('Ctrl Pts',(-28.2795019009908,37.8065307949999,
-61.2273317382593));
#145051=CARTESIAN_POINT('Ctrl Pts',(-28.2706820191605,35.1297158291743,
-66.2515800426151));
#145052=CARTESIAN_POINT('Ctrl Pts',(-28.2608542879989,32.4163856120597,
-71.2554899486297));
#145053=CARTESIAN_POINT('Ctrl Pts',(-28.2496025504691,29.6431021990262,
-76.2257351951279));
#145054=CARTESIAN_POINT('Ctrl Pts',(-22.2890532034791,29.4093902975657,
-83.1809305852948));
#145055=CARTESIAN_POINT('Ctrl Pts',(-22.3038722896351,33.2381690976656,
-75.8991829023387));
#145056=CARTESIAN_POINT('Ctrl Pts',(-22.3157407792727,36.9852293035361,
-68.5739513473019));
#145057=CARTESIAN_POINT('Ctrl Pts',(-22.3259225534137,40.6914751389564,
-61.2273317382593));
#145058=CARTESIAN_POINT('Ctrl Pts',(-22.,41.1098595241823,-61.4386408691297));
#145059=CARTESIAN_POINT('Ctrl Pts',(-22.,40.7995210108967,-61.2819013639433));
#145060=CARTESIAN_POINT('Ctrl Pts',(-22.3259225534138,40.6914751389564,
-61.2273317382593));
#145061=CARTESIAN_POINT('Ctrl Pts',(-22.,41.1233751604146,-61.4118804447591));
#145062=CARTESIAN_POINT('Ctrl Pts',(-22.,40.8194184511061,-61.2339961299344));
#145063=CARTESIAN_POINT('Ctrl Pts',(-22.3307532272019,40.7164963923335,
-61.1738110360374));
#145064=CARTESIAN_POINT('Ctrl Pts',(-22.,41.1392509618672,-61.3865876948747));
#145065=CARTESIAN_POINT('Ctrl Pts',(-22.,40.8429002807173,-61.1881281443964));
#145066=CARTESIAN_POINT('Ctrl Pts',(-22.3364246839863,40.745888690896,-61.1232259520736));
#145067=CARTESIAN_POINT('Ctrl Pts',(-22.,41.1573899115079,-61.3627217630986));
#145068=CARTESIAN_POINT('Ctrl Pts',(-22.,40.8698280768405,-61.1441646043172));
#145069=CARTESIAN_POINT('Ctrl Pts',(-22.3428990418276,40.7794755973204,
-61.0754935261973));
#145070=CARTESIAN_POINT('Origin',(-22.5,41.1098595241823,-61.4386408691296));
#145071=CARTESIAN_POINT('Ctrl Pts',(-29.,38.7048160259599,-61.150138786574));
#145072=CARTESIAN_POINT('Ctrl Pts',(-29.,38.6926240909195,-60.6436056187277));
#145073=CARTESIAN_POINT('Ctrl Pts',(-28.4933647440612,38.6927858841382,
-60.650327573148));
#145074=CARTESIAN_POINT('Ctrl Pts',(-29.,38.6042425482601,-61.1525595652015));
#145075=CARTESIAN_POINT('Ctrl Pts',(-29.,38.5056874437974,-60.6032547660267));
#145076=CARTESIAN_POINT('Ctrl Pts',(-28.4508217728044,38.5151017970219,
-60.6551690977179));
#145077=CARTESIAN_POINT('Ctrl Pts',(-29.,38.5024684382473,-61.1789379706814));
#145078=CARTESIAN_POINT('Ctrl Pts',(-29.,38.2987442898004,-60.603134659432));
#145079=CARTESIAN_POINT('Ctrl Pts',(-28.4075947879363,38.335472514688,-60.707925961796));
#145080=CARTESIAN_POINT('Ctrl Pts',(-29.,38.3706532052714,-61.2520107824808));
#145081=CARTESIAN_POINT('Ctrl Pts',(-29.0000000000001,37.990375163389,-60.6863576421133));
#145082=CARTESIAN_POINT('Ctrl Pts',(-28.3514280416523,38.1029959208976,
-60.8540715547449));
#145083=CARTESIAN_POINT('Ctrl Pts',(-29.,38.3294709783247,-61.2822335925436));
#145084=CARTESIAN_POINT('Ctrl Pts',(-29.,37.8822359354345,-60.7316627868476));
#145085=CARTESIAN_POINT('Ctrl Pts',(-28.3338483525148,38.0303960306507,
-60.9145171861254));
#145086=CARTESIAN_POINT('Ctrl Pts',(-29.,38.2570904307121,-61.3534252594253));
#145087=CARTESIAN_POINT('Ctrl Pts',(-29.,37.6732261500514,-60.8640556435108));
#145088=CARTESIAN_POINT('Ctrl Pts',(-28.302912455342,37.9028346914031,-61.0569005178125));
#145089=CARTESIAN_POINT('Ctrl Pts',(-29.,38.2265217687548,-61.3934878926125));
#145090=CARTESIAN_POINT('Ctrl Pts',(-29.,37.5759010011862,-60.9505556565881));
#145091=CARTESIAN_POINT('Ctrl Pts',(-28.28982523324,37.8489775515987,-61.1370349799883));
#145092=CARTESIAN_POINT('Ctrl Pts',(-29.,38.2024209812184,-61.4386408691297));
#145093=CARTESIAN_POINT('Ctrl Pts',(-29.,37.4942143736512,-61.0606306836509));
#145094=CARTESIAN_POINT('Ctrl Pts',(-28.2795019009908,37.8065307949999,
-61.2273317382593));
#145095=CARTESIAN_POINT('Origin',(-28.5,38.2024209812184,-61.4386408691297));
#145096=CARTESIAN_POINT('Ctrl Pts',(-22.3259225534138,40.6914751389564,
-61.2273317382593));
#145097=CARTESIAN_POINT('Ctrl Pts',(-22.,40.7995210108967,-61.2819013639433));
#145098=CARTESIAN_POINT('Ctrl Pts',(-22.,41.1098595241823,-61.4386408691296));
#145099=CARTESIAN_POINT('Ctrl Pts',(-22.3157409333924,36.9852292354808,
-68.5739513464269));
#145100=CARTESIAN_POINT('Ctrl Pts',(-22.,37.1246521940256,-68.5757439011997));
#145101=CARTESIAN_POINT('Ctrl Pts',(-22.,37.3993732891074,-68.7852685139811));
#145102=CARTESIAN_POINT('Ctrl Pts',(-22.3038724392466,33.2381690210168,
-75.8991829107314));
#145103=CARTESIAN_POINT('Ctrl Pts',(-22.,33.3938486289533,-75.8821367178777));
#145104=CARTESIAN_POINT('Ctrl Pts',(-22.,33.6470169072337,-76.1105064350252));
#145105=CARTESIAN_POINT('Ctrl Pts',(-22.2890532034791,29.4093902975657,
-83.1809305852948));
#145106=CARTESIAN_POINT('Ctrl Pts',(-22.,29.5283900973743,-83.243628644349));
#145107=CARTESIAN_POINT('Ctrl Pts',(-22.,29.8104512658091,-83.3922397161652));
#145108=CARTESIAN_POINT('Origin',(-22.5,29.8104512658091,-83.3922397161652));
#145109=CARTESIAN_POINT('Ctrl Pts',(-22.,28.9209370328038,-87.2580513882026));
#145110=CARTESIAN_POINT('Ctrl Pts',(-21.999999999999,28.4137949053905,-87.2657118253129));
#145111=CARTESIAN_POINT('Ctrl Pts',(-22.5071523107133,28.4210424206146,
-87.2656152652095));
#145112=CARTESIAN_POINT('Ctrl Pts',(-22.,28.9107311888036,-86.5629863693187));
#145113=CARTESIAN_POINT('Ctrl Pts',(-22.000000000005,28.4408939884557,-86.5559074723074));
#145114=CARTESIAN_POINT('Ctrl Pts',(-22.468671524864,28.4096955954818,-86.5292441588387));
#145115=CARTESIAN_POINT('Ctrl Pts',(-22.,28.9839131874059,-85.8815326469363));
#145116=CARTESIAN_POINT('Ctrl Pts',(-22.,28.5474819289643,-85.8378355431043));
#145117=CARTESIAN_POINT('Ctrl Pts',(-22.4305087782965,28.4910039358137,
-85.8083788789715));
#145118=CARTESIAN_POINT('Ctrl Pts',(-22.,29.295020387663,-84.5463837617919));
#145119=CARTESIAN_POINT('Ctrl Pts',(-22.,28.9360692653603,-84.4506314222478));
#145120=CARTESIAN_POINT('Ctrl Pts',(-22.355087560244,28.8366692516703,-84.3978739445244));
#145121=CARTESIAN_POINT('Ctrl Pts',(-22.,29.5364895794699,-83.8869642769993));
#145122=CARTESIAN_POINT('Ctrl Pts',(-22.,29.2130027933481,-83.7664986820836));
#145123=CARTESIAN_POINT('Ctrl Pts',(-22.3174945400501,29.1049725391609,
-83.7022104338494));
#145124=CARTESIAN_POINT('Ctrl Pts',(-22.,29.8707648402079,-83.2803097208969));
#145125=CARTESIAN_POINT('Ctrl Pts',(-22.,29.5958623314302,-83.1287896750421));
#145126=CARTESIAN_POINT('Ctrl Pts',(-22.2826967104608,29.4763786725123,
-83.0629642223148));
#145127=CARTESIAN_POINT('Origin',(-22.5,28.91999998,-87.1305533863517));
#145128=CARTESIAN_POINT('Ctrl Pts',(-22.5,28.41999998,-87.1305533863517));
#145129=CARTESIAN_POINT('Ctrl Pts',(-22.4925022607297,28.4199999873068,
-86.9872865310408));
#145130=CARTESIAN_POINT('Ctrl Pts',(-22.4850006342183,28.4236086928051,
-86.8445929131946));
#145131=CARTESIAN_POINT('Ctrl Pts',(-22.4775177354222,28.4307308473477,
-86.7024958507061));
#145132=CARTESIAN_POINT('Ctrl Pts',(-22.4699230794522,28.4379593713449,
-86.5582765670637));
#145133=CARTESIAN_POINT('Ctrl Pts',(-22.4623471167486,28.4488065524411,
-86.4146711023061));
#145134=CARTESIAN_POINT('Ctrl Pts',(-22.4547938831896,28.4632181376622,
-86.2716829402881));
#145135=CARTESIAN_POINT('Ctrl Pts',(-22.4472338797339,28.4776426398602,
-86.1285666192395));
#145136=CARTESIAN_POINT('Ctrl Pts',(-22.4396959238395,28.4956377181282,
-85.9860679209476));
#145137=CARTESIAN_POINT('Ctrl Pts',(-22.4321746206815,28.5171995170665,
-85.8441807994112));
#145138=CARTESIAN_POINT('Ctrl Pts',(-22.4247161392233,28.5385812210358,
-85.703478790342));
#145139=CARTESIAN_POINT('Ctrl Pts',(-22.4172732887684,28.5634703812369,
-85.563377409009));
#145140=CARTESIAN_POINT('Ctrl Pts',(-22.4098425012551,28.5919139122317,
-85.4238730636314));
#145141=CARTESIAN_POINT('Ctrl Pts',(-22.4041287008053,28.613785168798,-85.3166031423822));
#145142=CARTESIAN_POINT('Ctrl Pts',(-22.3984219659058,28.637759060564,-85.2096861754146));
#145143=CARTESIAN_POINT('Ctrl Pts',(-22.3927255817788,28.6638766966531,
-85.1031257785058));
#145144=CARTESIAN_POINT('Ctrl Pts',(-22.3845799691,28.7012239230554,-84.9507484632194));
#145145=CARTESIAN_POINT('Ctrl Pts',(-22.3765086248503,28.7429980834321,
-84.7988713990416));
#145146=CARTESIAN_POINT('Ctrl Pts',(-22.3684633632018,28.7893041990692,
-84.6479093361407));
#145147=CARTESIAN_POINT('Ctrl Pts',(-22.3607674226928,28.8335997268858,
-84.5035019686805));
#145148=CARTESIAN_POINT('Ctrl Pts',(-22.3530953888868,28.8820428891203,
-84.3599318427346));
#145149=CARTESIAN_POINT('Ctrl Pts',(-22.3454424670516,28.9347184012903,
-84.2175904338271));
#145150=CARTESIAN_POINT('Ctrl Pts',(-22.3379638731583,28.9861940039585,
-84.0784914577315));
#145151=CARTESIAN_POINT('Ctrl Pts',(-22.3305035664366,29.0417120299716,
-83.9405658640323));
#145152=CARTESIAN_POINT('Ctrl Pts',(-22.3230932050103,29.1013344342888,
-83.8042070196682));
#145153=CARTESIAN_POINT('Ctrl Pts',(-22.3159094320307,29.1591337496624,
-83.6720176532777));
#145154=CARTESIAN_POINT('Ctrl Pts',(-22.3087727947964,29.2207908881213,
-83.5413008445181));
#145155=CARTESIAN_POINT('Ctrl Pts',(-22.3017446842256,29.2863365897173,
-83.4124403467295));
#145156=CARTESIAN_POINT('Ctrl Pts',(-22.2974989203793,29.3259335151363,
-83.3345942119541));
#145157=CARTESIAN_POINT('Ctrl Pts',(-22.2932933884543,29.3669490393746,
-83.2574260278765));
#145158=CARTESIAN_POINT('Ctrl Pts',(-22.289147100448,29.4093837384563,-83.1810246462237));
#145159=CARTESIAN_POINT('Origin',(-22.5,28.9199999800001,-55.24995));
#145160=CARTESIAN_POINT('Origin',(-21.5,43.91999998,-58.24995));
#145161=CARTESIAN_POINT('Origin',(-21.5,43.91999998,-58.24995));
#145162=CARTESIAN_POINT('Origin',(0.,43.91999998,-58.24995));
#145163=CARTESIAN_POINT('Origin',(-21.,43.91999998,-58.24995));
#145164=CARTESIAN_POINT('Origin',(-21.,43.91999998,-58.24995));
#145165=CARTESIAN_POINT('Origin',(-20.,28.9199999800001,-55.24995));
#145166=CARTESIAN_POINT('Origin',(-20.,28.9199999800001,-89.3628471840452));
#145167=CARTESIAN_POINT('Ctrl Pts',(-20.5,29.8613644840354,-85.690726129678));
#145168=CARTESIAN_POINT('Ctrl Pts',(-20.4999999999939,29.1873928364402,
-85.3058817835744));
#145169=CARTESIAN_POINT('Ctrl Pts',(-19.7932806530567,29.4660338803574,
-85.4648851598992));
#145170=CARTESIAN_POINT('Ctrl Pts',(-20.5,29.5176010887559,-86.2951263081817));
#145171=CARTESIAN_POINT('Ctrl Pts',(-20.500000000012,28.8766555508427,-85.9756966173608));
#145172=CARTESIAN_POINT('Ctrl Pts',(-19.8280358121594,29.0840893038539,
-86.104597627145));
#145173=CARTESIAN_POINT('Ctrl Pts',(-20.5,29.2776631432131,-86.9330351311447));
#145174=CARTESIAN_POINT('Ctrl Pts',(-20.5,28.6555724448382,-86.6950722871695));
#145175=CARTESIAN_POINT('Ctrl Pts',(-19.8643899928891,28.8174577851778,
-86.7807486916538));
#145176=CARTESIAN_POINT('Ctrl Pts',(-20.5,28.9676187538565,-88.2625011309141));
#145177=CARTESIAN_POINT('Ctrl Pts',(-20.5,28.4126392368736,-88.1554121614486));
#145178=CARTESIAN_POINT('Ctrl Pts',(-19.9391390454861,28.4729318977163,
-88.1921218543361));
#145179=CARTESIAN_POINT('Ctrl Pts',(-20.5,28.8999739472064,-88.958655057919));
#145180=CARTESIAN_POINT('Ctrl Pts',(-20.5,28.3749512792384,-88.9062582006903));
#145181=CARTESIAN_POINT('Ctrl Pts',(-19.9777772185812,28.3977575511637,
-88.9322835714639));
#145182=CARTESIAN_POINT('Ctrl Pts',(-20.5,28.9251268357589,-89.6426008613895));
#145183=CARTESIAN_POINT('Ctrl Pts',(-20.5,28.4403470064429,-89.6603905900511));
#145184=CARTESIAN_POINT('Ctrl Pts',(-20.0151084810686,28.4256906082963,
-89.6607392320332));
#145185=CARTESIAN_POINT('Origin',(-20.,29.726759920701,-85.9392854774869));
#145186=CARTESIAN_POINT('Ctrl Pts',(-19.8077680666402,29.3163999141123,
-85.7279763466165));
#145187=CARTESIAN_POINT('Ctrl Pts',(-20.5,29.0600890554149,-85.5959926642051));
#145188=CARTESIAN_POINT('Ctrl Pts',(-20.5,29.726759920701,-85.9392854774869));
#145189=CARTESIAN_POINT('Ctrl Pts',(-19.8234665452012,33.5607487699413,
-77.4712163753771));
#145190=CARTESIAN_POINT('Ctrl Pts',(-20.5000000001728,33.2278557603418,
-77.5610859264982));
#145191=CARTESIAN_POINT('Ctrl Pts',(-20.5,33.9784532599698,-77.6825438045949));
#145192=CARTESIAN_POINT('Ctrl Pts',(-19.8355385600285,37.7216554195719,
-69.1708971047811));
#145193=CARTESIAN_POINT('Ctrl Pts',(-20.5000000002289,37.4529027206824,
-69.1923113693162));
#145194=CARTESIAN_POINT('Ctrl Pts',(-20.5,38.1440461521965,-69.3822166533219));
#145195=CARTESIAN_POINT('Ctrl Pts',(-19.8457268663587,41.8441333387867,
-60.8508735991007));
#145196=CARTESIAN_POINT('Ctrl Pts',(-20.5,41.6540022187559,-60.7565814715328));
#145197=CARTESIAN_POINT('Ctrl Pts',(-20.5,42.270218132516,-61.0621827299711));
#145198=CARTESIAN_POINT('Ctrl Pts',(-13.8920088064511,43.6468101642065,
-60.8508735991007));
#145199=CARTESIAN_POINT('Ctrl Pts',(-13.5,43.724980245498,-60.8884062566336));
#145200=CARTESIAN_POINT('Ctrl Pts',(-13.5,44.086908282047,-61.0621827299711));
#145201=CARTESIAN_POINT('Ctrl Pts',(-13.883422492558,38.8394158858892,-70.8677262129548));
#145202=CARTESIAN_POINT('Ctrl Pts',(-13.5,38.9561333124887,-70.8371780085667));
#145203=CARTESIAN_POINT('Ctrl Pts',(-13.5,39.2774015744131,-71.0790468430123));
#145204=CARTESIAN_POINT('Ctrl Pts',(-13.8729900235566,34.0078012896411,
-80.8725774805421));
#145205=CARTESIAN_POINT('Ctrl Pts',(-13.5000000000877,34.1527775267561,
-80.7999951426717));
#145206=CARTESIAN_POINT('Ctrl Pts',(-13.5,34.4430593692808,-81.0839048048873));
#145207=CARTESIAN_POINT('Ctrl Pts',(-13.8582614853459,29.115831713372,-90.8469388041467));
#145208=CARTESIAN_POINT('Ctrl Pts',(-13.5,29.2108963546553,-90.8936099040706));
#145209=CARTESIAN_POINT('Ctrl Pts',(-13.5,29.5462485400348,-91.058247935017));
#145210=CARTESIAN_POINT('Origin',(-14.,29.5462485400348,-91.058247935017));
#145211=CARTESIAN_POINT('Ctrl Pts',(-13.8582614853459,29.115831713372,-90.8469388041467));
#145212=CARTESIAN_POINT('Ctrl Pts',(-13.5,29.2108963546553,-90.8936099040706));
#145213=CARTESIAN_POINT('Ctrl Pts',(-13.5,29.5462485400348,-91.058247935017));
#145214=CARTESIAN_POINT('Ctrl Pts',(-13.8598257678503,29.1000938294036,
-90.8779461296248));
#145215=CARTESIAN_POINT('Ctrl Pts',(-13.5,29.1946688455411,-90.923776404174));
#145216=CARTESIAN_POINT('Ctrl Pts',(-13.5,29.5320844445084,-91.0870988658315));
#145217=CARTESIAN_POINT('Ctrl Pts',(-13.8613943096149,29.0846206527093,
-90.9090791787867));
#145218=CARTESIAN_POINT('Ctrl Pts',(-13.4999999999997,29.1787031940904,
-90.9540383533105));
#145219=CARTESIAN_POINT('Ctrl Pts',(-13.5,29.518158585283,-91.1160643410222));
#145220=CARTESIAN_POINT('Ctrl Pts',(-13.8629670146618,29.0694104105324,
-90.9403371832586));
#145221=CARTESIAN_POINT('Ctrl Pts',(-13.5,29.1629965026825,-90.9843933533492));
#145222=CARTESIAN_POINT('Ctrl Pts',(-13.5,29.5044693674792,-91.1451435916293));
#145223=CARTESIAN_POINT('Ctrl Pts',(-11.3834743397155,29.812801930373,-90.9273317382593));
#145224=CARTESIAN_POINT('Ctrl Pts',(-12.,29.679733250215,-90.8631216114043));
#145225=CARTESIAN_POINT('Ctrl Pts',(-12.,30.2507177004773,-91.1386408691297));
#145226=CARTESIAN_POINT('Ctrl Pts',(-11.3956361798112,34.6396513996494,
-80.9174913671817));
#145227=CARTESIAN_POINT('Ctrl Pts',(-11.9999999998861,34.4484178829812,
-81.0174669870403));
#145228=CARTESIAN_POINT('Ctrl Pts',(-12.,35.0807977947169,-81.1288119730547));
#145229=CARTESIAN_POINT('Ctrl Pts',(-11.4042255504145,39.4271199662976,
-70.8881122426161));
#145230=CARTESIAN_POINT('Ctrl Pts',(-11.999999999893,39.2806183751482,-70.92559601425));
#145231=CARTESIAN_POINT('Ctrl Pts',(-12.,39.8700921493796,-71.0994291820815));
#145232=CARTESIAN_POINT('Ctrl Pts',(-11.4112929481563,44.1984900402045,
-60.8508735991007));
#145233=CARTESIAN_POINT('Ctrl Pts',(-12.,44.102645384174,-60.8052987597771));
#145234=CARTESIAN_POINT('Ctrl Pts',(-12.,44.6428767076058,-61.062182729971));
#145235=CARTESIAN_POINT('Ctrl Pts',(-5.45757488824865,45.0702713246265,
-60.8508735991007));
#145236=CARTESIAN_POINT('Ctrl Pts',(-5.,45.1055585268383,-60.8674008824013));
#145237=CARTESIAN_POINT('Ctrl Pts',(-5.,45.5214348882082,-61.0621827299711));
#145238=CARTESIAN_POINT('Ctrl Pts',(-5.45419794131935,40.3738290579191,
-70.8788685457756));
#145239=CARTESIAN_POINT('Ctrl Pts',(-5.00000000013405,40.4263150647969,
-70.8653394730463));
#145240=CARTESIAN_POINT('Ctrl Pts',(-5.,40.8246742459034,-71.0901794372786));
#145241=CARTESIAN_POINT('Ctrl Pts',(-5.4500940393161,35.6738220550387,-80.9051511012611));
#145242=CARTESIAN_POINT('Ctrl Pts',(-5.00000000002896,35.7394456595583,
-80.8717315350143));
#145243=CARTESIAN_POINT('Ctrl Pts',(-5.,36.1242566254946,-81.1164625478583));
#145244=CARTESIAN_POINT('Ctrl Pts',(-5.44427033638569,30.9653765476951,
-90.9273317382593));
#145245=CARTESIAN_POINT('Ctrl Pts',(-4.99999999999999,31.0104747491644,
-90.9485222334823));
#145246=CARTESIAN_POINT('Ctrl Pts',(-5.,31.4150905187971,-91.1386408691297));
#145247=CARTESIAN_POINT('Origin',(-57.,11.11999998,-58.24995));
#145248=CARTESIAN_POINT('',(-60.,11.11999998,-58.24995));
#145249=CARTESIAN_POINT('Origin',(-57.,11.11999998,-58.24995));
#145250=CARTESIAN_POINT('Origin',(-59.5,11.11999998,-58.24995));
#145251=CARTESIAN_POINT('Origin',(-57.,-2.42462934179819E-14,-58.24995));
#145252=CARTESIAN_POINT('',(-60.,11.61999998,-58.24995));
#145253=CARTESIAN_POINT('Origin',(-57.,11.61999998,-58.24995));
#145254=CARTESIAN_POINT('',(-60.,-54.58000002,-58.24995));
#145255=CARTESIAN_POINT('Origin',(-57.,11.61999998,-58.24995));
#145256=CARTESIAN_POINT('Origin',(-59.5,11.61999998,-58.24995));
#145257=CARTESIAN_POINT('Origin',(-57.,-37.78000002,-58.24995));
#145258=CARTESIAN_POINT('',(-60.,-37.78000002,-58.24995));
#145259=CARTESIAN_POINT('Origin',(-57.,-37.78000002,-58.24995));
#145260=CARTESIAN_POINT('Origin',(-59.5,-37.78000002,-58.24995));
#145261=CARTESIAN_POINT('Origin',(-57.,-2.42462934179819E-14,-58.24995));
#145262=CARTESIAN_POINT('',(-60.,-37.28000002,-58.24995));
#145263=CARTESIAN_POINT('Origin',(-57.,-37.28000002,-58.24995));
#145264=CARTESIAN_POINT('',(-60.,-54.58000002,-58.24995));
#145265=CARTESIAN_POINT('Origin',(-57.,-37.28000002,-58.24995));
#145266=CARTESIAN_POINT('Origin',(-59.5,-37.28000002,-58.24995));
#145267=CARTESIAN_POINT('Origin',(-60.,-37.28000002,-176.84995));
#145268=CARTESIAN_POINT('',(-53.7578119323263,-37.28000002,-177.34995));
#145269=CARTESIAN_POINT('',(-57.,-37.28000002,-177.34995));
#145270=CARTESIAN_POINT('',(-60.,-37.28000002,-177.34995));
#145271=CARTESIAN_POINT('Origin',(-57.,-37.28000002,-176.84995));
#145272=CARTESIAN_POINT('Ctrl Pts',(-53.7578119323263,-37.28000002,-177.34995));
#145273=CARTESIAN_POINT('Ctrl Pts',(-53.8142255012181,-37.2176314844153,
-177.34995));
#145274=CARTESIAN_POINT('Ctrl Pts',(-53.8706043508049,-37.1546953024018,
-177.33811707005));
#145275=CARTESIAN_POINT('Ctrl Pts',(-53.9751511105352,-37.0369743252984,
-177.291477883886));
#145276=CARTESIAN_POINT('Ctrl Pts',(-54.0238234872226,-36.9816277442484,
-177.25641751247));
#145277=CARTESIAN_POINT('Ctrl Pts',(-54.1061105508192,-36.8874586360784,
-177.16641977034));
#145278=CARTESIAN_POINT('Ctrl Pts',(-54.1401753140075,-36.8481352183371,
-177.110787176626));
#145279=CARTESIAN_POINT('Ctrl Pts',(-54.1865253922149,-36.7944813746413,
-176.987117359946));
#145280=CARTESIAN_POINT('Ctrl Pts',(-54.1989607146972,-36.78000002,-176.918317891383));
#145281=CARTESIAN_POINT('Ctrl Pts',(-54.1989607257493,-36.78000002,-176.84995));
#145282=CARTESIAN_POINT('Origin',(-54.1989607257493,-36.28000002,-179.64995));
#145283=CARTESIAN_POINT('Origin',(-54.1989607257493,-36.28000002,-171.871644662643));
#145284=CARTESIAN_POINT('Origin',(-54.1989607257493,-36.28000002,-176.84995));
#145285=CARTESIAN_POINT('Ctrl Pts',(-53.7393383808294,-36.0824871697421,
-171.894658379227));
#145286=CARTESIAN_POINT('Ctrl Pts',(-53.4395062235889,-36.7800433691512,
-171.887030357483));
#145287=CARTESIAN_POINT('Ctrl Pts',(-54.198558315946,-36.7800000191852,
-171.906167818573));
#145288=CARTESIAN_POINT('Ctrl Pts',(-53.7436938429485,-36.0817727411102,
-171.73251549148));
#145289=CARTESIAN_POINT('Ctrl Pts',(-53.4406325939148,-36.7800434674344,
-171.778613128972));
#145290=CARTESIAN_POINT('Ctrl Pts',(-54.2046305452577,-36.7800000191843,
-171.662933242578));
#145291=CARTESIAN_POINT('Ctrl Pts',(-53.7019584052344,-36.0886165914289,
-171.572834421444));
#145292=CARTESIAN_POINT('Ctrl Pts',(-53.4304080193297,-36.7800425499783,
-171.672542976741));
#145293=CARTESIAN_POINT('Ctrl Pts',(-54.1464425180027,-36.7800000191923,
-171.423436673449));
#145294=CARTESIAN_POINT('Ctrl Pts',(-53.6182347475042,-36.1024349685042,
-171.42841039455));
#145295=CARTESIAN_POINT('Ctrl Pts',(-53.391611466063,-36.7800408062075,
-171.55046073112));
#145296=CARTESIAN_POINT('Ctrl Pts',(-54.0297882222689,-36.7800000192084,
-171.20677750911));
#145297=CARTESIAN_POINT('',(-53.6298444656516,-36.1005191032365,-171.449026400902));
#145298=CARTESIAN_POINT('Origin',(-54.0459394689003,-36.28000002,-171.237717270032));
#145299=CARTESIAN_POINT('Origin',(-52.5055674318865,-36.2860379741571,-171.88552542821));
#145300=CARTESIAN_POINT('Ctrl Pts',(-53.6298444656516,-36.1005191032365,
-171.449026400902));
#145301=CARTESIAN_POINT('Ctrl Pts',(-53.3968439469627,-36.78000002,-171.567353073206));
#145302=CARTESIAN_POINT('Ctrl Pts',(-54.0459394689003,-36.78000002,-171.237717270032));
#145303=CARTESIAN_POINT('Ctrl Pts',(-51.4138274897758,-36.0943068851322,
-167.080125911017));
#145304=CARTESIAN_POINT('Ctrl Pts',(-51.1479384960996,-36.78000002,-167.162122528925));
#145305=CARTESIAN_POINT('Ctrl Pts',(-51.827241891131,-36.78000002,-166.868814837648));
#145306=CARTESIAN_POINT('Ctrl Pts',(-49.181606116838,-36.0874694888798,
-162.719878659059));
#145307=CARTESIAN_POINT('Ctrl Pts',(-48.8961865333283,-36.7800000199664,
-162.797005637805));
#145308=CARTESIAN_POINT('Ctrl Pts',(-49.5919157423408,-36.78000002,-162.508569528187));
#145309=CARTESIAN_POINT('Ctrl Pts',(-44.6695423554902,-36.0720830782198,
-154.02490615155));
#145310=CARTESIAN_POINT('Ctrl Pts',(-44.3536351698063,-36.7800000200344,
-154.11869394055));
#145311=CARTESIAN_POINT('Ctrl Pts',(-45.0722737045335,-36.78000002,-153.813597020681));
#145312=CARTESIAN_POINT('Ctrl Pts',(-42.3899819460371,-36.0635378106947,
-149.6900251133));
#145313=CARTESIAN_POINT('Ctrl Pts',(-42.0456232774016,-36.78000002,-149.775736877395));
#145314=CARTESIAN_POINT('Ctrl Pts',(-42.7882496386931,-36.78000002,-149.478711493085));
#145315=CARTESIAN_POINT('Ctrl Pts',(-40.0734472163172,-36.0537915241817,
-145.374999642302));
#145316=CARTESIAN_POINT('Ctrl Pts',(-39.7490326214954,-36.78000002,-145.549584755123));
#145317=CARTESIAN_POINT('Ctrl Pts',(-40.4661024946855,-36.78000002,-145.163690511432));
#145318=CARTESIAN_POINT('',(-40.0734471921219,-36.0537915982708,-145.374999599156));
#145319=CARTESIAN_POINT('Origin',(-40.4661024946856,-36.28000002,-145.163690511432));
#145320=CARTESIAN_POINT('Ctrl Pts',(-40.0734472163172,-36.0537915241817,
-145.374999642303));
#145321=CARTESIAN_POINT('Ctrl Pts',(-42.3899819460361,-36.0635378106967,
-149.6900251133));
#145322=CARTESIAN_POINT('Ctrl Pts',(-44.6695423554893,-36.0720830782218,
-154.02490615155));
#145323=CARTESIAN_POINT('Ctrl Pts',(-49.1816061168372,-36.0874694888818,
-162.719878659059));
#145324=CARTESIAN_POINT('Ctrl Pts',(-51.413827489775,-36.0943068851342,
-167.080125911017));
#145325=CARTESIAN_POINT('Ctrl Pts',(-53.6298444656516,-36.1005191032365,
-171.449026400902));
#145326=CARTESIAN_POINT('Ctrl Pts',(-39.5,-36.78000002,-141.149515588739));
#145327=CARTESIAN_POINT('Ctrl Pts',(-38.9999999999999,-36.78000002,-141.149515588739));
#145328=CARTESIAN_POINT('Ctrl Pts',(-39.,-36.28000002,-141.149515588739));
#145329=CARTESIAN_POINT('Ctrl Pts',(-39.5000000020403,-36.78000002,-141.848776286889));
#145330=CARTESIAN_POINT('Ctrl Pts',(-38.9595709612524,-36.78000002,-141.917511819575));
#145331=CARTESIAN_POINT('Ctrl Pts',(-39.,-36.2411525212205,-141.887468602714));
#145332=CARTESIAN_POINT('Ctrl Pts',(-39.5789972525929,-36.78000002,-142.535527260215));
#145333=CARTESIAN_POINT('Ctrl Pts',(-39.0069624314851,-36.78000002,-142.654181226843));
#145334=CARTESIAN_POINT('Ctrl Pts',(-39.0877747262142,-36.202664552653,
-142.611197003283));
#145335=CARTESIAN_POINT('Ctrl Pts',(-39.8950301507098,-36.78000002,-143.883204247708));
#145336=CARTESIAN_POINT('Ctrl Pts',(-39.2475606867303,-36.78000002,-144.126025522057));
#145337=CARTESIAN_POINT('Ctrl Pts',(-39.4389223885666,-36.1266531472167,
-144.029685314679));
#145338=CARTESIAN_POINT('Ctrl Pts',(-40.1353628336737,-36.78000002,-144.549109040068));
#145339=CARTESIAN_POINT('Ctrl Pts',(-39.4615987310595,-36.78000002,-144.873235586497));
#145340=CARTESIAN_POINT('Ctrl Pts',(-39.7059668714196,-36.0888399354841,
-144.729666200452));
#145341=CARTESIAN_POINT('Ctrl Pts',(-40.4661024946855,-36.78000002,-145.163690511432));
#145342=CARTESIAN_POINT('Ctrl Pts',(-39.7490326214954,-36.78000002,-145.549584755123));
#145343=CARTESIAN_POINT('Ctrl Pts',(-40.0734472163172,-36.0537915241817,
-145.374999642303));
#145344=CARTESIAN_POINT('',(-39.000000000323,-36.28000002,-141.149515588739));
#145345=CARTESIAN_POINT('Origin',(-39.5,-36.28000002,-141.149515588739));
#145346=CARTESIAN_POINT('Ctrl Pts',(-39.,-36.28000002,-141.149515588739));
#145347=CARTESIAN_POINT('Ctrl Pts',(-39.,-36.2411525212205,-141.887468602714));
#145348=CARTESIAN_POINT('Ctrl Pts',(-39.0877747262142,-36.202664552653,
-142.611197003283));
#145349=CARTESIAN_POINT('Ctrl Pts',(-39.438922384402,-36.1266531481182,
-144.029685297855));
#145350=CARTESIAN_POINT('Ctrl Pts',(-39.705966858751,-36.088839937278,-144.729666167245));
#145351=CARTESIAN_POINT('Ctrl Pts',(-40.0734471901673,-36.0537915266758,
-145.374999596381));
#145352=CARTESIAN_POINT('Origin',(-39.5,-36.28000002,-55.24995));
#145353=CARTESIAN_POINT('',(-39.0000000003234,-36.28000002,-90.9091273827666));
#145354=CARTESIAN_POINT('Origin',(-39.5,-36.28000002,-90.9091273827666));
#145355=CARTESIAN_POINT('',(-39.,-36.28000002,-129.34995));
#145356=CARTESIAN_POINT('Ctrl Pts',(-40.6770017977572,-36.78000002,-86.5290501999886));
#145357=CARTESIAN_POINT('Ctrl Pts',(-39.9462151352518,-36.7800000199977,
-86.0754691928917));
#145358=CARTESIAN_POINT('Ctrl Pts',(-40.3079584328326,-36.0324776431912,
-86.2996877651884));
#145359=CARTESIAN_POINT('Ctrl Pts',(-40.2312592357455,-36.78000002,-87.252600640522));
#145360=CARTESIAN_POINT('Ctrl Pts',(-39.5535852275517,-36.7800000200034,
-86.8763713735618));
#145361=CARTESIAN_POINT('Ctrl Pts',(-39.8127216435129,-36.07379497991,-87.0589794447612));
#145362=CARTESIAN_POINT('Ctrl Pts',(-39.9312338876434,-36.78000002,-88.0264426730864));
#145363=CARTESIAN_POINT('Ctrl Pts',(-39.2777008559782,-36.78000002,-87.752028167821));
#145364=CARTESIAN_POINT('Ctrl Pts',(-39.4792833821553,-36.1178028681844,
-87.8722265567825));
#145365=CARTESIAN_POINT('Ctrl Pts',(-39.5486697096471,-36.78000002,-89.6471359721043));
#145366=CARTESIAN_POINT('Ctrl Pts',(-38.9856597630179,-36.78000002,-89.5246670643281));
#145367=CARTESIAN_POINT('Ctrl Pts',(-39.0541288673858,-36.2092330444632,
-89.5780096393087));
#145368=CARTESIAN_POINT('Ctrl Pts',(-39.470934045995,-36.78000002,-90.4953146912642));
#145369=CARTESIAN_POINT('Ctrl Pts',(-38.9434898522956,-36.7800000199999,
-90.4333580855596));
#145370=CARTESIAN_POINT('Ctrl Pts',(-38.967723555261,-36.2567217271198,
-90.4720476855702));
#145371=CARTESIAN_POINT('Ctrl Pts',(-39.5096795928158,-36.78000002,-91.3254326715997));
#145372=CARTESIAN_POINT('Ctrl Pts',(-39.0324507754533,-36.78000002,-91.348061068846));
#145373=CARTESIAN_POINT('Ctrl Pts',(-39.0107369205707,-36.302690307335,
-91.3486055792047));
#145374=CARTESIAN_POINT('Origin',(-40.4661024946855,-36.28000002,-86.8949524600738));
#145375=CARTESIAN_POINT('Ctrl Pts',(-40.0734472049734,-36.0537916894494,
-86.683643483585));
#145376=CARTESIAN_POINT('Ctrl Pts',(-40.0114299049165,-36.0597067375102,
-86.7925528685563));
#145377=CARTESIAN_POINT('Ctrl Pts',(-39.9525082269032,-36.0657556651474,
-86.9025541827257));
#145378=CARTESIAN_POINT('Ctrl Pts',(-39.8965331132721,-36.071857980972,
-87.0135362800466));
#145379=CARTESIAN_POINT('Ctrl Pts',(-39.8393965078108,-36.0780869207464,
-87.1268212721892));
#145380=CARTESIAN_POINT('Ctrl Pts',(-39.7853292584481,-36.0843716935665,
-87.2411283173954));
#145381=CARTESIAN_POINT('Ctrl Pts',(-39.7341789370736,-36.0906669132536,
-87.3563756163275));
#145382=CARTESIAN_POINT('Ctrl Pts',(-39.6814728827467,-36.0971536015463,
-87.4751281526814));
#145383=CARTESIAN_POINT('Ctrl Pts',(-39.6318631125474,-36.1036516536209,
-87.5948792120369));
#145384=CARTESIAN_POINT('Ctrl Pts',(-39.585201243061,-36.1101500863352,
-87.7155749645938));
#145385=CARTESIAN_POINT('Ctrl Pts',(-39.5379048483671,-36.1167368871198,
-87.8379119822408));
#145386=CARTESIAN_POINT('Ctrl Pts',(-39.4936364182298,-36.1233245580757,
-87.9612199614972));
#145387=CARTESIAN_POINT('Ctrl Pts',(-39.4522709948862,-36.1299348761892,
-88.0854741526894));
#145388=CARTESIAN_POINT('Ctrl Pts',(-39.410242901257,-36.1366510909922,
-88.2117188846207));
#145389=CARTESIAN_POINT('Ctrl Pts',(-39.3712109975668,-36.1433912403681,
-88.3389408708692));
#145390=CARTESIAN_POINT('Ctrl Pts',(-39.3350839554796,-36.1502043283924,
-88.4671395179936));
#145391=CARTESIAN_POINT('Ctrl Pts',(-39.3109789632385,-36.1547502149216,
-88.5526773095123));
#145392=CARTESIAN_POINT('Ctrl Pts',(-39.2881680479569,-36.1593291055865,
-88.6386504236153));
#145393=CARTESIAN_POINT('Ctrl Pts',(-39.2666353702995,-36.1639599373599,
-88.7250630960682));
#145394=CARTESIAN_POINT('Ctrl Pts',(-39.2122577419081,-36.1756544257708,
-88.9432856629837));
#145395=CARTESIAN_POINT('Ctrl Pts',(-39.1661135646958,-36.1874916418147,
-89.1641945089367));
#145396=CARTESIAN_POINT('Ctrl Pts',(-39.1282921823357,-36.1993765320403,
-89.3868152665253));
#145397=CARTESIAN_POINT('Ctrl Pts',(-39.088819852784,-36.2117802115041,
-89.6191536782976));
#145398=CARTESIAN_POINT('Ctrl Pts',(-39.0584124114518,-36.2242363436397,
-89.8533578805103));
#145399=CARTESIAN_POINT('Ctrl Pts',(-39.0371354777509,-36.2366815663543,
-90.0883178712863));
#145400=CARTESIAN_POINT('Ctrl Pts',(-39.016148797974,-36.2489570148533,
-90.320072604186));
#145401=CARTESIAN_POINT('Ctrl Pts',(-39.0040453665294,-36.2612227588303,
-90.5525637896143));
#145402=CARTESIAN_POINT('Ctrl Pts',(-39.0008560407261,-36.2734488399052,
-90.7847063396569));
#145403=CARTESIAN_POINT('Ctrl Pts',(-39.0002860653393,-36.2756338049164,
-90.826193333433));
#145404=CARTESIAN_POINT('Ctrl Pts',(-39.0000007020242,-36.2778175640703,
-90.8676691154279));
#145405=CARTESIAN_POINT('Ctrl Pts',(-39.0000000012937,-36.28000002,-90.9091273827666));
#145406=CARTESIAN_POINT('Ctrl Pts',(-40.0734472163172,-36.0537915241817,
-86.6836433292035));
#145407=CARTESIAN_POINT('Ctrl Pts',(-39.7490326214953,-36.78000002,-86.5090582163831));
#145408=CARTESIAN_POINT('Ctrl Pts',(-40.4661024946855,-36.78000002,-86.8949524600738));
#145409=CARTESIAN_POINT('Ctrl Pts',(-42.3689613408276,-36.0634493712886,
-82.407773086856));
#145410=CARTESIAN_POINT('Ctrl Pts',(-42.0251435460116,-36.78000002,-82.3205925927599));
#145411=CARTESIAN_POINT('Ctrl Pts',(-42.7671781583824,-36.78000002,-82.6190865682492));
#145412=CARTESIAN_POINT('Ctrl Pts',(-44.6279666698635,-36.0719269202766,
-78.1127593269182));
#145413=CARTESIAN_POINT('Ctrl Pts',(-44.3122026972581,-36.7800000199999,
-78.0178858717772));
#145414=CARTESIAN_POINT('Ctrl Pts',(-45.0306161020287,-36.78000002,-78.3240684577782));
#145415=CARTESIAN_POINT('Ctrl Pts',(-49.0993449617391,-36.0872029629615,
-69.4983516685814));
#145416=CARTESIAN_POINT('Ctrl Pts',(-48.8138634148613,-36.78000002,-69.420066134471));
#145417=CARTESIAN_POINT('Ctrl Pts',(-49.5095281828678,-36.78000002,-69.7096607994621));
#145418=CARTESIAN_POINT('Ctrl Pts',(-51.3114450013405,-36.0939978375791,
-65.1788088209436));
#145419=CARTESIAN_POINT('Ctrl Pts',(-51.0452850559209,-36.7800000200001,
-65.0958859597511));
#145420=CARTESIAN_POINT('Ctrl Pts',(-51.7247198970815,-36.78000002,-65.3901198450985));
#145421=CARTESIAN_POINT('Ctrl Pts',(-53.5074514076768,-36.1001753985996,
-60.8508735991007));
#145422=CARTESIAN_POINT('Ctrl Pts',(-53.2738374538033,-36.7800000199999,
-60.7321930665019));
#145423=CARTESIAN_POINT('Ctrl Pts',(-53.9233979868778,-36.78000002,-61.0621827299711));
#145424=CARTESIAN_POINT('Origin',(-59.5,-37.28000002,-55.24995));
#145425=CARTESIAN_POINT('',(-60.,-37.28000002,-174.34995));
#145426=CARTESIAN_POINT('Origin',(-59.5,-37.28000002,-174.34995));
#145427=CARTESIAN_POINT('',(-60.,-37.28000002,-58.24995));
#145428=CARTESIAN_POINT('Origin',(-57.,-37.28000002,-174.34995));
#145429=CARTESIAN_POINT('Origin',(-57.,-37.28000002,-174.34995));
#145430=CARTESIAN_POINT('Ctrl Pts',(-39.,-38.3588510099497,-88.7507007177297));
#145431=CARTESIAN_POINT('Ctrl Pts',(-39.,-37.0899493132599,-87.566881951549));
#145432=CARTESIAN_POINT('Ctrl Pts',(-40.0751063884513,-36.0938884806558,
-86.6376094090262));
#145433=CARTESIAN_POINT('Ctrl Pts',(-39.,-37.1517824539261,-90.044523203833));
#145434=CARTESIAN_POINT('Ctrl Pts',(-38.9999999999755,-35.9377762186181,
-88.8634929468774));
#145435=CARTESIAN_POINT('Ctrl Pts',(-40.0284942066422,-34.9676073874133,
-87.9314164096932));
#145436=CARTESIAN_POINT('Ctrl Pts',(-39.,-35.9043080884012,-91.3133047711639));
#145437=CARTESIAN_POINT('Ctrl Pts',(-39.0000000000062,-34.7456425298457,
-90.138609363953));
#145438=CARTESIAN_POINT('Ctrl Pts',(-39.9811083568879,-33.8078923846355,
-89.2002134624161));
#145439=CARTESIAN_POINT('Ctrl Pts',(-39.,-33.3065376953223,-93.7717385435459));
#145440=CARTESIAN_POINT('Ctrl Pts',(-38.9999999999938,-32.2660375633753,
-92.6092802152048));
#145441=CARTESIAN_POINT('Ctrl Pts',(-39.8860349814824,-31.4034505542693,
-91.6586472348866));
#145442=CARTESIAN_POINT('Ctrl Pts',(-39.,-31.9694828580011,-94.9490286570666));
#145443=CARTESIAN_POINT('Ctrl Pts',(-39.,-30.9915371636578,-93.792984660173));
#145444=CARTESIAN_POINT('Ctrl Pts',(-39.8388209456929,-30.1709967638591,
-92.8359193626927));
#145445=CARTESIAN_POINT('Ctrl Pts',(-39.,-30.5806160716777,-96.0559019707015));
#145446=CARTESIAN_POINT('Ctrl Pts',(-39.,-29.6660656545474,-94.9083553778138));
#145447=CARTESIAN_POINT('Ctrl Pts',(-39.7930043023957,-28.8965637205256,
-93.942810661998));
#145448=CARTESIAN_POINT('',(-39.,-30.63000002,-96.0164973302555));
#145449=CARTESIAN_POINT('Ctrl Pts',(-39.,-30.63000002,-96.0164973302555));
#145450=CARTESIAN_POINT('Ctrl Pts',(-39.0000000000004,-31.0448154973603,
-95.6851069386961));
#145451=CARTESIAN_POINT('Ctrl Pts',(-39.0000000000118,-31.4542117376853,
-95.3480909235783));
#145452=CARTESIAN_POINT('Ctrl Pts',(-39.0000000000377,-31.8588908811782,
-95.0057530542713));
#145453=CARTESIAN_POINT('Ctrl Pts',(-39.0000000000646,-32.2780518714119,
-94.651164282894));
#145454=CARTESIAN_POINT('Ctrl Pts',(-39.0000000001072,-32.692151896703,
-94.2908656551339));
#145455=CARTESIAN_POINT('Ctrl Pts',(-39.0000000001713,-33.101937367171,
-93.925148764688));
#145456=CARTESIAN_POINT('Ctrl Pts',(-39.0000000002394,-33.5373888365781,
-93.5365260125201));
#145457=CARTESIAN_POINT('Ctrl Pts',(-39.0000000003318,-33.9679681800119,
-93.1417847772573));
#145458=CARTESIAN_POINT('Ctrl Pts',(-39.0000000004578,-34.3945363851635,
-92.7412278682546));
#145459=CARTESIAN_POINT('Ctrl Pts',(-39.0000000004786,-34.4649233357429,
-92.6751329764701));
#145460=CARTESIAN_POINT('Ctrl Pts',(-39.0000000005003,-34.5352010050805,
-92.6088796460175));
#145461=CARTESIAN_POINT('Ctrl Pts',(-39.000000000523,-34.605373184231,-92.5424691324455));
#145462=CARTESIAN_POINT('Ctrl Pts',(-39.0000000006715,-35.0646606142765,
-92.1078023674154));
#145463=CARTESIAN_POINT('Ctrl Pts',(-39.0000000008613,-35.5177770524177,
-91.6679502774283));
#145464=CARTESIAN_POINT('Ctrl Pts',(-39.0000000011092,-35.9656372187857,
-91.2230746457426));
#145465=CARTESIAN_POINT('Ctrl Pts',(-39.0000000011674,-36.0707105046109,
-91.1187015670117));
#145466=CARTESIAN_POINT('Ctrl Pts',(-39.0000000012288,-36.1754942796843,
-91.0140518531514));
#145467=CARTESIAN_POINT('Ctrl Pts',(-39.0000000012937,-36.28000002,-90.9091273827666));
#145468=CARTESIAN_POINT('Ctrl Pts',(-39.,-30.63000002,-96.0164973302555));
#145469=CARTESIAN_POINT('Ctrl Pts',(-39.0000000079586,-30.6231766417215,
-95.8820262726144));
#145470=CARTESIAN_POINT('Ctrl Pts',(-39.0035821145827,-30.6163413437257,
-95.7481485193516));
#145471=CARTESIAN_POINT('Ctrl Pts',(-39.0106426175382,-30.6095153827799,
-95.6148868536627));
#145472=CARTESIAN_POINT('Ctrl Pts',(-39.0178214769745,-30.6025749970231,
-95.4793912987054));
#145473=CARTESIAN_POINT('Ctrl Pts',(-39.0285958092194,-30.5956437403606,
-95.3445319365772));
#145474=CARTESIAN_POINT('Ctrl Pts',(-39.0429017264386,-30.5887258812893,
-95.2103098405928));
#145475=CARTESIAN_POINT('Ctrl Pts',(-39.0572494516417,-30.5817878052871,
-95.0756954904708));
#145476=CARTESIAN_POINT('Ctrl Pts',(-39.0751492079689,-30.5748625588069,
-94.9417213032506));
#145477=CARTESIAN_POINT('Ctrl Pts',(-39.0965870557023,-30.5679453488797,
-94.808377425016));
#145478=CARTESIAN_POINT('Ctrl Pts',(-39.1179306962842,-30.5610585361571,
-94.6756195173088));
#145479=CARTESIAN_POINT('Ctrl Pts',(-39.1427814447475,-30.5541790046426,
-94.5434855565985));
#145480=CARTESIAN_POINT('Ctrl Pts',(-39.1711767973116,-30.5473030129425,
-94.4119675106066));
#145481=CARTESIAN_POINT('Ctrl Pts',(-39.1839235911889,-30.5442163511831,
-94.3529285034445));
#145482=CARTESIAN_POINT('Ctrl Pts',(-39.1973853608932,-30.5411304784574,
-94.2940137110658));
#145483=CARTESIAN_POINT('Ctrl Pts',(-39.2115687799563,-30.5380456903908,
-94.2352231979354));
#145484=CARTESIAN_POINT('Ctrl Pts',(-39.2472280937484,-30.5302900550844,
-94.0874147360689));
#145485=CARTESIAN_POINT('Ctrl Pts',(-39.2874998404854,-30.522578402994,
-93.9401454048209));
#145486=CARTESIAN_POINT('Ctrl Pts',(-39.332455133363,-30.5148808266874,
-93.793846273556));
#145487=CARTESIAN_POINT('Ctrl Pts',(-39.3763272094434,-30.507368726738,
-93.6510722817411));
#145488=CARTESIAN_POINT('Ctrl Pts',(-39.4246605045649,-30.4998700742262,
-93.5092222546581));
#145489=CARTESIAN_POINT('Ctrl Pts',(-39.4775038131332,-30.4923933804749,
-93.3687230037208));
#145490=CARTESIAN_POINT('Ctrl Pts',(-39.530512762818,-30.4848932504942,
-93.227783347869));
#145491=CARTESIAN_POINT('Ctrl Pts',(-39.5880608773232,-30.4774152181983,
-93.0882029261299));
#145492=CARTESIAN_POINT('Ctrl Pts',(-39.6501685426812,-30.4700048105513,
-92.9504399167027));
#145493=CARTESIAN_POINT('Ctrl Pts',(-39.7091203015329,-30.4629709514925,
-92.8196771249667));
#145494=CARTESIAN_POINT('Ctrl Pts',(-39.7721804412542,-30.4559984296717,
-92.6905520637433));
#145495=CARTESIAN_POINT('Ctrl Pts',(-39.8393317526662,-30.4491558380067,
-92.5634785170804));
#145496=CARTESIAN_POINT('Ctrl Pts',(-39.8429266116615,-30.4487895286722,
-92.5566757983741));
#145497=CARTESIAN_POINT('Ctrl Pts',(-39.8465331858288,-30.4484235982178,
-92.5498789637867));
#145498=CARTESIAN_POINT('Ctrl Pts',(-39.8501514691891,-30.4480580593471,
-92.543088078389));
#145499=CARTESIAN_POINT('Ctrl Pts',(-55.5967474138374,-30.4937575588533,
-60.8508735991007));
#145500=CARTESIAN_POINT('Ctrl Pts',(-55.6892944482707,-30.13000002,-60.8961225062558));
#145501=CARTESIAN_POINT('Ctrl Pts',(-56.0289353856639,-30.13000002,-61.0621827299711));
#145502=CARTESIAN_POINT('Ctrl Pts',(-53.0072677069205,-30.4880260434848,
-66.1508000801069));
#145503=CARTESIAN_POINT('Ctrl Pts',(-53.1140955473737,-30.1300000200305,
-66.1737552088486));
#145504=CARTESIAN_POINT('Ctrl Pts',(-53.4376477846732,-30.13000002,-66.3621114555649));
#145505=CARTESIAN_POINT('Ctrl Pts',(-50.405384759569,-30.4815921581836,
-71.4443972343972));
#145506=CARTESIAN_POINT('Ctrl Pts',(-50.518482898395,-30.13000002,-71.4624685012804));
#145507=CARTESIAN_POINT('Ctrl Pts',(-50.8336218773704,-30.13000002,-71.655706365272));
#145508=CARTESIAN_POINT('Ctrl Pts',(-45.1629315870884,-30.4666308723541,
-82.01174695052));
#145509=CARTESIAN_POINT('Ctrl Pts',(-45.2819556815256,-30.13000002,-82.0338364947541));
#145510=CARTESIAN_POINT('Ctrl Pts',(-45.5856873606873,-30.13000002,-82.223056081386));
#145511=CARTESIAN_POINT('Ctrl Pts',(-42.5227129344255,-30.4581147715466,
-87.2856833539494));
#145512=CARTESIAN_POINT('Ctrl Pts',(-42.650123001142,-30.13000002,-87.3003867975457));
#145513=CARTESIAN_POINT('Ctrl Pts',(-42.94214612644,-30.13000002,-87.4969984415611));
#145514=CARTESIAN_POINT('Ctrl Pts',(-39.850159149164,-30.447965242174,-92.5429803300057));
#145515=CARTESIAN_POINT('Ctrl Pts',(-39.9609182162754,-30.13000002,-92.5993786427328));
#145516=CARTESIAN_POINT('Ctrl Pts',(-40.2651432342477,-30.13000002,-92.7542894608761));
#145517=CARTESIAN_POINT('Origin',(-40.2651432342477,-30.63000002,-92.754289460876));
#145518=CARTESIAN_POINT('Ctrl Pts',(-39.5006706228584,-30.13000002,-96.1170957262314));
#145519=CARTESIAN_POINT('Ctrl Pts',(-38.9951731461558,-30.13000002,-96.1239966937518));
#145520=CARTESIAN_POINT('Ctrl Pts',(-39.0007459084378,-30.6355158392231,
-96.123928310321));
#145521=CARTESIAN_POINT('Ctrl Pts',(-39.4926444736916,-30.13000002,-95.5146217937464));
#145522=CARTESIAN_POINT('Ctrl Pts',(-39.018727596565,-30.1300000199999,
-95.5002240857988));
#145523=CARTESIAN_POINT('Ctrl Pts',(-38.9918233137184,-30.6029340469193,
-95.4804746285911));
#145524=CARTESIAN_POINT('Ctrl Pts',(-39.5567080597613,-30.13000002,-94.9242583718701));
#145525=CARTESIAN_POINT('Ctrl Pts',(-39.1128426389465,-30.13000002,-94.8742326636326));
#145526=CARTESIAN_POINT('Ctrl Pts',(-39.0630015628091,-30.5704212349622,
-94.8509849588091));
#145527=CARTESIAN_POINT('Ctrl Pts',(-39.824074198694,-30.13000002,-93.7675786356602));
#145528=CARTESIAN_POINT('Ctrl Pts',(-39.4497207067778,-30.13000002,-93.6636460107682));
#145529=CARTESIAN_POINT('Ctrl Pts',(-39.3600684015271,-30.5057885431007,
-93.6194738625269));
#145530=CARTESIAN_POINT('Ctrl Pts',(-40.0302908384928,-30.13000002,-93.1965579604184));
#145531=CARTESIAN_POINT('Ctrl Pts',(-39.6888362216248,-30.13000002,-93.0681539889851));
#145532=CARTESIAN_POINT('Ctrl Pts',(-39.5891998109869,-30.4733919576177,
-93.0124665383103));
#145533=CARTESIAN_POINT('Ctrl Pts',(-40.3113967419659,-30.13000002,-92.6651768309653));
#145534=CARTESIAN_POINT('Ctrl Pts',(-40.0131400269601,-30.13000002,-92.5073906291708));
#145535=CARTESIAN_POINT('Ctrl Pts',(-39.9015329389956,-30.4429085637657,
-92.4483628961121));
#145536=CARTESIAN_POINT('Origin',(-39.5,-30.63000002,-96.0164973302555));
#145537=CARTESIAN_POINT('Origin',(-39.5,-30.63000002,-55.24995));
#145538=CARTESIAN_POINT('',(-39.,-30.63000002,-136.04214564125));
#145539=CARTESIAN_POINT('Origin',(-39.5,-30.63000002,-136.04214564125));
#145540=CARTESIAN_POINT('',(-39.,-30.63000002,-129.34995));
#145541=CARTESIAN_POINT('Ctrl Pts',(-40.2651432342477,-30.13000002,-139.30435351063));
#145542=CARTESIAN_POINT('Ctrl Pts',(-39.9609182162754,-30.13000002,-139.459264328773));
#145543=CARTESIAN_POINT('Ctrl Pts',(-39.850159149164,-30.447965242174,-139.5156626415));
#145544=CARTESIAN_POINT('Ctrl Pts',(-40.0075294671789,-30.13000002,-138.798433034953));
#145545=CARTESIAN_POINT('Ctrl Pts',(-39.6630612728547,-30.13000002,-138.925676053694));
#145546=CARTESIAN_POINT('Ctrl Pts',(-39.5639348330521,-30.4769451657213,
-138.978519823589));
#145547=CARTESIAN_POINT('Ctrl Pts',(-39.8201451200256,-30.13000002,-138.270288236581));
#145548=CARTESIAN_POINT('Ctrl Pts',(-39.4450625268456,-30.13000002,-138.37488926852));
#145549=CARTESIAN_POINT('Ctrl Pts',(-39.3557167999464,-30.5068849023477,
-138.41703103581));
#145550=CARTESIAN_POINT('Ctrl Pts',(-39.5656143592083,-30.13000002,-137.176619865119));
#145551=CARTESIAN_POINT('Ctrl Pts',(-39.1248051359359,-30.13000002,-137.23047141255));
#145552=CARTESIAN_POINT('Ctrl Pts',(-39.0729048436467,-30.5680016657979,
-137.252632910085));
#145553=CARTESIAN_POINT('Ctrl Pts',(-39.5000000014551,-30.13000002,-136.607413315277));
#145554=CARTESIAN_POINT('Ctrl Pts',(-39.0297176446585,-30.13000002,-136.627803193949));
#145555=CARTESIAN_POINT('Ctrl Pts',(-39.,-30.5993710675033,-136.645762741564));
#145556=CARTESIAN_POINT('Ctrl Pts',(-39.5,-30.13000002,-136.04214564125));
#145557=CARTESIAN_POINT('Ctrl Pts',(-39.,-30.13000002,-136.04214564125));
#145558=CARTESIAN_POINT('Ctrl Pts',(-39.,-30.63000002,-136.04214564125));
#145559=CARTESIAN_POINT('',(-39.850159149164,-30.447965242174,-139.5156626415));
#145560=CARTESIAN_POINT('Origin',(-40.2651432342477,-30.63000002,-139.30435351063));
#145561=CARTESIAN_POINT('Ctrl Pts',(-39.8501336361171,-30.4479678253678,
-139.515614761992));
#145562=CARTESIAN_POINT('Ctrl Pts',(-39.5639224597867,-30.4769469448861,
-138.978486457187));
#145563=CARTESIAN_POINT('Ctrl Pts',(-39.3557125984323,-30.5068858103113,
-138.417013737266));
#145564=CARTESIAN_POINT('Ctrl Pts',(-39.0729048436467,-30.5680016657979,
-137.252632910085));
#145565=CARTESIAN_POINT('Ctrl Pts',(-39.,-30.5993710675033,-136.645762741564));
#145566=CARTESIAN_POINT('Ctrl Pts',(-39.,-30.63000002,-136.04214564125));
#145567=CARTESIAN_POINT('Ctrl Pts',(-39.850159149164,-30.447965242174,-139.5156626415));
#145568=CARTESIAN_POINT('Ctrl Pts',(-39.9609182162754,-30.1300000199999,
-139.459264328773));
#145569=CARTESIAN_POINT('Ctrl Pts',(-40.2651432342477,-30.13000002,-139.30435351063));
#145570=CARTESIAN_POINT('Ctrl Pts',(-42.5429900246349,-30.4581917776324,
-144.812847565038));
#145571=CARTESIAN_POINT('Ctrl Pts',(-42.6706800009636,-30.13000002,-144.798763083095));
#145572=CARTESIAN_POINT('Ctrl Pts',(-42.9624569131523,-30.13000002,-144.601532315192));
#145573=CARTESIAN_POINT('Ctrl Pts',(-45.2030035072277,-30.4667604203174,
-150.126917764117));
#145574=CARTESIAN_POINT('Ctrl Pts',(-45.3221739986871,-30.1300000200307,
-150.105257848785));
#145575=CARTESIAN_POINT('Ctrl Pts',(-45.6258101137111,-30.13000002,-149.91560863326));
#145576=CARTESIAN_POINT('Ctrl Pts',(-50.484627394531,-30.4818027714,-160.774746655264));
#145577=CARTESIAN_POINT('Ctrl Pts',(-50.5978344679358,-30.1300000199689,
-160.757133407541));
#145578=CARTESIAN_POINT('Ctrl Pts',(-50.9129382266982,-30.13000002,-160.563437524381));
#145579=CARTESIAN_POINT('Ctrl Pts',(-53.105875183067,-30.4882648083968,
-166.108694936931));
#145580=CARTESIAN_POINT('Ctrl Pts',(-53.2127313470812,-30.1300000198871,
-166.08608254617));
#145581=CARTESIAN_POINT('Ctrl Pts',(-53.53633422979,-30.13000002,-165.897383514726));
#145582=CARTESIAN_POINT('Ctrl Pts',(-55.7146117108563,-30.4940179634924,
-171.449026400902));
#145583=CARTESIAN_POINT('Ctrl Pts',(-55.8070372118623,-30.13000002,-171.403845487572));
#145584=CARTESIAN_POINT('Ctrl Pts',(-56.1468816861249,-30.13000002,-171.237717270032));
#145585=CARTESIAN_POINT('',(-55.7146117108563,-30.4940179634924,-171.449026400902));
#145586=CARTESIAN_POINT('Origin',(-56.146881686125,-30.63000002,-171.237717270032));
#145587=CARTESIAN_POINT('Ctrl Pts',(-55.7146117108563,-30.4940179634924,
-171.449026400902));
#145588=CARTESIAN_POINT('Ctrl Pts',(-53.105875183067,-30.4882648083968,
-166.108694936931));
#145589=CARTESIAN_POINT('Ctrl Pts',(-50.484627394531,-30.4818027714,-160.774746655264));
#145590=CARTESIAN_POINT('Ctrl Pts',(-45.2030035072277,-30.4667604203174,
-150.126917764117));
#145591=CARTESIAN_POINT('Ctrl Pts',(-42.5429900246349,-30.4581917776324,
-144.812847565038));
#145592=CARTESIAN_POINT('Ctrl Pts',(-39.850159149164,-30.447965242174,-139.5156626415));
#145593=CARTESIAN_POINT('Ctrl Pts',(-55.6935671754689,-30.4968373543262,
-171.410008924778));
#145594=CARTESIAN_POINT('Ctrl Pts',(-55.7825352402592,-30.1299356988045,
-171.361452749053));
#145595=CARTESIAN_POINT('Ctrl Pts',(-56.1167176003611,-30.1300000271399,
-171.179145966886));
#145596=CARTESIAN_POINT('Ctrl Pts',(-55.7814946229066,-30.4850537049709,
-171.564548662911));
#145597=CARTESIAN_POINT('Ctrl Pts',(-55.8840206261747,-30.1299383387469,
-171.527291609574));
#145598=CARTESIAN_POINT('Ctrl Pts',(-56.2430624746474,-30.1300000269106,
-171.410992898787));
#145599=CARTESIAN_POINT('Ctrl Pts',(-55.8246219322658,-30.4793202225602,
-171.737832654878));
#145600=CARTESIAN_POINT('Ctrl Pts',(-55.9360241189749,-30.1299395985436,
-171.722483207042));
#145601=CARTESIAN_POINT('Ctrl Pts',(-56.3050537145652,-30.130000026799,
-171.670900042786));
#145602=CARTESIAN_POINT('Ctrl Pts',(-55.8160539307423,-30.4804600576221,
-171.916099630748));
#145603=CARTESIAN_POINT('Ctrl Pts',(-55.925777764091,-30.1299393505852,
-171.921245295793));
#145604=CARTESIAN_POINT('Ctrl Pts',(-56.2927384034373,-30.1300000268212,
-171.938334598151));
#145605=CARTESIAN_POINT('Origin',(-56.294192362543,-30.63000002,-171.871644662643));
#145606=CARTESIAN_POINT('Origin',(-54.6808724388942,-30.6336549073814,-171.881456078396));
#145607=CARTESIAN_POINT('Origin',(-56.294192362543,-30.63000002,-179.64995));
#145608=CARTESIAN_POINT('Origin',(-56.294192362543,-30.63000002,-176.84995));
#145609=CARTESIAN_POINT('Origin',(83.2809572255632,-29.6300000199999,-176.84995));
#145610=CARTESIAN_POINT('',(-57.,-29.63000002,-177.34995));
#145611=CARTESIAN_POINT('Origin',(-57.,-29.63000002,-176.84995));
#145612=CARTESIAN_POINT('',(-56.5982428503831,-29.63000002,-177.34995));
#145613=CARTESIAN_POINT('',(-60.,-29.63000002,-177.34995));
#145614=CARTESIAN_POINT('Ctrl Pts',(-56.294192362543,-30.13000002,-176.84995));
#145615=CARTESIAN_POINT('Ctrl Pts',(-56.2941923707649,-30.1300000200003,
-176.98587944854));
#145616=CARTESIAN_POINT('Ctrl Pts',(-56.3301688951883,-30.0730055436657,
-177.116037754475));
#145617=CARTESIAN_POINT('Ctrl Pts',(-56.4164036466448,-29.9329688836733,
-177.253030654974));
#145618=CARTESIAN_POINT('Ctrl Pts',(-56.4500227583409,-29.8779487295679,
-177.288930648015));
#145619=CARTESIAN_POINT('Ctrl Pts',(-56.5223271856603,-29.7580969359688,
-177.337570500007));
#145620=CARTESIAN_POINT('Ctrl Pts',(-56.5603834356575,-29.6942993846806,
-177.34995));
#145621=CARTESIAN_POINT('Ctrl Pts',(-56.5982428503831,-29.63000002,-177.34995));
#145622=CARTESIAN_POINT('Origin',(-57.,-29.63000002,-174.34995));
#145623=CARTESIAN_POINT('',(-60.,-29.63000002,-174.34995));
#145624=CARTESIAN_POINT('Origin',(-59.5,-29.63000002,-174.34995));
#145625=CARTESIAN_POINT('Origin',(-57.,-29.63000002,-174.34995));
#145626=CARTESIAN_POINT('Origin',(-59.5,-29.63000002,-55.24995));
#145627=CARTESIAN_POINT('',(-60.,-29.63000002,-58.24995));
#145628=CARTESIAN_POINT('Origin',(-59.5,-29.63000002,-58.24995));
#145629=CARTESIAN_POINT('',(-60.,-29.63000002,-174.34995));
#145630=CARTESIAN_POINT('Origin',(-57.,-29.63000002,-58.24995));
#145631=CARTESIAN_POINT('Origin',(-57.,-29.63000002,-58.24995));
#145632=CARTESIAN_POINT('Origin',(-57.,-2.42462934179819E-14,-58.24995));
#145633=CARTESIAN_POINT('',(-60.,-29.13000002,-58.24995));
#145634=CARTESIAN_POINT('Origin',(-57.,-29.13000002,-58.24995));
#145635=CARTESIAN_POINT('',(-60.,-54.58000002,-58.24995));
#145636=CARTESIAN_POINT('Origin',(-57.,-29.13000002,-58.24995));
#145637=CARTESIAN_POINT('Origin',(-59.5,-29.13000002,-58.24995));
#145638=CARTESIAN_POINT('Ctrl Pts',(-39.7602371906926,-27.9700232578782,
-94.7283182364936));
#145639=CARTESIAN_POINT('Ctrl Pts',(-39.5607615517246,-28.6300000199999,
-94.628899882694));
#145640=CARTESIAN_POINT('Ctrl Pts',(-40.1842134716234,-28.63000002,-94.9396273673639));
#145641=CARTESIAN_POINT('Ctrl Pts',(-42.5604321400969,-27.9797945689722,
-89.1025347299149));
#145642=CARTESIAN_POINT('Ctrl Pts',(-42.3373257946448,-28.63000002,-89.0914456452771));
#145643=CARTESIAN_POINT('Ctrl Pts',(-42.9880924510224,-28.63000002,-89.3138497353063));
#145644=CARTESIAN_POINT('Ctrl Pts',(-45.3330806261701,-27.9878402480233,
-83.4627911786917));
#145645=CARTESIAN_POINT('Ctrl Pts',(-45.1354691768678,-28.630000020022,
-83.4336169877673));
#145646=CARTESIAN_POINT('Ctrl Pts',(-45.7634210292322,-28.63000002,-83.6741003095587));
#145647=CARTESIAN_POINT('Ctrl Pts',(-50.8469740031289,-28.0018438144725,
-72.1674540521641));
#145648=CARTESIAN_POINT('Ctrl Pts',(-50.6710028559025,-28.6300000199784,
-72.148355955617));
#145649=CARTESIAN_POINT('Ctrl Pts',(-51.2816902902029,-28.63000002,-72.3787631830378));
#145650=CARTESIAN_POINT('Ctrl Pts',(-53.5878832423525,-28.0077864042225,
-66.5116884426403));
#145651=CARTESIAN_POINT('Ctrl Pts',(-53.4278489247074,-28.6300000200659,
-66.4825194498726));
#145652=CARTESIAN_POINT('Ctrl Pts',(-54.0242786911866,-28.63000002,-66.7229996739341));
#145653=CARTESIAN_POINT('Ctrl Pts',(-56.3187331343194,-28.0130417005584,
-60.8508735991007));
#145654=CARTESIAN_POINT('Ctrl Pts',(-56.1850547298497,-28.63000002,-60.7863522634768));
#145655=CARTESIAN_POINT('Ctrl Pts',(-56.7565335485771,-28.63000002,-61.0621827299711));
#145656=CARTESIAN_POINT('Origin',(-40.1842134716234,-28.13000002,-94.9396273673639));
#145657=CARTESIAN_POINT('Origin',(-59.5,-29.13000002,-55.24995));
#145658=CARTESIAN_POINT('',(-60.,-29.13000002,-174.34995));
#145659=CARTESIAN_POINT('Origin',(-59.5,-29.13000002,-174.34995));
#145660=CARTESIAN_POINT('',(-60.,-29.13000002,-58.24995));
#145661=CARTESIAN_POINT('Origin',(-57.,-29.13000002,-174.34995));
#145662=CARTESIAN_POINT('',(-57.,-29.13000002,-177.34995));
#145663=CARTESIAN_POINT('',(-57.,-28.664523125878,-177.032518510534));
#145664=CARTESIAN_POINT('Origin',(-57.,-29.13000002,-176.84995));
#145665=CARTESIAN_POINT('Origin',(-57.,-29.13000002,-174.34995));
#145666=CARTESIAN_POINT('Ctrl Pts',(-57.,-28.664523125878,-177.032518510534));
#145667=CARTESIAN_POINT('Ctrl Pts',(-57.0114676733044,-28.6416054347749,
-176.974087537723));
#145668=CARTESIAN_POINT('Ctrl Pts',(-57.0179413444383,-28.63000002,-176.912963832989));
#145669=CARTESIAN_POINT('Ctrl Pts',(-57.0184057454332,-28.63000002,-176.849882244789));
#145670=CARTESIAN_POINT('Origin',(-57.0184057454332,-28.13000002,-179.64995));
#145671=CARTESIAN_POINT('Origin',(-57.0184057454332,-28.13000002,-171.871644662643));
#145672=CARTESIAN_POINT('Origin',(-57.0184057454332,-28.13000002,-176.849882244789));
#145673=CARTESIAN_POINT('Ctrl Pts',(-56.5341822214496,-28.0016231613287,
-171.915549358366));
#145674=CARTESIAN_POINT('Ctrl Pts',(-56.3674234002834,-28.6301310958619,
-171.907871533399));
#145675=CARTESIAN_POINT('Ctrl Pts',(-57.0170289507251,-28.6300000098419,
-171.937510237498));
#145676=CARTESIAN_POINT('Ctrl Pts',(-56.5423215389878,-28.0006714526254,
-171.739685194435));
#145677=CARTESIAN_POINT('Ctrl Pts',(-56.3722793953445,-28.6301314641988,
-171.762633256233));
#145678=CARTESIAN_POINT('Ctrl Pts',(-57.0288581213359,-28.6300000098265,
-171.673675468004));
#145679=CARTESIAN_POINT('Ctrl Pts',(-56.5015214234675,-28.0054385079109,
-171.56638157453));
#145680=CARTESIAN_POINT('Ctrl Pts',(-56.3485431365434,-28.6301296243107,
-171.621528645646));
#145681=CARTESIAN_POINT('Ctrl Pts',(-56.9695606031425,-28.6300000099035,
-171.413737441436));
#145682=CARTESIAN_POINT('Ctrl Pts',(-56.4142663415167,-28.0157208016423,
-171.409463522487));
#145683=CARTESIAN_POINT('Ctrl Pts',(-56.287357164279,-28.6301257916421,
-171.477955081175));
#145684=CARTESIAN_POINT('Ctrl Pts',(-56.8427717751314,-28.6300000100697,
-171.178320644756));
#145685=CARTESIAN_POINT('',(-56.4351108624337,-28.0132652467914,-171.449026400902));
#145686=CARTESIAN_POINT('Origin',(-56.8729709358987,-28.13000002,-171.237717270032));
#145687=CARTESIAN_POINT('Origin',(-55.1751592863144,-28.1616555077833,-171.933533580786));
#145688=CARTESIAN_POINT('Ctrl Pts',(-56.4351108624337,-28.0132652467914,
-171.449026400902));
#145689=CARTESIAN_POINT('Ctrl Pts',(-56.3017476121307,-28.63000002,-171.51338685352));
#145690=CARTESIAN_POINT('Ctrl Pts',(-56.8729709358987,-28.63000002,-171.237717270032));
#145691=CARTESIAN_POINT('Ctrl Pts',(-53.6851592779725,-28.007992698407,
-165.747855383941));
#145692=CARTESIAN_POINT('Ctrl Pts',(-53.5252373050999,-28.6300000202211,
-165.776484176476));
#145693=CARTESIAN_POINT('Ctrl Pts',(-54.1216126416942,-28.63000002,-165.536544112802));
#145694=CARTESIAN_POINT('Ctrl Pts',(-50.9250693333912,-28.0020271923581,
-160.051772415584));
#145695=CARTESIAN_POINT('Ctrl Pts',(-50.7490667135706,-28.63000002,-160.070107012222));
#145696=CARTESIAN_POINT('Ctrl Pts',(-51.3598402340296,-28.63000002,-159.840463284713));
#145697=CARTESIAN_POINT('Ctrl Pts',(-45.3724783922449,-27.9879549525026,
-148.675968242465));
#145698=CARTESIAN_POINT('Ctrl Pts',(-45.1747354310855,-28.63000002,-148.704407489125));
#145699=CARTESIAN_POINT('Ctrl Pts',(-45.8028572712098,-28.63000002,-148.464659111595));
#145700=CARTESIAN_POINT('Ctrl Pts',(-42.5803228338128,-27.9798639777307,
-142.996070008035));
#145701=CARTESIAN_POINT('Ctrl Pts',(-42.3567693699165,-28.6300000199999,
-143.005974713683));
#145702=CARTESIAN_POINT('Ctrl Pts',(-43.0080092605004,-28.63000002,-142.784754854138));
#145703=CARTESIAN_POINT('Ctrl Pts',(-39.7602371906926,-27.9700232578782,
-137.330324735012));
#145704=CARTESIAN_POINT('Ctrl Pts',(-39.5607615517247,-28.63000002,-137.429743088812));
#145705=CARTESIAN_POINT('Ctrl Pts',(-40.1842134716234,-28.63000002,-137.119015604142));
#145706=CARTESIAN_POINT('',(-39.7602371906121,-27.9700232581448,-137.330324735053));
#145707=CARTESIAN_POINT('Origin',(-40.1842134716235,-28.13000002,-137.119015604142));
#145708=CARTESIAN_POINT('Ctrl Pts',(-39.7602371906927,-27.9700232578782,
-137.330324735012));
#145709=CARTESIAN_POINT('Ctrl Pts',(-42.5803228332686,-27.9798639793132,
-142.996070008059));
#145710=CARTESIAN_POINT('Ctrl Pts',(-45.3724783917581,-27.9879549540833,
-148.675968242535));
#145711=CARTESIAN_POINT('Ctrl Pts',(-50.9250693329494,-28.0020271939342,
-160.051772415631));
#145712=CARTESIAN_POINT('Ctrl Pts',(-53.6851592775679,-28.0079926999806,
-165.747855384014));
#145713=CARTESIAN_POINT('Ctrl Pts',(-56.4351108624337,-28.0132652467914,
-171.449026400902));
#145714=CARTESIAN_POINT('Ctrl Pts',(-39.5,-28.63000002,-134.169022080262));
#145715=CARTESIAN_POINT('Ctrl Pts',(-39.,-28.63000002,-134.169022080263));
#145716=CARTESIAN_POINT('Ctrl Pts',(-39.,-28.13000002,-134.169022080262));
#145717=CARTESIAN_POINT('Ctrl Pts',(-39.500000002646,-28.63000002,-134.681913680777));
#145718=CARTESIAN_POINT('Ctrl Pts',(-38.9725065924499,-28.63000002,-134.735408648257));
#145719=CARTESIAN_POINT('Ctrl Pts',(-39.,-28.1032444606982,-134.720208320017));
#145720=CARTESIAN_POINT('Ctrl Pts',(-39.5577923442835,-28.63000002,-135.185082649765));
#145721=CARTESIAN_POINT('Ctrl Pts',(-39.0091060618314,-28.6300000199999,
-135.282961361938));
#145722=CARTESIAN_POINT('Ctrl Pts',(-39.0642137165569,-28.076417661445,
-135.260142317137));
#145723=CARTESIAN_POINT('Ctrl Pts',(-39.7843604313674,-28.63000002,-136.172328627912));
#145724=CARTESIAN_POINT('Ctrl Pts',(-39.1926311399543,-28.63000002,-136.37231025087));
#145725=CARTESIAN_POINT('Ctrl Pts',(-39.3159560341664,-28.0228058044255,
-136.318039323049));
#145726=CARTESIAN_POINT('Ctrl Pts',(-39.9554204749436,-28.63000002,-136.659959223536));
#145727=CARTESIAN_POINT('Ctrl Pts',(-39.3499007457719,-28.63000002,-136.920217264961));
#145728=CARTESIAN_POINT('Ctrl Pts',(-39.5060247583741,-27.995814073424,
-136.839791694484));
#145729=CARTESIAN_POINT('Ctrl Pts',(-40.1842134716234,-28.63000002,-137.119015604142));
#145730=CARTESIAN_POINT('Ctrl Pts',(-39.5607615517247,-28.63000002,-137.429743088812));
#145731=CARTESIAN_POINT('Ctrl Pts',(-39.7602371906926,-27.9700232578782,
-137.330324735012));
#145732=CARTESIAN_POINT('',(-39.0000000005543,-28.13000002,-134.169022080262));
#145733=CARTESIAN_POINT('Origin',(-39.5,-28.13000002,-134.169022080262));
#145734=CARTESIAN_POINT('Ctrl Pts',(-39.,-28.13000002,-134.169022080262));
#145735=CARTESIAN_POINT('Ctrl Pts',(-38.9999999999924,-28.1032444608434,
-134.720208320021));
#145736=CARTESIAN_POINT('Ctrl Pts',(-39.0642137165422,-28.0764176615931,
-135.260142317143));
#145737=CARTESIAN_POINT('Ctrl Pts',(-39.3159560341354,-28.0228058045779,
-136.318039323063));
#145738=CARTESIAN_POINT('Ctrl Pts',(-39.5060247583362,-27.9958140735776,
-136.839791694503));
#145739=CARTESIAN_POINT('Ctrl Pts',(-39.7602371906927,-27.9700232578782,
-137.330324735012));
#145740=CARTESIAN_POINT('Origin',(-39.5,-28.13000002,-55.24995));
#145741=CARTESIAN_POINT('',(-39.,-28.13000002,-97.8896208912436));
#145742=CARTESIAN_POINT('Origin',(-39.5,-28.13000002,-97.8896208912436));
#145743=CARTESIAN_POINT('',(-39.,-28.13000002,-129.34995));
#145744=CARTESIAN_POINT('Ctrl Pts',(-40.2462900890831,-28.63000002,-94.8183794182931));
#145745=CARTESIAN_POINT('Ctrl Pts',(-39.6202740741427,-28.6300000199999,
-94.4888005385705));
#145746=CARTESIAN_POINT('Ctrl Pts',(-39.829240962964,-27.9630991838752,
-94.598792800159));
#145747=CARTESIAN_POINT('Ctrl Pts',(-39.9855126261077,-28.63000002,-95.3144293640507));
#145748=CARTESIAN_POINT('Ctrl Pts',(-39.3786468753042,-28.6300000200001,
-95.0400168527107));
#145749=CARTESIAN_POINT('Ctrl Pts',(-39.5394940969938,-27.9910419130939,
-95.1287084620502));
#145750=CARTESIAN_POINT('Ctrl Pts',(-39.7974846477126,-28.63000002,-95.8327740427122));
#145751=CARTESIAN_POINT('Ctrl Pts',(-39.2039361117733,-28.63000002,-95.6237032606678));
#145752=CARTESIAN_POINT('Ctrl Pts',(-39.3305596959349,-28.0197890414477,
-95.6832525232954));
#145753=CARTESIAN_POINT('Ctrl Pts',(-39.5490809018585,-28.63000002,-96.907936854151));
#145754=CARTESIAN_POINT('Ctrl Pts',(-39.0023017017761,-28.63000002,-96.8105692004775));
#145755=CARTESIAN_POINT('Ctrl Pts',(-39.054543707667,-28.078192313553,-96.8353311856082));
#145756=CARTESIAN_POINT('Ctrl Pts',(-39.4899744060911,-28.63000002,-97.4691620834926));
#145757=CARTESIAN_POINT('Ctrl Pts',(-38.9664569591492,-28.630000020001,
-97.4208997464886));
#145758=CARTESIAN_POINT('Ctrl Pts',(-38.9888645974602,-28.1080699462563,
-97.4376221179531));
#145759=CARTESIAN_POINT('Ctrl Pts',(-39.501388445999,-28.63000002,-98.0251051604236));
#145760=CARTESIAN_POINT('Ctrl Pts',(-39.0084033239769,-28.6300000199997,
-98.0351337801891));
#145761=CARTESIAN_POINT('Ctrl Pts',(-39.0015413990503,-28.1369597759577,
-98.0352430155923));
#145762=CARTESIAN_POINT('Ctrl Pts',(-39.760237187334,-27.9700232996177,
-94.7283182916262));
#145763=CARTESIAN_POINT('Ctrl Pts',(-39.7044170752792,-27.9756864894409,
-94.8360299998448));
#145764=CARTESIAN_POINT('Ctrl Pts',(-39.6518994857077,-27.9814177835746,
-94.9447812612047));
#145765=CARTESIAN_POINT('Ctrl Pts',(-39.6025567448821,-27.9871721516943,
-95.0544919306715));
#145766=CARTESIAN_POINT('Ctrl Pts',(-39.5517891646793,-27.9930926850929,
-95.167370646326));
#145767=CARTESIAN_POINT('Ctrl Pts',(-39.5043816087621,-27.9990379606581,
-95.2812653110876));
#145768=CARTESIAN_POINT('Ctrl Pts',(-39.4602180947879,-28.0049899521968,
-95.3961280885268));
#145769=CARTESIAN_POINT('Ctrl Pts',(-39.4155272969176,-28.0110130066788,
-95.5123622535062));
#145770=CARTESIAN_POINT('Ctrl Pts',(-39.3741578024,-28.0170434313907,-95.6295883656512));
#145771=CARTESIAN_POINT('Ctrl Pts',(-39.3360241014405,-28.0230875256045,
-95.7477895402997));
#145772=CARTESIAN_POINT('Ctrl Pts',(-39.2974753811385,-28.0291973993243,
-95.8672771301809));
#145773=CARTESIAN_POINT('Ctrl Pts',(-39.2622327498326,-28.0353218042364,
-95.9877618235928));
#145774=CARTESIAN_POINT('Ctrl Pts',(-39.2302521220656,-28.041484578967,
-96.1092496303843));
#145775=CARTESIAN_POINT('Ctrl Pts',(-39.2171315325446,-28.044012960778,
-96.1590920429952));
#145776=CARTESIAN_POINT('Ctrl Pts',(-39.2045605552519,-28.0465479531573,
-96.2091035093114));
#145777=CARTESIAN_POINT('Ctrl Pts',(-39.1925385381225,-28.0490916877327,
-96.2592851281618));
#145778=CARTESIAN_POINT('Ctrl Pts',(-39.1566966697309,-28.0566754566536,
-96.4088942128223));
#145779=CARTESIAN_POINT('Ctrl Pts',(-39.1256874125126,-28.0643165321069,
-96.5602560280547));
#145780=CARTESIAN_POINT('Ctrl Pts',(-39.0996770774813,-28.0719711520587,
-96.7128532814895));
#145781=CARTESIAN_POINT('Ctrl Pts',(-39.0738134555235,-28.0795825956031,
-96.8645897996801));
#145782=CARTESIAN_POINT('Ctrl Pts',(-39.052892611788,-28.0872070957307,
-97.0175476213926));
#145783=CARTESIAN_POINT('Ctrl Pts',(-39.0370318360345,-28.0948111078542,
-97.1711980730793));
#145784=CARTESIAN_POINT('Ctrl Pts',(-39.0213056660934,-28.1023505869281,
-97.3235445378627));
#145785=CARTESIAN_POINT('Ctrl Pts',(-39.010554075202,-28.1098696306334,
-97.4765716712978));
#145786=CARTESIAN_POINT('Ctrl Pts',(-39.004844939737,-28.1173495596137,
-97.6297480128119));
#145787=CARTESIAN_POINT('Ctrl Pts',(-39.0016168605909,-28.1215788869617,
-97.7163575102999));
#145788=CARTESIAN_POINT('Ctrl Pts',(-39.0000000254363,-28.1257959890489,
-97.803014437355));
#145789=CARTESIAN_POINT('Ctrl Pts',(-39.0000000000003,-28.13000002,-97.8896208912436));
#145790=CARTESIAN_POINT('Ctrl Pts',(-39.,-29.6093496431988,-96.8114293882212));
#145791=CARTESIAN_POINT('Ctrl Pts',(-39.,-28.741729147553,-95.6677964063875));
#145792=CARTESIAN_POINT('Ctrl Pts',(-39.7614971661825,-28.0062467616585,
-94.6983380795177));
#145793=CARTESIAN_POINT('Ctrl Pts',(-39.,-29.0535677480794,-97.2330749436175));
#145794=CARTESIAN_POINT('Ctrl Pts',(-39.,-28.2134674407351,-96.0912283932403));
#145795=CARTESIAN_POINT('Ctrl Pts',(-39.7437819827477,-27.4973039569491,
-95.1199826758911));
#145796=CARTESIAN_POINT('Ctrl Pts',(-39.,-28.4877143439141,-97.6439384126816));
#145797=CARTESIAN_POINT('Ctrl Pts',(-39.,-27.6753857963049,-96.504280291422));
#145798=CARTESIAN_POINT('Ctrl Pts',(-39.7262969548998,-26.9800167700376,
-95.5308471039398));
#145799=CARTESIAN_POINT('Ctrl Pts',(-39.,-27.3325353334211,-98.4405542704251));
#145800=CARTESIAN_POINT('Ctrl Pts',(-39.,-26.5774575077333,-97.3050952674327));
#145801=CARTESIAN_POINT('Ctrl Pts',(-39.6919956601185,-25.9258412309992,
-96.3274629617598));
#145802=CARTESIAN_POINT('Ctrl Pts',(-39.,-26.741479037393,-98.8273374953048));
#145803=CARTESIAN_POINT('Ctrl Pts',(-39.,-26.0159584590169,-97.6939770973016));
#145804=CARTESIAN_POINT('Ctrl Pts',(-39.6751334260609,-25.3873798477126,
-96.7142461865699));
#145805=CARTESIAN_POINT('Ctrl Pts',(-39.,-24.9430461321624,-99.9336024831245));
#145806=CARTESIAN_POINT('Ctrl Pts',(-39.,-24.3098005849941,-98.8051808316371));
#145807=CARTESIAN_POINT('Ctrl Pts',(-39.6263764589698,-23.7517847228855,
-97.8205111744839));
#145808=CARTESIAN_POINT('Ctrl Pts',(-39.,-23.7104174150638,-100.600117065969));
#145809=CARTESIAN_POINT('Ctrl Pts',(-38.9999999999805,-23.1402109105079,
-99.4757726121153));
#145810=CARTESIAN_POINT('Ctrl Pts',(-39.5962627317006,-22.634454054442,
-98.4870223585708));
#145811=CARTESIAN_POINT('Ctrl Pts',(-39.,-22.4346346021703,-101.175614049055));
#145812=CARTESIAN_POINT('Ctrl Pts',(-39.,-21.9292338920902,-100.055223222194));
#145813=CARTESIAN_POINT('Ctrl Pts',(-39.5698473334291,-21.4814334314007,
-99.0625227403511));
#145814=CARTESIAN_POINT('',(-39.,-22.48000002,-101.155103165204));
#145815=CARTESIAN_POINT('Ctrl Pts',(-39.,-22.48000002,-101.155103165204));
#145816=CARTESIAN_POINT('Ctrl Pts',(-39.0000000000003,-23.0421399014201,
-100.900364693921));
#145817=CARTESIAN_POINT('Ctrl Pts',(-39.0000000001808,-23.5949958654236,
-100.62835315127));
#145818=CARTESIAN_POINT('Ctrl Pts',(-39.0000000005377,-24.1395638864485,
-100.340934396651));
#145819=CARTESIAN_POINT('Ctrl Pts',(-39.0000000008113,-24.556943999504,
-100.120644427968));
#145820=CARTESIAN_POINT('Ctrl Pts',(-39.0000000009101,-24.9694552602955,
-99.8913025435703));
#145821=CARTESIAN_POINT('Ctrl Pts',(-39.0000000004916,-25.3775420853185,
-99.6537285981461));
#145822=CARTESIAN_POINT('Ctrl Pts',(-39.0000000002285,-25.6341396980635,
-99.5043463992897));
#145823=CARTESIAN_POINT('Ctrl Pts',(-39.0000000001306,-25.8888446969123,
-99.35177201821));
#145824=CARTESIAN_POINT('Ctrl Pts',(-39.0000000000752,-26.1419870362595,
-99.1960691366333));
#145825=CARTESIAN_POINT('Ctrl Pts',(-39.0000000000073,-26.4522179455434,
-99.005252196827));
#145826=CARTESIAN_POINT('Ctrl Pts',(-39.0000000000056,-26.7601021070991,
-98.8096624723068));
#145827=CARTESIAN_POINT('Ctrl Pts',(-39.0000000000023,-27.0653588164938,
-98.6099244013003));
#145828=CARTESIAN_POINT('Ctrl Pts',(-38.9999999999992,-27.3493059604975,
-98.424129779706));
#145829=CARTESIAN_POINT('Ctrl Pts',(-39.0000000000001,-27.6309803020601,
-98.2347441815219));
#145830=CARTESIAN_POINT('Ctrl Pts',(-39.0000000000002,-27.9101240577928,
-98.0422452092007));
#145831=CARTESIAN_POINT('Ctrl Pts',(-39.0000000000002,-27.9835605023139,
-97.9916030586567));
#145832=CARTESIAN_POINT('Ctrl Pts',(-39.0000000000002,-28.0568495646841,
-97.9407287002963));
#145833=CARTESIAN_POINT('Ctrl Pts',(-39.0000000000003,-28.13000002,-97.8896208912436));
#145834=CARTESIAN_POINT('Ctrl Pts',(-39.,-22.48000002,-101.155103165204));
#145835=CARTESIAN_POINT('Ctrl Pts',(-39.0000000057918,-22.4754395071655,
-101.035865090646));
#145836=CARTESIAN_POINT('Ctrl Pts',(-39.0036588655062,-22.4708531165579,
-100.917240445859));
#145837=CARTESIAN_POINT('Ctrl Pts',(-39.0108683903437,-22.4662513204906,
-100.799247589009));
#145838=CARTESIAN_POINT('Ctrl Pts',(-39.0181431578016,-22.4616078804535,
-100.680186955385));
#145839=CARTESIAN_POINT('Ctrl Pts',(-39.029032762941,-22.4569483804398,
-100.561768681035));
#145840=CARTESIAN_POINT('Ctrl Pts',(-39.0434732513881,-22.4522736097561,
-100.443988180248));
#145841=CARTESIAN_POINT('Ctrl Pts',(-39.0580014482079,-22.4475704455364,
-100.325492306425));
#145842=CARTESIAN_POINT('Ctrl Pts',(-39.076123635818,-22.4428513856762,
-100.2076409891));
#145843=CARTESIAN_POINT('Ctrl Pts',(-39.0978263127888,-22.4381133533492,
-100.09042036964));
#145844=CARTESIAN_POINT('Ctrl Pts',(-39.1130274182268,-22.4347947153274,
-100.008316074474));
#145845=CARTESIAN_POINT('Ctrl Pts',(-39.1299862043444,-22.4314666759937,
-99.9265209885234));
#145846=CARTESIAN_POINT('Ctrl Pts',(-39.1487132156732,-22.4281288757921,
-99.8450316540307));
#145847=CARTESIAN_POINT('Ctrl Pts',(-39.1782377095244,-22.4228665912877,
-99.7165577981164));
#145848=CARTESIAN_POINT('Ctrl Pts',(-39.2122145373374,-22.4175906493126,
-99.5886109020029));
#145849=CARTESIAN_POINT('Ctrl Pts',(-39.2506379380908,-22.41229684322,-99.4616289686943));
#145850=CARTESIAN_POINT('Ctrl Pts',(-39.2887401124853,-22.4070472942733,
-99.3357086265846));
#145851=CARTESIAN_POINT('Ctrl Pts',(-39.3312150950707,-22.4017804193251,
-99.2107375266136));
#145852=CARTESIAN_POINT('Ctrl Pts',(-39.3780123572035,-22.3965150583138,
-99.0871503677225));
#145853=CARTESIAN_POINT('Ctrl Pts',(-39.4243143618565,-22.3913054208491,
-98.96487113716));
#145854=CARTESIAN_POINT('Ctrl Pts',(-39.474847826133,-22.3860975663706,
-98.8439471061793));
#145855=CARTESIAN_POINT('Ctrl Pts',(-39.529516301983,-22.3809282592383,
-98.7248012575205));
#145856=CARTESIAN_POINT('Ctrl Pts',(-39.5495316353077,-22.3790356620202,
-98.6811793376099));
#145857=CARTESIAN_POINT('Ctrl Pts',(-39.5701007714082,-22.3771483895887,
-98.6377957636978));
#145858=CARTESIAN_POINT('Ctrl Pts',(-39.5912172963669,-22.3752687460488,
-98.5946711914791));
#145859=CARTESIAN_POINT('Ctrl Pts',(-57.5245249214072,-22.4066238608121,
-60.8508735991008));
#145860=CARTESIAN_POINT('Ctrl Pts',(-57.5817506954796,-21.98000002,-60.8779152752782));
#145861=CARTESIAN_POINT('Ctrl Pts',(-57.9716987024741,-21.98000002,-61.0621827299711));
#145862=CARTESIAN_POINT('Ctrl Pts',(-51.5741970743562,-22.3992883743679,
-73.4455439799432));
#145863=CARTESIAN_POINT('Ctrl Pts',(-51.6744341991619,-21.980000020072,
-73.3940563428121));
#145864=CARTESIAN_POINT('Ctrl Pts',(-52.0201596782203,-21.98000002,-73.6568689967289));
#145865=CARTESIAN_POINT('Ctrl Pts',(-45.6084483216386,-22.3901517945239,
-86.0327992211263));
#145866=CARTESIAN_POINT('Ctrl Pts',(-45.7509404552383,-21.98000002,-85.9093076925101));
#145867=CARTESIAN_POINT('Ctrl Pts',(-46.0528581107812,-21.98000002,-86.2441334050211));
#145868=CARTESIAN_POINT('Ctrl Pts',(-39.5912209089315,-22.3752378108182,
-98.5946087902654));
#145869=CARTESIAN_POINT('Ctrl Pts',(-39.6675936435968,-21.98000002,-98.6312136095384));
#145870=CARTESIAN_POINT('Ctrl Pts',(-40.032098818038,-21.98000002,-98.8059179211357));
#145871=CARTESIAN_POINT('Origin',(-40.032098818038,-22.4800000199998,-98.8059179211357));
#145872=CARTESIAN_POINT('Ctrl Pts',(-39.5000802079448,-21.98000002,-101.18483134797));
#145873=CARTESIAN_POINT('Ctrl Pts',(-38.9988245498377,-21.98000002,-101.187579451807));
#145874=CARTESIAN_POINT('Ctrl Pts',(-39.0000891720766,-22.4812615520007,
-101.187572533131));
#145875=CARTESIAN_POINT('Ctrl Pts',(-39.4978248085922,-21.98000002,-100.766749896626));
#145876=CARTESIAN_POINT('Ctrl Pts',(-39.0135806132542,-21.98000002,-100.738591066592));
#145877=CARTESIAN_POINT('Ctrl Pts',(-38.9975824433844,-22.4638259428356,
-100.730929118733));
#145878=CARTESIAN_POINT('Ctrl Pts',(-39.5431523621162,-21.98000002,-100.356681579714));
#145879=CARTESIAN_POINT('Ctrl Pts',(-39.0782818391802,-21.9800000199993,
-100.29429926997));
#145880=CARTESIAN_POINT('Ctrl Pts',(-39.047945770245,-22.4461087815554,
-100.283504254757));
#145881=CARTESIAN_POINT('Ctrl Pts',(-39.7245173679265,-21.98000002,-99.5521100005686));
#145882=CARTESIAN_POINT('Ctrl Pts',(-39.3065757091719,-21.9800000200007,
-99.4303875276426));
#145883=CARTESIAN_POINT('Ctrl Pts',(-39.2494612149797,-22.4101874992009,
-99.4065735026009));
#145884=CARTESIAN_POINT('Ctrl Pts',(-39.862287275171,-21.98000002,-99.1549631973435));
#145885=CARTESIAN_POINT('Ctrl Pts',(-39.4691358483957,-21.9800000199999,
-99.0065780221483));
#145886=CARTESIAN_POINT('Ctrl Pts',(-39.402539249954,-22.3918503540147,
-98.9741976287182));
#145887=CARTESIAN_POINT('Ctrl Pts',(-40.0449984320234,-21.98000002,-98.7791972647193));
#145888=CARTESIAN_POINT('Ctrl Pts',(-39.6824251849823,-21.9800000199999,
-98.6029227401544));
#145889=CARTESIAN_POINT('Ctrl Pts',(-39.6055502466993,-22.3739864322111,
-98.5655472422949));
#145890=CARTESIAN_POINT('Origin',(-39.5,-22.48000002,-101.155103165204));
#145891=CARTESIAN_POINT('Origin',(-39.5,-22.48000002,-55.24995));
#145892=CARTESIAN_POINT('',(-39.,-22.48000002,-130.903539806302));
#145893=CARTESIAN_POINT('Origin',(-39.5,-22.48000002,-130.903539806302));
#145894=CARTESIAN_POINT('',(-39.,-22.48000002,-129.34995));
#145895=CARTESIAN_POINT('Ctrl Pts',(-40.0320988180411,-21.98000002,-133.252725050377));
#145896=CARTESIAN_POINT('Ctrl Pts',(-39.6675936435998,-21.98000002,-133.427429361974));
#145897=CARTESIAN_POINT('Ctrl Pts',(-39.5912209089345,-22.3752378108182,
-133.464034181247));
#145898=CARTESIAN_POINT('Ctrl Pts',(-39.8558398148562,-21.98000002,-132.884976140755));
#145899=CARTESIAN_POINT('Ctrl Pts',(-39.4616506489997,-21.98000002,-133.032398833922));
#145900=CARTESIAN_POINT('Ctrl Pts',(-39.3953798878174,-22.3926947961315,
-133.064083894138));
#145901=CARTESIAN_POINT('Ctrl Pts',(-39.7245793327553,-21.98000002,-132.504273278823));
#145902=CARTESIAN_POINT('Ctrl Pts',(-39.306634221246,-21.98000002,-132.626108677501));
#145903=CARTESIAN_POINT('Ctrl Pts',(-39.2495325922488,-22.4102623065174,
-132.649599803771));
#145904=CARTESIAN_POINT('Ctrl Pts',(-39.5464016190797,-21.98000002,-131.71886357396));
#145905=CARTESIAN_POINT('Ctrl Pts',(-39.0825794362701,-21.9800000199999,
-131.782866385322));
#145906=CARTESIAN_POINT('Ctrl Pts',(-39.0515573542344,-22.4453411404847,
-131.793566113248));
#145907=CARTESIAN_POINT('Ctrl Pts',(-39.5000000005303,-21.98000002,-131.311180490184));
#145908=CARTESIAN_POINT('Ctrl Pts',(-39.0167438766121,-21.98000002,-131.341321155374));
#145909=CARTESIAN_POINT('Ctrl Pts',(-39.,-22.4629715740863,-131.348761468896));
#145910=CARTESIAN_POINT('Ctrl Pts',(-39.5,-21.98000002,-130.903539806302));
#145911=CARTESIAN_POINT('Ctrl Pts',(-39.,-21.98000002,-130.903539806302));
#145912=CARTESIAN_POINT('Ctrl Pts',(-39.,-22.48000002,-130.903539806302));
#145913=CARTESIAN_POINT('',(-39.5912209088598,-22.3752378112049,-133.464034181283));
#145914=CARTESIAN_POINT('Origin',(-40.0320988180411,-22.48000002,-133.252725050377));
#145915=CARTESIAN_POINT('Ctrl Pts',(-39.5912209089345,-22.3752378108182,
-133.464034181247));
#145916=CARTESIAN_POINT('Ctrl Pts',(-39.3953798878174,-22.3926947961315,
-133.064083894138));
#145917=CARTESIAN_POINT('Ctrl Pts',(-39.2495325922488,-22.4102623065174,
-132.649599803771));
#145918=CARTESIAN_POINT('Ctrl Pts',(-39.0515573542344,-22.4453411404847,
-131.793566113248));
#145919=CARTESIAN_POINT('Ctrl Pts',(-39.,-22.4629715740863,-131.348761468896));
#145920=CARTESIAN_POINT('Ctrl Pts',(-39.,-22.48000002,-130.903539806302));
#145921=CARTESIAN_POINT('Ctrl Pts',(-39.5912209089345,-22.3752378108182,
-133.464034181247));
#145922=CARTESIAN_POINT('Ctrl Pts',(-39.6675936435998,-21.98000002,-133.427429361974));
#145923=CARTESIAN_POINT('Ctrl Pts',(-40.0320988180411,-21.98000002,-133.252725050377));
#145924=CARTESIAN_POINT('Ctrl Pts',(-45.6468692907591,-22.3902470227078,
-146.106052933848));
#145925=CARTESIAN_POINT('Ctrl Pts',(-45.790260298639,-21.98000002,-146.231563592216));
#145926=CARTESIAN_POINT('Ctrl Pts',(-46.0913014593244,-21.98000002,-145.894718230889));
#145927=CARTESIAN_POINT('Ctrl Pts',(-51.6504270099243,-22.3994099070849,
-158.773819030963));
#145928=CARTESIAN_POINT('Ctrl Pts',(-51.7509431131532,-21.9800000203624,
-158.826102375503));
#145929=CARTESIAN_POINT('Ctrl Pts',(-52.0964117641256,-21.98000002,-158.56249372189));
#145930=CARTESIAN_POINT('Ctrl Pts',(-57.638503474757,-22.4067641070473,
-171.449026400902));
#145931=CARTESIAN_POINT('Ctrl Pts',(-57.6956367824858,-21.98000002,-171.422029807066));
#145932=CARTESIAN_POINT('Ctrl Pts',(-58.085700246061,-21.98000002,-171.237717270032));
#145933=CARTESIAN_POINT('',(-57.638503474757,-22.4067641070473,-171.449026400902));
#145934=CARTESIAN_POINT('Origin',(-58.085700246061,-22.48000002,-171.237717270032));
#145935=CARTESIAN_POINT('Ctrl Pts',(-57.638503474757,-22.4067641070473,
-171.449026400902));
#145936=CARTESIAN_POINT('Ctrl Pts',(-51.650427014377,-22.3994098885056,
-158.773819033279));
#145937=CARTESIAN_POINT('Ctrl Pts',(-45.6468692971616,-22.39024700439,-146.106052939452));
#145938=CARTESIAN_POINT('Ctrl Pts',(-39.5912209089345,-22.3752378108181,
-133.464034181247));
#145939=CARTESIAN_POINT('Ctrl Pts',(-57.6186574596683,-22.4082912353334,
-171.40978315061));
#145940=CARTESIAN_POINT('Ctrl Pts',(-57.6735493970763,-21.9798882430102,
-171.380807602766));
#145941=CARTESIAN_POINT('Ctrl Pts',(-58.0564197191617,-21.9800000366742,
-171.178790026127));
#145942=CARTESIAN_POINT('Ctrl Pts',(-57.7016369198821,-22.4019038408433,
-171.565352937794));
#145943=CARTESIAN_POINT('Ctrl Pts',(-57.7654281245283,-21.9798905214978,
-171.542966774725));
#145944=CARTESIAN_POINT('Ctrl Pts',(-58.1793335836445,-21.9800000364255,
-171.412176181737));
#145945=CARTESIAN_POINT('Ctrl Pts',(-57.7416081447113,-22.3988541543228,
-171.738094620076));
#145946=CARTESIAN_POINT('Ctrl Pts',(-57.811087281066,-21.9798915951361,
-171.728859197825));
#145947=CARTESIAN_POINT('Ctrl Pts',(-58.2385448347245,-21.9800000363068,
-171.671295447806));
#145948=CARTESIAN_POINT('Ctrl Pts',(-57.7336548687769,-22.399461430235,
-171.916008414622));
#145949=CARTESIAN_POINT('Ctrl Pts',(-57.8020514502591,-21.9798913838386,
-171.91910344938));
#145950=CARTESIAN_POINT('Ctrl Pts',(-58.2267633341816,-21.9800000363304,
-171.938197690258));
#145951=CARTESIAN_POINT('Origin',(-58.2281061322669,-22.48000002,-171.871644662643));
#145952=CARTESIAN_POINT('Origin',(-56.6903638456505,-22.4806382361538,-171.875913019551));
#145953=CARTESIAN_POINT('Origin',(-58.2281061322669,-22.48000002,-179.64995));
#145954=CARTESIAN_POINT('Origin',(-58.2281061322669,-22.48000002,-176.657965001855));
#145955=CARTESIAN_POINT('Ctrl Pts',(-60.,-21.48000002,-174.47822483969));
#145956=CARTESIAN_POINT('Ctrl Pts',(-60.,-21.98000002,-174.47822483969));
#145957=CARTESIAN_POINT('Ctrl Pts',(-59.5,-21.98000002,-174.47822483969));
#145958=CARTESIAN_POINT('Ctrl Pts',(-60.,-21.4822140856788,-174.77632287275));
#145959=CARTESIAN_POINT('Ctrl Pts',(-59.9977907999382,-21.9800000199965,
-174.775666642734));
#145960=CARTESIAN_POINT('Ctrl Pts',(-59.4999999932692,-21.98000002,-174.72672222605));
#145961=CARTESIAN_POINT('Ctrl Pts',(-59.9565698697824,-21.4843793273514,
-175.067148740399));
#145962=CARTESIAN_POINT('Ctrl Pts',(-59.9524075929633,-21.98000002,-175.065899995449));
#145963=CARTESIAN_POINT('Ctrl Pts',(-59.4638082272143,-21.98000002,-174.969157756816));
#145964=CARTESIAN_POINT('Ctrl Pts',(-59.8274910918555,-21.4875521339025,
-175.492414399022));
#145965=CARTESIAN_POINT('Ctrl Pts',(-59.8205081565721,-21.98000002,-175.489804158754));
#145966=CARTESIAN_POINT('Ctrl Pts',(-59.3562425753485,-21.98000002,-175.323664095203));
#145967=CARTESIAN_POINT('Ctrl Pts',(-59.7735239255666,-21.4885940652802,
-175.631914079949));
#145968=CARTESIAN_POINT('Ctrl Pts',(-59.7657533403762,-21.9800000200007,
-175.628582862653));
#145969=CARTESIAN_POINT('Ctrl Pts',(-59.3112699374162,-21.98000002,-175.439952697294));
#145970=CARTESIAN_POINT('Ctrl Pts',(-59.6473451018805,-21.4905837846614,
-175.89805223939));
#145971=CARTESIAN_POINT('Ctrl Pts',(-59.6382394618755,-21.9800000199994,
-175.893067776338));
#145972=CARTESIAN_POINT('Ctrl Pts',(-59.2061209187896,-21.98000002,-175.661808757878));
#145973=CARTESIAN_POINT('Ctrl Pts',(-59.5748118056443,-21.4915405113197,
-176.025889197601));
#145974=CARTESIAN_POINT('Ctrl Pts',(-59.5651790529315,-21.9800000199994,
-176.020005430174));
#145975=CARTESIAN_POINT('Ctrl Pts',(-59.1456765053938,-21.98000002,-175.768375282423));
#145976=CARTESIAN_POINT('Ctrl Pts',(-59.4107666107714,-21.493376849955,
-176.271048580335));
#145977=CARTESIAN_POINT('Ctrl Pts',(-59.4003458450454,-21.9800000200006,
-176.263201660659));
#145978=CARTESIAN_POINT('Ctrl Pts',(-59.0089721749525,-21.98000002,-175.972743369523));
#145979=CARTESIAN_POINT('Ctrl Pts',(-59.3183914660909,-21.4942625520954,
-176.389181693558));
#145980=CARTESIAN_POINT('Ctrl Pts',(-59.3077278616495,-21.9800000199987,
-176.380304393309));
#145981=CARTESIAN_POINT('Ctrl Pts',(-58.9319928876421,-21.98000002,-176.071220734744));
#145982=CARTESIAN_POINT('Ctrl Pts',(-59.1195126442718,-21.495903657329,
-176.607905725284));
#145983=CARTESIAN_POINT('Ctrl Pts',(-59.1086757415209,-21.9800000200013,
-176.59692321781));
#145984=CARTESIAN_POINT('Ctrl Pts',(-58.7662605376602,-21.98000002,-176.253552125047));
#145985=CARTESIAN_POINT('Ctrl Pts',(-59.012812502338,-21.4966636432885,
-176.7091099968));
#145986=CARTESIAN_POINT('Ctrl Pts',(-59.0020443621077,-21.9800000199996,
-176.697095400112));
#145987=CARTESIAN_POINT('Ctrl Pts',(-58.6773437522104,-21.98000002,-176.337917446619));
#145988=CARTESIAN_POINT('Ctrl Pts',(-58.6712299408253,-21.4987636190772,
-176.988586760981));
#145989=CARTESIAN_POINT('Ctrl Pts',(-58.6613611188049,-21.9800000200008,
-176.973308002926));
#145990=CARTESIAN_POINT('Ctrl Pts',(-58.3926916168304,-21.98000002,-176.570893328242));
#145991=CARTESIAN_POINT('Ctrl Pts',(-58.4110432062101,-21.4999301516852,
-177.143590179504));
#145992=CARTESIAN_POINT('Ctrl Pts',(-58.4021689190209,-21.9800000199881,
-177.126531916838));
#145993=CARTESIAN_POINT('Ctrl Pts',(-58.1758692424685,-21.98000002,-176.700106570217));
#145994=CARTESIAN_POINT('Ctrl Pts',(-58.140200132617,-21.5007687140674,
-177.254954590203));
#145995=CARTESIAN_POINT('Ctrl Pts',(-58.132621442372,-21.98000002,-177.23652912386));
#145996=CARTESIAN_POINT('Ctrl Pts',(-57.9501667771809,-21.98000002,-176.792941619423));
#145997=CARTESIAN_POINT('',(-60.,-21.48000002,-174.47822483969));
#145998=CARTESIAN_POINT('Origin',(-59.5,-21.48000002,-174.47822483969));
#145999=CARTESIAN_POINT('',(-58.1799818946227,-21.5006430239517,-177.238261718428));
#146000=CARTESIAN_POINT('Ctrl Pts',(-60.,-21.48000002,-174.47822483969));
#146001=CARTESIAN_POINT('Ctrl Pts',(-60.,-21.4822140856788,-174.77632287275));
#146002=CARTESIAN_POINT('Ctrl Pts',(-59.9565698697824,-21.4843793273514,
-175.067148740399));
#146003=CARTESIAN_POINT('Ctrl Pts',(-59.8274910918555,-21.4875521339025,
-175.492414399022));
#146004=CARTESIAN_POINT('Ctrl Pts',(-59.7735239255666,-21.4885940652802,
-175.631914079949));
#146005=CARTESIAN_POINT('Ctrl Pts',(-59.6473451018805,-21.4905837846614,
-175.89805223939));
#146006=CARTESIAN_POINT('Ctrl Pts',(-59.5748118056443,-21.4915405113197,
-176.025889197601));
#146007=CARTESIAN_POINT('Ctrl Pts',(-59.4107666107714,-21.493376849955,
-176.271048580335));
#146008=CARTESIAN_POINT('Ctrl Pts',(-59.3183914660909,-21.4942625520954,
-176.389181693558));
#146009=CARTESIAN_POINT('Ctrl Pts',(-59.1195126442718,-21.495903657329,
-176.607905725284));
#146010=CARTESIAN_POINT('Ctrl Pts',(-59.012812502338,-21.4966636432885,
-176.7091099968));
#146011=CARTESIAN_POINT('Ctrl Pts',(-58.6824004740714,-21.4986949450522,
-176.979447229759));
#146012=CARTESIAN_POINT('Ctrl Pts',(-58.4364911965918,-21.4998151450696,
-177.128307927537));
#146013=CARTESIAN_POINT('Ctrl Pts',(-58.1799818947148,-21.5006430233981,
-177.238261718413));
#146014=CARTESIAN_POINT('Ctrl Pts',(-58.2281061322669,-21.98000002,-176.657965001855));
#146015=CARTESIAN_POINT('Ctrl Pts',(-58.1997838724148,-21.98000002,-176.740111438881));
#146016=CARTESIAN_POINT('Ctrl Pts',(-58.1775901524469,-21.9698497118448,
-176.818815489061));
#146017=CARTESIAN_POINT('Ctrl Pts',(-58.1467121091855,-21.9264637442851,
-176.962169933093));
#146018=CARTESIAN_POINT('Ctrl Pts',(-58.1379476084663,-21.8930112710375,
-177.027055273752));
#146019=CARTESIAN_POINT('Ctrl Pts',(-58.1325374345936,-21.8059684297317,
-177.133613057603));
#146020=CARTESIAN_POINT('Ctrl Pts',(-58.135834617463,-21.751763745641,-177.175847704912));
#146021=CARTESIAN_POINT('Ctrl Pts',(-58.1516959167317,-21.6321056009482,
-177.229926261063));
#146022=CARTESIAN_POINT('Ctrl Pts',(-58.1643305096628,-21.5659716479372,
-177.242027715059));
#146023=CARTESIAN_POINT('Ctrl Pts',(-58.1799818947148,-21.5006430233981,
-177.238261718413));
#146024=CARTESIAN_POINT('Origin',(-59.5,-21.48000002,-55.24995));
#146025=CARTESIAN_POINT('',(-60.,-21.48000002,-174.45635375974));
#146026=CARTESIAN_POINT('Origin',(-60.,-2.55003103885676E-14,0.));
#146027=CARTESIAN_POINT('',(-60.,-20.98000002,-174.500886972636));
#146028=CARTESIAN_POINT('',(-60.,-20.98000002,-58.1134713856835));
#146029=CARTESIAN_POINT('Ctrl Pts',(-60.,-21.48000002,-174.47822483969));
#146030=CARTESIAN_POINT('Ctrl Pts',(-60.,-21.3133292808184,-174.485664661366));
#146031=CARTESIAN_POINT('Ctrl Pts',(-60.,-21.1466632268706,-174.493235890728));
#146032=CARTESIAN_POINT('Ctrl Pts',(-60.,-20.98000002,-174.500886972636));
#146033=CARTESIAN_POINT('Origin',(-59.5,-20.98000002,-55.24995));
#146034=CARTESIAN_POINT('Origin',(-59.5,-20.98000002,-174.500886972636));
#146035=CARTESIAN_POINT('Ctrl Pts',(-39.5365899624517,-19.9017174575869,
-99.7816873060563));
#146036=CARTESIAN_POINT('Ctrl Pts',(-39.4537365768202,-20.48000002,-99.742462415759));
#146037=CARTESIAN_POINT('Ctrl Pts',(-39.9829309662066,-20.48000002,-99.9929964369266));
#146038=CARTESIAN_POINT('Ctrl Pts',(-45.6728806075319,-19.9133770447829,
-86.815892326284));
#146039=CARTESIAN_POINT('Ctrl Pts',(-45.5211976544485,-20.48000002,-86.9586415917399));
#146040=CARTESIAN_POINT('Ctrl Pts',(-46.1212593572987,-20.48000002,-87.0272166609364));
#146041=CARTESIAN_POINT('Ctrl Pts',(-51.7792721521254,-19.9203329608279,
-73.8354504790526));
#146042=CARTESIAN_POINT('Ctrl Pts',(-51.6794916123544,-20.4800000199249,
-73.8897477208158));
#146043=CARTESIAN_POINT('Ctrl Pts',(-52.2285110086243,-20.48000002,-74.0467697366574));
#146044=CARTESIAN_POINT('Ctrl Pts',(-57.8770125754992,-19.9259080025173,
-60.8508735991007));
#146045=CARTESIAN_POINT('Ctrl Pts',(-57.8224346115608,-20.48000002,-60.8252402001721));
#146046=CARTESIAN_POINT('Ctrl Pts',(-58.3269264615434,-20.48000002,-61.0621827299711));
#146047=CARTESIAN_POINT('Origin',(-39.9829309662066,-19.98000002,-99.9929964369266));
#146048=CARTESIAN_POINT('Ctrl Pts',(-59.5,-20.48000002,-174.500886972636));
#146049=CARTESIAN_POINT('Ctrl Pts',(-60.,-20.48000002,-174.500886972636));
#146050=CARTESIAN_POINT('Ctrl Pts',(-60.,-20.98000002,-174.500886972636));
#146051=CARTESIAN_POINT('Ctrl Pts',(-59.4999999934397,-20.48000002,-174.74311983516));
#146052=CARTESIAN_POINT('Ctrl Pts',(-60.0022242907223,-20.48000002,-174.792108323791));
#146053=CARTESIAN_POINT('Ctrl Pts',(-60.,-20.9822194010082,-174.791464522024));
#146054=CARTESIAN_POINT('Ctrl Pts',(-59.4655777479701,-20.48000002,-174.979582459221));
#146055=CARTESIAN_POINT('Ctrl Pts',(-59.9629392387446,-20.4800000199999,
-175.076359449429));
#146056=CARTESIAN_POINT('Ctrl Pts',(-59.9586932949262,-20.9843889926879,
-175.075119998302));
#146057=CARTESIAN_POINT('Ctrl Pts',(-59.3634105452706,-20.48000002,-175.325604118318));
#146058=CARTESIAN_POINT('Ctrl Pts',(-59.8433264812564,-20.48000002,-175.492827860986));
#146059=CARTESIAN_POINT('Ctrl Pts',(-59.8360926556437,-20.9875676565265,
-175.49019987132));
#146060=CARTESIAN_POINT('Ctrl Pts',(-59.3205935345334,-20.48000002,-175.43951222267));
#146061=CARTESIAN_POINT('Ctrl Pts',(-59.7928073162253,-20.4800000200006,
-175.630213503224));
#146062=CARTESIAN_POINT('Ctrl Pts',(-59.7847122422101,-20.9886147234176,
-175.626841448369));
#146063=CARTESIAN_POINT('Ctrl Pts',(-59.2204432327122,-20.48000002,-175.657072445029));
#146064=CARTESIAN_POINT('Ctrl Pts',(-59.674123349008,-20.4800000199994,
-175.892915048025));
#146065=CARTESIAN_POINT('Ctrl Pts',(-59.6645318784846,-20.9906156905346,
-175.887821675912));
#146066=CARTESIAN_POINT('Ctrl Pts',(-59.162871562207,-20.48000002,-175.761697975082));
#146067=CARTESIAN_POINT('Ctrl Pts',(-59.605650654114,-20.4800000200002,
-176.019368430779));
#146068=CARTESIAN_POINT('Ctrl Pts',(-59.5954458739788,-20.9915785299556,
-176.013328010605));
#146069=CARTESIAN_POINT('Ctrl Pts',(-59.032749049719,-20.48000002,-175.962647558431));
#146070=CARTESIAN_POINT('Ctrl Pts',(-59.4504692034509,-20.4800000199998,
-176.262509186853));
#146071=CARTESIAN_POINT('Ctrl Pts',(-59.4392988603324,-20.9934287142977,
-176.254382360717));
#146072=CARTESIAN_POINT('Ctrl Pts',(-58.9595157418279,-20.48000002,-176.059697515632));
#146073=CARTESIAN_POINT('Ctrl Pts',(-59.3629214966957,-20.48000002,-176.380037040048));
#146074=CARTESIAN_POINT('Ctrl Pts',(-59.3514188912717,-20.9943227517297,
-176.370801152158));
#146075=CARTESIAN_POINT('Ctrl Pts',(-58.800974443077,-20.48000002,-176.240813845549));
#146076=CARTESIAN_POINT('Ctrl Pts',(-59.1730156260874,-20.48000002,-176.599598651605));
#146077=CARTESIAN_POINT('Ctrl Pts',(-59.1611693306144,-20.9959919273243,
-176.588063887092));
#146078=CARTESIAN_POINT('Ctrl Pts',(-58.7159164062094,-20.48000002,-176.324867284949));
#146079=CARTESIAN_POINT('Ctrl Pts',(-59.0709534896778,-20.4800000200012,
-176.701568343258));
#146080=CARTESIAN_POINT('Ctrl Pts',(-59.0590996873029,-20.9967669365736,
-176.688892319953));
#146081=CARTESIAN_POINT('Ctrl Pts',(-58.4437643988224,-20.48000002,-176.557945321316));
#146082=CARTESIAN_POINT('Ctrl Pts',(-58.7436561080181,-20.4800000199975,
-176.984811315106));
#146083=CARTESIAN_POINT('Ctrl Pts',(-58.7325172788836,-20.9989167502369,
-176.968486930424));
#146084=CARTESIAN_POINT('Ctrl Pts',(-58.2366741051621,-20.48000002,-176.68900326854));
#146085=CARTESIAN_POINT('Ctrl Pts',(-58.4942266187642,-20.4800000200099,
-177.144085084891));
#146086=CARTESIAN_POINT('Ctrl Pts',(-58.484009011739,-21.0001266369645,
-177.125700665905));
#146087=CARTESIAN_POINT('Ctrl Pts',(-58.0184329245781,-20.48000002,-176.786456163744));
#146088=CARTESIAN_POINT('Ctrl Pts',(-58.2310611931749,-20.4800000199999,
-177.262627176116));
#146089=CARTESIAN_POINT('Ctrl Pts',(-58.2221195094937,-21.0010265837306,
-177.24260269584));
#146090=CARTESIAN_POINT('',(-58.2408314794356,-21.0009616714991,-177.234172657581));
#146091=CARTESIAN_POINT('Ctrl Pts',(-58.2408316684982,-21.000961690655,
-177.234173073119));
#146092=CARTESIAN_POINT('Ctrl Pts',(-58.4958429921241,-21.0000687461186,
-177.118186472847));
#146093=CARTESIAN_POINT('Ctrl Pts',(-58.7377089067135,-20.998882511313,
-176.964042263202));
#146094=CARTESIAN_POINT('Ctrl Pts',(-59.0590996887611,-20.9967668730019,
-176.688892321512));
#146095=CARTESIAN_POINT('Ctrl Pts',(-59.1611693320729,-20.995991863797,
-176.588063888513));
#146096=CARTESIAN_POINT('Ctrl Pts',(-59.3514188926903,-20.9943226882988,
-176.370801153298));
#146097=CARTESIAN_POINT('Ctrl Pts',(-59.4392988617113,-20.9934286509189,
-176.25438236172));
#146098=CARTESIAN_POINT('Ctrl Pts',(-59.5954458752409,-20.9915784666852,
-176.013328011352));
#146099=CARTESIAN_POINT('Ctrl Pts',(-59.664531879672,-20.990615627321,-175.887821676543));
#146100=CARTESIAN_POINT('Ctrl Pts',(-59.7847122432143,-20.9886146603231,
-175.626841448787));
#146101=CARTESIAN_POINT('Ctrl Pts',(-59.836092656542,-20.9875675934948,
-175.490199871646));
#146102=CARTESIAN_POINT('Ctrl Pts',(-59.9586932954552,-20.984388929849,
-175.075119998456));
#146103=CARTESIAN_POINT('Ctrl Pts',(-60.0000000002777,-20.9822193383029,
-174.791464522104));
#146104=CARTESIAN_POINT('Ctrl Pts',(-60.,-20.98000002,-174.500886972636));
#146105=CARTESIAN_POINT('Ctrl Pts',(-58.2408309122627,-21.0009616140329,
-177.234171411));
#146106=CARTESIAN_POINT('Ctrl Pts',(-58.2451692158037,-20.9815789540505,
-177.233091079908));
#146107=CARTESIAN_POINT('Ctrl Pts',(-58.2497081333482,-20.962409235832,
-177.230657978534));
#146108=CARTESIAN_POINT('Ctrl Pts',(-58.2544730703504,-20.943543143678,
-177.226940751589));
#146109=CARTESIAN_POINT('Ctrl Pts',(-58.259312250581,-20.9243830959921,
-177.22316560595));
#146110=CARTESIAN_POINT('Ctrl Pts',(-58.2643851390725,-20.9055354515583,
-177.218067292576));
#146111=CARTESIAN_POINT('Ctrl Pts',(-58.269703032832,-20.8870439871654,
-177.211703850792));
#146112=CARTESIAN_POINT('Ctrl Pts',(-58.2751367003253,-20.8681499525119,
-177.205201873067));
#146113=CARTESIAN_POINT('Ctrl Pts',(-58.28082669489,-20.8496264838163,-177.197380013113));
#146114=CARTESIAN_POINT('Ctrl Pts',(-58.2867604599995,-20.8314829595576,
-177.18826855295));
#146115=CARTESIAN_POINT('Ctrl Pts',(-58.2918979870607,-20.8157740723432,
-177.180379738296));
#146116=CARTESIAN_POINT('Ctrl Pts',(-58.2972179599825,-20.8003487350648,
-177.171523735368));
#146117=CARTESIAN_POINT('Ctrl Pts',(-58.3026938424719,-20.7852040043215,
-177.161696010758));
#146118=CARTESIAN_POINT('Ctrl Pts',(-58.309742257017,-20.7657100979675,
-177.149046017406));
#146119=CARTESIAN_POINT('Ctrl Pts',(-58.3169594019401,-20.7470208494275,
-177.134987393464));
#146120=CARTESIAN_POINT('Ctrl Pts',(-58.3243946994305,-20.729187882357,
-177.119617493859));
#146121=CARTESIAN_POINT('Ctrl Pts',(-58.3320743703935,-20.710768805034,
-177.10374243683));
#146122=CARTESIAN_POINT('Ctrl Pts',(-58.3399872192437,-20.6932616945543,
-177.086468930266));
#146123=CARTESIAN_POINT('Ctrl Pts',(-58.3481588912673,-20.6766903075191,
-177.06786817926));
#146124=CARTESIAN_POINT('Ctrl Pts',(-58.3567372752991,-20.659294146548,
-177.048341650914));
#146125=CARTESIAN_POINT('Ctrl Pts',(-58.3656012090582,-20.6429273606653,
-177.027352254574));
#146126=CARTESIAN_POINT('Ctrl Pts',(-58.3747427271629,-20.6276079654216,
-177.004940996223));
#146127=CARTESIAN_POINT('Ctrl Pts',(-58.377271631966,-20.6233700159071,
-176.998741157395));
#146128=CARTESIAN_POINT('Ctrl Pts',(-58.3798215549078,-20.6192122591398,
-176.992432289584));
#146129=CARTESIAN_POINT('Ctrl Pts',(-58.3823918217751,-20.6151352360893,
-176.986014819637));
#146130=CARTESIAN_POINT('Ctrl Pts',(-58.3921799248114,-20.5996090966801,
-176.961575778744));
#146131=CARTESIAN_POINT('Ctrl Pts',(-58.402161806076,-20.5854344582556,
-176.935836605802));
#146132=CARTESIAN_POINT('Ctrl Pts',(-58.4123668786042,-20.5726356287647,
-176.908971720649));
#146133=CARTESIAN_POINT('Ctrl Pts',(-58.4230115467541,-20.5592854744898,
-176.880949598656));
#146134=CARTESIAN_POINT('Ctrl Pts',(-58.4338992850076,-20.5474313492243,
-176.851703114916));
#146135=CARTESIAN_POINT('Ctrl Pts',(-58.4450457241721,-20.5370573305028,
-176.821397121147));
#146136=CARTESIAN_POINT('Ctrl Pts',(-58.4570445066189,-20.5258900337632,
-176.788773695792));
#146137=CARTESIAN_POINT('Ctrl Pts',(-58.469343309893,-20.5164370754064,
-176.754922805974));
#146138=CARTESIAN_POINT('Ctrl Pts',(-58.4819374094809,-20.5086424875326,
-176.720006455305));
#146139=CARTESIAN_POINT('Ctrl Pts',(-58.4951021738506,-20.5004947107105,
-176.683507972345));
#146140=CARTESIAN_POINT('Ctrl Pts',(-58.5085896080475,-20.49415825095,-176.645845027844));
#146141=CARTESIAN_POINT('Ctrl Pts',(-58.5223669924781,-20.4895440418049,
-176.607156904439));
#146142=CARTESIAN_POINT('Ctrl Pts',(-58.5368459438342,-20.4846948695911,
-176.566498718578));
#146143=CARTESIAN_POINT('Ctrl Pts',(-58.5516451680495,-20.4817475506061,
-176.524707986652));
#146144=CARTESIAN_POINT('Ctrl Pts',(-58.5666969888986,-20.4805798588946,
-176.481901643726));
#146145=CARTESIAN_POINT('Ctrl Pts',(-58.5716977806305,-20.4801919069574,
-176.467679736096));
#146146=CARTESIAN_POINT('Ctrl Pts',(-58.5767262175753,-20.4800002580357,
-176.453345390789));
#146147=CARTESIAN_POINT('Ctrl Pts',(-58.5817791104913,-20.4800000202216,
-176.438901946458));
#146148=CARTESIAN_POINT('Origin',(-58.5817791104913,-19.98000002,-179.64995));
#146149=CARTESIAN_POINT('Origin',(-58.5817791104913,-19.98000002,-176.438901946458));
#146150=CARTESIAN_POINT('Origin',(-58.5817791104913,-19.98000002,-171.871644662643));
#146151=CARTESIAN_POINT('Ctrl Pts',(-58.0853233553177,-19.9205720538986,
-171.871644662643));
#146152=CARTESIAN_POINT('Ctrl Pts',(-58.0183573349639,-20.48000002,-171.871644662643));
#146153=CARTESIAN_POINT('Ctrl Pts',(-58.5817791104913,-20.48000002,-171.871644662643));
#146154=CARTESIAN_POINT('Ctrl Pts',(-58.0853233550829,-19.9205720558596,
-171.725723025901));
#146155=CARTESIAN_POINT('Ctrl Pts',(-58.018357325283,-20.48000002,-171.735617762033));
#146156=CARTESIAN_POINT('Ctrl Pts',(-58.5817790937258,-20.48000002,-171.652759539508));
#146157=CARTESIAN_POINT('Ctrl Pts',(-58.0534084851269,-19.9223906228206,
-171.582455328445));
#146158=CARTESIAN_POINT('Ctrl Pts',(-57.9913238325147,-20.4800000200031,
-171.602371122267));
#146159=CARTESIAN_POINT('Ctrl Pts',(-58.5342346140381,-20.48000002,-171.437864213701));
#146160=CARTESIAN_POINT('Ctrl Pts',(-57.9903087491627,-19.9260113903464,
-171.449026400902));
#146161=CARTESIAN_POINT('Ctrl Pts',(-57.9358462259716,-20.48000002,-171.474604875281));
#146162=CARTESIAN_POINT('Ctrl Pts',(-58.4402350532158,-20.48000002,-171.237717270032));
#146163=CARTESIAN_POINT('',(-57.9903087491627,-19.9260113903464,-171.449026400902));
#146164=CARTESIAN_POINT('Origin',(-58.4402350532158,-19.98000002,-171.237717270032));
#146165=CARTESIAN_POINT('Origin',(-56.628753050575,-20.0041469075947,-171.968943421328));
#146166=CARTESIAN_POINT('Ctrl Pts',(-57.9903087491627,-19.9260113903464,
-171.449026400902));
#146167=CARTESIAN_POINT('Ctrl Pts',(-57.9358462259716,-20.48000002,-171.474604875281));
#146168=CARTESIAN_POINT('Ctrl Pts',(-58.4402350532158,-20.48000002,-171.237717270032));
#146169=CARTESIAN_POINT('Ctrl Pts',(-51.8549375290089,-19.9204232153646,
-158.383965825354));
#146170=CARTESIAN_POINT('Ctrl Pts',(-51.754926284906,-20.4800000196472,
-158.328906441527));
#146171=CARTESIAN_POINT('Ctrl Pts',(-52.3041884424236,-20.48000002,-158.172646387016));
#146172=CARTESIAN_POINT('Ctrl Pts',(-45.7108852546953,-19.9134492574988,
-145.323053305542));
#146173=CARTESIAN_POINT('Ctrl Pts',(-45.5582765746385,-20.48000002,-145.178124710387));
#146174=CARTESIAN_POINT('Ctrl Pts',(-46.1592765266851,-20.48000002,-145.111728668187));
#146175=CARTESIAN_POINT('Ctrl Pts',(-39.5365899624517,-19.9017174575869,
-132.27695566545));
#146176=CARTESIAN_POINT('Ctrl Pts',(-39.4537365768201,-20.48000002,-132.316180555747));
#146177=CARTESIAN_POINT('Ctrl Pts',(-39.9829309662066,-20.48000002,-132.065646534579));
#146178=CARTESIAN_POINT('',(-39.5365899624061,-19.9017174579054,-132.276955665471));
#146179=CARTESIAN_POINT('Origin',(-39.9829309662066,-19.98000002,-132.065646534579));
#146180=CARTESIAN_POINT('Ctrl Pts',(-39.5365899624517,-19.9017174575869,
-132.27695566545));
#146181=CARTESIAN_POINT('Ctrl Pts',(-45.7108852544235,-19.9134492585078,
-145.323053305284));
#146182=CARTESIAN_POINT('Ctrl Pts',(-51.8549375288294,-19.9204232163692,
-158.383965825256));
#146183=CARTESIAN_POINT('Ctrl Pts',(-57.9903087491627,-19.9260113903464,
-171.449026400902));
#146184=CARTESIAN_POINT('Ctrl Pts',(-39.5,-20.48000002,-129.914446011788));
#146185=CARTESIAN_POINT('Ctrl Pts',(-39.,-20.48000002,-129.914446011788));
#146186=CARTESIAN_POINT('Ctrl Pts',(-39.,-19.98000002,-129.914446011788));
#146187=CARTESIAN_POINT('Ctrl Pts',(-39.5000000028435,-20.48000002,-130.287671434236));
#146188=CARTESIAN_POINT('Ctrl Pts',(-38.9872746975485,-20.48000002,-130.330124066848));
#146189=CARTESIAN_POINT('Ctrl Pts',(-39.,-19.9674346440713,-130.324899900514));
#146190=CARTESIAN_POINT('Ctrl Pts',(-39.5411198836701,-20.48000002,-130.653963774132));
#146191=CARTESIAN_POINT('Ctrl Pts',(-39.0203709824336,-20.48000002,-130.73585622864));
#146192=CARTESIAN_POINT('Ctrl Pts',(-39.0456887600695,-19.9546004036482,
-130.727459443406));
#146193=CARTESIAN_POINT('Ctrl Pts',(-39.7019669306849,-20.48000002,-131.373086703203));
#146194=CARTESIAN_POINT('Ctrl Pts',(-39.1707024462744,-20.48000002,-131.538360679722));
#146195=CARTESIAN_POINT('Ctrl Pts',(-39.2244077003248,-19.9284125341257,
-131.517220896748));
#146196=CARTESIAN_POINT('Ctrl Pts',(-39.8231470367065,-20.48000002,-131.72814043837));
#146197=CARTESIAN_POINT('Ctrl Pts',(-39.2920635693995,-20.48000002,-131.938092167695));
#146198=CARTESIAN_POINT('Ctrl Pts',(-39.3590527322559,-19.9149653023259,
-131.906857743156));
#146199=CARTESIAN_POINT('Ctrl Pts',(-39.9829309662066,-20.48000002,-132.065646534579));
#146200=CARTESIAN_POINT('Ctrl Pts',(-39.4537365768201,-20.48000002,-132.316180555747));
#146201=CARTESIAN_POINT('Ctrl Pts',(-39.5365899624517,-19.9017174575869,
-132.27695566545));
#146202=CARTESIAN_POINT('',(-39.,-19.98000002,-129.914446011788));
#146203=CARTESIAN_POINT('Origin',(-39.5,-19.98000002,-129.914446011788));
#146204=CARTESIAN_POINT('Ctrl Pts',(-39.,-19.98000002,-129.914446011788));
#146205=CARTESIAN_POINT('Ctrl Pts',(-39.,-19.9674346440713,-130.324899900514));
#146206=CARTESIAN_POINT('Ctrl Pts',(-39.0456887600695,-19.9546004036482,
-130.727459443406));
#146207=CARTESIAN_POINT('Ctrl Pts',(-39.1350482301972,-19.9415064688869,
-131.122340170077));
#146208=CARTESIAN_POINT('Ctrl Pts',(-39.2244077003248,-19.9284125341257,
-131.517220896748));
#146209=CARTESIAN_POINT('Ctrl Pts',(-39.3590527322559,-19.9149653023259,
-131.906857743156));
#146210=CARTESIAN_POINT('Ctrl Pts',(-39.5365899624517,-19.9017174575869,
-132.27695566545));
#146211=CARTESIAN_POINT('Origin',(-39.5,-19.98000002,-55.24995));
#146212=CARTESIAN_POINT('',(-39.,-19.9800000199999,-102.144196959718));
#146213=CARTESIAN_POINT('Origin',(-39.5,-19.98000002,-102.144196959718));
#146214=CARTESIAN_POINT('',(-39.,-19.98000002,-129.34995));
#146215=CARTESIAN_POINT('Ctrl Pts',(-40.0012502563217,-20.48000002,-99.954717797516));
#146216=CARTESIAN_POINT('Ctrl Pts',(-39.4725489992773,-20.48000002,-99.6988739218247));
#146217=CARTESIAN_POINT('Ctrl Pts',(-39.5569491658928,-19.9001814680542,
-99.7397158520094));
#146218=CARTESIAN_POINT('Ctrl Pts',(-39.8323199385717,-20.48000002,-100.303930668773));
#146219=CARTESIAN_POINT('Ctrl Pts',(-39.301375019511,-20.48000002,-100.090148174869));
#146220=CARTESIAN_POINT('Ctrl Pts',(-39.3692493188849,-19.9139264408504,
-100.122626239893));
#146221=CARTESIAN_POINT('Ctrl Pts',(-39.7069896112656,-20.48000002,-100.665459816052));
#146222=CARTESIAN_POINT('Ctrl Pts',(-39.1755409765978,-20.48000002,-100.497354008517));
#146223=CARTESIAN_POINT('Ctrl Pts',(-39.2299915028605,-19.9276433576926,
-100.519356460951));
#146224=CARTESIAN_POINT('Ctrl Pts',(-39.5390449391743,-20.48000002,-101.411637934188));
#146225=CARTESIAN_POINT('Ctrl Pts',(-39.018406306162,-20.48000002,-101.330154470495));
#146226=CARTESIAN_POINT('Ctrl Pts',(-39.0433847037664,-19.9548298743016,
-101.338822719377));
#146227=CARTESIAN_POINT('Ctrl Pts',(-39.4968660312411,-20.48000002,-101.799124124856));
#146228=CARTESIAN_POINT('Ctrl Pts',(-38.9847617214833,-20.48000002,-101.759282695456));
#146229=CARTESIAN_POINT('Ctrl Pts',(-38.9965184980456,-19.9683907683482,
-101.764681199409));
#146230=CARTESIAN_POINT('Ctrl Pts',(-39.5001813816655,-20.48000002,-102.186616395301));
#146231=CARTESIAN_POINT('Ctrl Pts',(-39.001593844989,-20.48000002,-102.190836991961));
#146232=CARTESIAN_POINT('Ctrl Pts',(-39.0002014519442,-19.9813964268796,
-102.190849108877));
#146233=CARTESIAN_POINT('Ctrl Pts',(-39.5365899564018,-19.9017175093585,
-99.7816874458032));
#146234=CARTESIAN_POINT('Ctrl Pts',(-39.4868412510969,-19.9054297760661,
-99.8853949251705));
#146235=CARTESIAN_POINT('Ctrl Pts',(-39.4406574931192,-19.9091517930361,
-99.990138214928));
#146236=CARTESIAN_POINT('Ctrl Pts',(-39.3979429037,-19.9128649009136,-100.095860132891));
#146237=CARTESIAN_POINT('Ctrl Pts',(-39.3547717131843,-19.9166177003614,
-100.202712173941));
#146238=CARTESIAN_POINT('Ctrl Pts',(-39.3151435367721,-19.9203617208069,
-100.310564614436));
#146239=CARTESIAN_POINT('Ctrl Pts',(-39.2789942567738,-19.924093206991,
-100.419396332393));
#146240=CARTESIAN_POINT('Ctrl Pts',(-39.2425575305557,-19.9278543646264,
-100.529093441471));
#146241=CARTESIAN_POINT('Ctrl Pts',(-39.2096547048051,-19.931603147313,
-100.639786363507));
#146242=CARTESIAN_POINT('Ctrl Pts',(-39.1802648150382,-19.9353461978555,
-100.751479335446));
#146243=CARTESIAN_POINT('Ctrl Pts',(-39.1647600945192,-19.9373208548893,
-100.81040328268));
#146244=CARTESIAN_POINT('Ctrl Pts',(-39.1502338657269,-19.9392940583882,
-100.869605905783));
#146245=CARTESIAN_POINT('Ctrl Pts',(-39.1366886677995,-19.9412674210986,
-100.929089335053));
#146246=CARTESIAN_POINT('Ctrl Pts',(-39.1088256225296,-19.945326711692,
-101.051449265963));
#146247=CARTESIAN_POINT('Ctrl Pts',(-39.0850665637736,-19.9493899507519,
-101.175230562368));
#146248=CARTESIAN_POINT('Ctrl Pts',(-39.0655733708748,-19.9534338869003,
-101.300036499352));
#146249=CARTESIAN_POINT('Ctrl Pts',(-39.0461769195927,-19.9574577536366,
-101.424223044317));
#146250=CARTESIAN_POINT('Ctrl Pts',(-39.0310043253741,-19.9614623125903,
-101.549423682696));
#146251=CARTESIAN_POINT('Ctrl Pts',(-39.0201697390594,-19.9654321073935,
-101.675224312219));
#146252=CARTESIAN_POINT('Ctrl Pts',(-39.0093951990674,-19.9693799012109,
-101.800327742515));
#146253=CARTESIAN_POINT('Ctrl Pts',(-39.0029108630928,-19.9732931398505,
-101.926024090876));
#146254=CARTESIAN_POINT('Ctrl Pts',(-39.0007812701477,-19.9771667798669,
-102.05188934728));
#146255=CARTESIAN_POINT('Ctrl Pts',(-39.0002608009155,-19.978113491514,
-102.082650621869));
#146256=CARTESIAN_POINT('Ctrl Pts',(-39.0000002133804,-19.9790578925252,
-102.113421924474));
#146257=CARTESIAN_POINT('Ctrl Pts',(-39.000000000131,-19.9800000199999,
-102.144196959718));
#146258=CARTESIAN_POINT('Ctrl Pts',(-39.4705101402401,-14.154883972851,
-101.179273599517));
#146259=CARTESIAN_POINT('Ctrl Pts',(-39.,-14.2196500163134,-102.183653245897));
#146260=CARTESIAN_POINT('Ctrl Pts',(-39.,-14.2911437666779,-103.292364908221));
#146261=CARTESIAN_POINT('Ctrl Pts',(-39.473885603051,-15.1336440339978,
-101.108924169704));
#146262=CARTESIAN_POINT('Ctrl Pts',(-38.9999999999962,-15.2519052464411,
-102.112898232639));
#146263=CARTESIAN_POINT('Ctrl Pts',(-39.,-15.3821188871317,-103.222014874282));
#146264=CARTESIAN_POINT('Ctrl Pts',(-39.4814699289176,-16.1148163368312,
-100.950916925651));
#146265=CARTESIAN_POINT('Ctrl Pts',(-39.,-16.2866475513133,-101.953874758818));
#146266=CARTESIAN_POINT('Ctrl Pts',(-39.,-16.4753328054123,-103.064008234267));
#146267=CARTESIAN_POINT('Ctrl Pts',(-39.5044475737172,-18.0667048767241,
-100.467247875485));
#146268=CARTESIAN_POINT('Ctrl Pts',(-39.,-18.3422738396393,-101.467519549647));
#146269=CARTESIAN_POINT('Ctrl Pts',(-39.,-18.6473032869024,-102.580339184276));
#146270=CARTESIAN_POINT('Ctrl Pts',(-39.5194922305763,-19.012479411179,
-100.148762913439));
#146271=CARTESIAN_POINT('Ctrl Pts',(-39.,-19.3376015901503,-101.147059506123));
#146272=CARTESIAN_POINT('Ctrl Pts',(-39.,-19.6982839688054,-102.261854767811));
#146273=CARTESIAN_POINT('Ctrl Pts',(-39.5372194307944,-19.9345274212658,
-99.7681750639369));
#146274=CARTESIAN_POINT('Ctrl Pts',(-39.,-20.3054076594241,-100.764738681203));
#146275=CARTESIAN_POINT('Ctrl Pts',(-39.,-20.7209336217775,-101.88126637264));
#146276=CARTESIAN_POINT('',(-39.0000000000002,-14.330000015482,-103.28982244638));
#146277=CARTESIAN_POINT('Ctrl Pts',(-39.,-14.3300000071455,-103.289822320808));
#146278=CARTESIAN_POINT('Ctrl Pts',(-39.,-14.6503224302959,-103.268556852662));
#146279=CARTESIAN_POINT('Ctrl Pts',(-38.9999999999999,-14.9696787697432,
-103.239819970848));
#146280=CARTESIAN_POINT('Ctrl Pts',(-39.0000000000001,-15.2880843675558,
-103.203826801699));
#146281=CARTESIAN_POINT('Ctrl Pts',(-39.0000000000004,-15.6115732353053,
-103.167259010131));
#146282=CARTESIAN_POINT('Ctrl Pts',(-38.9999999999999,-15.9340810135531,
-103.123201376372));
#146283=CARTESIAN_POINT('Ctrl Pts',(-39.0000000000089,-16.2556315657684,
-103.071825704719));
#146284=CARTESIAN_POINT('Ctrl Pts',(-39.0000000000177,-16.568088880393,
-103.021902903184));
#146285=CARTESIAN_POINT('Ctrl Pts',(-39.0000000000333,-16.8796426042166,
-102.965069752024));
#146286=CARTESIAN_POINT('Ctrl Pts',(-39.000000000099,-17.1903180517835,
-102.90143687879));
#146287=CARTESIAN_POINT('Ctrl Pts',(-39.0000000001251,-17.3140185734884,
-102.87610040731));
#146288=CARTESIAN_POINT('Ctrl Pts',(-39.0000000001567,-17.4376802476524,
-102.849665441423));
#146289=CARTESIAN_POINT('Ctrl Pts',(-39.0000000001917,-17.5613085289994,
-102.822130971399));
#146290=CARTESIAN_POINT('Ctrl Pts',(-39.000000000283,-17.8840119032273,
-102.750258530179));
#146291=CARTESIAN_POINT('Ctrl Pts',(-39.0000000004,-18.2040368478248,-102.671531783398));
#146292=CARTESIAN_POINT('Ctrl Pts',(-39.0000000004561,-18.5218724866246,
-102.586181685713));
#146293=CARTESIAN_POINT('Ctrl Pts',(-39.0000000005153,-18.8564962428641,
-102.496323385396));
#146294=CARTESIAN_POINT('Ctrl Pts',(-39.0000000004874,-19.1886932216437,
-102.399123389359));
#146295=CARTESIAN_POINT('Ctrl Pts',(-39.0000000003521,-19.519010542234,
-102.294797669286));
#146296=CARTESIAN_POINT('Ctrl Pts',(-39.000000000289,-19.6730648764625,
-102.246141942363));
#146297=CARTESIAN_POINT('Ctrl Pts',(-39.0000000002054,-19.8267100435457,
-102.195935559143));
#146298=CARTESIAN_POINT('Ctrl Pts',(-39.000000000131,-19.98000002,-102.144196959718));
#146299=CARTESIAN_POINT('Origin',(-46.4345084630437,-14.3111647034258,-103.828563644064));
#146300=CARTESIAN_POINT('Ctrl Pts',(-58.2781275348581,-14.3194901627709,
-60.8508735991007));
#146301=CARTESIAN_POINT('Ctrl Pts',(-58.2874540965012,-13.83000002,-60.8552238163692));
#146302=CARTESIAN_POINT('Ctrl Pts',(-58.7311595360587,-13.83000002,-61.0621827299711));
#146303=CARTESIAN_POINT('Ctrl Pts',(-52.0097486856907,-14.3183690440453,
-74.2898953083048));
#146304=CARTESIAN_POINT('Ctrl Pts',(-52.0270272593534,-13.8300000198715,
-74.2797364934824));
#146305=CARTESIAN_POINT('Ctrl Pts',(-52.4627544636864,-13.83000002,-74.5012048985427));
#146306=CARTESIAN_POINT('Ctrl Pts',(-45.7410317152176,-14.3169685900793,
-87.7287563851229));
#146307=CARTESIAN_POINT('Ctrl Pts',(-45.7671827316852,-13.8300000198453,
-87.7027488289555));
#146308=CARTESIAN_POINT('Ctrl Pts',(-46.194004389791,-13.83000002,-87.9400661652057));
#146309=CARTESIAN_POINT('Ctrl Pts',(-39.4710976496822,-14.3145440753934,
-101.167027481326));
#146310=CARTESIAN_POINT('Ctrl Pts',(-39.4846775617168,-13.83000002,-101.173363584839));
#146311=CARTESIAN_POINT('Ctrl Pts',(-39.923987884714,-13.83000002,-101.378336612196));
#146312=CARTESIAN_POINT('Origin',(-39.923987884714,-14.33000002,-101.378336612196));
#146313=CARTESIAN_POINT('Ctrl Pts',(-39.5,-13.83000002,-103.289822573788));
#146314=CARTESIAN_POINT('Ctrl Pts',(-39.,-13.83000002,-103.289822573788));
#146315=CARTESIAN_POINT('Ctrl Pts',(-39.,-14.33000002,-103.289822573788));
#146316=CARTESIAN_POINT('Ctrl Pts',(-39.5000000055327,-13.83000002,-102.630037977128));
#146317=CARTESIAN_POINT('Ctrl Pts',(-39.0048213824044,-13.83000002,-102.560555788171));
#146318=CARTESIAN_POINT('Ctrl Pts',(-39.,-14.3251554673834,-102.557050168938));
#146319=CARTESIAN_POINT('Ctrl Pts',(-39.6421844024665,-13.83000002,-101.982314517002));
#146320=CARTESIAN_POINT('Ctrl Pts',(-39.1662598483009,-13.830000019993,
-101.843408229318));
#146321=CARTESIAN_POINT('Ctrl Pts',(-39.1579830770898,-14.319921441001,
-101.837719843386));
#146322=CARTESIAN_POINT('Ctrl Pts',(-39.923987884714,-13.83000002,-101.378336612196));
#146323=CARTESIAN_POINT('Ctrl Pts',(-39.4846775617168,-13.83000002,-101.173363584839));
#146324=CARTESIAN_POINT('Ctrl Pts',(-39.4710976496822,-14.3145440753935,
-101.167027481325));
#146325=CARTESIAN_POINT('Origin',(-39.5,-14.33000002,-103.289822573788));
#146326=CARTESIAN_POINT('Origin',(-39.5,-14.33000002,-55.24995));
#146327=CARTESIAN_POINT('',(-39.,-14.3300000196436,-128.768820403088));
#146328=CARTESIAN_POINT('Origin',(-39.5,-14.33000002,-128.768820397718));
#146329=CARTESIAN_POINT('',(-39.,-14.33000002,-129.34995));
#146330=CARTESIAN_POINT('Ctrl Pts',(-39.923987884714,-13.83000002,-130.68030635931));
#146331=CARTESIAN_POINT('Ctrl Pts',(-39.4846775617168,-13.83000002,-130.885279386667));
#146332=CARTESIAN_POINT('Ctrl Pts',(-39.4710976496822,-14.3145440753934,
-130.89161549018));
#146333=CARTESIAN_POINT('Ctrl Pts',(-39.6450175280278,-13.83000002,-130.082400567686));
#146334=CARTESIAN_POINT('Ctrl Pts',(-39.1694803296317,-13.83000002,-130.222011573448));
#146335=CARTESIAN_POINT('Ctrl Pts',(-39.1611309974652,-14.3198673792142,
-130.227665983087));
#146336=CARTESIAN_POINT('Ctrl Pts',(-39.5000000016417,-13.83000002,-129.435305216167));
#146337=CARTESIAN_POINT('Ctrl Pts',(-39.0048700588287,-13.83000002,-129.505450476954));
#146338=CARTESIAN_POINT('Ctrl Pts',(-39.,-14.325106270286,-129.50903420183));
#146339=CARTESIAN_POINT('Ctrl Pts',(-39.5,-13.83000002,-128.768820397718));
#146340=CARTESIAN_POINT('Ctrl Pts',(-38.9999999999999,-13.83000002,-128.768820397718));
#146341=CARTESIAN_POINT('Ctrl Pts',(-39.,-14.33000002,-128.768820397718));
#146342=CARTESIAN_POINT('',(-39.4710976496822,-14.3145440753934,-130.89161549018));
#146343=CARTESIAN_POINT('Origin',(-39.923987884714,-14.33000002,-130.68030635931));
#146344=CARTESIAN_POINT('Origin',(-46.4348610974772,-14.3111430565211,-128.233135964139));
#146345=CARTESIAN_POINT('Ctrl Pts',(-39.4710976496822,-14.3145440753934,
-130.89161549018));
#146346=CARTESIAN_POINT('Ctrl Pts',(-39.4846775617168,-13.83000002,-130.885279386667));
#146347=CARTESIAN_POINT('Ctrl Pts',(-39.923987884714,-13.83000002,-130.68030635931));
#146348=CARTESIAN_POINT('Ctrl Pts',(-45.7785509549148,-14.3169830983588,
-144.410301102566));
#146349=CARTESIAN_POINT('Ctrl Pts',(-45.8048635488014,-13.83000002,-144.43668735532));
#146350=CARTESIAN_POINT('Ctrl Pts',(-46.2315241188232,-13.83000002,-144.198991310165));
#146351=CARTESIAN_POINT('Ctrl Pts',(-52.0847736772191,-14.3183867301138,
-157.929583215096));
#146352=CARTESIAN_POINT('Ctrl Pts',(-52.1020957034304,-13.8300000201034,
-157.939875120093));
#146353=CARTESIAN_POINT('Ctrl Pts',(-52.5377799111353,-13.83000002,-157.718273616974));
#146354=CARTESIAN_POINT('Ctrl Pts',(-58.3906572805143,-14.3195102506022,
-171.449026400902));
#146355=CARTESIAN_POINT('Ctrl Pts',(-58.3999663918639,-13.83000002,-171.444684327491));
#146356=CARTESIAN_POINT('Ctrl Pts',(-58.8436897472855,-13.83000002,-171.237717270032));
#146357=CARTESIAN_POINT('',(-58.3906572805143,-14.3195102506022,-171.449026400902));
#146358=CARTESIAN_POINT('Origin',(-58.8436897472855,-14.33000002,-171.237717270032));
#146359=CARTESIAN_POINT('Ctrl Pts',(-58.3906572805143,-14.3195102506022,
-171.449026400902));
#146360=CARTESIAN_POINT('Ctrl Pts',(-52.0847736772191,-14.3183867301138,
-157.929583215096));
#146361=CARTESIAN_POINT('Ctrl Pts',(-45.7785509549148,-14.3169830983588,
-144.410301102566));
#146362=CARTESIAN_POINT('Ctrl Pts',(-39.4710976496822,-14.3145440753934,
-130.89161549018));
#146363=CARTESIAN_POINT('Ctrl Pts',(-58.3906572805143,-14.3195102506022,
-171.449026400902));
#146364=CARTESIAN_POINT('Ctrl Pts',(-58.3999663918639,-13.83000002,-171.444684327491));
#146365=CARTESIAN_POINT('Ctrl Pts',(-58.8436897472855,-13.83000002,-171.237717270032));
#146366=CARTESIAN_POINT('Ctrl Pts',(-58.452336355597,-14.3188132239679,
-171.581227559315));
#146367=CARTESIAN_POINT('Ctrl Pts',(-58.4628431558437,-13.8300000200007,
-171.577873523862));
#146368=CARTESIAN_POINT('Ctrl Pts',(-58.9361841983689,-13.83000002,-171.436019148456));
#146369=CARTESIAN_POINT('Ctrl Pts',(-58.484398987579,-14.3184534099214,
-171.72428852145));
#146370=CARTESIAN_POINT('Ctrl Pts',(-58.4956819559116,-13.83000002,-171.722618633075));
#146371=CARTESIAN_POINT('Ctrl Pts',(-58.9842656416468,-13.83000002,-171.650610345097));
#146372=CARTESIAN_POINT('Ctrl Pts',(-58.4843989875811,-14.3184534098307,
-171.871644662643));
#146373=CARTESIAN_POINT('Ctrl Pts',(-58.4956819583251,-13.83000002,-171.871644662643));
#146374=CARTESIAN_POINT('Ctrl Pts',(-58.9842656455947,-13.83000002,-171.871644662643));
#146375=CARTESIAN_POINT('Origin',(-58.9842656455946,-14.33000002,-171.871644662643));
#146376=CARTESIAN_POINT('Origin',(-57.4849665102709,-14.329895034911,-171.871652207609));
#146377=CARTESIAN_POINT('Origin',(-58.9842656455947,-14.33000002,-179.64995));
#146378=CARTESIAN_POINT('Origin',(-58.9842656455946,-14.33000002,-176.2719717603));
#146379=CARTESIAN_POINT('Ctrl Pts',(-60.,-13.33000002,-174.751208632418));
#146380=CARTESIAN_POINT('Ctrl Pts',(-60.,-13.83000002,-174.751208632417));
#146381=CARTESIAN_POINT('Ctrl Pts',(-59.5,-13.83000002,-174.751208632418));
#146382=CARTESIAN_POINT('Ctrl Pts',(-60.,-13.3301495200469,-174.995764866376));
#146383=CARTESIAN_POINT('Ctrl Pts',(-59.9998505155736,-13.83000002,-174.995728395116));
#146384=CARTESIAN_POINT('Ctrl Pts',(-59.499999994458,-13.83000002,-174.955005950799));
#146385=CARTESIAN_POINT('Ctrl Pts',(-59.9705302647519,-13.3302950638363,
-175.235357479373));
#146386=CARTESIAN_POINT('Ctrl Pts',(-59.9702437452671,-13.8300000199993,
-175.235287718005));
#146387=CARTESIAN_POINT('Ctrl Pts',(-59.4754418884424,-13.83000002,-175.154666905584));
#146388=CARTESIAN_POINT('Ctrl Pts',(-59.8546684450659,-13.3305785951146,
-175.704793574078));
#146389=CARTESIAN_POINT('Ctrl Pts',(-59.8541239849711,-13.8300000200007,
-175.704587709371));
#146390=CARTESIAN_POINT('Ctrl Pts',(-59.3788903697392,-13.83000002,-175.545864512034));
#146391=CARTESIAN_POINT('Ctrl Pts',(-59.7669119843163,-13.3307170303008,
-175.935426552567));
#146392=CARTESIAN_POINT('Ctrl Pts',(-59.7662611489698,-13.8300000199988,
-175.935125812779));
#146393=CARTESIAN_POINT('Ctrl Pts',(-59.3057599866248,-13.83000002,-175.738059080183));
#146394=CARTESIAN_POINT('Ctrl Pts',(-59.5422070340633,-13.3309719059141,
-176.362223209373));
#146395=CARTESIAN_POINT('Ctrl Pts',(-59.5413945721013,-13.8300000200012,
-176.361684206804));
#146396=CARTESIAN_POINT('Ctrl Pts',(-59.1185058620249,-13.83000002,-176.093723731171));
#146397=CARTESIAN_POINT('Ctrl Pts',(-59.4027363887007,-13.331091646732,
-176.563890694693));
#146398=CARTESIAN_POINT('Ctrl Pts',(-59.4018755020326,-13.8300000199995,
-176.563219594419));
#146399=CARTESIAN_POINT('Ctrl Pts',(-59.0022803225031,-13.83000002,-176.261780328219));
#146400=CARTESIAN_POINT('Ctrl Pts',(-59.0800292616587,-13.3313061338651,
-176.92662799811));
#146401=CARTESIAN_POINT('Ctrl Pts',(-59.0791375439908,-13.8300000200005,
-176.925670411677));
#146402=CARTESIAN_POINT('Ctrl Pts',(-58.7333577194631,-13.83000002,-176.564062061699));
#146403=CARTESIAN_POINT('Ctrl Pts',(-58.8992210551541,-13.3313999972609,
-177.086172425279));
#146404=CARTESIAN_POINT('Ctrl Pts',(-58.8983479608961,-13.830000020003,
-177.085078467603));
#146405=CARTESIAN_POINT('Ctrl Pts',(-58.5826842101506,-13.83000002,-176.697016027753));
#146406=CARTESIAN_POINT('Ctrl Pts',(-58.6989442326066,-13.3314807280565,
-177.223786737086));
#146407=CARTESIAN_POINT('Ctrl Pts',(-58.698108161756,-13.83000002,-177.222569964948));
#146408=CARTESIAN_POINT('Ctrl Pts',(-58.4157868605055,-13.83000002,-176.811694866106));
#146409=CARTESIAN_POINT('',(-60.,-13.33000002,-174.751208632418));
#146410=CARTESIAN_POINT('Origin',(-59.5,-13.33000002,-174.751208632418));
#146411=CARTESIAN_POINT('',(-58.7133156820334,-13.3314748988427,-177.213850299147));
#146412=CARTESIAN_POINT('Ctrl Pts',(-60.,-13.33000002,-174.751208632418));
#146413=CARTESIAN_POINT('Ctrl Pts',(-59.9999999999956,-13.3301495346025,
-174.995764866375));
#146414=CARTESIAN_POINT('Ctrl Pts',(-59.9705302647436,-13.3302950783898,
-175.235357479371));
#146415=CARTESIAN_POINT('Ctrl Pts',(-59.8546684450501,-13.330578609664,
-175.704793574072));
#146416=CARTESIAN_POINT('Ctrl Pts',(-59.7669119842973,-13.3307170448482,
-175.935426552558));
#146417=CARTESIAN_POINT('Ctrl Pts',(-59.5422070340396,-13.3309719204577,
-176.362223209358));
#146418=CARTESIAN_POINT('Ctrl Pts',(-59.4027363886756,-13.3310916612739,
-176.563890694673));
#146419=CARTESIAN_POINT('Ctrl Pts',(-59.0838978236773,-13.3313035771661,
-176.922279560609));
#146420=CARTESIAN_POINT('Ctrl Pts',(-58.9078798727822,-13.3313955032287,
-177.078509506427));
#146421=CARTESIAN_POINT('Ctrl Pts',(-58.7133155825256,-13.3314748983292,
-177.213850156091));
#146422=CARTESIAN_POINT('Ctrl Pts',(-58.9842656455839,-13.8300000182384,
-176.2719717603));
#146423=CARTESIAN_POINT('Ctrl Pts',(-58.9705475680472,-13.8299985684035,
-176.318283990653));
#146424=CARTESIAN_POINT('Ctrl Pts',(-58.9568482086768,-13.8291036195285,
-176.363544967324));
#146425=CARTESIAN_POINT('Ctrl Pts',(-58.9433630154086,-13.8271227458294,
-176.407719581748));
#146426=CARTESIAN_POINT('Ctrl Pts',(-58.9375094778774,-13.8262629050906,
-176.426894521128));
#146427=CARTESIAN_POINT('Ctrl Pts',(-58.9316958151412,-13.8251982285538,
-176.445864414423));
#146428=CARTESIAN_POINT('Ctrl Pts',(-58.9259357951406,-13.8239121842354,
-176.464624333952));
#146429=CARTESIAN_POINT('Ctrl Pts',(-58.9141476212573,-13.8212802291303,
-176.503017463389));
#146430=CARTESIAN_POINT('Ctrl Pts',(-58.9026487920717,-13.8177209175776,
-176.540494484498));
#146431=CARTESIAN_POINT('Ctrl Pts',(-58.8915082859054,-13.8130914358196,
-176.577029027276));
#146432=CARTESIAN_POINT('Ctrl Pts',(-58.8808983823344,-13.8086824480856,
-176.61182349443));
#146433=CARTESIAN_POINT('Ctrl Pts',(-58.8706133980374,-13.8033020833572,
-176.645763126895));
#146434=CARTESIAN_POINT('Ctrl Pts',(-58.8607007260993,-13.7968342336531,
-176.678780444292));
#146435=CARTESIAN_POINT('Ctrl Pts',(-58.8510239250903,-13.7905202857153,
-176.711012118285));
#146436=CARTESIAN_POINT('Ctrl Pts',(-58.8417018329604,-13.7831691988171,
-176.742364795295));
#146437=CARTESIAN_POINT('Ctrl Pts',(-58.8327678658211,-13.7746910572516,
-176.77273210973));
#146438=CARTESIAN_POINT('Ctrl Pts',(-58.8241038159165,-13.7664690613032,
-176.802181952519));
#146439=CARTESIAN_POINT('Ctrl Pts',(-58.8158046324015,-13.7571863673228,
-176.830704717276));
#146440=CARTESIAN_POINT('Ctrl Pts',(-58.8078925277743,-13.7467891715621,
-176.858164968786));
#146441=CARTESIAN_POINT('Ctrl Pts',(-58.8013265549649,-13.7381609104514,
-176.880953249939));
#146442=CARTESIAN_POINT('Ctrl Pts',(-58.7950269503204,-13.7287653913972,
-176.903008963654));
#146443=CARTESIAN_POINT('Ctrl Pts',(-58.7890032485162,-13.7185926712373,
-176.924237158836));
#146444=CARTESIAN_POINT('Ctrl Pts',(-58.7821559295512,-13.7070290411075,
-176.948367872505));
#146445=CARTESIAN_POINT('Ctrl Pts',(-58.7757052330373,-13.6944274034058,
-176.971448103492));
#146446=CARTESIAN_POINT('Ctrl Pts',(-58.7696820480974,-13.6807980296988,
-176.993291172281));
#146447=CARTESIAN_POINT('Ctrl Pts',(-58.7637361328157,-13.6673435031963,
-177.014854022801));
#146448=CARTESIAN_POINT('Ctrl Pts',(-58.7582066537988,-13.652887074821,
-177.035210397418));
#146449=CARTESIAN_POINT('Ctrl Pts',(-58.7531241153642,-13.6374870520949,
-177.054167379287));
#146450=CARTESIAN_POINT('Ctrl Pts',(-58.748098500889,-13.622259508196,-177.072912044716));
#146451=CARTESIAN_POINT('Ctrl Pts',(-58.7435097100686,-13.6061093469723,
-177.09028749886));
#146452=CARTESIAN_POINT('Ctrl Pts',(-58.7393905432394,-13.5891436743187,
-177.106107850033));
#146453=CARTESIAN_POINT('Ctrl Pts',(-58.7366479699053,-13.5778477974228,
-177.116641162973));
#146454=CARTESIAN_POINT('Ctrl Pts',(-58.734113656591,-13.566191488644,-177.126485125293));
#146455=CARTESIAN_POINT('Ctrl Pts',(-58.731798600167,-13.5542186631085,
-177.135588421566));
#146456=CARTESIAN_POINT('Ctrl Pts',(-58.7283814629564,-13.5365461834111,
-177.149025334857));
#146457=CARTESIAN_POINT('Ctrl Pts',(-58.7254282875152,-13.5181135256879,
-177.160900208221));
#146458=CARTESIAN_POINT('Ctrl Pts',(-58.7229449134023,-13.4990734099497,
-177.171064863308));
#146459=CARTESIAN_POINT('Ctrl Pts',(-58.720478237815,-13.4801613223885,
-177.181161169952));
#146460=CARTESIAN_POINT('Ctrl Pts',(-58.718474856036,-13.4606504791436,
-177.189569223433));
#146461=CARTESIAN_POINT('Ctrl Pts',(-58.7169426300318,-13.4407334079337,
-177.196171639718));
#146462=CARTESIAN_POINT('Ctrl Pts',(-58.7154162187833,-13.4208919214619,
-177.202749000014));
#146463=CARTESIAN_POINT('Ctrl Pts',(-58.7143572377876,-13.4006482027158,
-177.207533658972));
#146464=CARTESIAN_POINT('Ctrl Pts',(-58.7137783664067,-13.3802242025167,
-177.210450127637));
#146465=CARTESIAN_POINT('Ctrl Pts',(-58.7133198720031,-13.3640473969248,
-177.21276011325));
#146466=CARTESIAN_POINT('Ctrl Pts',(-58.7131626636372,-13.3477583510132,
-177.213898867151));
#146467=CARTESIAN_POINT('Ctrl Pts',(-58.7133159805679,-13.3314749003853,
-177.213850728308));
#146468=CARTESIAN_POINT('Origin',(-59.5,-13.33000002,-55.24995));
#146469=CARTESIAN_POINT('',(-60.,-13.33000002,-174.748117418411));
#146470=CARTESIAN_POINT('Origin',(-60.,-2.55003103885676E-14,0.));
#146471=CARTESIAN_POINT('',(-60.,-12.83000002,-174.751778045593));
#146472=CARTESIAN_POINT('',(-60.,-12.83000002,-57.911664394164));
#146473=CARTESIAN_POINT('Origin',(-60.,-12.9674774176428,-75.9457339865586));
#146474=CARTESIAN_POINT('Origin',(-59.5,-12.83000002,-55.24995));
#146475=CARTESIAN_POINT('Origin',(-59.5,-12.83000002,-174.751778045594));
#146476=CARTESIAN_POINT('Ctrl Pts',(-39.4702993039609,-11.842906113671,
-101.183667521985));
#146477=CARTESIAN_POINT('Ctrl Pts',(-39.4816972464314,-12.33000002,-101.188984626754));
#146478=CARTESIAN_POINT('Ctrl Pts',(-39.9232693735648,-12.33000002,-101.394976652855));
#146479=CARTESIAN_POINT('Ctrl Pts',(-45.741803891981,-11.8408803347909,
-87.7397145657271));
#146480=CARTESIAN_POINT('Ctrl Pts',(-45.7637467547491,-12.3300000200387,
-87.7178689736084));
#146481=CARTESIAN_POINT('Ctrl Pts',(-46.1948314689912,-12.33000002,-87.9510241496856));
#146482=CARTESIAN_POINT('Ctrl Pts',(-52.0124594137882,-11.8397106642502,
-74.2953500811619));
#146483=CARTESIAN_POINT('Ctrl Pts',(-52.0269437270063,-12.3300000197686,
-74.2868280745294));
#146484=CARTESIAN_POINT('Ctrl Pts',(-52.4655100689676,-12.33000002,-74.5066595330064));
#146485=CARTESIAN_POINT('Ctrl Pts',(-58.2828791719688,-11.838774304476,
-60.8508735991007));
#146486=CARTESIAN_POINT('Ctrl Pts',(-58.2906927660831,-12.33000002,-60.8545178210735));
#146487=CARTESIAN_POINT('Ctrl Pts',(-58.7359481105893,-12.33000002,-61.0621827299711));
#146488=CARTESIAN_POINT('Origin',(-39.9232693735648,-11.83000002,-101.394976652855));
#146489=CARTESIAN_POINT('Ctrl Pts',(-59.5,-12.33000002,-174.751778045593));
#146490=CARTESIAN_POINT('Ctrl Pts',(-60.,-12.33000002,-174.751778045593));
#146491=CARTESIAN_POINT('Ctrl Pts',(-60.,-12.83000002,-174.751778045593));
#146492=CARTESIAN_POINT('Ctrl Pts',(-59.4999999944591,-12.33000002,-174.955507700223));
#146493=CARTESIAN_POINT('Ctrl Pts',(-59.9999432570754,-12.33000002,-174.996239713811));
#146494=CARTESIAN_POINT('Ctrl Pts',(-60.,-12.8299432805227,-174.99625355239));
#146495=CARTESIAN_POINT('Ctrl Pts',(-59.4754576845908,-12.33000002,-175.155103617038));
#146496=CARTESIAN_POINT('Ctrl Pts',(-59.970440441932,-12.33000002,-175.235742099222));
#146497=CARTESIAN_POINT('Ctrl Pts',(-59.9705492201332,-12.8298880430416,
-175.2357685753));
#146498=CARTESIAN_POINT('Ctrl Pts',(-59.3789691429701,-12.33000002,-175.546176541216));
#146499=CARTESIAN_POINT('Ctrl Pts',(-59.8545561835904,-12.33000002,-175.704977777008));
#146500=CARTESIAN_POINT('Ctrl Pts',(-59.8547629729398,-12.8297804365705,
-175.705055936053));
#146501=CARTESIAN_POINT('Ctrl Pts',(-59.3058851982286,-12.33000002,-175.738316981093));
#146502=CARTESIAN_POINT('Ctrl Pts',(-59.7668149966741,-12.3300000199993,
-175.935510188038));
#146503=CARTESIAN_POINT('Ctrl Pts',(-59.7670622382429,-12.8297278961218,
-175.935624391263));
#146504=CARTESIAN_POINT('Ctrl Pts',(-59.1187478700854,-12.33000002,-176.093893786804));
#146505=CARTESIAN_POINT('Ctrl Pts',(-59.5421886833106,-12.3300000200007,
-176.362111673427));
#146506=CARTESIAN_POINT('Ctrl Pts',(-59.5424974437338,-12.829631160742,
-176.362316424594));
#146507=CARTESIAN_POINT('Ctrl Pts',(-59.0025998517383,-12.33000002,-176.261909367341));
#146508=CARTESIAN_POINT('Ctrl Pts',(-59.4027925942033,-12.3300000200005,
-176.563680085108));
#146509=CARTESIAN_POINT('Ctrl Pts',(-59.4031198237833,-12.8295857148276,
-176.563935060575));
#146510=CARTESIAN_POINT('Ctrl Pts',(-58.73383039456,-12.33000002,-176.564162347066));
#146511=CARTESIAN_POINT('Ctrl Pts',(-59.0802573870172,-12.3300000199995,
-176.926274585031));
#146512=CARTESIAN_POINT('Ctrl Pts',(-59.0805964717746,-12.8295042980195,
-176.926638521725));
#146513=CARTESIAN_POINT('Ctrl Pts',(-58.5832426931945,-12.33000002,-176.697112268189));
#146514=CARTESIAN_POINT('Ctrl Pts',(-58.8995591592806,-12.3300000199849,
-177.085762552869));
#146515=CARTESIAN_POINT('Ctrl Pts',(-58.8998912349101,-12.8294686666967,
-177.086178383746));
#146516=CARTESIAN_POINT('Ctrl Pts',(-58.4164435759292,-12.33000002,-176.811801263203));
#146517=CARTESIAN_POINT('Ctrl Pts',(-58.699414230519,-12.33000002,-177.223342557405));
#146518=CARTESIAN_POINT('Ctrl Pts',(-58.699732291115,-12.8294380172077,
-177.223805132118));
#146519=CARTESIAN_POINT('',(-58.7141461350347,-12.8294402383603,-177.213832217127));
#146520=CARTESIAN_POINT('Ctrl Pts',(-58.7141461350374,-12.8294402383603,
-177.213832217125));
#146521=CARTESIAN_POINT('Ctrl Pts',(-58.9085758506643,-12.8294703748154,
-177.078488401254));
#146522=CARTESIAN_POINT('Ctrl Pts',(-59.0844765777018,-12.8295052680351,
-176.922275030383));
#146523=CARTESIAN_POINT('Ctrl Pts',(-59.4031198237771,-12.8295857053604,
-176.56393506057));
#146524=CARTESIAN_POINT('Ctrl Pts',(-59.542497443728,-12.8296311512744,
-176.36231642459));
#146525=CARTESIAN_POINT('Ctrl Pts',(-59.7670622382382,-12.8297278866533,
-175.93562439126));
#146526=CARTESIAN_POINT('Ctrl Pts',(-59.8547629729359,-12.8297804271015,
-175.705055936052));
#146527=CARTESIAN_POINT('Ctrl Pts',(-59.9705492201311,-12.8298880335715,
-175.235768575299));
#146528=CARTESIAN_POINT('Ctrl Pts',(-59.9999999999989,-12.8299432710521,
-174.996253552389));
#146529=CARTESIAN_POINT('Ctrl Pts',(-60.,-12.83000002,-174.751778045593));
#146530=CARTESIAN_POINT('Ctrl Pts',(-58.7141461350374,-12.8294402383603,
-177.213832217125));
#146531=CARTESIAN_POINT('Ctrl Pts',(-58.71386124121,-12.7496539972645,-177.213921724807));
#146532=CARTESIAN_POINT('Ctrl Pts',(-58.7207402303504,-12.6723026604245,
-177.185595547246));
#146533=CARTESIAN_POINT('Ctrl Pts',(-58.7409598721377,-12.5716812769085,
-177.108237839695));
#146534=CARTESIAN_POINT('Ctrl Pts',(-58.7491768361659,-12.5414135007217,
-177.077379300711));
#146535=CARTESIAN_POINT('Ctrl Pts',(-58.7686983660461,-12.486608549538,
-177.006030037118));
#146536=CARTESIAN_POINT('Ctrl Pts',(-58.7801197877863,-12.4620381958002,
-176.965157505607));
#146537=CARTESIAN_POINT('Ctrl Pts',(-58.817725908538,-12.3995214017445,
-176.833790628028));
#146538=CARTESIAN_POINT('Ctrl Pts',(-58.8482938287677,-12.3711206280572,
-176.731313674606));
#146539=CARTESIAN_POINT('Ctrl Pts',(-58.9148079297158,-12.3367286443605,
-176.512401023853));
#146540=CARTESIAN_POINT('Ctrl Pts',(-58.9511729872876,-12.33000002,-176.394565470062));
#146541=CARTESIAN_POINT('Ctrl Pts',(-58.9890336736409,-12.33000002,-176.26629097911));
#146542=CARTESIAN_POINT('Origin',(-58.9890336736409,-11.83000002,-179.64995));
#146543=CARTESIAN_POINT('Origin',(-58.9890336736409,-11.83000002,-176.26629097911));
#146544=CARTESIAN_POINT('Origin',(-58.9890336736409,-11.83000002,-171.871644662643));
#146545=CARTESIAN_POINT('Ctrl Pts',(-58.48912660861,-11.8396398505087,-171.871644662643));
#146546=CARTESIAN_POINT('Ctrl Pts',(-58.4985823439911,-12.33000002,-171.871644662643));
#146547=CARTESIAN_POINT('Ctrl Pts',(-58.9890336736409,-12.33000002,-171.871644662643));
#146548=CARTESIAN_POINT('Ctrl Pts',(-58.4891266086039,-11.8396398501934,
-171.725770040011));
#146549=CARTESIAN_POINT('Ctrl Pts',(-58.4985823327705,-12.33000002,-171.724385262387));
#146550=CARTESIAN_POINT('Ctrl Pts',(-58.9890336571231,-12.33000002,-171.652832645897));
#146551=CARTESIAN_POINT('Ctrl Pts',(-58.4576958292209,-11.8393453695788,
-171.582571135794));
#146552=CARTESIAN_POINT('Ctrl Pts',(-58.46651035226,-12.3300000200013,-171.579769437466));
#146553=CARTESIAN_POINT('Ctrl Pts',(-58.9418960593107,-12.33000002,-171.438034482585));
#146554=CARTESIAN_POINT('Ctrl Pts',(-58.3953999019963,-11.8387575339013,
-171.449026400902));
#146555=CARTESIAN_POINT('Ctrl Pts',(-58.4031988243933,-12.33000002,-171.445389024352));
#146556=CARTESIAN_POINT('Ctrl Pts',(-58.8484691650909,-12.33000002,-171.237717270032));
#146557=CARTESIAN_POINT('',(-58.3953999019963,-11.8387575339013,-171.449026400902));
#146558=CARTESIAN_POINT('Origin',(-58.8484691650909,-11.83000002,-171.237717270032));
#146559=CARTESIAN_POINT('Origin',(-57.4895222060999,-11.8300902499738,-171.871649915017));
#146560=CARTESIAN_POINT('Ctrl Pts',(-58.3953999019963,-11.8387575339013,
-171.449026400902));
#146561=CARTESIAN_POINT('Ctrl Pts',(-58.4031988243933,-12.33000002,-171.445389024352));
#146562=CARTESIAN_POINT('Ctrl Pts',(-58.8484691650909,-12.33000002,-171.237717270032));
#146563=CARTESIAN_POINT('Ctrl Pts',(-52.0874768317228,-11.839695897332,
-157.924129189572));
#146564=CARTESIAN_POINT('Ctrl Pts',(-52.1019974789428,-12.3300000202716,
-157.93276270106));
#146565=CARTESIAN_POINT('Ctrl Pts',(-52.5405278046811,-12.33000002,-157.712819732222));
#146566=CARTESIAN_POINT('Ctrl Pts',(-45.7793173035632,-11.8408682174628,
-144.399344282617));
#146567=CARTESIAN_POINT('Ctrl Pts',(-45.801395679434,-12.33000002,-144.421507685211));
#146568=CARTESIAN_POINT('Ctrl Pts',(-46.2323452217992,-12.33000002,-144.188034690057));
#146569=CARTESIAN_POINT('Ctrl Pts',(-39.4702993039609,-11.842906113671,
-130.874975449521));
#146570=CARTESIAN_POINT('Ctrl Pts',(-39.4816972464314,-12.33000002,-130.869658344752));
#146571=CARTESIAN_POINT('Ctrl Pts',(-39.9232693735648,-12.33000002,-130.663666318651));
#146572=CARTESIAN_POINT('',(-39.4702993039609,-11.842906113671,-130.874975449521));
#146573=CARTESIAN_POINT('Origin',(-39.9232693735648,-11.83000002,-130.663666318651));
#146574=CARTESIAN_POINT('Ctrl Pts',(-39.4702993039609,-11.842906113671,
-130.874975449521));
#146575=CARTESIAN_POINT('Ctrl Pts',(-45.7793173035632,-11.8408682174628,
-144.399344282617));
#146576=CARTESIAN_POINT('Ctrl Pts',(-52.0874768317228,-11.839695897332,
-157.924129189572));
#146577=CARTESIAN_POINT('Ctrl Pts',(-58.3953999019963,-11.8387575339013,
-171.449026400902));
#146578=CARTESIAN_POINT('Ctrl Pts',(-39.5,-12.33000002,-128.755118184993));
#146579=CARTESIAN_POINT('Ctrl Pts',(-39.,-12.33000002,-128.755118184993));
#146580=CARTESIAN_POINT('Ctrl Pts',(-39.,-11.83000002,-128.755118184993));
#146581=CARTESIAN_POINT('Ctrl Pts',(-39.5000000055219,-12.33000002,-129.413887248834));
#146582=CARTESIAN_POINT('Ctrl Pts',(-39.0040281122736,-12.33000002,-129.483935534574));
#146583=CARTESIAN_POINT('Ctrl Pts',(-39.,-11.8340442872404,-129.486859645108));
#146584=CARTESIAN_POINT('Ctrl Pts',(-39.6419410176262,-12.33000002,-130.060600444225));
#146585=CARTESIAN_POINT('Ctrl Pts',(-39.1646430478985,-12.33000002,-130.200415506093));
#146586=CARTESIAN_POINT('Ctrl Pts',(-39.1577125252496,-11.8384144493887,
-130.205177204234));
#146587=CARTESIAN_POINT('Ctrl Pts',(-39.9232693735648,-12.33000002,-130.663666318651));
#146588=CARTESIAN_POINT('Ctrl Pts',(-39.4816972464314,-12.33000002,-130.869658344752));
#146589=CARTESIAN_POINT('Ctrl Pts',(-39.4702993039609,-11.8429061136709,
-130.874975449521));
#146590=CARTESIAN_POINT('',(-39.,-11.8300000206964,-128.75511820843));
#146591=CARTESIAN_POINT('Origin',(-39.5,-11.83000002,-128.755118184993));
#146592=CARTESIAN_POINT('Origin',(-46.4327247058357,-11.8457999179355,-128.216011994814));
#146593=CARTESIAN_POINT('Origin',(-39.5,-11.83000002,-55.24995));
#146594=CARTESIAN_POINT('',(-39.,-11.8300000202903,-103.303524781275));
#146595=CARTESIAN_POINT('Origin',(-39.5,-11.83000002,-103.303524786513));
#146596=CARTESIAN_POINT('',(-39.,-11.83000002,-129.34995));
#146597=CARTESIAN_POINT('Ctrl Pts',(-39.9232693735648,-12.33000002,-101.394976652855));
#146598=CARTESIAN_POINT('Ctrl Pts',(-39.4816972464314,-12.33000002,-101.188984626754));
#146599=CARTESIAN_POINT('Ctrl Pts',(-39.4702993039609,-11.842906113671,
-101.183667521985));
#146600=CARTESIAN_POINT('Ctrl Pts',(-39.6447687306727,-12.33000002,-101.991980946201));
#146601=CARTESIAN_POINT('Ctrl Pts',(-39.1678459389433,-12.3300000200023,
-101.851466764233));
#146602=CARTESIAN_POINT('Ctrl Pts',(-39.1608544296035,-11.8384595965422,
-101.84673342232));
#146603=CARTESIAN_POINT('Ctrl Pts',(-39.5000000016323,-12.33000002,-102.638067201068));
#146604=CARTESIAN_POINT('Ctrl Pts',(-39.0040688095373,-12.3300000199977,
-102.567343181294));
#146605=CARTESIAN_POINT('Ctrl Pts',(-39.,-11.834085348836,-102.564353929887));
#146606=CARTESIAN_POINT('Ctrl Pts',(-39.5,-12.33000002,-103.303524786513));
#146607=CARTESIAN_POINT('Ctrl Pts',(-39.,-12.33000002,-103.303524786513));
#146608=CARTESIAN_POINT('Ctrl Pts',(-39.,-11.83000002,-103.303524786513));
#146609=CARTESIAN_POINT('Origin',(-46.4332003469387,-11.8458180863447,-103.839606692281));
#146610=CARTESIAN_POINT('Ctrl Pts',(-39.5330007135517,-6.22310220971892,
-99.8586617838914));
#146611=CARTESIAN_POINT('Ctrl Pts',(-39.,-5.86351617202512,-100.855722952121));
#146612=CARTESIAN_POINT('Ctrl Pts',(-39.,-5.46102446043621,-101.971753092595));
#146613=CARTESIAN_POINT('Ctrl Pts',(-39.5158163721933,-7.1434218710037,
-100.226898392254));
#146614=CARTESIAN_POINT('Ctrl Pts',(-39.0000000000075,-6.82975403393395,
-101.225648609944));
#146615=CARTESIAN_POINT('Ctrl Pts',(-39.,-6.48207062104881,-102.33998922066));
#146616=CARTESIAN_POINT('Ctrl Pts',(-39.50142226749,-8.08385740698738,-100.53114117287));
#146617=CARTESIAN_POINT('Ctrl Pts',(-39.,-7.81966925102655,-101.531783862877));
#146618=CARTESIAN_POINT('Ctrl Pts',(-39.,-7.52739464652098,-102.644232481647));
#146619=CARTESIAN_POINT('Ctrl Pts',(-39.485193560998,-9.53196095727464,
-100.872391313355));
#146620=CARTESIAN_POINT('Ctrl Pts',(-39.,-9.34536808184436,-101.875027810475));
#146621=CARTESIAN_POINT('Ctrl Pts',(-39.,-9.13906178103241,-102.985482622022));
#146622=CARTESIAN_POINT('Ctrl Pts',(-39.4806657492121,-10.0234751165263,
-100.967196566129));
#146623=CARTESIAN_POINT('Ctrl Pts',(-39.,-9.86335482772211,-101.970380205613));
#146624=CARTESIAN_POINT('Ctrl Pts',(-39.,-9.68642581410213,-103.080287874832));
#146625=CARTESIAN_POINT('Ctrl Pts',(-39.4737139394979,-11.0038787161503,
-101.11251041402));
#146626=CARTESIAN_POINT('Ctrl Pts',(-39.,-10.8967689955421,-102.116504004052));
#146627=CARTESIAN_POINT('Ctrl Pts',(-39.,-10.7786703656218,-103.225601722724));
#146628=CARTESIAN_POINT('Ctrl Pts',(-39.4712727906473,-11.493239882702,
-101.16338521793));
#146629=CARTESIAN_POINT('Ctrl Pts',(-39.0000000000038,-11.4127969575427,
-102.167673995048));
#146630=CARTESIAN_POINT('Ctrl Pts',(-39.,-11.32407160958,-103.276476522877));
#146631=CARTESIAN_POINT('Ctrl Pts',(-39.4698732852484,-11.9818774403001,
-101.192544694569));
#146632=CARTESIAN_POINT('Ctrl Pts',(-39.,-11.9281041096302,-102.196998431102));
#146633=CARTESIAN_POINT('Ctrl Pts',(-39.,-11.8687533077036,-103.305636003273));
#146634=CARTESIAN_POINT('',(-39.,-6.18000001999998,-102.218950121094));
#146635=CARTESIAN_POINT('Ctrl Pts',(-39.0000000000558,-6.18000001999998,
-102.218950121094));
#146636=CARTESIAN_POINT('Ctrl Pts',(-39.0000000001314,-6.5292524637215,
-102.333137272009));
#146637=CARTESIAN_POINT('Ctrl Pts',(-39.0000000002528,-6.88066423664115,
-102.43942079016));
#146638=CARTESIAN_POINT('Ctrl Pts',(-39.0000000003133,-7.23418430799942,
-102.53736711789));
#146639=CARTESIAN_POINT('Ctrl Pts',(-39.0000000003723,-7.57920291835826,
-102.632958029471));
#146640=CARTESIAN_POINT('Ctrl Pts',(-39.0000000003716,-7.92622968243009,
-102.720607819346));
#146641=CARTESIAN_POINT('Ctrl Pts',(-39.0000000003073,-8.2751996248623,
-102.799960112763));
#146642=CARTESIAN_POINT('Ctrl Pts',(-39.0000000002873,-8.38389527497889,
-102.824676422314));
#146643=CARTESIAN_POINT('Ctrl Pts',(-39.0000000002619,-8.49277931386626,
-102.848588085813));
#146644=CARTESIAN_POINT('Ctrl Pts',(-39.0000000002334,-8.60184941027751,
-102.871685311886));
#146645=CARTESIAN_POINT('Ctrl Pts',(-39.0000000002017,-8.72319901066901,
-102.897382906795));
#146646=CARTESIAN_POINT('Ctrl Pts',(-39.0000000001662,-8.84492476936504,
-102.922084618583));
#146647=CARTESIAN_POINT('Ctrl Pts',(-39.0000000001318,-8.96688496783026,
-102.945759157014));
#146648=CARTESIAN_POINT('Ctrl Pts',(-39.0000000000546,-9.2409571131078,
-102.998961198483));
#146649=CARTESIAN_POINT('Ctrl Pts',(-39.0000000000303,-9.5168957930922,
-103.04710594614));
#146650=CARTESIAN_POINT('Ctrl Pts',(-39.0000000000166,-9.79353842563631,
-103.08982360864));
#146651=CARTESIAN_POINT('Ctrl Pts',(-39.0000000000094,-9.93973590489248,
-103.112398634476));
#146652=CARTESIAN_POINT('Ctrl Pts',(-39.0000000000059,-10.0861301614979,
-103.133457170461));
#146653=CARTESIAN_POINT('Ctrl Pts',(-39.0000000000038,-10.2325489057379,
-103.152938666286));
#146654=CARTESIAN_POINT('Ctrl Pts',(-38.9999999999998,-10.5104673644924,
-103.189916631927));
#146655=CARTESIAN_POINT('Ctrl Pts',(-39.0000000000001,-10.7886085240243,
-103.221310636521));
#146656=CARTESIAN_POINT('Ctrl Pts',(-39.,-11.0672887212858,-103.24709706551));
#146657=CARTESIAN_POINT('Ctrl Pts',(-39.,-11.3209998818248,-103.270573096062));
#146658=CARTESIAN_POINT('Ctrl Pts',(-39.,-11.5751577965224,-103.289400790235));
#146659=CARTESIAN_POINT('Ctrl Pts',(-39.,-11.8300000206635,-103.303524774541));
#146660=CARTESIAN_POINT('Ctrl Pts',(-39.,-6.18000001999998,-102.218950121094));
#146661=CARTESIAN_POINT('Ctrl Pts',(-39.,-6.19216140385576,-101.811197248376));
#146662=CARTESIAN_POINT('Ctrl Pts',(-39.0453283089643,-6.20458878978192,
-101.411268531309));
#146663=CARTESIAN_POINT('Ctrl Pts',(-39.133992622656,-6.21727492932601,
-101.018951298921));
#146664=CARTESIAN_POINT('Ctrl Pts',(-39.2226569363477,-6.22996106887011,
-100.626634066533));
#146665=CARTESIAN_POINT('Ctrl Pts',(-39.3562549507175,-6.2429965854182,
-100.239515789679));
#146666=CARTESIAN_POINT('Ctrl Pts',(-39.5323905962559,-6.25584930059377,
-99.8717339663646));
#146667=CARTESIAN_POINT('Ctrl Pts',(-57.9034184448965,-6.23235646472971,
-60.8508735991007));
#146668=CARTESIAN_POINT('Ctrl Pts',(-57.8507724536939,-5.68000001999999,
-60.826158857425));
#146669=CARTESIAN_POINT('Ctrl Pts',(-58.3535376001277,-5.68000001999999,
-61.0621827299711));
#146670=CARTESIAN_POINT('Ctrl Pts',(-51.794541964381,-6.23776491179514,
-73.865008277307));
#146671=CARTESIAN_POINT('Ctrl Pts',(-51.698167660392,-5.68000001999999,
-73.9177186732266));
#146672=CARTESIAN_POINT('Ctrl Pts',(-52.2440275184664,-5.68000001999999,
-74.0763270103718));
#146673=CARTESIAN_POINT('Ctrl Pts',(-45.6775416788308,-6.24451367719405,
-86.8752616229197));
#146674=CARTESIAN_POINT('Ctrl Pts',(-45.5309288684318,-5.68000001999999,
-87.0138122441779));
#146675=CARTESIAN_POINT('Ctrl Pts',(-46.1262203434603,-5.68000001999998,
-87.0865851147193));
#146676=CARTESIAN_POINT('Ctrl Pts',(-39.532390596256,-6.25584930059378,
-99.8717339663645));
#146677=CARTESIAN_POINT('Ctrl Pts',(-39.4524980147409,-5.68000001999998,
-99.8339463478929));
#146678=CARTESIAN_POINT('Ctrl Pts',(-39.9791515366304,-5.68000001999998,
-100.083043097235));
#146679=CARTESIAN_POINT('Origin',(-39.9791515366304,-6.18000001999998,-100.083043097235));
#146680=CARTESIAN_POINT('Ctrl Pts',(-39.5,-5.68000001999998,-102.218950121094));
#146681=CARTESIAN_POINT('Ctrl Pts',(-39.,-5.68000001999997,-102.218950121094));
#146682=CARTESIAN_POINT('Ctrl Pts',(-39.,-6.18000001999998,-102.218950121094));
#146683=CARTESIAN_POINT('Ctrl Pts',(-39.5000000028438,-5.68000001999998,
-101.848394057804));
#146684=CARTESIAN_POINT('Ctrl Pts',(-38.9876888787772,-5.68000001999998,
-101.806176686079));
#146685=CARTESIAN_POINT('Ctrl Pts',(-39.,-6.19216140385576,-101.811197248376));
#146686=CARTESIAN_POINT('Ctrl Pts',(-39.5407954776771,-5.68000001999998,
-101.484716832152));
#146687=CARTESIAN_POINT('Ctrl Pts',(-39.0208449410789,-5.68000001999935,
-101.403186844504));
#146688=CARTESIAN_POINT('Ctrl Pts',(-39.0453283089643,-6.20458878978192,
-101.411268531309));
#146689=CARTESIAN_POINT('Ctrl Pts',(-39.7003912431037,-5.68000001999998,
-100.770720159946));
#146690=CARTESIAN_POINT('Ctrl Pts',(-39.1707994584459,-5.68000002000062,
-100.606268005686));
#146691=CARTESIAN_POINT('Ctrl Pts',(-39.2226569363477,-6.22996106887011,
-100.626634066533));
#146692=CARTESIAN_POINT('Ctrl Pts',(-39.8206290570768,-5.68000001999998,
-100.418199709297));
#146693=CARTESIAN_POINT('Ctrl Pts',(-39.2916053087195,-5.68000001999999,
-100.209430566875));
#146694=CARTESIAN_POINT('Ctrl Pts',(-39.3562549507175,-6.24299658541821,
-100.239515789679));
#146695=CARTESIAN_POINT('Ctrl Pts',(-39.9791515366304,-5.68000001999998,
-100.083043097235));
#146696=CARTESIAN_POINT('Ctrl Pts',(-39.4524980147409,-5.68000001999997,
-99.8339463478928));
#146697=CARTESIAN_POINT('Ctrl Pts',(-39.532390596256,-6.25584930059378,
-99.8717339663646));
#146698=CARTESIAN_POINT('Origin',(-39.5,-6.18000001999998,-102.218950121094));
#146699=CARTESIAN_POINT('Origin',(-39.5,-6.18000001999998,-55.24995));
#146700=CARTESIAN_POINT('',(-39.,-6.180000128392,-129.839693182379));
#146701=CARTESIAN_POINT('Origin',(-39.5,-6.18000001999998,-129.839692850412));
#146702=CARTESIAN_POINT('',(-39.,-6.18000001999998,-129.34995));
#146703=CARTESIAN_POINT('Ctrl Pts',(-39.9969223514525,-5.68000001999998,
-132.012776560392));
#146704=CARTESIAN_POINT('Ctrl Pts',(-39.470792948266,-5.68000002000005,
-132.267009143905));
#146705=CARTESIAN_POINT('Ctrl Pts',(-39.5521401151701,-6.25730737076538,
-132.227701231429));
#146706=CARTESIAN_POINT('Ctrl Pts',(-39.8295349406256,-5.68000001999998,
-131.666258024272));
#146707=CARTESIAN_POINT('Ctrl Pts',(-39.3006695783278,-5.68000001999948,
-131.878729031704));
#146708=CARTESIAN_POINT('Ctrl Pts',(-39.3661545598248,-6.24398265079956,
-131.8474745135));
#146709=CARTESIAN_POINT('Ctrl Pts',(-39.7053043876582,-5.68000001999998,
-131.307566389594));
#146710=CARTESIAN_POINT('Ctrl Pts',(-39.1755529568228,-5.68000001999998,
-131.474771483057));
#146711=CARTESIAN_POINT('Ctrl Pts',(-39.2281188468193,-6.23069539389422,
-131.453591269587));
#146712=CARTESIAN_POINT('Ctrl Pts',(-39.5388026007107,-5.68000001999998,
-130.56730645407));
#146713=CARTESIAN_POINT('Ctrl Pts',(-39.0189458914379,-5.68000001999998,
-130.64844019392));
#146714=CARTESIAN_POINT('Ctrl Pts',(-39.0431153529893,-6.20437672316564,
-130.640102780831));
#146715=CARTESIAN_POINT('Ctrl Pts',(-39.4969580610254,-5.68000001999998,
-130.182934036597));
#146716=CARTESIAN_POINT('Ctrl Pts',(-38.9852239260594,-5.68000001999999,
-130.222593346134));
#146717=CARTESIAN_POINT('Ctrl Pts',(-38.9966207132988,-6.19125736973878,
-130.217409891789));
#146718=CARTESIAN_POINT('Ctrl Pts',(-39.5001721107769,-5.68000001999998,
-129.798501466855));
#146719=CARTESIAN_POINT('Ctrl Pts',(-39.0015087008599,-5.68000001999997,
-129.794376582926));
#146720=CARTESIAN_POINT('Ctrl Pts',(-39.0001911577035,-6.17867888247173,
-129.794365306846));
#146721=CARTESIAN_POINT('',(-39.5323905961839,-6.25584930016544,-132.186909003948));
#146722=CARTESIAN_POINT('Origin',(-39.9791515366304,-6.18000001999998,-131.975599874271));
#146723=CARTESIAN_POINT('Ctrl Pts',(-39.5323905963862,-6.25584929916185,
-132.186909001152));
#146724=CARTESIAN_POINT('Ctrl Pts',(-39.4827974250407,-6.25223045792151,
-132.083355469824));
#146725=CARTESIAN_POINT('Ctrl Pts',(-39.4367726852657,-6.24860303206125,
-131.978767031507));
#146726=CARTESIAN_POINT('Ctrl Pts',(-39.3942214051111,-6.24498502939129,
-131.873200439616));
#146727=CARTESIAN_POINT('Ctrl Pts',(-39.3512191473345,-6.24132868150033,
-131.766515005461));
#146728=CARTESIAN_POINT('Ctrl Pts',(-39.3117636484726,-6.23768164276984,
-131.658829829889));
#146729=CARTESIAN_POINT('Ctrl Pts',(-39.2757918197085,-6.23404744051803,
-131.550165596048));
#146730=CARTESIAN_POINT('Ctrl Pts',(-39.2395417371362,-6.23038512652847,
-131.440660808978));
#146731=CARTESIAN_POINT('Ctrl Pts',(-39.2068288893847,-6.22673549716918,
-131.330160851267));
#146732=CARTESIAN_POINT('Ctrl Pts',(-39.1776335251109,-6.22309201957265,
-131.218661164678));
#146733=CARTESIAN_POINT('Ctrl Pts',(-39.1627061939244,-6.22122914174575,
-131.161652362414));
#146734=CARTESIAN_POINT('Ctrl Pts',(-39.1486991701159,-6.21936774251756,
-131.104381884175));
#146735=CARTESIAN_POINT('Ctrl Pts',(-39.1356148793413,-6.21750639488709,
-131.046847777288));
#146736=CARTESIAN_POINT('Ctrl Pts',(-39.1079099645233,-6.21356514362349,
-130.925024014895));
#146737=CARTESIAN_POINT('Ctrl Pts',(-39.0842950823765,-6.20962076305806,
-130.801786127621));
#146738=CARTESIAN_POINT('Ctrl Pts',(-39.0649315130416,-6.20569589299001,
-130.677528828003));
#146739=CARTESIAN_POINT('Ctrl Pts',(-39.0456626856946,-6.20179022650919,
-130.553879493961));
#146740=CARTESIAN_POINT('Ctrl Pts',(-39.0306039018712,-6.19790406888684,
-130.42922110532));
#146741=CARTESIAN_POINT('Ctrl Pts',(-39.0198687243699,-6.19405235733965,
-130.303965852542));
#146742=CARTESIAN_POINT('Ctrl Pts',(-39.0091916684706,-6.19022149944355,
-130.179388747469));
#146743=CARTESIAN_POINT('Ctrl Pts',(-39.002791676982,-6.18642488444214,
-130.054221669759));
#146744=CARTESIAN_POINT('Ctrl Pts',(-39.0007326738071,-6.18266722871172,
-129.928886829007));
#146745=CARTESIAN_POINT('Ctrl Pts',(-39.0002443724431,-6.1817760846664,
-129.899163138222));
#146746=CARTESIAN_POINT('Ctrl Pts',(-39.0000000000001,-6.18088708117259,
-129.869430069098));
#146747=CARTESIAN_POINT('Ctrl Pts',(-39.,-6.18000018270164,-129.839693348042));
#146748=CARTESIAN_POINT('Ctrl Pts',(-39.532390596256,-6.25584930059378,
-132.186909005141));
#146749=CARTESIAN_POINT('Ctrl Pts',(-39.452498014741,-5.68000001999998,
-132.224696623613));
#146750=CARTESIAN_POINT('Ctrl Pts',(-39.9791515366304,-5.68000001999998,
-131.975599874271));
#146751=CARTESIAN_POINT('Ctrl Pts',(-45.7155147614494,-6.24444363034862,
-145.263691191481));
#146752=CARTESIAN_POINT('Ctrl Pts',(-45.5680069655751,-5.68000001999999,
-145.12303284731));
#146753=CARTESIAN_POINT('Ctrl Pts',(-46.164205183661,-5.68000001999998,
-145.052367414711));
#146754=CARTESIAN_POINT('Ctrl Pts',(-51.870165118292,-6.23767750446664,
-158.354412070984));
#146755=CARTESIAN_POINT('Ctrl Pts',(-51.7735675289641,-5.68000001999999,
-158.300965634462));
#146756=CARTESIAN_POINT('Ctrl Pts',(-52.3196619691199,-5.68000001999999,
-158.143093167052));
#146757=CARTESIAN_POINT('Ctrl Pts',(-58.0166638356104,-6.23225639415715,
-171.449026400902));
#146758=CARTESIAN_POINT('Ctrl Pts',(-57.9641288550927,-5.68000001999999,
-171.47368839131));
#146759=CARTESIAN_POINT('Ctrl Pts',(-58.4667946194619,-5.68000001999999,
-171.237717270032));
#146760=CARTESIAN_POINT('',(-58.0166638356104,-6.23225639415715,-171.449026400902));
#146761=CARTESIAN_POINT('Origin',(-58.4667946194619,-6.18000001999999,-171.237717270032));
#146762=CARTESIAN_POINT('Ctrl Pts',(-58.0166638356104,-6.23225639415715,
-171.449026400902));
#146763=CARTESIAN_POINT('Ctrl Pts',(-51.8701651180199,-6.23767750289604,
-158.354412070834));
#146764=CARTESIAN_POINT('Ctrl Pts',(-45.7155147610371,-6.24444362877111,
-145.263691191088));
#146765=CARTESIAN_POINT('Ctrl Pts',(-39.532390596256,-6.25584930059378,
-132.186909005141));
#146766=CARTESIAN_POINT('Ctrl Pts',(-58.0166638356104,-6.23225639415715,
-171.449026400902));
#146767=CARTESIAN_POINT('Ctrl Pts',(-57.9641288550927,-5.68000002000002,
-171.47368839131));
#146768=CARTESIAN_POINT('Ctrl Pts',(-58.4667946194619,-5.68000001999999,
-171.237717270032));
#146769=CARTESIAN_POINT('Ctrl Pts',(-58.0790703543615,-6.23572556787351,
-171.581106868264));
#146770=CARTESIAN_POINT('Ctrl Pts',(-58.0192749608379,-5.68000001999239,
-171.600361788065));
#146771=CARTESIAN_POINT('Ctrl Pts',(-58.559801654985,-5.68000001999999,
-171.435840927268));
#146772=CARTESIAN_POINT('Ctrl Pts',(-58.1115942404139,-6.23752120598293,
-171.724230304954));
#146773=CARTESIAN_POINT('Ctrl Pts',(-58.0470269895722,-5.68000001999999,
-171.733866658521));
#146774=CARTESIAN_POINT('Ctrl Pts',(-58.608274529079,-5.68000001999999,
-171.650520905847));
#146775=CARTESIAN_POINT('Ctrl Pts',(-58.1115942404669,-6.2375212064409,
-171.871644662643));
#146776=CARTESIAN_POINT('Ctrl Pts',(-58.0470269915054,-5.68000001999999,
-171.871644662643));
#146777=CARTESIAN_POINT('Ctrl Pts',(-58.6082745331205,-5.68000001999999,
-171.871644662643));
#146778=CARTESIAN_POINT('Origin',(-58.6082745331205,-6.18000001999999,-171.871644662643));
#146779=CARTESIAN_POINT('Origin',(-56.6529025639176,-6.15643989082879,-171.969043985007));
#146780=CARTESIAN_POINT('Origin',(-58.6082745331205,-6.18000001999999,-179.64995));
#146781=CARTESIAN_POINT('Origin',(-58.6082745331205,-6.18000001999999,-176.427328712824));
#146782=CARTESIAN_POINT('Ctrl Pts',(-60.,-5.18000001999999,-174.511260182693));
#146783=CARTESIAN_POINT('Ctrl Pts',(-60.,-5.68000001999998,-174.511260182694));
#146784=CARTESIAN_POINT('Ctrl Pts',(-59.5,-5.68000001999999,-174.511260182693));
#146785=CARTESIAN_POINT('Ctrl Pts',(-60.,-5.17778160006748,-174.799392136338));
#146786=CARTESIAN_POINT('Ctrl Pts',(-60.0022233258349,-5.68000002000248,
-174.800030292485));
#146787=CARTESIAN_POINT('Ctrl Pts',(-59.4999999934949,-5.68000001999999,
-174.751455697725));
#146788=CARTESIAN_POINT('Ctrl Pts',(-59.9593729581191,-5.1756134281897,
-175.080714219829));
#146789=CARTESIAN_POINT('Ctrl Pts',(-59.9636195754477,-5.68000001999999,
-175.081942695907));
#146790=CARTESIAN_POINT('Ctrl Pts',(-59.4661441339012,-5.68000001999999,
-174.985974426754));
#146791=CARTESIAN_POINT('Ctrl Pts',(-59.8388406974375,-5.17243729299778,
-175.492475419334));
#146792=CARTESIAN_POINT('Ctrl Pts',(-59.8460772881358,-5.68000001999999,
-175.49508011951));
#146793=CARTESIAN_POINT('Ctrl Pts',(-59.3657005801303,-5.68000001999999,
-175.329231362388));
#146794=CARTESIAN_POINT('Ctrl Pts',(-59.7882941049042,-5.17139018325129,
-175.628164866621));
#146795=CARTESIAN_POINT('Ctrl Pts',(-59.7963955952484,-5.68000002000071,
-175.631508024916));
#146796=CARTESIAN_POINT('Ctrl Pts',(-59.3235784200839,-5.68000001999999,
-175.4423463311));
#146797=CARTESIAN_POINT('Ctrl Pts',(-59.6700340607039,-5.16938852396119,
-175.887451075324));
#146798=CARTESIAN_POINT('Ctrl Pts',(-59.6796421793893,-5.68000001999927,
-175.892503005072));
#146799=CARTESIAN_POINT('Ctrl Pts',(-59.2250283845896,-5.68000001999999,
-175.658495472519));
#146800=CARTESIAN_POINT('Ctrl Pts',(-59.6020511144931,-5.16842516963192,
-176.012189602522));
#146801=CARTESIAN_POINT('Ctrl Pts',(-59.6122794132826,-5.6800000200009,
-176.018182187565));
#146802=CARTESIAN_POINT('Ctrl Pts',(-59.1683759292615,-5.68000001999999,
-175.762481455964));
#146803=CARTESIAN_POINT('Ctrl Pts',(-59.4484275192731,-5.16657340194589,
-176.251884189743));
#146804=CARTESIAN_POINT('Ctrl Pts',(-59.4596388112852,-5.68000001999906,
-176.259950074275));
#146805=CARTESIAN_POINT('Ctrl Pts',(-59.0403562655437,-5.68000001999999,
-175.962298484052));
#146806=CARTESIAN_POINT('Ctrl Pts',(-59.3620233301153,-5.16567852041965,
-176.367676771746));
#146807=CARTESIAN_POINT('Ctrl Pts',(-59.3735776050024,-5.68000001999968,
-176.376845479805));
#146808=CARTESIAN_POINT('Ctrl Pts',(-58.9683527741555,-5.68000001999999,
-176.058826880554));
#146809=CARTESIAN_POINT('Ctrl Pts',(-59.1745444884326,-5.16400295101772,
-176.584424539694));
#146810=CARTESIAN_POINT('Ctrl Pts',(-59.1864690073094,-5.6800000200003,
-176.595885870473));
#146811=CARTESIAN_POINT('Ctrl Pts',(-58.8121204079676,-5.68000001999999,
-176.239514776908));
#146812=CARTESIAN_POINT('Ctrl Pts',(-59.0739603306682,-5.16322437006847,
-176.685107962755));
#146813=CARTESIAN_POINT('Ctrl Pts',(-59.0859070073554,-5.68000001999999,
-176.697708952909));
#146814=CARTESIAN_POINT('Ctrl Pts',(-58.7283002756348,-5.68000001999999,
-176.3234477233));
#146815=CARTESIAN_POINT('Ctrl Pts',(-58.7521818176688,-5.16106213487567,
-176.9646578323));
#146816=CARTESIAN_POINT('Ctrl Pts',(-58.7634647581383,-5.68000001999999,
-176.980908577071));
#146817=CARTESIAN_POINT('Ctrl Pts',(-58.460151514568,-5.68000001999999,
-176.556489535136));
#146818=CARTESIAN_POINT('Ctrl Pts',(-58.5075501754184,-5.15984115636875,
-177.122423932479));
#146819=CARTESIAN_POINT('Ctrl Pts',(-58.5179479000405,-5.68000002000922,
-177.140745767071));
#146820=CARTESIAN_POINT('Ctrl Pts',(-58.2562917522372,-5.68000001999999,
-176.688008530437));
#146821=CARTESIAN_POINT('Ctrl Pts',(-58.2485390147982,-5.15892282666644,
-177.241058641939));
#146822=CARTESIAN_POINT('Ctrl Pts',(-58.2576969618386,-5.68000001999996,
-177.261045698521));
#146823=CARTESIAN_POINT('Ctrl Pts',(-58.0404491789985,-5.68000001999999,
-176.786906275262));
#146824=CARTESIAN_POINT('',(-60.,-5.18000001999999,-174.511260182693));
#146825=CARTESIAN_POINT('Origin',(-59.5,-5.18000001999999,-174.511260182693));
#146826=CARTESIAN_POINT('',(-58.2670189319755,-5.15898895260712,-177.232517863302));
#146827=CARTESIAN_POINT('Ctrl Pts',(-60.,-5.18000001999999,-174.511260182693));
#146828=CARTESIAN_POINT('Ctrl Pts',(-60.,-5.17778160006748,-174.799392136338));
#146829=CARTESIAN_POINT('Ctrl Pts',(-59.9593729581191,-5.1756134281897,
-175.080714219829));
#146830=CARTESIAN_POINT('Ctrl Pts',(-59.8388406974375,-5.17243729299778,
-175.492475419334));
#146831=CARTESIAN_POINT('Ctrl Pts',(-59.7882941049042,-5.17139018325129,
-175.628164866621));
#146832=CARTESIAN_POINT('Ctrl Pts',(-59.6700340607039,-5.16938852396119,
-175.887451075324));
#146833=CARTESIAN_POINT('Ctrl Pts',(-59.6020511144931,-5.16842516963192,
-176.012189602522));
#146834=CARTESIAN_POINT('Ctrl Pts',(-59.4484275192731,-5.16657340194589,
-176.251884189743));
#146835=CARTESIAN_POINT('Ctrl Pts',(-59.3620233301153,-5.16567852041965,
-176.367676771746));
#146836=CARTESIAN_POINT('Ctrl Pts',(-59.1745444884326,-5.16400295101772,
-176.584424539694));
#146837=CARTESIAN_POINT('Ctrl Pts',(-59.0739603306682,-5.16322437006847,
-176.685107962755));
#146838=CARTESIAN_POINT('Ctrl Pts',(-58.757290323262,-5.16109646218508,
-176.960219742078));
#146839=CARTESIAN_POINT('Ctrl Pts',(-58.5191843003194,-5.15989943361415,
-177.114893703118));
#146840=CARTESIAN_POINT('Ctrl Pts',(-58.267019098174,-5.15898893607586,
-177.232518219478));
#146841=CARTESIAN_POINT('Ctrl Pts',(-58.6082745331212,-5.6800000199515,
-176.427328712824));
#146842=CARTESIAN_POINT('Ctrl Pts',(-58.5950348472832,-5.67999973335255,
-176.465341940165));
#146843=CARTESIAN_POINT('Ctrl Pts',(-58.5820378685848,-5.67873096779289,
-176.502404330564));
#146844=CARTESIAN_POINT('Ctrl Pts',(-58.5692957758333,-5.6761247427438,
-176.538599126011));
#146845=CARTESIAN_POINT('Ctrl Pts',(-58.5575251017621,-5.67371720842369,
-176.572034539534));
#146846=CARTESIAN_POINT('Ctrl Pts',(-58.5459718188596,-5.67016847694687,
-176.604730379523));
#146847=CARTESIAN_POINT('Ctrl Pts',(-58.5346113579762,-5.66540164772652,
-176.636740993982));
#146848=CARTESIAN_POINT('Ctrl Pts',(-58.5234535848567,-5.66071986593212,
-176.668180490779));
#146849=CARTESIAN_POINT('Ctrl Pts',(-58.5124820659697,-5.65486292007998,
-176.698960019499));
#146850=CARTESIAN_POINT('Ctrl Pts',(-58.5016375963336,-5.64773536444049,
-176.729106516791));
#146851=CARTESIAN_POINT('Ctrl Pts',(-58.4887024183243,-5.63923368533013,
-176.765064965835));
#146852=CARTESIAN_POINT('Ctrl Pts',(-58.4761091181577,-5.62901675142965,
-176.799703323515));
#146853=CARTESIAN_POINT('Ctrl Pts',(-58.4638764455671,-5.61705712797886,
-176.832892052454));
#146854=CARTESIAN_POINT('Ctrl Pts',(-58.4526854472824,-5.60611592731065,
-176.863254592272));
#146855=CARTESIAN_POINT('Ctrl Pts',(-58.4417961169189,-5.5937155379102,
-176.892404008976));
#146856=CARTESIAN_POINT('Ctrl Pts',(-58.4311972672537,-5.57985231740509,
-176.920211869705));
#146857=CARTESIAN_POINT('Ctrl Pts',(-58.4230739091552,-5.56922702238551,
-176.941524862887));
#146858=CARTESIAN_POINT('Ctrl Pts',(-58.4151206678837,-5.55774254710736,
-176.962049198181));
#146859=CARTESIAN_POINT('Ctrl Pts',(-58.4073220826608,-5.54540973774009,
-176.981713767982));
#146860=CARTESIAN_POINT('Ctrl Pts',(-58.3980439115344,-5.53073708718778,
-177.005109196579));
#146861=CARTESIAN_POINT('Ctrl Pts',(-58.3890004170057,-5.51486733758817,
-177.027269841537));
#146862=CARTESIAN_POINT('Ctrl Pts',(-58.380218810449,-5.49787963522563,
-177.048004584116));
#146863=CARTESIAN_POINT('Ctrl Pts',(-58.3716510587059,-5.48130562731634,
-177.06823438213));
#146864=CARTESIAN_POINT('Ctrl Pts',(-58.3633324493104,-5.46366723978173,
-177.08710603058));
#146865=CARTESIAN_POINT('Ctrl Pts',(-58.3552874425923,-5.44508712768701,
-177.104443177883));
#146866=CARTESIAN_POINT('Ctrl Pts',(-58.3474557388646,-5.42699964333175,
-177.121320653057));
#146867=CARTESIAN_POINT('Ctrl Pts',(-58.3398831703244,-5.40801984922685,
-177.136743017005));
#146868=CARTESIAN_POINT('Ctrl Pts',(-58.3325937137739,-5.38830856612735,
-177.150561531819));
#146869=CARTESIAN_POINT('Ctrl Pts',(-58.3309779449681,-5.38393939592455,
-177.153624520812));
#146870=CARTESIAN_POINT('Ctrl Pts',(-58.3293760968208,-5.37953446911859,
-177.156608794961));
#146871=CARTESIAN_POINT('Ctrl Pts',(-58.3277884517205,-5.37509584628772,
-177.159512900979));
#146872=CARTESIAN_POINT('Ctrl Pts',(-58.3210194032167,-5.35617143224425,
-177.171894783105));
#146873=CARTESIAN_POINT('Ctrl Pts',(-58.3144830662044,-5.33655034723311,
-177.182868588345));
#146874=CARTESIAN_POINT('Ctrl Pts',(-58.3082161502908,-5.31639591374794,
-177.192297826593));
#146875=CARTESIAN_POINT('Ctrl Pts',(-58.30204887787,-5.29656193424289,-177.201577140661));
#146876=CARTESIAN_POINT('Ctrl Pts',(-58.2961423730487,-5.27621189722801,
-177.209359719377));
#146877=CARTESIAN_POINT('Ctrl Pts',(-58.2905359191037,-5.25554184478381,
-177.215544429679));
#146878=CARTESIAN_POINT('Ctrl Pts',(-58.2850147109265,-5.23518607914303,
-177.221635101863));
#146879=CARTESIAN_POINT('Ctrl Pts',(-58.279784399567,-5.21452076912564,
-177.226175439045));
#146880=CARTESIAN_POINT('Ctrl Pts',(-58.2748885905143,-5.19376312460734,
-177.229108942955));
#146881=CARTESIAN_POINT('Ctrl Pts',(-58.2721582012751,-5.18218660097016,
-177.230744956007));
#146882=CARTESIAN_POINT('Ctrl Pts',(-58.2695319717949,-5.17058183724987,
-177.231881985786));
#146883=CARTESIAN_POINT('Ctrl Pts',(-58.2670184333942,-5.15898900219905,
-177.232516794804));
#146884=CARTESIAN_POINT('Origin',(-59.5,-5.18000001999999,-55.24995));
#146885=CARTESIAN_POINT('',(-60.,-5.18000001999999,-174.534521368494));
#146886=CARTESIAN_POINT('Origin',(-60.,-2.55003103885676E-14,0.));
#146887=CARTESIAN_POINT('',(-60.,-4.68000001999999,-174.488343624884));
#146888=CARTESIAN_POINT('',(-60.,-4.68000001999999,-58.1637190207452));
#146889=CARTESIAN_POINT('Ctrl Pts',(-60.,-5.18000001999999,-174.511260182694));
#146890=CARTESIAN_POINT('Ctrl Pts',(-60.,-5.01333573888012,-174.503547232447));
#146891=CARTESIAN_POINT('Ctrl Pts',(-60.,-4.84666961885575,-174.495891400547));
#146892=CARTESIAN_POINT('Ctrl Pts',(-60.,-4.68000001999999,-174.488343624884));
#146893=CARTESIAN_POINT('Origin',(-59.5,-4.68000001999999,-55.24995));
#146894=CARTESIAN_POINT('Origin',(-59.5,-4.68000001999999,-174.488343624884));
#146895=CARTESIAN_POINT('Ctrl Pts',(-39.585730865631,-3.7824242910708,-98.7152302188737));
#146896=CARTESIAN_POINT('Ctrl Pts',(-39.6607823401664,-4.18000001999998,
-98.7511570311542));
#146897=CARTESIAN_POINT('Ctrl Pts',(-40.0271577790679,-4.18000001999998,
-98.926539349744));
#146898=CARTESIAN_POINT('Ctrl Pts',(-45.6152479999264,-3.76777550625849,
-86.1124074338642));
#146899=CARTESIAN_POINT('Ctrl Pts',(-45.7555532717617,-4.18000001999998,
-85.989998533184));
#146900=CARTESIAN_POINT('Ctrl Pts',(-46.0600623067188,-4.18000001999998,
-86.3237407210712));
#146901=CARTESIAN_POINT('Ctrl Pts',(-51.5953561718106,-3.75882512748543,
-73.4851842533606));
#146902=CARTESIAN_POINT('Ctrl Pts',(-51.6938180895878,-4.18000002,-73.4342549076826));
#146903=CARTESIAN_POINT('Ctrl Pts',(-52.0416537250564,-4.18000001999999,
-73.6965087765536));
#146904=CARTESIAN_POINT('Ctrl Pts',(-57.5607154366947,-3.75164060643487,
-60.8508735991007));
#146905=CARTESIAN_POINT('Ctrl Pts',(-57.6167925372613,-4.18000001999999,
-60.8773558160983));
#146906=CARTESIAN_POINT('Ctrl Pts',(-58.0081705490647,-4.18000001999999,
-61.0621827299711));
#146907=CARTESIAN_POINT('Origin',(-40.0271577790679,-3.68000001999999,-98.926539349744));
#146908=CARTESIAN_POINT('Ctrl Pts',(-59.5,-4.18000001999999,-174.488343624884));
#146909=CARTESIAN_POINT('Ctrl Pts',(-60.,-4.18000002,-174.488343624884));
#146910=CARTESIAN_POINT('Ctrl Pts',(-60.,-4.68000001999999,-174.488343624884));
#146911=CARTESIAN_POINT('Ctrl Pts',(-59.499999993334,-4.18000001999999,
-174.734541991424));
#146912=CARTESIAN_POINT('Ctrl Pts',(-59.9977796185047,-4.18000001999829,
-174.78302738694));
#146913=CARTESIAN_POINT('Ctrl Pts',(-60.,-4.67777472283721,-174.78368089075));
#146914=CARTESIAN_POINT('Ctrl Pts',(-59.4644630183961,-4.18000001999999,
-174.974786360247));
#146915=CARTESIAN_POINT('Ctrl Pts',(-59.9531694408477,-4.18000002000085,
-175.070632089297));
#146916=CARTESIAN_POINT('Ctrl Pts',(-59.9573556192874,-4.67559899657361,
-175.071875505894));
#146917=CARTESIAN_POINT('Ctrl Pts',(-59.3588972809293,-4.18000001999999,
-175.326182058073));
#146918=CARTESIAN_POINT('Ctrl Pts',(-59.8236519200077,-4.18000001999958,
-175.490806712526));
#146919=CARTESIAN_POINT('Ctrl Pts',(-59.8306767385091,-4.67241126250759,
-175.493405719049));
#146920=CARTESIAN_POINT('Ctrl Pts',(-59.3147195516479,-4.18000001999999,
-175.441607525732));
#146921=CARTESIAN_POINT('Ctrl Pts',(-59.7698424718428,-4.18000001999956,
-175.628550598836));
#146922=CARTESIAN_POINT('Ctrl Pts',(-59.7776634626824,-4.67136322522169,
-175.631868709625));
#146923=CARTESIAN_POINT('Ctrl Pts',(-59.2114199113778,-4.18000001999999,
-175.661895244315));
#146924=CARTESIAN_POINT('Ctrl Pts',(-59.6445293525488,-4.18000002000041,
-175.891155901683));
#146925=CARTESIAN_POINT('Ctrl Pts',(-59.6537038929485,-4.66936150715186,
-175.896123076728));
#146926=CARTESIAN_POINT('Ctrl Pts',(-59.1520385607459,-4.18000001999999,
-175.767754281813));
#146927=CARTESIAN_POINT('Ctrl Pts',(-59.5727342923808,-4.18000002000089,
-176.017245435328));
#146928=CARTESIAN_POINT('Ctrl Pts',(-59.5824462721252,-4.66839878682381,
-176.023110187492));
#146929=CARTESIAN_POINT('Ctrl Pts',(-59.0177715691528,-4.18000001999999,
-175.970879863896));
#146930=CARTESIAN_POINT('Ctrl Pts',(-59.4108028292072,-4.1800000199991,
-176.258951716569));
#146931=CARTESIAN_POINT('Ctrl Pts',(-59.4213258837533,-4.66655021592386,
-176.266776880891));
#146932=CARTESIAN_POINT('Ctrl Pts',(-58.9421612688066,-4.18000001999999,
-176.06886452411));
#146933=CARTESIAN_POINT('Ctrl Pts',(-59.3198146755637,-4.18000001999915,
-176.37546218739));
#146934=CARTESIAN_POINT('Ctrl Pts',(-59.3305935235461,-4.66565781609966,
-176.3843179035));
#146935=CARTESIAN_POINT('Ctrl Pts',(-58.7790852805764,-4.18000001999999,
-176.250769420981));
#146936=CARTESIAN_POINT('Ctrl Pts',(-59.1239216856836,-4.18000002000084,
-176.591561815318));
#146937=CARTESIAN_POINT('Ctrl Pts',(-59.1349023357136,-4.66400011582949,
-176.602528392516));
#146938=CARTESIAN_POINT('Ctrl Pts',(-58.6915944853457,-4.18000001999999,
-176.33503132506));
#146939=CARTESIAN_POINT('Ctrl Pts',(-59.0189867750955,-4.18000001999871,
-176.691604703902));
#146940=CARTESIAN_POINT('Ctrl Pts',(-59.0299133821615,-4.66323171680632,
-176.703607721972));
#146941=CARTESIAN_POINT('Ctrl Pts',(-58.4115655020993,-4.18000001999999,
-176.56808461344));
#146942=CARTESIAN_POINT('Ctrl Pts',(-58.6838036746477,-4.18000002000249,
-176.967887143763));
#146943=CARTESIAN_POINT('Ctrl Pts',(-58.6938786030259,-4.66110543474911,
-176.983174915482));
#146944=CARTESIAN_POINT('Ctrl Pts',(-58.1982641486948,-4.18000001999999,
-176.698056997615));
#146945=CARTESIAN_POINT('Ctrl Pts',(-58.4288067817606,-4.18000002000125,
-177.121996578829));
#146946=CARTESIAN_POINT('Ctrl Pts',(-58.437917085704,-4.65991812350376,
-177.139087667033));
#146947=CARTESIAN_POINT('Ctrl Pts',(-57.9753315069797,-4.18000001999999,
-176.792613205276));
#146948=CARTESIAN_POINT('Ctrl Pts',(-58.1625546348518,-4.18000002,-177.234024164027));
#146949=CARTESIAN_POINT('Ctrl Pts',(-58.1703978083756,-4.65905396057624,
-177.252515804372));
#146950=CARTESIAN_POINT('',(-58.2078173720072,-4.65917712473139,-177.236349008097));
#146951=CARTESIAN_POINT('Ctrl Pts',(-58.2078173720829,-4.65917712520045,
-177.236349008084));
#146952=CARTESIAN_POINT('Ctrl Pts',(-58.4617634457135,-4.66002956379037,
-177.124453281026));
#146953=CARTESIAN_POINT('Ctrl Pts',(-58.7043445390845,-4.66117165864448,
-176.974467684704));
#146954=CARTESIAN_POINT('Ctrl Pts',(-59.0299133821615,-4.66323171680632,
-176.703607721972));
#146955=CARTESIAN_POINT('Ctrl Pts',(-59.1349023357136,-4.66400011582949,
-176.602528392516));
#146956=CARTESIAN_POINT('Ctrl Pts',(-59.3305935235461,-4.66565781609966,
-176.3843179035));
#146957=CARTESIAN_POINT('Ctrl Pts',(-59.4213258837533,-4.66655021592386,
-176.266776880891));
#146958=CARTESIAN_POINT('Ctrl Pts',(-59.5824462721252,-4.66839878682381,
-176.023110187492));
#146959=CARTESIAN_POINT('Ctrl Pts',(-59.6537038929485,-4.66936150715186,
-175.896123076728));
#146960=CARTESIAN_POINT('Ctrl Pts',(-59.7776634626824,-4.67136322522169,
-175.631868709625));
#146961=CARTESIAN_POINT('Ctrl Pts',(-59.8306767385091,-4.67241126250759,
-175.493405719049));
#146962=CARTESIAN_POINT('Ctrl Pts',(-59.9573556192874,-4.67559899657361,
-175.071875505894));
#146963=CARTESIAN_POINT('Ctrl Pts',(-60.,-4.67777472283721,-174.78368089075));
#146964=CARTESIAN_POINT('Ctrl Pts',(-60.,-4.68000001999999,-174.488343624884));
#146965=CARTESIAN_POINT('Ctrl Pts',(-58.2078173720829,-4.65917712520045,
-177.236349008084));
#146966=CARTESIAN_POINT('Ctrl Pts',(-58.1766173277935,-4.52496538336098,
-177.243973427637));
#146967=CARTESIAN_POINT('Ctrl Pts',(-58.1596733704946,-4.39698767568444,
-177.184652644663));
#146968=CARTESIAN_POINT('Ctrl Pts',(-58.1740867503666,-4.22134717274183,
-176.965019674666));
#146969=CARTESIAN_POINT('Ctrl Pts',(-58.2063099446428,-4.18000001999999,
-176.814456128226));
#146970=CARTESIAN_POINT('Ctrl Pts',(-58.2644174754153,-4.18000001999999,
-176.647241333324));
#146971=CARTESIAN_POINT('Origin',(-58.2644174754153,-3.68000001999999,-179.64995));
#146972=CARTESIAN_POINT('Origin',(-58.2644174754153,-3.68000001999999,-176.647241333324));
#146973=CARTESIAN_POINT('Origin',(-58.2644174754153,-3.68000001999999,-171.871644662643));
#146974=CARTESIAN_POINT('Ctrl Pts',(-57.7706512256236,-3.75870764711888,
-171.871644662643));
#146975=CARTESIAN_POINT('Ctrl Pts',(-57.8378063278745,-4.18000001999999,
-171.871644662643));
#146976=CARTESIAN_POINT('Ctrl Pts',(-58.2644174754153,-4.18000001999999,
-171.871644662643));
#146977=CARTESIAN_POINT('Ctrl Pts',(-57.7706512252069,-3.75870764450445,
-171.725685252419));
#146978=CARTESIAN_POINT('Ctrl Pts',(-57.8378063150439,-4.18000001999999,
-171.715730578987));
#146979=CARTESIAN_POINT('Ctrl Pts',(-58.2644174584531,-4.18000001999999,
-171.652701076652));
#146980=CARTESIAN_POINT('Ctrl Pts',(-57.7383541282856,-3.7562957918519,
-171.582363368286));
#146981=CARTESIAN_POINT('Ctrl Pts',(-57.801183875227,-4.18000002000114,
-171.562158552623));
#146982=CARTESIAN_POINT('Ctrl Pts',(-58.2165506240601,-4.18000001999999,
-171.437728673605));
#146983=CARTESIAN_POINT('Ctrl Pts',(-57.6746235421417,-3.75150367745622,
-171.449026400902));
#146984=CARTESIAN_POINT('Ctrl Pts',(-57.7306096110337,-4.18000001999999,
-171.422588467367));
#146985=CARTESIAN_POINT('Ctrl Pts',(-58.1221005562789,-4.18000001999999,
-171.237717270032));
#146986=CARTESIAN_POINT('',(-57.6746235421417,-3.75150367745622,-171.449026400902));
#146987=CARTESIAN_POINT('Origin',(-58.1221005562789,-3.68000001999999,-171.237717270032));
#146988=CARTESIAN_POINT('Origin',(-56.7293330762435,-3.67954981718445,-171.875507808352));
#146989=CARTESIAN_POINT('Ctrl Pts',(-57.6746235421417,-3.75150367745622,
-171.449026400902));
#146990=CARTESIAN_POINT('Ctrl Pts',(-57.7306096110337,-4.18000001999999,
-171.422588467367));
#146991=CARTESIAN_POINT('Ctrl Pts',(-58.1221005562789,-4.18000001999999,
-171.237717270032));
#146992=CARTESIAN_POINT('Ctrl Pts',(-51.6715280616305,-3.75870638021677,
-158.734184170827));
#146993=CARTESIAN_POINT('Ctrl Pts',(-51.7702631771107,-4.18000001999999,
-158.785894332693));
#146994=CARTESIAN_POINT('Ctrl Pts',(-52.1178467328245,-4.18000001999999,
-158.52285936551));
#146995=CARTESIAN_POINT('Ctrl Pts',(-45.6536266465224,-3.76768226491552,
-146.026454114168));
#146996=CARTESIAN_POINT('Ctrl Pts',(-45.7948164697718,-4.18000001999998,
-146.15085325192));
#146997=CARTESIAN_POINT('Ctrl Pts',(-46.0984623496487,-4.18000001999998,
-145.815120328436));
#146998=CARTESIAN_POINT('Ctrl Pts',(-39.5857308656265,-3.78242429107081,
-133.343412752623));
#146999=CARTESIAN_POINT('Ctrl Pts',(-39.660782340162,-4.18000001999998,
-133.307485940342));
#147000=CARTESIAN_POINT('Ctrl Pts',(-40.0271577790634,-4.18000001999998,
-133.132103621752));
#147001=CARTESIAN_POINT('',(-39.5857307322485,-3.78242358451346,-133.343412816471));
#147002=CARTESIAN_POINT('Origin',(-40.0271577790634,-3.68000001999999,-133.132103621752));
#147003=CARTESIAN_POINT('Ctrl Pts',(-39.5857308656309,-3.78242429107441,
-133.34341275263));
#147004=CARTESIAN_POINT('Ctrl Pts',(-45.6536266516538,-3.7676822799009,
-146.026454118689));
#147005=CARTESIAN_POINT('Ctrl Pts',(-51.6715280651912,-3.75870639540982,
-158.734184172691));
#147006=CARTESIAN_POINT('Ctrl Pts',(-57.6746235421417,-3.75150367745622,
-171.449026400902));
#147007=CARTESIAN_POINT('Ctrl Pts',(-39.5000746910952,-4.18000001999998,
-130.774156597103));
#147008=CARTESIAN_POINT('Ctrl Pts',(-38.9988856571825,-4.18000001999998,
-130.771495097562));
#147009=CARTESIAN_POINT('Ctrl Pts',(-39.0000830375701,-3.67880541495414,
-130.771501481495));
#147010=CARTESIAN_POINT('Ctrl Pts',(-39.4979098764889,-4.18000001999998,
-131.188377903755));
#147011=CARTESIAN_POINT('Ctrl Pts',(-39.0133259194552,-4.18000001999998,
-131.216802997827));
#147012=CARTESIAN_POINT('Ctrl Pts',(-38.9976770037577,-3.69581922809734,
-131.224220780693));
#147013=CARTESIAN_POINT('Ctrl Pts',(-39.5428199578347,-4.18000001999998,
-131.594670912653));
#147014=CARTESIAN_POINT('Ctrl Pts',(-39.0772732138211,-4.18000001999999,
-131.657324358274));
#147015=CARTESIAN_POINT('Ctrl Pts',(-39.0475765097186,-3.71311681177937,
-131.667826133903));
#147016=CARTESIAN_POINT('Ctrl Pts',(-39.7223936198539,-4.18000001999998,
-132.391873207535));
#147017=CARTESIAN_POINT('Ctrl Pts',(-39.3031001496673,-4.18000001999998,
-132.514074181288));
#147018=CARTESIAN_POINT('Ctrl Pts',(-39.247101643641,-3.74820970445091,
-132.537336227375));
#147019=CARTESIAN_POINT('Ctrl Pts',(-39.8587693570671,-4.18000001999998,
-132.785389893012));
#147020=CARTESIAN_POINT('Ctrl Pts',(-39.4640070783496,-4.18000001999999,
-132.934381121693));
#147021=CARTESIAN_POINT('Ctrl Pts',(-39.3986305924887,-3.76613472203319,
-132.966073941729));
#147022=CARTESIAN_POINT('Ctrl Pts',(-40.0395629979198,-4.18000001999998,
-133.157837806796));
#147023=CARTESIAN_POINT('Ctrl Pts',(-39.6750481329511,-4.18000001999998,
-133.334759037945));
#147024=CARTESIAN_POINT('Ctrl Pts',(-39.5995110806651,-3.78361375906165,
-133.371422516669));
#147025=CARTESIAN_POINT('',(-39.,-3.68000001999998,-130.802732351058));
#147026=CARTESIAN_POINT('Origin',(-39.5,-3.68000001999999,-130.802732351058));
#147027=CARTESIAN_POINT('Ctrl Pts',(-39.,-3.68000001999998,-130.802732351058));
#147028=CARTESIAN_POINT('Ctrl Pts',(-39.0000000012333,-3.68447440683702,
-130.921592018194));
#147029=CARTESIAN_POINT('Ctrl Pts',(-39.0036588240764,-3.68897484526234,
-131.039838409487));
#147030=CARTESIAN_POINT('Ctrl Pts',(-39.0108684419194,-3.69349116787911,
-131.157453391765));
#147031=CARTESIAN_POINT('Ctrl Pts',(-39.018143549427,-3.698048515202,-131.276136747693));
#147032=CARTESIAN_POINT('Ctrl Pts',(-39.0290338743149,-3.70262240489881,
-131.394178091007));
#147033=CARTESIAN_POINT('Ctrl Pts',(-39.0434756876213,-3.70721214335521,
-131.51158216155));
#147034=CARTESIAN_POINT('Ctrl Pts',(-39.0580054854929,-3.71182984409958,
-131.629701498652));
#147035=CARTESIAN_POINT('Ctrl Pts',(-39.0761300225471,-3.71646401900972,
-131.747176766763));
#147036=CARTESIAN_POINT('Ctrl Pts',(-39.0978360495535,-3.72111772532618,
-131.864021839488));
#147037=CARTESIAN_POINT('Ctrl Pts',(-39.1126626346933,-3.72429650018426,
-131.943834391939));
#147038=CARTESIAN_POINT('Ctrl Pts',(-39.1291613559977,-3.72748446873514,
-132.023353094883));
#147039=CARTESIAN_POINT('Ctrl Pts',(-39.1473419267964,-3.73068197101817,
-132.102581139799));
#147040=CARTESIAN_POINT('Ctrl Pts',(-39.1767331515572,-3.73585114360985,
-132.230663437175));
#147041=CARTESIAN_POINT('Ctrl Pts',(-39.2105770847552,-3.74103515521041,
-132.358219146246));
#147042=CARTESIAN_POINT('Ctrl Pts',(-39.2488673046334,-3.74623841689841,
-132.484810818648));
#147043=CARTESIAN_POINT('Ctrl Pts',(-39.2868385612724,-3.75139833464094,
-132.610347963549));
#147044=CARTESIAN_POINT('Ctrl Pts',(-39.3291826030354,-3.75657694721291,
-132.734936713211));
#147045=CARTESIAN_POINT('Ctrl Pts',(-39.3758480040126,-3.76175604867458,
-132.858142986391));
#147046=CARTESIAN_POINT('Ctrl Pts',(-39.4220236042586,-3.76688079021157,
-132.980056084726));
#147047=CARTESIAN_POINT('Ctrl Pts',(-39.4724305009679,-3.77200571552313,
-133.100615173967));
#147048=CARTESIAN_POINT('Ctrl Pts',(-39.5269712029935,-3.77709501234611,
-133.219397957436));
#147049=CARTESIAN_POINT('Ctrl Pts',(-39.5460539232582,-3.77887565733251,
-133.260957720053));
#147050=CARTESIAN_POINT('Ctrl Pts',(-39.565642246535,-3.78065179793913,
-133.302300046887));
#147051=CARTESIAN_POINT('Ctrl Pts',(-39.5857305461208,-3.78242147649458,
-133.343406945925));
#147052=CARTESIAN_POINT('Origin',(-39.5,-3.68000001999999,-55.24995));
#147053=CARTESIAN_POINT('',(-39.,-3.68000001999999,-101.255910620448));
#147054=CARTESIAN_POINT('Origin',(-39.5,-3.68000001999999,-101.255910620448));
#147055=CARTESIAN_POINT('',(-39.,-3.68000001999999,-129.34995));
#147056=CARTESIAN_POINT('Ctrl Pts',(-40.0271577790679,-4.18000001999998,
-98.926539349744));
#147057=CARTESIAN_POINT('Ctrl Pts',(-39.6607823401664,-4.18000001999998,
-98.7511570311542));
#147058=CARTESIAN_POINT('Ctrl Pts',(-39.585730865631,-3.7824242910708,-98.7152302188737));
#147059=CARTESIAN_POINT('Ctrl Pts',(-39.8525718691684,-4.18000001999998,
-99.2912510907428));
#147060=CARTESIAN_POINT('Ctrl Pts',(-39.4568105653931,-4.18000001999998,
-99.1432082613171));
#147061=CARTESIAN_POINT('Ctrl Pts',(-39.3917487041449,-3.76533335821317,
-99.1121767214752));
#147062=CARTESIAN_POINT('Ctrl Pts',(-39.7225112880865,-4.18000001999998,
-99.6687555669174));
#147063=CARTESIAN_POINT('Ctrl Pts',(-39.3032261512475,-4.18000001999998,
-99.546440425348));
#147064=CARTESIAN_POINT('Ctrl Pts',(-39.247234764848,-3.74814762956703,
-99.5234791492765));
#147065=CARTESIAN_POINT('Ctrl Pts',(-39.5459737882558,-4.18000001999998,
-100.447508896771));
#147066=CARTESIAN_POINT('Ctrl Pts',(-39.0814385609748,-4.18000001999998,
-100.383271856169));
#147067=CARTESIAN_POINT('Ctrl Pts',(-39.0510819866434,-3.71385382853417,
-100.372855479779));
#147068=CARTESIAN_POINT('Ctrl Pts',(-39.5000000005413,-4.18000001999998,
-100.851700064103));
#147069=CARTESIAN_POINT('Ctrl Pts',(-39.0163583103527,-4.18000001999998,
-100.821360983603));
#147070=CARTESIAN_POINT('Ctrl Pts',(-39.,-3.69662981211624,-100.814149183564));
#147071=CARTESIAN_POINT('Ctrl Pts',(-39.5,-4.18000001999998,-101.255910620448));
#147072=CARTESIAN_POINT('Ctrl Pts',(-39.,-4.18000001999998,-101.255910620448));
#147073=CARTESIAN_POINT('Ctrl Pts',(-39.,-3.68000001999999,-101.255910620448));
#147074=CARTESIAN_POINT('Ctrl Pts',(-39.585730865631,-3.78242429107081,
-98.7152302188737));
#147075=CARTESIAN_POINT('Ctrl Pts',(-39.3917487041449,-3.76533335821317,
-99.1121767214752));
#147076=CARTESIAN_POINT('Ctrl Pts',(-39.247234764848,-3.74814762956703,
-99.5234791492765));
#147077=CARTESIAN_POINT('Ctrl Pts',(-39.0510819866434,-3.71385382853417,
-100.372855479779));
#147078=CARTESIAN_POINT('Ctrl Pts',(-39.,-3.69662981211624,-100.814149183564));
#147079=CARTESIAN_POINT('Ctrl Pts',(-39.,-3.68000001999999,-101.255910620448));
#147080=CARTESIAN_POINT('Ctrl Pts',(-39.7537575098556,1.84791950156463,
-94.88221628274));
#147081=CARTESIAN_POINT('Ctrl Pts',(-39.,2.57466119081605,-95.8526318986117));
#147082=CARTESIAN_POINT('Ctrl Pts',(-39.,3.43040799630139,-96.9953075914435));
#147083=CARTESIAN_POINT('Ctrl Pts',(-39.7190124561908,0.840911054897691,
-95.7061821932407));
#147084=CARTESIAN_POINT('Ctrl Pts',(-38.999999999981,1.53000629023279,-96.6793461871002));
#147085=CARTESIAN_POINT('Ctrl Pts',(-39.,2.33014533501219,-97.8192913905431));
#147086=CARTESIAN_POINT('Ctrl Pts',(-39.6851659166312,-0.199330185460902,
-96.4883583800562));
#147087=CARTESIAN_POINT('Ctrl Pts',(-39.,0.446335000557117,-97.4659519416263));
#147088=CARTESIAN_POINT('Ctrl Pts',(-39.,1.18987438490308,-98.6014496888564));
#147089=CARTESIAN_POINT('Ctrl Pts',(-39.6371406048982,-1.82970860306462,
-97.5751506494424));
#147090=CARTESIAN_POINT('Ctrl Pts',(-39.,-1.25780287903679,-98.559490287645));
#147091=CARTESIAN_POINT('Ctrl Pts',(-39.,-0.603530653465397,-99.6882419580977));
#147092=CARTESIAN_POINT('Ctrl Pts',(-39.6215565252267,-2.38668519024414,
-97.9237506811802));
#147093=CARTESIAN_POINT('Ctrl Pts',(-39.0000000000024,-1.8401867654384,
-98.9100191480635));
#147094=CARTESIAN_POINT('Ctrl Pts',(-39.,-1.21720470538169,-100.036841989918));
#147095=CARTESIAN_POINT('Ctrl Pts',(-39.5921016697827,-3.5111206545489,
-98.5763198411428));
#147096=CARTESIAN_POINT('Ctrl Pts',(-38.9999999999976,-3.01722910704029,
-99.5661158351118));
#147097=CARTESIAN_POINT('Ctrl Pts',(-39.,-2.45808495944723,-100.689411149812));
#147098=CARTESIAN_POINT('Ctrl Pts',(-39.5781805091624,-4.08013436254483,
-98.8814533069127));
#147099=CARTESIAN_POINT('Ctrl Pts',(-38.9999999999927,-3.61357659227868,
-99.872970636237));
#147100=CARTESIAN_POINT('Ctrl Pts',(-39.,-3.08699664896505,-100.99454469153));
#147101=CARTESIAN_POINT('Ctrl Pts',(-39.5652360655961,-4.65691592725724,
-99.1628818945567));
#147102=CARTESIAN_POINT('Ctrl Pts',(-39.,-4.21906349874734,-100.156129970618));
#147103=CARTESIAN_POINT('Ctrl Pts',(-39.,-3.72540427022208,-101.27597320326));
#147104=CARTESIAN_POINT('',(-39.0000000006157,1.96999998000003,-98.0457798926543));
#147105=CARTESIAN_POINT('Ctrl Pts',(-39.0000000024628,1.96999998000006,
-98.0457798926544));
#147106=CARTESIAN_POINT('Ctrl Pts',(-39.0000000032442,1.50691588072647,
-98.365026252185));
#147107=CARTESIAN_POINT('Ctrl Pts',(-39.0000000016551,1.03814546726177,
-98.6748799793953));
#147108=CARTESIAN_POINT('Ctrl Pts',(-39.0000000008071,0.562698589434805,
-98.9745405549415));
#147109=CARTESIAN_POINT('Ctrl Pts',(-39.0000000004711,0.374284444265228,
-99.0932926044673));
#147110=CARTESIAN_POINT('Ctrl Pts',(-39.0000000002453,0.184822272632785,
-99.2104442275566));
#147111=CARTESIAN_POINT('Ctrl Pts',(-39.0000000001311,-0.00574774121677549,
-99.3259468990427));
#147112=CARTESIAN_POINT('Ctrl Pts',(-38.9999999999777,-0.26189475793881,
-99.4811951677863));
#147113=CARTESIAN_POINT('Ctrl Pts',(-39.,-0.520415976845914,-99.6335997492721));
#147114=CARTESIAN_POINT('Ctrl Pts',(-39.,-0.780592906922155,-99.7825242060483));
#147115=CARTESIAN_POINT('Ctrl Pts',(-39.,-1.12946683952906,-99.9822185482085));
#147116=CARTESIAN_POINT('Ctrl Pts',(-39.,-1.48228932648713,-100.176247523887));
#147117=CARTESIAN_POINT('Ctrl Pts',(-39.,-1.83764512720227,-100.363126009317));
#147118=CARTESIAN_POINT('Ctrl Pts',(-39.0000000000001,-2.17904755464651,
-100.542666538653));
#147119=CARTESIAN_POINT('Ctrl Pts',(-39.0000000000001,-2.52330369642182,
-100.715959269877));
#147120=CARTESIAN_POINT('Ctrl Pts',(-39.0000000000001,-2.87085998622629,
-100.882657599431));
#147121=CARTESIAN_POINT('Ctrl Pts',(-39.0000000000001,-3.13854475842017,
-101.011047174533));
#147122=CARTESIAN_POINT('Ctrl Pts',(-39.,-3.40818747901881,-101.135524193408));
#147123=CARTESIAN_POINT('Ctrl Pts',(-39.,-3.68000001999998,-101.255910620448));
#147124=CARTESIAN_POINT('Ctrl Pts',(-39.,1.96999998000002,-98.0457798926543));
#147125=CARTESIAN_POINT('Ctrl Pts',(-38.9999999999933,1.94361525900156,
-97.4993505936098));
#147126=CARTESIAN_POINT('Ctrl Pts',(-39.0635968999836,1.91714776127833,
-96.9640681661433));
#147127=CARTESIAN_POINT('Ctrl Pts',(-39.3128539180174,1.86422808137617,
-95.9152577284781));
#147128=CARTESIAN_POINT('Ctrl Pts',(-39.5010226635731,1.83757264806834,
-95.3979932721565));
#147129=CARTESIAN_POINT('Ctrl Pts',(-39.7525219240432,1.8120830678168,-94.9115092131337));
#147130=CARTESIAN_POINT('Ctrl Pts',(-56.377904566775,1.85477723331148,-60.8508735991007));
#147131=CARTESIAN_POINT('Ctrl Pts',(-56.246666128119,2.46999998000001,-60.7875964218516));
#147132=CARTESIAN_POINT('Ctrl Pts',(-56.8161649572467,2.46999998000001,
-61.0621827299711));
#147133=CARTESIAN_POINT('Ctrl Pts',(-53.635317996248,1.84957228639176,-66.5419044818116));
#147134=CARTESIAN_POINT('Ctrl Pts',(-53.4780298924679,2.46999998009932,
-66.5137036410044));
#147135=CARTESIAN_POINT('Ctrl Pts',(-54.072208955501,2.46999998000001,-66.753215691109));
#147136=CARTESIAN_POINT('Ctrl Pts',(-50.8828928487864,1.84368306851814,
-72.2280037103763));
#147137=CARTESIAN_POINT('Ctrl Pts',(-50.7098482191461,2.46999998,-72.2098982919583));
#147138=CARTESIAN_POINT('Ctrl Pts',(-51.318146010607,2.46999998000001,-72.4393128412535));
#147139=CARTESIAN_POINT('Ctrl Pts',(-45.3466144966389,1.82978958392005,
-83.5843555039948));
#147140=CARTESIAN_POINT('Ctrl Pts',(-45.1522541442582,2.46999998,-83.5563536764924));
#147141=CARTESIAN_POINT('Ctrl Pts',(-45.7775928276463,2.46999998000002,
-83.7956646348582));
#147142=CARTESIAN_POINT('Ctrl Pts',(-42.5630938966436,1.8218009521478,-89.2547782578028));
#147143=CARTESIAN_POINT('Ctrl Pts',(-42.3434811549778,2.46999997991896,
-89.2449404232873));
#147144=CARTESIAN_POINT('Ctrl Pts',(-42.9914518100362,2.46999998000002,
-89.4660932271532));
#147145=CARTESIAN_POINT('Ctrl Pts',(-39.7525219240432,1.81208306781681,
-94.9115092131337));
#147146=CARTESIAN_POINT('Ctrl Pts',(-39.5564442323333,2.46999998000002,
-94.8139619018177));
#147147=CARTESIAN_POINT('Ctrl Pts',(-40.1772697316389,2.46999998000002,
-95.1228183440041));
#147148=CARTESIAN_POINT('Origin',(-40.1772697316389,1.96999998000002,-95.1228183440041));
#147149=CARTESIAN_POINT('Ctrl Pts',(-39.5,2.46999998000002,-98.0457798926543));
#147150=CARTESIAN_POINT('Ctrl Pts',(-39.,2.46999998000002,-98.0457798926543));
#147151=CARTESIAN_POINT('Ctrl Pts',(-39.,1.96999998000002,-98.0457798926543));
#147152=CARTESIAN_POINT('Ctrl Pts',(-39.5000000026568,2.46999998000002,
-97.5376233160284));
#147153=CARTESIAN_POINT('Ctrl Pts',(-38.9728980858888,2.46999998000002,
-97.4844974242186));
#147154=CARTESIAN_POINT('Ctrl Pts',(-39.,1.9436152588707,-97.4993505936135));
#147155=CARTESIAN_POINT('Ctrl Pts',(-39.5572372093883,2.46999998000002,
-97.0390962063516));
#147156=CARTESIAN_POINT('Ctrl Pts',(-39.0092761144151,2.46999998000002,
-96.9417291681898));
#147157=CARTESIAN_POINT('Ctrl Pts',(-39.0635968999967,1.91714776114478,
-96.9640681661487));
#147158=CARTESIAN_POINT('Ctrl Pts',(-39.7815685268491,2.46999998000002,
-96.0609362825129));
#147159=CARTESIAN_POINT('Ctrl Pts',(-39.1914722350304,2.46999998000002,
-95.8620324116114));
#147160=CARTESIAN_POINT('Ctrl Pts',(-39.312853918045,1.86422808123875,-95.9152577284902));
#147161=CARTESIAN_POINT('Ctrl Pts',(-39.9509186646822,2.46999998000002,
-95.5778016189611));
#147162=CARTESIAN_POINT('Ctrl Pts',(-39.3474064560568,2.46999997999991,
-95.3191244694837));
#147163=CARTESIAN_POINT('Ctrl Pts',(-39.5010226636067,1.83757264792979,
-95.3979932721737));
#147164=CARTESIAN_POINT('Ctrl Pts',(-40.1772697316389,2.46999998000002,
-95.1228183440041));
#147165=CARTESIAN_POINT('Ctrl Pts',(-39.5564442323333,2.46999998000002,
-94.8139619018179));
#147166=CARTESIAN_POINT('Ctrl Pts',(-39.7525219240431,1.81208306781681,
-94.9115092131337));
#147167=CARTESIAN_POINT('Origin',(-39.5,1.96999998000002,-98.0457798926543));
#147168=CARTESIAN_POINT('Origin',(-39.5,1.96999998000002,-55.24995));
#147169=CARTESIAN_POINT('',(-39.0000000009311,1.96999998000004,-134.012863078852));
#147170=CARTESIAN_POINT('Origin',(-39.5,1.96999998000002,-134.012863078852));
#147171=CARTESIAN_POINT('',(-39.,1.96999998000002,-129.34995));
#147172=CARTESIAN_POINT('Ctrl Pts',(-40.2368360569361,2.46999998000002,
-137.052481127874));
#147173=CARTESIAN_POINT('Ctrl Pts',(-39.6136204540295,2.46999998000002,
-137.379413138382));
#147174=CARTESIAN_POINT('Ctrl Pts',(-39.8187349738493,1.80543983340093,
-137.271832963441));
#147175=CARTESIAN_POINT('Ctrl Pts',(-39.9798259099587,2.46999998000002,
-136.561879380276));
#147176=CARTESIAN_POINT('Ctrl Pts',(-39.3750396288604,2.46999997999999,
-136.834113716861));
#147177=CARTESIAN_POINT('Ctrl Pts',(-39.533173705558,1.83299741787672,-136.747405829844));
#147178=CARTESIAN_POINT('Ctrl Pts',(-39.7942596598039,2.46999998000002,
-136.049446128364));
#147179=CARTESIAN_POINT('Ctrl Pts',(-39.2024243343545,2.46999998000014,
-136.257081974912));
#147180=CARTESIAN_POINT('Ctrl Pts',(-39.3269752687565,1.86132354549721,
-136.198841734389));
#147181=CARTESIAN_POINT('Ctrl Pts',(-39.548909562734,2.46999998000002,-134.986769967065));
#147182=CARTESIAN_POINT('Ctrl Pts',(-39.002744048575,2.4699999799999,-135.08361190439));
#147183=CARTESIAN_POINT('Ctrl Pts',(-39.0543528686939,1.91883278031583,
-135.059436829036));
#147184=CARTESIAN_POINT('Ctrl Pts',(-39.4903493414456,2.46999998000002,
-134.432158073852));
#147185=CARTESIAN_POINT('Ctrl Pts',(-38.9670451935713,2.46999998000003,
-134.480163550531));
#147186=CARTESIAN_POINT('Ctrl Pts',(-38.9892810036075,1.94823440239765,
-134.463878808121));
#147187=CARTESIAN_POINT('Ctrl Pts',(-39.5012955382995,2.46999998000002,
-133.88255272146));
#147188=CARTESIAN_POINT('Ctrl Pts',(-39.0080109328159,2.46999998000002,
-133.872820118988));
#147189=CARTESIAN_POINT('Ctrl Pts',(-39.0014382726235,1.9766623627072,-133.872717663268));
#147190=CARTESIAN_POINT('',(-39.7525219025349,1.81208317107913,-137.147133709894));
#147191=CARTESIAN_POINT('Origin',(-40.1772697316389,1.96999998000002,-136.935824627502));
#147192=CARTESIAN_POINT('Ctrl Pts',(-39.7525219099498,1.81208323948034,
-137.14713352867));
#147193=CARTESIAN_POINT('Ctrl Pts',(-39.6968925343529,1.81772142131488,
-137.039526872226));
#147194=CARTESIAN_POINT('Ctrl Pts',(-39.6445718142832,1.8234260406068,-136.930881467314));
#147195=CARTESIAN_POINT('Ctrl Pts',(-39.5954328440081,1.82915287678578,
-136.821276650554));
#147196=CARTESIAN_POINT('Ctrl Pts',(-39.5448884088858,1.83504351100306,
-136.708536934625));
#147197=CARTESIAN_POINT('Ctrl Pts',(-39.4977095071828,1.84095797203305,
-136.594781798714));
#147198=CARTESIAN_POINT('Ctrl Pts',(-39.4537815356419,1.8468787701165,-136.48005817389));
#147199=CARTESIAN_POINT('Ctrl Pts',(-39.409336899226,1.8528692064804,-136.363985211385));
#147200=CARTESIAN_POINT('Ctrl Pts',(-39.3682194543804,1.85886662434155,
-136.246920256174));
#147201=CARTESIAN_POINT('Ctrl Pts',(-39.3303455734763,1.86487745082245,
-136.128879413488));
#147202=CARTESIAN_POINT('Ctrl Pts',(-39.2920753921181,1.87095117271324,
-136.009603428312));
#147203=CARTESIAN_POINT('Ctrl Pts',(-39.2571164969226,1.87703914799669,
-135.889330315293));
#147204=CARTESIAN_POINT('Ctrl Pts',(-39.2254271316397,1.88316486453392,
-135.768053582341));
#147205=CARTESIAN_POINT('Ctrl Pts',(-39.2133661623124,1.88549631164886,
-135.72189566964));
#147206=CARTESIAN_POINT('Ctrl Pts',(-39.2017792998293,1.88783335377127,
-135.675592196414));
#147207=CARTESIAN_POINT('Ctrl Pts',(-39.1906661181429,1.89017765116493,
-135.629142282584));
#147208=CARTESIAN_POINT('Ctrl Pts',(-39.1550653416186,1.89768754436866,
-135.480341241757));
#147209=CARTESIAN_POINT('Ctrl Pts',(-39.1242778288881,1.90525270160959,
-135.329794467711));
#147210=CARTESIAN_POINT('Ctrl Pts',(-39.0984708604229,1.91283024764293,
-135.178016532208));
#147211=CARTESIAN_POINT('Ctrl Pts',(-39.0728066063579,1.92036588929918,
-135.027077939654));
#147212=CARTESIAN_POINT('Ctrl Pts',(-39.0520680596019,1.92791344971714,
-134.87492201065));
#147213=CARTESIAN_POINT('Ctrl Pts',(-39.0363734628629,1.93543991782654,
-134.7220749885));
#147214=CARTESIAN_POINT('Ctrl Pts',(-39.0208096281387,1.94290367797656,
-134.570501435488));
#147215=CARTESIAN_POINT('Ctrl Pts',(-39.0102060825658,1.95034640301488,
-134.418248521206));
#147216=CARTESIAN_POINT('Ctrl Pts',(-39.0046315415482,1.95774958009969,
-134.265845522775));
#147217=CARTESIAN_POINT('Ctrl Pts',(-39.0015475992384,1.96184515872506,
-134.181533280117));
#147218=CARTESIAN_POINT('Ctrl Pts',(-39.000001959376,1.96592890236697,-134.097175367266));
#147219=CARTESIAN_POINT('Ctrl Pts',(-39.0000000018622,1.96999998000005,
-134.012863078852));
#147220=CARTESIAN_POINT('Ctrl Pts',(-39.7525219240432,1.81208306781681,
-137.147133758372));
#147221=CARTESIAN_POINT('Ctrl Pts',(-39.5564442323333,2.46999998000002,
-137.244681069688));
#147222=CARTESIAN_POINT('Ctrl Pts',(-40.1772697316389,2.46999998000002,
-136.935824627502));
#147223=CARTESIAN_POINT('Ctrl Pts',(-42.5829522730059,1.82186961480941,
-142.84383290998));
#147224=CARTESIAN_POINT('Ctrl Pts',(-42.3628976020159,2.46999998000001,
-142.852500243629));
#147225=CARTESIAN_POINT('Ctrl Pts',(-43.0113356415696,2.46999998000002,
-142.632517793947));
#147226=CARTESIAN_POINT('Ctrl Pts',(-45.385956606115,1.82990288117652,-148.554412051289));
#147227=CARTESIAN_POINT('Ctrl Pts',(-45.1914659347836,2.46999998002648,
-148.581690034117));
#147228=CARTESIAN_POINT('Ctrl Pts',(-45.8169723643538,2.46999998000002,
-148.343102920422));
#147229=CARTESIAN_POINT('Ctrl Pts',(-50.9608945753704,1.84386393970469,
-159.991229777381));
#147230=CARTESIAN_POINT('Ctrl Pts',(-50.7878173967191,2.46999997997405,
-160.008583439984));
#147231=CARTESIAN_POINT('Ctrl Pts',(-51.3962007668006,2.46999998000001,
-159.779920646508));
#147232=CARTESIAN_POINT('Ctrl Pts',(-53.7324859673961,1.84977562860519,
-165.717643463624));
#147233=CARTESIAN_POINT('Ctrl Pts',(-53.5753070147928,2.46999998000001,
-165.745313705806));
#147234=CARTESIAN_POINT('Ctrl Pts',(-54.1694331140562,2.46999998000001,
-165.506332215193));
#147235=CARTESIAN_POINT('Ctrl Pts',(-56.4941621559325,1.85499746228791,
-171.449026400902));
#147236=CARTESIAN_POINT('Ctrl Pts',(-56.3632322083114,2.46999998,-171.512146507354));
#147237=CARTESIAN_POINT('Ctrl Pts',(-56.9324803875071,2.46999998000001,
-171.237717270032));
#147238=CARTESIAN_POINT('',(-56.4941621559325,1.85499746228791,-171.449026400902));
#147239=CARTESIAN_POINT('Origin',(-56.9324803875071,1.96999998000001,-171.237717270032));
#147240=CARTESIAN_POINT('Ctrl Pts',(-56.4941621559325,1.85499746228791,
-171.449026400902));
#147241=CARTESIAN_POINT('Ctrl Pts',(-53.7324859673955,1.8497756286075,-165.717643463624));
#147242=CARTESIAN_POINT('Ctrl Pts',(-50.9608945753698,1.84386393970701,
-159.991229777381));
#147243=CARTESIAN_POINT('Ctrl Pts',(-45.3859566061143,1.82990288117884,
-148.554412051289));
#147244=CARTESIAN_POINT('Ctrl Pts',(-42.5829522730051,1.82186961481174,
-142.84383290998));
#147245=CARTESIAN_POINT('Ctrl Pts',(-39.7525219240432,1.81208306781682,
-137.147133758372));
#147246=CARTESIAN_POINT('Ctrl Pts',(-56.4736088945599,1.8573874935658,-171.409915902424));
#147247=CARTESIAN_POINT('Ctrl Pts',(-56.3489175136905,2.47012711531616,
-171.477038599322));
#147248=CARTESIAN_POINT('Ctrl Pts',(-56.9026784671178,2.46999996978156,
-171.178999526256));
#147249=CARTESIAN_POINT('Ctrl Pts',(-56.5595092645592,1.84739527439962,
-171.564880044108));
#147250=CARTESIAN_POINT('Ctrl Pts',(-56.4096617452282,2.47013088089768,
-171.619083147105));
#147251=CARTESIAN_POINT('Ctrl Pts',(-57.0276127026275,2.4699999696149,-171.411480993498));
#147252=CARTESIAN_POINT('Ctrl Pts',(-56.6013299245167,1.84257107601692,
-171.737940501487));
#147253=CARTESIAN_POINT('Ctrl Pts',(-56.4344504334064,2.4701327527474,-171.760758212924));
#147254=CARTESIAN_POINT('Ctrl Pts',(-57.0884505381249,2.46999996953445,
-171.671060999849));
#147255=CARTESIAN_POINT('Ctrl Pts',(-56.5930162481435,1.8435307818068,-171.916062071863));
#147256=CARTESIAN_POINT('Ctrl Pts',(-56.4294059961933,2.47013238231052,
-171.908444781729));
#147257=CARTESIAN_POINT('Ctrl Pts',(-57.0763566157493,2.46999996955046,
-171.938278709053));
#147258=CARTESIAN_POINT('Origin',(-57.077763566464,1.96999998000001,-171.871644662643));
#147259=CARTESIAN_POINT('Origin',(-55.230246199376,2.00193147732671,-171.934196687458));
#147260=CARTESIAN_POINT('Origin',(-57.077763566464,1.96999998000001,-179.64995));
#147261=CARTESIAN_POINT('Origin',(-57.077763566464,1.96999998000001,-176.848740272858));
#147262=CARTESIAN_POINT('Origin',(-57.,2.96999998000001,-174.34995));
#147263=CARTESIAN_POINT('',(-60.,2.96999998000001,-174.34995));
#147264=CARTESIAN_POINT('Origin',(-59.5,2.96999998000001,-174.34995));
#147265=CARTESIAN_POINT('',(-57.,2.96999998000001,-177.34995));
#147266=CARTESIAN_POINT('Origin',(-57.,2.96999998000001,-174.34995));
#147267=CARTESIAN_POINT('',(-57.,2.61702308584989,-177.204078948543));
#147268=CARTESIAN_POINT('Origin',(-57.,2.96999998000001,-176.84995));
#147269=CARTESIAN_POINT('Ctrl Pts',(-57.077763566464,2.46999998000001,-176.848740272858));
#147270=CARTESIAN_POINT('Ctrl Pts',(-57.0736014896981,2.46999998000001,
-176.982739539051));
#147271=CARTESIAN_POINT('Ctrl Pts',(-57.043897408659,2.52469464001198,-177.112050866152));
#147272=CARTESIAN_POINT('Ctrl Pts',(-57.,2.61702308584989,-177.204078948543));
#147273=CARTESIAN_POINT('Origin',(-59.5,2.96999998000001,-55.24995));
#147274=CARTESIAN_POINT('',(-60.,2.96999998000001,-58.24995));
#147275=CARTESIAN_POINT('Origin',(-59.5,2.96999998000001,-58.24995));
#147276=CARTESIAN_POINT('',(-60.,2.96999998000001,-174.34995));
#147277=CARTESIAN_POINT('Origin',(-57.,2.96999998000001,-58.24995));
#147278=CARTESIAN_POINT('Origin',(-57.,2.96999998000001,-58.24995));
#147279=CARTESIAN_POINT('Origin',(-57.,-2.42462934179819E-14,-58.24995));
#147280=CARTESIAN_POINT('',(-60.,3.46999998000001,-58.24995));
#147281=CARTESIAN_POINT('Origin',(-57.,3.46999998000001,-58.24995));
#147282=CARTESIAN_POINT('',(-60.,-54.58000002,-58.24995));
#147283=CARTESIAN_POINT('Origin',(-57.,3.46999998000001,-58.24995));
#147284=CARTESIAN_POINT('Origin',(-59.5,3.46999998000001,-58.24995));
#147285=CARTESIAN_POINT('Ctrl Pts',(-39.8417798628559,4.28988750369336,
-92.7506121713693));
#147286=CARTESIAN_POINT('Ctrl Pts',(-39.9519009607656,3.96999998000002,
-92.8065726369586));
#147287=CARTESIAN_POINT('Ctrl Pts',(-40.2576018765703,3.96999998000001,
-92.9619213022396));
#147288=CARTESIAN_POINT('Ctrl Pts',(-42.5267665504115,4.30001893486917,
-87.4583592347964));
#147289=CARTESIAN_POINT('Ctrl Pts',(-42.6535990616308,3.96999998005189,
-87.4723136103566));
#147290=CARTESIAN_POINT('Ctrl Pts',(-42.9469739380577,3.96999998000001,
-87.6696743385966));
#147291=CARTESIAN_POINT('Ctrl Pts',(-45.1797873789129,4.30850505828642,
-82.1496810404423));
#147292=CARTESIAN_POINT('Ctrl Pts',(-45.2981339154354,3.96999997998722,
-82.1711713234106));
#147293=CARTESIAN_POINT('Ctrl Pts',(-45.6032617662856,3.96999998000001,
-82.3609901713122));
#147294=CARTESIAN_POINT('Ctrl Pts',(-50.4483866457226,4.32340039588272,
-71.5131546212415));
#147295=CARTESIAN_POINT('Ctrl Pts',(-50.5607523082128,3.96999998001296,
-71.5306210575042));
#147296=CARTESIAN_POINT('Ctrl Pts',(-50.8772452803079,3.96999998000001,
-71.7244637521124));
#147297=CARTESIAN_POINT('Ctrl Pts',(-53.0636135580956,4.32979794413352,
-66.1851229312852));
#147298=CARTESIAN_POINT('Ctrl Pts',(-53.1696590969437,3.96999998001539,
-66.20755441643));
#147299=CARTESIAN_POINT('Ctrl Pts',(-53.4945734938964,3.96999998000001,
-66.3964343016074));
#147300=CARTESIAN_POINT('Ctrl Pts',(-55.6666368275827,4.33549309160632,
-60.8508735991007));
#147301=CARTESIAN_POINT('Ctrl Pts',(-55.7583700098454,3.96999998000001,
-60.8956682801396));
#147302=CARTESIAN_POINT('Ctrl Pts',(-56.0993680931338,3.96999998000001,
-61.0621827299711));
#147303=CARTESIAN_POINT('Origin',(-40.2576018765703,4.46999998000001,-92.9619213022396));
#147304=CARTESIAN_POINT('Origin',(-59.5,3.46999998000001,-55.24995));
#147305=CARTESIAN_POINT('',(-60.,3.46999998000001,-174.34995));
#147306=CARTESIAN_POINT('Origin',(-59.5,3.46999998000001,-174.34995));
#147307=CARTESIAN_POINT('',(-60.,3.46999998000001,-58.24995));
#147308=CARTESIAN_POINT('Origin',(-57.,3.46999998000001,-174.34995));
#147309=CARTESIAN_POINT('',(-57.,3.46999998000002,-177.34995));
#147310=CARTESIAN_POINT('Origin',(-57.,3.46999998000001,-176.84995));
#147311=CARTESIAN_POINT('Origin',(-57.,3.46999998000001,-174.34995));
#147312=CARTESIAN_POINT('Origin',(-60.,3.46999998000001,-176.84995));
#147313=CARTESIAN_POINT('',(-56.6639973329545,3.46999998000001,-177.34995));
#147314=CARTESIAN_POINT('',(-60.,3.46999998000001,-177.34995));
#147315=CARTESIAN_POINT('Ctrl Pts',(-56.6639973329545,3.46999998000001,
-177.34995));
#147316=CARTESIAN_POINT('Ctrl Pts',(-56.6512525237428,3.49196718394931,
-177.34995));
#147317=CARTESIAN_POINT('Ctrl Pts',(-56.638409424179,3.51400749072922,-177.348497985071));
#147318=CARTESIAN_POINT('Ctrl Pts',(-56.6256111772538,3.53587766712532,
-177.345591130597));
#147319=CARTESIAN_POINT('Ctrl Pts',(-56.6128072828548,3.55775749415936,
-177.342682993417));
#147320=CARTESIAN_POINT('Ctrl Pts',(-56.6000482806874,3.57946622894872,
-177.338318792525));
#147321=CARTESIAN_POINT('Ctrl Pts',(-56.5874775033198,3.60076486111489,
-177.332547706032));
#147322=CARTESIAN_POINT('Ctrl Pts',(-56.5758782741082,3.62041740201721,
-177.327222645132));
#147323=CARTESIAN_POINT('Ctrl Pts',(-56.5644392996185,3.63972036831063,
-177.320700481022));
#147324=CARTESIAN_POINT('Ctrl Pts',(-56.55327318179,3.65849822816206,-177.313057342243));
#147325=CARTESIAN_POINT('Ctrl Pts',(-56.5409041295215,3.6792990412609,-177.304590802261));
#147326=CARTESIAN_POINT('Ctrl Pts',(-56.528767320844,3.69963447340031,-177.294675450318));
#147327=CARTESIAN_POINT('Ctrl Pts',(-56.5170063855842,3.71926351161968,
-177.283387067871));
#147328=CARTESIAN_POINT('Ctrl Pts',(-56.505259388952,3.73886928622555,-177.272112063999));
#147329=CARTESIAN_POINT('Ctrl Pts',(-56.4938873753229,3.75776959928665,
-177.259467555873));
#147330=CARTESIAN_POINT('Ctrl Pts',(-56.4830334644546,3.77574315014845,
-177.245577493872));
#147331=CARTESIAN_POINT('Ctrl Pts',(-56.4736856290318,3.79122271299519,
-177.233614799948));
#147332=CARTESIAN_POINT('Ctrl Pts',(-56.4647220893045,3.80601492740013,
-177.220729185059));
#147333=CARTESIAN_POINT('Ctrl Pts',(-56.4562342721766,3.81999568465454,
-177.207025631657));
#147334=CARTESIAN_POINT('Ctrl Pts',(-56.4462721306327,3.8364048839292,-177.190941786237));
#147335=CARTESIAN_POINT('Ctrl Pts',(-56.4369089397934,3.85179681888003,
-177.173631278226));
#147336=CARTESIAN_POINT('Ctrl Pts',(-56.428262942834,3.86596506309141,-177.155255835143));
#147337=CARTESIAN_POINT('Ctrl Pts',(-56.4196371964386,3.88010012258878,
-177.136923430832));
#147338=CARTESIAN_POINT('Ctrl Pts',(-56.4117252882495,3.89301662424524,
-177.117531554289));
#147339=CARTESIAN_POINT('Ctrl Pts',(-56.4046446325427,3.90454306311565,
-177.097280363919));
#147340=CARTESIAN_POINT('Ctrl Pts',(-56.3987249342272,3.91417960577361,
-177.080349596136));
#147341=CARTESIAN_POINT('Ctrl Pts',(-56.3933862479742,3.92284500927668,
-177.06281908411));
#147342=CARTESIAN_POINT('Ctrl Pts',(-56.3886971856441,3.93046120142969,
-177.044822942092));
#147343=CARTESIAN_POINT('Ctrl Pts',(-56.3832835309579,3.9392543100379,-177.024045888662));
#147344=CARTESIAN_POINT('Ctrl Pts',(-56.3787297459052,3.94667107841779,
-177.002591890815));
#147345=CARTESIAN_POINT('Ctrl Pts',(-56.3750770606607,3.95260434330808,
-176.980690309454));
#147346=CARTESIAN_POINT('Ctrl Pts',(-56.3714253659076,3.95853599928657,
-176.958794667101));
#147347=CARTESIAN_POINT('Ctrl Pts',(-56.3686742823299,3.96298466796628,
-176.936452422772));
#147348=CARTESIAN_POINT('Ctrl Pts',(-56.3668650065705,3.96589210375174,
-176.913910938087));
#147349=CARTESIAN_POINT('Ctrl Pts',(-56.3651621901663,3.96862846349338,
-176.892695813916));
#147350=CARTESIAN_POINT('Ctrl Pts',(-56.3642936087743,3.96999998000001,
-176.871304903324));
#147351=CARTESIAN_POINT('Ctrl Pts',(-56.3642936064049,3.96999998000001,
-176.84995));
#147352=CARTESIAN_POINT('Origin',(-56.3642936064049,4.46999998000001,-179.64995));
#147353=CARTESIAN_POINT('Origin',(-56.3642936064049,4.46999998000001,-171.871644662643));
#147354=CARTESIAN_POINT('Origin',(-56.3642936064049,4.46999998000001,-176.84995));
#147355=CARTESIAN_POINT('Ctrl Pts',(-55.8855878616368,4.32236176169507,
-171.915575297858));
#147356=CARTESIAN_POINT('Ctrl Pts',(-55.9943718457987,3.96993791925994,
-171.920606124721));
#147357=CARTESIAN_POINT('Ctrl Pts',(-56.362878117604,3.96999998707827,-171.9375490258));
#147358=CARTESIAN_POINT('Ctrl Pts',(-55.8939328694509,4.32126340276226,
-171.739613349113));
#147359=CARTESIAN_POINT('Ctrl Pts',(-56.0043522879837,3.96993816409125,
-171.724641829017));
#147360=CARTESIAN_POINT('Ctrl Pts',(-56.3748852598388,3.96999998705621,
-171.673567304561));
#147361=CARTESIAN_POINT('Ctrl Pts',(-55.8520802190683,4.32676800360642,
-171.566123460328));
#147362=CARTESIAN_POINT('Ctrl Pts',(-55.9538751380083,3.96993692936931,
-171.529346602164));
#147363=CARTESIAN_POINT('Ctrl Pts',(-56.3146644389369,3.96999998716678,
-171.413359333373));
#147364=CARTESIAN_POINT('Ctrl Pts',(-55.7630923089791,4.33856909837021,
-171.409535679069));
#147365=CARTESIAN_POINT('Ctrl Pts',(-55.8512265932963,3.96993423686637,
-171.361424046831));
#147366=CARTESIAN_POINT('Ctrl Pts',(-56.1866565229903,3.96999998740383,
-171.178434208374));
#147367=CARTESIAN_POINT('',(-55.7843555297028,4.33575017898885,-171.449026400902));
#147368=CARTESIAN_POINT('Origin',(-56.2171666226051,4.46999998000001,-171.237717270032));
#147369=CARTESIAN_POINT('Origin',(-54.7568819751872,4.47301625251356,-171.880572980261));
#147370=CARTESIAN_POINT('Ctrl Pts',(-55.7843555297028,4.33575017898885,
-171.449026400902));
#147371=CARTESIAN_POINT('Ctrl Pts',(-55.8759673883189,3.96999998,-171.404299214979));
#147372=CARTESIAN_POINT('Ctrl Pts',(-56.2171666226051,3.96999998000001,
-171.237717270032));
#147373=CARTESIAN_POINT('Ctrl Pts',(-53.1620910906406,4.33003381235646,
-166.074376691472));
#147374=CARTESIAN_POINT('Ctrl Pts',(-53.2681640678716,3.96999998006972,
-166.052285867785));
#147375=CARTESIAN_POINT('Ctrl Pts',(-53.5931279590331,3.96999998000001,
-165.863065274939));
#147376=CARTESIAN_POINT('Ctrl Pts',(-50.5275177831741,4.32360860554286,
-160.70599701099));
#147377=CARTESIAN_POINT('Ctrl Pts',(-50.6399914208629,3.96999998001567,
-160.688987094682));
#147378=CARTESIAN_POINT('Ctrl Pts',(-50.9564483006955,3.96999998000001,
-160.494687880121));
#147379=CARTESIAN_POINT('Ctrl Pts',(-45.2197944205701,4.30863333062082,
-149.988992475295));
#147380=CARTESIAN_POINT('Ctrl Pts',(-45.3382862796144,3.96999997998453,
-149.967930534599));
#147381=CARTESIAN_POINT('Ctrl Pts',(-45.6433184787346,3.96999998000001,
-149.777683344423));
#147382=CARTESIAN_POINT('Ctrl Pts',(-42.547006853164,4.30009530891334,-144.640178460294));
#147383=CARTESIAN_POINT('Ctrl Pts',(-42.6741187750921,3.96999998000002,
-144.626843683376));
#147384=CARTESIAN_POINT('Ctrl Pts',(-42.9672472399765,3.96999998000001,
-144.428863195016));
#147385=CARTESIAN_POINT('Ctrl Pts',(-39.8417798628559,4.28988750369336,
-139.308030800137));
#147386=CARTESIAN_POINT('Ctrl Pts',(-39.9519009607656,3.96999998000002,
-139.252070334547));
#147387=CARTESIAN_POINT('Ctrl Pts',(-40.2576018765703,3.96999998000001,
-139.096721669266));
#147388=CARTESIAN_POINT('',(-39.8417798628559,4.28988750369336,-139.308030800137));
#147389=CARTESIAN_POINT('Origin',(-40.2576018765703,4.46999998000001,-139.096721669266));
#147390=CARTESIAN_POINT('Ctrl Pts',(-39.8417798628559,4.28988750369336,
-139.308030800137));
#147391=CARTESIAN_POINT('Ctrl Pts',(-42.547006853164,4.30009530891334,-144.640178460294));
#147392=CARTESIAN_POINT('Ctrl Pts',(-45.2197944205701,4.30863333062082,
-149.988992475295));
#147393=CARTESIAN_POINT('Ctrl Pts',(-50.5275177831741,4.32360860554286,
-160.70599701099));
#147394=CARTESIAN_POINT('Ctrl Pts',(-53.1620910906406,4.33003381235646,
-166.074376691472));
#147395=CARTESIAN_POINT('Ctrl Pts',(-55.7843555297028,4.33575017898885,
-171.449026400902));
#147396=CARTESIAN_POINT('Ctrl Pts',(-39.5006452494647,3.96999998000002,
-135.765140647295));
#147397=CARTESIAN_POINT('Ctrl Pts',(-38.9952902504278,3.96999998000001,
-135.758345202901));
#147398=CARTESIAN_POINT('Ctrl Pts',(-39.0007176781796,4.47537333373487,
-135.758410867476));
#147399=CARTESIAN_POINT('Ctrl Pts',(-39.4928147031327,3.96999998000002,
-136.361732614249));
#147400=CARTESIAN_POINT('Ctrl Pts',(-39.0186539030837,3.96999997999999,
-136.376595312284));
#147401=CARTESIAN_POINT('Ctrl Pts',(-38.9920125861994,4.44319084885118,
-136.395928609904));
#147402=CARTESIAN_POINT('Ctrl Pts',(-39.5563016945132,3.96999998000002,
-136.946343610491));
#147403=CARTESIAN_POINT('Ctrl Pts',(-39.1119466604377,3.96999998000028,
-136.996763230774));
#147404=CARTESIAN_POINT('Ctrl Pts',(-39.0625502874059,4.41106266091723,
-137.019624934458));
#147405=CARTESIAN_POINT('Ctrl Pts',(-39.8209093071024,3.96999998000002,
-138.091801575276));
#147406=CARTESIAN_POINT('Ctrl Pts',(-39.4455065674113,3.96999997999977,
-138.196241930898));
#147407=CARTESIAN_POINT('Ctrl Pts',(-39.3565523056356,4.34716680534984,
-138.239852049834));
#147408=CARTESIAN_POINT('Ctrl Pts',(-40.0249067020314,3.96999998000001,
-138.657274953305));
#147409=CARTESIAN_POINT('Ctrl Pts',(-39.6822172442077,3.96999997999977,
-138.786193354514));
#147410=CARTESIAN_POINT('Ctrl Pts',(-39.5832177453656,4.31512711082335,
-138.841288520716));
#147411=CARTESIAN_POINT('Ctrl Pts',(-40.3026878259433,3.96999998000001,
-139.183790066217));
#147412=CARTESIAN_POINT('Ctrl Pts',(-40.0028354069033,3.96999998000006,
-139.341990301777));
#147413=CARTESIAN_POINT('Ctrl Pts',(-39.8918569639406,4.28495188925998,
-139.400527284681));
#147414=CARTESIAN_POINT('',(-39.,4.46999998000001,-135.863383986541));
#147415=CARTESIAN_POINT('Origin',(-39.5,4.46999998000001,-135.863383986541));
#147416=CARTESIAN_POINT('Ctrl Pts',(-39.,4.46999998000001,-135.863383986541));
#147417=CARTESIAN_POINT('Ctrl Pts',(-39.0000000079857,4.46322313781914,
-135.997345455347));
#147418=CARTESIAN_POINT('Ctrl Pts',(-39.0035816630906,4.45643395135115,
-136.13071326381));
#147419=CARTESIAN_POINT('Ctrl Pts',(-39.0106410212532,4.44965345252242,
-136.263464717827));
#147420=CARTESIAN_POINT('Ctrl Pts',(-39.0178191132844,4.4427589100598,-136.398448966009));
#147421=CARTESIAN_POINT('Ctrl Pts',(-39.0285923600607,4.43587283021838,
-136.532796678209));
#147422=CARTESIAN_POINT('Ctrl Pts',(-39.0428966292102,4.42899941624294,
-136.66650693885));
#147423=CARTESIAN_POINT('Ctrl Pts',(-39.0572438241962,4.42210537576492,
-136.800618452064));
#147424=CARTESIAN_POINT('Ctrl Pts',(-39.0751430414656,4.4152234353718,-136.934089519031));
#147425=CARTESIAN_POINT('Ctrl Pts',(-39.0965800947071,4.40834883766489,
-137.066930171756));
#147426=CARTESIAN_POINT('Ctrl Pts',(-39.1179262242621,4.40150339805911,
-137.199207390612));
#147427=CARTESIAN_POINT('Ctrl Pts',(-39.1427802868893,4.39466455837632,
-137.330860369876));
#147428=CARTESIAN_POINT('Ctrl Pts',(-39.1711795471352,4.38782864206007,
-137.461897287268));
#147429=CARTESIAN_POINT('Ctrl Pts',(-39.1833297324556,4.38490400073638,
-137.517959410589));
#147430=CARTESIAN_POINT('Ctrl Pts',(-39.1961294752992,4.38197996731975,
-137.573908673113));
#147431=CARTESIAN_POINT('Ctrl Pts',(-39.2095844945887,4.37905678995323,
-137.629745040165));
#147432=CARTESIAN_POINT('Ctrl Pts',(-39.2451525049022,4.37132944296962,
-137.777347093828));
#147433=CARTESIAN_POINT('Ctrl Pts',(-39.2853508698145,4.36364419626997,
-137.924407380269));
#147434=CARTESIAN_POINT('Ctrl Pts',(-39.3302483641922,4.35597229663866,
-138.070491499552));
#147435=CARTESIAN_POINT('Ctrl Pts',(-39.3740760812887,4.34848319616003,
-138.213094857289));
#147436=CARTESIAN_POINT('Ctrl Pts',(-39.4223823137413,4.34100686721553,
-138.354768046511));
#147437=CARTESIAN_POINT('Ctrl Pts',(-39.4752127095435,4.3335527104114,-138.49508114583));
#147438=CARTESIAN_POINT('Ctrl Pts',(-39.527445058374,4.32618293563461,-138.633805882562));
#147439=CARTESIAN_POINT('Ctrl Pts',(-39.5841004388002,4.31883493157336,
-138.771201096999));
#147440=CARTESIAN_POINT('Ctrl Pts',(-39.6451946704874,4.31155255374419,
-138.906825786004));
#147441=CARTESIAN_POINT('Ctrl Pts',(-39.7062889021745,4.30427017591502,
-139.04245047501));
#147442=CARTESIAN_POINT('Ctrl Pts',(-39.771822798885,4.29705359933063,-139.176304484137));
#147443=CARTESIAN_POINT('Ctrl Pts',(-39.8417721751959,4.28997973064454,
-139.307922594137));
#147444=CARTESIAN_POINT('Origin',(-39.5,4.46999998000002,-55.24995));
#147445=CARTESIAN_POINT('',(-39.,4.46999998000002,-96.1952589849652));
#147446=CARTESIAN_POINT('Origin',(-39.5,4.46999998000001,-96.1952589849652));
#147447=CARTESIAN_POINT('',(-39.,4.46999998000002,-129.34995));
#147448=CARTESIAN_POINT('Ctrl Pts',(-40.2576018765703,3.96999998000001,
-92.9619213022396));
#147449=CARTESIAN_POINT('Ctrl Pts',(-39.9519009607655,3.96999998000001,
-92.8065726369586));
#147450=CARTESIAN_POINT('Ctrl Pts',(-39.8417798628559,4.28988750369336,
-92.7506121713693));
#147451=CARTESIAN_POINT('Ctrl Pts',(-40.0026978626623,3.96999998000001,
-93.4635309699092));
#147452=CARTESIAN_POINT('Ctrl Pts',(-39.6570458949425,3.9699999800025,-93.3357860473751));
#147453=CARTESIAN_POINT('Ctrl Pts',(-39.558565846057,4.31859237238363,-93.2834642887004));
#147454=CARTESIAN_POINT('Ctrl Pts',(-39.817114250256,3.96999998000002,-93.9870091547076));
#147455=CARTESIAN_POINT('Ctrl Pts',(-39.4410018196003,3.96999998000002,
-93.8819356839734));
#147456=CARTESIAN_POINT('Ctrl Pts',(-39.3523491668799,4.34822838553358,
-93.8402926529419));
#147457=CARTESIAN_POINT('Ctrl Pts',(-39.5650235754014,3.96999998000002,
-95.0708764103351));
#147458=CARTESIAN_POINT('Ctrl Pts',(-39.1236627362708,3.96999998000002,
-95.0167026881129));
#147459=CARTESIAN_POINT('Ctrl Pts',(-39.0722484171839,4.40869400027786,
-94.9948839370727));
#147460=CARTESIAN_POINT('Ctrl Pts',(-39.500000001452,3.96999998000002,-95.6349699403799));
#147461=CARTESIAN_POINT('Ctrl Pts',(-39.0293922558424,3.96999998000002,
-95.61424653503));
#147462=CARTESIAN_POINT('Ctrl Pts',(-39.,4.43971662334272,-95.5966316298752));
#147463=CARTESIAN_POINT('Ctrl Pts',(-39.5,3.96999998000002,-96.1952589849652));
#147464=CARTESIAN_POINT('Ctrl Pts',(-39.,3.96999998000001,-96.1952589849652));
#147465=CARTESIAN_POINT('Ctrl Pts',(-39.,4.46999998000002,-96.1952589849652));
#147466=CARTESIAN_POINT('Ctrl Pts',(-39.8417543268295,4.28989009189502,
-92.7506602165031));
#147467=CARTESIAN_POINT('Ctrl Pts',(-39.5585534503141,4.31859415382189,
-93.2834977599907));
#147468=CARTESIAN_POINT('Ctrl Pts',(-39.3523449576258,4.34822929418925,
-93.8403100037277));
#147469=CARTESIAN_POINT('Ctrl Pts',(-39.2122987920319,4.3784611929057,-94.4175882950073));
#147470=CARTESIAN_POINT('Ctrl Pts',(-39.072248417184,4.40869400027783,-94.9948839370727));
#147471=CARTESIAN_POINT('Ctrl Pts',(-39.,4.43971662334269,-95.5966316298752));
#147472=CARTESIAN_POINT('Ctrl Pts',(-39.,4.46999997999998,-96.1952589849652));
#147473=CARTESIAN_POINT('Ctrl Pts',(-40.0658654432757,9.93538940172282,
-86.8935063764011));
#147474=CARTESIAN_POINT('Ctrl Pts',(-39.,10.9256777712437,-87.8240033916746));
#147475=CARTESIAN_POINT('Ctrl Pts',(-39.,12.1842625441365,-89.0065976851046));
#147476=CARTESIAN_POINT('Ctrl Pts',(-40.0194662171323,8.81210183467955,
-88.1753591901201));
#147477=CARTESIAN_POINT('Ctrl Pts',(-39.,9.77616182941803,-89.1086695731953));
#147478=CARTESIAN_POINT('Ctrl Pts',(-39.,10.9797897629302,-90.28846680179));
#147479=CARTESIAN_POINT('Ctrl Pts',(-39.9723426990601,7.65560021428954,
-89.4314931216999));
#147480=CARTESIAN_POINT('Ctrl Pts',(-39.,8.58691729751272,-90.3710832422126));
#147481=CARTESIAN_POINT('Ctrl Pts',(-39.,9.73513866768107,-91.5445844304498));
#147482=CARTESIAN_POINT('Ctrl Pts',(-39.8778703452952,5.25671151505436,
-91.8642463668096));
#147483=CARTESIAN_POINT('Ctrl Pts',(-39.,6.11218708321155,-92.8159732515183));
#147484=CARTESIAN_POINT('Ctrl Pts',(-39.,7.14206310577898,-93.9773376754667));
#147485=CARTESIAN_POINT('Ctrl Pts',(-39.8310091356278,4.02698776925249,
-93.0281766935241));
#147486=CARTESIAN_POINT('Ctrl Pts',(-38.9999999999877,4.84006269065046,
-93.9862863085864));
#147487=CARTESIAN_POINT('Ctrl Pts',(-39.,5.80730703259943,-95.141285808143));
#147488=CARTESIAN_POINT('Ctrl Pts',(-39.7856125955649,2.75522821384069,
-94.1210748292835));
#147489=CARTESIAN_POINT('Ctrl Pts',(-39.,3.51696389869249,-95.0875400976674));
#147490=CARTESIAN_POINT('Ctrl Pts',(-39.,4.4206962941175,-96.234166137987));
#147491=CARTESIAN_POINT('',(-39.0000000003509,10.11999998,-91.1341759094044));
#147492=CARTESIAN_POINT('Ctrl Pts',(-39.0000000014036,10.11999998,-91.1341759094044));
#147493=CARTESIAN_POINT('Ctrl Pts',(-39.0000000011199,9.67730365003607,
-91.5752858705177));
#147494=CARTESIAN_POINT('Ctrl Pts',(-39.0000000008905,9.22960685182023,
-92.0113795712675));
#147495=CARTESIAN_POINT('Ctrl Pts',(-39.0000000007062,8.77598048479483,
-92.4423316323824));
#147496=CARTESIAN_POINT('Ctrl Pts',(-39.0000000006606,8.66387047827009,
-92.5488378716476));
#147497=CARTESIAN_POINT('Ctrl Pts',(-39.0000000006178,8.55139809473461,
-92.655029929952));
#147498=CARTESIAN_POINT('Ctrl Pts',(-39.0000000005776,8.43854888592042,
-92.7609056252126));
#147499=CARTESIAN_POINT('Ctrl Pts',(-39.0000000004289,8.02088208267292,
-93.1527627205862));
#147500=CARTESIAN_POINT('Ctrl Pts',(-39.000000000316,7.59947404052636,-93.538972567434));
#147501=CARTESIAN_POINT('Ctrl Pts',(-39.0000000002313,7.17350510091871,
-93.9192513866139));
#147502=CARTESIAN_POINT('Ctrl Pts',(-39.0000000001502,6.76608030666306,
-94.2829751355963));
#147503=CARTESIAN_POINT('Ctrl Pts',(-39.000000000095,6.35448332404243,-94.6412733528635));
#147504=CARTESIAN_POINT('Ctrl Pts',(-39.0000000000588,5.93796915879824,
-94.9938596180162));
#147505=CARTESIAN_POINT('Ctrl Pts',(-39.0000000000244,5.54178994091724,
-95.3292320072887));
#147506=CARTESIAN_POINT('Ctrl Pts',(-39.0000000000072,5.14116207582966,
-95.6594367346931));
#147507=CARTESIAN_POINT('Ctrl Pts',(-39.0000000000019,4.7354162137309,-95.9841886223937));
#147508=CARTESIAN_POINT('Ctrl Pts',(-39.0000000000007,4.64718860219477,
-96.0548044587339));
#147509=CARTESIAN_POINT('Ctrl Pts',(-39.0000000000001,4.55871888403425,
-96.1251623137627));
#147510=CARTESIAN_POINT('Ctrl Pts',(-39.,4.46999998000004,-96.1952589849652));
#147511=CARTESIAN_POINT('Ctrl Pts',(-39.,10.11999998,-91.1341759094044));
#147512=CARTESIAN_POINT('Ctrl Pts',(-39.,10.0814485101051,-90.4015548889157));
#147513=CARTESIAN_POINT('Ctrl Pts',(-39.0871202471367,10.0432464379346,
-89.6831085829417));
#147514=CARTESIAN_POINT('Ctrl Pts',(-39.4353702716187,9.96778569194113,
-88.2750332463665));
#147515=CARTESIAN_POINT('Ctrl Pts',(-39.7001620921283,9.93023578423926,
-87.5801598805708));
#147516=CARTESIAN_POINT('Ctrl Pts',(-40.0642139577648,9.89540181781398,
-86.9391114735715));
#147517=CARTESIAN_POINT('Ctrl Pts',(-53.6034226162473,9.94191093135267,
-60.8508735991007));
#147518=CARTESIAN_POINT('Ctrl Pts',(-53.3728980178288,10.61999998,-60.7339721953768));
#147519=CARTESIAN_POINT('Ctrl Pts',(-54.0201152391274,10.61999998,-61.0621827299711));
#147520=CARTESIAN_POINT('Ctrl Pts',(-51.389560409622,9.93573232969473,-65.2217230132311));
#147521=CARTESIAN_POINT('Ctrl Pts',(-51.1265017070351,10.6199999801373,
-65.1408421794535));
#147522=CARTESIAN_POINT('Ctrl Pts',(-51.803611404114,10.61999998,-65.4330340644));
#147523=CARTESIAN_POINT('Ctrl Pts',(-49.1597584431958,9.92893027259159,
-69.5840753787896));
#147524=CARTESIAN_POINT('Ctrl Pts',(-48.8773807075708,10.619999979979,-69.5080715791473));
#147525=CARTESIAN_POINT('Ctrl Pts',(-49.5707491962873,10.61999998,-69.7953845096657));
#147526=CARTESIAN_POINT('Ctrl Pts',(-44.653312474994,9.91361721971961,-78.2837188426078));
#147527=CARTESIAN_POINT('Ctrl Pts',(-44.3407772417843,10.6199999800215,
-78.1912921743765));
#147528=CARTESIAN_POINT('Ctrl Pts',(-45.0568309856751,10.61999998,-78.4950279734725));
#147529=CARTESIAN_POINT('Ctrl Pts',(-42.3769453400103,9.90511004010749,
-82.6211625596856));
#147530=CARTESIAN_POINT('Ctrl Pts',(-42.0362703406502,10.6199999800752,
-82.5368298570061));
#147531=CARTESIAN_POINT('Ctrl Pts',(-42.7760616201669,10.61999998,-82.8324761280086));
#147532=CARTESIAN_POINT('Ctrl Pts',(-40.064213984323,9.8954018152728,-86.9391114268059));
#147533=CARTESIAN_POINT('Ctrl Pts',(-39.7432392475337,10.61999998,-86.7667827168808));
#147534=CARTESIAN_POINT('Ctrl Pts',(-40.4577925858907,10.61999998,-87.1504205576762));
#147535=CARTESIAN_POINT('Origin',(-40.4577925858907,10.11999998,-87.1504205576762));
#147536=CARTESIAN_POINT('Ctrl Pts',(-53.7132658667155,9.94427345760885,
-171.427096642113));
#147537=CARTESIAN_POINT('Ctrl Pts',(-53.4900212150555,10.6200436404067,
-171.547539040488));
#147538=CARTESIAN_POINT('Ctrl Pts',(-54.1252562655568,10.6199999790853,
-171.204806771057));
#147539=CARTESIAN_POINT('Ctrl Pts',(-53.7965641368282,9.93061460392252,
-171.570704923163));
#147540=CARTESIAN_POINT('Ctrl Pts',(-53.5293152990567,10.6200454840217,
-171.669460818784));
#147541=CARTESIAN_POINT('Ctrl Pts',(-54.2414728015497,10.6199999790668,
-171.420234627167));
#147542=CARTESIAN_POINT('Ctrl Pts',(-53.8395077234189,9.92361807935438,
-171.731386846755));
#147543=CARTESIAN_POINT('Ctrl Pts',(-53.5404438804703,10.6200464809797,
-171.777144153382));
#147544=CARTESIAN_POINT('Ctrl Pts',(-54.3014296083321,10.6199999790573,
-171.661245462915));
#147545=CARTESIAN_POINT('Ctrl Pts',(-53.8346934801606,9.92440268025274,
-171.896703002604));
#147546=CARTESIAN_POINT('Ctrl Pts',(-53.5391294683121,10.6200463684923,
-171.888526671099));
#147547=CARTESIAN_POINT('Ctrl Pts',(-54.2947083191068,10.6199999790584,
-171.909234173462));
#147548=CARTESIAN_POINT('',(-53.7255998841352,9.94225131873297,-171.449026400902));
#147549=CARTESIAN_POINT('Origin',(-54.1424378198232,10.11999998,-171.237717270032));
#147550=CARTESIAN_POINT('Origin',(-54.2951871140408,10.11999998,-171.871644662643));
#147551=CARTESIAN_POINT('Origin',(-52.5986019878193,10.1270016580449,-171.886013583419));
#147552=CARTESIAN_POINT('Origin',(-54.2951871140408,10.11999998,-179.64995));
#147553=CARTESIAN_POINT('Origin',(-54.2951871140408,10.11999998,-176.84995));
#147554=CARTESIAN_POINT('Origin',(83.2809572255632,11.1199999800001,-176.84995));
#147555=CARTESIAN_POINT('',(-57.,11.11999998,-177.34995));
#147556=CARTESIAN_POINT('Origin',(-57.,11.11999998,-176.84995));
#147557=CARTESIAN_POINT('',(-53.8590042959267,11.11999998,-177.34995));
#147558=CARTESIAN_POINT('',(-60.,11.11999998,-177.34995));
#147559=CARTESIAN_POINT('Ctrl Pts',(-54.2951871140408,10.61999998,-176.84995));
#147560=CARTESIAN_POINT('Ctrl Pts',(-54.2951871094022,10.61999998,-176.919796282647));
#147561=CARTESIAN_POINT('Ctrl Pts',(-54.282897054019,10.6344777440414,-176.987189324297));
#147562=CARTESIAN_POINT('Ctrl Pts',(-54.2369068974943,10.6883272976786,
-177.111149481396));
#147563=CARTESIAN_POINT('Ctrl Pts',(-54.2036611796727,10.7271494012897,
-177.166153898004));
#147564=CARTESIAN_POINT('Ctrl Pts',(-54.1215658763003,10.8221729031368,
-177.256908861057));
#147565=CARTESIAN_POINT('Ctrl Pts',(-54.0742219292009,10.8766241714759,
-177.291358543608));
#147566=CARTESIAN_POINT('Ctrl Pts',(-53.9700011606116,10.9953079956486,
-177.338340413074));
#147567=CARTESIAN_POINT('Ctrl Pts',(-53.9152095126149,11.0571633006792,
-177.34995));
#147568=CARTESIAN_POINT('Ctrl Pts',(-53.8590042959267,11.11999998,-177.34995));
#147569=CARTESIAN_POINT('Origin',(-57.,11.11999998,-174.34995));
#147570=CARTESIAN_POINT('',(-60.,11.11999998,-174.34995));
#147571=CARTESIAN_POINT('Origin',(-59.5,11.11999998,-174.34995));
#147572=CARTESIAN_POINT('Origin',(-57.,11.11999998,-174.34995));
#147573=CARTESIAN_POINT('Origin',(-59.5,11.11999998,-55.24995));
#147574=CARTESIAN_POINT('',(-60.,11.11999998,-174.34995));
#147575=CARTESIAN_POINT('Ctrl Pts',(-39.5,10.61999998,-91.1341759094044));
#147576=CARTESIAN_POINT('Ctrl Pts',(-39.,10.61999998,-91.1341759094044));
#147577=CARTESIAN_POINT('Ctrl Pts',(-39.,10.11999998,-91.1341759094044));
#147578=CARTESIAN_POINT('Ctrl Pts',(-39.5000000020536,10.61999998,-90.4402448608912));
#147579=CARTESIAN_POINT('Ctrl Pts',(-38.9598916786063,10.61999998,-90.3719688890004));
#147580=CARTESIAN_POINT('Ctrl Pts',(-39.,10.0814485101051,-90.4015548889157));
#147581=CARTESIAN_POINT('Ctrl Pts',(-39.5784082214306,10.61999998,-89.7587725653299));
#147582=CARTESIAN_POINT('Ctrl Pts',(-39.0069350308393,10.61999998,-89.6407441936901));
#147583=CARTESIAN_POINT('Ctrl Pts',(-39.0871202471367,10.0432464379346,
-89.6831085829417));
#147584=CARTESIAN_POINT('Ctrl Pts',(-39.89183324926,10.61999998,-88.4214995542899));
#147585=CARTESIAN_POINT('Ctrl Pts',(-39.245797474144,10.61999998,-88.1799493597601));
#147586=CARTESIAN_POINT('Ctrl Pts',(-39.4353702758529,9.96778569102363,
-88.2750332292462));
#147587=CARTESIAN_POINT('Ctrl Pts',(-40.1301388343916,10.61999998,-87.7606994776464));
#147588=CARTESIAN_POINT('Ctrl Pts',(-39.4581171327344,10.61999998,-87.4384896017421));
#147589=CARTESIAN_POINT('Ctrl Pts',(-39.7001621050063,9.93023578241304,
-87.580159846776));
#147590=CARTESIAN_POINT('Ctrl Pts',(-40.4577925858907,10.61999998,-87.1504205576762));
#147591=CARTESIAN_POINT('Ctrl Pts',(-39.7432392475336,10.61999998,-86.7667827168808));
#147592=CARTESIAN_POINT('Ctrl Pts',(-40.064213984323,9.8954018152728,-86.9391114268059));
#147593=CARTESIAN_POINT('Origin',(-39.5,10.11999998,-91.1341759094044));
#147594=CARTESIAN_POINT('Origin',(-39.5,10.11999998,-55.24995));
#147595=CARTESIAN_POINT('',(-39.0000000003307,10.11999998,-140.924467062102));
#147596=CARTESIAN_POINT('Origin',(-39.5,10.11999998,-140.924467062102));
#147597=CARTESIAN_POINT('',(-39.,10.11999998,-129.34995));
#147598=CARTESIAN_POINT('Ctrl Pts',(-40.6666545727859,10.61999998,-145.271541906631));
#147599=CARTESIAN_POINT('Ctrl Pts',(-39.9386298681517,10.61999998,-145.722049280659));
#147600=CARTESIAN_POINT('Ctrl Pts',(-40.2964538775261,9.87423053204576,
-145.500920636949));
#147601=CARTESIAN_POINT('Ctrl Pts',(-40.2252930694247,10.61999998,-144.553023210506));
#147602=CARTESIAN_POINT('Ctrl Pts',(-39.5493658636703,10.61999998,-144.926690587367));
#147603=CARTESIAN_POINT('Ctrl Pts',(-39.8060841900594,9.91530069853091,
-144.746634756903));
#147604=CARTESIAN_POINT('Ctrl Pts',(-39.9277556139221,10.61999998,-143.785038173526));
#147605=CARTESIAN_POINT('Ctrl Pts',(-39.275725873409,10.61999998,-144.057794964171));
#147606=CARTESIAN_POINT('Ctrl Pts',(-39.4754129960987,9.95900873040137,
-143.939244770734));
#147607=CARTESIAN_POINT('Ctrl Pts',(-39.5483465195115,10.61999998,-142.176898403278));
#147608=CARTESIAN_POINT('Ctrl Pts',(-38.9857875579427,10.61999998,-142.298553027766));
#147609=CARTESIAN_POINT('Ctrl Pts',(-39.053767673473,10.0497742339444,-142.246026638163));
#147610=CARTESIAN_POINT('Ctrl Pts',(-39.471139351319,10.61999998,-141.33510811083));
#147611=CARTESIAN_POINT('Ctrl Pts',(-38.9439335251668,10.61999998,-141.396464936279));
#147612=CARTESIAN_POINT('Ctrl Pts',(-38.9679508580438,10.0969150082091,
-141.358373831859));
#147613=CARTESIAN_POINT('Ctrl Pts',(-39.5096103982927,10.61999998,-140.51133866194));
#147614=CARTESIAN_POINT('Ctrl Pts',(-39.0322223955025,10.61999998,-140.488711952169));
#147615=CARTESIAN_POINT('Ctrl Pts',(-39.0106607951198,10.1425265025536,
-140.488167507581));
#147616=CARTESIAN_POINT('',(-40.0642139705729,9.89540191650284,-145.11953147077));
#147617=CARTESIAN_POINT('Origin',(-40.4577925858907,10.11999998,-144.90822241383));
#147618=CARTESIAN_POINT('Ctrl Pts',(-40.0642139728404,9.89540198157303,
-145.11953138824));
#147619=CARTESIAN_POINT('Ctrl Pts',(-40.002351458265,9.90132139175144,-145.010598868768));
#147620=CARTESIAN_POINT('Ctrl Pts',(-39.94358948579,9.90737279989773,-144.900576570422));
#147621=CARTESIAN_POINT('Ctrl Pts',(-39.8877792387549,9.91347673417978,
-144.789574845718));
#147622=CARTESIAN_POINT('Ctrl Pts',(-39.8308107857465,9.919707340776,-144.676269550121));
#147623=CARTESIAN_POINT('Ctrl Pts',(-39.7769170800584,9.92599288696455,
-144.561943605637));
#147624=CARTESIAN_POINT('Ctrl Pts',(-39.7259463774167,9.93228888280149,
-144.446677879912));
#147625=CARTESIAN_POINT('Ctrl Pts',(-39.6734351827218,9.93877516307736,
-144.327928467966));
#147626=CARTESIAN_POINT('Ctrl Pts',(-39.6240255672203,9.94527281200331,
-144.208181399467));
#147627=CARTESIAN_POINT('Ctrl Pts',(-39.5775704396244,9.95177155785657,
-144.087489445839));
#147628=CARTESIAN_POINT('Ctrl Pts',(-39.5304878255662,9.95835808465577,
-143.965167261688));
#147629=CARTESIAN_POINT('Ctrl Pts',(-39.4864394012381,9.96494622145986,
-143.841874086364));
#147630=CARTESIAN_POINT('Ctrl Pts',(-39.4453020254186,9.97155811034743,
-143.717633667422));
#147631=CARTESIAN_POINT('Ctrl Pts',(-39.4035199172632,9.97827362515868,
-143.591446069937));
#147632=CARTESIAN_POINT('Ctrl Pts',(-39.3647402527405,9.98501420275193,
-143.464280813464));
#147633=CARTESIAN_POINT('Ctrl Pts',(-39.3288740919353,9.99182873162542,
-143.336137664792));
#147634=CARTESIAN_POINT('Ctrl Pts',(-39.3062701153551,9.99612346090792,
-143.255377843655));
#147635=CARTESIAN_POINT('Ctrl Pts',(-39.2848241991159,10.0004480486441,
-143.174229132943));
#147636=CARTESIAN_POINT('Ctrl Pts',(-39.2645234280954,10.0048182625419,
-143.092687886665));
#147637=CARTESIAN_POINT('Ctrl Pts',(-39.2108307463155,10.0163768631431,
-142.877022768137));
#147638=CARTESIAN_POINT('Ctrl Pts',(-39.1652210086604,10.0280753656729,
-142.65870232555));
#147639=CARTESIAN_POINT('Ctrl Pts',(-39.1277908815641,10.0398210480943,
-142.438684630891));
#147640=CARTESIAN_POINT('Ctrl Pts',(-39.089043042221,10.0519802324398,-142.210921303682));
#147641=CARTESIAN_POINT('Ctrl Pts',(-39.0590605395586,10.0641904270523,
-141.981338102442));
#147642=CARTESIAN_POINT('Ctrl Pts',(-39.037912413284,10.0763900147051,-141.751001744749));
#147643=CARTESIAN_POINT('Ctrl Pts',(-39.0170605976466,10.0884186714896,
-141.523892675944));
#147644=CARTESIAN_POINT('Ctrl Pts',(-39.0047974378935,10.1004377695582,
-141.296050430499));
#147645=CARTESIAN_POINT('Ctrl Pts',(-39.0011547572432,10.11241789425,-141.068516354615));
#147646=CARTESIAN_POINT('Ctrl Pts',(-39.0003857691051,10.1149469586025,
-141.020482771066));
#147647=CARTESIAN_POINT('Ctrl Pts',(-39.0000008244016,10.11747437054,-140.972463017993));
#147648=CARTESIAN_POINT('Ctrl Pts',(-39.0000000013228,10.1199999800001,
-140.924467062102));
#147649=CARTESIAN_POINT('Ctrl Pts',(-40.064213984323,9.8954018152728,-145.1195315447));
#147650=CARTESIAN_POINT('Ctrl Pts',(-39.7432392475336,10.61999998,-145.291860254625));
#147651=CARTESIAN_POINT('Ctrl Pts',(-40.4577925858907,10.61999998,-144.90822241383));
#147652=CARTESIAN_POINT('Ctrl Pts',(-42.3982233528881,9.90519935947367,
-149.477207192598));
#147653=CARTESIAN_POINT('Ctrl Pts',(-42.0569998298599,10.61999998,-149.560052788611));
#147654=CARTESIAN_POINT('Ctrl Pts',(-42.7973905232547,10.61999998,-149.265893474329));
#147655=CARTESIAN_POINT('Ctrl Pts',(-44.6952062210366,9.91377387366803,
-153.854728198786));
#147656=CARTESIAN_POINT('Ctrl Pts',(-44.3825306854435,10.6199999800261,
-153.946076900384));
#147657=CARTESIAN_POINT('Ctrl Pts',(-45.0988060523808,10.61999998,-153.643419067924));
#147658=CARTESIAN_POINT('Ctrl Pts',(-49.2422260788803,9.92919580612355,
-162.634871500674));
#147659=CARTESIAN_POINT('Ctrl Pts',(-48.9599089008669,10.6199999799746,
-162.709726895544));
#147660=CARTESIAN_POINT('Ctrl Pts',(-49.6533413888222,10.61999998,-162.423562369795));
#147661=CARTESIAN_POINT('Ctrl Pts',(-51.491975374397,9.936039246645,-167.037652347168));
#147662=CARTESIAN_POINT('Ctrl Pts',(-51.2291869847762,10.6199999797401,
-167.117625919029));
#147663=CARTESIAN_POINT('Ctrl Pts',(-51.9061633492443,10.61999998,-166.826341244199));
#147664=CARTESIAN_POINT('Ctrl Pts',(-53.7255998841352,9.94225131873298,
-171.449026400902));
#147665=CARTESIAN_POINT('Ctrl Pts',(-53.4956787755832,10.61999998,-171.565581122671));
#147666=CARTESIAN_POINT('Ctrl Pts',(-54.1424378198232,10.61999998,-171.237717270032));
#147667=CARTESIAN_POINT('Ctrl Pts',(-53.7255998841352,9.94225131873297,
-171.449026400902));
#147668=CARTESIAN_POINT('Ctrl Pts',(-51.4919753743962,9.93603924664709,
-167.037652347168));
#147669=CARTESIAN_POINT('Ctrl Pts',(-49.2422260788795,9.92919580612563,
-162.634871500674));
#147670=CARTESIAN_POINT('Ctrl Pts',(-44.6952062210357,9.91377387367011,
-153.854728198786));
#147671=CARTESIAN_POINT('Ctrl Pts',(-42.3982233528871,9.90519935947574,
-149.477207192598));
#147672=CARTESIAN_POINT('Ctrl Pts',(-40.064213984323,9.8954018152728,-145.1195315447));
#147673=CARTESIAN_POINT('Ctrl Pts',(-38.8323560497301,-56.2084592670262,
-61.2273317382593));
#147674=CARTESIAN_POINT('Ctrl Pts',(-39.0122500629964,-56.4087764892537,
-60.6499500000001));
#147675=CARTESIAN_POINT('Ctrl Pts',(-39.4379155619868,-56.882767417621,
-60.64995));
#147676=CARTESIAN_POINT('Ctrl Pts',(-38.9597499727218,-56.0859430057577,
-61.2402727589806));
#147677=CARTESIAN_POINT('Ctrl Pts',(-39.1308890120013,-56.2886813392436,
-60.64995));
#147678=CARTESIAN_POINT('Ctrl Pts',(-39.5470561894999,-56.7847541538272,
-60.64995));
#147679=CARTESIAN_POINT('Ctrl Pts',(-39.0917129041016,-55.9712198429402,
-61.2536666704059));
#147680=CARTESIAN_POINT('Ctrl Pts',(-39.2535572856597,-56.1757390223779,
-60.64995));
#147681=CARTESIAN_POINT('Ctrl Pts',(-39.6600993514669,-56.6929757051825,
-60.64995));
#147682=CARTESIAN_POINT('Ctrl Pts',(-39.2278317447683,-55.8636034060938,
-61.2674693219905));
#147683=CARTESIAN_POINT('Ctrl Pts',(-39.3796800351166,-56.0692409848678,
-60.64995));
#147684=CARTESIAN_POINT('Ctrl Pts',(-39.7766890844069,-56.606882728875,
-60.64995));
#147685=CARTESIAN_POINT('',(-39.2253966502056,-55.8655297208509,-61.2672223984388));
#147686=CARTESIAN_POINT('',(-38.8323576630952,-56.2084583512428,-61.2273323469212));
#147687=CARTESIAN_POINT('Ctrl Pts',(-39.2253966502054,-55.865529720851,
-61.2672223984388));
#147688=CARTESIAN_POINT('Ctrl Pts',(-39.0894849099381,-55.973106721351,
-61.2534405956196));
#147689=CARTESIAN_POINT('Ctrl Pts',(-38.9583675005087,-56.087272628509,
-61.2401323247394));
#147690=CARTESIAN_POINT('Ctrl Pts',(-38.8323573704738,-56.2084579968516,
-61.227331872424));
#147691=CARTESIAN_POINT('Origin',(-39.4379155619868,-56.882767417621,-61.64995));
#147692=CARTESIAN_POINT('Ctrl Pts',(-39.2253966502054,-55.865529720851,
-61.2672223984388));
#147693=CARTESIAN_POINT('Ctrl Pts',(-39.2371501417372,-55.9108514932488,
-61.1623844624743));
#147694=CARTESIAN_POINT('Ctrl Pts',(-39.2529884923231,-55.9713882406491,
-61.071384516352));
#147695=CARTESIAN_POINT('Ctrl Pts',(-39.2917636103596,-56.1160106335832,
-60.9126819775317));
#147696=CARTESIAN_POINT('Ctrl Pts',(-39.3137989788887,-56.1967066207402,
-60.8488138257101));
#147697=CARTESIAN_POINT('Ctrl Pts',(-39.3624939333409,-56.3700857302443,
-60.7466874393643));
#147698=CARTESIAN_POINT('Ctrl Pts',(-39.388248240317,-56.4595484948523,
-60.710350981156));
#147699=CARTESIAN_POINT('Ctrl Pts',(-39.4424275296133,-56.6422462965493,
-60.6618415351963));
#147700=CARTESIAN_POINT('Ctrl Pts',(-39.4710350160438,-56.736024652106,
-60.6499500783916));
#147701=CARTESIAN_POINT('Ctrl Pts',(-39.4999997135852,-56.828045000138,
-60.6499500000004));
#147702=CARTESIAN_POINT('Origin',(-39.5,-12.9675000200281,-61.14995));
#147703=CARTESIAN_POINT('Origin',(-39.5,-56.8280459100727,-61.14995));
#147704=CARTESIAN_POINT('Origin',(-33.85,67.7009572055632,-61.14995));
#147705=CARTESIAN_POINT('Origin',(-33.85,-61.3211699373828,-61.14995));
#147706=CARTESIAN_POINT('Origin',(0.,-12.9675000200281,-61.64995));
#147707=CARTESIAN_POINT('',(-33.5881101525803,-60.3971457002532,-61.2273317382593));
#147708=CARTESIAN_POINT('Origin',(0.,-12.9675000200281,-61.2273317382593));
#147709=CARTESIAN_POINT('Ctrl Pts',(-33.85,-61.3211699373828,-60.64995));
#147710=CARTESIAN_POINT('Ctrl Pts',(-33.7991562663074,-61.1403193911197,
-60.64995));
#147711=CARTESIAN_POINT('Ctrl Pts',(-33.7471512515707,-60.9562715767294,
-60.6978885776012));
#147712=CARTESIAN_POINT('Ctrl Pts',(-33.6552207448938,-60.6322769136983,
-60.8896846949796));
#147713=CARTESIAN_POINT('Ctrl Pts',(-33.6142503615382,-60.4886315879339,
-61.034824258355));
#147714=CARTESIAN_POINT('Ctrl Pts',(-33.5881101525803,-60.3971457002532,
-61.2273317382593));
#147715=CARTESIAN_POINT('Ctrl Pts',(-39.5,-62.6133861954129,-171.64995));
#147716=CARTESIAN_POINT('Ctrl Pts',(-40.,-62.6133861954129,-171.64995));
#147717=CARTESIAN_POINT('Ctrl Pts',(-40.,-62.6133861954129,-171.14995));
#147718=CARTESIAN_POINT('Ctrl Pts',(-39.4908895000012,-62.7468765389391,
-171.64995));
#147719=CARTESIAN_POINT('Ctrl Pts',(-39.9999999999999,-62.7481681417254,
-171.659148653594));
#147720=CARTESIAN_POINT('Ctrl Pts',(-40.,-62.8117011147884,-171.149950000016));
#147721=CARTESIAN_POINT('Ctrl Pts',(-39.4817858670191,-62.8802662644338,
-171.67597732698));
#147722=CARTESIAN_POINT('Ctrl Pts',(-40.,-62.8775589599766,-171.69520402023));
#147723=CARTESIAN_POINT('Ctrl Pts',(-40.,-63.0098665547682,-171.18899099047));
#147724=CARTESIAN_POINT('Ctrl Pts',(-39.4649548930126,-63.1268797875294,
-171.776163607997));
#147725=CARTESIAN_POINT('Ctrl Pts',(-40.0000000000001,-63.1103377557996,
-171.809929875206));
#147726=CARTESIAN_POINT('Ctrl Pts',(-40.,-63.3762386807026,-171.339270411997));
#147727=CARTESIAN_POINT('Ctrl Pts',(-39.4572358131761,-63.2399825392123,
-171.850283164391));
#147728=CARTESIAN_POINT('Ctrl Pts',(-40.000000000002,-63.2129124685353,
-171.888983273332));
#147729=CARTESIAN_POINT('Ctrl Pts',(-40.,-63.5442655393439,-171.450449746589));
#147730=CARTESIAN_POINT('Ctrl Pts',(-39.4443539433762,-63.4287323580851,
-172.035403273235));
#147731=CARTESIAN_POINT('Ctrl Pts',(-39.9999999999979,-63.3805692396919,
-172.075215659168));
#147732=CARTESIAN_POINT('Ctrl Pts',(-40.,-63.8246746245531,-171.728129909852));
#147733=CARTESIAN_POINT('Ctrl Pts',(-39.4391962191206,-63.5043052007179,
-172.14633102856));
#147734=CARTESIAN_POINT('Ctrl Pts',(-40.,-63.4448403055015,-172.182182441317));
#147735=CARTESIAN_POINT('Ctrl Pts',(-40.,-63.9369465821947,-171.894521542842));
#147736=CARTESIAN_POINT('Ctrl Pts',(-39.4322246014262,-63.6064558665446,
-172.38820210671));
#147737=CARTESIAN_POINT('Ctrl Pts',(-40.,-63.5312736349196,-172.409726298163));
#147738=CARTESIAN_POINT('Ctrl Pts',(-40.,-64.0887028854776,-172.257328160063));
#147739=CARTESIAN_POINT('Ctrl Pts',(-39.4304134495212,-63.6329935198199,
-172.51902671195));
#147740=CARTESIAN_POINT('Ctrl Pts',(-40.,-63.5529433505843,-172.529650273728));
#147741=CARTESIAN_POINT('Ctrl Pts',(-40.,-64.1281275541786,-172.453565067926));
#147742=CARTESIAN_POINT('Ctrl Pts',(-39.43041344952,-63.63299351982,-172.64995));
#147743=CARTESIAN_POINT('Ctrl Pts',(-40.,-63.5529433505803,-172.64995));
#147744=CARTESIAN_POINT('Ctrl Pts',(-40.,-64.1281275541908,-172.64995));
#147745=CARTESIAN_POINT('',(-39.5,-62.6133861954129,-171.64995));
#147746=CARTESIAN_POINT('Origin',(-39.5,-62.6133861954129,-171.14995));
#147747=CARTESIAN_POINT('',(-39.5,-63.6281275541908,-172.64995));
#147748=CARTESIAN_POINT('Origin',(-39.5,-64.1281275541908,-172.64995));
#147749=CARTESIAN_POINT('Origin',(-39.5,-64.1281275541908,-172.64995));
#147750=CARTESIAN_POINT('Ctrl Pts',(-39.43041344952,-63.6329935198201,-172.64995));
#147751=CARTESIAN_POINT('Ctrl Pts',(-39.4304134495212,-63.6329935198199,
-172.51902671195));
#147752=CARTESIAN_POINT('Ctrl Pts',(-39.4322246014262,-63.6064558665446,
-172.38820210671));
#147753=CARTESIAN_POINT('Ctrl Pts',(-39.4391962191206,-63.5043052007179,
-172.14633102856));
#147754=CARTESIAN_POINT('Ctrl Pts',(-39.4443539433762,-63.4287323580851,
-172.035403273235));
#147755=CARTESIAN_POINT('Ctrl Pts',(-39.4572358131761,-63.2399825392123,
-171.850283164391));
#147756=CARTESIAN_POINT('Ctrl Pts',(-39.4649548930126,-63.1268797875294,
-171.776163607997));
#147757=CARTESIAN_POINT('Ctrl Pts',(-39.4817858670191,-62.8802662644338,
-171.67597732698));
#147758=CARTESIAN_POINT('Ctrl Pts',(-39.4908895000012,-62.7468765389391,
-171.64995));
#147759=CARTESIAN_POINT('Ctrl Pts',(-39.5,-62.6133861954129,-171.64995));
#147760=CARTESIAN_POINT('Origin',(-39.5,-64.1281275541909,-55.24995));
#147761=CARTESIAN_POINT('Origin',(-39.5,-64.1281275541909,-176.84995));
#147762=CARTESIAN_POINT('Origin',(-40.5,67.7009572055632,-176.84995));
#147763=CARTESIAN_POINT('',(-40.5,-70.08000002,-177.34995));
#147764=CARTESIAN_POINT('Origin',(-40.5,-70.08000002,-176.84995));
#147765=CARTESIAN_POINT('',(-40.5,-63.9875867194884,-177.34995));
#147766=CARTESIAN_POINT('',(-40.5,-73.08000002,-177.34995));
#147767=CARTESIAN_POINT('Ctrl Pts',(-40.,-64.1281275541909,-176.84995));
#147768=CARTESIAN_POINT('Ctrl Pts',(-40.,-64.1281275541799,-176.981217345763));
#147769=CARTESIAN_POINT('Ctrl Pts',(-40.0538865634702,-64.1129810289718,
-177.110943344657));
#147770=CARTESIAN_POINT('Ctrl Pts',(-40.2390066553433,-64.0609471645084,
-177.29606343653));
#147771=CARTESIAN_POINT('Ctrl Pts',(-40.3687326542369,-64.0244835641743,
-177.34995));
#147772=CARTESIAN_POINT('Ctrl Pts',(-40.5,-63.9875867194884,-177.34995));
#147773=CARTESIAN_POINT('Origin',(-40.5,-70.08000002,-174.34995));
#147774=CARTESIAN_POINT('',(-40.5,-73.08000002,-174.34995));
#147775=CARTESIAN_POINT('Origin',(-40.5,-72.58000002,-174.34995));
#147776=CARTESIAN_POINT('Origin',(-40.5,-70.08000002,-174.34995));
#147777=CARTESIAN_POINT('Origin',(-40.5,-72.58000002,-55.24995));
#147778=CARTESIAN_POINT('',(-40.5,-73.08000002,-58.24995));
#147779=CARTESIAN_POINT('Origin',(-40.5,-72.58000002,-58.24995));
#147780=CARTESIAN_POINT('',(-40.5,-73.08000002,-174.34995));
#147781=CARTESIAN_POINT('Origin',(-40.5,-70.08000002,-58.24995));
#147782=CARTESIAN_POINT('Origin',(-40.5,-70.08000002,-58.24995));
#147783=CARTESIAN_POINT('Ctrl Pts',(-40.,-56.2369767507698,-61.4585861992214));
#147784=CARTESIAN_POINT('Ctrl Pts',(-40.,-55.4129915017071,-61.0340816633164));
#147785=CARTESIAN_POINT('Ctrl Pts',(-39.2253966502054,-55.8655297208549,
-61.2672223984414));
#147786=CARTESIAN_POINT('Ctrl Pts',(-40.,-56.2639883391117,-61.4061555156247));
#147787=CARTESIAN_POINT('Ctrl Pts',(-39.9999999999999,-55.5211143346859,
-60.8908068027146));
#147788=CARTESIAN_POINT('Ctrl Pts',(-39.2371501417372,-55.9108514932488,
-61.1623844624743));
#147789=CARTESIAN_POINT('Ctrl Pts',(-40.,-56.3001438773882,-61.3606672793622));
#147790=CARTESIAN_POINT('Ctrl Pts',(-40.0000000000002,-55.6524517483454,
-60.789214714877));
#147791=CARTESIAN_POINT('Ctrl Pts',(-39.2529884923231,-55.9713882406491,
-61.071384516352));
#147792=CARTESIAN_POINT('Ctrl Pts',(-40.,-56.3871674054812,-61.2813159675772));
#147793=CARTESIAN_POINT('Ctrl Pts',(-39.9999999999997,-55.9239397495629,
-60.6499875251594));
#147794=CARTESIAN_POINT('Ctrl Pts',(-39.2917636103596,-56.1160106335832,
-60.9126819775317));
#147795=CARTESIAN_POINT('Ctrl Pts',(-40.,-56.4359944422203,-61.2493819347541));
#147796=CARTESIAN_POINT('Ctrl Pts',(-40.0000000000002,-56.0556314220498,
-60.6123860933136));
#147797=CARTESIAN_POINT('Ctrl Pts',(-39.3137989788887,-56.1967066207402,
-60.8488138257101));
#147798=CARTESIAN_POINT('Ctrl Pts',(-40.,-56.5418574657904,-61.1983186977834));
#147799=CARTESIAN_POINT('Ctrl Pts',(-39.9999999999998,-56.3054150365844,
-60.5765024526906));
#147800=CARTESIAN_POINT('Ctrl Pts',(-39.3624939333409,-56.3700857302443,
-60.7466874393643));
#147801=CARTESIAN_POINT('Ctrl Pts',(-40.,-56.5969271200065,-61.1801504966336));
#147802=CARTESIAN_POINT('Ctrl Pts',(-40.0000000000002,-56.4198805079413,
-60.5763728571923));
#147803=CARTESIAN_POINT('Ctrl Pts',(-39.388248240317,-56.4595484948523,
-60.710350981156));
#147804=CARTESIAN_POINT('Ctrl Pts',(-40.,-56.7105746147406,-61.1558957215692));
#147805=CARTESIAN_POINT('Ctrl Pts',(-39.9999999999997,-56.6330323209014,
-60.5986229708875));
#147806=CARTESIAN_POINT('Ctrl Pts',(-39.4424276189043,-56.6422465976472,
-60.6618414552496));
#147807=CARTESIAN_POINT('Ctrl Pts',(-40.,-56.769502228095,-61.1499499952173));
#147808=CARTESIAN_POINT('Ctrl Pts',(-40.,-56.733312609114,-60.6201312992477));
#147809=CARTESIAN_POINT('Ctrl Pts',(-39.4710352046322,-56.7360252703185,
-60.64995));
#147810=CARTESIAN_POINT('Ctrl Pts',(-40.,-56.8280459100727,-61.14995));
#147811=CARTESIAN_POINT('Ctrl Pts',(-40.,-56.8280459100727,-60.64995));
#147812=CARTESIAN_POINT('Ctrl Pts',(-39.5,-56.8280459100727,-60.64995));
#147813=CARTESIAN_POINT('Origin',(-39.5,-56.2369767507657,-61.4585861992193));
#147814=CARTESIAN_POINT('Ctrl Pts',(-40.,-55.08000002,-66.6681042685293));
#147815=CARTESIAN_POINT('Ctrl Pts',(-39.9999999999999,-54.5800000200005,
-66.6681042685296));
#147816=CARTESIAN_POINT('Ctrl Pts',(-39.5,-54.58000002,-66.6681042685296));
#147817=CARTESIAN_POINT('Ctrl Pts',(-40.,-55.0800000210321,-65.7666038778627));
#147818=CARTESIAN_POINT('Ctrl Pts',(-40.000000000023,-54.5300790303385,
-65.6851286065597));
#147819=CARTESIAN_POINT('Ctrl Pts',(-39.4524759569592,-54.5800000199993,
-65.7323260169345));
#147820=CARTESIAN_POINT('Ctrl Pts',(-40.,-55.1697676396346,-64.8773517277477));
#147821=CARTESIAN_POINT('Ctrl Pts',(-40.,-54.5798306201335,-64.744699921287));
#147822=CARTESIAN_POINT('Ctrl Pts',(-39.4055862633018,-54.6797418208431,
-64.8099001089231));
#147823=CARTESIAN_POINT('Ctrl Pts',(-40.,-55.4484096194251,-63.5638700072085));
#147824=CARTESIAN_POINT('Ctrl Pts',(-40.,-54.7700293023446,-63.3785482937886));
#147825=CARTESIAN_POINT('Ctrl Pts',(-39.336341776171,-54.9893440187367,
-63.4482326198876));
#147826=CARTESIAN_POINT('Ctrl Pts',(-40.,-55.5665711459207,-63.1272943707367));
#147827=CARTESIAN_POINT('Ctrl Pts',(-40.,-54.8613740727702,-62.9031901152049));
#147828=CARTESIAN_POINT('Ctrl Pts',(-39.3133286552319,-55.1206346051679,
-62.9957806797004));
#147829=CARTESIAN_POINT('Ctrl Pts',(-40.,-55.8576823946199,-62.2755058384848));
#147830=CARTESIAN_POINT('Ctrl Pts',(-40.,-55.0944248813133,-61.958211698159));
#147831=CARTESIAN_POINT('Ctrl Pts',(-39.2684369452391,-55.4440915465439,
-62.113263414855));
#147832=CARTESIAN_POINT('Ctrl Pts',(-40.,-56.0300729172808,-61.8601972461309));
#147833=CARTESIAN_POINT('Ctrl Pts',(-39.9999999999954,-55.2406041652953,
-61.4857700511268));
#147834=CARTESIAN_POINT('Ctrl Pts',(-39.2465526403215,-55.635643675915,
-61.6830846593873));
#147835=CARTESIAN_POINT('Ctrl Pts',(-40.,-56.2369767507657,-61.4585861992193));
#147836=CARTESIAN_POINT('Ctrl Pts',(-39.9999999999999,-55.4129915017042,
-61.0340816633138));
#147837=CARTESIAN_POINT('Ctrl Pts',(-39.2253966502057,-55.8655297208508,
-61.2672223984388));
#147838=CARTESIAN_POINT('',(-39.4999999999985,-54.58000002,-66.6681042685273));
#147839=CARTESIAN_POINT('Origin',(-39.5,-55.08000002,-66.6681042685293));
#147840=CARTESIAN_POINT('Ctrl Pts',(-39.4999999999998,-54.58000002,-66.6681042685264));
#147841=CARTESIAN_POINT('Ctrl Pts',(-39.4524759569591,-54.5800000199995,
-65.7323260169324));
#147842=CARTESIAN_POINT('Ctrl Pts',(-39.4055862633018,-54.6797418208433,
-64.8099001089221));
#147843=CARTESIAN_POINT('Ctrl Pts',(-39.3594232718812,-54.8861432861055,
-63.9021217828994));
#147844=CARTESIAN_POINT('Ctrl Pts',(-39.336341776171,-54.9893440187367,
-63.4482326198876));
#147845=CARTESIAN_POINT('Ctrl Pts',(-39.3133286552319,-55.1206346051679,
-62.9957806797004));
#147846=CARTESIAN_POINT('Ctrl Pts',(-39.2908828002355,-55.2823630758559,
-62.5545220472777));
#147847=CARTESIAN_POINT('Ctrl Pts',(-39.2684369452391,-55.4440915465439,
-62.113263414855));
#147848=CARTESIAN_POINT('Ctrl Pts',(-39.2465526403215,-55.635643675915,
-61.6830846593873));
#147849=CARTESIAN_POINT('Ctrl Pts',(-39.2253966502057,-55.8655297208508,
-61.2672223984388));
#147850=CARTESIAN_POINT('Origin',(-39.5,-55.08000002,-55.24995));
#147851=CARTESIAN_POINT('',(-39.500000000001,-54.5800000272407,-165.390538702985));
#147852=CARTESIAN_POINT('Origin',(-39.5,-55.08000002,-165.390538702986));
#147853=CARTESIAN_POINT('',(-39.5,-54.58000002,-65.9723506080548));
#147854=CARTESIAN_POINT('Ctrl Pts',(-40.,-56.6722032836053,-171.341255501002));
#147855=CARTESIAN_POINT('Ctrl Pts',(-40.0000000001137,-55.8041715439994,
-171.924697687766));
#147856=CARTESIAN_POINT('Ctrl Pts',(-39.1858850120268,-56.3494037900291,
-171.558563918009));
#147857=CARTESIAN_POINT('Ctrl Pts',(-40.,-56.2965099144784,-170.777391973768));
#147858=CARTESIAN_POINT('Ctrl Pts',(-39.9999999999143,-55.4797123312201,
-171.269409810123));
#147859=CARTESIAN_POINT('Ctrl Pts',(-39.2155551754103,-55.9319856785339,
-170.974971030089));
#147860=CARTESIAN_POINT('Ctrl Pts',(-40.,-56.0109271117334,-170.180744149099));
#147861=CARTESIAN_POINT('Ctrl Pts',(-39.9999999999952,-55.2256104869306,
-170.571031243329));
#147862=CARTESIAN_POINT('Ctrl Pts',(-39.2469773767058,-55.6146249695499,
-170.357118875318));
#147863=CARTESIAN_POINT('Ctrl Pts',(-40.,-55.6233617621208,-169.121472747772));
#147864=CARTESIAN_POINT('Ctrl Pts',(-40.0000000000031,-54.9053220020434,
-169.365642604229));
#147865=CARTESIAN_POINT('Ctrl Pts',(-39.3027883964039,-55.1839423830242,
-169.259798402231));
#147866=CARTESIAN_POINT('Ctrl Pts',(-40.,-55.4926189390281,-168.669060842998));
#147867=CARTESIAN_POINT('Ctrl Pts',(-39.9999999999966,-54.8025817540441,
-168.87099339974));
#147868=CARTESIAN_POINT('Ctrl Pts',(-39.3266337428489,-55.0386476654379,
-168.790991740383));
#147869=CARTESIAN_POINT('Ctrl Pts',(-40.,-55.2841712278759,-167.745175405929));
#147870=CARTESIAN_POINT('Ctrl Pts',(-40.0000000000032,-54.652921563694,
-167.876994762206));
#147871=CARTESIAN_POINT('Ctrl Pts',(-39.3753411897441,-54.8069842833506,
-167.833305054064));
#147872=CARTESIAN_POINT('Ctrl Pts',(-40.,-55.2073915453443,-167.276463616742));
#147873=CARTESIAN_POINT('Ctrl Pts',(-39.9999999999983,-54.6026909074407,
-167.378313758009));
#147874=CARTESIAN_POINT('Ctrl Pts',(-39.4000576364837,-54.7216476273791,
-167.347287707124));
#147875=CARTESIAN_POINT('Ctrl Pts',(-40.,-55.0850969980186,-166.149497422722));
#147876=CARTESIAN_POINT('Ctrl Pts',(-40.0000000000022,-54.5458436605536,
-166.205385693978));
#147877=CARTESIAN_POINT('Ctrl Pts',(-39.4594926871994,-54.5856996258501,
-166.178289848186));
#147878=CARTESIAN_POINT('Ctrl Pts',(-40.,-55.0636927642167,-165.48708770397));
#147879=CARTESIAN_POINT('Ctrl Pts',(-39.9999999999982,-54.5563796453996,
-165.512919816513));
#147880=CARTESIAN_POINT('Ctrl Pts',(-39.4944321648363,-54.5618858497227,
-165.490853406471));
#147881=CARTESIAN_POINT('Ctrl Pts',(-40.,-55.0922303077977,-164.819732953691));
#147882=CARTESIAN_POINT('Ctrl Pts',(-40.000000000001,-54.6215232574257,
-164.799179282796));
#147883=CARTESIAN_POINT('Ctrl Pts',(-39.5296265256636,-54.5935615132292,
-164.79794189457));
#147884=CARTESIAN_POINT('',(-39.2122208635193,-56.0150383143298,-171.050417704751));
#147885=CARTESIAN_POINT('Origin',(-39.5,-56.3715344108516,-170.85018387548));
#147886=CARTESIAN_POINT('Ctrl Pts',(-39.2122209299349,-56.0150383965967,
-171.050417658543));
#147887=CARTESIAN_POINT('Ctrl Pts',(-39.2176920240228,-55.9502202919629,
-170.942877531713));
#147888=CARTESIAN_POINT('Ctrl Pts',(-39.223270534427,-55.8882949524817,
-170.834314512742));
#147889=CARTESIAN_POINT('Ctrl Pts',(-39.2288829748732,-55.8290588250374,
-170.724845259101));
#147890=CARTESIAN_POINT('Ctrl Pts',(-39.2343962193041,-55.7708696553047,
-170.617310799043));
#147891=CARTESIAN_POINT('Ctrl Pts',(-39.2399426498585,-55.7152747925546,
-170.508901566233));
#147892=CARTESIAN_POINT('Ctrl Pts',(-39.2454989375751,-55.6620831693815,
-170.399696352995));
#147893=CARTESIAN_POINT('Ctrl Pts',(-39.2512051809869,-55.6074559857685,
-170.287543858313));
#147894=CARTESIAN_POINT('Ctrl Pts',(-39.2569220065517,-55.5553628501384,
-170.174551727666));
#147895=CARTESIAN_POINT('Ctrl Pts',(-39.2626691268043,-55.5056090682723,
-170.060774196067));
#147896=CARTESIAN_POINT('Ctrl Pts',(-39.2684162470568,-55.4558552864062,
-169.946996664467));
#147897=CARTESIAN_POINT('Ctrl Pts',(-39.2741940917426,-55.4084403442429,
-169.832433450238));
#147898=CARTESIAN_POINT('Ctrl Pts',(-39.2800617718131,-55.3631904849041,
-169.717111289443));
#147899=CARTESIAN_POINT('Ctrl Pts',(-39.2871522937894,-55.3085104208571,
-169.577755648775));
#147900=CARTESIAN_POINT('Ctrl Pts',(-39.294325000306,-55.2570245901798,
-169.437305122195));
#147901=CARTESIAN_POINT('Ctrl Pts',(-39.3015373451061,-55.2085712742073,
-169.295831576444));
#147902=CARTESIAN_POINT('Ctrl Pts',(-39.3088735883845,-55.1592855947966,
-169.151927703592));
#147903=CARTESIAN_POINT('Ctrl Pts',(-39.3162513066387,-55.1131368408751,
-169.006965058834));
#147904=CARTESIAN_POINT('Ctrl Pts',(-39.3236655900776,-55.0699792255175,
-168.860991534233));
#147905=CARTESIAN_POINT('Ctrl Pts',(-39.3312378630505,-55.0259019728685,
-168.711907487985));
#147906=CARTESIAN_POINT('Ctrl Pts',(-39.338848831729,-54.9849440780085,
-168.561768651607));
#147907=CARTESIAN_POINT('Ctrl Pts',(-39.3465267116663,-54.9469854226183,
-168.410602488952));
#147908=CARTESIAN_POINT('Ctrl Pts',(-39.3481905542304,-54.9387595546668,
-168.377843876194));
#147909=CARTESIAN_POINT('Ctrl Pts',(-39.3498576428533,-54.9306746831772,
-168.345036944899));
#147910=CARTESIAN_POINT('Ctrl Pts',(-39.3515284245708,-54.9227298376717,
-168.312181860565));
#147911=CARTESIAN_POINT('Ctrl Pts',(-39.3614981829113,-54.8753219752868,
-168.116131564091));
#147912=CARTESIAN_POINT('Ctrl Pts',(-39.3715435135549,-54.8330294768335,
-167.918870234154));
#147913=CARTESIAN_POINT('Ctrl Pts',(-39.3816147897886,-54.7957193986694,
-167.72083429289));
#147914=CARTESIAN_POINT('Ctrl Pts',(-39.3923369317758,-54.755998121411,
-167.510000091592));
#147915=CARTESIAN_POINT('Ctrl Pts',(-39.4030889139488,-54.7219231119699,
-167.298287584114));
#147916=CARTESIAN_POINT('Ctrl Pts',(-39.4138599647255,-54.6933495306438,
-167.086193912557));
#147917=CARTESIAN_POINT('Ctrl Pts',(-39.4176831357619,-54.6832073735972,
-167.010911528422));
#147918=CARTESIAN_POINT('Ctrl Pts',(-39.4215091024699,-54.6737585376848,
-166.935580892192));
#147919=CARTESIAN_POINT('Ctrl Pts',(-39.4253385442059,-54.6649972877646,
-166.860223572993));
#147920=CARTESIAN_POINT('Ctrl Pts',(-39.4341538597949,-54.6448290260898,
-166.686752190876));
#147921=CARTESIAN_POINT('Ctrl Pts',(-39.4429806358386,-54.6282782237945,
-166.51292724887));
#147922=CARTESIAN_POINT('Ctrl Pts',(-39.4518268440872,-54.6152997906991,
-166.338743654899));
#147923=CARTESIAN_POINT('Ctrl Pts',(-39.4606992732954,-54.6022828883569,
-166.164043765037));
#147924=CARTESIAN_POINT('Ctrl Pts',(-39.4695921259226,-54.5928597871802,
-165.98898246163));
#147925=CARTESIAN_POINT('Ctrl Pts',(-39.4785063203304,-54.5870365021765,
-165.813559429325));
#147926=CARTESIAN_POINT('Ctrl Pts',(-39.485659909963,-54.5823633495253,
-165.672783457004));
#147927=CARTESIAN_POINT('Ctrl Pts',(-39.4928272584983,-54.5800095666538,
-165.531774511173));
#147928=CARTESIAN_POINT('Ctrl Pts',(-39.5000000000025,-54.5800000489627,
-165.390538702984));
#147929=CARTESIAN_POINT('Ctrl Pts',(-39.2122207971108,-56.0150382320575,
-171.05041775096));
#147930=CARTESIAN_POINT('Ctrl Pts',(-39.9999999999999,-55.5316163075193,
-171.321942247435));
#147931=CARTESIAN_POINT('Ctrl Pts',(-40.,-56.3715344108516,-170.85018387548));
#147932=CARTESIAN_POINT('Ctrl Pts',(-39.2305303132587,-56.0826793050571,
-171.197160563313));
#147933=CARTESIAN_POINT('Ctrl Pts',(-40.0000000000016,-55.7019737694774,
-171.520946951432));
#147934=CARTESIAN_POINT('Ctrl Pts',(-40.,-56.4127345596313,-170.923536275602));
#147935=CARTESIAN_POINT('Ctrl Pts',(-39.2581734308863,-56.1834313742016,
-171.318842218969));
#147936=CARTESIAN_POINT('Ctrl Pts',(-40.0000000000015,-55.9148019306841,
-171.629811017638));
#147937=CARTESIAN_POINT('Ctrl Pts',(-40.,-56.4743979142815,-170.984396086855));
#147938=CARTESIAN_POINT('Ctrl Pts',(-39.3228477027581,-56.4100322256565,
-171.502227500722));
#147939=CARTESIAN_POINT('Ctrl Pts',(-39.9999999999985,-56.2996107654989,
-171.733927689933));
#147940=CARTESIAN_POINT('Ctrl Pts',(-40.,-56.6150166715838,-171.07608877299));
#147941=CARTESIAN_POINT('Ctrl Pts',(-39.3604560080182,-56.5377771955238,
-171.565812105304));
#147942=CARTESIAN_POINT('Ctrl Pts',(-39.9999999999952,-56.4773256662664,
-171.740119136472));
#147943=CARTESIAN_POINT('Ctrl Pts',(-40.,-56.6951614830789,-171.107874245193));
#147944=CARTESIAN_POINT('Ctrl Pts',(-39.399271366643,-56.6641713142699,
-171.60362375617));
#147945=CARTESIAN_POINT('Ctrl Pts',(-40.,-56.6359876224367,-171.723920704753));
#147946=CARTESIAN_POINT('Ctrl Pts',(-40.,-56.7758867300388,-171.126786878085));
#147947=CARTESIAN_POINT('',(-39.3992713666431,-56.66417131427,-171.60362375617));
#147948=CARTESIAN_POINT('Origin',(-39.5,-56.7758867300388,-171.126786878085));
#147949=CARTESIAN_POINT('Ctrl Pts',(-39.3992713666431,-56.66417131427,-171.60362375617));
#147950=CARTESIAN_POINT('Ctrl Pts',(-39.3604560080182,-56.5377771955238,
-171.565812105304));
#147951=CARTESIAN_POINT('Ctrl Pts',(-39.3228477027581,-56.4100322256565,
-171.502227500722));
#147952=CARTESIAN_POINT('Ctrl Pts',(-39.2581734308863,-56.1834313742016,
-171.318842218969));
#147953=CARTESIAN_POINT('Ctrl Pts',(-39.2305303132587,-56.0826793050571,
-171.197160563313));
#147954=CARTESIAN_POINT('Ctrl Pts',(-39.2122207971107,-56.0150382320571,
-171.050417750959));
#147955=CARTESIAN_POINT('Ctrl Pts',(-40.,-56.978215522411,-171.14995));
#147956=CARTESIAN_POINT('Ctrl Pts',(-40.,-56.9782155224109,-171.64995));
#147957=CARTESIAN_POINT('Ctrl Pts',(-39.5,-56.978215522411,-171.64995));
#147958=CARTESIAN_POINT('Ctrl Pts',(-40.,-56.9099188320733,-171.149949989769));
#147959=CARTESIAN_POINT('Ctrl Pts',(-40.000000000001,-56.8683451300554,
-171.685098426659));
#147960=CARTESIAN_POINT('Ctrl Pts',(-39.4660557514084,-56.8721092179034,
-171.64995));
#147961=CARTESIAN_POINT('Ctrl Pts',(-40.,-56.8423993478631,-171.142369716128));
#147962=CARTESIAN_POINT('Ctrl Pts',(-40.0000000000047,-56.7549311731639,
-171.710009011284));
#147963=CARTESIAN_POINT('Ctrl Pts',(-39.4324273161011,-56.7672721138937,
-171.634782634301));
#147964=CARTESIAN_POINT('Ctrl Pts',(-40.,-56.7758867300387,-171.126786878085));
#147965=CARTESIAN_POINT('Ctrl Pts',(-40.,-56.6359876224365,-171.723920704752));
#147966=CARTESIAN_POINT('Ctrl Pts',(-39.399271366643,-56.6641713142698,
-171.60362375617));
#147967=CARTESIAN_POINT('',(-39.5,-56.978215522411,-171.64995));
#147968=CARTESIAN_POINT('Origin',(-39.5,-56.978215522411,-171.14995));
#147969=CARTESIAN_POINT('Origin',(-39.9792151682723,-58.6764055302657,-160.124501606025));
#147970=CARTESIAN_POINT('Origin',(-39.5,67.7009572055632,-171.14995));
#147971=CARTESIAN_POINT('',(-39.5,-56.5665827677457,-171.64995));
#147972=CARTESIAN_POINT('Origin',(3.3975957231091E-14,-70.08000002,-58.24995));
#147973=CARTESIAN_POINT('',(-41.,-73.08000002,-58.24995));
#147974=CARTESIAN_POINT('',(41.5,-73.0800000199999,-58.24995));
#147975=CARTESIAN_POINT('Origin',(-41.,-70.08000002,-58.24995));
#147976=CARTESIAN_POINT('Origin',(-41.,-70.08000002,-58.24995));
#147977=CARTESIAN_POINT('Origin',(-41.,-72.58000002,-58.24995));
#147978=CARTESIAN_POINT('Origin',(-42.,-73.08000002,-171.14995));
#147979=CARTESIAN_POINT('Origin',(-42.,-55.58000002,-171.14995));
#147980=CARTESIAN_POINT('Origin',(-42.5,-55.58000002,-177.34995));
#147981=CARTESIAN_POINT('Origin',(-42.5,-55.58000002,-61.14995));
#147982=CARTESIAN_POINT('Origin',(-42.5,-55.58000002,-171.14995));
#147983=CARTESIAN_POINT('Origin',(-42.,-12.9675000200281,-61.14995));
#147984=CARTESIAN_POINT('Origin',(-42.,-56.3473237326805,-61.14995));
#147985=CARTESIAN_POINT('',(-42.,-55.58000002,-60.64995));
#147986=CARTESIAN_POINT('',(-42.,-12.9675000200281,-60.64995));
#147987=CARTESIAN_POINT('Origin',(-42.,-55.58000002,-61.14995));
#147988=CARTESIAN_POINT('Ctrl Pts',(-41.5,-58.6035812240174,-61.14995));
#147989=CARTESIAN_POINT('Ctrl Pts',(-41.5,-58.6035812240174,-60.6498882197787));
#147990=CARTESIAN_POINT('Ctrl Pts',(-42.0000617764046,-58.6035812240174,
-60.6499500038163));
#147991=CARTESIAN_POINT('Ctrl Pts',(-41.5,-58.4156885491981,-61.1499499554112));
#147992=CARTESIAN_POINT('Ctrl Pts',(-41.4999999999964,-58.4568531764755,
-60.7159032420905));
#147993=CARTESIAN_POINT('Ctrl Pts',(-41.9298643117028,-58.4475344566847,
-60.6499412757882));
#147994=CARTESIAN_POINT('Ctrl Pts',(-41.5,-58.2277855029442,-61.1325395579243));
#147995=CARTESIAN_POINT('Ctrl Pts',(-41.5000000000007,-58.2676804549562,
-60.7523419094271));
#147996=CARTESIAN_POINT('Ctrl Pts',(-41.8681695534325,-58.2705723212611,
-60.6499357694868));
#147997=CARTESIAN_POINT('Ctrl Pts',(-41.5,-57.8520667952968,-61.1008454187365));
#147998=CARTESIAN_POINT('Ctrl Pts',(-41.4999999999994,-57.8827900893775,
-60.7882832533183));
#147999=CARTESIAN_POINT('Ctrl Pts',(-41.7820591277972,-57.8880263314595,
-60.6499295039941));
#148000=CARTESIAN_POINT('Ctrl Pts',(-41.5,-57.6641810084401,-61.0874868365943));
#148001=CARTESIAN_POINT('Ctrl Pts',(-41.5000000000007,-57.6764631965609,
-60.7926167355675));
#148002=CARTESIAN_POINT('Ctrl Pts',(-41.7580490411453,-57.6823964313119,
-60.6499285241464));
#148003=CARTESIAN_POINT('Ctrl Pts',(-41.5,-57.2881262594113,-61.0874286718719));
#148004=CARTESIAN_POINT('Ctrl Pts',(-41.4999999999994,-57.2759508310879,
-60.7926435723737));
#148005=CARTESIAN_POINT('Ctrl Pts',(-41.7579337455089,-57.270046180586,
-60.6499285183491));
#148006=CARTESIAN_POINT('Ctrl Pts',(-41.5,-57.0999570266671,-61.1007545617424));
#148007=CARTESIAN_POINT('Ctrl Pts',(-41.5,-57.0692704467339,-60.7883470172518));
#148008=CARTESIAN_POINT('Ctrl Pts',(-41.7818539242553,-57.0640562802561,
-60.6499294916166));
#148009=CARTESIAN_POINT('Ctrl Pts',(-41.5,-56.7235644715484,-61.1324985063765));
#148010=CARTESIAN_POINT('Ctrl Pts',(-41.5,-56.6836417097814,-60.7524277281085));
#148011=CARTESIAN_POINT('Ctrl Pts',(-41.8680165447744,-56.6807474451004,
-60.6499357558287));
#148012=CARTESIAN_POINT('Ctrl Pts',(-41.5,-56.5353526996978,-61.1499499536044));
#148013=CARTESIAN_POINT('Ctrl Pts',(-41.5000000000006,-56.4941497059427,
-60.7159472955962));
#148014=CARTESIAN_POINT('Ctrl Pts',(-41.9298158029953,-56.5034783375499,
-60.6499412695178));
#148015=CARTESIAN_POINT('Ctrl Pts',(-41.5,-56.3473237326805,-61.14995));
#148016=CARTESIAN_POINT('Ctrl Pts',(-41.5,-56.3473237326805,-60.6498882197787));
#148017=CARTESIAN_POINT('Ctrl Pts',(-42.0000617764046,-56.3473237326805,
-60.6499500038163));
#148018=CARTESIAN_POINT('Origin',(-41.,-72.58000002,-4.66002702801304E-15));
#148019=CARTESIAN_POINT('',(-41.,-73.08000002,-174.34995));
#148020=CARTESIAN_POINT('Origin',(-41.,-72.58000002,-174.34995));
#148021=CARTESIAN_POINT('',(-41.,-73.08000002,-58.24995));
#148022=CARTESIAN_POINT('Origin',(-41.,-70.08000002,-174.34995));
#148023=CARTESIAN_POINT('',(-41.,-70.08000002,-177.34995));
#148024=CARTESIAN_POINT('Origin',(-41.,-70.08000002,-176.84995));
#148025=CARTESIAN_POINT('Origin',(-41.,-70.08000002,-174.34995));
#148026=CARTESIAN_POINT('Origin',(-41.,-73.08000002,-176.84995));
#148027=CARTESIAN_POINT('',(-41.,-63.9173163021373,-177.34995));
#148028=CARTESIAN_POINT('',(-41.,-73.08000002,-177.34995));
#148029=CARTESIAN_POINT('Ctrl Pts',(-41.,-63.9173163021373,-177.34995));
#148030=CARTESIAN_POINT('Ctrl Pts',(-41.1312673457634,-63.8804194574513,
-177.34995));
#148031=CARTESIAN_POINT('Ctrl Pts',(-41.2609933446562,-63.8439558571173,
-177.296063436531));
#148032=CARTESIAN_POINT('Ctrl Pts',(-41.4461134365302,-63.7919219926539,
-177.110943344657));
#148033=CARTESIAN_POINT('Ctrl Pts',(-41.5,-63.7767754674458,-176.981217345763));
#148034=CARTESIAN_POINT('Ctrl Pts',(-41.5,-63.7767754674349,-176.84995));
#148035=CARTESIAN_POINT('Origin',(-42.,-63.7767754674349,-171.64995));
#148036=CARTESIAN_POINT('Origin',(-42.,-63.7767754674349,-176.84995));
#148037=CARTESIAN_POINT('Origin',(-42.,-63.7767754674349,-172.64995));
#148038=CARTESIAN_POINT('Ctrl Pts',(-41.9304134495199,-63.2816414330641,
-172.64995));
#148039=CARTESIAN_POINT('Ctrl Pts',(-41.5,-63.3421320985268,-172.64995));
#148040=CARTESIAN_POINT('Ctrl Pts',(-41.5,-63.7767754674349,-172.64995));
#148041=CARTESIAN_POINT('Ctrl Pts',(-41.9304134495211,-63.2816414330639,
-172.51902671195));
#148042=CARTESIAN_POINT('Ctrl Pts',(-41.5,-63.3421320985213,-172.511015867074));
#148043=CARTESIAN_POINT('Ctrl Pts',(-41.5,-63.7767754674226,-172.453565067926));
#148044=CARTESIAN_POINT('Ctrl Pts',(-41.9322246014262,-63.2551037797886,
-172.38820210671));
#148045=CARTESIAN_POINT('Ctrl Pts',(-41.4999999999999,-63.3123764134035,
-172.371853931892));
#148046=CARTESIAN_POINT('Ctrl Pts',(-41.5,-63.7373507987217,-172.257328160063));
#148047=CARTESIAN_POINT('Ctrl Pts',(-41.9391962191206,-63.152953113962,
-172.14633102856));
#148048=CARTESIAN_POINT('Ctrl Pts',(-41.5,-63.1995654042688,-172.118296873734));
#148049=CARTESIAN_POINT('Ctrl Pts',(-41.5,-63.5855944954388,-171.894521542842));
#148050=CARTESIAN_POINT('Ctrl Pts',(-41.9443539433762,-63.0773802713291,
-172.035403273235));
#148051=CARTESIAN_POINT('Ctrl Pts',(-41.500000000002,-63.1159963120049,
-172.003556970023));
#148052=CARTESIAN_POINT('Ctrl Pts',(-41.5,-63.4733225377971,-171.728129909852));
#148053=CARTESIAN_POINT('Ctrl Pts',(-41.9572358131761,-62.8886304524563,
-171.850283164391));
#148054=CARTESIAN_POINT('Ctrl Pts',(-41.499999999998,-62.9115510926292,
-171.817687494207));
#148055=CARTESIAN_POINT('Ctrl Pts',(-41.5,-63.192913452588,-171.450449746589));
#148056=CARTESIAN_POINT('Ctrl Pts',(-41.9649548930126,-62.7755277007723,
-171.776163607997));
#148057=CARTESIAN_POINT('Ctrl Pts',(-41.4999999999999,-62.7899873764732,
-171.746711574348));
#148058=CARTESIAN_POINT('Ctrl Pts',(-41.5,-63.0248865939453,-171.339270411997));
#148059=CARTESIAN_POINT('Ctrl Pts',(-41.981785867019,-62.528914177679,-171.675977326981));
#148060=CARTESIAN_POINT('Ctrl Pts',(-41.5,-62.5315521155723,-171.658003579003));
#148061=CARTESIAN_POINT('Ctrl Pts',(-41.5,-62.6585144680136,-171.18899099047));
#148062=CARTESIAN_POINT('Ctrl Pts',(-41.9908895000012,-62.3955244521823,
-171.64995));
#148063=CARTESIAN_POINT('Ctrl Pts',(-41.4999999999999,-62.3942825374201,
-171.640924254979));
#148064=CARTESIAN_POINT('Ctrl Pts',(-41.5,-62.4603490280314,-171.149950000016));
#148065=CARTESIAN_POINT('Ctrl Pts',(-42.,-62.2620341086569,-171.64995));
#148066=CARTESIAN_POINT('Ctrl Pts',(-41.4999999999999,-62.2620341086569,
-171.64995));
#148067=CARTESIAN_POINT('Ctrl Pts',(-41.5,-62.2620341086569,-171.14995));
#148068=CARTESIAN_POINT('Origin',(-42.,-62.2620341086569,-171.14995));
#148069=CARTESIAN_POINT('Ctrl Pts',(-42.,-62.2620341086569,-171.64995));
#148070=CARTESIAN_POINT('Ctrl Pts',(-41.9908895000012,-62.3955244521823,
-171.64995));
#148071=CARTESIAN_POINT('Ctrl Pts',(-41.981785867019,-62.528914177679,-171.675977326981));
#148072=CARTESIAN_POINT('Ctrl Pts',(-41.9649548930126,-62.7755277007723,
-171.776163607997));
#148073=CARTESIAN_POINT('Ctrl Pts',(-41.9572358131761,-62.8886304524563,
-171.850283164391));
#148074=CARTESIAN_POINT('Ctrl Pts',(-41.9443539433762,-63.0773802713291,
-172.035403273235));
#148075=CARTESIAN_POINT('Ctrl Pts',(-41.9391962191206,-63.152953113962,
-172.14633102856));
#148076=CARTESIAN_POINT('Ctrl Pts',(-41.9322246014262,-63.2551037797886,
-172.38820210671));
#148077=CARTESIAN_POINT('Ctrl Pts',(-41.9304134495211,-63.2816414330639,
-172.51902671195));
#148078=CARTESIAN_POINT('Ctrl Pts',(-41.9304134495199,-63.2816414330641,
-172.64995));
#148079=CARTESIAN_POINT('Origin',(-42.,-73.08000002,-171.14995));
#148080=CARTESIAN_POINT('Ctrl Pts',(-25.2,-65.7473676730093,-61.2659196908482));
#148081=CARTESIAN_POINT('Ctrl Pts',(-25.2,-65.5225267460558,-60.9659777046635));
#148082=CARTESIAN_POINT('Ctrl Pts',(-25.5598256882329,-65.4594929016704,
-60.8818893816965));
#148083=CARTESIAN_POINT('Ctrl Pts',(-25.2,-65.68613088204,-61.3118237091767));
#148084=CARTESIAN_POINT('Ctrl Pts',(-25.1999999999999,-65.4328856316129,
-61.057360567634));
#148085=CARTESIAN_POINT('Ctrl Pts',(-25.5355900377414,-65.3488148482479,
-60.9737014968053));
#148086=CARTESIAN_POINT('Ctrl Pts',(-25.2,-65.635123981304,-61.3698711298632));
#148087=CARTESIAN_POINT('Ctrl Pts',(-25.2,-65.3589455123936,-61.1652193216821));
#148088=CARTESIAN_POINT('Ctrl Pts',(-25.5153438106255,-65.2566822918862,
-61.0897986661581));
#148089=CARTESIAN_POINT('Ctrl Pts',(-25.2,-65.5994372375941,-61.4386408691297));
#148090=CARTESIAN_POINT('Ctrl Pts',(-25.2,-65.3080942147004,-61.2874541854323));
#148091=CARTESIAN_POINT('Ctrl Pts',(-25.5011648721215,-65.1922357602732,
-61.2273317382593));
#148092=CARTESIAN_POINT('Origin',(-25.7,-65.5994372375942,-61.4386408691297));
#148093=CARTESIAN_POINT('Ctrl Pts',(-25.5486065204957,-65.6266003779639,
-171.854014632591));
#148094=CARTESIAN_POINT('Ctrl Pts',(-25.1999999999999,-65.7373527968364,
-171.85401463259));
#148095=CARTESIAN_POINT('Ctrl Pts',(-25.2,-66.1031295107182,-171.854014632589));
#148096=CARTESIAN_POINT('Ctrl Pts',(-25.5332781069629,-65.6314702205409,
-171.740892625582));
#148097=CARTESIAN_POINT('Ctrl Pts',(-25.2,-65.7495636563843,-171.730197187823));
#148098=CARTESIAN_POINT('Ctrl Pts',(-25.2,-66.1031295051642,-171.688945996574));
#148099=CARTESIAN_POINT('Ctrl Pts',(-25.5254918386358,-65.6165368852731,
-171.632443841085));
#148100=CARTESIAN_POINT('Ctrl Pts',(-25.2,-65.7357529125625,-171.605967390697));
#148101=CARTESIAN_POINT('Ctrl Pts',(-25.2,-66.0766766441701,-171.528325399449));
#148102=CARTESIAN_POINT('Ctrl Pts',(-25.5190396326646,-65.5455021430107,
-171.42367336987));
#148103=CARTESIAN_POINT('Ctrl Pts',(-25.1999999999999,-65.6576340206492,
-171.369178819378));
#148104=CARTESIAN_POINT('Ctrl Pts',(-25.2,-65.9668265905144,-171.216885108557));
#148105=CARTESIAN_POINT('Ctrl Pts',(-25.5204167023824,-65.4915081760158,
-171.329224126564));
#148106=CARTESIAN_POINT('Ctrl Pts',(-25.2,-65.5955175213768,-171.261530708485));
#148107=CARTESIAN_POINT('Ctrl Pts',(-25.2,-65.8865499901975,-171.074857506769));
#148108=CARTESIAN_POINT('Ctrl Pts',(-25.5241645957028,-65.4203114663335,
-171.244965273984));
#148109=CARTESIAN_POINT('Ctrl Pts',(-25.1999999999999,-65.5143246899125,
-171.167561256232));
#148110=CARTESIAN_POINT('Ctrl Pts',(-25.2,-65.7816577220592,-170.947457636992));
#148111=CARTESIAN_POINT('Origin',(-25.7,-65.7816577220592,-170.947457636992));
#148112=CARTESIAN_POINT('Ctrl Pts',(-25.2,-65.7246041881209,-170.861259130871));
#148113=CARTESIAN_POINT('Ctrl Pts',(-25.2,-65.4329690822618,-171.012528323755));
#148114=CARTESIAN_POINT('Ctrl Pts',(-25.5015460489969,-65.3172168042439,
-171.07256826174));
#148115=CARTESIAN_POINT('Ctrl Pts',(-25.2,-65.7405566104338,-170.892014084856));
#148116=CARTESIAN_POINT('Ctrl Pts',(-25.2,-65.4555942264487,-171.066917428723));
#148117=CARTESIAN_POINT('Ctrl Pts',(-25.5078751098564,-65.3460382794916,
-171.13407782586));
#148118=CARTESIAN_POINT('Ctrl Pts',(-25.2,-65.7596409576893,-170.920716557309));
#148119=CARTESIAN_POINT('Ctrl Pts',(-25.1999999999994,-65.4828113676634,
-171.118510663779));
#148120=CARTESIAN_POINT('Ctrl Pts',(-25.5154426820321,-65.380521047679,
-171.191481806562));
#148121=CARTESIAN_POINT('Ctrl Pts',(-25.2,-65.7816577220592,-170.947457636992));
#148122=CARTESIAN_POINT('Ctrl Pts',(-25.2,-65.5143246899125,-171.167561256232));
#148123=CARTESIAN_POINT('Ctrl Pts',(-25.5241645957028,-65.4203114663335,
-171.244965273984));
#148124=CARTESIAN_POINT('',(-25.5015460489969,-65.317216804244,-171.07256826174));
#148125=CARTESIAN_POINT('Origin',(-25.7,-65.7246041881209,-170.861259130871));
#148126=CARTESIAN_POINT('Origin',(-25.6922800193975,-66.1910492956378,-170.643493704359));
#148127=CARTESIAN_POINT('Ctrl Pts',(-25.5015460489969,-65.317216804244,
-171.07256826174));
#148128=CARTESIAN_POINT('Ctrl Pts',(-25.2,-65.4329690822618,-171.012528323755));
#148129=CARTESIAN_POINT('Ctrl Pts',(-25.2,-65.7246041881209,-170.861259130871));
#148130=CARTESIAN_POINT('Ctrl Pts',(-25.4919266567716,-62.1578398412392,
-164.972503788787));
#148131=CARTESIAN_POINT('Ctrl Pts',(-25.1999999998579,-62.297876586317,
-164.952133926682));
#148132=CARTESIAN_POINT('Ctrl Pts',(-25.2,-62.5605386715726,-164.761189683274));
#148133=CARTESIAN_POINT('Ctrl Pts',(-25.4809754250192,-58.9585757861229,
-158.893982149016));
#148134=CARTESIAN_POINT('Ctrl Pts',(-25.2,-59.109002613422,-158.883754709366));
#148135=CARTESIAN_POINT('Ctrl Pts',(-25.2,-59.3555677916457,-158.682664145768));
#148136=CARTESIAN_POINT('Ctrl Pts',(-25.4679548160676,-55.6876551762764,
-152.854600597735));
#148137=CARTESIAN_POINT('Ctrl Pts',(-25.2,-55.8110355215084,-152.787619396006));
#148138=CARTESIAN_POINT('Ctrl Pts',(-25.2,-56.0768896606488,-152.643291466864));
#148139=CARTESIAN_POINT('',(-25.4679548160676,-55.6876551762764,-152.854600597735));
#148140=CARTESIAN_POINT('Origin',(-25.7,-56.0768896606488,-152.643291466864));
#148141=CARTESIAN_POINT('Ctrl Pts',(-25.4679548160676,-55.6876551762764,
-152.854600597735));
#148142=CARTESIAN_POINT('Ctrl Pts',(-25.4809753053448,-58.9585758501934,
-158.89398214466));
#148143=CARTESIAN_POINT('Ctrl Pts',(-25.4919265333855,-62.1578399004274,
-164.972503780177));
#148144=CARTESIAN_POINT('Ctrl Pts',(-25.5015460489969,-65.317216804244,
-171.07256826174));
#148145=CARTESIAN_POINT('Ctrl Pts',(-25.2,-55.0810255612707,-148.372593301835));
#148146=CARTESIAN_POINT('Ctrl Pts',(-25.1999999999977,-54.5731343323654,
-148.364947473313));
#148147=CARTESIAN_POINT('Ctrl Pts',(-25.7078909275495,-54.5811410568989,
-148.365051987889));
#148148=CARTESIAN_POINT('Ctrl Pts',(-25.2,-55.0698197461487,-149.14066186414));
#148149=CARTESIAN_POINT('Ctrl Pts',(-25.2000000000109,-54.6032311838736,
-149.141970394971));
#148150=CARTESIAN_POINT('Ctrl Pts',(-25.6652819751675,-54.5686815890185,
-149.174446315097));
#148151=CARTESIAN_POINT('Ctrl Pts',(-25.2,-55.1504277383396,-149.894402552637));
#148152=CARTESIAN_POINT('Ctrl Pts',(-25.1999999999999,-54.719333665426,
-149.93311152841));
#148153=CARTESIAN_POINT('Ctrl Pts',(-25.6231363511229,-54.6582401725082,
-149.967634915182));
#148154=CARTESIAN_POINT('Ctrl Pts',(-25.2,-55.4970587519645,-151.371835493675));
#148155=CARTESIAN_POINT('Ctrl Pts',(-25.2,-55.1489528075744,-151.46123340427));
#148156=CARTESIAN_POINT('Ctrl Pts',(-25.5400582915436,-55.0433748333577,
-151.520527347314));
#148157=CARTESIAN_POINT('Ctrl Pts',(-25.2,-55.7668139911694,-152.10111968119));
#148158=CARTESIAN_POINT('Ctrl Pts',(-25.2,-55.4558433261223,-152.21575400765));
#148159=CARTESIAN_POINT('Ctrl Pts',(-25.4988024926329,-55.3431110792067,
-152.286087899488));
#148160=CARTESIAN_POINT('Ctrl Pts',(-25.2,-56.1447163878713,-152.765324933197));
#148161=CARTESIAN_POINT('Ctrl Pts',(-25.2,-55.886418136883,-152.912368886688));
#148162=CARTESIAN_POINT('Ctrl Pts',(-25.4610913766845,-55.7629867532576,
-152.982594400152));
#148163=CARTESIAN_POINT('',(-25.7,-54.58000002,-148.513004346424));
#148164=CARTESIAN_POINT('Origin',(-25.7,-55.08000002,-148.513004346424));
#148165=CARTESIAN_POINT('Ctrl Pts',(-25.7,-54.58000002,-148.513004346424));
#148166=CARTESIAN_POINT('Ctrl Pts',(-25.6920855143309,-54.5800000317253,
-148.663195106218));
#148167=CARTESIAN_POINT('Ctrl Pts',(-25.6841718538579,-54.5836287914609,
-148.812839156877));
#148168=CARTESIAN_POINT('Ctrl Pts',(-25.6762813054516,-54.5907991607014,
-148.961912671116));
#148169=CARTESIAN_POINT('Ctrl Pts',(-25.6682875469831,-54.5980633199066,
-149.112936098834));
#148170=CARTESIAN_POINT('Ctrl Pts',(-25.660316862259,-54.6089618260389,
-149.263374635832));
#148171=CARTESIAN_POINT('Ctrl Pts',(-25.6523724200598,-54.6234496539193,
-149.413223047264));
#148172=CARTESIAN_POINT('Ctrl Pts',(-25.6444353407179,-54.6379240545753,
-149.562932580165));
#148173=CARTESIAN_POINT('Ctrl Pts',(-25.6365236874188,-54.65598091595,-149.712053836966));
#148174=CARTESIAN_POINT('Ctrl Pts',(-25.6286315318916,-54.6776258877763,
-149.860590148905));
#148175=CARTESIAN_POINT('Ctrl Pts',(-25.6207455186128,-54.6992540139137,
-150.009010859101));
#148176=CARTESIAN_POINT('Ctrl Pts',(-25.6128781619883,-54.7244646682897,
-150.156848301768));
#148177=CARTESIAN_POINT('Ctrl Pts',(-25.6050263127155,-54.7533155629583,
-150.304102915368));
#148178=CARTESIAN_POINT('Ctrl Pts',(-25.5971744634426,-54.7821664576269,
-150.451357528967));
#148179=CARTESIAN_POINT('Ctrl Pts',(-25.5893372800479,-54.814657808455,
-150.598030081328));
#148180=CARTESIAN_POINT('Ctrl Pts',(-25.5815267843809,-54.8508978232776,
-150.744106601026));
#148181=CARTESIAN_POINT('Ctrl Pts',(-25.5733098976718,-54.8890234568904,
-150.897783686886));
#148182=CARTESIAN_POINT('Ctrl Pts',(-25.5651918395491,-54.9313235556008,
-151.050969095924));
#148183=CARTESIAN_POINT('Ctrl Pts',(-25.5571115988274,-54.9779166473137,
-151.203276624969));
#148184=CARTESIAN_POINT('Ctrl Pts',(-25.5493889213721,-55.02244792198,-151.348844308081));
#148185=CARTESIAN_POINT('Ctrl Pts',(-25.5417007566369,-55.0709013570447,
-151.49361015005));
#148186=CARTESIAN_POINT('Ctrl Pts',(-25.534031385493,-55.1233796653412,
-151.637208739292));
#148187=CARTESIAN_POINT('Ctrl Pts',(-25.5265369085761,-55.1746612453797,
-151.777532670965));
#148188=CARTESIAN_POINT('Ctrl Pts',(-25.5190603419181,-55.2297869278435,
-151.916742020613));
#148189=CARTESIAN_POINT('Ctrl Pts',(-25.5116243691151,-55.2888416006855,
-152.054467340709));
#148190=CARTESIAN_POINT('Ctrl Pts',(-25.5042409693129,-55.3474787516445,
-152.191218930323));
#148191=CARTESIAN_POINT('Ctrl Pts',(-25.496897587104,-55.4099903172709,
-152.326507400918));
#148192=CARTESIAN_POINT('Ctrl Pts',(-25.4896541364441,-55.4764373972532,
-152.459942269866));
#148193=CARTESIAN_POINT('Ctrl Pts',(-25.4824106857843,-55.5428844772355,
-152.593377138814));
#148194=CARTESIAN_POINT('Ctrl Pts',(-25.4752672708635,-55.613267946895,
-152.724958308978));
#148195=CARTESIAN_POINT('Ctrl Pts',(-25.468320993909,-55.6876143391068,
-152.85426703406));
#148196=CARTESIAN_POINT('Origin',(-25.7,-55.08000002,-55.24995));
#148197=CARTESIAN_POINT('',(-25.7,-54.58000002,-83.5456386250818));
#148198=CARTESIAN_POINT('Origin',(-25.7,-55.08000002,-83.5456386250819));
#148199=CARTESIAN_POINT('',(-25.7,-54.58000002,-147.999168907581));
#148200=CARTESIAN_POINT('Ctrl Pts',(-25.2,-56.0768896606488,-79.4153515046414));
#148201=CARTESIAN_POINT('Ctrl Pts',(-25.2,-55.8110355215084,-79.2710235754997));
#148202=CARTESIAN_POINT('Ctrl Pts',(-25.4679548160676,-55.6876551762764,
-79.2040423737711));
#148203=CARTESIAN_POINT('Ctrl Pts',(-25.2,-55.7330239637487,-80.0487571235243));
#148204=CARTESIAN_POINT('Ctrl Pts',(-25.2,-55.4183788566373,-79.9347575264689));
#148205=CARTESIAN_POINT('Ctrl Pts',(-25.5038900524126,-55.3056215869824,
-79.8682921770632));
#148206=CARTESIAN_POINT('Ctrl Pts',(-25.2,-55.4909001541243,-80.7176024822967));
#148207=CARTESIAN_POINT('Ctrl Pts',(-25.2000000000012,-55.1418983306402,
-80.6264944503603));
#148208=CARTESIAN_POINT('Ctrl Pts',(-25.541710547536,-55.0365557241775,
-80.5705069627783));
#148209=CARTESIAN_POINT('Ctrl Pts',(-25.2,-55.2446154752418,-81.7605756924265));
#148210=CARTESIAN_POINT('Ctrl Pts',(-25.1999999999993,-54.8419593173495,
-81.6877104640905));
#148211=CARTESIAN_POINT('Ctrl Pts',(-25.6003533292375,-54.7629060815823,
-81.666730198729));
#148212=CARTESIAN_POINT('Ctrl Pts',(-25.2,-55.1827439360829,-82.1162012744658));
#148213=CARTESIAN_POINT('Ctrl Pts',(-25.2,-54.7609521776091,-82.0570705103581));
#148214=CARTESIAN_POINT('Ctrl Pts',(-25.6202954530102,-54.6941599265733,
-82.0407267561828));
#148215=CARTESIAN_POINT('Ctrl Pts',(-25.2,-55.1006621337656,-82.8281867002427));
#148216=CARTESIAN_POINT('Ctrl Pts',(-25.2,-54.6393723317538,-82.7989454077316));
#148217=CARTESIAN_POINT('Ctrl Pts',(-25.6600938511042,-54.6029579243694,
-82.7899562024642));
#148218=CARTESIAN_POINT('Ctrl Pts',(-25.2,-55.0800000206675,-83.1859979964978));
#148219=CARTESIAN_POINT('Ctrl Pts',(-25.2,-54.5995766430915,-83.1741390671131));
#148220=CARTESIAN_POINT('Ctrl Pts',(-25.6800320694526,-54.58000002,-83.1667133317899));
#148221=CARTESIAN_POINT('Ctrl Pts',(-25.2,-55.08000002,-83.5456386250819));
#148222=CARTESIAN_POINT('Ctrl Pts',(-25.2,-54.58000002,-83.5456386250818));
#148223=CARTESIAN_POINT('Ctrl Pts',(-25.7,-54.58000002,-83.5456386250819));
#148224=CARTESIAN_POINT('',(-25.4679548160676,-55.6876551762764,-79.2040423737711));
#148225=CARTESIAN_POINT('Origin',(-25.7,-56.0768896606488,-79.4153515046414));
#148226=CARTESIAN_POINT('Ctrl Pts',(-25.4679630512114,-55.687567629395,
-79.2041945974705));
#148227=CARTESIAN_POINT('Ctrl Pts',(-25.5038958305178,-55.3055804804405,
-79.8683994594255));
#148228=CARTESIAN_POINT('Ctrl Pts',(-25.5417135339568,-55.0365417883965,
-80.5705627886394));
#148229=CARTESIAN_POINT('Ctrl Pts',(-25.6003533292375,-54.7629060815823,
-81.666730198729));
#148230=CARTESIAN_POINT('Ctrl Pts',(-25.6202954530102,-54.6941599265733,
-82.0407267561828));
#148231=CARTESIAN_POINT('Ctrl Pts',(-25.6600938511042,-54.6029579243694,
-82.7899562024642));
#148232=CARTESIAN_POINT('Ctrl Pts',(-25.6800320694526,-54.58000002,-83.1667133317899));
#148233=CARTESIAN_POINT('Ctrl Pts',(-25.7,-54.58000002,-83.5456386250818));
#148234=CARTESIAN_POINT('Ctrl Pts',(-25.4679548160676,-55.6876551762764,
-79.2040423737711));
#148235=CARTESIAN_POINT('Ctrl Pts',(-25.2,-55.8110355215084,-79.2710235754996));
#148236=CARTESIAN_POINT('Ctrl Pts',(-25.2,-56.0768896606488,-79.4153515046414));
#148237=CARTESIAN_POINT('Ctrl Pts',(-25.4808037502955,-58.9154492031739,
-73.2442891352868));
#148238=CARTESIAN_POINT('Ctrl Pts',(-25.2000000000118,-59.0651351497249,
-73.255975182323));
#148239=CARTESIAN_POINT('Ctrl Pts',(-25.2,-59.3123390931711,-73.4556067153995));
#148240=CARTESIAN_POINT('Ctrl Pts',(-25.4916367264251,-62.0734180747052,
-67.2463887183684));
#148241=CARTESIAN_POINT('Ctrl Pts',(-25.200000000035,-62.2130344026582,
-67.2677845851136));
#148242=CARTESIAN_POINT('Ctrl Pts',(-25.2,-62.4759645157842,-67.4577026174502));
#148243=CARTESIAN_POINT('Ctrl Pts',(-25.5011648721215,-65.1922357602732,
-61.2273317382594));
#148244=CARTESIAN_POINT('Ctrl Pts',(-25.1999999999999,-65.3080942147003,
-61.2874541854323));
#148245=CARTESIAN_POINT('Ctrl Pts',(-25.2,-65.5994372375941,-61.4386408691297));
#148246=CARTESIAN_POINT('Ctrl Pts',(-25.5011648721215,-65.1922357602732,
-61.2273317382593));
#148247=CARTESIAN_POINT('Ctrl Pts',(-25.4916365654323,-62.0734181517779,
-67.2463887301796));
#148248=CARTESIAN_POINT('Ctrl Pts',(-25.4808035940994,-58.9154492864362,
-73.2442891417871));
#148249=CARTESIAN_POINT('Ctrl Pts',(-25.4679548160676,-55.6876551762764,
-79.2040423737711));
#148250=CARTESIAN_POINT('Origin',(-24.7,-72.58000002,-55.24995));
#148251=CARTESIAN_POINT('',(-24.7,-73.08000002,-174.34995));
#148252=CARTESIAN_POINT('Origin',(-24.7,-72.58000002,-174.34995));
#148253=CARTESIAN_POINT('',(-24.7,-73.08000002,-58.24995));
#148254=CARTESIAN_POINT('Origin',(-24.7,-70.08000002,-174.34995));
#148255=CARTESIAN_POINT('Origin',(-24.7,-70.08000002,-174.34995));
#148256=CARTESIAN_POINT('Origin',(0.,-12.9675000200281,-60.64995));
#148257=CARTESIAN_POINT('',(-31.0842852491212,-55.9092501930852,-72.1786663403248));
#148258=CARTESIAN_POINT('Ctrl Pts',(-25.4683317116696,-55.6876147551788,
-79.2043632317979));
#148259=CARTESIAN_POINT('Ctrl Pts',(-27.4082623732412,-55.7634597160082,
-76.9351801749559));
#148260=CARTESIAN_POINT('Ctrl Pts',(-29.2789232576535,-55.8380366706268,
-74.5726148012184));
#148261=CARTESIAN_POINT('Ctrl Pts',(-31.0842854210862,-55.9092502160976,
-72.1786665455479));
#148262=CARTESIAN_POINT('Ctrl Pts',(-31.0842850915596,-55.9092502513102,
-72.178666283495));
#148263=CARTESIAN_POINT('Ctrl Pts',(-31.0926997270338,-57.9933062771889,
-68.5477739115119));
#148264=CARTESIAN_POINT('Ctrl Pts',(-31.1003697028526,-60.0396054894506,
-64.8950530444828));
#148265=CARTESIAN_POINT('Ctrl Pts',(-31.1074520910898,-62.0598503138784,
-61.2273317382593));
#148266=CARTESIAN_POINT('Ctrl Pts',(-31.85,-62.4426282692183,-61.4386408691297));
#148267=CARTESIAN_POINT('Ctrl Pts',(-31.8499999999999,-61.6992317916067,
-61.028255523305));
#148268=CARTESIAN_POINT('Ctrl Pts',(-31.1074520910898,-62.0598503138784,
-61.2273317382593));
#148269=CARTESIAN_POINT('Ctrl Pts',(-31.85,-62.4685470764636,-61.3916901534439));
#148270=CARTESIAN_POINT('Ctrl Pts',(-31.8500000000001,-61.7930681218295,
-60.9114185604269));
#148271=CARTESIAN_POINT('Ctrl Pts',(-31.1192593280084,-62.1041984096607,
-61.1334442002736));
#148272=CARTESIAN_POINT('Ctrl Pts',(-31.85,-62.5015432853809,-61.3504740791978));
#148273=CARTESIAN_POINT('Ctrl Pts',(-31.8499999999998,-61.9033127772783,
-60.8239692453656));
#148274=CARTESIAN_POINT('Ctrl Pts',(-31.1342845229578,-62.1606836378221,
-61.0509981549565));
#148275=CARTESIAN_POINT('Ctrl Pts',(-31.85,-62.5794711033445,-61.2778158898142));
#148276=CARTESIAN_POINT('Ctrl Pts',(-31.8500000000002,-62.1341758421231,
-60.6961222616711));
#148277=CARTESIAN_POINT('Ctrl Pts',(-31.1697097530512,-62.2941363459118,
-60.9056817830676));
#148278=CARTESIAN_POINT('Ctrl Pts',(-31.85,-62.6234753527752,-61.2474602210686));
#148279=CARTESIAN_POINT('Ctrl Pts',(-31.8500000000001,-62.2503354665,-60.6558084251244));
#148280=CARTESIAN_POINT('Ctrl Pts',(-31.1896892584046,-62.369523292851,
-60.8449704353912));
#148281=CARTESIAN_POINT('Ctrl Pts',(-31.85,-62.765153261125,-61.1743645550205));
#148282=CARTESIAN_POINT('Ctrl Pts',(-31.8499999999996,-62.5772240699999,
-60.5884818802849));
#148283=CARTESIAN_POINT('Ctrl Pts',(-31.2539016024624,-62.6123775685824,
-60.6987791235328));
#148284=CARTESIAN_POINT('Ctrl Pts',(-31.85,-62.8714721065165,-61.1499500118284));
#148285=CARTESIAN_POINT('Ctrl Pts',(-31.85,-62.7861985042763,-60.599633723582));
#148286=CARTESIAN_POINT('Ctrl Pts',(-31.3019361194217,-62.7947963971694,
-60.64995));
#148287=CARTESIAN_POINT('Ctrl Pts',(-31.85,-62.9782728042642,-61.14995));
#148288=CARTESIAN_POINT('Ctrl Pts',(-31.8499999999999,-62.9782728042642,
-60.64995));
#148289=CARTESIAN_POINT('Ctrl Pts',(-31.35,-62.9782728042642,-60.64995));
#148290=CARTESIAN_POINT('Origin',(-31.35,-62.4426282692182,-61.4386408691297));
#148291=CARTESIAN_POINT('Origin',(-31.35,-62.9782728042642,-61.14995));
#148292=CARTESIAN_POINT('Origin',(-31.35,67.7009572055632,-61.14995));
#148293=CARTESIAN_POINT('Ctrl Pts',(-31.1074520910898,-62.0598503138784,
-61.2273317382593));
#148294=CARTESIAN_POINT('Ctrl Pts',(-31.85,-61.6992317916068,-61.0282555233051));
#148295=CARTESIAN_POINT('Ctrl Pts',(-31.85,-62.4426282692182,-61.4386408691297));
#148296=CARTESIAN_POINT('Ctrl Pts',(-31.1003696873064,-60.0396054978548,
-64.8950530477878));
#148297=CARTESIAN_POINT('Ctrl Pts',(-31.8500000000147,-59.6343590655212,
-64.7356884621635));
#148298=CARTESIAN_POINT('Ctrl Pts',(-31.85,-60.4178950612392,-65.1063632921145));
#148299=CARTESIAN_POINT('Ctrl Pts',(-31.0926997115701,-57.9933062860146,
-68.5477739147732));
#148300=CARTESIAN_POINT('Ctrl Pts',(-31.85,-57.56108933629,-68.3880588333245));
#148301=CARTESIAN_POINT('Ctrl Pts',(-31.85,-58.3664713365843,-68.7590848262753));
#148302=CARTESIAN_POINT('Ctrl Pts',(-31.0842850915597,-55.9092502513102,
-72.178666283495));
#148303=CARTESIAN_POINT('Ctrl Pts',(-31.85,-55.4929314270087,-71.9390096071439));
#148304=CARTESIAN_POINT('Ctrl Pts',(-31.85,-56.2763252281792,-72.3899754143654));
#148305=CARTESIAN_POINT('Origin',(-31.35,-56.2763252281792,-72.3899754143654));
#148306=CARTESIAN_POINT('Ctrl Pts',(-31.85,-55.08000002,-77.227263173365));
#148307=CARTESIAN_POINT('Ctrl Pts',(-31.85,-54.5800000200009,-77.2272631733658));
#148308=CARTESIAN_POINT('Ctrl Pts',(-31.3500000000009,-54.58000002,-77.2272631733658));
#148309=CARTESIAN_POINT('Ctrl Pts',(-31.85,-55.0800000215433,-76.3831770294161));
#148310=CARTESIAN_POINT('Ctrl Pts',(-31.85,-54.5315963664815,-76.3014537863538));
#148311=CARTESIAN_POINT('Ctrl Pts',(-31.3038531467957,-54.5800000199985,
-76.3446192991014));
#148312=CARTESIAN_POINT('Ctrl Pts',(-31.85,-55.1744276549191,-75.5528673220433));
#148313=CARTESIAN_POINT('Ctrl Pts',(-31.85,-54.5888070575115,-75.4165208091089));
#148314=CARTESIAN_POINT('Ctrl Pts',(-31.258313471615,-54.6849196157793,
-75.4773117729577));
#148315=CARTESIAN_POINT('Ctrl Pts',(-31.85,-55.4647382256782,-74.3299545388963));
#148316=CARTESIAN_POINT('Ctrl Pts',(-31.85,-54.7984161464127,-74.129239130374));
#148317=CARTESIAN_POINT('Ctrl Pts',(-31.1911093410829,-55.0074869144856,
-74.2010813719198));
#148318=CARTESIAN_POINT('Ctrl Pts',(-31.85,-55.5878027790484,-73.9239717796963));
#148319=CARTESIAN_POINT('Ctrl Pts',(-31.85,-54.8981200391591,-73.6821630179211));
#148320=CARTESIAN_POINT('Ctrl Pts',(-31.1687759778426,-55.1442253086702,
-73.7776011027959));
#148321=CARTESIAN_POINT('Ctrl Pts',(-31.85,-55.8881616831611,-73.1379857970122));
#148322=CARTESIAN_POINT('Ctrl Pts',(-31.85,-55.1503671712329,-72.798619733739));
#148323=CARTESIAN_POINT('Ctrl Pts',(-31.1255062785665,-55.4779574226737,
-72.9580899132975));
#148324=CARTESIAN_POINT('Ctrl Pts',(-31.85,-56.0652689851553,-72.7566110978467));
#148325=CARTESIAN_POINT('Ctrl Pts',(-31.8500000000028,-55.3074747056296,
-72.358974665281));
#148326=CARTESIAN_POINT('Ctrl Pts',(-31.1044941422599,-55.6747504070549,
-72.5606146570313));
#148327=CARTESIAN_POINT('Ctrl Pts',(-31.85,-56.2763252281792,-72.3899754143654));
#148328=CARTESIAN_POINT('Ctrl Pts',(-31.85,-55.4929314270087,-71.9390096071439));
#148329=CARTESIAN_POINT('Ctrl Pts',(-31.0842850915597,-55.9092502513102,
-72.178666283495));
#148330=CARTESIAN_POINT('',(-31.3499999999941,-54.58000002,-77.227263173365));
#148331=CARTESIAN_POINT('Origin',(-31.35,-55.08000002,-77.2272631733642));
#148332=CARTESIAN_POINT('Ctrl Pts',(-31.3500000000009,-54.58000002,-77.227263173365));
#148333=CARTESIAN_POINT('Ctrl Pts',(-31.3038531467958,-54.5800000199986,
-76.3446192991009));
#148334=CARTESIAN_POINT('Ctrl Pts',(-31.2583134716152,-54.6849196157794,
-75.4773117729574));
#148335=CARTESIAN_POINT('Ctrl Pts',(-31.2135107179272,-54.8999644815834,
-74.6264915055991));
#148336=CARTESIAN_POINT('Ctrl Pts',(-31.1911093410832,-55.0074869144855,
-74.2010813719198));
#148337=CARTESIAN_POINT('Ctrl Pts',(-31.1687759778429,-55.1442253086701,
-73.7776011027959));
#148338=CARTESIAN_POINT('Ctrl Pts',(-31.147141128205,-55.3110913656718,
-73.3678455080466));
#148339=CARTESIAN_POINT('Ctrl Pts',(-31.125506279948,-55.4779574120224,
-72.9580899394523));
#148340=CARTESIAN_POINT('Ctrl Pts',(-31.1044941449429,-55.6747503819319,
-72.5606147077732));
#148341=CARTESIAN_POINT('Ctrl Pts',(-31.0842850954301,-55.9092502064053,
-72.1786663566345));
#148342=CARTESIAN_POINT('Origin',(-31.35,-55.08000002,-55.24995));
#148343=CARTESIAN_POINT('',(-31.3500000000014,-54.5800000295902,-154.831379798157));
#148344=CARTESIAN_POINT('Origin',(-31.35,-55.08000002,-154.831379798159));
#148345=CARTESIAN_POINT('',(-31.35,-54.58000002,-76.6255854122387));
#148346=CARTESIAN_POINT('Ctrl Pts',(-31.85,-56.5198937114388,-160.061984623621));
#148347=CARTESIAN_POINT('Ctrl Pts',(-31.8500000000001,-55.7195063092811,
-160.597458213624));
#148348=CARTESIAN_POINT('Ctrl Pts',(-31.0622729759187,-56.1800587903026,
-160.289522595203));
#148349=CARTESIAN_POINT('Ctrl Pts',(-31.85,-56.196322380357,-159.575614753933));
#148350=CARTESIAN_POINT('Ctrl Pts',(-31.8499999999999,-55.4302476503449,
-160.032901980985));
#148351=CARTESIAN_POINT('Ctrl Pts',(-31.0890805685714,-55.8205456059185,
-159.783030537725));
#148352=CARTESIAN_POINT('Ctrl Pts',(-31.85,-55.9428521111973,-159.062977148996));
#148353=CARTESIAN_POINT('Ctrl Pts',(-31.85,-55.1997164518874,-159.434441959105));
#148354=CARTESIAN_POINT('Ctrl Pts',(-31.1173271740076,-55.5388836657292,
-159.248854752969));
#148355=CARTESIAN_POINT('Ctrl Pts',(-31.85,-55.5903137943537,-158.141820520556));
#148356=CARTESIAN_POINT('Ctrl Pts',(-31.8499999999999,-54.8995758370652,
-158.384410590095));
#148357=CARTESIAN_POINT('Ctrl Pts',(-31.1680335221376,-55.1471418726124,
-158.288448312723));
#148358=CARTESIAN_POINT('Ctrl Pts',(-31.85,-55.4683430012288,-157.741722853926));
#148359=CARTESIAN_POINT('Ctrl Pts',(-31.8499999999999,-54.8007327275664,
-157.943927818991));
#148360=CARTESIAN_POINT('Ctrl Pts',(-31.1900434374137,-55.0116036525937,
-157.87112199741));
#148361=CARTESIAN_POINT('Ctrl Pts',(-31.85,-55.2730856891008,-156.923456306516));
#148362=CARTESIAN_POINT('Ctrl Pts',(-31.8499999999999,-54.6553685473472,
-157.056547547799));
#148363=CARTESIAN_POINT('Ctrl Pts',(-31.2350144161398,-54.7946179131854,
-157.017203864823));
#148364=CARTESIAN_POINT('Ctrl Pts',(-31.85,-55.2005310139637,-156.507030856831));
#148365=CARTESIAN_POINT('Ctrl Pts',(-31.8500000000015,-54.6061056306454,
-156.61011452235));
#148366=CARTESIAN_POINT('Ctrl Pts',(-31.2578793589119,-54.7139857241292,
-156.582429725824));
#148367=CARTESIAN_POINT('Ctrl Pts',(-31.85,-55.0867689945819,-155.521921774446));
#148368=CARTESIAN_POINT('Ctrl Pts',(-31.8499999999981,-54.5497265489757,
-155.574697108694));
#148369=CARTESIAN_POINT('Ctrl Pts',(-31.3119027856115,-54.5875443127981,
-155.553382086724));
#148370=CARTESIAN_POINT('Ctrl Pts',(-31.85,-55.0656087290325,-154.94924650253));
#148371=CARTESIAN_POINT('Ctrl Pts',(-31.8500000000013,-54.5573584552804,
-154.971890850079));
#148372=CARTESIAN_POINT('Ctrl Pts',(-31.3432560810077,-54.5640138310673,
-154.954760169123));
#148373=CARTESIAN_POINT('Ctrl Pts',(-31.85,-55.0895347934625,-154.371949728242));
#148374=CARTESIAN_POINT('Ctrl Pts',(-31.8499999999992,-54.6141856226549,
-154.351866222665));
#148375=CARTESIAN_POINT('Ctrl Pts',(-31.3747904412016,-54.590578610047,
-154.350869818715));
#148376=CARTESIAN_POINT('',(-31.084285288415,-55.9092502162754,-159.879976566996));
#148377=CARTESIAN_POINT('Origin',(-31.35,-56.2763252281792,-159.66866755714));
#148378=CARTESIAN_POINT('Ctrl Pts',(-31.0842854211463,-55.9092502161047,
-159.87997642591));
#148379=CARTESIAN_POINT('Ctrl Pts',(-31.0896514277362,-55.8469879056698,
-159.77856394342));
#148380=CARTESIAN_POINT('Ctrl Pts',(-31.095109779591,-55.7874666718174,
-159.676149018302));
#148381=CARTESIAN_POINT('Ctrl Pts',(-31.1006032503633,-55.7305129240826,
-159.572833254483));
#148382=CARTESIAN_POINT('Ctrl Pts',(-31.1061823346791,-55.672671574981,
-159.46790735583));
#148383=CARTESIAN_POINT('Ctrl Pts',(-31.1117978298489,-55.6174776776756,
-159.362052199246));
#148384=CARTESIAN_POINT('Ctrl Pts',(-31.1174329116102,-55.5647534325291,
-159.255340693208));
#148385=CARTESIAN_POINT('Ctrl Pts',(-31.1231991622453,-55.5108019150638,
-159.146145243073));
#148386=CARTESIAN_POINT('Ctrl Pts',(-31.1289861521601,-55.4594356856543,
-159.036052959027));
#148387=CARTESIAN_POINT('Ctrl Pts',(-31.1348175145198,-55.4104789077723,
-158.925109188129));
#148388=CARTESIAN_POINT('Ctrl Pts',(-31.1388264610931,-55.3768220888628,
-158.848837534484));
#148389=CARTESIAN_POINT('Ctrl Pts',(-31.1428572605651,-55.3443043684264,
-158.772162749669));
#148390=CARTESIAN_POINT('Ctrl Pts',(-31.1469275973672,-55.3128748584107,
-158.695091598692));
#148391=CARTESIAN_POINT('Ctrl Pts',(-31.1539498174176,-55.2586520886162,
-158.562127028925));
#148392=CARTESIAN_POINT('Ctrl Pts',(-31.1610514741968,-55.2076908016112,
-158.427997684076));
#148393=CARTESIAN_POINT('Ctrl Pts',(-31.1681970280243,-55.159847533947,
-158.292768518215));
#148394=CARTESIAN_POINT('Ctrl Pts',(-31.1755499129171,-55.1106160749836,
-158.153615624719));
#148395=CARTESIAN_POINT('Ctrl Pts',(-31.1829497326462,-55.0646854243966,
-158.013297832529));
#148396=CARTESIAN_POINT('Ctrl Pts',(-31.1903953483088,-55.0219287506999,
-157.871856051504));
#148397=CARTESIAN_POINT('Ctrl Pts',(-31.1978409639714,-54.9791720770031,
-157.73041427048));
#148398=CARTESIAN_POINT('Ctrl Pts',(-31.205333071078,-54.9395888987774,
-157.587847970466));
#148399=CARTESIAN_POINT('Ctrl Pts',(-31.2128985676693,-54.9030908083614,
-157.4441753669));
#148400=CARTESIAN_POINT('Ctrl Pts',(-31.222941383244,-54.854641432111,-157.253457223902));
#148401=CARTESIAN_POINT('Ctrl Pts',(-31.233071348161,-54.8117414293067,
-157.061174547668));
#148402=CARTESIAN_POINT('Ctrl Pts',(-31.2432320500935,-54.7743373143562,
-156.867957719114));
#148403=CARTESIAN_POINT('Ctrl Pts',(-31.2539055300877,-54.7350455336035,
-156.664989856478));
#148404=CARTESIAN_POINT('Ctrl Pts',(-31.2646128592783,-54.7018177706184,
-156.460991131094));
#148405=CARTESIAN_POINT('Ctrl Pts',(-31.2753335192659,-54.6745648754831,
-156.25666969964));
#148406=CARTESIAN_POINT('Ctrl Pts',(-31.2772548724241,-54.6696806205773,
-156.220051279873));
#148407=CARTESIAN_POINT('Ctrl Pts',(-31.2791767652949,-54.6649882224971,
-156.183422440874));
#148408=CARTESIAN_POINT('Ctrl Pts',(-31.2810992223836,-54.6604871030235,
-156.146787191114));
#148409=CARTESIAN_POINT('Ctrl Pts',(-31.2894544615779,-54.6409246742618,
-155.987565809011));
#148410=CARTESIAN_POINT('Ctrl Pts',(-31.2978181349023,-54.6249422843353,
-155.827972968174));
#148411=CARTESIAN_POINT('Ctrl Pts',(-31.3061986924678,-54.6125104976354,
-155.668000735124));
#148412=CARTESIAN_POINT('Ctrl Pts',(-31.3145757427008,-54.6000839137411,
-155.508095451776));
#148413=CARTESIAN_POINT('Ctrl Pts',(-31.3229704705527,-54.5912052112514,
-155.347810416513));
#148414=CARTESIAN_POINT('Ctrl Pts',(-31.3313828706828,-54.5858956626337,
-155.187144207599));
#148415=CARTESIAN_POINT('Ctrl Pts',(-31.337581338876,-54.5819834535472,
-155.068761300189));
#148416=CARTESIAN_POINT('Ctrl Pts',(-31.3437892685361,-54.5800100820981,
-154.950171544755));
#148417=CARTESIAN_POINT('Ctrl Pts',(-31.3500000000037,-54.5800000583607,
-154.831379798155));
#148418=CARTESIAN_POINT('Ctrl Pts',(-31.0842850915597,-55.9092502513102,
-159.879976688011));
#148419=CARTESIAN_POINT('Ctrl Pts',(-31.8499999999999,-55.4929314270088,
-160.119633364362));
#148420=CARTESIAN_POINT('Ctrl Pts',(-31.85,-56.2763252281792,-159.66866755714));
#148421=CARTESIAN_POINT('Ctrl Pts',(-31.0928842088245,-58.0390008802754,
-163.590479273921));
#148422=CARTESIAN_POINT('Ctrl Pts',(-31.8500000000438,-57.6056192097127,
-163.747040286917));
#148423=CARTESIAN_POINT('Ctrl Pts',(-31.85,-58.4122993941661,-163.37916820794));
#148424=CARTESIAN_POINT('Ctrl Pts',(-31.1007058108654,-60.129339000976,
-167.323759171684));
#148425=CARTESIAN_POINT('Ctrl Pts',(-31.8499999999999,-59.7238064590067,
-167.480553670321));
#148426=CARTESIAN_POINT('Ctrl Pts',(-31.85,-60.5078533703316,-167.112448841938));
#148427=CARTESIAN_POINT('Ctrl Pts',(-31.1079170675507,-62.1926886331265,
-171.07256826174));
#148428=CARTESIAN_POINT('Ctrl Pts',(-31.8499999999999,-61.8331341426276,
-171.27090462831));
#148429=CARTESIAN_POINT('Ctrl Pts',(-31.85,-62.5757608260975,-170.861259130871));
#148430=CARTESIAN_POINT('',(-31.1079170675507,-62.1926886331265,-171.07256826174));
#148431=CARTESIAN_POINT('Origin',(-31.35,-62.5757608260974,-170.861259130871));
#148432=CARTESIAN_POINT('Ctrl Pts',(-31.1079170675507,-62.1926886331265,
-171.07256826174));
#148433=CARTESIAN_POINT('Ctrl Pts',(-31.1007058117848,-60.1293390004784,
-167.323759171876));
#148434=CARTESIAN_POINT('Ctrl Pts',(-31.092884209739,-58.0390008797519,
-163.59047927411));
#148435=CARTESIAN_POINT('Ctrl Pts',(-31.0842850915597,-55.9092502513102,
-159.879976688011));
#148436=CARTESIAN_POINT('Ctrl Pts',(-31.85,-63.1109998882233,-171.14995));
#148437=CARTESIAN_POINT('Ctrl Pts',(-31.8499999999999,-63.1109998882232,
-171.64995));
#148438=CARTESIAN_POINT('Ctrl Pts',(-31.35,-63.1109998882233,-171.64995));
#148439=CARTESIAN_POINT('Ctrl Pts',(-31.85,-63.0574084096236,-171.149949978884));
#148440=CARTESIAN_POINT('Ctrl Pts',(-31.8499999999969,-63.0165988837716,
-171.67463547811));
#148441=CARTESIAN_POINT('Ctrl Pts',(-31.3259104704307,-63.0188778416583,
-171.64995));
#148442=CARTESIAN_POINT('Ctrl Pts',(-31.85,-63.0049471542817,-171.14386632127));
#148443=CARTESIAN_POINT('Ctrl Pts',(-31.8500000000009,-62.9206095930479,
-171.689168561081));
#148444=CARTESIAN_POINT('Ctrl Pts',(-31.3022843203587,-62.9287506782315,
-171.637782628619));
#148445=CARTESIAN_POINT('Ctrl Pts',(-31.85,-62.9022833467989,-171.11979081221));
#148446=CARTESIAN_POINT('Ctrl Pts',(-31.8499999999991,-62.7178130579107,
-171.697646145438));
#148447=CARTESIAN_POINT('Ctrl Pts',(-31.2559687677351,-62.752470972064,
-171.58963163834));
#148448=CARTESIAN_POINT('Ctrl Pts',(-31.85,-62.8513307506207,-171.101350238814));
#148449=CARTESIAN_POINT('Ctrl Pts',(-31.8499999999999,-62.6084779204031,
-171.690011580914));
#148450=CARTESIAN_POINT('Ctrl Pts',(-31.2329391869239,-62.6650327081311,
-171.552750471208));
#148451=CARTESIAN_POINT('Ctrl Pts',(-31.85,-62.7572432252394,-171.052906534958));
#148452=CARTESIAN_POINT('Ctrl Pts',(-31.85,-62.3853423742397,-171.644110259622));
#148453=CARTESIAN_POINT('Ctrl Pts',(-31.1903462652202,-62.5036508698849,
-171.455863076335));
#148454=CARTESIAN_POINT('Ctrl Pts',(-31.85,-62.7137529944933,-171.02308307076));
#148455=CARTESIAN_POINT('Ctrl Pts',(-31.8499999999993,-62.2707897308557,
-171.604668782303));
#148456=CARTESIAN_POINT('Ctrl Pts',(-31.1706237499557,-62.4290960074683,
-171.396216101863));
#148457=CARTESIAN_POINT('Ctrl Pts',(-31.85,-62.6352107798375,-170.950134506763));
#148458=CARTESIAN_POINT('Ctrl Pts',(-31.8500000000008,-62.0386786747199,
-171.476624739535));
#148459=CARTESIAN_POINT('Ctrl Pts',(-31.1349614654849,-62.2945035389765,
-171.250319053184));
#148460=CARTESIAN_POINT('Ctrl Pts',(-31.85,-62.6016585634489,-170.908207754234));
#148461=CARTESIAN_POINT('Ctrl Pts',(-31.8499999999999,-61.9268239314477,
-171.387766739956));
#148462=CARTESIAN_POINT('Ctrl Pts',(-31.1197024222507,-62.2370348840453,
-171.166463157496));
#148463=CARTESIAN_POINT('Ctrl Pts',(-31.85,-62.5757608260974,-170.861259130871));
#148464=CARTESIAN_POINT('Ctrl Pts',(-31.85,-61.8331341426276,-171.270904628311));
#148465=CARTESIAN_POINT('Ctrl Pts',(-31.1079170675507,-62.1926886331265,
-171.07256826174));
#148466=CARTESIAN_POINT('',(-31.35,-63.1109998882233,-171.64995));
#148467=CARTESIAN_POINT('Origin',(-31.35,-63.1109998882233,-171.14995));
#148468=CARTESIAN_POINT('Ctrl Pts',(-31.35,-63.1109998882233,-171.64995));
#148469=CARTESIAN_POINT('Ctrl Pts',(-31.3259104704307,-63.0188778416583,
-171.64995));
#148470=CARTESIAN_POINT('Ctrl Pts',(-31.3022843203587,-62.9287506782315,
-171.637782628619));
#148471=CARTESIAN_POINT('Ctrl Pts',(-31.2559687677351,-62.752470972064,
-171.58963163834));
#148472=CARTESIAN_POINT('Ctrl Pts',(-31.2329391869239,-62.6650327081311,
-171.552750471208));
#148473=CARTESIAN_POINT('Ctrl Pts',(-31.1903462652202,-62.5036508698849,
-171.455863076335));
#148474=CARTESIAN_POINT('Ctrl Pts',(-31.1706237499557,-62.4290960074683,
-171.396216101863));
#148475=CARTESIAN_POINT('Ctrl Pts',(-31.1349614654849,-62.2945035389765,
-171.250319053184));
#148476=CARTESIAN_POINT('Ctrl Pts',(-31.1197024222507,-62.2370348840453,
-171.166463157496));
#148477=CARTESIAN_POINT('Ctrl Pts',(-31.1079170675507,-62.1926886331265,
-171.07256826174));
#148478=CARTESIAN_POINT('Origin',(-31.35,-12.9675000200281,-171.14995));
#148479=CARTESIAN_POINT('',(-31.35,-63.7587939982373,-171.64995));
#148480=CARTESIAN_POINT('Origin',(-31.35,-63.7587939982373,-171.14995));
#148481=CARTESIAN_POINT('',(-31.35,-62.7949079300497,-171.64995));
#148482=CARTESIAN_POINT('Ctrl Pts',(-31.35,-63.7587939982373,-171.64995));
#148483=CARTESIAN_POINT('Ctrl Pts',(-31.8499999999999,-63.7587939982373,
-171.64995));
#148484=CARTESIAN_POINT('Ctrl Pts',(-31.85,-63.7587939982373,-171.14995));
#148485=CARTESIAN_POINT('Ctrl Pts',(-31.3408895000012,-63.8922843417627,
-171.64995));
#148486=CARTESIAN_POINT('Ctrl Pts',(-31.85,-63.8935759445488,-171.659148653594));
#148487=CARTESIAN_POINT('Ctrl Pts',(-31.85,-63.9571089176128,-171.149950000016));
#148488=CARTESIAN_POINT('Ctrl Pts',(-31.331785867019,-64.0256740672594,
-171.675977326981));
#148489=CARTESIAN_POINT('Ctrl Pts',(-31.85,-64.0229667628024,-171.69520402023));
#148490=CARTESIAN_POINT('Ctrl Pts',(-31.85,-64.1552743575927,-171.18899099047));
#148491=CARTESIAN_POINT('Ctrl Pts',(-31.3149548930126,-64.2722875903527,
-171.776163607997));
#148492=CARTESIAN_POINT('Ctrl Pts',(-31.85,-64.2557455586227,-171.809929875206));
#148493=CARTESIAN_POINT('Ctrl Pts',(-31.85,-64.521646483527,-171.339270411997));
#148494=CARTESIAN_POINT('Ctrl Pts',(-31.3072358131761,-64.3853903420367,
-171.850283164391));
#148495=CARTESIAN_POINT('Ctrl Pts',(-31.850000000002,-64.3583202713598,
-171.888983273332));
#148496=CARTESIAN_POINT('Ctrl Pts',(-31.85,-64.6896733421684,-171.450449746589));
#148497=CARTESIAN_POINT('Ctrl Pts',(-31.2943539433762,-64.5741401609095,
-172.035403273235));
#148498=CARTESIAN_POINT('Ctrl Pts',(-31.8499999999979,-64.5259770425163,
-172.075215659168));
#148499=CARTESIAN_POINT('Ctrl Pts',(-31.85,-64.9700824273775,-171.728129909852));
#148500=CARTESIAN_POINT('Ctrl Pts',(-31.2891962191206,-64.6497130035424,
-172.14633102856));
#148501=CARTESIAN_POINT('Ctrl Pts',(-31.85,-64.590248108326,-172.182182441317));
#148502=CARTESIAN_POINT('Ctrl Pts',(-31.85,-65.0823543850191,-171.894521542842));
#148503=CARTESIAN_POINT('Ctrl Pts',(-31.2822246014263,-64.751863669369,
-172.38820210671));
#148504=CARTESIAN_POINT('Ctrl Pts',(-31.8499999999999,-64.676681437744,
-172.409726298163));
#148505=CARTESIAN_POINT('Ctrl Pts',(-31.85,-65.2341106883021,-172.257328160063));
#148506=CARTESIAN_POINT('Ctrl Pts',(-31.2804134495219,-64.7784013226442,
-172.51902671195));
#148507=CARTESIAN_POINT('Ctrl Pts',(-31.85,-64.6983511534103,-172.529650273729));
#148508=CARTESIAN_POINT('Ctrl Pts',(-31.85,-65.273535357003,-172.453565067926));
#148509=CARTESIAN_POINT('Ctrl Pts',(-31.28041344952,-64.7784013226445,-172.64995));
#148510=CARTESIAN_POINT('Ctrl Pts',(-31.85,-64.6983511534048,-172.64995));
#148511=CARTESIAN_POINT('Ctrl Pts',(-31.85,-65.2735353570153,-172.64995));
#148512=CARTESIAN_POINT('Origin',(-31.35,-65.2735353570153,-172.64995));
#148513=CARTESIAN_POINT('Ctrl Pts',(-31.28041344952,-64.7784013226445,-172.64995));
#148514=CARTESIAN_POINT('Ctrl Pts',(-31.2804134495219,-64.7784013226442,
-172.51902671195));
#148515=CARTESIAN_POINT('Ctrl Pts',(-31.2822246014263,-64.751863669369,
-172.38820210671));
#148516=CARTESIAN_POINT('Ctrl Pts',(-31.2891962191206,-64.6497130035424,
-172.14633102856));
#148517=CARTESIAN_POINT('Ctrl Pts',(-31.2943539433762,-64.5741401609095,
-172.035403273235));
#148518=CARTESIAN_POINT('Ctrl Pts',(-31.3072358131761,-64.3853903420367,
-171.850283164391));
#148519=CARTESIAN_POINT('Ctrl Pts',(-31.3149548930126,-64.2722875903527,
-171.776163607997));
#148520=CARTESIAN_POINT('Ctrl Pts',(-31.331785867019,-64.0256740672594,
-171.675977326981));
#148521=CARTESIAN_POINT('Ctrl Pts',(-31.3408895000012,-63.8922843417627,
-171.64995));
#148522=CARTESIAN_POINT('Ctrl Pts',(-31.35,-63.7587939982373,-171.64995));
#148523=CARTESIAN_POINT('Origin',(-31.35,-65.2735353570153,-171.64995));
#148524=CARTESIAN_POINT('Origin',(-31.35,-65.2735353570153,-176.84995));
#148525=CARTESIAN_POINT('Origin',(-32.35,67.7009572055632,-176.84995));
#148526=CARTESIAN_POINT('',(-32.35,-70.08000002,-177.34995));
#148527=CARTESIAN_POINT('Origin',(-32.35,-70.08000002,-176.84995));
#148528=CARTESIAN_POINT('',(-32.35,-65.1329945223129,-177.34995));
#148529=CARTESIAN_POINT('',(-32.35,-73.08000002,-177.34995));
#148530=CARTESIAN_POINT('Ctrl Pts',(-31.85,-65.2735353570153,-176.84995));
#148531=CARTESIAN_POINT('Ctrl Pts',(-31.85,-65.2735353570043,-176.981217345763));
#148532=CARTESIAN_POINT('Ctrl Pts',(-31.9038865634697,-65.2583888317962,
-177.110943344657));
#148533=CARTESIAN_POINT('Ctrl Pts',(-32.0890066553437,-65.2063549673329,
-177.296063436531));
#148534=CARTESIAN_POINT('Ctrl Pts',(-32.2187326542366,-65.1698913669989,
-177.34995));
#148535=CARTESIAN_POINT('Ctrl Pts',(-32.35,-65.1329945223129,-177.34995));
#148536=CARTESIAN_POINT('Origin',(-32.35,-70.08000002,-174.34995));
#148537=CARTESIAN_POINT('',(-32.35,-73.08000002,-174.34995));
#148538=CARTESIAN_POINT('Origin',(-32.35,-72.58000002,-174.34995));
#148539=CARTESIAN_POINT('Origin',(-32.35,-70.08000002,-174.34995));
#148540=CARTESIAN_POINT('Origin',(-32.35,-72.58000002,-55.24995));
#148541=CARTESIAN_POINT('',(-32.35,-73.08000002,-58.24995));
#148542=CARTESIAN_POINT('Origin',(-32.35,-72.58000002,-58.24995));
#148543=CARTESIAN_POINT('',(-32.35,-73.08000002,-174.34995));
#148544=CARTESIAN_POINT('Origin',(-32.35,-70.08000002,-58.24995));
#148545=CARTESIAN_POINT('Origin',(-32.35,-70.08000002,-58.24995));
#148546=CARTESIAN_POINT('Origin',(3.3975957231091E-14,-70.08000002,-58.24995));
#148547=CARTESIAN_POINT('',(-32.85,-73.08000002,-58.24995));
#148548=CARTESIAN_POINT('Origin',(-32.85,-70.08000002,-58.24995));
#148549=CARTESIAN_POINT('',(41.5,-73.0800000199999,-58.24995));
#148550=CARTESIAN_POINT('Origin',(-32.85,-70.08000002,-58.24995));
#148551=CARTESIAN_POINT('Origin',(-32.85,-72.58000002,-58.24995));
#148552=CARTESIAN_POINT('Origin',(-32.85,-73.08000002,-176.84995));
#148553=CARTESIAN_POINT('',(-32.85,-65.0627241049617,-177.34995));
#148554=CARTESIAN_POINT('',(-32.85,-70.08000002,-177.34995));
#148555=CARTESIAN_POINT('',(-32.85,-73.08000002,-177.34995));
#148556=CARTESIAN_POINT('Origin',(-32.85,-70.08000002,-176.84995));
#148557=CARTESIAN_POINT('Ctrl Pts',(-32.85,-65.0627241049617,-177.34995));
#148558=CARTESIAN_POINT('Ctrl Pts',(-32.9812673457631,-65.0258272602758,
-177.34995));
#148559=CARTESIAN_POINT('Ctrl Pts',(-33.1109933446567,-64.9893636599417,
-177.29606343653));
#148560=CARTESIAN_POINT('Ctrl Pts',(-33.2961134365298,-64.9373297954784,
-177.110943344657));
#148561=CARTESIAN_POINT('Ctrl Pts',(-33.35,-64.9221832702703,-176.981217345763));
#148562=CARTESIAN_POINT('Ctrl Pts',(-33.35,-64.9221832702593,-176.84995));
#148563=CARTESIAN_POINT('Origin',(-33.85,-64.9221832702593,-171.64995));
#148564=CARTESIAN_POINT('Origin',(-33.85,-64.9221832702593,-176.84995));
#148565=CARTESIAN_POINT('Origin',(-33.85,-64.9221832702593,-172.64995));
#148566=CARTESIAN_POINT('Ctrl Pts',(-33.7804134495199,-64.4270492358885,
-172.64995));
#148567=CARTESIAN_POINT('Ctrl Pts',(-33.3499999999999,-64.4875399013512,
-172.64995));
#148568=CARTESIAN_POINT('Ctrl Pts',(-33.35,-64.9221832702593,-172.64995));
#148569=CARTESIAN_POINT('Ctrl Pts',(-33.7804134495211,-64.4270492358883,
-172.51902671195));
#148570=CARTESIAN_POINT('Ctrl Pts',(-33.35,-64.4875399013443,-172.511015867074));
#148571=CARTESIAN_POINT('Ctrl Pts',(-33.35,-64.922183270247,-172.453565067926));
#148572=CARTESIAN_POINT('Ctrl Pts',(-33.7822246014263,-64.4005115826131,
-172.38820210671));
#148573=CARTESIAN_POINT('Ctrl Pts',(-33.35,-64.4577842162266,-172.371853931892));
#148574=CARTESIAN_POINT('Ctrl Pts',(-33.35,-64.8827586015461,-172.257328160063));
#148575=CARTESIAN_POINT('Ctrl Pts',(-33.7891962191206,-64.2983609167864,
-172.14633102856));
#148576=CARTESIAN_POINT('Ctrl Pts',(-33.35,-64.3449732070946,-172.118296873734));
#148577=CARTESIAN_POINT('Ctrl Pts',(-33.35,-64.7310022982632,-171.894521542842));
#148578=CARTESIAN_POINT('Ctrl Pts',(-33.7943539433762,-64.2227880741536,
-172.035403273235));
#148579=CARTESIAN_POINT('Ctrl Pts',(-33.3500000000013,-64.2614041148292,
-172.003556970023));
#148580=CARTESIAN_POINT('Ctrl Pts',(-33.35,-64.6187303406215,-171.728129909852));
#148581=CARTESIAN_POINT('Ctrl Pts',(-33.8072358131761,-64.0340382552807,
-171.850283164391));
#148582=CARTESIAN_POINT('Ctrl Pts',(-33.3499999999986,-64.0569588954535,
-171.817687494207));
#148583=CARTESIAN_POINT('Ctrl Pts',(-33.35,-64.3383212554124,-171.450449746589));
#148584=CARTESIAN_POINT('Ctrl Pts',(-33.8149548930127,-63.9209355035967,
-171.776163607997));
#148585=CARTESIAN_POINT('Ctrl Pts',(-33.3499999999999,-63.9353951792977,
-171.746711574348));
#148586=CARTESIAN_POINT('Ctrl Pts',(-33.35,-64.1702943967697,-171.339270411997));
#148587=CARTESIAN_POINT('Ctrl Pts',(-33.831785867019,-63.6743219805034,
-171.675977326981));
#148588=CARTESIAN_POINT('Ctrl Pts',(-33.3499999999999,-63.6769599183967,
-171.658003579003));
#148589=CARTESIAN_POINT('Ctrl Pts',(-33.35,-63.8039222708381,-171.18899099047));
#148590=CARTESIAN_POINT('Ctrl Pts',(-33.8408895000012,-63.5409322550068,
-171.64995));
#148591=CARTESIAN_POINT('Ctrl Pts',(-33.35,-63.5396903402446,-171.640924254979));
#148592=CARTESIAN_POINT('Ctrl Pts',(-33.35,-63.6057568308558,-171.149950000016));
#148593=CARTESIAN_POINT('Ctrl Pts',(-33.85,-63.4074419114814,-171.64995));
#148594=CARTESIAN_POINT('Ctrl Pts',(-33.35,-63.4074419114814,-171.64995));
#148595=CARTESIAN_POINT('Ctrl Pts',(-33.35,-63.4074419114814,-171.14995));
#148596=CARTESIAN_POINT('',(-33.85,-63.4074419114814,-171.64995));
#148597=CARTESIAN_POINT('Origin',(-33.85,-63.4074419114814,-171.14995));
#148598=CARTESIAN_POINT('Ctrl Pts',(-33.85,-63.4074419114814,-171.64995));
#148599=CARTESIAN_POINT('Ctrl Pts',(-33.8408895000012,-63.5409322550068,
-171.64995));
#148600=CARTESIAN_POINT('Ctrl Pts',(-33.831785867019,-63.6743219805034,
-171.675977326981));
#148601=CARTESIAN_POINT('Ctrl Pts',(-33.8149548930127,-63.9209355035967,
-171.776163607997));
#148602=CARTESIAN_POINT('Ctrl Pts',(-33.8072358131761,-64.0340382552807,
-171.850283164391));
#148603=CARTESIAN_POINT('Ctrl Pts',(-33.7943539433762,-64.2227880741536,
-172.035403273235));
#148604=CARTESIAN_POINT('Ctrl Pts',(-33.7891962191206,-64.2983609167864,
-172.14633102856));
#148605=CARTESIAN_POINT('Ctrl Pts',(-33.7822246014263,-64.4005115826131,
-172.38820210671));
#148606=CARTESIAN_POINT('Ctrl Pts',(-33.7804134495211,-64.4270492358883,
-172.51902671195));
#148607=CARTESIAN_POINT('Ctrl Pts',(-33.7804134495199,-64.4270492358885,
-172.64995));
#148608=CARTESIAN_POINT('Origin',(-33.85,-12.9675000200281,-171.14995));
#148609=CARTESIAN_POINT('',(-33.85,-61.4584329769396,-171.64995));
#148610=CARTESIAN_POINT('Origin',(-33.85,-61.4584329769396,-171.14995));
#148611=CARTESIAN_POINT('',(-33.85,-63.4777123288326,-171.64995));
#148612=CARTESIAN_POINT('Ctrl Pts',(-33.35,-60.9047458754482,-170.861259130871));
#148613=CARTESIAN_POINT('Ctrl Pts',(-33.35,-60.6616577186179,-171.000024903864));
#148614=CARTESIAN_POINT('Ctrl Pts',(-33.5886122085038,-60.5345771657123,
-171.07256826174));
#148615=CARTESIAN_POINT('Ctrl Pts',(-33.35,-60.9589985837086,-170.956298004649));
#148616=CARTESIAN_POINT('Ctrl Pts',(-33.35,-60.7324577567303,-171.164705534849));
#148617=CARTESIAN_POINT('Ctrl Pts',(-33.6143702523473,-60.6248836296038,
-171.262628507825));
#148618=CARTESIAN_POINT('Ctrl Pts',(-33.35,-61.0447979165095,-171.029411101528));
#148619=CARTESIAN_POINT('Ctrl Pts',(-33.35,-60.8476105616749,-171.30214317251));
#148620=CARTESIAN_POINT('Ctrl Pts',(-33.6550624512799,-60.7677941641835,
-171.408872220814));
#148621=CARTESIAN_POINT('Ctrl Pts',(-33.35,-61.2401222274203,-171.126096896401));
#148622=CARTESIAN_POINT('Ctrl Pts',(-33.35,-61.1206228774013,-171.52051244062));
#148623=CARTESIAN_POINT('Ctrl Pts',(-33.7473474982865,-61.0935989844289,
-171.602243775044));
#148624=CARTESIAN_POINT('Ctrl Pts',(-33.35,-61.3489942654266,-171.149949989359));
#148625=CARTESIAN_POINT('Ctrl Pts',(-33.35,-61.28441455953,-171.601111075884));
#148626=CARTESIAN_POINT('Ctrl Pts',(-33.7986334045837,-61.2754078195329,
-171.64995));
#148627=CARTESIAN_POINT('Ctrl Pts',(-33.35,-61.4584329769396,-171.14995));
#148628=CARTESIAN_POINT('Ctrl Pts',(-33.35,-61.4584329769396,-171.64995));
#148629=CARTESIAN_POINT('Ctrl Pts',(-33.85,-61.4584329769396,-171.64995));
#148630=CARTESIAN_POINT('',(-33.5886122085038,-60.5345771657123,-171.07256826174));
#148631=CARTESIAN_POINT('Origin',(-33.85,-60.9047458754482,-170.861259130871));
#148632=CARTESIAN_POINT('Ctrl Pts',(-33.5886122085038,-60.5345771657123,
-171.07256826174));
#148633=CARTESIAN_POINT('Ctrl Pts',(-33.6143702523473,-60.6248836296038,
-171.262628507825));
#148634=CARTESIAN_POINT('Ctrl Pts',(-33.6550624512799,-60.7677941641835,
-171.408872220814));
#148635=CARTESIAN_POINT('Ctrl Pts',(-33.7473474982865,-61.0935989844289,
-171.602243775044));
#148636=CARTESIAN_POINT('Ctrl Pts',(-33.7986334045837,-61.2754078195329,
-171.64995));
#148637=CARTESIAN_POINT('Ctrl Pts',(-33.85,-61.4584329769396,-171.64995));
#148638=CARTESIAN_POINT('Ctrl Pts',(-33.5886122085038,-60.5345771657124,
-171.07256826174));
#148639=CARTESIAN_POINT('Ctrl Pts',(-33.35,-60.6616577186179,-171.000024903864));
#148640=CARTESIAN_POINT('Ctrl Pts',(-33.35,-60.9047458754482,-170.861259130871));
#148641=CARTESIAN_POINT('Ctrl Pts',(-33.5831748521597,-59.0440141159766,
-168.454692464379));
#148642=CARTESIAN_POINT('Ctrl Pts',(-33.3499999999583,-59.1768144406969,
-168.390475993822));
#148643=CARTESIAN_POINT('Ctrl Pts',(-33.35,-59.4103431251365,-168.243382962268));
#148644=CARTESIAN_POINT('Ctrl Pts',(-33.5774199132796,-57.5365496870091,
-165.846853703856));
#148645=CARTESIAN_POINT('Ctrl Pts',(-33.3500000000315,-57.6703808898087,
-165.782543034447));
#148646=CARTESIAN_POINT('Ctrl Pts',(-33.35,-57.8986390322929,-165.635544032027));
#148647=CARTESIAN_POINT('Ctrl Pts',(-33.5712930253539,-56.0068938993568,
-163.252219719633));
#148648=CARTESIAN_POINT('Ctrl Pts',(-33.35,-56.1347789227867,-163.176590079091));
#148649=CARTESIAN_POINT('Ctrl Pts',(-33.35,-56.364204511422,-163.040910588762));
#148650=CARTESIAN_POINT('',(-33.5716736357884,-56.0068703689372,-163.251931093946));
#148651=CARTESIAN_POINT('Origin',(-33.85,-56.3642045114216,-163.040910588762));
#148652=CARTESIAN_POINT('Ctrl Pts',(-33.5712930253608,-56.0068938993483,
-163.252219719627));
#148653=CARTESIAN_POINT('Ctrl Pts',(-33.5774199132796,-57.5365496870091,
-165.846853703856));
#148654=CARTESIAN_POINT('Ctrl Pts',(-33.5831748521597,-59.0440141159766,
-168.454692464379));
#148655=CARTESIAN_POINT('Ctrl Pts',(-33.5886122085038,-60.5345771657123,
-171.07256826174));
#148656=CARTESIAN_POINT('Ctrl Pts',(-33.35,-55.0808765597097,-157.757860472338));
#148657=CARTESIAN_POINT('Ctrl Pts',(-33.35,-54.572872815689,-157.751515483814));
#148658=CARTESIAN_POINT('Ctrl Pts',(-33.8579839047711,-54.5809755801308,
-157.751597589538));
#148659=CARTESIAN_POINT('Ctrl Pts',(-33.35,-55.0694930553304,-158.705257460135));
#148660=CARTESIAN_POINT('Ctrl Pts',(-33.3499999999996,-54.6110102505827,
-158.691991727223));
#148661=CARTESIAN_POINT('Ctrl Pts',(-33.80673251536,-54.5683165271959,-158.739783519818));
#148662=CARTESIAN_POINT('Ctrl Pts',(-33.35,-55.1688504851514,-159.636950827836));
#148663=CARTESIAN_POINT('Ctrl Pts',(-33.3500000000034,-54.7494053948693,
-159.663263893567));
#148664=CARTESIAN_POINT('Ctrl Pts',(-33.7562189642388,-54.6787070453326,
-159.710574965063));
#148665=CARTESIAN_POINT('Ctrl Pts',(-33.35,-55.4903395816263,-160.984647645179));
#148666=CARTESIAN_POINT('Ctrl Pts',(-33.3499999999985,-55.1481757182452,
-161.073717268302));
#148667=CARTESIAN_POINT('Ctrl Pts',(-33.6830697051085,-55.0359064417903,
-161.113596033539));
#148668=CARTESIAN_POINT('Ctrl Pts',(-33.35,-55.6220934455112,-161.416204912461));
#148669=CARTESIAN_POINT('Ctrl Pts',(-33.3499999999999,-55.3013349864854,
-161.515699606681));
#148670=CARTESIAN_POINT('Ctrl Pts',(-33.659632768152,-55.1822975465829,
-161.56267650153));
#148671=CARTESIAN_POINT('Ctrl Pts',(-33.35,-55.9619578801892,-162.294644651832));
#148672=CARTESIAN_POINT('Ctrl Pts',(-33.35,-55.6869269417485,-162.409962964754));
#148673=CARTESIAN_POINT('Ctrl Pts',(-33.6119102026057,-55.5599217541785,
-162.476435800135));
#148674=CARTESIAN_POINT('Ctrl Pts',(-33.35,-56.176692790625,-162.740743620178));
#148675=CARTESIAN_POINT('Ctrl Pts',(-33.3500000000058,-55.9251276981362,
-162.865361276924));
#148676=CARTESIAN_POINT('Ctrl Pts',(-33.5876645600733,-55.7985279932288,
-162.94028227478));
#148677=CARTESIAN_POINT('Ctrl Pts',(-33.35,-56.4397410822123,-163.165758499336));
#148678=CARTESIAN_POINT('Ctrl Pts',(-33.3499999999981,-56.217599796636,
-163.303416706069));
#148679=CARTESIAN_POINT('Ctrl Pts',(-33.5645633535224,-56.0907870577493,
-163.381999868627));
#148680=CARTESIAN_POINT('',(-33.85,-54.58000002,-157.903547609535));
#148681=CARTESIAN_POINT('Origin',(-33.85,-55.08000002,-157.903547609535));
#148682=CARTESIAN_POINT('Ctrl Pts',(-33.85,-54.58000002,-157.903547609535));
#148683=CARTESIAN_POINT('Ctrl Pts',(-33.8413583508933,-54.5800000297389,
-158.070131241816));
#148684=CARTESIAN_POINT('Ctrl Pts',(-33.8327288620928,-54.5836479443981,
-158.236223407547));
#148685=CARTESIAN_POINT('Ctrl Pts',(-33.8241299270602,-54.5908750783497,
-158.401801779095));
#148686=CARTESIAN_POINT('Ctrl Pts',(-33.8154839223325,-54.5981417728969,
-158.568286509794));
#148687=CARTESIAN_POINT('Ctrl Pts',(-33.8068680592598,-54.6090265097566,
-158.734252422455));
#148688=CARTESIAN_POINT('Ctrl Pts',(-33.7982810557359,-54.6235053947455,
-158.899692634749));
#148689=CARTESIAN_POINT('Ctrl Pts',(-33.789726461072,-54.6379296338786,
-159.064508446613));
#148690=CARTESIAN_POINT('Ctrl Pts',(-33.7811996706316,-54.6559207511339,
-159.228803188151));
#148691=CARTESIAN_POINT('Ctrl Pts',(-33.7726915920417,-54.6775054187261,
-159.392576016311));
#148692=CARTESIAN_POINT('Ctrl Pts',(-33.7642741433225,-54.6988601618283,
-159.55460430132));
#148693=CARTESIAN_POINT('Ctrl Pts',(-33.7558741693399,-54.7237323809422,
-159.716122386248));
#148694=CARTESIAN_POINT('Ctrl Pts',(-33.7474876838614,-54.7521979722951,
-159.877125459224));
#148695=CARTESIAN_POINT('Ctrl Pts',(-33.7393031126239,-54.7799782219408,
-160.034252198857));
#148696=CARTESIAN_POINT('Ctrl Pts',(-33.7311306553308,-54.8111812601365,
-160.190888981756));
#148697=CARTESIAN_POINT('Ctrl Pts',(-33.7229827232003,-54.8459221337957,
-160.347018683881));
#148698=CARTESIAN_POINT('Ctrl Pts',(-33.7174882513588,-54.8693492744507,
-160.452303096932));
#148699=CARTESIAN_POINT('Ctrl Pts',(-33.7120052711149,-54.8943861173903,
-160.55735665573));
#148700=CARTESIAN_POINT('Ctrl Pts',(-33.7065443988847,-54.9210783233629,
-160.662168853243));
#148701=CARTESIAN_POINT('Ctrl Pts',(-33.6983891423225,-54.9609404147537,
-160.818695196566));
#148702=CARTESIAN_POINT('Ctrl Pts',(-33.6902654326991,-55.0045623826382,
-160.974930621019));
#148703=CARTESIAN_POINT('Ctrl Pts',(-33.6821730230048,-55.0520345142193,
-161.130338629735));
#148704=CARTESIAN_POINT('Ctrl Pts',(-33.6742415228735,-55.0985627094162,
-161.282656503904));
#148705=CARTESIAN_POINT('Ctrl Pts',(-33.6663403863785,-55.1487899099227,
-161.434179332344));
#148706=CARTESIAN_POINT('Ctrl Pts',(-33.658499112823,-55.2027656519471,
-161.584384445067));
#148707=CARTESIAN_POINT('Ctrl Pts',(-33.6512693155289,-55.252532270962,
-161.722876299715));
#148708=CARTESIAN_POINT('Ctrl Pts',(-33.64409090952,-55.3054855287205,-161.860247619697));
#148709=CARTESIAN_POINT('Ctrl Pts',(-33.6370064807475,-55.3616319074669,
-161.996077647676));
#148710=CARTESIAN_POINT('Ctrl Pts',(-33.6310339771099,-55.4089659215521,
-162.110588691862));
#148711=CARTESIAN_POINT('Ctrl Pts',(-33.6251574486299,-55.4585971099375,
-162.224128770533));
#148712=CARTESIAN_POINT('Ctrl Pts',(-33.6193265052801,-55.5106817363739,
-162.336662125923));
#148713=CARTESIAN_POINT('Ctrl Pts',(-33.6135805978345,-55.5620067836071,
-162.447554344527));
#148714=CARTESIAN_POINT('Ctrl Pts',(-33.6078786491602,-55.6157148224026,
-162.557469198455));
#148715=CARTESIAN_POINT('Ctrl Pts',(-33.6022090581942,-55.6719741097404,
-162.66634452554));
#148716=CARTESIAN_POINT('Ctrl Pts',(-33.5966802445508,-55.7268364652903,
-162.772516451774));
#148717=CARTESIAN_POINT('Ctrl Pts',(-33.5911820484159,-55.7841255741681,
-162.877699928124));
#148718=CARTESIAN_POINT('Ctrl Pts',(-33.5857420390386,-55.844006448796,
-162.981808400476));
#148719=CARTESIAN_POINT('Ctrl Pts',(-33.5809929344731,-55.8962821923382,
-163.072694644792));
#148720=CARTESIAN_POINT('Ctrl Pts',(-33.5762886530756,-55.9505335934556,
-163.162761236236));
#148721=CARTESIAN_POINT('Ctrl Pts',(-33.5716736357884,-56.0068703689372,
-163.251931093946));
#148722=CARTESIAN_POINT('Origin',(-33.85,-55.08000002,-55.24995));
#148723=CARTESIAN_POINT('',(-33.8499999999899,-54.58000002,-74.1550953619836));
#148724=CARTESIAN_POINT('Origin',(-33.85,-55.08000002,-74.155095361993));
#148725=CARTESIAN_POINT('',(-33.85,-54.58000002,-157.276549545042));
#148726=CARTESIAN_POINT('Ctrl Pts',(-33.35,-56.3642045114132,-69.0177323827589));
#148727=CARTESIAN_POINT('Ctrl Pts',(-33.35,-56.134778922778,-68.8820528924306));
#148728=CARTESIAN_POINT('Ctrl Pts',(-33.5712930253538,-56.006893899348,
-68.8064232518886));
#148729=CARTESIAN_POINT('Ctrl Pts',(-33.35,-56.1349989919057,-69.4053046881168));
#148730=CARTESIAN_POINT('Ctrl Pts',(-33.35,-55.8795696344188,-69.2811581349632));
#148731=CARTESIAN_POINT('Ctrl Pts',(-33.5923541472839,-55.7522317441443,
-69.2092624885051));
#148732=CARTESIAN_POINT('Ctrl Pts',(-33.35,-55.9450970231818,-69.808093015459));
#148733=CARTESIAN_POINT('Ctrl Pts',(-33.35,-55.6684723180091,-69.6920753057542));
#148734=CARTESIAN_POINT('Ctrl Pts',(-33.6142403739361,-55.5412189114063,
-69.628091942105));
#148735=CARTESIAN_POINT('Ctrl Pts',(-33.35,-55.6242976847011,-70.6362303826783));
#148736=CARTESIAN_POINT('Ctrl Pts',(-33.35,-55.3039535321835,-70.5365374259244));
#148737=CARTESIAN_POINT('Ctrl Pts',(-33.659221513549,-55.1847752040192,
-70.4895195351988));
#148738=CARTESIAN_POINT('Ctrl Pts',(-33.35,-55.4937179039915,-71.0617579129361));
#148739=CARTESIAN_POINT('Ctrl Pts',(-33.35,-55.152213923386,-70.9724898647665));
#148740=CARTESIAN_POINT('Ctrl Pts',(-33.682327027756,-55.0396865574335,
-70.9323196038346));
#148741=CARTESIAN_POINT('Ctrl Pts',(-33.35,-55.1806225291757,-72.3685609104781));
#148742=CARTESIAN_POINT('Ctrl Pts',(-33.35,-54.7649354301353,-72.3373662781827));
#148743=CARTESIAN_POINT('Ctrl Pts',(-33.7532457656832,-54.6918028086424,
-72.2927601348896));
#148744=CARTESIAN_POINT('Ctrl Pts',(-33.35,-55.0800000211738,-73.2600087408747));
#148745=CARTESIAN_POINT('Ctrl Pts',(-33.3499999999911,-54.6261840530745,
-73.2648134588722));
#148746=CARTESIAN_POINT('Ctrl Pts',(-33.801572917506,-54.5800000199981,
-73.221574548752));
#148747=CARTESIAN_POINT('Ctrl Pts',(-33.35,-55.08000002,-74.155095361993));
#148748=CARTESIAN_POINT('Ctrl Pts',(-33.35,-54.5800000199987,-74.155095361994));
#148749=CARTESIAN_POINT('Ctrl Pts',(-33.8500000000012,-54.58000002,-74.155095361994));
#148750=CARTESIAN_POINT('',(-33.5713955981573,-56.0068423841382,-68.80655523181));
#148751=CARTESIAN_POINT('Origin',(-33.85,-56.3642045114132,-69.0177323827589));
#148752=CARTESIAN_POINT('Ctrl Pts',(-33.5712993597704,-56.0068173078863,
-68.8065444112298));
#148753=CARTESIAN_POINT('Ctrl Pts',(-33.592358535658,-55.7521894346693,
-69.2093464673669));
#148754=CARTESIAN_POINT('Ctrl Pts',(-33.614242628708,-55.5412010439342,
-69.6281351229303));
#148755=CARTESIAN_POINT('Ctrl Pts',(-33.659221513549,-55.1847752040192,
-70.4895195351988));
#148756=CARTESIAN_POINT('Ctrl Pts',(-33.682327027756,-55.0396865574335,
-70.9323196038346));
#148757=CARTESIAN_POINT('Ctrl Pts',(-33.7532457656832,-54.6918028086424,
-72.2927601348896));
#148758=CARTESIAN_POINT('Ctrl Pts',(-33.801572917506,-54.5800000199981,
-73.221574548752));
#148759=CARTESIAN_POINT('Ctrl Pts',(-33.8499999999899,-54.58000002,-74.1550953619836));
#148760=CARTESIAN_POINT('Ctrl Pts',(-33.5712930253538,-56.006893899348,
-68.8064232518886));
#148761=CARTESIAN_POINT('Ctrl Pts',(-33.35,-56.134778922778,-68.8820528924306));
#148762=CARTESIAN_POINT('Ctrl Pts',(-33.35,-56.3642045114132,-69.0177323827589));
#148763=CARTESIAN_POINT('Ctrl Pts',(-33.5772316679252,-57.489551829777,
-66.2915080112617));
#148764=CARTESIAN_POINT('Ctrl Pts',(-33.35,-57.623019767821,-66.3564728841549));
#148765=CARTESIAN_POINT('Ctrl Pts',(-33.35,-57.8514943778664,-66.5028176210733));
#148766=CARTESIAN_POINT('Ctrl Pts',(-33.5828208370019,-58.9513545007691,
-63.7641770795492));
#148767=CARTESIAN_POINT('Ctrl Pts',(-33.35,-59.0838703919199,-63.828995910853));
#148768=CARTESIAN_POINT('Ctrl Pts',(-33.35,-59.3174222737568,-63.975486542669));
#148769=CARTESIAN_POINT('Ctrl Pts',(-33.5881101525803,-60.3971457002532,
-61.2273317382593));
#148770=CARTESIAN_POINT('Ctrl Pts',(-33.35,-60.5242644024533,-61.2999665374096));
#148771=CARTESIAN_POINT('Ctrl Pts',(-33.35,-60.7669593817595,-61.4386408691297));
#148772=CARTESIAN_POINT('Origin',(-33.85,-60.7669593817595,-61.4386408691297));
#148773=CARTESIAN_POINT('Ctrl Pts',(-33.5881101525803,-60.3971457002532,
-61.2273317382593));
#148774=CARTESIAN_POINT('Ctrl Pts',(-33.5828208370019,-58.9513545007691,
-63.7641770795492));
#148775=CARTESIAN_POINT('Ctrl Pts',(-33.5772316679252,-57.489551829777,
-66.2915080112617));
#148776=CARTESIAN_POINT('Ctrl Pts',(-33.5712930253538,-56.006893899348,
-68.8064232518886));
#148777=CARTESIAN_POINT('Ctrl Pts',(-33.35,-61.3211699373828,-61.14995));
#148778=CARTESIAN_POINT('Ctrl Pts',(-33.35,-61.3211699373828,-60.64995));
#148779=CARTESIAN_POINT('Ctrl Pts',(-33.85,-61.3211699373828,-60.64995));
#148780=CARTESIAN_POINT('Ctrl Pts',(-33.35,-61.2129519920939,-61.1499500348135));
#148781=CARTESIAN_POINT('Ctrl Pts',(-33.3499999999981,-61.1490609397226,
-60.6983362970117));
#148782=CARTESIAN_POINT('Ctrl Pts',(-33.7991562663074,-61.1403193911197,
-60.64995));
#148783=CARTESIAN_POINT('Ctrl Pts',(-33.35,-61.1026558608156,-61.1739192791944));
#148784=CARTESIAN_POINT('Ctrl Pts',(-33.35,-60.9832965997767,-60.7797248720816));
#148785=CARTESIAN_POINT('Ctrl Pts',(-33.7471512515707,-60.9562715767294,
-60.6978885776012));
#148786=CARTESIAN_POINT('Ctrl Pts',(-33.35,-60.9082690803677,-61.269817357096));
#148787=CARTESIAN_POINT('Ctrl Pts',(-33.35,-60.7117483921024,-60.9965405405777));
#148788=CARTESIAN_POINT('Ctrl Pts',(-33.6552207448938,-60.6322769136983,
-60.8896846949796));
#148789=CARTESIAN_POINT('Ctrl Pts',(-33.35,-60.8219736344732,-61.3423603399148));
#148790=CARTESIAN_POINT('Ctrl Pts',(-33.3499999999996,-60.5960155996905,
-61.1331508909766));
#148791=CARTESIAN_POINT('Ctrl Pts',(-33.6142503615382,-60.4886315879339,
-61.034824258355));
#148792=CARTESIAN_POINT('Ctrl Pts',(-33.35,-60.7669593817595,-61.4386408691297));
#148793=CARTESIAN_POINT('Ctrl Pts',(-33.35,-60.5242644024533,-61.2999665374096));
#148794=CARTESIAN_POINT('Ctrl Pts',(-33.5881101525803,-60.3971457002532,
-61.2273317382593));
#148795=CARTESIAN_POINT('Origin',(-32.85,-72.58000002,-55.24995));
#148796=CARTESIAN_POINT('',(-32.85,-73.08000002,-174.34995));
#148797=CARTESIAN_POINT('Origin',(-32.85,-72.58000002,-174.34995));
#148798=CARTESIAN_POINT('',(-32.85,-73.08000002,-58.24995));
#148799=CARTESIAN_POINT('Origin',(-32.85,-70.08000002,-174.34995));
#148800=CARTESIAN_POINT('Origin',(-32.85,-70.08000002,-174.34995));
#148801=CARTESIAN_POINT('Origin',(0.,-12.9675000200281,-61.64995));
#148802=CARTESIAN_POINT('',(-30.7601599624812,36.3431985357226,-61.2273317382593));
#148803=CARTESIAN_POINT('',(-36.7137393100582,32.0861766206928,-61.2273317382593));
#148804=CARTESIAN_POINT('Origin',(0.,-12.9675000200281,-61.2273317382593));
#148805=CARTESIAN_POINT('Ctrl Pts',(-37.,33.02054075664,-60.64995));
#148806=CARTESIAN_POINT('Ctrl Pts',(-36.9450144953722,32.8396166159335,
-60.64995));
#148807=CARTESIAN_POINT('Ctrl Pts',(-36.8889168804295,32.6559426968113,
-60.6963841656953));
#148808=CARTESIAN_POINT('Ctrl Pts',(-36.8135029743542,32.4100449984504,
-60.8387768064376));
#148809=CARTESIAN_POINT('Ctrl Pts',(-36.7895122380439,32.3319990572285,
-60.8990185151424));
#148810=CARTESIAN_POINT('Ctrl Pts',(-36.7467810375704,32.1932186054134,
-61.0450197081848));
#148811=CARTESIAN_POINT('Ctrl Pts',(-36.7283245477951,32.1334017245463,
-61.1290643654114));
#148812=CARTESIAN_POINT('Ctrl Pts',(-36.7137393100582,32.0861766206928,
-61.2273317382593));
#148813=CARTESIAN_POINT('Ctrl Pts',(-30.7601599624812,36.3431985357226,
-61.2273317382593));
#148814=CARTESIAN_POINT('Ctrl Pts',(-30.7833440352389,36.4311997587239,
-61.0408976853214));
#148815=CARTESIAN_POINT('Ctrl Pts',(-30.820204224048,36.5713423922847,-60.8940610213177));
#148816=CARTESIAN_POINT('Ctrl Pts',(-30.9048607560821,36.8949030802612,
-60.6989334962026));
#148817=CARTESIAN_POINT('Ctrl Pts',(-30.9524183405754,37.0774198714491,
-60.64995));
#148818=CARTESIAN_POINT('Ctrl Pts',(-31.,37.2609769076718,-60.64995));
#148819=CARTESIAN_POINT('Origin',(-31.,-9.33460238845303,-61.14995));
#148820=CARTESIAN_POINT('Origin',(-31.,37.2609769076718,-61.14995));
#148821=CARTESIAN_POINT('Origin',(-37.,-12.9675000200281,-61.14995));
#148822=CARTESIAN_POINT('Origin',(-37.,33.02054075664,-61.14995));
#148823=CARTESIAN_POINT('Ctrl Pts',(-30.5,36.7276789742547,-61.4386408691297));
#148824=CARTESIAN_POINT('Ctrl Pts',(-30.5,36.4678387256643,-61.2958335593366));
#148825=CARTESIAN_POINT('Ctrl Pts',(-30.7601599624812,36.3431985357226,
-61.2273317382593));
#148826=CARTESIAN_POINT('Ctrl Pts',(-30.5,36.7789093803379,-61.3454266101228));
#148827=CARTESIAN_POINT('Ctrl Pts',(-30.5,36.536757012545,-61.1328271281761));
#148828=CARTESIAN_POINT('Ctrl Pts',(-30.7833440352389,36.4311997587239,
-61.0408976853214));
#148829=CARTESIAN_POINT('Ctrl Pts',(-30.5,36.8604662025248,-61.2720055170969));
#148830=CARTESIAN_POINT('Ctrl Pts',(-30.5000000000002,36.6495790716841,
-60.9942767827739));
#148831=CARTESIAN_POINT('Ctrl Pts',(-30.820204224048,36.5713423922847,-60.8940610213177));
#148832=CARTESIAN_POINT('Ctrl Pts',(-30.5,37.0485310665384,-61.1744417416632));
#148833=CARTESIAN_POINT('Ctrl Pts',(-30.4999999999998,36.921160791843,-60.7754981362285));
#148834=CARTESIAN_POINT('Ctrl Pts',(-30.9048607560821,36.8949030802612,
-60.6989334962026));
#148835=CARTESIAN_POINT('Ctrl Pts',(-30.5,37.1545174137893,-61.1499500119967));
#148836=CARTESIAN_POINT('Ctrl Pts',(-30.5,37.0857740751484,-60.6953661941756));
#148837=CARTESIAN_POINT('Ctrl Pts',(-30.9524183405754,37.0774198714491,
-60.64995));
#148838=CARTESIAN_POINT('Ctrl Pts',(-30.5,37.2609769076718,-61.14995));
#148839=CARTESIAN_POINT('Ctrl Pts',(-30.5,37.2609769076718,-60.64995));
#148840=CARTESIAN_POINT('Ctrl Pts',(-31.,37.2609769076718,-60.64995));
#148841=CARTESIAN_POINT('Origin',(-31.,36.7276789742547,-61.4386408691296));
#148842=CARTESIAN_POINT('Ctrl Pts',(-30.7601599624812,36.3431985357226,
-61.2273317382593));
#148843=CARTESIAN_POINT('Ctrl Pts',(-30.5,36.4678387256643,-61.2958335593366));
#148844=CARTESIAN_POINT('Ctrl Pts',(-30.5,36.7276789742547,-61.4386408691296));
#148845=CARTESIAN_POINT('Ctrl Pts',(-30.7526164452201,34.1766563796975,
-65.1779528603621));
#148846=CARTESIAN_POINT('Ctrl Pts',(-30.5,34.3134045700868,-65.2278638132481));
#148847=CARTESIAN_POINT('Ctrl Pts',(-30.5,34.5564303542403,-65.3892634389964));
#148848=CARTESIAN_POINT('Ctrl Pts',(-30.7443983582191,31.9809814038522,
-69.1118639196982));
#148849=CARTESIAN_POINT('Ctrl Pts',(-30.5,32.1210861733241,-69.1599841087648));
#148850=CARTESIAN_POINT('Ctrl Pts',(-30.5,32.3553350664733,-69.3231754387568));
#148851=CARTESIAN_POINT('Ctrl Pts',(-30.7353076117347,29.741870145346,-73.0207363867641));
#148852=CARTESIAN_POINT('Ctrl Pts',(-30.5,29.8691857803939,-73.0938794170475));
#148853=CARTESIAN_POINT('Ctrl Pts',(-30.5,30.1096831288108,-73.2320455176344));
#148854=CARTESIAN_POINT('',(-30.735362854857,29.74186581737,-73.0207804888355));
#148855=CARTESIAN_POINT('Origin',(-31.,30.1096831288108,-73.2320455176344));
#148856=CARTESIAN_POINT('Ctrl Pts',(-30.7353076117299,29.7418701453522,
-73.0207363867594));
#148857=CARTESIAN_POINT('Ctrl Pts',(-30.7443983582191,31.9809814038522,
-69.1118639196982));
#148858=CARTESIAN_POINT('Ctrl Pts',(-30.7526164452201,34.1766563796975,
-65.1779528603621));
#148859=CARTESIAN_POINT('Ctrl Pts',(-30.7601599624812,36.3431985357226,
-61.2273317382593));
#148860=CARTESIAN_POINT('Ctrl Pts',(-30.5,28.920951499305,-78.1925828079988));
#148861=CARTESIAN_POINT('Ctrl Pts',(-30.5000000000003,28.4128149071901,
-78.1994146967941));
#148862=CARTESIAN_POINT('Ctrl Pts',(-31.0081211823014,28.4210588880653,
-78.1993225690759));
#148863=CARTESIAN_POINT('Ctrl Pts',(-30.5,28.9094064694558,-77.302118472504));
#148864=CARTESIAN_POINT('Ctrl Pts',(-30.4999999999984,28.4483980825612,
-77.3106418208197));
#148865=CARTESIAN_POINT('Ctrl Pts',(-30.9594146236477,28.4082208355605,
-77.2678456234727));
#148866=CARTESIAN_POINT('Ctrl Pts',(-30.5,29.002822674508,-76.426962221765));
#148867=CARTESIAN_POINT('Ctrl Pts',(-30.5,28.579933321534,-76.3966655405999));
#148868=CARTESIAN_POINT('Ctrl Pts',(-30.9113712398487,28.5120100836853,
-76.353449058608));
#148869=CARTESIAN_POINT('Ctrl Pts',(-30.5,29.3028136269337,-75.1629449138939));
#148870=CARTESIAN_POINT('Ctrl Pts',(-30.5,28.9539620571574,-75.0718448818203));
#148871=CARTESIAN_POINT('Ctrl Pts',(-30.8418282567564,28.8453229371035,
-75.0340563370096));
#148872=CARTESIAN_POINT('Ctrl Pts',(-30.5,29.4252185218281,-74.758955076818));
#148873=CARTESIAN_POINT('Ctrl Pts',(-30.5000000000007,29.0970410698504,
-74.6573521788374));
#148874=CARTESIAN_POINT('Ctrl Pts',(-30.8195774733883,28.9813262599642,
-74.6125704712075));
#148875=CARTESIAN_POINT('Ctrl Pts',(-30.5,29.7412533702373,-73.9312213579753));
#148876=CARTESIAN_POINT('Ctrl Pts',(-30.4999999999992,29.4573184808354,
-73.8131874683998));
#148877=CARTESIAN_POINT('Ctrl Pts',(-30.7739516476249,29.3324729246049,
-73.7493614137364));
#148878=CARTESIAN_POINT('Ctrl Pts',(-30.5,29.9412605039864,-73.5090015627542));
#148879=CARTESIAN_POINT('Ctrl Pts',(-30.5000000000002,29.6801451335267,
-73.3815386187724));
#148880=CARTESIAN_POINT('Ctrl Pts',(-30.7506559835889,29.5547110389812,
-73.3092557539648));
#148881=CARTESIAN_POINT('Ctrl Pts',(-30.5,30.1841529915896,-73.1054052864862));
#148882=CARTESIAN_POINT('Ctrl Pts',(-30.5,29.9511540345493,-72.9650282514353));
#148883=CARTESIAN_POINT('Ctrl Pts',(-30.7283768517831,29.8245792311644,
-72.888770763772));
#148884=CARTESIAN_POINT('Origin',(-31.,28.91999998,-78.0460091084363));
#148885=CARTESIAN_POINT('Ctrl Pts',(-31.,28.41999998,-78.0460091084363));
#148886=CARTESIAN_POINT('Ctrl Pts',(-30.9915553765912,28.4199999839581,
-77.8845784212935));
#148887=CARTESIAN_POINT('Ctrl Pts',(-30.9831189817359,28.4236427988899,
-77.7236551810799));
#148888=CARTESIAN_POINT('Ctrl Pts',(-30.974710992956,28.4308536388649,-77.5632621201644));
#148889=CARTESIAN_POINT('Ctrl Pts',(-30.9662475726578,28.4381120178909,
-77.4018116326618));
#148890=CARTESIAN_POINT('Ctrl Pts',(-30.9578122144729,28.4489851481422,
-77.240897706449));
#148891=CARTESIAN_POINT('Ctrl Pts',(-30.9494053624499,28.4634423631753,
-77.0805267505334));
#148892=CARTESIAN_POINT('Ctrl Pts',(-30.9410119089526,28.477876536841,-76.9204113878366));
#148893=CARTESIAN_POINT('Ctrl Pts',(-30.9326460542808,28.4958831701324,
-76.7608365749435));
#148894=CARTESIAN_POINT('Ctrl Pts',(-30.9242998354382,28.5174821139553,
-76.6018020101865));
#148895=CARTESIAN_POINT('Ctrl Pts',(-30.9160313168687,28.5388799794379,
-76.4442479995983));
#148896=CARTESIAN_POINT('Ctrl Pts',(-30.9077812401549,28.5638036464743,
-76.287223543863));
#148897=CARTESIAN_POINT('Ctrl Pts',(-30.8995458905796,28.5923228488236,
-76.1307320214001));
#148898=CARTESIAN_POINT('Ctrl Pts',(-30.8914871613302,28.620230410979,-75.9775967114978));
#148899=CARTESIAN_POINT('Ctrl Pts',(-30.8834417951,28.6515812866277,-75.8249711322362));
#148900=CARTESIAN_POINT('Ctrl Pts',(-30.8754216976956,28.6864860901755,
-75.6728712878223));
#148901=CARTESIAN_POINT('Ctrl Pts',(-30.8716293533375,28.7029910062798,
-75.6009500931339));
#148902=CARTESIAN_POINT('Ctrl Pts',(-30.8678429521625,28.7202911839302,
-75.5291466906985));
#148903=CARTESIAN_POINT('Ctrl Pts',(-30.8640657072001,28.7384015524274,
-75.4574643697372));
#148904=CARTESIAN_POINT('Ctrl Pts',(-30.8560438465024,28.7768631440684,
-75.3052302416943));
#148905=CARTESIAN_POINT('Ctrl Pts',(-30.8480465637921,28.8190554047428,
-75.1532523926285));
#148906=CARTESIAN_POINT('Ctrl Pts',(-30.8400772928907,28.86505678019,-75.0020584970304));
#148907=CARTESIAN_POINT('Ctrl Pts',(-30.8322415679512,28.9102872823649,
-74.8533982503052));
#148908=CARTESIAN_POINT('Ctrl Pts',(-30.8244332481999,28.9592007097099,
-74.7054961433376));
#148909=CARTESIAN_POINT('Ctrl Pts',(-30.816683261254,29.0118331998908,-74.5588697982428));
#148910=CARTESIAN_POINT('Ctrl Pts',(-30.8103937252398,29.0545473289367,
-74.4398745425673));
#148911=CARTESIAN_POINT('Ctrl Pts',(-30.804143211839,29.0997102947523,-74.3217198951437));
#148912=CARTESIAN_POINT('Ctrl Pts',(-30.7979595444717,29.1473196130014,
-74.2046886808605));
#148913=CARTESIAN_POINT('Ctrl Pts',(-30.7918740622196,29.1941729839906,
-74.0895157041872));
#148914=CARTESIAN_POINT('Ctrl Pts',(-30.7858770793326,29.243410990576,-73.975346469923));
#148915=CARTESIAN_POINT('Ctrl Pts',(-30.7799226196483,29.2951820844478,
-73.862212594861));
#148916=CARTESIAN_POINT('Ctrl Pts',(-30.7740541865778,29.3462052192879,
-73.7507132130523));
#148917=CARTESIAN_POINT('Ctrl Pts',(-30.7682267315409,29.3996893836541,
-73.64021925808));
#148918=CARTESIAN_POINT('Ctrl Pts',(-30.7624318804288,29.4557967629243,
-73.5307896724718));
#148919=CARTESIAN_POINT('Ctrl Pts',(-30.7567739030089,29.5105788925869,
-73.4239448006263));
#148920=CARTESIAN_POINT('Ctrl Pts',(-30.751146830599,29.5678624292832,-73.3181144970074));
#148921=CARTESIAN_POINT('Ctrl Pts',(-30.7455806691336,29.6278083791469,
-73.2133836177019));
#148922=CARTESIAN_POINT('Ctrl Pts',(-30.7421458129149,29.6648007876413,
-73.1487546064333));
#148923=CARTESIAN_POINT('Ctrl Pts',(-30.7387349098385,29.7028072292658,
-73.0845448640455));
#148924=CARTESIAN_POINT('Ctrl Pts',(-30.735362854857,29.74186581737,-73.0207804888355));
#148925=CARTESIAN_POINT('Origin',(-31.,28.91999998,-55.24995));
#148926=CARTESIAN_POINT('Origin',(-30.,43.91999998,-58.24995));
#148927=CARTESIAN_POINT('Origin',(-30.,43.91999998,-58.24995));
#148928=CARTESIAN_POINT('Origin',(0.,43.91999998,-58.24995));
#148929=CARTESIAN_POINT('Origin',(-29.5,43.91999998,-58.24995));
#148930=CARTESIAN_POINT('Origin',(-29.5,43.91999998,-58.24995));
#148931=CARTESIAN_POINT('Origin',(-28.5,28.91999998,-55.24995));
#148932=CARTESIAN_POINT('Origin',(-28.5,28.91999998,-80.9397703408579));
#148933=CARTESIAN_POINT('Ctrl Pts',(-29.,30.190901134448,-76.1489606194832));
#148934=CARTESIAN_POINT('Ctrl Pts',(-29.,29.4220372877054,-75.6687700201129));
#148935=CARTESIAN_POINT('Ctrl Pts',(-28.2332370915911,29.8322352061969,
-75.9248722755917));
#148936=CARTESIAN_POINT('Ctrl Pts',(-29.,29.9217980586497,-76.5811393756123));
#148937=CARTESIAN_POINT('Ctrl Pts',(-29.,29.1809262360145,-76.1656388830817));
#148938=CARTESIAN_POINT('Ctrl Pts',(-28.2574251716161,29.5332350272111,
-76.376269388315));
#148939=CARTESIAN_POINT('Ctrl Pts',(-29.,29.7057519229925,-77.032432603564));
#148940=CARTESIAN_POINT('Ctrl Pts',(-28.9999999999999,28.9849557677507,
-76.6882938526006));
#148941=CARTESIAN_POINT('Ctrl Pts',(-28.2826568860398,29.2931653796995,
-76.8479190563244));
#148942=CARTESIAN_POINT('Ctrl Pts',(-29.,29.392736442598,-77.861168463682));
#148943=CARTESIAN_POINT('Ctrl Pts',(-29.,28.7176256604522,-77.6280825227319));
#148944=CARTESIAN_POINT('Ctrl Pts',(-28.3289101078372,28.945348491788,-77.7145676490796));
#148945=CARTESIAN_POINT('Ctrl Pts',(-29.,29.2801830215621,-78.2330925203216));
#148946=CARTESIAN_POINT('Ctrl Pts',(-29.,28.6258554431304,-78.0379074931216));
#148947=CARTESIAN_POINT('Ctrl Pts',(-28.3496415967673,28.8202788507468,
-78.1036928430455));
#148948=CARTESIAN_POINT('Ctrl Pts',(-29.,29.0997153099535,-78.9928975231766));
#148949=CARTESIAN_POINT('Ctrl Pts',(-29.,28.4904715640779,-78.8635127668171));
#148950=CARTESIAN_POINT('Ctrl Pts',(-28.391922778916,28.6197368000676,-78.8990673308349));
#148951=CARTESIAN_POINT('Ctrl Pts',(-29.,29.0321487487139,-79.3807788748604));
#148952=CARTESIAN_POINT('Ctrl Pts',(-29.,28.4443634216833,-79.2803384248115));
#148953=CARTESIAN_POINT('Ctrl Pts',(-28.4134719614193,28.5446520387322,
-79.3053196265795));
#148954=CARTESIAN_POINT('Ctrl Pts',(-29.,28.9298976880956,-80.2665661129666));
#148955=CARTESIAN_POINT('Ctrl Pts',(-29.,28.3932524579211,-80.2165321508882));
#148956=CARTESIAN_POINT('Ctrl Pts',(-28.4625827973001,28.4310142561314,
-80.23358931143));
#148957=CARTESIAN_POINT('Ctrl Pts',(-29.,28.9090504215435,-80.7677709009127));
#148958=CARTESIAN_POINT('Ctrl Pts',(-29.,28.3982322973888,-80.7457941266633));
#148959=CARTESIAN_POINT('Ctrl Pts',(-28.4902997525053,28.4078381678252,
-80.7592040367449));
#148960=CARTESIAN_POINT('Ctrl Pts',(-29.,28.9253917285729,-81.2725388309494));
#148961=CARTESIAN_POINT('Ctrl Pts',(-29.,28.4434678656906,-81.2883860649699));
#148962=CARTESIAN_POINT('Ctrl Pts',(-28.5181235174212,28.4259824926159,
-81.288955297043));
#148963=CARTESIAN_POINT('Origin',(-28.5,30.0207919771236,-76.4370443259982));
#148964=CARTESIAN_POINT('Ctrl Pts',(-28.2496026843433,29.6431021904052,
-76.2257353081032));
#148965=CARTESIAN_POINT('Ctrl Pts',(-28.2550962738409,29.5820653332084,
-76.3283221218245));
#148966=CARTESIAN_POINT('Ctrl Pts',(-28.2606732058844,29.5238127198801,
-76.4318902828666));
#148967=CARTESIAN_POINT('Ctrl Pts',(-28.2662832665929,29.4681738066383,
-76.5363451683756));
#148968=CARTESIAN_POINT('Ctrl Pts',(-28.2719809006041,29.4116663674314,
-76.6424305993962));
#148969=CARTESIAN_POINT('Ctrl Pts',(-28.2777129255254,29.3578541761501,
-76.749430806199));
#148970=CARTESIAN_POINT('Ctrl Pts',(-28.283468252918,29.3065658506586,-76.8572811154413));
#148971=CARTESIAN_POINT('Ctrl Pts',(-28.2893486242973,29.2541632016442,
-76.9674746506592));
#148972=CARTESIAN_POINT('Ctrl Pts',(-28.2952535950716,29.2043946076021,
-77.0785558251055));
#148973=CARTESIAN_POINT('Ctrl Pts',(-28.3012106132358,29.1570952891048,
-77.1904887281123));
#148974=CARTESIAN_POINT('Ctrl Pts',(-28.3037621110354,29.1368361420388,
-77.2384315995022));
#148975=CARTESIAN_POINT('Ctrl Pts',(-28.3063236154331,29.1170302805272,
-77.2865311147115));
#148976=CARTESIAN_POINT('Ctrl Pts',(-28.3088992066467,29.0976661808502,
-77.3347860946956));
#148977=CARTESIAN_POINT('Ctrl Pts',(-28.3159268080949,29.0448304768712,
-77.4664516965293));
#148978=CARTESIAN_POINT('Ctrl Pts',(-28.3230277381525,28.9952999216831,
-77.599259998328));
#148979=CARTESIAN_POINT('Ctrl Pts',(-28.330171515793,28.9489397170328,-77.7331526861724));
#148980=CARTESIAN_POINT('Ctrl Pts',(-28.3374902152524,28.9014443410868,
-77.8703238568681));
#148981=CARTESIAN_POINT('Ctrl Pts',(-28.3448543969108,28.8572757382811,
-78.008633563989));
#148982=CARTESIAN_POINT('Ctrl Pts',(-28.3522654021615,28.816321248413,-78.148048277229));
#148983=CARTESIAN_POINT('Ctrl Pts',(-28.3584846660916,28.7819525260875,
-78.2650441324539));
#148984=CARTESIAN_POINT('Ctrl Pts',(-28.3647377201567,28.7498477794226,
-78.3828188721135));
#148985=CARTESIAN_POINT('Ctrl Pts',(-28.3710388306812,28.7199623512604,
-78.5013644791918));
#148986=CARTESIAN_POINT('Ctrl Pts',(-28.3798275485611,28.6782784931823,
-78.6667105546906));
#148987=CARTESIAN_POINT('Ctrl Pts',(-28.3886940030905,28.6409287992575,
-78.8335385750663));
#148988=CARTESIAN_POINT('Ctrl Pts',(-28.3975938613373,28.6079545239895,
-79.001265263691));
#148989=CARTESIAN_POINT('Ctrl Pts',(-28.4065760881628,28.5746750703563,
-79.1705442701821));
#148990=CARTESIAN_POINT('Ctrl Pts',(-28.4155919241668,28.5458521783277,
-79.3407383620272));
#148991=CARTESIAN_POINT('Ctrl Pts',(-28.4246146635513,28.5214788033205,
-79.5112521906048));
#148992=CARTESIAN_POINT('Ctrl Pts',(-28.4281545108594,28.5119165160557,
-79.5781490487952));
#148993=CARTESIAN_POINT('Ctrl Pts',(-28.4316956575249,28.5030385796938,
-79.6450951903288));
#148994=CARTESIAN_POINT('Ctrl Pts',(-28.4352374739099,28.494842646572,-79.7120549851513));
#148995=CARTESIAN_POINT('Ctrl Pts',(-28.4433977632336,28.4759593453834,
-79.8663293007611));
#148996=CARTESIAN_POINT('Ctrl Pts',(-28.4515635189675,28.4606589509008,
-80.0209567625393));
#148997=CARTESIAN_POINT('Ctrl Pts',(-28.4597425456804,28.4489176045266,
-80.1759457293561));
#148998=CARTESIAN_POINT('Ctrl Pts',(-28.4679114902169,28.4371907315526,
-80.3307436433532));
#148999=CARTESIAN_POINT('Ctrl Pts',(-28.4760944511414,28.4290144033317,
-80.4859028728578));
#149000=CARTESIAN_POINT('Ctrl Pts',(-28.4842901842144,28.4244151626594,
-80.641424208971));
#149001=CARTESIAN_POINT('Ctrl Pts',(-28.4895232658188,28.4214784879847,
-80.7407265942301));
#149002=CARTESIAN_POINT('Ctrl Pts',(-28.4947613318242,28.4200012042165,
-80.8401764231172));
#149003=CARTESIAN_POINT('Ctrl Pts',(-28.5,28.4199999807603,-80.9397703408579));
#149004=CARTESIAN_POINT('Ctrl Pts',(-28.2496025504691,29.6431021990262,
-76.2257351951278));
#149005=CARTESIAN_POINT('Ctrl Pts',(-29.,29.2642096076976,-76.0137531166873));
#149006=CARTESIAN_POINT('Ctrl Pts',(-29.,30.0207919771236,-76.4370443259982));
#149007=CARTESIAN_POINT('Ctrl Pts',(-28.2608542879989,32.4163856120597,
-71.2554899486297));
#149008=CARTESIAN_POINT('Ctrl Pts',(-29.,32.0024463153694,-71.1716406391234));
#149009=CARTESIAN_POINT('Ctrl Pts',(-29.,32.8015320477175,-71.4668042994815));
#149010=CARTESIAN_POINT('Ctrl Pts',(-28.2706820191605,35.1297158291743,
-66.2515800426151));
#149011=CARTESIAN_POINT('Ctrl Pts',(-28.9999999999899,34.7556963975018,
-66.1533445021367));
#149012=CARTESIAN_POINT('Ctrl Pts',(-29.,35.5206920342409,-66.4628921538691));
#149013=CARTESIAN_POINT('Ctrl Pts',(-28.2795019009908,37.8065307949999,
-61.2273317382593));
#149014=CARTESIAN_POINT('Ctrl Pts',(-29.,37.4942143736512,-61.0606306836509));
#149015=CARTESIAN_POINT('Ctrl Pts',(-29.,38.2024209812184,-61.4386408691297));
#149016=CARTESIAN_POINT('Origin',(-40.,31.080768958446,-179.64995));
#149017=CARTESIAN_POINT('',(-39.3277310924369,30.340461916791,-179.64995));
#149018=CARTESIAN_POINT('Origin',(-38.5,46.41999998,-129.34995));
#149019=CARTESIAN_POINT('Origin',(-38.5,46.41999998,-58.24995));
#149020=CARTESIAN_POINT('Origin',(-38.5,43.91999998,-58.24995));
#149021=CARTESIAN_POINT('Origin',(-38.5,43.91999998,-58.24995));
#149022=CARTESIAN_POINT('Origin',(0.,43.91999998,-58.24995));
#149023=CARTESIAN_POINT('Origin',(-38.,43.91999998,-58.24995));
#149024=CARTESIAN_POINT('Origin',(-38.,43.91999998,-58.24995));
#149025=CARTESIAN_POINT('Origin',(-37.,28.91999998,-55.24995));
#149026=CARTESIAN_POINT('Origin',(-37.,28.91999998,-70.4461836365688));
#149027=CARTESIAN_POINT('Ctrl Pts',(-37.5,30.3198029183707,-64.9254179945125));
#149028=CARTESIAN_POINT('Ctrl Pts',(-37.5,29.4819543139285,-64.4114488783659));
#149029=CARTESIAN_POINT('Ctrl Pts',(-36.7055659807485,29.9753365781889,
-64.7141088636423));
#149030=CARTESIAN_POINT('Ctrl Pts',(-37.5,30.066275812609,-65.3387061138468));
#149031=CARTESIAN_POINT('Ctrl Pts',(-37.5,29.2617307842025,-64.8907595368038));
#149032=CARTESIAN_POINT('Ctrl Pts',(-36.7276066422259,29.6936558584646,
-65.1425806750807));
#149033=CARTESIAN_POINT('Ctrl Pts',(-37.5,29.8583501338385,-65.770493027413));
#149034=CARTESIAN_POINT('Ctrl Pts',(-37.4999999999999,29.0782932545581,
-65.3939122854256));
#149035=CARTESIAN_POINT('Ctrl Pts',(-36.7506399492972,29.4626112609503,
-65.5904100084171));
#149036=CARTESIAN_POINT('Ctrl Pts',(-37.5,29.5081290337376,-66.6603034853058));
#149037=CARTESIAN_POINT('Ctrl Pts',(-37.5,28.7875108426025,-66.3978618624443));
#149038=CARTESIAN_POINT('Ctrl Pts',(-36.7981064172734,29.0734767074675,
-66.5135522731121));
#149039=CARTESIAN_POINT('Ctrl Pts',(-37.5,29.3662299161008,-67.1188991703195));
#149040=CARTESIAN_POINT('Ctrl Pts',(-37.5,28.6734901542511,-66.902255679337));
#149041=CARTESIAN_POINT('Ctrl Pts',(-36.8225713421442,28.9158110192433,
-66.9894827414662));
#149042=CARTESIAN_POINT('Ctrl Pts',(-37.5,29.0270605890893,-68.5274557979285));
#149043=CARTESIAN_POINT('Ctrl Pts',(-37.5,28.43212483966,-68.3736721849867));
#149044=CARTESIAN_POINT('Ctrl Pts',(-36.8977082013987,28.5389562140588,
-68.4518423383231));
#149045=CARTESIAN_POINT('Ctrl Pts',(-37.5,28.9199999811121,-69.4807175010263));
#149046=CARTESIAN_POINT('Ctrl Pts',(-37.5,28.3657190858733,-69.3869874906105));
#149047=CARTESIAN_POINT('Ctrl Pts',(-36.9485508209842,28.41999998,-69.4422434553462));
#149048=CARTESIAN_POINT('Ctrl Pts',(-37.5,28.91999998,-70.4461836365688));
#149049=CARTESIAN_POINT('Ctrl Pts',(-37.5,28.41999998,-70.4461836365687));
#149050=CARTESIAN_POINT('Ctrl Pts',(-37.,28.41999998,-70.4461836365688));
#149051=CARTESIAN_POINT('',(-36.7055660333102,29.9753365541058,-64.7141088836342));
#149052=CARTESIAN_POINT('Origin',(-37.,30.3198029183592,-64.9254179945062));
#149053=CARTESIAN_POINT('Ctrl Pts',(-36.7055659821207,29.9753365605306,
-64.714108890491));
#149054=CARTESIAN_POINT('Ctrl Pts',(-36.7276066431882,29.6936558488113,
-65.1425806937914));
#149055=CARTESIAN_POINT('Ctrl Pts',(-36.750639949793,29.4626112568857,-65.5904100180595));
#149056=CARTESIAN_POINT('Ctrl Pts',(-36.7981064172734,29.0734767074675,
-66.5135522731121));
#149057=CARTESIAN_POINT('Ctrl Pts',(-36.8225713421442,28.9158110192433,
-66.9894827414662));
#149058=CARTESIAN_POINT('Ctrl Pts',(-36.8977082013987,28.5389562140588,
-68.4518423383231));
#149059=CARTESIAN_POINT('Ctrl Pts',(-36.9485508209842,28.41999998,-69.4422434553462));
#149060=CARTESIAN_POINT('Ctrl Pts',(-37.,28.41999998,-70.4461836365688));
#149061=CARTESIAN_POINT('Ctrl Pts',(-36.7055659807482,29.9753365781776,
-64.714108863636));
#149062=CARTESIAN_POINT('Ctrl Pts',(-37.5,29.4819543139165,-64.4114488783587));
#149063=CARTESIAN_POINT('Ctrl Pts',(-37.5,30.3198029183591,-64.9254179945063));
#149064=CARTESIAN_POINT('Ctrl Pts',(-36.7083606505135,30.6839990376866,
-63.5549861665061));
#149065=CARTESIAN_POINT('Ctrl Pts',(-37.5,30.1937476367692,-63.2670920970213));
#149066=CARTESIAN_POINT('Ctrl Pts',(-37.5,31.0308541172825,-63.7662953234662));
#149067=CARTESIAN_POINT('Ctrl Pts',(-36.7110836457466,31.3874027455588,
-62.3925965705953));
#149068=CARTESIAN_POINT('Ctrl Pts',(-37.5,30.9051975556495,-62.1106946535587));
#149069=CARTESIAN_POINT('Ctrl Pts',(-37.5,31.7365266751429,-62.6039057229559));
#149070=CARTESIAN_POINT('Ctrl Pts',(-36.7137393100582,32.0861766206928,
-61.2273317382593));
#149071=CARTESIAN_POINT('Ctrl Pts',(-37.5,31.6156971887288,-60.9443257831195));
#149072=CARTESIAN_POINT('Ctrl Pts',(-37.5,32.4374646344434,-61.4386408691296));
#149073=CARTESIAN_POINT('Origin',(-37.,32.4374646344434,-61.4386408691297));
#149074=CARTESIAN_POINT('Ctrl Pts',(-36.7137393100582,32.0861766206928,
-61.2273317382593));
#149075=CARTESIAN_POINT('Ctrl Pts',(-36.7110837808245,31.3874382843756,
-62.3925373065787));
#149076=CARTESIAN_POINT('Ctrl Pts',(-36.7083607806502,30.6840320430885,
-63.5549321813014));
#149077=CARTESIAN_POINT('Ctrl Pts',(-36.7055659807394,29.9753365781839,
-64.7141088636381));
#149078=CARTESIAN_POINT('Ctrl Pts',(-37.5,33.02054075664,-61.14995));
#149079=CARTESIAN_POINT('Ctrl Pts',(-37.5,33.0205407566399,-60.64995));
#149080=CARTESIAN_POINT('Ctrl Pts',(-37.,33.02054075664,-60.64995));
#149081=CARTESIAN_POINT('Ctrl Pts',(-37.5,32.9079637588407,-61.149950027061));
#149082=CARTESIAN_POINT('Ctrl Pts',(-37.4999999999984,32.829451263505,-60.5918750690658));
#149083=CARTESIAN_POINT('Ctrl Pts',(-36.9450144953722,32.8396166159335,
-60.64995));
#149084=CARTESIAN_POINT('Ctrl Pts',(-37.5,32.7934674553098,-61.173167066129));
#149085=CARTESIAN_POINT('Ctrl Pts',(-37.5,32.6176893530803,-60.5649300622629));
#149086=CARTESIAN_POINT('Ctrl Pts',(-36.8889168804295,32.6559426968113,
-60.6963841656953));
#149087=CARTESIAN_POINT('Ctrl Pts',(-37.5,32.6399623596936,-61.2443634115781));
#149088=CARTESIAN_POINT('Ctrl Pts',(-37.5,32.2741011266166,-60.5989161145872));
#149089=CARTESIAN_POINT('Ctrl Pts',(-36.8135029743542,32.4100449984504,
-60.8387768064376));
#149090=CARTESIAN_POINT('Ctrl Pts',(-37.5,32.5912011068259,-61.27448425119));
#149091=CARTESIAN_POINT('Ctrl Pts',(-37.5,32.1451108386466,-60.6268090630372));
#149092=CARTESIAN_POINT('Ctrl Pts',(-36.7895122380439,32.3319990572285,
-60.8990185151424));
#149093=CARTESIAN_POINT('Ctrl Pts',(-37.5,32.5044425233165,-61.3474848604736));
#149094=CARTESIAN_POINT('Ctrl Pts',(-37.4999999999999,31.876172903305,-60.7353807030111));
#149095=CARTESIAN_POINT('Ctrl Pts',(-36.7467810375704,32.1932186054134,
-61.0450197081848));
#149096=CARTESIAN_POINT('Ctrl Pts',(-37.5,32.4670287634048,-61.3894925929396));
#149097=CARTESIAN_POINT('Ctrl Pts',(-37.5,31.7388049050588,-60.8179479783099));
#149098=CARTESIAN_POINT('Ctrl Pts',(-36.7283245477951,32.1334017245463,
-61.1290643654114));
#149099=CARTESIAN_POINT('Ctrl Pts',(-37.5,32.4374646344434,-61.4386408691296));
#149100=CARTESIAN_POINT('Ctrl Pts',(-37.5,31.6156971887288,-60.9443257831194));
#149101=CARTESIAN_POINT('Ctrl Pts',(-36.7137393100582,32.0861766206928,
-61.2273317382593));
#149102=CARTESIAN_POINT('Origin',(0.,-12.9675000200281,-61.64995));
#149103=CARTESIAN_POINT('',(-43.0147613882085,26.1152677387813,-61.2273317382593));
#149104=CARTESIAN_POINT('',(-47.508501172308,20.508980519813,-61.2273317382593));
#149105=CARTESIAN_POINT('Origin',(0.,-12.9675000200281,-61.2273317382593));
#149106=CARTESIAN_POINT('Ctrl Pts',(-48.4322308821779,20.76999998,-60.64995));
#149107=CARTESIAN_POINT('Ctrl Pts',(-48.2513645254321,20.7193046642187,
-60.64995));
#149108=CARTESIAN_POINT('Ctrl Pts',(-48.0673245582317,20.6674580465872,
-60.6979267287055));
#149109=CARTESIAN_POINT('Ctrl Pts',(-47.7433968711081,20.5758225659973,
-60.8898150965897));
#149110=CARTESIAN_POINT('Ctrl Pts',(-47.5998785057972,20.5350112502637,
-61.0349912654872));
#149111=CARTESIAN_POINT('Ctrl Pts',(-47.508501172308,20.508980519813,-61.2273317382593));
#149112=CARTESIAN_POINT('Ctrl Pts',(-43.0147613882085,26.1152677387813,
-61.2273317382593));
#149113=CARTESIAN_POINT('Ctrl Pts',(-43.0636216624014,26.1311367864154,
-61.1268955825468));
#149114=CARTESIAN_POINT('Ctrl Pts',(-43.1254911751643,26.1512115744493,
-61.0418249229491));
#149115=CARTESIAN_POINT('Ctrl Pts',(-43.2683662178942,26.1974732479793,
-60.8948259755643));
#149116=CARTESIAN_POINT('Ctrl Pts',(-43.3469540657763,26.2228767030678,
-60.8357750676355));
#149117=CARTESIAN_POINT('Ctrl Pts',(-43.512870268579,26.2763890014657,-60.7418969884463));
#149118=CARTESIAN_POINT('Ctrl Pts',(-43.6010803778225,26.3047810522968,
-60.7070015638854));
#149119=CARTESIAN_POINT('Ctrl Pts',(-43.7785234711652,26.3617623367046,
-60.6613392327119));
#149120=CARTESIAN_POINT('Ctrl Pts',(-43.8687620016371,26.3906766531834,
-60.64995));
#149121=CARTESIAN_POINT('Ctrl Pts',(-43.9604906504041,26.41999998,-60.64995));
#149122=CARTESIAN_POINT('Origin',(-1.64641978096591E-14,26.4199999800001,
-61.14995));
#149123=CARTESIAN_POINT('Origin',(-43.9604906504041,26.41999998,-61.14995));
#149124=CARTESIAN_POINT('Origin',(83.2809572255632,20.76999998,-61.14995));
#149125=CARTESIAN_POINT('Origin',(-48.4322308821779,20.76999998,-61.14995));
#149126=CARTESIAN_POINT('Ctrl Pts',(-49.6616970192851,26.41999998,-171.64995));
#149127=CARTESIAN_POINT('Ctrl Pts',(-49.6616970192851,26.91999998,-171.64995));
#149128=CARTESIAN_POINT('Ctrl Pts',(-49.6616970192851,26.91999998,-171.14995));
#149129=CARTESIAN_POINT('Ctrl Pts',(-49.7951873628098,26.4108894799999,
-171.64995));
#149130=CARTESIAN_POINT('Ctrl Pts',(-49.7964789655964,26.91999998,-171.659148653595));
#149131=CARTESIAN_POINT('Ctrl Pts',(-49.8600119386601,26.91999998,-171.149950000016));
#149132=CARTESIAN_POINT('Ctrl Pts',(-49.9285770883077,26.4017858470187,
-171.675977326981));
#149133=CARTESIAN_POINT('Ctrl Pts',(-49.9258697838501,26.91999998,-171.69520402023));
#149134=CARTESIAN_POINT('Ctrl Pts',(-50.058177378641,26.91999998,-171.18899099047));
#149135=CARTESIAN_POINT('Ctrl Pts',(-50.1751906113998,26.3849548730131,
-171.776163607997));
#149136=CARTESIAN_POINT('Ctrl Pts',(-50.1586485796703,26.91999998,-171.809929875206));
#149137=CARTESIAN_POINT('Ctrl Pts',(-50.4245495045741,26.91999998,-171.339270411997));
#149138=CARTESIAN_POINT('Ctrl Pts',(-50.2882933630855,26.3772357931757,
-171.850283164393));
#149139=CARTESIAN_POINT('Ctrl Pts',(-50.2612232924101,26.9199999800027,
-171.888983273332));
#149140=CARTESIAN_POINT('Ctrl Pts',(-50.5925763632168,26.91999998,-171.450449746589));
#149141=CARTESIAN_POINT('Ctrl Pts',(-50.4770431819562,26.3643539233768,
-172.035403273234));
#149142=CARTESIAN_POINT('Ctrl Pts',(-50.4288800635612,26.9199999799973,
-172.075215659168));
#149143=CARTESIAN_POINT('Ctrl Pts',(-50.8729854484245,26.91999998,-171.728129909852));
#149144=CARTESIAN_POINT('Ctrl Pts',(-50.5526160245901,26.3591961991206,
-172.14633102856));
#149145=CARTESIAN_POINT('Ctrl Pts',(-50.493151129373,26.91999998,-172.18218244132));
#149146=CARTESIAN_POINT('Ctrl Pts',(-50.9852574060669,26.91999998,-171.894521542842));
#149147=CARTESIAN_POINT('Ctrl Pts',(-50.6547666904167,26.3522245814263,
-172.38820210671));
#149148=CARTESIAN_POINT('Ctrl Pts',(-50.5795844587924,26.91999998,-172.40972629816));
#149149=CARTESIAN_POINT('Ctrl Pts',(-51.1370137093498,26.91999998,-172.257328160063));
#149150=CARTESIAN_POINT('Ctrl Pts',(-50.6813043436918,26.3504134295228,
-172.51902671195));
#149151=CARTESIAN_POINT('Ctrl Pts',(-50.6012541744511,26.91999998,-172.529650273731));
#149152=CARTESIAN_POINT('Ctrl Pts',(-51.176438378046,26.91999998,-172.453565067926));
#149153=CARTESIAN_POINT('Ctrl Pts',(-50.6813043436922,26.35041342952,-172.64995));
#149154=CARTESIAN_POINT('Ctrl Pts',(-50.6012541744525,26.9199999800001,
-172.64995));
#149155=CARTESIAN_POINT('Ctrl Pts',(-51.176438378063,26.91999998,-172.64995));
#149156=CARTESIAN_POINT('',(-49.6616970192851,26.41999998,-171.64995));
#149157=CARTESIAN_POINT('Origin',(-49.6616970192851,26.41999998,-171.14995));
#149158=CARTESIAN_POINT('',(-50.676438378063,26.41999998,-172.64995));
#149159=CARTESIAN_POINT('Origin',(-51.176438378063,26.41999998,-172.64995));
#149160=CARTESIAN_POINT('Origin',(-51.176438378063,26.41999998,-172.64995));
#149161=CARTESIAN_POINT('Ctrl Pts',(-50.6813043436922,26.35041342952,-172.64995));
#149162=CARTESIAN_POINT('Ctrl Pts',(-50.6813043436918,26.3504134295228,
-172.51902671195));
#149163=CARTESIAN_POINT('Ctrl Pts',(-50.6547666904167,26.3522245814263,
-172.38820210671));
#149164=CARTESIAN_POINT('Ctrl Pts',(-50.5526160245901,26.3591961991206,
-172.14633102856));
#149165=CARTESIAN_POINT('Ctrl Pts',(-50.4770431819562,26.3643539233768,
-172.035403273234));
#149166=CARTESIAN_POINT('Ctrl Pts',(-50.2882933630855,26.3772357931757,
-171.850283164393));
#149167=CARTESIAN_POINT('Ctrl Pts',(-50.1751906113998,26.3849548730131,
-171.776163607997));
#149168=CARTESIAN_POINT('Ctrl Pts',(-49.9285770883077,26.4017858470187,
-171.675977326981));
#149169=CARTESIAN_POINT('Ctrl Pts',(-49.7951873628098,26.4108894799999,
-171.64995));
#149170=CARTESIAN_POINT('Ctrl Pts',(-49.6616970192851,26.41999998,-171.64995));
#149171=CARTESIAN_POINT('Origin',(-51.176438378063,26.41999998,-55.24995));
#149172=CARTESIAN_POINT('Origin',(-51.176438378063,26.41999998,-176.84995));
#149173=CARTESIAN_POINT('Origin',(83.2809572255632,27.41999998,-176.84995));
#149174=CARTESIAN_POINT('',(-57.,27.41999998,-177.34995));
#149175=CARTESIAN_POINT('Origin',(-57.,27.41999998,-176.84995));
#149176=CARTESIAN_POINT('',(-51.0358975433606,27.41999998,-177.34995));
#149177=CARTESIAN_POINT('',(-60.,27.41999998,-177.34995));
#149178=CARTESIAN_POINT('Ctrl Pts',(-51.176438378063,26.91999998,-176.84995));
#149179=CARTESIAN_POINT('Ctrl Pts',(-51.1764383780557,26.91999998,-176.981217345763));
#149180=CARTESIAN_POINT('Ctrl Pts',(-51.161291852844,26.9738865434699,-177.110943344657));
#149181=CARTESIAN_POINT('Ctrl Pts',(-51.1092579883806,27.1590066353435,
-177.29606343653));
#149182=CARTESIAN_POINT('Ctrl Pts',(-51.0727943880466,27.2887326342368,
-177.34995));
#149183=CARTESIAN_POINT('Ctrl Pts',(-51.0358975433606,27.41999998,-177.34995));
#149184=CARTESIAN_POINT('Origin',(-57.,27.41999998,-174.34995));
#149185=CARTESIAN_POINT('',(-60.,27.41999998,-174.34995));
#149186=CARTESIAN_POINT('Origin',(-59.5,27.41999998,-174.34995));
#149187=CARTESIAN_POINT('Origin',(-57.,27.41999998,-174.34995));
#149188=CARTESIAN_POINT('Origin',(-59.5,27.41999998,-55.24995));
#149189=CARTESIAN_POINT('',(-60.,27.41999998,-58.24995));
#149190=CARTESIAN_POINT('Origin',(-59.5,27.41999998,-58.24995));
#149191=CARTESIAN_POINT('',(-60.,27.41999998,-174.34995));
#149192=CARTESIAN_POINT('Origin',(-57.,27.41999998,-58.24995));
#149193=CARTESIAN_POINT('Origin',(-57.,27.41999998,-58.24995));
#149194=CARTESIAN_POINT('Ctrl Pts',(-43.3501517762232,26.91999998,-61.4386408691297));
#149195=CARTESIAN_POINT('Ctrl Pts',(-42.4913556541499,26.91999998,-60.8975655472507));
#149196=CARTESIAN_POINT('Ctrl Pts',(-43.0147613882086,26.1152677387813,
-61.2273317382593));
#149197=CARTESIAN_POINT('Ctrl Pts',(-43.3818037825525,26.91999998,-61.3884029511195));
#149198=CARTESIAN_POINT('Ctrl Pts',(-42.6316122966568,26.9199999800009,
-60.7676176413114));
#149199=CARTESIAN_POINT('Ctrl Pts',(-43.0636216624014,26.1311367864154,
-61.1268955825468));
#149200=CARTESIAN_POINT('Ctrl Pts',(-43.4218378639138,26.91999998,-61.3458874687825));
#149201=CARTESIAN_POINT('Ctrl Pts',(-42.7839211391678,26.91999998,-60.6895038034116));
#149202=CARTESIAN_POINT('Ctrl Pts',(-43.1254911751643,26.1512115744493,
-61.0418249229491));
#149203=CARTESIAN_POINT('Ctrl Pts',(-43.5142348068871,26.91999998,-61.2723879804742));
#149204=CARTESIAN_POINT('Ctrl Pts',(-43.0730867590013,26.91999998,-60.5931776502515));
#149205=CARTESIAN_POINT('Ctrl Pts',(-43.2683662178942,26.1974732479793,
-60.8948259755643));
#149206=CARTESIAN_POINT('Ctrl Pts',(-43.5650210354047,26.91999998,-61.2428625417913));
#149207=CARTESIAN_POINT('Ctrl Pts',(-43.2058848140176,26.9199999800003,
-60.57262210769));
#149208=CARTESIAN_POINT('Ctrl Pts',(-43.3469540657763,26.2228767030678,
-60.8357750676355));
#149209=CARTESIAN_POINT('Ctrl Pts',(-43.6721398787422,26.91999998,-61.1959234862494));
#149210=CARTESIAN_POINT('Ctrl Pts',(-43.4490485146957,26.9199999799997,
-60.5604852270767));
#149211=CARTESIAN_POINT('Ctrl Pts',(-43.512870268579,26.2763890014657,-60.7418969884463));
#149212=CARTESIAN_POINT('Ctrl Pts',(-43.7290408259741,26.91999998,-61.1784757886431));
#149213=CARTESIAN_POINT('Ctrl Pts',(-43.5624944559174,26.9199999800001,
-60.5672455602404));
#149214=CARTESIAN_POINT('Ctrl Pts',(-43.6010803778225,26.3047810522968,
-60.7070015638854));
#149215=CARTESIAN_POINT('Ctrl Pts',(-43.8433908708859,26.91999998,-61.1556446096555));
#149216=CARTESIAN_POINT('Ctrl Pts',(-43.7695073126827,26.9199999799999,
-60.5973801431191));
#149217=CARTESIAN_POINT('Ctrl Pts',(-43.7785234711652,26.3617623367046,
-60.6613392327119));
#149218=CARTESIAN_POINT('Ctrl Pts',(-43.901489846726,26.91999998,-61.1499500121981));
#149219=CARTESIAN_POINT('Ctrl Pts',(-43.8659505814334,26.91999998,-60.6197279239548));
#149220=CARTESIAN_POINT('Ctrl Pts',(-43.8687620016371,26.3906766531834,
-60.64995));
#149221=CARTESIAN_POINT('Ctrl Pts',(-43.9604906504041,26.91999998,-61.14995));
#149222=CARTESIAN_POINT('Ctrl Pts',(-43.9604906504041,26.91999998,-60.64995));
#149223=CARTESIAN_POINT('Ctrl Pts',(-43.9604906504041,26.41999998,-60.64995));
#149224=CARTESIAN_POINT('Origin',(-43.3501517762232,26.41999998,-61.4386408691297));
#149225=CARTESIAN_POINT('Ctrl Pts',(-43.0147613882085,26.1152677387813,
-61.2273317382593));
#149226=CARTESIAN_POINT('Ctrl Pts',(-42.4913556541499,26.91999998,-60.8975655472507));
#149227=CARTESIAN_POINT('Ctrl Pts',(-43.3501517762232,26.91999998,-61.4386408691297));
#149228=CARTESIAN_POINT('Ctrl Pts',(-42.2597213352523,26.1123501122717,
-62.4299407790815));
#149229=CARTESIAN_POINT('Ctrl Pts',(-41.7218722762073,26.9199999800149,
-62.1010809579055));
#149230=CARTESIAN_POINT('Ctrl Pts',(-42.5924607769204,26.91999998,-62.641249943458));
#149231=CARTESIAN_POINT('Ctrl Pts',(-41.4984253110313,26.1093585902154,
-63.6284728402189));
#149232=CARTESIAN_POINT('Ctrl Pts',(-40.950890457431,26.91999998,-63.291651632712));
#149233=CARTESIAN_POINT('Ctrl Pts',(-41.828377509759,26.91999998,-63.839782013441));
#149234=CARTESIAN_POINT('Ctrl Pts',(-40.7299249439368,26.1062890581501,
-64.8223083020179));
#149235=CARTESIAN_POINT('Ctrl Pts',(-40.1792441039523,26.91999998,-64.466463596043));
#149236=CARTESIAN_POINT('Ctrl Pts',(-41.0569324495432,26.91999998,-65.0336174328882));
#149237=CARTESIAN_POINT('',(-40.7299249193735,26.1062892385305,-64.8223083970342));
#149238=CARTESIAN_POINT('Origin',(-41.0569324495432,26.41999998,-65.0336174328882));
#149239=CARTESIAN_POINT('Ctrl Pts',(-40.7299249439368,26.1062890581501,
-64.8223083020179));
#149240=CARTESIAN_POINT('Ctrl Pts',(-41.4984715481572,26.1093587748547,
-63.6284010127));
#149241=CARTESIAN_POINT('Ctrl Pts',(-42.2597732523974,26.1123503129199,
-62.4298580866994));
#149242=CARTESIAN_POINT('Ctrl Pts',(-43.0147613882085,26.1152677387813,
-61.2273317382593));
#149243=CARTESIAN_POINT('Ctrl Pts',(-39.5144819943711,26.91999998,-71.6866097071051));
#149244=CARTESIAN_POINT('Ctrl Pts',(-39.0463811742787,26.9199999800001,
-71.7084369835555));
#149245=CARTESIAN_POINT('Ctrl Pts',(-39.0160373395819,26.4523138460616,
-71.7098742332801));
#149246=CARTESIAN_POINT('Ctrl Pts',(-39.4806747297125,26.91999998,-70.9435045713511));
#149247=CARTESIAN_POINT('Ctrl Pts',(-38.9720076653828,26.91999998,-70.912377553647));
#149248=CARTESIAN_POINT('Ctrl Pts',(-38.978537754162,26.4135029236992,-70.9394725339304));
#149249=CARTESIAN_POINT('Ctrl Pts',(-39.5061138838564,26.91999998,-70.2084683216835));
#149250=CARTESIAN_POINT('Ctrl Pts',(-38.9629719358347,26.91999998,-70.1446290088561));
#149251=CARTESIAN_POINT('Ctrl Pts',(-39.0068635113108,26.3751216436924,
-70.177811990567));
#149252=CARTESIAN_POINT('Ctrl Pts',(-39.6502847005361,26.91999998,-68.962325974017));
#149253=CARTESIAN_POINT('Ctrl Pts',(-39.0341587958529,26.91999998,-68.8494630385759));
#149254=CARTESIAN_POINT('Ctrl Pts',(-39.167181524895,26.3100882014274,-68.8871399937697));
#149255=CARTESIAN_POINT('Ctrl Pts',(-39.7402010400563,26.91999998,-68.4472152479348));
#149256=CARTESIAN_POINT('Ctrl Pts',(-39.0948775434837,26.91999998,-68.3006173151149));
#149257=CARTESIAN_POINT('Ctrl Pts',(-39.2671383510483,26.2832177198684,
-68.3538279338855));
#149258=CARTESIAN_POINT('Ctrl Pts',(-39.9875645500817,26.91999998,-67.4263054007275));
#149259=CARTESIAN_POINT('Ctrl Pts',(-39.2756374048449,26.9199999800001,
-67.1987893176786));
#149260=CARTESIAN_POINT('Ctrl Pts',(-39.5420936115266,26.229992717107,-67.2971964534767));
#149261=CARTESIAN_POINT('Ctrl Pts',(-40.1455341066151,26.91999998,-66.9202222962256));
#149262=CARTESIAN_POINT('Ctrl Pts',(-39.4018640899458,26.91999998,-66.6416836709376));
#149263=CARTESIAN_POINT('Ctrl Pts',(-39.7176630408463,26.2036238867825,
-66.7735892994237));
#149264=CARTESIAN_POINT('Ctrl Pts',(-40.61463744109,26.91999998,-65.7539057414421));
#149265=CARTESIAN_POINT('Ctrl Pts',(-39.796333686452,26.91999998,-65.2926622581118));
#149266=CARTESIAN_POINT('Ctrl Pts',(-40.2389877944043,26.1428985608433,
-65.5672893219614));
#149267=CARTESIAN_POINT('Ctrl Pts',(-40.9615610612356,26.91999998,-65.1057170341448));
#149268=CARTESIAN_POINT('Ctrl Pts',(-40.11277553943,26.91999998,-64.5135594045473));
#149269=CARTESIAN_POINT('Ctrl Pts',(-40.6245440189136,26.1091814001426,
-64.8971044625718));
#149270=CARTESIAN_POINT('Ctrl Pts',(-41.4294996031359,26.91999998,-64.5117188784924));
#149271=CARTESIAN_POINT('Ctrl Pts',(-40.529229952824,26.9199999800001,-63.7929022611462));
#149272=CARTESIAN_POINT('Ctrl Pts',(-41.1444123040958,26.0783301967522,
-64.2833612530845));
#149273=CARTESIAN_POINT('',(-39.000000010887,26.4199999800102,-71.0516396909909));
#149274=CARTESIAN_POINT('Origin',(-39.5,26.41999998,-71.0516396909898));
#149275=CARTESIAN_POINT('Ctrl Pts',(-39.0000000435479,26.4199999800162,
-71.0516396909931));
#149276=CARTESIAN_POINT('Ctrl Pts',(-39.0000145113878,26.4110146624994,
-70.873151997142));
#149277=CARTESIAN_POINT('Ctrl Pts',(-39.0036304228359,26.4020422627355,
-70.695134532768));
#149278=CARTESIAN_POINT('Ctrl Pts',(-39.0107908237139,26.3931003506741,
-70.5175991632096));
#149279=CARTESIAN_POINT('Ctrl Pts',(-39.0181773354903,26.383876071214,-70.3344575877166));
#149280=CARTESIAN_POINT('Ctrl Pts',(-39.0293349875578,26.3746834666836,
-70.1518284820121));
#149281=CARTESIAN_POINT('Ctrl Pts',(-39.0442524846789,26.3655198198259,
-69.9697097783002));
#149282=CARTESIAN_POINT('Ctrl Pts',(-39.0591699818001,26.3563561729682,
-69.7875910745883));
#149283=CARTESIAN_POINT('Ctrl Pts',(-39.0778470554579,26.3472204702714,
-69.6059820644029));
#149284=CARTESIAN_POINT('Ctrl Pts',(-39.1003301500804,26.3381020579365,
-69.4248755353872));
#149285=CARTESIAN_POINT('Ctrl Pts',(-39.1213238524142,26.3295876946992,
-69.2557664058523));
#149286=CARTESIAN_POINT('Ctrl Pts',(-39.1456304742869,26.3211123234295,
-69.0871090856946));
#149287=CARTESIAN_POINT('Ctrl Pts',(-39.1733342259095,26.3126536217979,
-68.9189042123943));
#149288=CARTESIAN_POINT('Ctrl Pts',(-39.2006004315504,26.3043285147409,
-68.7533559239289));
#149289=CARTESIAN_POINT('Ctrl Pts',(-39.2311575812492,26.2960187931794,
-68.588245391205));
#149290=CARTESIAN_POINT('Ctrl Pts',(-39.2651315757516,26.2877200435148,
-68.4235850326121));
#149291=CARTESIAN_POINT('Ctrl Pts',(-39.2982115270493,26.2796396797319,
-68.2632577963625));
#149292=CARTESIAN_POINT('Ctrl Pts',(-39.3345313341293,26.271569099348,-68.103356945394));
#149293=CARTESIAN_POINT('Ctrl Pts',(-39.374245173882,26.2635303553443,-67.9439118935694));
#149294=CARTESIAN_POINT('Ctrl Pts',(-39.3840891720875,26.2615377658078,
-67.9043897316779));
#149295=CARTESIAN_POINT('Ctrl Pts',(-39.3941418699496,26.2595472856189,
-67.8648956791587));
#149296=CARTESIAN_POINT('Ctrl Pts',(-39.4044059318906,26.257559574683,-67.8254304044373));
#149297=CARTESIAN_POINT('Ctrl Pts',(-39.4477904535049,26.2491578436181,
-67.658617102451));
#149298=CARTESIAN_POINT('Ctrl Pts',(-39.4949549804392,26.2408118245717,
-67.4922912802412));
#149299=CARTESIAN_POINT('Ctrl Pts',(-39.5460345952973,26.2325004784911,
-67.3269367477042));
#149300=CARTESIAN_POINT('Ctrl Pts',(-39.5960590796543,26.2243608164527,
-67.1649978754315));
#149301=CARTESIAN_POINT('Ctrl Pts',(-39.6498392227994,26.2162544279808,
-67.0039905928097));
#149302=CARTESIAN_POINT('Ctrl Pts',(-39.7074854141219,26.2082016737779,
-66.8443933108068));
#149303=CARTESIAN_POINT('Ctrl Pts',(-39.7636025178171,26.2003625220096,
-66.6890294087318));
#149304=CARTESIAN_POINT('Ctrl Pts',(-39.8233838830514,26.1925743712279,
-66.535001809439));
#149305=CARTESIAN_POINT('Ctrl Pts',(-39.886906568172,26.1848929410533,-66.3827738490702));
#149306=CARTESIAN_POINT('Ctrl Pts',(-39.9025350537342,26.183003078867,-66.3453212055576));
#149307=CARTESIAN_POINT('Ctrl Pts',(-39.9183898602438,26.1811198480103,
-66.3079775972808));
#149308=CARTESIAN_POINT('Ctrl Pts',(-39.9344718328247,26.1792444109355,
-66.2707501214404));
#149309=CARTESIAN_POINT('Ctrl Pts',(-39.9822660966514,26.1736707703951,
-66.1601132084024));
#149310=CARTESIAN_POINT('Ctrl Pts',(-40.0320921744015,26.1682149601011,
-66.0503548440615));
#149311=CARTESIAN_POINT('Ctrl Pts',(-40.0841320620358,26.1628014935,-65.9415105087306));
#149312=CARTESIAN_POINT('Ctrl Pts',(-40.1349313000628,26.1575170858865,
-65.8352610614368));
#149313=CARTESIAN_POINT('Ctrl Pts',(-40.1878406174558,26.152272806562,-65.7298824473367));
#149314=CARTESIAN_POINT('Ctrl Pts',(-40.2430471767249,26.1470364906056,
-65.6254334149233));
#149315=CARTESIAN_POINT('Ctrl Pts',(-40.2974041735934,26.1418807552399,
-65.5225917272148));
#149316=CARTESIAN_POINT('Ctrl Pts',(-40.353988821302,26.1367325300632,-65.4206511037866));
#149317=CARTESIAN_POINT('Ctrl Pts',(-40.4129890297332,26.1316016887989,
-65.3196948551107));
#149318=CARTESIAN_POINT('Ctrl Pts',(-40.4705491871184,26.1265960788436,
-65.2212027019928));
#149319=CARTESIAN_POINT('Ctrl Pts',(-40.5304090124457,26.1216069449867,
-65.1236474232294));
#149320=CARTESIAN_POINT('Ctrl Pts',(-40.5927434226748,26.1166843178501,
-65.0271336117946));
#149321=CARTESIAN_POINT('Ctrl Pts',(-40.637191990793,26.1131741582642,-64.9583128640543));
#149322=CARTESIAN_POINT('Ctrl Pts',(-40.6828988377376,26.1096986589903,
-64.8900222275229));
#149323=CARTESIAN_POINT('Ctrl Pts',(-40.7299249270772,26.1062893712319,
-64.8223085129012));
#149324=CARTESIAN_POINT('Origin',(-39.5,26.41999998,-55.24995));
#149325=CARTESIAN_POINT('',(-39.0000000108873,26.4199999800017,-161.007003280499));
#149326=CARTESIAN_POINT('Origin',(-39.5,26.41999998,-161.0070032805));
#149327=CARTESIAN_POINT('',(-39.,26.41999998,-129.34995));
#149328=CARTESIAN_POINT('Ctrl Pts',(-41.4298327884615,26.91999998,-167.547398188302));
#149329=CARTESIAN_POINT('Ctrl Pts',(-40.5295342387659,26.9199999800211,
-168.266393711463));
#149330=CARTESIAN_POINT('Ctrl Pts',(-41.1447896171409,26.078294457151,-167.775763627336));
#149331=CARTESIAN_POINT('Ctrl Pts',(-40.9612348539621,26.91999998,-166.952514419193));
#149332=CARTESIAN_POINT('Ctrl Pts',(-40.1124742201721,26.919999979984,-167.544709932801));
#149333=CARTESIAN_POINT('Ctrl Pts',(-40.6241898364545,26.109190890174,-167.161108892939));
#149334=CARTESIAN_POINT('Ctrl Pts',(-40.6146946127263,26.91999998,-166.304618713242));
#149335=CARTESIAN_POINT('Ctrl Pts',(-39.796315247074,26.91999998,-166.765696010883));
#149336=CARTESIAN_POINT('Ctrl Pts',(-40.239058378987,26.1428924785697,-166.491226580831));
#149337=CARTESIAN_POINT('Ctrl Pts',(-40.2438971241064,26.91999998,-165.383070268286));
#149338=CARTESIAN_POINT('Ctrl Pts',(-39.4770684823812,26.91999998,-165.674348404122));
#149339=CARTESIAN_POINT('Ctrl Pts',(-39.826994448169,26.1908718557831,-165.538116630435));
#149340=CARTESIAN_POINT('Ctrl Pts',(-40.1559725857258,26.91999998,-165.136425734968));
#149341=CARTESIAN_POINT('Ctrl Pts',(-39.4061926872737,26.91999998,-165.399736081576));
#149342=CARTESIAN_POINT('Ctrl Pts',(-39.7292761024087,26.2037183818383,
-165.282971165658));
#149343=CARTESIAN_POINT('Ctrl Pts',(-39.9974565076864,26.91999998,-164.635718209756));
#149344=CARTESIAN_POINT('Ctrl Pts',(-39.2823615806739,26.91999998,-164.849118133022));
#149345=CARTESIAN_POINT('Ctrl Pts',(-39.5530950653548,26.2298065015692,
-164.764919225151));
#149346=CARTESIAN_POINT('Ctrl Pts',(-39.9267078667251,26.91999998,-164.380863661625));
#149347=CARTESIAN_POINT('Ctrl Pts',(-39.2284349479001,26.91999998,-164.571842280085));
#149348=CARTESIAN_POINT('Ctrl Pts',(-39.4744590694183,26.2430893614396,
-164.501193577802));
#149349=CARTESIAN_POINT('Ctrl Pts',(-39.7405665669667,26.91999998,-163.613547303229));
#149350=CARTESIAN_POINT('Ctrl Pts',(-39.0951163240011,26.91999998,-163.76037459309));
#149351=CARTESIAN_POINT('Ctrl Pts',(-39.2675481437431,26.2830943322452,
-163.707008328011));
#149352=CARTESIAN_POINT('Ctrl Pts',(-39.6504680302044,26.91999998,-163.097634164455));
#149353=CARTESIAN_POINT('Ctrl Pts',(-39.034250805552,26.919999979999,-163.210613020243));
#149354=CARTESIAN_POINT('Ctrl Pts',(-39.1673881282116,26.3100067475891,
-163.172866145833));
#149355=CARTESIAN_POINT('Ctrl Pts',(-39.5060746903532,26.91999998,-161.850209820763));
#149356=CARTESIAN_POINT('Ctrl Pts',(-38.9629253593384,26.9199999800013,
-161.914115824651));
#149357=CARTESIAN_POINT('Ctrl Pts',(-39.0068209359397,26.3751075091203,
-161.880866818163));
#149358=CARTESIAN_POINT('Ctrl Pts',(-39.4806915865888,26.91999998,-161.114953773424));
#149359=CARTESIAN_POINT('Ctrl Pts',(-38.9720162576935,26.9199999800008,
-161.146047041293));
#149360=CARTESIAN_POINT('Ctrl Pts',(-38.9785566343046,26.4135006774998,
-161.118978397722));
#149361=CARTESIAN_POINT('Ctrl Pts',(-39.5144747798535,26.91999998,-160.372187822257));
#149362=CARTESIAN_POINT('Ctrl Pts',(-39.0463593412646,26.9199999799985,
-160.350365998772));
#149363=CARTESIAN_POINT('Ctrl Pts',(-39.0160285899416,26.45229437412,-160.348928929189));
#149364=CARTESIAN_POINT('',(-40.7299249193732,26.1062892385183,-167.236334574448));
#149365=CARTESIAN_POINT('Origin',(-41.0569324495328,26.41999998,-167.025025538602));
#149366=CARTESIAN_POINT('Ctrl Pts',(-40.7299249270775,26.1062893712214,
-167.236334458579));
#149367=CARTESIAN_POINT('Ctrl Pts',(-40.6645853304908,26.1110263480999,
-167.142250794741));
#149368=CARTESIAN_POINT('Ctrl Pts',(-40.6018092312385,26.1158892443008,
-167.047079458829));
#149369=CARTESIAN_POINT('Ctrl Pts',(-40.5414282215195,26.1207982581812,
-166.950942290991));
#149370=CARTESIAN_POINT('Ctrl Pts',(-40.4792943195239,26.1258497833008,
-166.852014210915));
#149371=CARTESIAN_POINT('Ctrl Pts',(-40.4196959436351,26.1309501291377,
-166.752063428848));
#149372=CARTESIAN_POINT('Ctrl Pts',(-40.3624432000981,26.1360584358626,
-166.651192119132));
#149373=CARTESIAN_POINT('Ctrl Pts',(-40.3043231046772,26.1412441310092,
-166.548792656962));
#149374=CARTESIAN_POINT('Ctrl Pts',(-40.248619615909,26.1464382085178,-166.445444459256));
#149375=CARTESIAN_POINT('Ctrl Pts',(-40.1951374467669,26.1516433268258,
-166.341224092504));
#149376=CARTESIAN_POINT('Ctrl Pts',(-40.1404552306636,26.1569652389458,
-166.234665201784));
#149377=CARTESIAN_POINT('Ctrl Pts',(-40.0880945140287,26.1622988986898,
-166.127194440059));
#149378=CARTESIAN_POINT('Ctrl Pts',(-40.0378597432825,26.1676913791697,
-166.018863887683));
#149379=CARTESIAN_POINT('Ctrl Pts',(-40.0025451368701,26.1714822459918,
-165.942708452658));
#149380=CARTESIAN_POINT('Ctrl Pts',(-39.968281445585,26.1753031256121,-165.866127477038));
#149381=CARTESIAN_POINT('Ctrl Pts',(-39.9350068722586,26.1791820283199,
-165.789131151273));
#149382=CARTESIAN_POINT('Ctrl Pts',(-39.8781104841659,26.1858145868105,
-165.657474682251));
#149383=CARTESIAN_POINT('Ctrl Pts',(-39.824173358347,26.1925157729063,-165.524625114876));
#149384=CARTESIAN_POINT('Ctrl Pts',(-39.7730275511278,26.1992640596196,
-165.39065734938));
#149385=CARTESIAN_POINT('Ctrl Pts',(-39.726719856284,26.2053739954839,-165.2693621985));
#149386=CARTESIAN_POINT('Ctrl Pts',(-39.6827002133185,26.2115233790131,
-165.147149841886));
#149387=CARTESIAN_POINT('Ctrl Pts',(-39.6408588199536,26.2177241633614,
-165.024056999754));
#149388=CARTESIAN_POINT('Ctrl Pts',(-39.593547601588,26.2247355613755,-164.8848725256));
#149389=CARTESIAN_POINT('Ctrl Pts',(-39.5489550215303,26.2318160157631,
-164.744332341484));
#149390=CARTESIAN_POINT('Ctrl Pts',(-39.5071363085111,26.238934446759,-164.60301081883));
#149391=CARTESIAN_POINT('Ctrl Pts',(-39.4711232425277,26.2450646336215,
-164.481308811457));
#149392=CARTESIAN_POINT('Ctrl Pts',(-39.4371664077637,26.25122276278,-164.359027557099));
#149393=CARTESIAN_POINT('Ctrl Pts',(-39.4052702587627,26.2573922922468,
-164.236533904511));
#149394=CARTESIAN_POINT('Ctrl Pts',(-39.3636932871594,26.2654343399386,
-164.076862117327));
#149395=CARTESIAN_POINT('Ctrl Pts',(-39.325582511077,26.2735180911288,-163.916749616534));
#149396=CARTESIAN_POINT('Ctrl Pts',(-39.2907701194594,26.2816124879209,
-163.756231489263));
#149397=CARTESIAN_POINT('Ctrl Pts',(-39.2553129100334,26.2898568144063,
-163.592740140613));
#149398=CARTESIAN_POINT('Ctrl Pts',(-39.2232769169584,26.2981128611817,
-163.428827555342));
#149399=CARTESIAN_POINT('Ctrl Pts',(-39.1945240576485,26.3063791197979,
-163.264509373524));
#149400=CARTESIAN_POINT('Ctrl Pts',(-39.1651338062026,26.3148286244759,
-163.096548593391));
#149401=CARTESIAN_POINT('Ctrl Pts',(-39.1391734849508,26.3232895602475,
-162.928163525903));
#149402=CARTESIAN_POINT('Ctrl Pts',(-39.1165429759402,26.3317816876087,
-162.759356000773));
#149403=CARTESIAN_POINT('Ctrl Pts',(-39.1109704816533,26.333872773195,-162.717789150953));
#149404=CARTESIAN_POINT('Ctrl Pts',(-39.105600118859,26.3359658181642,-162.67619663796));
#149405=CARTESIAN_POINT('Ctrl Pts',(-39.1004308539458,26.3380612268828,
-162.634578411071));
#149406=CARTESIAN_POINT('Ctrl Pts',(-39.0785784610887,26.3469192938001,
-162.458642787875));
#149407=CARTESIAN_POINT('Ctrl Pts',(-39.0603220000318,26.3557925737031,
-162.282263412771));
#149408=CARTESIAN_POINT('Ctrl Pts',(-39.0456144734669,26.3646901587427,
-162.105434547007));
#149409=CARTESIAN_POINT('Ctrl Pts',(-39.0304671535062,26.3738538047763,
-161.923318037057));
#149410=CARTESIAN_POINT('Ctrl Pts',(-39.0190841572563,26.3830442343986,
-161.740724053985));
#149411=CARTESIAN_POINT('Ctrl Pts',(-39.0114709868334,26.3922645834336,
-161.557650702015));
#149412=CARTESIAN_POINT('Ctrl Pts',(-39.0038578164105,26.4014849324685,
-161.374577350044));
#149413=CARTESIAN_POINT('Ctrl Pts',(-39.0000149601043,26.4107361238319,
-161.191023970058));
#149414=CARTESIAN_POINT('Ctrl Pts',(-39.0000000435492,26.4199999800048,
-161.007003280497));
#149415=CARTESIAN_POINT('Ctrl Pts',(-40.7299249439265,26.10628905815,-167.236334669472));
#149416=CARTESIAN_POINT('Ctrl Pts',(-40.1792441039419,26.91999998,-167.592179375447));
#149417=CARTESIAN_POINT('Ctrl Pts',(-41.0569324495328,26.91999998,-167.025025538602));
#149418=CARTESIAN_POINT('Ctrl Pts',(-41.5498055229506,26.1095638122232,
-168.509987294195));
#149419=CARTESIAN_POINT('Ctrl Pts',(-41.0020315723371,26.9199999800235,
-168.844852386549));
#149420=CARTESIAN_POINT('Ctrl Pts',(-41.879954591083,26.91999998,-168.29867810854));
#149421=CARTESIAN_POINT('Ctrl Pts',(-42.361486708359,26.1127497675934,-169.788980903725));
#149422=CARTESIAN_POINT('Ctrl Pts',(-41.8241014260219,26.9199999799921,
-170.115499778852));
#149423=CARTESIAN_POINT('Ctrl Pts',(-42.6945981803054,26.91999998,-169.577671730211));
#149424=CARTESIAN_POINT('Ctrl Pts',(-43.1661128544364,26.1158519257145,
-171.07256826174));
#149425=CARTESIAN_POINT('Ctrl Pts',(-42.6444458925864,26.91999998,-171.400720533971));
#149426=CARTESIAN_POINT('Ctrl Pts',(-43.502033101348,26.91999998,-170.861259130871));
#149427=CARTESIAN_POINT('',(-43.1661128544364,26.1158519257145,-171.07256826174));
#149428=CARTESIAN_POINT('Origin',(-43.5020331013479,26.41999998,-170.861259130871));
#149429=CARTESIAN_POINT('Ctrl Pts',(-43.1661128544364,26.1158519257145,
-171.07256826174));
#149430=CARTESIAN_POINT('Ctrl Pts',(-42.3615449736022,26.1127499922191,
-169.789073851883));
#149431=CARTESIAN_POINT('Ctrl Pts',(-41.5498582787394,26.1095640229222,
-168.510069248237));
#149432=CARTESIAN_POINT('Ctrl Pts',(-40.7299249439363,26.1062890581356,
-167.236334669465));
#149433=CARTESIAN_POINT('Ctrl Pts',(-44.1114262156583,26.91999998,-171.14995));
#149434=CARTESIAN_POINT('Ctrl Pts',(-44.1114262156583,26.91999998,-171.64995));
#149435=CARTESIAN_POINT('Ctrl Pts',(-44.1114262156583,26.41999998,-171.64995));
#149436=CARTESIAN_POINT('Ctrl Pts',(-43.9948946430299,26.91999998,-171.149949978158));
#149437=CARTESIAN_POINT('Ctrl Pts',(-43.9189401667911,26.91999998,-171.71139261988));
#149438=CARTESIAN_POINT('Ctrl Pts',(-43.9300489743418,26.362103375035,-171.64995));
#149439=CARTESIAN_POINT('Ctrl Pts',(-43.8763450763459,26.91999998,-171.127242425404));
#149440=CARTESIAN_POINT('Ctrl Pts',(-43.7068322349107,26.91999998,-171.744547621103));
#149441=CARTESIAN_POINT('Ctrl Pts',(-43.7459157865524,26.3030441696697,
-171.604534812847));
#149442=CARTESIAN_POINT('Ctrl Pts',(-43.7162275365378,26.91999998,-171.05684827667));
#149443=CARTESIAN_POINT('Ctrl Pts',(-43.3564708632233,26.91999998,-171.726334995184));
#149444=CARTESIAN_POINT('Ctrl Pts',(-43.4976348610037,26.2230846254426,
-171.46374657232));
#149445=CARTESIAN_POINT('Ctrl Pts',(-43.665002290469,26.91999998,-171.026908215035));
#149446=CARTESIAN_POINT('Ctrl Pts',(-43.2222824786043,26.91999998,-171.705069685313));
#149447=CARTESIAN_POINT('Ctrl Pts',(-43.4182794830488,26.1974705898599,
-171.403866413424));
#149448=CARTESIAN_POINT('Ctrl Pts',(-43.5734725485514,26.91999998,-170.953826827844));
#149449=CARTESIAN_POINT('Ctrl Pts',(-42.9355727403744,26.91999998,-171.608576267085));
#149450=CARTESIAN_POINT('Ctrl Pts',(-43.2765868661323,26.1516592710682,
-171.257703672334));
#149451=CARTESIAN_POINT('Ctrl Pts',(-43.5336346878404,26.91999998,-170.91149625204));
#149452=CARTESIAN_POINT('Ctrl Pts',(-42.7841822677167,26.9199999800011,
-171.530641542159));
#149453=CARTESIAN_POINT('Ctrl Pts',(-43.2149501334587,26.1316898999239,
-171.173001781957));
#149454=CARTESIAN_POINT('Ctrl Pts',(-43.5020331013479,26.91999998,-170.861259130871));
#149455=CARTESIAN_POINT('Ctrl Pts',(-42.6444458925863,26.91999998,-171.400720533971));
#149456=CARTESIAN_POINT('Ctrl Pts',(-43.1661128544364,26.1158519257145,
-171.07256826174));
#149457=CARTESIAN_POINT('',(-44.1114262156583,26.41999998,-171.64995));
#149458=CARTESIAN_POINT('Origin',(-44.1114262156583,26.41999998,-171.14995));
#149459=CARTESIAN_POINT('Ctrl Pts',(-44.1114262156583,26.41999998,-171.64995));
#149460=CARTESIAN_POINT('Ctrl Pts',(-43.9300489743418,26.362103375035,-171.64995));
#149461=CARTESIAN_POINT('Ctrl Pts',(-43.7459157865524,26.3030441696697,
-171.604534812847));
#149462=CARTESIAN_POINT('Ctrl Pts',(-43.4976348610037,26.2230846254426,
-171.46374657232));
#149463=CARTESIAN_POINT('Ctrl Pts',(-43.4182794830488,26.1974705898599,
-171.403866413424));
#149464=CARTESIAN_POINT('Ctrl Pts',(-43.2765868661323,26.1516592710682,
-171.257703672334));
#149465=CARTESIAN_POINT('Ctrl Pts',(-43.2149501334587,26.1316898999239,
-171.173001781957));
#149466=CARTESIAN_POINT('Ctrl Pts',(-43.1661128544364,26.1158519257145,
-171.07256826174));
#149467=CARTESIAN_POINT('Origin',(83.2809572255632,26.4199999800001,-171.14995));
#149468=CARTESIAN_POINT('',(-43.6598261881496,26.41999998,-171.64995));
#149469=CARTESIAN_POINT('Origin',(-57.,-2.42462934179819E-14,-58.24995));
#149470=CARTESIAN_POINT('',(-60.,27.91999998,-58.24995));
#149471=CARTESIAN_POINT('',(-60.,-54.58000002,-58.24995));
#149472=CARTESIAN_POINT('Origin',(-57.,27.91999998,-58.24995));
#149473=CARTESIAN_POINT('Origin',(-57.,27.91999998,-58.24995));
#149474=CARTESIAN_POINT('Origin',(-59.5,27.91999998,-58.24995));
#149475=CARTESIAN_POINT('Origin',(-41.7558360441701,29.41999998,-179.64995));
#149476=CARTESIAN_POINT('',(-41.0540572871253,28.7076050220164,-179.64995));
#149477=CARTESIAN_POINT('Ctrl Pts',(-45.342056117244,28.41999998,-61.14995));
#149478=CARTESIAN_POINT('Ctrl Pts',(-45.342056117244,28.41999998,-60.6499449120928));
#149479=CARTESIAN_POINT('Ctrl Pts',(-45.342056117244,28.9200050678813,-60.6499500000259));
#149480=CARTESIAN_POINT('Ctrl Pts',(-45.2032855852163,28.41999998,-61.1499499725599));
#149481=CARTESIAN_POINT('Ctrl Pts',(-45.2207546457868,28.41999998,-60.688556379456));
#149482=CARTESIAN_POINT('Ctrl Pts',(-45.2161093325487,28.8799153348109,
-60.6499495913736));
#149483=CARTESIAN_POINT('Ctrl Pts',(-45.0642313709311,28.41999998,-61.1448442113686));
#149484=CARTESIAN_POINT('Ctrl Pts',(-45.0814092233342,28.4199999800005,
-60.7134256454893));
#149485=CARTESIAN_POINT('Ctrl Pts',(-45.0809055449378,28.8470468727513,
-60.6499493090119));
#149486=CARTESIAN_POINT('Ctrl Pts',(-44.7862672310244,28.41999998,-61.1362430899869));
#149487=CARTESIAN_POINT('Ctrl Pts',(-44.7998786663716,28.4199999799995,
-60.7430249240652));
#149488=CARTESIAN_POINT('Ctrl Pts',(-44.7999542633237,28.8023061531432,
-60.6499489465081));
#149489=CARTESIAN_POINT('Ctrl Pts',(-44.647272115325,28.41999998,-61.1328798677618));
#149490=CARTESIAN_POINT('Ctrl Pts',(-44.652744176702,28.41999998,-60.7493138199263));
#149491=CARTESIAN_POINT('Ctrl Pts',(-44.6541596767004,28.7904721518728,
-60.6499488654503));
#149492=CARTESIAN_POINT('Ctrl Pts',(-44.3691883762669,28.41999998,-61.1328719599062));
#149493=CARTESIAN_POINT('Ctrl Pts',(-44.3637416796284,28.41999998,-60.7493310407855));
#149494=CARTESIAN_POINT('Ctrl Pts',(-44.36232828092,28.7904412154038,-60.6499488652048));
#149495=CARTESIAN_POINT('Ctrl Pts',(-44.2300913879779,28.41999998,-61.1362301431742));
#149496=CARTESIAN_POINT('Ctrl Pts',(-44.2164931090599,28.41999998,-60.7430562060495));
#149497=CARTESIAN_POINT('Ctrl Pts',(-44.2164190292987,28.8022526047183,
-60.6499489461074));
#149498=CARTESIAN_POINT('Ctrl Pts',(-43.952003265591,28.41999998,-61.1448329195507));
#149499=CARTESIAN_POINT('Ctrl Pts',(-43.9348222136893,28.41999998,-60.7134784063315));
#149500=CARTESIAN_POINT('Ctrl Pts',(-43.9353228646302,28.8469743774063,
-60.6499493083947));
#149501=CARTESIAN_POINT('Ctrl Pts',(-43.812959462792,28.41999998,-61.149949972467));
#149502=CARTESIAN_POINT('Ctrl Pts',(-43.7954409326635,28.4199999800005,
-60.6886488998596));
#149503=CARTESIAN_POINT('Ctrl Pts',(-43.8001087095939,28.8798156648002,
-60.6499495903585));
#149504=CARTESIAN_POINT('Ctrl Pts',(-43.6738487993976,28.41999998,-61.14995));
#149505=CARTESIAN_POINT('Ctrl Pts',(-43.6738487993976,28.41999998,-60.6499449120928));
#149506=CARTESIAN_POINT('Ctrl Pts',(-43.6738487993976,28.9200050678813,
-60.6499500000259));
#149507=CARTESIAN_POINT('Origin',(-59.5,27.91999998,0.));
#149508=CARTESIAN_POINT('',(-60.,27.91999998,-174.34995));
#149509=CARTESIAN_POINT('Origin',(-59.5,27.91999998,-174.34995));
#149510=CARTESIAN_POINT('',(-60.,27.91999998,-58.24995));
#149511=CARTESIAN_POINT('Origin',(-57.,27.91999998,-174.34995));
#149512=CARTESIAN_POINT('',(-57.,27.91999998,-177.34995));
#149513=CARTESIAN_POINT('Origin',(-57.,27.91999998,-176.84995));
#149514=CARTESIAN_POINT('Origin',(-57.,27.91999998,-174.34995));
#149515=CARTESIAN_POINT('Origin',(-60.,27.91999998,-176.84995));
#149516=CARTESIAN_POINT('',(-50.9656271260094,27.91999998,-177.34995));
#149517=CARTESIAN_POINT('',(-60.,27.91999998,-177.34995));
#149518=CARTESIAN_POINT('Ctrl Pts',(-50.9656271260094,27.91999998,-177.34995));
#149519=CARTESIAN_POINT('Ctrl Pts',(-50.9287302813235,28.0512673257631,
-177.34995));
#149520=CARTESIAN_POINT('Ctrl Pts',(-50.8922666809894,28.1809933246567,
-177.29606343653));
#149521=CARTESIAN_POINT('Ctrl Pts',(-50.840232816526,28.3661134165298,-177.110943344657));
#149522=CARTESIAN_POINT('Ctrl Pts',(-50.8250862913143,28.41999998,-176.981217345763));
#149523=CARTESIAN_POINT('Ctrl Pts',(-50.825086291307,28.41999998,-176.84995));
#149524=CARTESIAN_POINT('Origin',(-50.825086291307,28.91999998,-171.64995));
#149525=CARTESIAN_POINT('Origin',(-50.825086291307,28.91999998,-176.84995));
#149526=CARTESIAN_POINT('Origin',(-50.825086291307,28.91999998,-172.64995));
#149527=CARTESIAN_POINT('Ctrl Pts',(-50.3299522569362,28.85041342952,-172.64995));
#149528=CARTESIAN_POINT('Ctrl Pts',(-50.3904429223989,28.41999998,-172.64995));
#149529=CARTESIAN_POINT('Ctrl Pts',(-50.825086291307,28.41999998,-172.64995));
#149530=CARTESIAN_POINT('Ctrl Pts',(-50.3299522569358,28.8504134295228,
-172.51902671195));
#149531=CARTESIAN_POINT('Ctrl Pts',(-50.3904429223853,28.4199999800017,
-172.511015867074));
#149532=CARTESIAN_POINT('Ctrl Pts',(-50.82508629129,28.41999998,-172.453565067926));
#149533=CARTESIAN_POINT('Ctrl Pts',(-50.3034146036607,28.8522245814264,
-172.38820210671));
#149534=CARTESIAN_POINT('Ctrl Pts',(-50.3606872372737,28.41999998,-172.371853931892));
#149535=CARTESIAN_POINT('Ctrl Pts',(-50.7856616225938,28.41999998,-172.257328160063));
#149536=CARTESIAN_POINT('Ctrl Pts',(-50.2012639378342,28.8591961991206,
-172.14633102856));
#149537=CARTESIAN_POINT('Ctrl Pts',(-50.247876228143,28.41999998,-172.118296873734));
#149538=CARTESIAN_POINT('Ctrl Pts',(-50.6339053193109,28.41999998,-171.894521542842));
#149539=CARTESIAN_POINT('Ctrl Pts',(-50.1256910952006,28.8643539233763,
-172.035403273235));
#149540=CARTESIAN_POINT('Ctrl Pts',(-50.1643071358756,28.4199999800017,
-172.003556970023));
#149541=CARTESIAN_POINT('Ctrl Pts',(-50.5216333616693,28.41999998,-171.728129909852));
#149542=CARTESIAN_POINT('Ctrl Pts',(-49.9369412763291,28.8772357931761,
-171.850283164392));
#149543=CARTESIAN_POINT('Ctrl Pts',(-49.9598619165025,28.4199999799983,
-171.817687494207));
#149544=CARTESIAN_POINT('Ctrl Pts',(-50.2412242764601,28.41999998,-171.450449746589));
#149545=CARTESIAN_POINT('Ctrl Pts',(-49.8238385246439,28.8849548730131,
-171.776163607997));
#149546=CARTESIAN_POINT('Ctrl Pts',(-49.8382982003454,28.4199999800004,
-171.746711574348));
#149547=CARTESIAN_POINT('Ctrl Pts',(-50.0731974178181,28.41999998,-171.339270411997));
#149548=CARTESIAN_POINT('Ctrl Pts',(-49.5772250015517,28.9017858470187,
-171.675977326981));
#149549=CARTESIAN_POINT('Ctrl Pts',(-49.5798629394444,28.4199999799996,
-171.658003579003));
#149550=CARTESIAN_POINT('Ctrl Pts',(-49.7068252918851,28.41999998,-171.18899099047));
#149551=CARTESIAN_POINT('Ctrl Pts',(-49.443835276054,28.9108894800008,-171.64995));
#149552=CARTESIAN_POINT('Ctrl Pts',(-49.4425933612922,28.41999998,-171.640924254978));
#149553=CARTESIAN_POINT('Ctrl Pts',(-49.5086598519041,28.41999998,-171.149950000016));
#149554=CARTESIAN_POINT('Ctrl Pts',(-49.3103449325291,28.91999998,-171.64995));
#149555=CARTESIAN_POINT('Ctrl Pts',(-49.3103449325291,28.41999998,-171.64995));
#149556=CARTESIAN_POINT('Ctrl Pts',(-49.3103449325291,28.41999998,-171.14995));
#149557=CARTESIAN_POINT('Origin',(-49.3103449325291,28.91999998,-171.14995));
#149558=CARTESIAN_POINT('Ctrl Pts',(-49.3103449325291,28.91999998,-171.64995));
#149559=CARTESIAN_POINT('Ctrl Pts',(-49.443835276054,28.9108894800008,-171.64995));
#149560=CARTESIAN_POINT('Ctrl Pts',(-49.5772250015517,28.9017858470187,
-171.675977326981));
#149561=CARTESIAN_POINT('Ctrl Pts',(-49.8238385246439,28.8849548730131,
-171.776163607997));
#149562=CARTESIAN_POINT('Ctrl Pts',(-49.9369412763291,28.8772357931761,
-171.850283164392));
#149563=CARTESIAN_POINT('Ctrl Pts',(-50.1256910952006,28.8643539233763,
-172.035403273235));
#149564=CARTESIAN_POINT('Ctrl Pts',(-50.2012639378342,28.8591961991206,
-172.14633102856));
#149565=CARTESIAN_POINT('Ctrl Pts',(-50.3034146036607,28.8522245814264,
-172.38820210671));
#149566=CARTESIAN_POINT('Ctrl Pts',(-50.3299522569358,28.8504134295228,
-172.51902671195));
#149567=CARTESIAN_POINT('Ctrl Pts',(-50.3299522569362,28.85041342952,-172.64995));
#149568=CARTESIAN_POINT('Origin',(-60.,28.91999998,-171.14995));
#149569=CARTESIAN_POINT('Origin',(-60.,28.91999998,-171.14995));
#149570=CARTESIAN_POINT('Origin',(-42.,28.91999998,-171.14995));
#149571=CARTESIAN_POINT('Origin',(-60.,11.61999998,-176.84995));
#149572=CARTESIAN_POINT('',(-53.6325912458891,11.61999998,-177.34995));
#149573=CARTESIAN_POINT('',(-53.3846587239314,11.8868850448361,-177.272764808359));
#149574=CARTESIAN_POINT('Ctrl Pts',(-53.6325912458891,11.61999998,-177.34995));
#149575=CARTESIAN_POINT('Ctrl Pts',(-53.6010140858531,11.6544395308136,
-177.34995));
#149576=CARTESIAN_POINT('Ctrl Pts',(-53.5694844728451,11.6886293911647,
-177.346396020703));
#149577=CARTESIAN_POINT('Ctrl Pts',(-53.5384795926869,11.7220946388468,
-177.339415709356));
#149578=CARTESIAN_POINT('Ctrl Pts',(-53.5095770053376,11.7532907679517,
-177.332908699574));
#149579=CARTESIAN_POINT('Ctrl Pts',(-53.4811304040669,11.7838607674282,
-177.323423109353));
#149580=CARTESIAN_POINT('Ctrl Pts',(-53.4535263405212,11.8134148549189,
-177.311025575324));
#149581=CARTESIAN_POINT('Ctrl Pts',(-53.4298706264844,11.8387416710648,
-177.300401323598));
#149582=CARTESIAN_POINT('Ctrl Pts',(-53.4068336627752,11.8633233108441,
-177.287637217697));
#149583=CARTESIAN_POINT('Ctrl Pts',(-53.3846587239314,11.886885044836,-177.272764808359));
#149584=CARTESIAN_POINT('',(-57.,11.61999998,-177.34995));
#149585=CARTESIAN_POINT('',(-60.,11.61999998,-177.34995));
#149586=CARTESIAN_POINT('Origin',(-57.,11.61999998,-176.84995));
#149587=CARTESIAN_POINT('Ctrl Pts',(-53.3846587239314,11.8868850448361,
-177.272764808359));
#149588=CARTESIAN_POINT('Ctrl Pts',(-53.3209180569567,11.9546120038032,
-177.230014853822));
#149589=CARTESIAN_POINT('Ctrl Pts',(-53.2731270360347,12.0145014233151,
-177.168462633103));
#149590=CARTESIAN_POINT('Ctrl Pts',(-53.2113113817619,12.0970286741326,
-177.021779308321));
#149591=CARTESIAN_POINT('Ctrl Pts',(-53.1963133903003,12.11999998,-176.935788696125));
#149592=CARTESIAN_POINT('Ctrl Pts',(-53.1963133798215,12.11999998,-176.84995));
#149593=CARTESIAN_POINT('Origin',(-53.1963133798215,12.61999998,-179.64995));
#149594=CARTESIAN_POINT('Origin',(-53.1963133798215,12.61999998,-171.855638188259));
#149595=CARTESIAN_POINT('Origin',(-53.1963133798215,12.61999998,-176.84995));
#149596=CARTESIAN_POINT('Ctrl Pts',(-52.7217372011832,12.4615824973952,
-171.881858542095));
#149597=CARTESIAN_POINT('Ctrl Pts',(-52.8357962988228,12.1199999800004,
-171.884866486815));
#149598=CARTESIAN_POINT('Ctrl Pts',(-53.1958197283118,12.11999998,-171.894290758533));
#149599=CARTESIAN_POINT('Ctrl Pts',(-52.7290806418237,12.4488888857452,
-171.760397092706));
#149600=CARTESIAN_POINT('Ctrl Pts',(-52.8493435053801,12.1199999799985,
-171.750925740441));
#149601=CARTESIAN_POINT('Ctrl Pts',(-53.2003775471301,12.11999998,-171.715353582304));
#149602=CARTESIAN_POINT('Ctrl Pts',(-52.7133768168196,12.4424829119345,
-171.643651148372));
#149603=CARTESIAN_POINT('Ctrl Pts',(-52.8340183717379,12.11999998,-171.617247566893));
#149604=CARTESIAN_POINT('Ctrl Pts',(-53.1734142621322,12.11999998,-171.541767472582));
#149605=CARTESIAN_POINT('Ctrl Pts',(-52.6344997605979,12.4386942197548,
-171.419334545233));
#149606=CARTESIAN_POINT('Ctrl Pts',(-52.7460023418722,12.11999998,-171.362905444502));
#149607=CARTESIAN_POINT('Ctrl Pts',(-53.0531021129573,12.11999998,-171.206197136279));
#149608=CARTESIAN_POINT('Ctrl Pts',(-52.5738654759387,12.4413473579302,
-171.318822511501));
#149609=CARTESIAN_POINT('Ctrl Pts',(-52.6758688342237,12.1199999799997,
-171.248558765417));
#149610=CARTESIAN_POINT('Ctrl Pts',(-52.9635655392073,12.11999998,-171.054813778703));
#149611=CARTESIAN_POINT('Ctrl Pts',(-52.4932465322732,12.4468321277953,
-171.230060927849));
#149612=CARTESIAN_POINT('Ctrl Pts',(-52.5838617435422,12.1199999800001,
-171.150392701598));
#149613=CARTESIAN_POINT('Ctrl Pts',(-52.8454881851277,12.11999998,-170.920313606715));
#149614=CARTESIAN_POINT('',(-52.5103993912278,12.4456688534686,-171.249463176904));
#149615=CARTESIAN_POINT('Origin',(-52.8706140943225,12.61999998,-170.949706593448));
#149616=CARTESIAN_POINT('Ctrl Pts',(-52.5103994272594,12.4456688709067,
-171.249463146917));
#149617=CARTESIAN_POINT('Ctrl Pts',(-52.5325366961564,12.4442258341098,
-171.275226079363));
#149618=CARTESIAN_POINT('Ctrl Pts',(-52.5530277603095,12.4430004743987,
-171.301970103452));
#149619=CARTESIAN_POINT('Ctrl Pts',(-52.5718680671356,12.4420632072567,
-171.329650850542));
#149620=CARTESIAN_POINT('Ctrl Pts',(-52.5908098491538,12.4411208919293,
-171.357480688046));
#149621=CARTESIAN_POINT('Ctrl Pts',(-52.6080841933948,12.4404700110404,
-171.386258116276));
#149622=CARTESIAN_POINT('Ctrl Pts',(-52.623669495073,12.4401548684418,-171.415979764924));
#149623=CARTESIAN_POINT('Ctrl Pts',(-52.6392009898804,12.4398408138451,
-171.445598802217));
#149624=CARTESIAN_POINT('Ctrl Pts',(-52.6530559575077,12.439860219518,-171.476156593959));
#149625=CARTESIAN_POINT('Ctrl Pts',(-52.665181108264,12.4402279645502,-171.507677529715));
#149626=CARTESIAN_POINT('Ctrl Pts',(-52.6682114522294,12.4403198721859,
-171.515555310319));
#149627=CARTESIAN_POINT('Ctrl Pts',(-52.6711335593541,12.4404333955636,
-171.523493340927));
#149628=CARTESIAN_POINT('Ctrl Pts',(-52.6739461945108,12.4405684861021,
-171.531492148308));
#149629=CARTESIAN_POINT('Ctrl Pts',(-52.6852405434796,12.4411109523655,
-171.563611963663));
#149630=CARTESIAN_POINT('Ctrl Pts',(-52.6945617501349,12.4420117639115,
-171.596133997172));
#149631=CARTESIAN_POINT('Ctrl Pts',(-52.7019620487256,12.4433297091624,
-171.629022442916));
#149632=CARTESIAN_POINT('Ctrl Pts',(-52.7094702315576,12.444666867898,-171.66239034837));
#149633=CARTESIAN_POINT('Ctrl Pts',(-52.7150019789283,12.4464332409464,
-171.696136308534));
#149634=CARTESIAN_POINT('Ctrl Pts',(-52.7185804246579,12.4486728316355,
-171.730263044942));
#149635=CARTESIAN_POINT('Ctrl Pts',(-52.7221795352094,12.4509253555213,
-171.764586856555));
#149636=CARTESIAN_POINT('Ctrl Pts',(-52.723803419686,12.4536561359556,-171.799296939246));
#149637=CARTESIAN_POINT('Ctrl Pts',(-52.7234321145001,12.4568970612263,
-171.834421393416));
#149638=CARTESIAN_POINT('Ctrl Pts',(-52.723357573706,12.4575476881298,-171.841472748491));
#149639=CARTESIAN_POINT('Ctrl Pts',(-52.7232024646285,12.458218847644,-171.84854085354));
#149640=CARTESIAN_POINT('Ctrl Pts',(-52.7229663801057,12.4589107657309,
-171.855625995355));
#149641=CARTESIAN_POINT('Ctrl Pts',(-52.811758955289,12.11999998,-170.861259130871));
#149642=CARTESIAN_POINT('Ctrl Pts',(-52.5194581681217,12.11999998,-171.0127167027));
#149643=CARTESIAN_POINT('Ctrl Pts',(-52.4039495302269,12.4224147476539,
-171.07256826174));
#149644=CARTESIAN_POINT('Ctrl Pts',(-52.8281457246307,12.11999998,-170.892884198111));
#149645=CARTESIAN_POINT('Ctrl Pts',(-52.5427333133061,12.11999998,-171.068676662146));
#149646=CARTESIAN_POINT('Ctrl Pts',(-52.4335834030071,12.4288943780099,
-171.135818022105));
#149647=CARTESIAN_POINT('Ctrl Pts',(-52.8478360402188,12.11999998,-170.922334416373));
#149648=CARTESIAN_POINT('Ctrl Pts',(-52.5708615508922,12.11999998,-171.121670121752));
#149649=CARTESIAN_POINT('Ctrl Pts',(-52.4691942899059,12.4366759982665,
-171.194717391534));
#149650=CARTESIAN_POINT('Ctrl Pts',(-52.8706140943225,12.11999998,-170.949706593448));
#149651=CARTESIAN_POINT('Ctrl Pts',(-52.6035237155536,12.11999998,-171.171968757444));
#149652=CARTESIAN_POINT('Ctrl Pts',(-52.5103993792154,12.4456688476555,
-171.249463186897));
#149653=CARTESIAN_POINT('',(-52.4039495302269,12.4224147476539,-171.07256826174));
#149654=CARTESIAN_POINT('Origin',(-52.811758955289,12.61999998,-170.861259130871));
#149655=CARTESIAN_POINT('Origin',(-53.2781268802541,12.612394155154,-170.643546468484));
#149656=CARTESIAN_POINT('Ctrl Pts',(-52.4039495302269,12.4224147476539,
-171.07256826174));
#149657=CARTESIAN_POINT('Ctrl Pts',(-52.5194581681217,12.11999998,-171.0127167027));
#149658=CARTESIAN_POINT('Ctrl Pts',(-52.811758955289,12.11999998,-170.861259130871));
#149659=CARTESIAN_POINT('Ctrl Pts',(-50.4067968770089,12.4163544181458,
-167.212559451309));
#149660=CARTESIAN_POINT('Ctrl Pts',(-50.5326451268968,12.11999998,-167.168095406566));
#149661=CARTESIAN_POINT('Ctrl Pts',(-50.8116692616976,12.11999998,-167.001248800573));
#149662=CARTESIAN_POINT('Ctrl Pts',(-48.3933978906048,12.4097551621214,
-163.361420582663));
#149663=CARTESIAN_POINT('Ctrl Pts',(-48.5227235736013,12.1199999799924,
-163.318503470872));
#149664=CARTESIAN_POINT('Ctrl Pts',(-48.7949136859973,12.11999998,-163.150111451781));
#149665=CARTESIAN_POINT('Ctrl Pts',(-44.3204976166945,12.3951430089669,
-155.684386060413));
#149666=CARTESIAN_POINT('Ctrl Pts',(-44.4529340155615,12.1199999800075,
-155.63827143996));
#149667=CARTESIAN_POINT('Ctrl Pts',(-44.7140165615046,12.11999998,-155.473076929555));
#149668=CARTESIAN_POINT('Ctrl Pts',(-42.2612000992887,12.3871318438137,
-151.858374821466));
#149669=CARTESIAN_POINT('Ctrl Pts',(-42.3975527923274,12.11999998,-151.814329756678));
#149670=CARTESIAN_POINT('Ctrl Pts',(-42.6500851427248,12.11999998,-151.647062446733));
#149671=CARTESIAN_POINT('Ctrl Pts',(-40.1676286103837,12.3781782553102,
-148.051158746523));
#149672=CARTESIAN_POINT('Ctrl Pts',(-40.2925576368927,12.11999998,-147.98227543296));
#149673=CARTESIAN_POINT('Ctrl Pts',(-40.5508657493446,12.11999998,-147.839849615653));
#149674=CARTESIAN_POINT('',(-40.1676233686655,12.3782630082023,-148.051084687213));
#149675=CARTESIAN_POINT('Origin',(-40.5508657493455,12.6199999799991,-147.839849615653));
#149676=CARTESIAN_POINT('Ctrl Pts',(-40.1676286103913,12.3781782553039,
-148.05115874653));
#149677=CARTESIAN_POINT('Ctrl Pts',(-42.2612000992887,12.3871318438137,
-151.858374821466));
#149678=CARTESIAN_POINT('Ctrl Pts',(-44.3204976166945,12.3951430089669,
-155.684386060413));
#149679=CARTESIAN_POINT('Ctrl Pts',(-48.3933978906048,12.4097551621214,
-163.361420582663));
#149680=CARTESIAN_POINT('Ctrl Pts',(-50.4067968770089,12.4163544181458,
-167.212559451309));
#149681=CARTESIAN_POINT('Ctrl Pts',(-52.4039495302269,12.4224147476539,
-171.07256826174));
#149682=CARTESIAN_POINT('Ctrl Pts',(-39.5011854382618,12.11999998,-143.364449166524));
#149683=CARTESIAN_POINT('Ctrl Pts',(-38.9925241823799,12.11999998,-143.356382176468));
#149684=CARTESIAN_POINT('Ctrl Pts',(-39.0013190202884,12.6286555741689,
-143.356503342193));
#149685=CARTESIAN_POINT('Ctrl Pts',(-39.4888154687586,12.11999998,-144.170854505439));
#149686=CARTESIAN_POINT('Ctrl Pts',(-39.0234415001674,12.11999998,-144.168885424266));
#149687=CARTESIAN_POINT('Ctrl Pts',(-38.9875647212365,12.5840154882559,
-144.20450574525));
#149688=CARTESIAN_POINT('Ctrl Pts',(-39.5732179658618,12.11999998,-144.962464848579));
#149689=CARTESIAN_POINT('Ctrl Pts',(-39.144316819298,12.11999998,-144.998554248167));
#149690=CARTESIAN_POINT('Ctrl Pts',(-39.0813386654269,12.5398855005079,
-145.035762056675));
#149691=CARTESIAN_POINT('Ctrl Pts',(-39.9390749458245,12.11999998,-146.514415033293));
#149692=CARTESIAN_POINT('Ctrl Pts',(-39.5960174049575,12.11999998,-146.600763849103));
#149693=CARTESIAN_POINT('Ctrl Pts',(-39.4878341117614,12.4529560363788,
-146.663462436008));
#149694=CARTESIAN_POINT('Ctrl Pts',(-40.2242048982474,12.11999998,-147.279924873294));
#149695=CARTESIAN_POINT('Ctrl Pts',(-39.9191166230722,12.11999998,-147.391920922171));
#149696=CARTESIAN_POINT('Ctrl Pts',(-39.8046575553952,12.4098586926345,
-147.465310993273));
#149697=CARTESIAN_POINT('Ctrl Pts',(-40.6264968255545,12.11999998,-147.973584999442));
#149698=CARTESIAN_POINT('Ctrl Pts',(-40.3763612390272,12.11999998,-148.118773982031));
#149699=CARTESIAN_POINT('Ctrl Pts',(-40.2516272065149,12.3706972604334,
-148.191122309056));
#149700=CARTESIAN_POINT('',(-39.,12.61999998,-143.518796834034));
#149701=CARTESIAN_POINT('Origin',(-39.5,12.61999998,-143.518796834034));
#149702=CARTESIAN_POINT('Ctrl Pts',(-39.,12.61999998,-143.518796834034));
#149703=CARTESIAN_POINT('Ctrl Pts',(-39.0000000062752,12.6119352885895,
-143.671852275596));
#149704=CARTESIAN_POINT('Ctrl Pts',(-39.0036267878565,12.6038716318385,
-143.824372346437));
#149705=CARTESIAN_POINT('Ctrl Pts',(-39.0107948009928,12.5958320293859,
-143.976333330001));
#149706=CARTESIAN_POINT('Ctrl Pts',(-39.018273628606,12.5874438191974,-144.134883541672));
#149707=CARTESIAN_POINT('Ctrl Pts',(-39.0296066235717,12.5790811718621,
-144.292825751123));
#149708=CARTESIAN_POINT('Ctrl Pts',(-39.0447472042233,12.5707473406039,
-144.450154052002));
#149709=CARTESIAN_POINT('Ctrl Pts',(-39.0594100046057,12.562676493985,-144.602517658352));
#149710=CARTESIAN_POINT('Ctrl Pts',(-39.0776439179631,12.5546318065498,
-144.754306301496));
#149711=CARTESIAN_POINT('Ctrl Pts',(-39.0994578733345,12.5466067917887,
-144.905522814717));
#149712=CARTESIAN_POINT('Ctrl Pts',(-39.1211182504263,12.538638276087,-145.055674707993));
#149713=CARTESIAN_POINT('Ctrl Pts',(-39.1463084852436,12.53068835278,-145.205263225827));
#149714=CARTESIAN_POINT('Ctrl Pts',(-39.175088270677,12.5227534543617,-145.354288091831));
#149715=CARTESIAN_POINT('Ctrl Pts',(-39.2033745208226,12.5149546289654,
-145.500757378319));
#149716=CARTESIAN_POINT('Ctrl Pts',(-39.2351285884225,12.5071695759667,
-145.64668282469));
#149717=CARTESIAN_POINT('Ctrl Pts',(-39.2704536342457,12.4994090078912,
-145.792051096222));
#149718=CARTESIAN_POINT('Ctrl Pts',(-39.2751179610196,12.4983843007857,
-145.811245554577));
#149719=CARTESIAN_POINT('Ctrl Pts',(-39.2798446093254,12.4973600503235,
-145.830430271798));
#149720=CARTESIAN_POINT('Ctrl Pts',(-39.2846338730941,12.4963363105606,
-145.84960519063));
#149721=CARTESIAN_POINT('Ctrl Pts',(-39.3228940288552,12.4881579255985,
-146.002788522491));
#149722=CARTESIAN_POINT('Ctrl Pts',(-39.3651577699322,12.4800894902938,
-146.155474174756));
#149723=CARTESIAN_POINT('Ctrl Pts',(-39.4115476402542,12.4720604749179,
-146.307305745164));
#149724=CARTESIAN_POINT('Ctrl Pts',(-39.4576308395821,12.4640845372098,
-146.458133597771));
#149725=CARTESIAN_POINT('Ctrl Pts',(-39.5077865778487,12.4561471247028,
-146.608118946099));
#149726=CARTESIAN_POINT('Ctrl Pts',(-39.5621399172821,12.4482218744652,
-146.756880619399));
#149727=CARTESIAN_POINT('Ctrl Pts',(-39.6132477630658,12.4407698490485,
-146.896759580596));
#149728=CARTESIAN_POINT('Ctrl Pts',(-39.6680675972591,12.4333287413512,
-147.035556528922));
#149729=CARTESIAN_POINT('Ctrl Pts',(-39.7266970656795,12.4259153625784,
-147.172925407409));
#149730=CARTESIAN_POINT('Ctrl Pts',(-39.7840967394881,12.4186574846744,
-147.307412876408));
#149731=CARTESIAN_POINT('Ctrl Pts',(-39.8451486132704,12.4114262190347,
-147.440531530225));
#149732=CARTESIAN_POINT('Ctrl Pts',(-39.9099278090628,12.4042745591491,
-147.571928505937));
#149733=CARTESIAN_POINT('Ctrl Pts',(-39.9729591449271,12.397315863989,-147.699780153467));
#149734=CARTESIAN_POINT('Ctrl Pts',(-40.0395200099146,12.3904327283686,
-147.826001622394));
#149735=CARTESIAN_POINT('Ctrl Pts',(-40.1096540546844,12.3837078549757,
-147.950242323608));
#149736=CARTESIAN_POINT('Ctrl Pts',(-40.1287133093867,12.3818803391771,
-147.984005315271));
#149737=CARTESIAN_POINT('Ctrl Pts',(-40.1480362664377,12.3800646988528,
-148.017621885214));
#149738=CARTESIAN_POINT('Ctrl Pts',(-40.1676233686655,12.3782630082023,
-148.051084687213));
#149739=CARTESIAN_POINT('Origin',(-39.5,12.61999998,-55.24995));
#149740=CARTESIAN_POINT('',(-39.,12.61999998,-88.5398461374725));
#149741=CARTESIAN_POINT('Origin',(-39.5,12.61999998,-88.5398461374725));
#149742=CARTESIAN_POINT('',(-39.,12.61999998,-129.34995));
#149743=CARTESIAN_POINT('Ctrl Pts',(-40.5508657493525,12.11999998,-84.2187933558389));
#149744=CARTESIAN_POINT('Ctrl Pts',(-40.2925576369006,12.11999998,-84.0763675385317));
#149745=CARTESIAN_POINT('Ctrl Pts',(-40.1676286103916,12.3781782553103,
-84.0074842249685));
#149746=CARTESIAN_POINT('Ctrl Pts',(-40.1865238705097,12.11999998,-84.8795757011402));
#149747=CARTESIAN_POINT('Ctrl Pts',(-39.8775141197021,12.1199999800054,
-84.7681083762916));
#149748=CARTESIAN_POINT('Ctrl Pts',(-39.7628532325843,12.4154575211986,
-84.6989357525887));
#149749=CARTESIAN_POINT('Ctrl Pts',(-39.9318518139617,12.11999998,-85.5794220290239));
#149750=CARTESIAN_POINT('Ctrl Pts',(-39.5877950605282,12.11999998,-85.491056146558));
#149751=CARTESIAN_POINT('Ctrl Pts',(-39.4798353483971,12.4548420036467,
-85.4321181873043));
#149752=CARTESIAN_POINT('Ctrl Pts',(-39.6727396192083,12.11999998,-86.6717926677035));
#149753=CARTESIAN_POINT('Ctrl Pts',(-39.2736158380134,12.11999998,-86.5998217220713));
#149754=CARTESIAN_POINT('Ctrl Pts',(-39.1919329104561,12.5160219327601,
-86.5777868689076));
#149755=CARTESIAN_POINT('Ctrl Pts',(-39.6078129604692,12.11999998,-87.0440021565177));
#149756=CARTESIAN_POINT('Ctrl Pts',(-39.1889752494415,12.11999998,-86.9856596406021));
#149757=CARTESIAN_POINT('Ctrl Pts',(-39.1197921781136,12.5368211423774,
-86.9683825953982));
#149758=CARTESIAN_POINT('Ctrl Pts',(-39.5216886477957,12.11999998,-87.7889298981597));
#149759=CARTESIAN_POINT('Ctrl Pts',(-39.0619634825428,12.11999998,-87.7602623143372));
#149760=CARTESIAN_POINT('Ctrl Pts',(-39.0240984977364,12.5783336340252,
-87.7505987241496));
#149761=CARTESIAN_POINT('Ctrl Pts',(-39.5000000006739,12.11999998,-88.163385731595));
#149762=CARTESIAN_POINT('Ctrl Pts',(-39.0204289960451,12.11999998,-88.152135192235));
#149763=CARTESIAN_POINT('Ctrl Pts',(-39.,12.5991444608023,-88.1440404246245));
#149764=CARTESIAN_POINT('Ctrl Pts',(-39.5,12.11999998,-88.5398461374725));
#149765=CARTESIAN_POINT('Ctrl Pts',(-39.,12.11999998,-88.5398461374725));
#149766=CARTESIAN_POINT('Ctrl Pts',(-39.,12.61999998,-88.5398461374725));
#149767=CARTESIAN_POINT('',(-40.1676094221395,12.3781800225324,-84.0075170032023));
#149768=CARTESIAN_POINT('Origin',(-40.5508657493525,12.61999998,-84.2187933558389));
#149769=CARTESIAN_POINT('Ctrl Pts',(-40.1676094221395,12.3781800225324,
-84.0075170032023));
#149770=CARTESIAN_POINT('Ctrl Pts',(-39.7628442883141,12.4154587658777,
-84.6989589235648));
#149771=CARTESIAN_POINT('Ctrl Pts',(-39.4798323155101,12.4548426481422,
-85.4321302562663));
#149772=CARTESIAN_POINT('Ctrl Pts',(-39.2879003897697,12.4956286230557,
-86.1958973083732));
#149773=CARTESIAN_POINT('Ctrl Pts',(-39.1919329104561,12.5160219327601,
-86.5777868689076));
#149774=CARTESIAN_POINT('Ctrl Pts',(-39.1197921781136,12.5368211423774,
-86.9683825953982));
#149775=CARTESIAN_POINT('Ctrl Pts',(-39.071945337925,12.5575773882013,-87.3594906597739));
#149776=CARTESIAN_POINT('Ctrl Pts',(-39.0240984977364,12.5783336340252,
-87.7505987241496));
#149777=CARTESIAN_POINT('Ctrl Pts',(-39.,12.5991444608023,-88.1440404246245));
#149778=CARTESIAN_POINT('Ctrl Pts',(-39.,12.61999998,-88.5398461374725));
#149779=CARTESIAN_POINT('Ctrl Pts',(-40.1676286103916,12.3781782553103,
-84.0074842249685));
#149780=CARTESIAN_POINT('Ctrl Pts',(-40.2925576369006,12.11999998,-84.0763675385317));
#149781=CARTESIAN_POINT('Ctrl Pts',(-40.5508657493525,12.11999998,-84.2187933558389));
#149782=CARTESIAN_POINT('Ctrl Pts',(-42.2393869130494,12.3870385552721,
-80.2399360160109));
#149783=CARTESIAN_POINT('Ctrl Pts',(-42.3754889509591,12.11999998,-80.2844795011615));
#149784=CARTESIAN_POINT('Ctrl Pts',(-42.6282131590433,12.11999998,-80.4512482683356));
#149785=CARTESIAN_POINT('Ctrl Pts',(-44.2775738677864,12.39497584134,-76.4539726940548));
#149786=CARTESIAN_POINT('Ctrl Pts',(-44.4098483480378,12.11999998,-76.5004916194052));
#149787=CARTESIAN_POINT('Ctrl Pts',(-44.6709958246245,12.11999998,-76.6652818249261));
#149788=CARTESIAN_POINT('Ctrl Pts',(-48.3090097368786,12.4094651694423,
-68.8574405644517));
#149789=CARTESIAN_POINT('Ctrl Pts',(-48.4382080167511,12.11999998,-68.9007945866128));
#149790=CARTESIAN_POINT('Ctrl Pts',(-48.710372157466,12.11999998,-69.0687496953211));
#149791=CARTESIAN_POINT('Ctrl Pts',(-50.3020637690764,12.4160155627679,
-65.046761180979));
#149792=CARTESIAN_POINT('Ctrl Pts',(-50.4278516292118,12.1199999799963,
-65.0915922935902));
#149793=CARTESIAN_POINT('Ctrl Pts',(-50.7067648613536,12.11999998,-65.2580717844373));
#149794=CARTESIAN_POINT('Ctrl Pts',(-52.2790965136749,12.4220352393542,
-61.2273317382593));
#149795=CARTESIAN_POINT('Ctrl Pts',(-52.3947118718251,12.11999998,-61.287265650179));
#149796=CARTESIAN_POINT('Ctrl Pts',(-52.6867218473722,12.11999998,-61.4386408691297));
#149797=CARTESIAN_POINT('Origin',(-52.6867218473722,12.61999998,-61.4386408691297));
#149798=CARTESIAN_POINT('Ctrl Pts',(-52.2790965136749,12.4220352393542,
-61.2273317382593));
#149799=CARTESIAN_POINT('Ctrl Pts',(-50.3020637710939,12.4160155580201,
-65.0467611816981));
#149800=CARTESIAN_POINT('Ctrl Pts',(-48.3090097389604,12.409465164778,-68.8574405651503));
#149801=CARTESIAN_POINT('Ctrl Pts',(-44.2775738699394,12.3949758368643,
-76.453972694812));
#149802=CARTESIAN_POINT('Ctrl Pts',(-42.2393869152768,12.3870385509018,
-80.2399360167399));
#149803=CARTESIAN_POINT('Ctrl Pts',(-40.1676286103916,12.3781782553103,
-84.0074842249685));
#149804=CARTESIAN_POINT('Ctrl Pts',(-52.8224784153177,12.11999998,-61.275204160084));
#149805=CARTESIAN_POINT('Ctrl Pts',(-52.5913010098401,12.11999998,-60.9843891047162));
#149806=CARTESIAN_POINT('Ctrl Pts',(-52.5245819708721,12.475697298624,-60.9004583201679));
#149807=CARTESIAN_POINT('Ctrl Pts',(-52.7664652938449,12.11999998,-61.3197306493527));
#149808=CARTESIAN_POINT('Ctrl Pts',(-52.5094515064391,12.1199999800004,
-61.0719533871486));
#149809=CARTESIAN_POINT('Ctrl Pts',(-52.4232534240833,12.4535953097813,
-60.9895181215267));
#149810=CARTESIAN_POINT('Ctrl Pts',(-52.7200145740509,12.11999998,-61.3744177048719));
#149811=CARTESIAN_POINT('Ctrl Pts',(-52.4421916143175,12.11999998,-61.1731178858937));
#149812=CARTESIAN_POINT('Ctrl Pts',(-52.339276259362,12.4352188308071,-61.0988911211005));
#149813=CARTESIAN_POINT('Ctrl Pts',(-52.6867218473722,12.11999998,-61.4386408691297));
#149814=CARTESIAN_POINT('Ctrl Pts',(-52.3947118718252,12.11999998,-61.287265650179));
#149815=CARTESIAN_POINT('Ctrl Pts',(-52.2790965136749,12.4220352393542,
-61.2273317382593));
#149816=CARTESIAN_POINT('Origin',(-52.8224784153158,12.6199999800056,-61.2752041600831));
#149817=CARTESIAN_POINT('Ctrl Pts',(-52.5245819708698,12.4756972986233,
-60.9004583201698));
#149818=CARTESIAN_POINT('Ctrl Pts',(-52.5913010098385,12.11999998,-60.9843891047178));
#149819=CARTESIAN_POINT('Ctrl Pts',(-52.8224784153175,12.11999998,-61.2752041600839));
#149820=CARTESIAN_POINT('Ctrl Pts',(-52.6505629615106,12.4839221309077,
-60.7971452199062));
#149821=CARTESIAN_POINT('Ctrl Pts',(-52.7297264322295,12.1199999799996,
-60.865773772671));
#149822=CARTESIAN_POINT('Ctrl Pts',(-53.0127900201976,12.11999998,-61.1239198608288));
#149823=CARTESIAN_POINT('Ctrl Pts',(-52.7486445377005,12.4996864767879,
-60.660571058145));
#149824=CARTESIAN_POINT('Ctrl Pts',(-52.8314129775774,12.1199999800002,
-60.7072763762979));
#149825=CARTESIAN_POINT('Ctrl Pts',(-53.1625689933938,12.11999998,-60.9259844495965));
#149826=CARTESIAN_POINT('Ctrl Pts',(-52.81219032515,12.5218539749099,-60.5055220850798));
#149827=CARTESIAN_POINT('Ctrl Pts',(-52.8857929788878,12.11999998,-60.5379900686008));
#149828=CARTESIAN_POINT('Ctrl Pts',(-53.2607580814926,12.11999998,-60.7033966151602));
#149829=CARTESIAN_POINT('Origin',(-59.5,11.61999998,-55.24995));
#149830=CARTESIAN_POINT('',(-60.,11.61999998,-174.34995));
#149831=CARTESIAN_POINT('Origin',(-59.5,11.61999998,-174.34995));
#149832=CARTESIAN_POINT('',(-60.,11.61999998,-58.24995));
#149833=CARTESIAN_POINT('Origin',(-57.,11.61999998,-174.34995));
#149834=CARTESIAN_POINT('Origin',(-57.,11.61999998,-174.34995));
#149835=CARTESIAN_POINT('Origin',(0.,-12.9675000200281,-60.64995));
#149836=CARTESIAN_POINT('',(-40.4031452851323,17.9943647515726,-76.7018642453134));
#149837=CARTESIAN_POINT('Ctrl Pts',(-40.1676234671477,12.3782653664715,
-84.0075554250447));
#149838=CARTESIAN_POINT('Ctrl Pts',(-40.1941985853479,13.012226003964,-83.2338432608986));
#149839=CARTESIAN_POINT('Ctrl Pts',(-40.2205526779777,13.6386751861752,
-82.4505770135348));
#149840=CARTESIAN_POINT('Ctrl Pts',(-40.2466278643551,14.2587699734049,
-81.6591515576613));
#149841=CARTESIAN_POINT('Ctrl Pts',(-40.3002576413502,15.5341413043586,
-80.0313982564001));
#149842=CARTESIAN_POINT('Ctrl Pts',(-40.352516590638,16.777641980889,-78.3751691578809));
#149843=CARTESIAN_POINT('Ctrl Pts',(-40.4031453084497,17.9943647931319,
-76.7018643085084));
#149844=CARTESIAN_POINT('Ctrl Pts',(-40.4031453149964,17.9943646866131,
-76.7018642268486));
#149845=CARTESIAN_POINT('Ctrl Pts',(-43.3980120961201,18.0071650557604,
-71.5873748987318));
#149846=CARTESIAN_POINT('Ctrl Pts',(-46.3056933853622,18.0183276393305,
-66.4219286454218));
#149847=CARTESIAN_POINT('Ctrl Pts',(-49.1629069712534,18.0283224583225,
-61.2273317382593));
#149848=CARTESIAN_POINT('Ctrl Pts',(-49.5462350640495,18.76999998,-61.4386408691297));
#149849=CARTESIAN_POINT('Ctrl Pts',(-48.8042785465888,18.76999998,-61.0296382684994));
#149850=CARTESIAN_POINT('Ctrl Pts',(-49.1629069712534,18.0283224583225,
-61.2273317382593));
#149851=CARTESIAN_POINT('Ctrl Pts',(-49.5720983755525,18.76999998,-61.3917233465932));
#149852=CARTESIAN_POINT('Ctrl Pts',(-48.8976639972856,18.7699999800003,
-60.912976735742));
#149853=CARTESIAN_POINT('Ctrl Pts',(-49.2072136788996,18.0400790290492,
-61.1335104039183));
#149854=CARTESIAN_POINT('Ctrl Pts',(-49.6050257059303,18.76999998,-61.3505216375984));
#149855=CARTESIAN_POINT('Ctrl Pts',(-49.0074625403989,18.7699999800005,
-60.8254916046238));
#149856=CARTESIAN_POINT('Ctrl Pts',(-49.2636489250068,18.0550404895701,
-61.0510932718963));
#149857=CARTESIAN_POINT('Ctrl Pts',(-49.6828096124638,18.76999998,-61.2778731737785));
#149858=CARTESIAN_POINT('Ctrl Pts',(-49.2376424762765,18.7699999799996,
-60.6973789326117));
#149859=CARTESIAN_POINT('Ctrl Pts',(-49.3970153298707,18.0903238932961,
-60.9057963508575));
#149860=CARTESIAN_POINT('Ctrl Pts',(-49.7267438680042,18.76999998,-61.2475100972213));
#149861=CARTESIAN_POINT('Ctrl Pts',(-49.3535760550633,18.7699999800002,
-60.656860805429));
#149862=CARTESIAN_POINT('Ctrl Pts',(-49.4723725947842,18.1102284712985,
-60.8450701877959));
#149863=CARTESIAN_POINT('Ctrl Pts',(-49.8682179142305,18.76999998,-61.1743894610928));
#149864=CARTESIAN_POINT('Ctrl Pts',(-49.6800903574717,18.7699999799997,
-60.5889551600382));
#149865=CARTESIAN_POINT('Ctrl Pts',(-49.7151670266325,18.1742094267258,
-60.6988289354793));
#149866=CARTESIAN_POINT('Ctrl Pts',(-49.9744290136678,18.76999998,-61.1499500118827));
#149867=CARTESIAN_POINT('Ctrl Pts',(-49.8890563478339,18.76999998,-60.5998057785282));
#149868=CARTESIAN_POINT('Ctrl Pts',(-49.897617121419,18.2220908968247,-60.64995));
#149869=CARTESIAN_POINT('Ctrl Pts',(-50.0811190791972,18.76999998,-61.14995));
#149870=CARTESIAN_POINT('Ctrl Pts',(-50.0811190791972,18.76999998,-60.64995));
#149871=CARTESIAN_POINT('Ctrl Pts',(-50.0811190791972,18.26999998,-60.64995));
#149872=CARTESIAN_POINT('Origin',(-49.5462350640495,18.26999998,-61.4386408691297));
#149873=CARTESIAN_POINT('Origin',(-50.0811190791972,18.26999998,-61.14995));
#149874=CARTESIAN_POINT('Origin',(83.2809572255632,18.26999998,-61.14995));
#149875=CARTESIAN_POINT('Ctrl Pts',(-49.1629069712534,18.0283224583225,
-61.2273317382593));
#149876=CARTESIAN_POINT('Ctrl Pts',(-48.8042785465888,18.76999998,-61.0296382684995));
#149877=CARTESIAN_POINT('Ctrl Pts',(-49.5462350640495,18.76999998,-61.4386408691297));
#149878=CARTESIAN_POINT('Ctrl Pts',(-46.3056933853622,18.0183276393305,
-66.4219286454218));
#149879=CARTESIAN_POINT('Ctrl Pts',(-45.867410270929,18.769999980105,-66.3106234612426));
#149880=CARTESIAN_POINT('Ctrl Pts',(-46.6827176097033,18.76999998,-66.6332421622494));
#149881=CARTESIAN_POINT('Ctrl Pts',(-43.3980120961201,18.0071650557604,
-71.5873748987318));
#149882=CARTESIAN_POINT('Ctrl Pts',(-42.9058979134104,18.76999997996,-71.4956126488948));
#149883=CARTESIAN_POINT('Ctrl Pts',(-43.7675014857899,18.76999998,-71.7986930470318));
#149884=CARTESIAN_POINT('Ctrl Pts',(-40.4031453149964,17.9943646866131,
-76.7018642268486));
#149885=CARTESIAN_POINT('Ctrl Pts',(-39.9612665046713,18.76999998,-76.4422678974524));
#149886=CARTESIAN_POINT('Ctrl Pts',(-40.7628307834967,18.76999998,-76.913173357719));
#149887=CARTESIAN_POINT('Origin',(-40.7628307834967,18.26999998,-76.9131733577189));
#149888=CARTESIAN_POINT('Ctrl Pts',(-39.5,18.76999998,-81.9737790469184));
#149889=CARTESIAN_POINT('Ctrl Pts',(-39.0000000000011,18.76999998,-81.9737790469193));
#149890=CARTESIAN_POINT('Ctrl Pts',(-39.,18.2699999800011,-81.9737790469193));
#149891=CARTESIAN_POINT('Ctrl Pts',(-39.5000000014778,18.76999998,-81.0900715307985));
#149892=CARTESIAN_POINT('Ctrl Pts',(-38.9495856510588,18.76999998,-81.0044062795137));
#149893=CARTESIAN_POINT('Ctrl Pts',(-38.9999999999983,18.2220313158448,
-81.0514322138321));
#149894=CARTESIAN_POINT('Ctrl Pts',(-39.5988774762002,18.76999998,-80.2205083311056));
#149895=CARTESIAN_POINT('Ctrl Pts',(-39.0100135050444,18.76999998,-80.0786830893324));
#149896=CARTESIAN_POINT('Ctrl Pts',(-39.1098638639319,18.1747125385734,
-80.1448153615248));
#149897=CARTESIAN_POINT('Ctrl Pts',(-39.9044907342272,18.76999998,-78.9396134649389));
#149898=CARTESIAN_POINT('Ctrl Pts',(-39.229508253648,18.7699999800001,-78.7338553009239));
#149899=CARTESIAN_POINT('Ctrl Pts',(-39.4494341483978,18.1049192927842,
-78.810548635267));
#149900=CARTESIAN_POINT('Ctrl Pts',(-40.0341671712988,18.76999998,-78.514605681855));
#149901=CARTESIAN_POINT('Ctrl Pts',(-39.3342349384753,18.76999998,-78.2659886991342));
#149902=CARTESIAN_POINT('Ctrl Pts',(-39.5935190801229,18.0817455339462,
-78.3680408652321));
#149903=CARTESIAN_POINT('Ctrl Pts',(-40.3511672955439,18.76999998,-77.6933701733068));
#149904=CARTESIAN_POINT('Ctrl Pts',(-39.5993180096537,18.76999998,-77.3418642254583));
#149905=CARTESIAN_POINT('Ctrl Pts',(-39.9457414385913,18.036947832209,-77.5133471330197));
#149906=CARTESIAN_POINT('Ctrl Pts',(-40.5384105179099,18.76999998,-77.2951763044633));
#149907=CARTESIAN_POINT('Ctrl Pts',(-39.7649903796933,18.76999998,-76.8813885224012));
#149908=CARTESIAN_POINT('Ctrl Pts',(-40.1537986734602,18.0152160834001,
-77.0990973343972));
#149909=CARTESIAN_POINT('Ctrl Pts',(-40.7628307834967,18.76999998,-76.913173357719));
#149910=CARTESIAN_POINT('Ctrl Pts',(-39.9612665046713,18.76999998,-76.4422678974524));
#149911=CARTESIAN_POINT('Ctrl Pts',(-40.4031453149964,17.9943646866131,
-76.7018642268486));
#149912=CARTESIAN_POINT('',(-39.,18.2699999799838,-81.9737790469184));
#149913=CARTESIAN_POINT('Origin',(-39.5,18.26999998,-81.9737790469175));
#149914=CARTESIAN_POINT('Ctrl Pts',(-39.,18.2699999800011,-81.9737790469184));
#149915=CARTESIAN_POINT('Ctrl Pts',(-38.9999999999983,18.2220313158448,
-81.0514322138315));
#149916=CARTESIAN_POINT('Ctrl Pts',(-39.109863863932,18.1747125385734,-80.1448153615245));
#149917=CARTESIAN_POINT('Ctrl Pts',(-39.3362440535758,18.1281837080473,
-79.2553042106863));
#149918=CARTESIAN_POINT('Ctrl Pts',(-39.4494341483978,18.1049192927842,
-78.810548635267));
#149919=CARTESIAN_POINT('Ctrl Pts',(-39.5935190801229,18.0817455339463,
-78.3680408652321));
#149920=CARTESIAN_POINT('Ctrl Pts',(-39.7696302593571,18.0593466830776,
-77.9406939991259));
#149921=CARTESIAN_POINT('Ctrl Pts',(-39.9457414342936,18.0369478327556,
-77.5133471434485));
#149922=CARTESIAN_POINT('Ctrl Pts',(-40.1537986633056,18.0152160844608,
-77.0990973546155));
#149923=CARTESIAN_POINT('Ctrl Pts',(-40.4031452967415,17.9943646881397,
-76.7018642559303));
#149924=CARTESIAN_POINT('Origin',(-39.5,18.26999998,-55.24995));
#149925=CARTESIAN_POINT('',(-39.,18.26999998,-150.084863924608));
#149926=CARTESIAN_POINT('Origin',(-39.5,18.26999998,-150.084863924608));
#149927=CARTESIAN_POINT('',(-39.,18.26999998,-129.34995));
#149928=CARTESIAN_POINT('Ctrl Pts',(-40.7628307834967,18.76999998,-155.145469613787));
#149929=CARTESIAN_POINT('Ctrl Pts',(-39.9612665046713,18.76999998,-155.616375074053));
#149930=CARTESIAN_POINT('Ctrl Pts',(-40.4031453149963,17.9943646866131,
-155.356778744658));
#149931=CARTESIAN_POINT('Ctrl Pts',(-40.5382265796732,18.76999998,-154.763153570891));
#149932=CARTESIAN_POINT('Ctrl Pts',(-39.7648410678857,18.76999998,-155.176920406762));
#149933=CARTESIAN_POINT('Ctrl Pts',(-40.1535949024652,18.0152331222464,
-154.959221008645));
#149934=CARTESIAN_POINT('Ctrl Pts',(-40.3517329455581,18.76999998,-154.366209991013));
#149935=CARTESIAN_POINT('Ctrl Pts',(-39.5997667004894,18.76999998,-154.717664579548));
#149936=CARTESIAN_POINT('Ctrl Pts',(-39.9463699385113,18.0368966498548,
-154.546270136328));
#149937=CARTESIAN_POINT('Ctrl Pts',(-40.0364383090907,18.76999998,-153.550444480173));
#149938=CARTESIAN_POINT('Ctrl Pts',(-39.3360417060011,18.76999998,-153.799575452297));
#149939=CARTESIAN_POINT('Ctrl Pts',(-39.5960425666541,18.0813960858844,
-153.697271402021));
#149940=CARTESIAN_POINT('Ctrl Pts',(-39.9079301282699,18.76999998,-153.131458232674));
#149941=CARTESIAN_POINT('Ctrl Pts',(-39.23220455254,18.76999998,-153.338508255374));
#149942=CARTESIAN_POINT('Ctrl Pts',(-39.4532556977585,18.1042418116532,
-153.261037480867));
#149943=CARTESIAN_POINT('Ctrl Pts',(-39.7023798052426,18.76999998,-152.273874561686));
#149944=CARTESIAN_POINT('Ctrl Pts',(-39.0797143668984,18.76999998,-152.409570079113));
#149945=CARTESIAN_POINT('Ctrl Pts',(-39.2248664505887,18.1509702537189,
-152.367727156036));
#149946=CARTESIAN_POINT('Ctrl Pts',(-39.6264148660465,18.76999998,-151.83867201801));
#149947=CARTESIAN_POINT('Ctrl Pts',(-39.0281802867267,18.76999998,-151.943644934638));
#149948=CARTESIAN_POINT('Ctrl Pts',(-39.1404609620539,18.1746678021094,
-151.914185519153));
#149949=CARTESIAN_POINT('Ctrl Pts',(-39.5253915082876,18.76999998,-150.965860868517));
#149950=CARTESIAN_POINT('Ctrl Pts',(-38.9776025606259,18.76999998,-151.019307709025));
#149951=CARTESIAN_POINT('Ctrl Pts',(-39.0282127872062,18.2221486757409,
-151.004139862532));
#149952=CARTESIAN_POINT('Ctrl Pts',(-39.5000000006086,18.76999998,-150.526727576342));
#149953=CARTESIAN_POINT('Ctrl Pts',(-38.9754245522527,18.76999998,-150.557403393481));
#149954=CARTESIAN_POINT('Ctrl Pts',(-39.,18.2460151034934,-150.546047809514));
#149955=CARTESIAN_POINT('Ctrl Pts',(-39.5,18.76999998,-150.084863924608));
#149956=CARTESIAN_POINT('Ctrl Pts',(-39.,18.76999998,-150.084863924608));
#149957=CARTESIAN_POINT('Ctrl Pts',(-39.,18.26999998,-150.084863924608));
#149958=CARTESIAN_POINT('',(-40.4031452850214,17.9943647518538,-155.356778726108));
#149959=CARTESIAN_POINT('Origin',(-40.7628307834967,18.26999998,-155.145469613787));
#149960=CARTESIAN_POINT('Ctrl Pts',(-40.4031452966654,17.994364688146,-155.356778715455));
#149961=CARTESIAN_POINT('Ctrl Pts',(-40.1535948923173,18.0152331233072,
-154.959220988423));
#149962=CARTESIAN_POINT('Ctrl Pts',(-39.9463699342223,18.0368966503995,
-154.546270125934));
#149963=CARTESIAN_POINT('Ctrl Pts',(-39.5960425666541,18.0813960858844,
-153.697271402021));
#149964=CARTESIAN_POINT('Ctrl Pts',(-39.4532556977585,18.1042418116532,
-153.261037480867));
#149965=CARTESIAN_POINT('Ctrl Pts',(-39.2248664505887,18.1509702537189,
-152.367727156036));
#149966=CARTESIAN_POINT('Ctrl Pts',(-39.1404609620539,18.1746678021094,
-151.914185519153));
#149967=CARTESIAN_POINT('Ctrl Pts',(-39.0282127872062,18.2221486757409,
-151.004139862532));
#149968=CARTESIAN_POINT('Ctrl Pts',(-39.,18.2460151034934,-150.546047809514));
#149969=CARTESIAN_POINT('Ctrl Pts',(-39.,18.26999998,-150.084863924608));
#149970=CARTESIAN_POINT('Ctrl Pts',(-40.4031453149964,17.9943646866131,
-155.356778744658));
#149971=CARTESIAN_POINT('Ctrl Pts',(-39.9612665046713,18.76999998,-155.616375074053));
#149972=CARTESIAN_POINT('Ctrl Pts',(-40.7628307834967,18.76999998,-155.145469613787));
#149973=CARTESIAN_POINT('Ctrl Pts',(-43.4443793123589,18.0073632340302,
-160.550451772752));
#149974=CARTESIAN_POINT('Ctrl Pts',(-42.9502082118644,18.76999998,-160.637466725898));
#149975=CARTESIAN_POINT('Ctrl Pts',(-43.8140202568649,18.76999998,-160.339133090562));
#149976=CARTESIAN_POINT('Ctrl Pts',(-46.3957674250336,18.0186733043079,
-165.796619822254));
#149977=CARTESIAN_POINT('Ctrl Pts',(-45.9568836537051,18.7699999799361,
-165.904661000913));
#149978=CARTESIAN_POINT('Ctrl Pts',(-46.773026135633,18.76999998,-165.585306091383));
#149979=CARTESIAN_POINT('Ctrl Pts',(-49.2955572616308,18.0287857662076,
-171.07256826174));
#149980=CARTESIAN_POINT('Ctrl Pts',(-48.9379852680023,18.76999998,-171.26952948831));
#149981=CARTESIAN_POINT('Ctrl Pts',(-49.6791770659623,18.76999998,-170.861259130871));
#149982=CARTESIAN_POINT('',(-49.2955572616308,18.0287857662077,-171.07256826174));
#149983=CARTESIAN_POINT('Origin',(-49.6791770659623,18.26999998,-170.861259130871));
#149984=CARTESIAN_POINT('Ctrl Pts',(-49.2955572616308,18.0287857662077,
-171.07256826174));
#149985=CARTESIAN_POINT('Ctrl Pts',(-46.3957674250336,18.0186733043079,
-165.796619822254));
#149986=CARTESIAN_POINT('Ctrl Pts',(-43.4443793123589,18.0073632340302,
-160.550451772752));
#149987=CARTESIAN_POINT('Ctrl Pts',(-40.4031453149964,17.9943646866131,
-155.356778744658));
#149988=CARTESIAN_POINT('Ctrl Pts',(-50.2136602208993,18.76999998,-171.14995));
#149989=CARTESIAN_POINT('Ctrl Pts',(-50.2136602208993,18.76999998,-171.64995));
#149990=CARTESIAN_POINT('Ctrl Pts',(-50.2136602208993,18.26999998,-171.64995));
#149991=CARTESIAN_POINT('Ctrl Pts',(-50.1601223770514,18.76999998,-171.149949978729));
#149992=CARTESIAN_POINT('Ctrl Pts',(-50.1192510514274,18.769999979997,-171.674554621579));
#149993=CARTESIAN_POINT('Ctrl Pts',(-50.1215225801538,18.2459873673078,
-171.64995));
#149994=CARTESIAN_POINT('Ctrl Pts',(-50.1077189781947,18.76999998,-171.143861566653));
#149995=CARTESIAN_POINT('Ctrl Pts',(-50.0232655392308,18.76999998,-171.688977816336));
#149996=CARTESIAN_POINT('Ctrl Pts',(-50.0313889586563,18.2224389306129,
-171.637773119416));
#149997=CARTESIAN_POINT('Ctrl Pts',(-50.005178217729,18.76999998,-171.11977321611));
#149998=CARTESIAN_POINT('Ctrl Pts',(-49.820539749869,18.76999998,-171.697170816346));
#149999=CARTESIAN_POINT('Ctrl Pts',(-49.8551127360827,18.1762799424075,
-171.589596446108));
#150000=CARTESIAN_POINT('Ctrl Pts',(-49.9542884930289,18.76999998,-171.101323338366));
#150001=CARTESIAN_POINT('Ctrl Pts',(-49.711275177471,18.7699999800001,-171.68935836961));
#150002=CARTESIAN_POINT('Ctrl Pts',(-49.7676788911518,18.1533289077801,
-171.552696670458));
#150003=CARTESIAN_POINT('Ctrl Pts',(-49.8603247967136,18.76999998,-171.052859322317));
#150004=CARTESIAN_POINT('Ctrl Pts',(-49.4884000599828,18.7699999799999,
-171.64306834795));
#150005=CARTESIAN_POINT('Ctrl Pts',(-49.6063178327574,18.1108845812496,
-171.455768650908));
#150006=CARTESIAN_POINT('Ctrl Pts',(-49.8169023670873,18.76999998,-171.023027979234));
#150007=CARTESIAN_POINT('Ctrl Pts',(-49.3740663050079,18.76999998,-171.603425591907));
#150008=CARTESIAN_POINT('Ctrl Pts',(-49.531790370394,18.0912355578117,-171.396105918926));
#150009=CARTESIAN_POINT('Ctrl Pts',(-49.7384998091177,18.76999998,-170.950084676266));
#150010=CARTESIAN_POINT('Ctrl Pts',(-49.1426233976849,18.76999998,-171.475106253347));
#150011=CARTESIAN_POINT('Ctrl Pts',(-49.3972764264867,18.0557138798866,
-171.250219392074));
#150012=CARTESIAN_POINT('Ctrl Pts',(-49.7050206304183,18.76999998,-170.908176521547));
#150013=CARTESIAN_POINT('Ctrl Pts',(-49.0312290116693,18.7699999799994,
-171.386219492649));
#150014=CARTESIAN_POINT('Ctrl Pts',(-49.3398639704239,18.040521010502,-171.166400641829));
#150015=CARTESIAN_POINT('Ctrl Pts',(-49.6791770659623,18.76999998,-170.861259130871));
#150016=CARTESIAN_POINT('Ctrl Pts',(-48.9379852680023,18.76999998,-171.26952948831));
#150017=CARTESIAN_POINT('Ctrl Pts',(-49.2955572616308,18.0287857662076,
-171.07256826174));
#150018=CARTESIAN_POINT('',(-50.2136602208993,18.26999998,-171.64995));
#150019=CARTESIAN_POINT('Origin',(-50.2136602208993,18.26999998,-171.14995));
#150020=CARTESIAN_POINT('Ctrl Pts',(-50.2136602208993,18.26999998,-171.64995));
#150021=CARTESIAN_POINT('Ctrl Pts',(-50.1215225801538,18.2459873673078,
-171.64995));
#150022=CARTESIAN_POINT('Ctrl Pts',(-50.0313889586563,18.2224389306129,
-171.637773119416));
#150023=CARTESIAN_POINT('Ctrl Pts',(-49.8551127360827,18.1762799424075,
-171.589596446108));
#150024=CARTESIAN_POINT('Ctrl Pts',(-49.7676788911518,18.1533289077801,
-171.552696670458));
#150025=CARTESIAN_POINT('Ctrl Pts',(-49.6063178327574,18.1108845812496,
-171.455768650908));
#150026=CARTESIAN_POINT('Ctrl Pts',(-49.531790370394,18.0912355578117,-171.396105918926));
#150027=CARTESIAN_POINT('Ctrl Pts',(-49.3972764264867,18.0557138798866,
-171.250219392074));
#150028=CARTESIAN_POINT('Ctrl Pts',(-49.3398639704239,18.040521010502,-171.166400641829));
#150029=CARTESIAN_POINT('Ctrl Pts',(-49.2955572616308,18.0287857662077,
-171.07256826174));
#150030=CARTESIAN_POINT('Origin',(-1.30574517062348E-14,18.26999998,-171.14995));
#150031=CARTESIAN_POINT('',(-50.8071048221096,18.26999998,-171.64995));
#150032=CARTESIAN_POINT('Origin',(-50.8071048221096,18.26999998,-171.14995));
#150033=CARTESIAN_POINT('',(-49.8991400004038,18.26999998,-171.64995));
#150034=CARTESIAN_POINT('Ctrl Pts',(-50.8071048221096,18.26999998,-171.64995));
#150035=CARTESIAN_POINT('Ctrl Pts',(-50.8071048221095,18.76999998,-171.64995));
#150036=CARTESIAN_POINT('Ctrl Pts',(-50.8071048221096,18.76999998,-171.14995));
#150037=CARTESIAN_POINT('Ctrl Pts',(-50.9405951656344,18.2608894800009,
-171.64995));
#150038=CARTESIAN_POINT('Ctrl Pts',(-50.9418867684204,18.76999998,-171.659148653595));
#150039=CARTESIAN_POINT('Ctrl Pts',(-51.0054197414846,18.76999998,-171.149950000016));
#150040=CARTESIAN_POINT('Ctrl Pts',(-51.0739848911322,18.2517858470187,
-171.675977326981));
#150041=CARTESIAN_POINT('Ctrl Pts',(-51.0712775866753,18.7699999800004,
-171.69520402023));
#150042=CARTESIAN_POINT('Ctrl Pts',(-51.2035851814656,18.76999998,-171.18899099047));
#150043=CARTESIAN_POINT('Ctrl Pts',(-51.3205984142243,18.2349548730131,
-171.776163607997));
#150044=CARTESIAN_POINT('Ctrl Pts',(-51.3040563824941,18.7699999799997,
-171.809929875206));
#150045=CARTESIAN_POINT('Ctrl Pts',(-51.5699573073986,18.76999998,-171.339270411997));
#150046=CARTESIAN_POINT('Ctrl Pts',(-51.43370116591,18.227235793176,-171.850283164393));
#150047=CARTESIAN_POINT('Ctrl Pts',(-51.406631095234,18.7699999800021,-171.888983273332));
#150048=CARTESIAN_POINT('Ctrl Pts',(-51.7379841660413,18.76999998,-171.450449746589));
#150049=CARTESIAN_POINT('Ctrl Pts',(-51.6224509847807,18.2143539233764,
-172.035403273234));
#150050=CARTESIAN_POINT('Ctrl Pts',(-51.5742878663865,18.769999979998,-172.075215659168));
#150051=CARTESIAN_POINT('Ctrl Pts',(-52.0183932512491,18.76999998,-171.728129909852));
#150052=CARTESIAN_POINT('Ctrl Pts',(-51.6980238274146,18.2091961991206,
-172.14633102856));
#150053=CARTESIAN_POINT('Ctrl Pts',(-51.6385589321982,18.76999998,-172.182182441318));
#150054=CARTESIAN_POINT('Ctrl Pts',(-52.1306652088914,18.76999998,-171.894521542842));
#150055=CARTESIAN_POINT('Ctrl Pts',(-51.8001744932412,18.2022245814263,
-172.38820210671));
#150056=CARTESIAN_POINT('Ctrl Pts',(-51.7249922616163,18.76999998,-172.409726298163));
#150057=CARTESIAN_POINT('Ctrl Pts',(-52.2824215121743,18.76999998,-172.257328160063));
#150058=CARTESIAN_POINT('Ctrl Pts',(-51.8267121465163,18.2004134295229,
-172.51902671195));
#150059=CARTESIAN_POINT('Ctrl Pts',(-51.746661977275,18.769999979999,-172.529650273729));
#150060=CARTESIAN_POINT('Ctrl Pts',(-52.3218461808705,18.76999998,-172.453565067926));
#150061=CARTESIAN_POINT('Ctrl Pts',(-51.8267121465167,18.20041342952,-172.64995));
#150062=CARTESIAN_POINT('Ctrl Pts',(-51.746661977277,18.76999998,-172.64995));
#150063=CARTESIAN_POINT('Ctrl Pts',(-52.3218461808875,18.76999998,-172.64995));
#150064=CARTESIAN_POINT('Origin',(-52.3218461808875,18.26999998,-172.64995));
#150065=CARTESIAN_POINT('Ctrl Pts',(-51.8267121465167,18.20041342952,-172.64995));
#150066=CARTESIAN_POINT('Ctrl Pts',(-51.8267121465163,18.2004134295229,
-172.51902671195));
#150067=CARTESIAN_POINT('Ctrl Pts',(-51.8001744932412,18.2022245814263,
-172.38820210671));
#150068=CARTESIAN_POINT('Ctrl Pts',(-51.6980238274146,18.2091961991206,
-172.14633102856));
#150069=CARTESIAN_POINT('Ctrl Pts',(-51.6224509847807,18.2143539233764,
-172.035403273234));
#150070=CARTESIAN_POINT('Ctrl Pts',(-51.43370116591,18.227235793176,-171.850283164393));
#150071=CARTESIAN_POINT('Ctrl Pts',(-51.3205984142243,18.2349548730131,
-171.776163607997));
#150072=CARTESIAN_POINT('Ctrl Pts',(-51.0739848911322,18.2517858470187,
-171.675977326981));
#150073=CARTESIAN_POINT('Ctrl Pts',(-50.9405951656344,18.2608894800009,
-171.64995));
#150074=CARTESIAN_POINT('Ctrl Pts',(-50.8071048221096,18.26999998,-171.64995));
#150075=CARTESIAN_POINT('Origin',(-52.3218461808875,18.26999998,-171.64995));
#150076=CARTESIAN_POINT('Origin',(-52.3218461808875,18.26999998,-176.84995));
#150077=CARTESIAN_POINT('Origin',(83.2809572255632,19.26999998,-176.84995));
#150078=CARTESIAN_POINT('',(-57.,19.26999998,-177.34995));
#150079=CARTESIAN_POINT('Origin',(-57.,19.26999998,-176.84995));
#150080=CARTESIAN_POINT('',(-52.1813053461851,19.26999998,-177.34995));
#150081=CARTESIAN_POINT('',(-60.,19.26999998,-177.34995));
#150082=CARTESIAN_POINT('Ctrl Pts',(-52.3218461808875,18.76999998,-176.84995));
#150083=CARTESIAN_POINT('Ctrl Pts',(-52.3218461808802,18.76999998,-176.981217345763));
#150084=CARTESIAN_POINT('Ctrl Pts',(-52.3066996556685,18.8238865434699,
-177.110943344657));
#150085=CARTESIAN_POINT('Ctrl Pts',(-52.2546657912052,19.0090066353435,
-177.29606343653));
#150086=CARTESIAN_POINT('Ctrl Pts',(-52.2182021908711,19.1387326342368,
-177.34995));
#150087=CARTESIAN_POINT('Ctrl Pts',(-52.1813053461851,19.26999998,-177.34995));
#150088=CARTESIAN_POINT('Origin',(-57.,19.26999998,-174.34995));
#150089=CARTESIAN_POINT('',(-60.,19.26999998,-174.34995));
#150090=CARTESIAN_POINT('Origin',(-59.5,19.26999998,-174.34995));
#150091=CARTESIAN_POINT('Origin',(-57.,19.26999998,-174.34995));
#150092=CARTESIAN_POINT('Origin',(-59.5,19.26999998,-55.24995));
#150093=CARTESIAN_POINT('',(-60.,19.26999998,-58.24995));
#150094=CARTESIAN_POINT('Origin',(-59.5,19.26999998,-58.24995));
#150095=CARTESIAN_POINT('',(-60.,19.26999998,-174.34995));
#150096=CARTESIAN_POINT('Origin',(-57.,19.26999998,-58.24995));
#150097=CARTESIAN_POINT('Origin',(-57.,19.26999998,-58.24995));
#150098=CARTESIAN_POINT('Origin',(-57.,-2.42462934179819E-14,-58.24995));
#150099=CARTESIAN_POINT('',(-60.,19.76999998,-58.24995));
#150100=CARTESIAN_POINT('Origin',(-57.,19.76999998,-58.24995));
#150101=CARTESIAN_POINT('',(-60.,-54.58000002,-58.24995));
#150102=CARTESIAN_POINT('Origin',(-57.,19.76999998,-58.24995));
#150103=CARTESIAN_POINT('Origin',(-59.5,19.76999998,-58.24995));
#150104=CARTESIAN_POINT('Origin',(-60.,19.76999998,-176.84995));
#150105=CARTESIAN_POINT('',(-52.1110349288339,19.76999998,-177.34995));
#150106=CARTESIAN_POINT('',(-57.,19.76999998,-177.34995));
#150107=CARTESIAN_POINT('',(-60.,19.76999998,-177.34995));
#150108=CARTESIAN_POINT('Origin',(-57.,19.76999998,-176.84995));
#150109=CARTESIAN_POINT('Ctrl Pts',(-52.1110349288339,19.76999998,-177.34995));
#150110=CARTESIAN_POINT('Ctrl Pts',(-52.0741380841476,19.9012673257632,
-177.34995));
#150111=CARTESIAN_POINT('Ctrl Pts',(-52.0376744838139,20.0309933246565,
-177.29606343653));
#150112=CARTESIAN_POINT('Ctrl Pts',(-51.9856406193506,20.2161134165301,
-177.110943344657));
#150113=CARTESIAN_POINT('Ctrl Pts',(-51.9704940941388,20.26999998,-176.981217345763));
#150114=CARTESIAN_POINT('Ctrl Pts',(-51.9704940941315,20.26999998,-176.84995));
#150115=CARTESIAN_POINT('Origin',(-51.9704940941315,20.76999998,-171.64995));
#150116=CARTESIAN_POINT('Origin',(-51.9704940941315,20.76999998,-176.84995));
#150117=CARTESIAN_POINT('Origin',(-51.9704940941315,20.76999998,-172.64995));
#150118=CARTESIAN_POINT('Ctrl Pts',(-51.4753600597607,20.70041342952,-172.64995));
#150119=CARTESIAN_POINT('Ctrl Pts',(-51.5358507252234,20.26999998,-172.64995));
#150120=CARTESIAN_POINT('Ctrl Pts',(-51.9704940941315,20.26999998,-172.64995));
#150121=CARTESIAN_POINT('Ctrl Pts',(-51.4753600597603,20.7004134295229,
-172.51902671195));
#150122=CARTESIAN_POINT('Ctrl Pts',(-51.5358507252071,20.26999998,-172.511015867074));
#150123=CARTESIAN_POINT('Ctrl Pts',(-51.9704940941145,20.26999998,-172.453565067926));
#150124=CARTESIAN_POINT('Ctrl Pts',(-51.4488224064852,20.7022245814263,
-172.38820210671));
#150125=CARTESIAN_POINT('Ctrl Pts',(-51.5060950400989,20.26999998,-172.371853931892));
#150126=CARTESIAN_POINT('Ctrl Pts',(-51.9310694254183,20.26999998,-172.257328160063));
#150127=CARTESIAN_POINT('Ctrl Pts',(-51.3466717406587,20.7091961991206,
-172.14633102856));
#150128=CARTESIAN_POINT('Ctrl Pts',(-51.3932840309667,20.26999998,-172.118296873734));
#150129=CARTESIAN_POINT('Ctrl Pts',(-51.7793131221354,20.26999998,-171.894521542842));
#150130=CARTESIAN_POINT('Ctrl Pts',(-51.2710988980251,20.7143539233764,
-172.035403273235));
#150131=CARTESIAN_POINT('Ctrl Pts',(-51.3097149387001,20.2699999800017,
-172.003556970023));
#150132=CARTESIAN_POINT('Ctrl Pts',(-51.6670411644938,20.26999998,-171.728129909852));
#150133=CARTESIAN_POINT('Ctrl Pts',(-51.0823490791536,20.727235793176,-171.850283164392));
#150134=CARTESIAN_POINT('Ctrl Pts',(-51.105269719327,20.2699999799983,-171.817687494207));
#150135=CARTESIAN_POINT('Ctrl Pts',(-51.3866320792846,20.26999998,-171.450449746589));
#150136=CARTESIAN_POINT('Ctrl Pts',(-50.9692463274684,20.7349548730131,
-171.776163607997));
#150137=CARTESIAN_POINT('Ctrl Pts',(-50.9837060031699,20.26999998,-171.746711574348));
#150138=CARTESIAN_POINT('Ctrl Pts',(-51.2186052206426,20.26999998,-171.339270411997));
#150139=CARTESIAN_POINT('Ctrl Pts',(-50.7226328043762,20.7517858470187,
-171.675977326981));
#150140=CARTESIAN_POINT('Ctrl Pts',(-50.725270742269,20.26999998,-171.658003579003));
#150141=CARTESIAN_POINT('Ctrl Pts',(-50.8522330947096,20.26999998,-171.18899099047));
#150142=CARTESIAN_POINT('Ctrl Pts',(-50.5892430788785,20.760889480001,-171.64995));
#150143=CARTESIAN_POINT('Ctrl Pts',(-50.5880011641168,20.26999998,-171.640924254979));
#150144=CARTESIAN_POINT('Ctrl Pts',(-50.6540676547286,20.26999998,-171.149950000016));
#150145=CARTESIAN_POINT('Ctrl Pts',(-50.4557527353536,20.76999998,-171.64995));
#150146=CARTESIAN_POINT('Ctrl Pts',(-50.4557527353535,20.26999998,-171.64995));
#150147=CARTESIAN_POINT('Ctrl Pts',(-50.4557527353536,20.26999998,-171.14995));
#150148=CARTESIAN_POINT('',(-50.4557527353536,20.76999998,-171.64995));
#150149=CARTESIAN_POINT('Origin',(-50.4557527353536,20.76999998,-171.14995));
#150150=CARTESIAN_POINT('Ctrl Pts',(-50.4557527353536,20.76999998,-171.64995));
#150151=CARTESIAN_POINT('Ctrl Pts',(-50.5892430788785,20.760889480001,-171.64995));
#150152=CARTESIAN_POINT('Ctrl Pts',(-50.7226328043762,20.7517858470187,
-171.675977326981));
#150153=CARTESIAN_POINT('Ctrl Pts',(-50.9692463274684,20.7349548730131,
-171.776163607997));
#150154=CARTESIAN_POINT('Ctrl Pts',(-51.0823490791536,20.727235793176,-171.850283164392));
#150155=CARTESIAN_POINT('Ctrl Pts',(-51.2710988980251,20.7143539233764,
-172.035403273235));
#150156=CARTESIAN_POINT('Ctrl Pts',(-51.3466717406587,20.7091961991206,
-172.14633102856));
#150157=CARTESIAN_POINT('Ctrl Pts',(-51.4488224064852,20.7022245814263,
-172.38820210671));
#150158=CARTESIAN_POINT('Ctrl Pts',(-51.4753600597603,20.7004134295229,
-172.51902671195));
#150159=CARTESIAN_POINT('Ctrl Pts',(-51.4753600597607,20.70041342952,-172.64995));
#150160=CARTESIAN_POINT('Origin',(-1.41024658483895E-14,20.76999998,-171.14995));
#150161=CARTESIAN_POINT('',(-48.5692718988023,20.76999998,-171.64995));
#150162=CARTESIAN_POINT('Origin',(-48.5692718988023,20.76999998,-171.14995));
#150163=CARTESIAN_POINT('',(-50.5260231527048,20.76999998,-171.64995));
#150164=CARTESIAN_POINT('Ctrl Pts',(-48.0164881467928,20.26999998,-170.861259130871));
#150165=CARTESIAN_POINT('Ctrl Pts',(-47.7727200234913,20.26999998,-171.000183411942));
#150166=CARTESIAN_POINT('Ctrl Pts',(-47.6457075325507,20.5094809071607,
-171.07256826174));
#150167=CARTESIAN_POINT('Ctrl Pts',(-48.0706057955098,20.26999998,-170.956218123485));
#150168=CARTESIAN_POINT('Ctrl Pts',(-47.8434294594086,20.2699999800004,
-171.164785257117));
#150169=CARTESIAN_POINT('Ctrl Pts',(-47.7359101824116,20.5351319377708,
-171.262470025419));
#150170=CARTESIAN_POINT('Ctrl Pts',(-48.1562174294056,20.26999998,-171.029346177368));
#150171=CARTESIAN_POINT('Ctrl Pts',(-47.9584699210001,20.26999998,-171.302270428196));
#150172=CARTESIAN_POINT('Ctrl Pts',(-47.8786973574541,20.5756668312168,
-171.408742372302));
#150173=CARTESIAN_POINT('Ctrl Pts',(-48.3512215443805,20.26999998,-171.126070092674));
#150174=CARTESIAN_POINT('Ctrl Pts',(-48.2313965321131,20.26999998,-171.520661616426));
#150175=CARTESIAN_POINT('Ctrl Pts',(-48.2043974294738,20.6676448702122,
-171.602190167782));
#150176=CARTESIAN_POINT('Ctrl Pts',(-48.4599658479004,20.26999998,-171.149949989306));
#150177=CARTESIAN_POINT('Ctrl Pts',(-48.3952116684766,20.26999998,-171.601246355348));
#150178=CARTESIAN_POINT('Ctrl Pts',(-48.3862309601951,20.7187835557883,
-171.64995));
#150179=CARTESIAN_POINT('Ctrl Pts',(-48.5692718988023,20.26999998,-171.14995));
#150180=CARTESIAN_POINT('Ctrl Pts',(-48.5692718988023,20.26999998,-171.64995));
#150181=CARTESIAN_POINT('Ctrl Pts',(-48.5692718988023,20.76999998,-171.64995));
#150182=CARTESIAN_POINT('',(-47.6457075325507,20.5094809071607,-171.07256826174));
#150183=CARTESIAN_POINT('Origin',(-48.0164881467928,20.76999998,-170.861259130871));
#150184=CARTESIAN_POINT('Ctrl Pts',(-47.6457075325507,20.5094809071607,
-171.07256826174));
#150185=CARTESIAN_POINT('Ctrl Pts',(-47.7359101824116,20.5351319377708,
-171.262470025419));
#150186=CARTESIAN_POINT('Ctrl Pts',(-47.8786973574541,20.5756668312168,
-171.408742372302));
#150187=CARTESIAN_POINT('Ctrl Pts',(-48.2043974294738,20.6676448702122,
-171.602190167782));
#150188=CARTESIAN_POINT('Ctrl Pts',(-48.3862309601951,20.7187835557883,
-171.64995));
#150189=CARTESIAN_POINT('Ctrl Pts',(-48.5692718988023,20.76999998,-171.64995));
#150190=CARTESIAN_POINT('Ctrl Pts',(-47.6457075325507,20.5094809071607,
-171.07256826174));
#150191=CARTESIAN_POINT('Ctrl Pts',(-47.7727200234913,20.26999998,-171.000183411942));
#150192=CARTESIAN_POINT('Ctrl Pts',(-48.0164881467928,20.26999998,-170.861259130871));
#150193=CARTESIAN_POINT('Ctrl Pts',(-45.3135333962397,20.5009878795767,
-166.96987023406));
#150194=CARTESIAN_POINT('Ctrl Pts',(-45.4541703457615,20.2699999799837,
-166.918724083766));
#150195=CARTESIAN_POINT('Ctrl Pts',(-45.6783453674058,20.26999998,-166.758558919217));
#150196=CARTESIAN_POINT('Ctrl Pts',(-42.941059217223,20.4917195215043,-162.891251079751));
#150197=CARTESIAN_POINT('Ctrl Pts',(-43.0850828436089,20.26999998,-162.842145218595));
#150198=CARTESIAN_POINT('Ctrl Pts',(-43.2989471172158,20.26999998,-162.679937821406));
#150199=CARTESIAN_POINT('Ctrl Pts',(-40.5058324224685,20.4814581622113,
-158.850394545248));
#150200=CARTESIAN_POINT('Ctrl Pts',(-40.6336903802499,20.26999998,-158.773072684364));
#150201=CARTESIAN_POINT('Ctrl Pts',(-40.8552491802207,20.26999998,-158.639085414378));
#150202=CARTESIAN_POINT('',(-40.5058112296754,20.4818276543828,-158.850123897688));
#150203=CARTESIAN_POINT('Origin',(-40.8552491802207,20.76999998,-158.639085414378));
#150204=CARTESIAN_POINT('Ctrl Pts',(-40.5058324224782,20.4814581622043,
-158.850394545254));
#150205=CARTESIAN_POINT('Ctrl Pts',(-42.941059217223,20.4917195215043,-162.891251079751));
#150206=CARTESIAN_POINT('Ctrl Pts',(-45.3135333962397,20.5009878795767,
-166.96987023406));
#150207=CARTESIAN_POINT('Ctrl Pts',(-47.6457075325507,20.5094809071607,
-171.07256826174));
#150208=CARTESIAN_POINT('Ctrl Pts',(-39.5009242507648,20.26999998,-153.115786956963));
#150209=CARTESIAN_POINT('Ctrl Pts',(-38.9925815845935,20.2699999799997,
-153.109400650742));
#150210=CARTESIAN_POINT('Ctrl Pts',(-39.0010287272926,20.7783180048152,
-153.109486542985));
#150211=CARTESIAN_POINT('Ctrl Pts',(-39.4889697665367,20.26999998,-154.10717684131));
#150212=CARTESIAN_POINT('Ctrl Pts',(-39.0319940367927,20.2699999800017,
-154.089975297154));
#150213=CARTESIAN_POINT('Ctrl Pts',(-38.9877342686064,20.7251370715181,
-154.141750666168));
#150214=CARTESIAN_POINT('Ctrl Pts',(-39.5928133816968,20.26999998,-155.082459683401));
#150215=CARTESIAN_POINT('Ctrl Pts',(-39.1755337328108,20.26999998,-155.105670642999));
#150216=CARTESIAN_POINT('Ctrl Pts',(-39.1031090110774,20.6727392618587,
-155.156196882157));
#150217=CARTESIAN_POINT('Ctrl Pts',(-39.9310881578732,20.26999998,-156.493265246185));
#150218=CARTESIAN_POINT('Ctrl Pts',(-39.5936268082786,20.26999998,-156.580999082022));
#150219=CARTESIAN_POINT('Ctrl Pts',(-39.4789583459802,20.5969029691765,
-156.622397172782));
#150220=CARTESIAN_POINT('Ctrl Pts',(-40.0698006899404,20.26999998,-156.944576655439));
#150221=CARTESIAN_POINT('Ctrl Pts',(-39.7542561576979,20.26999998,-157.042684697946));
#150222=CARTESIAN_POINT('Ctrl Pts',(-39.6330812307821,20.5726365813876,
-157.091232676227));
#150223=CARTESIAN_POINT('Ctrl Pts',(-40.4284839815743,20.26999998,-157.861855948356));
#150224=CARTESIAN_POINT('Ctrl Pts',(-40.1598249794629,20.26999998,-157.975302673127));
#150225=CARTESIAN_POINT('Ctrl Pts',(-40.0316153142837,20.5233115816645,
-158.043776827648));
#150226=CARTESIAN_POINT('Ctrl Pts',(-40.6556223798764,20.26999998,-158.327340856604));
#150227=CARTESIAN_POINT('Ctrl Pts',(-40.4110126646261,20.26999998,-158.450056605571));
#150228=CARTESIAN_POINT('Ctrl Pts',(-40.2840071293548,20.4982773543068,
-158.526971120527));
#150229=CARTESIAN_POINT('Ctrl Pts',(-40.9360042062312,20.26999998,-158.769481550799));
#150230=CARTESIAN_POINT('Ctrl Pts',(-40.7219957046872,20.26999998,-158.905394499841));
#150231=CARTESIAN_POINT('Ctrl Pts',(-40.5955208521275,20.4745034644437,
-158.985715203387));
#150232=CARTESIAN_POINT('',(-39.,20.76999998,-153.26884421004));
#150233=CARTESIAN_POINT('Origin',(-39.5,20.76999998,-153.26884421004));
#150234=CARTESIAN_POINT('Ctrl Pts',(-39.,20.76999998,-153.26884421004));
#150235=CARTESIAN_POINT('Ctrl Pts',(-39.0000000113268,20.7612499005546,
-153.438661222045));
#150236=CARTESIAN_POINT('Ctrl Pts',(-39.0036425975434,20.7525133314444,
-153.607997478032));
#150237=CARTESIAN_POINT('Ctrl Pts',(-39.0108614735808,20.7438083498483,
-153.776830647326));
#150238=CARTESIAN_POINT('Ctrl Pts',(-39.0181154374938,20.7350610570518,
-153.946484442602));
#150239=CARTESIAN_POINT('Ctrl Pts',(-39.0289800693621,20.7263449029416,
-154.115630850492));
#150240=CARTESIAN_POINT('Ctrl Pts',(-39.0434339731224,20.7176579343566,
-154.284262690438));
#150241=CARTESIAN_POINT('Ctrl Pts',(-39.0578177633858,20.7090131048196,
-154.452076525214));
#150242=CARTESIAN_POINT('Ctrl Pts',(-39.0757558973881,20.7003963326059,
-154.619381424156));
#150243=CARTESIAN_POINT('Ctrl Pts',(-39.0972774424432,20.6917977102686,
-154.786176160187));
#150244=CARTESIAN_POINT('Ctrl Pts',(-39.118556656787,20.6832959076654,-154.951092802107));
#150245=CARTESIAN_POINT('Ctrl Pts',(-39.1433391102861,20.6748110028389,
-155.115511340156));
#150246=CARTESIAN_POINT('Ctrl Pts',(-39.1717028274331,20.6663381714659,
-155.279426755488));
#150247=CARTESIAN_POINT('Ctrl Pts',(-39.1993404733963,20.6580822326346,
-155.439146167206));
#150248=CARTESIAN_POINT('Ctrl Pts',(-39.2303787405759,20.6498370259114,
-155.598388419814));
#150249=CARTESIAN_POINT('Ctrl Pts',(-39.2649340810352,20.6416141318001,
-155.757136681022));
#150250=CARTESIAN_POINT('Ctrl Pts',(-39.2935660208686,20.6348007881512,
-155.888672663684));
#150251=CARTESIAN_POINT('Ctrl Pts',(-39.3246135032229,20.6280028352214,
-156.019869432432));
#150252=CARTESIAN_POINT('Ctrl Pts',(-39.3581636245473,20.621240911696,-156.150706929915));
#150253=CARTESIAN_POINT('Ctrl Pts',(-39.3991815569979,20.6129738738596,
-156.31066711551));
#150254=CARTESIAN_POINT('Ctrl Pts',(-39.4439970735942,20.6047446721664,
-156.470288588488));
#150255=CARTESIAN_POINT('Ctrl Pts',(-39.4927105570457,20.5965487965378,
-156.629036157844));
#150256=CARTESIAN_POINT('Ctrl Pts',(-39.5402989256382,20.5885422176049,
-156.784117201293));
#150257=CARTESIAN_POINT('Ctrl Pts',(-39.5916077486878,20.5805677027968,
-156.938364068926));
#150258=CARTESIAN_POINT('Ctrl Pts',(-39.6466989484637,20.572653205052,-157.091258703666));
#150259=CARTESIAN_POINT('Ctrl Pts',(-39.7014925828694,20.5647814560667,
-157.243327505083));
#150260=CARTESIAN_POINT('Ctrl Pts',(-39.760028377299,20.5569693454962,-157.394058454827));
#150261=CARTESIAN_POINT('Ctrl Pts',(-39.8223280030638,20.5492728001288,
-157.542925319488));
#150262=CARTESIAN_POINT('Ctrl Pts',(-39.8698220890173,20.5434053429372,
-157.656413893121));
#150263=CARTESIAN_POINT('Ctrl Pts',(-39.9195353179802,20.5376387400302,
-157.768959999866));
#150264=CARTESIAN_POINT('Ctrl Pts',(-39.9716295140578,20.531917355076,-157.880527437696));
#150265=CARTESIAN_POINT('Ctrl Pts',(-40.0229635294114,20.5262794590109,
-157.990466835897));
#150266=CARTESIAN_POINT('Ctrl Pts',(-40.0766101067617,20.52068517217,-158.099456116636));
#150267=CARTESIAN_POINT('Ctrl Pts',(-40.1327424435931,20.515118298375,-158.207433310574));
#150268=CARTESIAN_POINT('Ctrl Pts',(-40.189569989177,20.5094824778801,-158.316747820836));
#150269=CARTESIAN_POINT('Ctrl Pts',(-40.2489458840389,20.5038743074662,
-158.42502532234));
#150270=CARTESIAN_POINT('Ctrl Pts',(-40.3110598226681,20.4983210960923,
-158.532169335452));
#150271=CARTESIAN_POINT('Ctrl Pts',(-40.3731737612972,20.4927678847185,
-158.639313348565));
#150272=CARTESIAN_POINT('Ctrl Pts',(-40.4380265406518,20.48726933986,-158.745324062406));
#150273=CARTESIAN_POINT('Ctrl Pts',(-40.5058069606272,20.4819020842353,
-158.850069378908));
#150274=CARTESIAN_POINT('Origin',(-39.5,20.76999998,-55.24995));
#150275=CARTESIAN_POINT('',(-39.,20.769999979994,-78.7897987614735));
#150276=CARTESIAN_POINT('Origin',(-39.5,20.76999998,-78.7897987614789));
#150277=CARTESIAN_POINT('',(-39.,20.76999998,-129.34995));
#150278=CARTESIAN_POINT('Ctrl Pts',(-40.9018414229103,20.26999998,-73.3435694268454));
#150279=CARTESIAN_POINT('Ctrl Pts',(-40.684666116315,20.26999998,-73.2084555874168));
#150280=CARTESIAN_POINT('Ctrl Pts',(-40.5575787214805,20.4774056435493,
-73.1293894159588));
#150281=CARTESIAN_POINT('Ctrl Pts',(-40.6368001443165,20.26999998,-73.7699218893582));
#150282=CARTESIAN_POINT('Ctrl Pts',(-40.390530128252,20.26999998,-73.6473693843928));
#150283=CARTESIAN_POINT('Ctrl Pts',(-40.2631070795345,20.5003287096446,
-73.5717684720406));
#150284=CARTESIAN_POINT('Ctrl Pts',(-40.4211667416632,20.26999998,-74.2159715169244));
#150285=CARTESIAN_POINT('Ctrl Pts',(-40.151872039737,20.26999998,-74.1021113025596));
#150286=CARTESIAN_POINT('Ctrl Pts',(-40.0234990701502,20.5243153760975,
-74.0347965829616));
#150287=CARTESIAN_POINT('Ctrl Pts',(-40.0717001001047,20.26999998,-75.1087680536759));
#150288=CARTESIAN_POINT('Ctrl Pts',(-39.7564818699868,20.26999998,-75.0104879262006));
#150289=CARTESIAN_POINT('Ctrl Pts',(-39.6352044867726,20.5723197033564,
-74.9619127222182));
#150290=CARTESIAN_POINT('Ctrl Pts',(-39.9341806290214,20.26999998,-75.5541367565536));
#150291=CARTESIAN_POINT('Ctrl Pts',(-39.5972778875,20.26999998,-75.4662534410499));
#150292=CARTESIAN_POINT('Ctrl Pts',(-39.4824063073862,20.5962647124333,
-75.4245702559575));
#150293=CARTESIAN_POINT('Ctrl Pts',(-39.5978219804271,20.26999998,-76.9519251307675));
#150294=CARTESIAN_POINT('Ctrl Pts',(-39.1821433177468,20.26999998,-76.9267633860652));
#150295=CARTESIAN_POINT('Ctrl Pts',(-39.1086810672092,20.6713961121791,
-76.8772353049354));
#150296=CARTESIAN_POINT('Ctrl Pts',(-39.4934964889571,20.26999998,-77.9105369836536));
#150297=CARTESIAN_POINT('Ctrl Pts',(-39.0385195691145,20.26999998,-77.9239546370935));
#150298=CARTESIAN_POINT('Ctrl Pts',(-38.9927679036048,20.7228955117014,
-77.8743245155055));
#150299=CARTESIAN_POINT('Ctrl Pts',(-39.500313254109,20.26999998,-78.8787081544503));
#150300=CARTESIAN_POINT('Ctrl Pts',(-38.9954730195525,20.26999998,-78.8823876098162));
#150301=CARTESIAN_POINT('Ctrl Pts',(-39.0003486606699,20.7748318783165,
-78.8823661670891));
#150302=CARTESIAN_POINT('',(-40.5058117853578,20.4818179386473,-73.2085119571815));
#150303=CARTESIAN_POINT('Origin',(-40.8552491802306,20.76999998,-73.4195575571114));
#150304=CARTESIAN_POINT('Ctrl Pts',(-40.505806959117,20.4819020767265,-73.2085735870852));
#150305=CARTESIAN_POINT('Ctrl Pts',(-40.4421126804931,20.4869458048838,
-73.3070042835559));
#150306=CARTESIAN_POINT('Ctrl Pts',(-40.3810512373412,20.4921043295325,
-73.4064758506061));
#150307=CARTESIAN_POINT('Ctrl Pts',(-40.3224551183704,20.497309951475,-73.5068769259294));
#150308=CARTESIAN_POINT('Ctrl Pts',(-40.2622487774598,20.502658623961,-73.6100370238146));
#150309=CARTESIAN_POINT('Ctrl Pts',(-40.2046444490715,20.5080570688536,
-73.7141784357249));
#150310=CARTESIAN_POINT('Ctrl Pts',(-40.1494592619306,20.5134764228891,
-73.819212537194));
#150311=CARTESIAN_POINT('Ctrl Pts',(-40.0934408446496,20.518977602671,-73.9258325276237));
#150312=CARTESIAN_POINT('Ctrl Pts',(-40.0399145313078,20.5245005572052,
-74.0333725142232));
#150313=CARTESIAN_POINT('Ctrl Pts',(-39.9886979257668,20.5300581159715,
-74.1417711463612));
#150314=CARTESIAN_POINT('Ctrl Pts',(-39.9364977330605,20.5357224046435,
-74.2522515155093));
#150315=CARTESIAN_POINT('Ctrl Pts',(-39.8866961963328,20.5414229208258,
-74.3636240099572));
#150316=CARTESIAN_POINT('Ctrl Pts',(-39.8391190270575,20.5472137255442,
-74.4758535022212));
#150317=CARTESIAN_POINT('Ctrl Pts',(-39.8339320212271,20.5478450564598,
-74.4880890984027));
#150318=CARTESIAN_POINT('Ctrl Pts',(-39.8287714776101,20.5484774968517,
-74.5003349078318));
#150319=CARTESIAN_POINT('Ctrl Pts',(-39.823637188238,20.5491111427775,-74.5125909043337));
#150320=CARTESIAN_POINT('Ctrl Pts',(-39.7672426362845,20.5560710500776,
-74.6472096181163));
#150321=CARTESIAN_POINT('Ctrl Pts',(-39.714047999184,20.5631207512728,-74.7830391075794));
#150322=CARTESIAN_POINT('Ctrl Pts',(-39.663900248601,20.5702172270692,-74.9200044351338));
#150323=CARTESIAN_POINT('Ctrl Pts',(-39.6129146480068,20.5774322681504,
-75.0592581285652));
#150324=CARTESIAN_POINT('Ctrl Pts',(-39.5650778944283,20.5846961163451,
-75.1996862413939));
#150325=CARTESIAN_POINT('Ctrl Pts',(-39.5202529103467,20.592002925974,-75.341239035909));
#150326=CARTESIAN_POINT('Ctrl Pts',(-39.4745072702815,20.5994598094544,
-75.485699169488));
#150327=CARTESIAN_POINT('Ctrl Pts',(-39.4318977457585,20.6069619918687,
-75.6313310442599));
#150328=CARTESIAN_POINT('Ctrl Pts',(-39.3923135370132,20.6145361975083,
-75.7781064604276));
#150329=CARTESIAN_POINT('Ctrl Pts',(-39.3814836461544,20.6166084334584,
-75.818262921507));
#150330=CARTESIAN_POINT('Ctrl Pts',(-39.3708804344681,20.618686219437,-75.8585050995266));
#150331=CARTESIAN_POINT('Ctrl Pts',(-39.3605021656695,20.6207704310745,
-75.8988326670837));
#150332=CARTESIAN_POINT('Ctrl Pts',(-39.3193535035498,20.6290340945156,
-76.0587269118477));
#150333=CARTESIAN_POINT('Ctrl Pts',(-39.2819485474107,20.6373550060547,
-76.219143860454));
#150334=CARTESIAN_POINT('Ctrl Pts',(-39.2481348789061,20.6456934458296,
-76.3800221605525));
#150335=CARTESIAN_POINT('Ctrl Pts',(-39.2135346702094,20.6542258461628,
-76.5446426529261));
#150336=CARTESIAN_POINT('Ctrl Pts',(-39.1826942310796,20.662777321259,-76.7097467270594));
#150337=CARTESIAN_POINT('Ctrl Pts',(-39.1554910444983,20.6713348080893,
-76.8752903404046));
#150338=CARTESIAN_POINT('Ctrl Pts',(-39.1275435484723,20.6801264372784,
-77.0453634111553));
#150339=CARTESIAN_POINT('Ctrl Pts',(-39.1034346619081,20.6889252566924,
-77.2159010245324));
#150340=CARTESIAN_POINT('Ctrl Pts',(-39.0830814703597,20.6977357804694,
-77.3868692663841));
#150341=CARTESIAN_POINT('Ctrl Pts',(-39.0625908672524,20.706605787193,-77.5589917750047));
#150342=CARTESIAN_POINT('Ctrl Pts',(-39.0459068328891,20.7154885933009,
-77.7315514531776));
#150343=CARTESIAN_POINT('Ctrl Pts',(-39.0329976347586,20.7243937714343,
-77.9045173161638));
#150344=CARTESIAN_POINT('Ctrl Pts',(-39.0200859150497,20.7333006890332,
-78.0775169649027));
#150345=CARTESIAN_POINT('Ctrl Pts',(-39.0109507853562,20.7422308710463,
-78.2509236424966));
#150346=CARTESIAN_POINT('Ctrl Pts',(-39.0056110895819,20.7511851236737,
-78.4246994601558));
#150347=CARTESIAN_POINT('Ctrl Pts',(-39.0018769231076,20.7574470291037,
-78.5462247042482));
#150348=CARTESIAN_POINT('Ctrl Pts',(-39.0000000081285,20.76372052433,-78.6679303367742));
#150349=CARTESIAN_POINT('Ctrl Pts',(-39.,20.769999979994,-78.7897987614735));
#150350=CARTESIAN_POINT('Ctrl Pts',(-40.5058324224785,20.4814581622114,
-73.2082484262411));
#150351=CARTESIAN_POINT('Ctrl Pts',(-40.6336903802598,20.26999998,-73.2855702871256));
#150352=CARTESIAN_POINT('Ctrl Pts',(-40.8552491802306,20.26999998,-73.4195575571114));
#150353=CARTESIAN_POINT('Ctrl Pts',(-42.8933128344149,20.4915183317059,
-69.2466191256953));
#150354=CARTESIAN_POINT('Ctrl Pts',(-43.0367110660153,20.26999998,-69.2967901887638));
#150355=CARTESIAN_POINT('Ctrl Pts',(-43.2510347775237,20.26999998,-69.4579320833189));
#150356=CARTESIAN_POINT('Ctrl Pts',(-45.2204439541918,20.5006239318743,
-65.2486577002759));
#150357=CARTESIAN_POINT('Ctrl Pts',(-45.3606391668745,20.269999980008,-65.3006916020456));
#150358=CARTESIAN_POINT('Ctrl Pts',(-45.5849829096511,20.26999998,-65.4599688790667));
#150359=CARTESIAN_POINT('Ctrl Pts',(-47.508501172308,20.508980519813,-61.2273317382593));
#150360=CARTESIAN_POINT('Ctrl Pts',(-47.6355531845903,20.26999998,-61.2998079338862));
#150361=CARTESIAN_POINT('Ctrl Pts',(-47.878929697957,20.26999998,-61.4386408691297));
#150362=CARTESIAN_POINT('Origin',(-47.878929697957,20.76999998,-61.4386408691297));
#150363=CARTESIAN_POINT('Ctrl Pts',(-47.508501172308,20.508980519813,-61.2273317382593));
#150364=CARTESIAN_POINT('Ctrl Pts',(-45.2204439541918,20.5006239318743,
-65.2486577002759));
#150365=CARTESIAN_POINT('Ctrl Pts',(-42.8933128344149,20.4915183317059,
-69.2466191256953));
#150366=CARTESIAN_POINT('Ctrl Pts',(-40.5058324224785,20.4814581622114,
-73.2082484262411));
#150367=CARTESIAN_POINT('Ctrl Pts',(-48.4322308821779,20.26999998,-61.14995));
#150368=CARTESIAN_POINT('Ctrl Pts',(-48.4322308821778,20.26999998,-60.64995));
#150369=CARTESIAN_POINT('Ctrl Pts',(-48.4322308821779,20.76999998,-60.64995));
#150370=CARTESIAN_POINT('Ctrl Pts',(-48.3241446058921,20.26999998,-61.1499500351048));
#150371=CARTESIAN_POINT('Ctrl Pts',(-48.2600808089264,20.2699999799996,
-60.6982023497825));
#150372=CARTESIAN_POINT('Ctrl Pts',(-48.2513645254321,20.7193046642187,
-60.64995));
#150373=CARTESIAN_POINT('Ctrl Pts',(-48.2139982277207,20.26999998,-61.1739383548812));
#150374=CARTESIAN_POINT('Ctrl Pts',(-48.0943216716052,20.2699999800004,
-60.7795557753816));
#150375=CARTESIAN_POINT('Ctrl Pts',(-48.0673245582317,20.6674580465872,
-60.6979267287055));
#150376=CARTESIAN_POINT('Ctrl Pts',(-48.0199090060446,20.26999998,-61.2698825577664));
#150377=CARTESIAN_POINT('Ctrl Pts',(-47.822827316261,20.2699999799996,-60.9964143345891));
#150378=CARTESIAN_POINT('Ctrl Pts',(-47.7433968711081,20.5758225659973,
-60.8898150965897));
#150379=CARTESIAN_POINT('Ctrl Pts',(-47.9338045255937,20.26999998,-61.3424446783372));
#150380=CARTESIAN_POINT('Ctrl Pts',(-47.7072095971588,20.2699999800002,
-61.1330776360543));
#150381=CARTESIAN_POINT('Ctrl Pts',(-47.5998785057972,20.5350112502637,
-61.0349912654872));
#150382=CARTESIAN_POINT('Ctrl Pts',(-47.878929697957,20.26999998,-61.4386408691297));
#150383=CARTESIAN_POINT('Ctrl Pts',(-47.6355531845903,20.26999998,-61.2998079338861));
#150384=CARTESIAN_POINT('Ctrl Pts',(-47.508501172308,20.508980519813,-61.2273317382593));
#150385=CARTESIAN_POINT('Origin',(-59.5,19.76999998,-55.24995));
#150386=CARTESIAN_POINT('',(-60.,19.76999998,-174.34995));
#150387=CARTESIAN_POINT('Origin',(-59.5,19.76999998,-174.34995));
#150388=CARTESIAN_POINT('',(-60.,19.76999998,-58.24995));
#150389=CARTESIAN_POINT('Origin',(-57.,19.76999998,-174.34995));
#150390=CARTESIAN_POINT('Origin',(-57.,19.76999998,-174.34995));
#150391=CARTESIAN_POINT('Origin',(0.,-12.9675000200281,-60.64995));
#150392=CARTESIAN_POINT('',(-40.4124516162212,-44.1531546065107,-76.3934867515094));
#150393=CARTESIAN_POINT('',(-40.1769968691274,-38.5367831471222,-83.7339979355897));
#150394=CARTESIAN_POINT('Ctrl Pts',(-40.4124516186295,-44.153154649867,
-76.3934867953418));
#150395=CARTESIAN_POINT('Ctrl Pts',(-40.3617744129706,-42.9337786094335,
-78.0770953638969));
#150396=CARTESIAN_POINT('Ctrl Pts',(-40.3094531768732,-41.687877666225,
-79.7436883163613));
#150397=CARTESIAN_POINT('Ctrl Pts',(-40.2557312547753,-40.4102611753384,
-81.3821766826868));
#150398=CARTESIAN_POINT('Ctrl Pts',(-40.2297515899839,-39.7924119460272,
-82.174541826367));
#150399=CARTESIAN_POINT('Ctrl Pts',(-40.2034884202245,-39.1682975463451,
-82.9589328525541));
#150400=CARTESIAN_POINT('Ctrl Pts',(-40.1769969653749,-38.5367854415027,
-83.7339951196695));
#150401=CARTESIAN_POINT('Ctrl Pts',(-49.0214378669496,-44.1865817238571,
-61.2273317382593));
#150402=CARTESIAN_POINT('Ctrl Pts',(-46.2131449010667,-44.1767154324357,
-66.3184583453296));
#150403=CARTESIAN_POINT('Ctrl Pts',(-43.3552388512871,-44.1657199195518,
-71.3808409460202));
#150404=CARTESIAN_POINT('Ctrl Pts',(-40.4124516249929,-44.1531545436406,
-76.3934867142621));
#150405=CARTESIAN_POINT('Ctrl Pts',(-40.1770020116941,-38.5366991465431,
-83.7339249799794));
#150406=CARTESIAN_POINT('Ctrl Pts',(-42.228714191533,-38.5454826541321,
-80.0118606023558));
#150407=CARTESIAN_POINT('Ctrl Pts',(-44.247123664849,-38.5533652514423,
-76.2714892021909));
#150408=CARTESIAN_POINT('Ctrl Pts',(-48.239176789686,-38.5677719010369,
-68.7661813852757));
#150409=CARTESIAN_POINT('Ctrl Pts',(-50.2126317933694,-38.5742944332221,
-65.0011376410615));
#150410=CARTESIAN_POINT('Ctrl Pts',(-52.1700794675439,-38.5802945048887,
-61.2273317382593));
#150411=CARTESIAN_POINT('Ctrl Pts',(-52.5768547844511,-38.28000002,-61.4386408691297));
#150412=CARTESIAN_POINT('Ctrl Pts',(-52.2861787013546,-38.28000002,-61.287642251635));
#150413=CARTESIAN_POINT('Ctrl Pts',(-52.1700794675439,-38.5802945048887,
-61.2273317382593));
#150414=CARTESIAN_POINT('Ctrl Pts',(-52.6146146074011,-38.28000002,-61.3659524750795));
#150415=CARTESIAN_POINT('Ctrl Pts',(-52.3399181230539,-38.28000002,-61.1584857199633));
#150416=CARTESIAN_POINT('Ctrl Pts',(-52.238210979969,-38.595348210897,-61.0819498253042));
#150417=CARTESIAN_POINT('Ctrl Pts',(-52.6705520955624,-38.28000002,-61.3040259447327));
#150418=CARTESIAN_POINT('Ctrl Pts',(-52.4211494089633,-38.28000002,-61.0428817134857));
#150419=CARTESIAN_POINT('Ctrl Pts',(-52.3391546482515,-38.6176244716287,
-60.958102271836));
#150420=CARTESIAN_POINT('Ctrl Pts',(-52.7375342894722,-38.28000002,-61.2567639997891));
#150421=CARTESIAN_POINT('Ctrl Pts',(-52.5193575501107,-38.28000002,-60.9475523661893));
#150422=CARTESIAN_POINT('Ctrl Pts',(-52.4601060488528,-38.6442121687577,
-60.8635779995782));
#150423=CARTESIAN_POINT('Origin',(-52.5768547844511,-38.78000002,-61.4386408691297));
#150424=CARTESIAN_POINT('Ctrl Pts',(-49.940073970993,-44.93000002,-61.14995));
#150425=CARTESIAN_POINT('Ctrl Pts',(-49.940073970993,-44.9300000199999,
-60.64995));
#150426=CARTESIAN_POINT('Ctrl Pts',(-49.940073970993,-44.43000002,-60.64995));
#150427=CARTESIAN_POINT('Ctrl Pts',(-49.8863992897437,-44.93000002,-61.1499500208808));
#150428=CARTESIAN_POINT('Ctrl Pts',(-49.8456849729423,-44.93000002,-60.6251406982113));
#150429=CARTESIAN_POINT('Ctrl Pts',(-49.847975325787,-44.405792727464,-60.64995));
#150430=CARTESIAN_POINT('Ctrl Pts',(-49.8338483436824,-44.93000002,-61.1560263819637));
#150431=CARTESIAN_POINT('Ctrl Pts',(-49.7496896969128,-44.93000002,-60.6104390400057));
#150432=CARTESIAN_POINT('Ctrl Pts',(-49.7578576522452,-44.382047471718,
-60.6621027778979));
#150433=CARTESIAN_POINT('Ctrl Pts',(-49.7309938571501,-44.93000002,-61.1800821203567));
#150434=CARTESIAN_POINT('Ctrl Pts',(-49.5467847765664,-44.93000002,-60.601523688823));
#150435=CARTESIAN_POINT('Ctrl Pts',(-49.581571905815,-44.3354917333839,
-60.7102142267434));
#150436=CARTESIAN_POINT('Ctrl Pts',(-49.6799439551145,-44.93000002,-61.1985082982007));
#150437=CARTESIAN_POINT('Ctrl Pts',(-49.4373419157212,-44.9300000199997,
-60.6088839981636));
#150438=CARTESIAN_POINT('Ctrl Pts',(-49.494126795535,-44.312341612126,-60.7470666030416));
#150439=CARTESIAN_POINT('Ctrl Pts',(-49.5856644732959,-44.93000002,-61.2469206297));
#150440=CARTESIAN_POINT('Ctrl Pts',(-49.2138065931458,-44.9300000200003,
-60.6541841685405));
#150441=CARTESIAN_POINT('Ctrl Pts',(-49.3327124735647,-44.2695203114938,
-60.8438912527599));
#150442=CARTESIAN_POINT('Ctrl Pts',(-49.5420691606389,-44.93000002,-61.2767318781126));
#150443=CARTESIAN_POINT('Ctrl Pts',(-49.0989170947817,-44.9300000200002,
-60.6933131425846));
#150444=CARTESIAN_POINT('Ctrl Pts',(-49.2581152115204,-44.2496846870305,
-60.9035137960622));
#150445=CARTESIAN_POINT('Ctrl Pts',(-49.4633104246523,-44.93000002,-61.3496883835064));
#150446=CARTESIAN_POINT('Ctrl Pts',(-48.8657738933764,-44.9300000199998,
-60.8209262952069));
#150447=CARTESIAN_POINT('Ctrl Pts',(-49.1234012768228,-44.2138057335947,
-61.0494267271759));
#150448=CARTESIAN_POINT('Ctrl Pts',(-49.4296447656355,-44.93000002,-61.3916439172571));
#150449=CARTESIAN_POINT('Ctrl Pts',(-48.7532051342216,-44.93000002,-60.9097365191184));
#150450=CARTESIAN_POINT('Ctrl Pts',(-49.0658454246046,-44.1984444719328,
-61.1333401037095));
#150451=CARTESIAN_POINT('Ctrl Pts',(-49.4036629110189,-44.93000002,-61.4386408691297));
#150452=CARTESIAN_POINT('Ctrl Pts',(-48.6588221091937,-44.93000002,-61.026863396898));
#150453=CARTESIAN_POINT('Ctrl Pts',(-49.0214378669497,-44.1865817238571,
-61.2273317382593));
#150454=CARTESIAN_POINT('Origin',(-49.4036629110189,-44.43000002,-61.4386408691297));
#150455=CARTESIAN_POINT('Origin',(-49.940073970993,-44.43000002,-61.14995));
#150456=CARTESIAN_POINT('Ctrl Pts',(-52.418503743379,-38.6078427661477,
-171.27120723903));
#150457=CARTESIAN_POINT('Ctrl Pts',(-52.508648517912,-38.28000002,-171.191647032252));
#150458=CARTESIAN_POINT('Ctrl Pts',(-52.7704579175044,-38.28000002,-170.960578619515));
#150459=CARTESIAN_POINT('Ctrl Pts',(-52.4966135335128,-38.6055762491043,
-171.358452481822));
#150460=CARTESIAN_POINT('Ctrl Pts',(-52.5972087752045,-38.2800000200018,
-171.289280606396));
#150461=CARTESIAN_POINT('Ctrl Pts',(-52.8865885798003,-38.28000002,-171.092159149585));
#150462=CARTESIAN_POINT('Ctrl Pts',(-52.5554277399439,-38.6065951776351,
-171.457851777602));
#150463=CARTESIAN_POINT('Ctrl Pts',(-52.6638881026927,-38.2800000200005,
-171.402873892562));
#150464=CARTESIAN_POINT('Ctrl Pts',(-52.9752899136351,-38.28000002,-171.24095231752));
#150465=CARTESIAN_POINT('Ctrl Pts',(-52.6330841414732,-38.6181228329597,
-171.679920679702));
#150466=CARTESIAN_POINT('Ctrl Pts',(-52.7468873373812,-38.2800000199994,
-171.654013242837));
#150467=CARTESIAN_POINT('Ctrl Pts',(-53.0969739026007,-38.28000002,-171.570371861396));
#150468=CARTESIAN_POINT('Ctrl Pts',(-52.6495272179227,-38.6283824768232,
-171.795722243821));
#150469=CARTESIAN_POINT('Ctrl Pts',(-52.7606056378773,-38.28000002,-171.785522775662));
#150470=CARTESIAN_POINT('Ctrl Pts',(-53.1262583244907,-38.28000002,-171.740763530748));
#150471=CARTESIAN_POINT('Ctrl Pts',(-52.6451348158641,-38.6439112191758,
-171.916267709546));
#150472=CARTESIAN_POINT('Ctrl Pts',(-52.748069378376,-38.28000002,-171.916267709546));
#150473=CARTESIAN_POINT('Ctrl Pts',(-53.1262583325313,-38.28000002,-171.916267709546));
#150474=CARTESIAN_POINT('',(-52.418503743379,-38.607842766148,-171.271207239029));
#150475=CARTESIAN_POINT('Origin',(-52.7704579175045,-38.78000002,-170.960578619515));
#150476=CARTESIAN_POINT('Origin',(-53.1262583325313,-38.78000002,-171.916267709546));
#150477=CARTESIAN_POINT('Ctrl Pts',(-52.6451348158641,-38.6439112191758,
-171.916267709546));
#150478=CARTESIAN_POINT('Ctrl Pts',(-52.6495272179227,-38.6283824768232,
-171.795722243821));
#150479=CARTESIAN_POINT('Ctrl Pts',(-52.6330841414732,-38.6181228329597,
-171.679920679702));
#150480=CARTESIAN_POINT('Ctrl Pts',(-52.5554277399439,-38.6065951776351,
-171.457851777602));
#150481=CARTESIAN_POINT('Ctrl Pts',(-52.4966135335128,-38.6055762491043,
-171.358452481822));
#150482=CARTESIAN_POINT('Ctrl Pts',(-52.418503743379,-38.6078427661481,
-171.27120723903));
#150483=CARTESIAN_POINT('Origin',(-53.1262583325313,-38.78000002,-179.64995));
#150484=CARTESIAN_POINT('Origin',(-53.1262583325313,-38.78000002,-176.84995));
#150485=CARTESIAN_POINT('Origin',(83.2809572255632,-37.78000002,-176.84995));
#150486=CARTESIAN_POINT('',(-53.3846587239314,-37.9343850848642,-177.325518346031));
#150487=CARTESIAN_POINT('Ctrl Pts',(-53.1262583325313,-38.28000002,-176.84995));
#150488=CARTESIAN_POINT('Ctrl Pts',(-53.1262583407606,-38.28000002,-176.958526013972));
#150489=CARTESIAN_POINT('Ctrl Pts',(-53.1455750275301,-38.2433781645652,
-177.065457314865));
#150490=CARTESIAN_POINT('Ctrl Pts',(-53.2302250969522,-38.1165826570878,
-177.234494972704));
#150491=CARTESIAN_POINT('Ctrl Pts',(-53.2963306348783,-38.0282371456548,
-177.295050892481));
#150492=CARTESIAN_POINT('Ctrl Pts',(-53.3846587239314,-37.9343850848642,
-177.325518346031));
#150493=CARTESIAN_POINT('',(-57.,-37.78000002,-177.34995));
#150494=CARTESIAN_POINT('Origin',(-57.,-37.78000002,-176.84995));
#150495=CARTESIAN_POINT('',(-53.5288692553037,-37.78000002,-177.34995));
#150496=CARTESIAN_POINT('',(-60.,-37.78000002,-177.34995));
#150497=CARTESIAN_POINT('Origin',(-53.5072457281298,-37.7806204038353,-176.855120810331));
#150498=CARTESIAN_POINT('Origin',(-57.,-37.78000002,-174.34995));
#150499=CARTESIAN_POINT('',(-60.,-37.78000002,-174.34995));
#150500=CARTESIAN_POINT('Origin',(-59.5,-37.78000002,-174.34995));
#150501=CARTESIAN_POINT('Origin',(-57.,-37.78000002,-174.34995));
#150502=CARTESIAN_POINT('Origin',(-59.5,-37.78000002,-55.2499500000007));
#150503=CARTESIAN_POINT('',(-60.,-37.78000002,-174.34995));
#150504=CARTESIAN_POINT('Ctrl Pts',(-52.1700794675439,-38.5802945048887,
-61.2273317382593));
#150505=CARTESIAN_POINT('Ctrl Pts',(-52.2861787013546,-38.28000002,-61.287642251635));
#150506=CARTESIAN_POINT('Ctrl Pts',(-52.5768547844511,-38.28000002,-61.4386408691297));
#150507=CARTESIAN_POINT('Ctrl Pts',(-50.2126317933694,-38.5742944332221,
-65.0011376410615));
#150508=CARTESIAN_POINT('Ctrl Pts',(-50.3387340734665,-38.2800000200587,
-65.0466233854387));
#150509=CARTESIAN_POINT('Ctrl Pts',(-50.6164606414324,-38.28000002,-65.2124482077584));
#150510=CARTESIAN_POINT('Ctrl Pts',(-48.239176789686,-38.5677719010369,
-68.7661813852757));
#150511=CARTESIAN_POINT('Ctrl Pts',(-48.3685987197966,-38.28000002,-68.8102729799503));
#150512=CARTESIAN_POINT('Ctrl Pts',(-48.6396458371624,-38.28000002,-68.9774905161504));
#150513=CARTESIAN_POINT('Ctrl Pts',(-44.247123664849,-38.5533652514423,
-76.2714892021909));
#150514=CARTESIAN_POINT('Ctrl Pts',(-44.3795316629781,-38.28000002,-76.3187098252974));
#150515=CARTESIAN_POINT('Ctrl Pts',(-44.6396194153305,-38.28000002,-76.4827983330569));
#150516=CARTESIAN_POINT('Ctrl Pts',(-42.228714191533,-38.5454826541321,
-80.0118606023558));
#150517=CARTESIAN_POINT('Ctrl Pts',(-42.3648252555903,-38.2800000199999,
-80.0572213824928));
#150518=CARTESIAN_POINT('Ctrl Pts',(-42.6166022657662,-38.28000002,-80.2231727548289));
#150519=CARTESIAN_POINT('Ctrl Pts',(-40.177002011694,-38.5366991465431,
-83.7339249799794));
#150520=CARTESIAN_POINT('Ctrl Pts',(-40.3021382496555,-38.28000002,-83.8030917170923));
#150521=CARTESIAN_POINT('Ctrl Pts',(-40.5593018105246,-38.28000002,-83.9452341108497));
#150522=CARTESIAN_POINT('Origin',(-40.5593018105246,-38.78000002,-83.9452341108497));
#150523=CARTESIAN_POINT('Ctrl Pts',(-39.501185810989,-38.28000002,-88.4514222001374));
#150524=CARTESIAN_POINT('Ctrl Pts',(-38.9924949303698,-38.2800000199999,
-88.4594633229731));
#150525=CARTESIAN_POINT('Ctrl Pts',(-39.0013194479405,-38.78868436226,-88.4593423056752));
#150526=CARTESIAN_POINT('Ctrl Pts',(-39.4887748891021,-38.28000002,-87.6395099780675));
#150527=CARTESIAN_POINT('Ctrl Pts',(-39.0236444192854,-38.2800000199999,
-87.6419250197084));
#150528=CARTESIAN_POINT('Ctrl Pts',(-38.9875195439244,-38.7437610060684,
-87.6058431711693));
#150529=CARTESIAN_POINT('Ctrl Pts',(-39.573744011109,-38.28000002,-86.8424396494651));
#150530=CARTESIAN_POINT('Ctrl Pts',(-39.1452121684012,-38.2800000199999,
-86.8067306385414));
#150531=CARTESIAN_POINT('Ctrl Pts',(-39.0819230239498,-38.6993578205918,
-86.7691329026017));
#150532=CARTESIAN_POINT('Ctrl Pts',(-39.9423232315955,-38.28000002,-85.2797330990276));
#150533=CARTESIAN_POINT('Ctrl Pts',(-39.6000058575066,-38.28000002,-85.1938582132543));
#150534=CARTESIAN_POINT('Ctrl Pts',(-39.4914430970225,-38.6119029144712,
-85.1306812313982));
#150535=CARTESIAN_POINT('Ctrl Pts',(-40.2295799875885,-38.28000002,-84.5090080181066));
#150536=CARTESIAN_POINT('Ctrl Pts',(-39.9253332832201,-38.28000002,-84.3974254090272));
#150537=CARTESIAN_POINT('Ctrl Pts',(-39.8106304317714,-38.5685582950589,
-84.3236210863548));
#150538=CARTESIAN_POINT('Ctrl Pts',(-40.6353602321306,-38.28000002,-83.8110748193107));
#150539=CARTESIAN_POINT('Ctrl Pts',(-40.3863780761056,-38.2800000199999,
-83.6661897145683));
#150540=CARTESIAN_POINT('Ctrl Pts',(-40.2614750853509,-38.5292032377738,
-83.5935603822576));
#150541=CARTESIAN_POINT('',(-39.,-38.78000002,-88.296486260558));
#150542=CARTESIAN_POINT('Origin',(-39.5,-38.78000002,-88.296486260558));
#150543=CARTESIAN_POINT('Ctrl Pts',(-39.,-38.7800000199999,-88.296486260558));
#150544=CARTESIAN_POINT('Ctrl Pts',(-39.0000000062169,-38.7719099009273,
-88.1429224351612));
#150545=CARTESIAN_POINT('Ctrl Pts',(-39.0036277971858,-38.7638211626808,
-87.9898921853818));
#150546=CARTESIAN_POINT('Ctrl Pts',(-39.0107984053575,-38.7557567490772,
-87.8374192038769));
#150547=CARTESIAN_POINT('Ctrl Pts',(-39.0183112214607,-38.7473074718426,
-87.677669648007));
#150548=CARTESIAN_POINT('Ctrl Pts',(-39.0297122017381,-38.7388842761647,
-87.5185312036824));
#150549=CARTESIAN_POINT('Ctrl Pts',(-39.0449550120729,-38.7304903061357,
-87.3600099107693));
#150550=CARTESIAN_POINT('Ctrl Pts',(-39.0596505316727,-38.7223977202955,
-87.207180300231));
#150551=CARTESIAN_POINT('Ctrl Pts',(-39.077917034903,-38.7143314169322,
-87.0549234998415));
#150552=CARTESIAN_POINT('Ctrl Pts',(-39.0997643567929,-38.7062848243322,
-86.9032368258097));
#150553=CARTESIAN_POINT('Ctrl Pts',(-39.1214542928114,-38.698296198562,
-86.7526428870573));
#150554=CARTESIAN_POINT('Ctrl Pts',(-39.1466736915941,-38.6903261944346,
-86.6026101662608));
#150555=CARTESIAN_POINT('Ctrl Pts',(-39.1754830928313,-38.6823712868514,
-86.4531391760827));
#150556=CARTESIAN_POINT('Ctrl Pts',(-39.2037909907832,-38.6745548553252,
-86.3062701210167));
#150557=CARTESIAN_POINT('Ctrl Pts',(-39.235565317799,-38.6667522576286,
-86.1599427682393));
#150558=CARTESIAN_POINT('Ctrl Pts',(-39.270909903876,-38.6589743777485,
-86.0141707055388));
#150559=CARTESIAN_POINT('Ctrl Pts',(-39.2761061202792,-38.6578309056783,
-85.9927398934287));
#150560=CARTESIAN_POINT('Ctrl Pts',(-39.2813795805843,-38.6566880047769,
-85.9713211164729));
#150561=CARTESIAN_POINT('Ctrl Pts',(-39.2867306934393,-38.6555457510815,
-85.9499144550484));
#150562=CARTESIAN_POINT('Ctrl Pts',(-39.3250047995163,-38.6473757235958,
-85.7968022235706));
#150563=CARTESIAN_POINT('Ctrl Pts',(-39.3672569048895,-38.6393176867488,
-85.6441886491297));
#150564=CARTESIAN_POINT('Ctrl Pts',(-39.4136102954607,-38.6312998630796,
-85.4924257215471));
#150565=CARTESIAN_POINT('Ctrl Pts',(-39.4600767763118,-38.6232624779951,
-85.340292531687));
#150566=CARTESIAN_POINT('Ctrl Pts',(-39.5106653738111,-38.6152650402226,
-85.18901375742));
#150567=CARTESIAN_POINT('Ctrl Pts',(-39.5655061564177,-38.6072793248838,
-85.038976709348));
#150568=CARTESIAN_POINT('Ctrl Pts',(-39.6166005030304,-38.5998391519308,
-84.8991894091933));
#150569=CARTESIAN_POINT('Ctrl Pts',(-39.6713866171152,-38.5924093742851,
-84.7604801244748));
#150570=CARTESIAN_POINT('Ctrl Pts',(-39.7299639667939,-38.5850061155278,
-84.623191394671));
#150571=CARTESIAN_POINT('Ctrl Pts',(-39.787313465737,-38.5777580378559,
-84.4887803995003));
#150572=CARTESIAN_POINT('Ctrl Pts',(-39.8482976383897,-38.5705354069193,
-84.3557310522515));
#150573=CARTESIAN_POINT('Ctrl Pts',(-39.9129938870569,-38.5633907141695,
-84.2243930007107));
#150574=CARTESIAN_POINT('Ctrl Pts',(-39.975932931367,-38.5564400772652,
-84.0966222007675));
#150575=CARTESIAN_POINT('Ctrl Pts',(-40.0423857789552,-38.5495633891073,
-83.9704711495694));
#150576=CARTESIAN_POINT('Ctrl Pts',(-40.1123986724843,-38.5428430665576,
-83.8462874167416));
#150577=CARTESIAN_POINT('Ctrl Pts',(-40.1336047881332,-38.5408075566678,
-83.8086735649592));
#150578=CARTESIAN_POINT('Ctrl Pts',(-40.1551372943644,-38.5387866226394,
-83.7712403709099));
#150579=CARTESIAN_POINT('Ctrl Pts',(-40.1769968691274,-38.5367831471222,
-83.7339979355897));
#150580=CARTESIAN_POINT('Origin',(-39.5,-38.78000002,-55.2499500000007));
#150581=CARTESIAN_POINT('',(-39.,-38.78000002,-143.762156710948));
#150582=CARTESIAN_POINT('Origin',(-39.5,-38.78000002,-143.762156710948));
#150583=CARTESIAN_POINT('',(-39.,-38.78000002,-129.34995));
#150584=CARTESIAN_POINT('Ctrl Pts',(-40.5593018105246,-38.28000002,-148.113408860656));
#150585=CARTESIAN_POINT('Ctrl Pts',(-40.3021382496555,-38.28000002,-148.255551254414));
#150586=CARTESIAN_POINT('Ctrl Pts',(-40.177002011694,-38.5366991465431,
-148.324717991527));
#150587=CARTESIAN_POINT('Ctrl Pts',(-40.1916835970713,-38.28000002,-147.4483151549));
#150588=CARTESIAN_POINT('Ctrl Pts',(-39.8835176458245,-38.2800000199999,
-147.559388080201));
#150589=CARTESIAN_POINT('Ctrl Pts',(-39.7685879100996,-38.5741769664791,
-147.628968394962));
#150590=CARTESIAN_POINT('Ctrl Pts',(-39.9350562729928,-38.28000002,-146.743548549419));
#150591=CARTESIAN_POINT('Ctrl Pts',(-39.5917422326584,-38.28000002,-146.831469990429));
#150592=CARTESIAN_POINT('Ctrl Pts',(-39.4833958584245,-38.6137964624649,
-146.890860603676));
#150593=CARTESIAN_POINT('Ctrl Pts',(-39.6739630147418,-38.28000002,-145.64333076277));
#150594=CARTESIAN_POINT('Ctrl Pts',(-39.2753714947002,-38.28000002,-145.715141322844));
#150595=CARTESIAN_POINT('Ctrl Pts',(-39.1932922388301,-38.6753614306792,
-145.737334852943));
#150596=CARTESIAN_POINT('Ctrl Pts',(-39.6085749933904,-38.28000002,-145.268506383101));
#150597=CARTESIAN_POINT('Ctrl Pts',(-39.1901844457866,-38.28000002,-145.326704913328));
#150598=CARTESIAN_POINT('Ctrl Pts',(-39.1206388813576,-38.6962900137231,
-145.344124086281));
#150599=CARTESIAN_POINT('Ctrl Pts',(-39.5218408888656,-38.28000002,-144.51836712325));
#150600=CARTESIAN_POINT('Ctrl Pts',(-39.0623543759033,-38.28000002,-144.546929015961));
#150601=CARTESIAN_POINT('Ctrl Pts',(-39.0242676544824,-38.7380634612154,
-144.556697955888));
#150602=CARTESIAN_POINT('Ctrl Pts',(-39.5000000006721,-38.28000002,-144.14127791415));
#150603=CARTESIAN_POINT('Ctrl Pts',(-39.0205601185727,-38.28000002,-144.152421745394));
#150604=CARTESIAN_POINT('Ctrl Pts',(-39.,-38.7590078240271,-144.160623302193));
#150605=CARTESIAN_POINT('Ctrl Pts',(-39.5,-38.28000002,-143.762156710948));
#150606=CARTESIAN_POINT('Ctrl Pts',(-38.9999999999999,-38.2800000199999,
-143.762156710948));
#150607=CARTESIAN_POINT('Ctrl Pts',(-39.,-38.78000002,-143.762156710948));
#150608=CARTESIAN_POINT('',(-40.1769830688311,-38.5367008848306,-148.324685721429));
#150609=CARTESIAN_POINT('Origin',(-40.5593018105246,-38.78000002,-148.113408860656));
#150610=CARTESIAN_POINT('Ctrl Pts',(-40.1769830688311,-38.5367008848306,
-148.324685721429));
#150611=CARTESIAN_POINT('Ctrl Pts',(-39.768579091655,-38.5741781915598,
-147.628945571812));
#150612=CARTESIAN_POINT('Ctrl Pts',(-39.4833928683118,-38.6137970970181,
-146.890848714228));
#150613=CARTESIAN_POINT('Ctrl Pts',(-39.2899934453616,-38.6548397746078,
-146.121843436521));
#150614=CARTESIAN_POINT('Ctrl Pts',(-39.1932922388302,-38.6753614306792,
-145.737334852943));
#150615=CARTESIAN_POINT('Ctrl Pts',(-39.1206388813576,-38.6962900137231,
-145.344124086281));
#150616=CARTESIAN_POINT('Ctrl Pts',(-39.07245326792,-38.7171767374692,-144.950411021085));
#150617=CARTESIAN_POINT('Ctrl Pts',(-39.0242676544824,-38.7380634612153,
-144.556697955888));
#150618=CARTESIAN_POINT('Ctrl Pts',(-39.,-38.759007824027,-144.160623302193));
#150619=CARTESIAN_POINT('Ctrl Pts',(-39.,-38.7800000199999,-143.762156710948));
#150620=CARTESIAN_POINT('Ctrl Pts',(-40.1770020116941,-38.5366991465431,
-148.324717991527));
#150621=CARTESIAN_POINT('Ctrl Pts',(-40.3021382496555,-38.28000002,-148.255551254414));
#150622=CARTESIAN_POINT('Ctrl Pts',(-40.5593018105247,-38.28000002,-148.113408860656));
#150623=CARTESIAN_POINT('Ctrl Pts',(-42.2505775009144,-38.5455762523402,
-152.086445166823));
#150624=CARTESIAN_POINT('Ctrl Pts',(-42.3869374257262,-38.280000019955,
-152.041577619703));
#150625=CARTESIAN_POINT('Ctrl Pts',(-42.6385250759047,-38.28000002,-151.875132894361));
#150626=CARTESIAN_POINT('Ctrl Pts',(-44.2901446089557,-38.5535332680681,
-155.866861850893));
#150627=CARTESIAN_POINT('Ctrl Pts',(-44.4227143745257,-38.2800000199852,
-155.82004311619));
#150628=CARTESIAN_POINT('Ctrl Pts',(-44.6827387638399,-38.28000002,-155.655552720034));
#150629=CARTESIAN_POINT('Ctrl Pts',(-48.3237478755738,-38.5680639323333,
-163.452672197745));
#150630=CARTESIAN_POINT('Ctrl Pts',(-48.4532973709855,-38.280000020015,
-163.409015135176));
#150631=CARTESIAN_POINT('Ctrl Pts',(-48.7243729558795,-38.28000002,-163.241363066864));
#150632=CARTESIAN_POINT('Ctrl Pts',(-50.3175866645898,-38.5746359826999,
-167.258178117331));
#150633=CARTESIAN_POINT('Ctrl Pts',(-50.4437502527583,-38.2800000199406,
-167.213058728775));
#150634=CARTESIAN_POINT('Ctrl Pts',(-50.7215899998133,-38.28000002,-167.046867503852));
#150635=CARTESIAN_POINT('Ctrl Pts',(-52.2951895046066,-38.58067735034,-171.07256826174));
#150636=CARTESIAN_POINT('Ctrl Pts',(-52.4111831155989,-38.28000002,-171.012340412829));
#150637=CARTESIAN_POINT('Ctrl Pts',(-52.7021525552272,-38.28000002,-170.861259130871));
#150638=CARTESIAN_POINT('',(-52.2951895046066,-38.58067735034,-171.07256826174));
#150639=CARTESIAN_POINT('Origin',(-52.7021525552272,-38.78000002,-170.861259130871));
#150640=CARTESIAN_POINT('Ctrl Pts',(-52.2951895046066,-38.58067735034,-171.07256826174));
#150641=CARTESIAN_POINT('Ctrl Pts',(-50.3175866666889,-38.5746359777978,
-167.25817811658));
#150642=CARTESIAN_POINT('Ctrl Pts',(-48.3237478777393,-38.5680639275182,
-163.452672197015));
#150643=CARTESIAN_POINT('Ctrl Pts',(-44.2901446111941,-38.5535332634494,
-155.866861850102));
#150644=CARTESIAN_POINT('Ctrl Pts',(-42.2505775032295,-38.5455762478314,
-152.086445166061));
#150645=CARTESIAN_POINT('Ctrl Pts',(-40.1770020116941,-38.5366991465431,
-148.324717991527));
#150646=CARTESIAN_POINT('Ctrl Pts',(-52.7704579175044,-38.28000002,-170.960578619515));
#150647=CARTESIAN_POINT('Ctrl Pts',(-52.5086485179119,-38.28000002,-171.191647032251));
#150648=CARTESIAN_POINT('Ctrl Pts',(-52.4185037433787,-38.6078427661476,
-171.271207239029));
#150649=CARTESIAN_POINT('Ctrl Pts',(-52.7436831755344,-38.28000002,-170.930241803514));
#150650=CARTESIAN_POINT('Ctrl Pts',(-52.4702729319568,-38.2800000200013,
-171.135526834247));
#150651=CARTESIAN_POINT('Ctrl Pts',(-52.370156234462,-38.5972036761564,
-171.210531232685));
#150652=CARTESIAN_POINT('Ctrl Pts',(-52.7208049303309,-38.28000002,-170.897181907961));
#150653=CARTESIAN_POINT('Ctrl Pts',(-52.4376229301059,-38.2800000199995,
-171.075889787111));
#150654=CARTESIAN_POINT('Ctrl Pts',(-52.3288572922619,-38.5881022353565,
-171.144413209532));
#150655=CARTESIAN_POINT('Ctrl Pts',(-52.7021525552272,-38.28000002,-170.861259130871));
#150656=CARTESIAN_POINT('Ctrl Pts',(-52.4111831155989,-38.28000002,-171.012340412829));
#150657=CARTESIAN_POINT('Ctrl Pts',(-52.2951895046066,-38.58067735034,-171.072568261741));
#150658=CARTESIAN_POINT('Origin',(-81.3222999502966,-44.9387978456672,-153.374633169906));
#150659=CARTESIAN_POINT('Ctrl Pts',(-49.2787232447289,-55.08000002,-171.64995));
#150660=CARTESIAN_POINT('Ctrl Pts',(-49.2787232447289,-54.58000002,-171.64995));
#150661=CARTESIAN_POINT('Ctrl Pts',(-49.2787232447289,-54.58000002,-171.14995));
#150662=CARTESIAN_POINT('Ctrl Pts',(-49.4122135882539,-55.0708895200012,
-171.64995));
#150663=CARTESIAN_POINT('Ctrl Pts',(-49.4109716734917,-54.58000002,-171.640924254979));
#150664=CARTESIAN_POINT('Ctrl Pts',(-49.477038164104,-54.58000002,-171.149950000016));
#150665=CARTESIAN_POINT('Ctrl Pts',(-49.5456033137516,-55.061785887019,
-171.675977326981));
#150666=CARTESIAN_POINT('Ctrl Pts',(-49.548241251645,-54.58000002,-171.658003579003));
#150667=CARTESIAN_POINT('Ctrl Pts',(-49.6752036040849,-54.58000002,-171.18899099047));
#150668=CARTESIAN_POINT('Ctrl Pts',(-49.7922168368437,-55.0449549130127,
-171.776163607997));
#150669=CARTESIAN_POINT('Ctrl Pts',(-49.8066765125445,-54.5800000199999,
-171.746711574348));
#150670=CARTESIAN_POINT('Ctrl Pts',(-50.0415757300179,-54.58000002,-171.339270411997));
#150671=CARTESIAN_POINT('Ctrl Pts',(-49.9053195885289,-55.037235833176,
-171.850283164392));
#150672=CARTESIAN_POINT('Ctrl Pts',(-49.9282402287017,-54.5800000199992,
-171.817687494207));
#150673=CARTESIAN_POINT('Ctrl Pts',(-50.2096025886599,-54.58000002,-171.450449746589));
#150674=CARTESIAN_POINT('Ctrl Pts',(-50.0940694074005,-55.0243539633763,
-172.035403273235));
#150675=CARTESIAN_POINT('Ctrl Pts',(-50.1326854480763,-54.5800000200006,
-172.003556970024));
#150676=CARTESIAN_POINT('Ctrl Pts',(-50.4900116738692,-54.58000002,-171.728129909852));
#150677=CARTESIAN_POINT('Ctrl Pts',(-50.1696422500339,-55.0191962391206,
-172.14633102856));
#150678=CARTESIAN_POINT('Ctrl Pts',(-50.2162545403414,-54.58000002,-172.118296873734));
#150679=CARTESIAN_POINT('Ctrl Pts',(-50.6022836315107,-54.58000002,-171.894521542842));
#150680=CARTESIAN_POINT('Ctrl Pts',(-50.2717929158607,-55.0122246214262,
-172.38820210671));
#150681=CARTESIAN_POINT('Ctrl Pts',(-50.3290655494749,-54.58000002,-172.371853931892));
#150682=CARTESIAN_POINT('Ctrl Pts',(-50.7540399347937,-54.58000002,-172.257328160063));
#150683=CARTESIAN_POINT('Ctrl Pts',(-50.2983305691357,-55.0104134695225,
-172.51902671195));
#150684=CARTESIAN_POINT('Ctrl Pts',(-50.3588212345858,-54.5800000199993,
-172.511015867073));
#150685=CARTESIAN_POINT('Ctrl Pts',(-50.7934646034919,-54.58000002,-172.453565067926));
#150686=CARTESIAN_POINT('Ctrl Pts',(-50.2983305691361,-55.0104134695199,
-172.64995));
#150687=CARTESIAN_POINT('Ctrl Pts',(-50.3588212345988,-54.5800000199999,
-172.64995));
#150688=CARTESIAN_POINT('Ctrl Pts',(-50.7934646035069,-54.58000002,-172.64995));
#150689=CARTESIAN_POINT('Origin',(-49.2787232447289,-55.08000002,-171.14995));
#150690=CARTESIAN_POINT('Origin',(-50.7934646035069,-55.08000002,-172.64995));
#150691=CARTESIAN_POINT('Ctrl Pts',(-50.2983305691361,-55.0104134695199,
-172.64995));
#150692=CARTESIAN_POINT('Ctrl Pts',(-50.2983305691357,-55.0104134695225,
-172.51902671195));
#150693=CARTESIAN_POINT('Ctrl Pts',(-50.2717929158607,-55.0122246214262,
-172.38820210671));
#150694=CARTESIAN_POINT('Ctrl Pts',(-50.1696422500339,-55.0191962391206,
-172.14633102856));
#150695=CARTESIAN_POINT('Ctrl Pts',(-50.0940694074005,-55.0243539633763,
-172.035403273235));
#150696=CARTESIAN_POINT('Ctrl Pts',(-49.9053195885289,-55.037235833176,
-171.850283164392));
#150697=CARTESIAN_POINT('Ctrl Pts',(-49.7922168368437,-55.0449549130127,
-171.776163607997));
#150698=CARTESIAN_POINT('Ctrl Pts',(-49.5456033137516,-55.061785887019,
-171.675977326981));
#150699=CARTESIAN_POINT('Ctrl Pts',(-49.4122135882539,-55.0708895200012,
-171.64995));
#150700=CARTESIAN_POINT('Ctrl Pts',(-49.2787232447289,-55.08000002,-171.64995));
#150701=CARTESIAN_POINT('Origin',(-50.7934646035069,-55.08000002,-171.64995));
#150702=CARTESIAN_POINT('Origin',(-50.7934646035069,-55.08000002,-176.84995));
#150703=CARTESIAN_POINT('Origin',(-60.,-54.08000002,-176.84995));
#150704=CARTESIAN_POINT('',(-57.,-54.08000002,-177.34995));
#150705=CARTESIAN_POINT('Origin',(-57.,-54.08000002,-176.84995));
#150706=CARTESIAN_POINT('',(-50.9340054382093,-54.08000002,-177.34995));
#150707=CARTESIAN_POINT('',(-60.,-54.08000002,-177.34995));
#150708=CARTESIAN_POINT('Ctrl Pts',(-50.7934646035069,-54.58000002,-176.84995));
#150709=CARTESIAN_POINT('Ctrl Pts',(-50.7934646035178,-54.58000002,-176.981217345763));
#150710=CARTESIAN_POINT('Ctrl Pts',(-50.8086111287259,-54.5261134565302,
-177.110943344657));
#150711=CARTESIAN_POINT('Ctrl Pts',(-50.8606449931892,-54.3409933646562,
-177.296063436531));
#150712=CARTESIAN_POINT('Ctrl Pts',(-50.8971085935234,-54.2112673657634,
-177.34995));
#150713=CARTESIAN_POINT('Ctrl Pts',(-50.9340054382093,-54.08000002,-177.34995));
#150714=CARTESIAN_POINT('Origin',(-57.,-54.08000002,-174.34995));
#150715=CARTESIAN_POINT('',(-60.,-54.08000002,-174.34995));
#150716=CARTESIAN_POINT('Origin',(-59.5,-54.08000002,-174.34995));
#150717=CARTESIAN_POINT('Origin',(-57.,-54.08000002,-174.34995));
#150718=CARTESIAN_POINT('Origin',(-59.5,-54.08000002,0.));
#150719=CARTESIAN_POINT('',(-60.,-54.08000002,-58.24995));
#150720=CARTESIAN_POINT('Origin',(-59.5,-54.08000002,-58.24995));
#150721=CARTESIAN_POINT('',(-60.,-54.08000002,-174.34995));
#150722=CARTESIAN_POINT('Origin',(-57.,-54.08000002,-58.24995));
#150723=CARTESIAN_POINT('Origin',(-57.,-54.08000002,-58.24995));
#150724=CARTESIAN_POINT('Ctrl Pts',(-43.1572831724516,-54.58000002,-61.14995));
#150725=CARTESIAN_POINT('Ctrl Pts',(-43.1572831724515,-54.58000002,-60.6498018765538));
#150726=CARTESIAN_POINT('Ctrl Pts',(-43.1572831724516,-55.0801481215056,
-60.6499500219341));
#150727=CARTESIAN_POINT('Ctrl Pts',(-43.3817682803708,-54.58000002,-61.1499499438652));
#150728=CARTESIAN_POINT('Ctrl Pts',(-43.3143913613969,-54.58000002,-60.738433940519));
#150729=CARTESIAN_POINT('Ctrl Pts',(-43.3271185292341,-54.9843723315204,
-60.6499212610322));
#150730=CARTESIAN_POINT('Ctrl Pts',(-43.6059648750607,-54.58000002,-61.1139843549936));
#150731=CARTESIAN_POINT('Ctrl Pts',(-43.5407821982001,-54.58000002,-60.7796882578929));
#150732=CARTESIAN_POINT('Ctrl Pts',(-43.5299471737832,-54.894339587696,
-60.6499049353895));
#150733=CARTESIAN_POINT('Ctrl Pts',(-44.0540062919343,-54.58000002,-61.0395265773532));
#150734=CARTESIAN_POINT('Ctrl Pts',(-44.0046317151094,-54.58000002,-60.8040236126606));
#150735=CARTESIAN_POINT('Ctrl Pts',(-43.9881565230544,-54.7646161135089,
-60.6498916468798));
#150736=CARTESIAN_POINT('Ctrl Pts',(-44.2780419706101,-54.58000002,-61.0029930876918));
#150737=CARTESIAN_POINT('Ctrl Pts',(-44.2580491347896,-54.58000002,-60.7962448835177));
#150738=CARTESIAN_POINT('Ctrl Pts',(-44.2440095987556,-54.7260645641702,
-60.6498933522813));
#150739=CARTESIAN_POINT('Ctrl Pts',(-44.7276655629963,-54.58000002,-61.0020306983307));
#150740=CARTESIAN_POINT('Ctrl Pts',(-44.7466180387412,-54.58000002,-60.7961110321463));
#150741=CARTESIAN_POINT('Ctrl Pts',(-44.7601884828711,-54.7249655177494,
-60.6498933671499));
#150742=CARTESIAN_POINT('Ctrl Pts',(-44.9532637149968,-54.58000002,-61.0380773886891));
#150743=CARTESIAN_POINT('Ctrl Pts',(-45.0021140860287,-54.58000002,-60.8040311529121));
#150744=CARTESIAN_POINT('Ctrl Pts',(-45.0183788445834,-54.7626525929485,
-60.6498915741974));
#150745=CARTESIAN_POINT('Ctrl Pts',(-45.4045230317319,-54.58000002,-61.1130978438444));
#150746=CARTESIAN_POINT('Ctrl Pts',(-45.4698465063654,-54.58000002,-60.7804647582876));
#150747=CARTESIAN_POINT('Ctrl Pts',(-45.4809398893316,-54.8922510295813,
-60.6499045972132));
#150748=CARTESIAN_POINT('Ctrl Pts',(-45.6299507757142,-54.58000002,-61.149949944621));
#150749=CARTESIAN_POINT('Ctrl Pts',(-45.6987517183195,-54.58000002,-60.7399919909285));
#150750=CARTESIAN_POINT('Ctrl Pts',(-45.6855420836464,-54.9825427397823,
-60.6499207098429));
#150751=CARTESIAN_POINT('Ctrl Pts',(-45.8586217441897,-54.58000002,-61.14995));
#150752=CARTESIAN_POINT('Ctrl Pts',(-45.8586217441896,-54.58000002,-60.6498018765538));
#150753=CARTESIAN_POINT('Ctrl Pts',(-45.8586217441897,-55.0801481215056,
-60.6499500219341));
#150754=CARTESIAN_POINT('Origin',(-43.1572831724516,-55.08000002,-61.14995));
#150755=CARTESIAN_POINT('Origin',(1.8445455022812E-14,-55.08000002,-61.14995));
#150756=CARTESIAN_POINT('',(-42.5,-55.08000002,-60.64995));
#150757=CARTESIAN_POINT('Origin',(-42.5,-55.08000002,-61.14995));
#150758=CARTESIAN_POINT('',(1.8445455022812E-14,-55.08000002,-60.64995));
#150759=CARTESIAN_POINT('Origin',(-60.,-55.08000002,-171.14995));
#150760=CARTESIAN_POINT('Origin',(-42.5,-55.08000002,-171.14995));
#150761=CARTESIAN_POINT('Origin',(-60.,-55.08000002,-171.14995));
#150762=CARTESIAN_POINT('Origin',(-57.,-2.42462934179819E-14,-58.24995));
#150763=CARTESIAN_POINT('',(-60.,-53.58000002,-58.24995));
#150764=CARTESIAN_POINT('Origin',(-57.,-53.58000002,-58.24995));
#150765=CARTESIAN_POINT('',(-60.,-54.58000002,-58.24995));
#150766=CARTESIAN_POINT('Origin',(-57.,-53.58000002,-58.24995));
#150767=CARTESIAN_POINT('Origin',(-59.5,-53.58000002,-58.24995));
#150768=CARTESIAN_POINT('Origin',(-60.,-53.58000002,-176.84995));
#150769=CARTESIAN_POINT('',(-51.0042758555605,-53.58000002,-177.34995));
#150770=CARTESIAN_POINT('',(-57.,-53.58000002,-177.34995));
#150771=CARTESIAN_POINT('',(-60.,-53.58000002,-177.34995));
#150772=CARTESIAN_POINT('Origin',(-57.,-53.58000002,-176.84995));
#150773=CARTESIAN_POINT('Ctrl Pts',(-51.0042758555605,-53.58000002,-177.34995));
#150774=CARTESIAN_POINT('Ctrl Pts',(-51.0411727002473,-53.4487326742368,
-177.34995));
#150775=CARTESIAN_POINT('Ctrl Pts',(-51.0776363005805,-53.3190066753437,
-177.296063436531));
#150776=CARTESIAN_POINT('Ctrl Pts',(-51.1296701650438,-53.1338865834697,
-177.110943344657));
#150777=CARTESIAN_POINT('Ctrl Pts',(-51.1448166902519,-53.08000002,-176.981217345763));
#150778=CARTESIAN_POINT('Ctrl Pts',(-51.1448166902628,-53.08000002,-176.84995));
#150779=CARTESIAN_POINT('Origin',(-51.1448166902628,-52.58000002,-171.64995));
#150780=CARTESIAN_POINT('',(-50.6448166902628,-52.58000002,-172.64995));
#150781=CARTESIAN_POINT('Origin',(-51.1448166902628,-52.58000002,-172.64995));
#150782=CARTESIAN_POINT('Origin',(-51.1448166902628,-52.58000002,-176.84995));
#150783=CARTESIAN_POINT('Origin',(-51.1448166902628,-52.58000002,-172.64995));
#150784=CARTESIAN_POINT('Ctrl Pts',(-50.6496826558921,-52.51041346952,-172.64995));
#150785=CARTESIAN_POINT('Ctrl Pts',(-50.5696324866524,-53.08000002,-172.64995));
#150786=CARTESIAN_POINT('Ctrl Pts',(-51.1448166902628,-53.08000002,-172.64995));
#150787=CARTESIAN_POINT('Ctrl Pts',(-50.6496826558917,-52.5104134695225,
-172.51902671195));
#150788=CARTESIAN_POINT('Ctrl Pts',(-50.5696324866503,-53.080000020002,
-172.529650273729));
#150789=CARTESIAN_POINT('Ctrl Pts',(-51.1448166902479,-53.08000002,-172.453565067926));
#150790=CARTESIAN_POINT('Ctrl Pts',(-50.6231450026166,-52.5122246214263,
-172.38820210671));
#150791=CARTESIAN_POINT('Ctrl Pts',(-50.5479627709917,-53.08000002,-172.409726298163));
#150792=CARTESIAN_POINT('Ctrl Pts',(-51.1053920215496,-53.08000002,-172.257328160063));
#150793=CARTESIAN_POINT('Ctrl Pts',(-50.5209943367899,-52.5191962391206,
-172.14633102856));
#150794=CARTESIAN_POINT('Ctrl Pts',(-50.4615294415736,-53.08000002,-172.182182441317));
#150795=CARTESIAN_POINT('Ctrl Pts',(-50.9536357182667,-53.08000002,-171.894521542842));
#150796=CARTESIAN_POINT('Ctrl Pts',(-50.4454214941564,-52.5243539633763,
-172.035403273235));
#150797=CARTESIAN_POINT('Ctrl Pts',(-50.3972583757626,-53.0800000199979,
-172.075215659168));
#150798=CARTESIAN_POINT('Ctrl Pts',(-50.8413637606251,-53.08000002,-171.728129909852));
#150799=CARTESIAN_POINT('Ctrl Pts',(-50.256671675285,-52.537235833176,-171.850283164392));
#150800=CARTESIAN_POINT('Ctrl Pts',(-50.2296016046087,-53.080000020002,
-171.888983273332));
#150801=CARTESIAN_POINT('Ctrl Pts',(-50.5609546754159,-53.08000002,-171.450449746589));
#150802=CARTESIAN_POINT('Ctrl Pts',(-50.1435689235997,-52.5449549130127,
-171.776163607997));
#150803=CARTESIAN_POINT('Ctrl Pts',(-50.1270268918696,-53.0800000200001,
-171.809929875206));
#150804=CARTESIAN_POINT('Ctrl Pts',(-50.3929278167739,-53.08000002,-171.339270411997));
#150805=CARTESIAN_POINT('Ctrl Pts',(-49.8969554005076,-52.561785887019,
-171.675977326981));
#150806=CARTESIAN_POINT('Ctrl Pts',(-49.8942480960507,-53.08000002,-171.69520402023));
#150807=CARTESIAN_POINT('Ctrl Pts',(-50.0265556908409,-53.08000002,-171.18899099047));
#150808=CARTESIAN_POINT('Ctrl Pts',(-49.7635656750098,-52.5708895200013,
-171.64995));
#150809=CARTESIAN_POINT('Ctrl Pts',(-49.7648572777959,-53.08000002,-171.659148653595));
#150810=CARTESIAN_POINT('Ctrl Pts',(-49.8283902508599,-53.08000002,-171.149950000016));
#150811=CARTESIAN_POINT('Ctrl Pts',(-49.6300753314849,-52.58000002,-171.64995));
#150812=CARTESIAN_POINT('Ctrl Pts',(-49.6300753314848,-53.0800000199999,
-171.64995));
#150813=CARTESIAN_POINT('Ctrl Pts',(-49.6300753314849,-53.08000002,-171.14995));
#150814=CARTESIAN_POINT('',(-49.6300753314849,-52.58000002,-171.64995));
#150815=CARTESIAN_POINT('Origin',(-49.6300753314849,-52.58000002,-171.14995));
#150816=CARTESIAN_POINT('Ctrl Pts',(-49.6300753314849,-52.58000002,-171.64995));
#150817=CARTESIAN_POINT('Ctrl Pts',(-49.7635656750098,-52.5708895200013,
-171.64995));
#150818=CARTESIAN_POINT('Ctrl Pts',(-49.8969554005076,-52.561785887019,
-171.675977326981));
#150819=CARTESIAN_POINT('Ctrl Pts',(-50.1435689235997,-52.5449549130127,
-171.776163607997));
#150820=CARTESIAN_POINT('Ctrl Pts',(-50.256671675285,-52.537235833176,-171.850283164392));
#150821=CARTESIAN_POINT('Ctrl Pts',(-50.4454214941564,-52.5243539633763,
-172.035403273235));
#150822=CARTESIAN_POINT('Ctrl Pts',(-50.5209943367899,-52.5191962391206,
-172.14633102856));
#150823=CARTESIAN_POINT('Ctrl Pts',(-50.6231450026166,-52.5122246214263,
-172.38820210671));
#150824=CARTESIAN_POINT('Ctrl Pts',(-50.6496826558917,-52.5104134695225,
-172.51902671195));
#150825=CARTESIAN_POINT('Ctrl Pts',(-50.6496826558921,-52.51041346952,-172.64995));
#150826=CARTESIAN_POINT('Origin',(83.2809572255632,-52.5800000199999,-171.14995));
#150827=CARTESIAN_POINT('',(-43.9094855672884,-52.58000002,-171.64995));
#150828=CARTESIAN_POINT('Origin',(-43.9094855672884,-52.58000002,-171.14995));
#150829=CARTESIAN_POINT('',(-49.5598049141337,-52.58000002,-171.64995));
#150830=CARTESIAN_POINT('Ctrl Pts',(-43.2972503047852,-53.08000002,-170.861259130871));
#150831=CARTESIAN_POINT('Ctrl Pts',(-42.4360603595898,-53.08000002,-171.405549026075));
#150832=CARTESIAN_POINT('Ctrl Pts',(-42.9629113790828,-52.2741145284007,
-171.07256826174));
#150833=CARTESIAN_POINT('Ctrl Pts',(-43.3290496999002,-53.08000002,-170.911572751073));
#150834=CARTESIAN_POINT('Ctrl Pts',(-42.5775224401932,-53.080000020001,
-171.535704796364));
#150835=CARTESIAN_POINT('Ctrl Pts',(-43.0118891450524,-52.2900672717484,
-171.173154953435));
#150836=CARTESIAN_POINT('Ctrl Pts',(-43.3692611707715,-53.08000002,-170.954112611118));
#150837=CARTESIAN_POINT('Ctrl Pts',(-42.7308220084871,-53.0800000200015,
-171.613444114474));
#150838=CARTESIAN_POINT('Ctrl Pts',(-43.073894673874,-52.3102438041593,
-171.258275237078));
#150839=CARTESIAN_POINT('Ctrl Pts',(-43.4620142194198,-53.08000002,-171.027622760172));
#150840=CARTESIAN_POINT('Ctrl Pts',(-43.0212179754289,-53.0800000199986,
-171.708873691595));
#150841=CARTESIAN_POINT('Ctrl Pts',(-43.2170017360461,-52.3567135560047,
-171.405295505501));
#150842=CARTESIAN_POINT('Ctrl Pts',(-43.512966485493,-53.08000002,-171.057128671245));
#150843=CARTESIAN_POINT('Ctrl Pts',(-43.154321777956,-53.080000020001,-171.728961938884));
#150844=CARTESIAN_POINT('Ctrl Pts',(-43.2956718648015,-52.3822166623249,
-171.464307358546));
#150845=CARTESIAN_POINT('Ctrl Pts',(-43.6204035532382,-53.08000002,-171.104030585588));
#150846=CARTESIAN_POINT('Ctrl Pts',(-43.3978292274293,-53.080000019999,
-171.740357884216));
#150847=CARTESIAN_POINT('Ctrl Pts',(-43.4617135157955,-52.4359237144093,
-171.55811115512));
#150848=CARTESIAN_POINT('Ctrl Pts',(-43.6774556997061,-53.08000002,-171.121458138538));
#150849=CARTESIAN_POINT('Ctrl Pts',(-43.5113479697337,-53.080000019999,
-171.733309812026));
#150850=CARTESIAN_POINT('Ctrl Pts',(-43.5499633272225,-52.4644105712997,
-171.592966290451));
#150851=CARTESIAN_POINT('Ctrl Pts',(-43.7921030708942,-53.08000002,-171.144263427359));
#150852=CARTESIAN_POINT('Ctrl Pts',(-43.718452515944,-53.080000020001,-171.702758245039));
#150853=CARTESIAN_POINT('Ctrl Pts',(-43.7274774238083,-52.5215797867686,
-171.638576841342));
#150854=CARTESIAN_POINT('Ctrl Pts',(-43.8503459614229,-53.08000002,-171.149949987963));
#150855=CARTESIAN_POINT('Ctrl Pts',(-43.8149201055142,-53.08000002,-171.680268286151));
#150856=CARTESIAN_POINT('Ctrl Pts',(-43.8177416070106,-52.5505863340359,
-171.64995));
#150857=CARTESIAN_POINT('Ctrl Pts',(-43.9094855672884,-53.08000002,-171.14995));
#150858=CARTESIAN_POINT('Ctrl Pts',(-43.9094855672884,-53.0800000199999,
-171.64995));
#150859=CARTESIAN_POINT('Ctrl Pts',(-43.9094855672884,-52.58000002,-171.64995));
#150860=CARTESIAN_POINT('',(-42.9629113790828,-52.2741145284007,-171.07256826174));
#150861=CARTESIAN_POINT('Origin',(-43.2972503047852,-52.58000002,-170.861259130871));
#150862=CARTESIAN_POINT('Ctrl Pts',(-42.9629113790828,-52.2741145284007,
-171.07256826174));
#150863=CARTESIAN_POINT('Ctrl Pts',(-43.0118891450524,-52.2900672717484,
-171.173154953435));
#150864=CARTESIAN_POINT('Ctrl Pts',(-43.073894673874,-52.3102438041593,
-171.258275237078));
#150865=CARTESIAN_POINT('Ctrl Pts',(-43.2170017360461,-52.3567135560047,
-171.405295505501));
#150866=CARTESIAN_POINT('Ctrl Pts',(-43.2956718648015,-52.3822166623249,
-171.464307358546));
#150867=CARTESIAN_POINT('Ctrl Pts',(-43.4617135157955,-52.4359237144093,
-171.55811115512));
#150868=CARTESIAN_POINT('Ctrl Pts',(-43.5499633272225,-52.4644105712997,
-171.592966290451));
#150869=CARTESIAN_POINT('Ctrl Pts',(-43.7274774238083,-52.5215797867686,
-171.638576841342));
#150870=CARTESIAN_POINT('Ctrl Pts',(-43.8177416070106,-52.5505863340359,
-171.64995));
#150871=CARTESIAN_POINT('Ctrl Pts',(-43.9094855672884,-52.58000002,-171.64995));
#150872=CARTESIAN_POINT('Ctrl Pts',(-42.9629113790828,-52.2741145284007,
-171.07256826174));
#150873=CARTESIAN_POINT('Ctrl Pts',(-42.4360603595898,-53.08000002,-171.405549026075));
#150874=CARTESIAN_POINT('Ctrl Pts',(-43.2972503047852,-53.08000002,-170.861259130871));
#150875=CARTESIAN_POINT('Ctrl Pts',(-42.2277314430405,-52.2712772274341,
-169.905239816447));
#150876=CARTESIAN_POINT('Ctrl Pts',(-41.6869083931944,-53.0800000201158,
-170.237641125793));
#150877=CARTESIAN_POINT('Ctrl Pts',(-42.5594745131554,-53.08000002,-169.693930655453));
#150878=CARTESIAN_POINT('Ctrl Pts',(-41.4865768015737,-52.2683704772926,
-168.741816047102));
#150879=CARTESIAN_POINT('Ctrl Pts',(-40.9363322060061,-53.08000002,-169.082082669019));
#150880=CARTESIAN_POINT('Ctrl Pts',(-41.8155944388483,-53.08000002,-168.530506878352));
#150881=CARTESIAN_POINT('Ctrl Pts',(-40.738568473807,-52.2653905871942,
-167.582872774143));
#150882=CARTESIAN_POINT('Ctrl Pts',(-40.1851006582006,-53.0800000199999,
-167.941466238826));
#150883=CARTESIAN_POINT('Ctrl Pts',(-41.0647116264263,-53.08000002,-167.371563643272));
#150884=CARTESIAN_POINT('',(-40.7385684496897,-52.2653907651306,-167.582872680651));
#150885=CARTESIAN_POINT('Origin',(-41.0647116264263,-52.58000002,-167.371563643272));
#150886=CARTESIAN_POINT('Ctrl Pts',(-40.738568473807,-52.2653905871942,
-167.582872774143));
#150887=CARTESIAN_POINT('Ctrl Pts',(-41.4866208523709,-52.2683706527206,
-168.741884298091));
#150888=CARTESIAN_POINT('Ctrl Pts',(-42.2277810204719,-52.2712774187735,
-169.905318536155));
#150889=CARTESIAN_POINT('Ctrl Pts',(-42.9629113790828,-52.2741145284007,
-171.07256826174));
#150890=CARTESIAN_POINT('Ctrl Pts',(-39.5145387173472,-53.08000002,-160.691745630313));
#150891=CARTESIAN_POINT('Ctrl Pts',(-39.046518301009,-53.0800000200001,
-160.669925623174));
#150892=CARTESIAN_POINT('Ctrl Pts',(-39.0160991280449,-52.6123983573548,
-160.668484445457));
#150893=CARTESIAN_POINT('Ctrl Pts',(-39.4806000144733,-53.08000002,-161.437914207565));
#150894=CARTESIAN_POINT('Ctrl Pts',(-38.9718867651858,-53.0800000199999,
-161.469235957258));
#150895=CARTESIAN_POINT('Ctrl Pts',(-38.9784549947027,-52.5734683914883,
-161.44194359172));
#150896=CARTESIAN_POINT('Ctrl Pts',(-39.5061329414855,-53.08000002,-162.175995192901));
#150897=CARTESIAN_POINT('Ctrl Pts',(-38.9628527118104,-53.08000002,-162.240077797041));
#150898=CARTESIAN_POINT('Ctrl Pts',(-39.0068863115613,-52.534969993258,
-162.206646800233));
#150899=CARTESIAN_POINT('Ctrl Pts',(-39.650908257113,-53.08000002,-163.427315362947));
#150900=CARTESIAN_POINT('Ctrl Pts',(-39.0343477235682,-53.0800000199999,
-163.540394308862));
#150901=CARTESIAN_POINT('Ctrl Pts',(-39.1678790396063,-52.4697392824198,
-163.502497688872));
#150902=CARTESIAN_POINT('Ctrl Pts',(-39.7412068397501,-53.08000002,-163.944571422167));
#150903=CARTESIAN_POINT('Ctrl Pts',(-39.0953266270306,-53.08000002,-164.09147487193));
#150904=CARTESIAN_POINT('Ctrl Pts',(-39.2682617425407,-52.4427876651683,
-164.03795625844));
#150905=CARTESIAN_POINT('Ctrl Pts',(-39.9897001844459,-53.08000002,-164.969734884811));
#150906=CARTESIAN_POINT('Ctrl Pts',(-39.2768635558283,-53.0800000199999,
-165.197823788181));
#150907=CARTESIAN_POINT('Ctrl Pts',(-39.5444749164239,-52.3894029704394,
-165.098845393713));
#150908=CARTESIAN_POINT('Ctrl Pts',(-40.1483999357838,-53.08000002,-165.477859388262));
#150909=CARTESIAN_POINT('Ctrl Pts',(-39.4036485964169,-53.08000002,-165.757191206274));
#150910=CARTESIAN_POINT('Ctrl Pts',(-39.7208567629119,-52.362959099468,
-165.624494361306));
#150911=CARTESIAN_POINT('Ctrl Pts',(-40.6198461801496,-53.08000002,-166.648725872017));
#150912=CARTESIAN_POINT('Ctrl Pts',(-39.8000071452162,-53.08000002,-167.111931394921));
#150913=CARTESIAN_POINT('Ctrl Pts',(-40.2447869076871,-52.3020702250487,
-166.835340537707));
#150914=CARTESIAN_POINT('Ctrl Pts',(-40.9685974766509,-53.08000002,-167.299349676832));
#150915=CARTESIAN_POINT('Ctrl Pts',(-40.1181633100728,-53.0800000199999,
-167.894540549612));
#150916=CARTESIAN_POINT('Ctrl Pts',(-40.6323757317604,-52.2682680312788,
-167.507958491073));
#150917=CARTESIAN_POINT('Ctrl Pts',(-41.4396558833968,-53.08000002,-167.895156212719));
#150918=CARTESIAN_POINT('Ctrl Pts',(-40.5374626513414,-53.0800000200001,
-168.618271993387));
#150919=CARTESIAN_POINT('Ctrl Pts',(-41.1557083615592,-52.2373619998033,
-168.123490399267));
#150920=CARTESIAN_POINT('',(-39.0000000106387,-52.5800000199908,-161.329336741014));
#150921=CARTESIAN_POINT('Origin',(-39.5,-52.58000002,-161.329336741016));
#150922=CARTESIAN_POINT('Ctrl Pts',(-39.0000000425548,-52.580000019989,
-161.329336741012));
#150923=CARTESIAN_POINT('Ctrl Pts',(-39.0000143473941,-52.5710036001899,
-161.508212762828));
#150924=CARTESIAN_POINT('Ctrl Pts',(-39.0036315660785,-52.5620200854199,
-161.686619320982));
#150925=CARTESIAN_POINT('Ctrl Pts',(-39.0107951000132,-52.5530670619587,
-161.86454449438));
#150926=CARTESIAN_POINT('Ctrl Pts',(-39.0182046362212,-52.5438065835258,
-162.048579780123));
#150927=CARTESIAN_POINT('Ctrl Pts',(-39.029407468258,-52.5345779583329,
-162.232100602006));
#150928=CARTESIAN_POINT('Ctrl Pts',(-39.044392703487,-52.5253784540501,
-162.415108947356));
#150929=CARTESIAN_POINT('Ctrl Pts',(-39.0593779387159,-52.5161789497673,
-162.598117292706));
#150930=CARTESIAN_POINT('Ctrl Pts',(-39.078145305281,-52.5070075369497,
-162.780613878806));
#150931=CARTESIAN_POINT('Ctrl Pts',(-39.1007423131417,-52.4978535392319,
-162.962605828642));
#150932=CARTESIAN_POINT('Ctrl Pts',(-39.1217650408907,-52.4893372788923,
-163.131918829615));
#150933=CARTESIAN_POINT('Ctrl Pts',(-39.1460968222467,-52.4808601821505,
-163.300781307826));
#150934=CARTESIAN_POINT('Ctrl Pts',(-39.1738223729434,-52.4723997023487,
-163.469192662811));
#150935=CARTESIAN_POINT('Ctrl Pts',(-39.2011086577874,-52.4640732649655,
-163.634935816242));
#150936=CARTESIAN_POINT('Ctrl Pts',(-39.2316823007795,-52.4557621613023,
-163.800242538063));
#150937=CARTESIAN_POINT('Ctrl Pts',(-39.2656696239975,-52.447461845679,
-163.965100428973));
#150938=CARTESIAN_POINT('Ctrl Pts',(-39.2987592557448,-52.4393807624587,
-164.125604004552));
#150939=CARTESIAN_POINT('Ctrl Pts',(-39.3350850983342,-52.4313092877518,
-164.285682551043));
#150940=CARTESIAN_POINT('Ctrl Pts',(-39.3748016229351,-52.423269407278,
-164.445306693126));
#150941=CARTESIAN_POINT('Ctrl Pts',(-39.3850253517464,-52.4211998012773,
-164.486396742086));
#150942=CARTESIAN_POINT('Ctrl Pts',(-39.3954739382909,-52.4191324533597,
-164.527456568598));
#150943=CARTESIAN_POINT('Ctrl Pts',(-39.4061503736799,-52.4170681050358,
-164.568485422985));
#150944=CARTESIAN_POINT('Ctrl Pts',(-39.4495891091557,-52.4086689832778,
-164.735417689015));
#150945=CARTESIAN_POINT('Ctrl Pts',(-39.4968013767408,-52.4003263288354,
-164.901856686214));
#150946=CARTESIAN_POINT('Ctrl Pts',(-39.5479233092373,-52.3920184089943,
-165.067322106566));
#150947=CARTESIAN_POINT('Ctrl Pts',(-39.5979804671909,-52.3838835276343,
-165.229341190702));
#150948=CARTESIAN_POINT('Ctrl Pts',(-39.6517867720346,-52.3757819588673,
-165.390426824107));
#150949=CARTESIAN_POINT('Ctrl Pts',(-39.7094542224162,-52.3677335878383,
-165.550104007737));
#150950=CARTESIAN_POINT('Ctrl Pts',(-39.7655755217695,-52.3599010057347,
-165.705500006053));
#150951=CARTESIAN_POINT('Ctrl Pts',(-39.8253542902578,-52.3521189747995,
-165.85956196005));
#150952=CARTESIAN_POINT('Ctrl Pts',(-39.8888695985127,-52.344443005944,
-166.011829898773));
#150953=CARTESIAN_POINT('Ctrl Pts',(-39.905244671204,-52.3424640413221,
-166.051086554116));
#150954=CARTESIAN_POINT('Ctrl Pts',(-39.9218679486955,-52.340492315133,
-166.090223853525));
#150955=CARTESIAN_POINT('Ctrl Pts',(-39.9387404404432,-52.3385291686761,
-166.129233683518));
#150956=CARTESIAN_POINT('Ctrl Pts',(-39.9865386305692,-52.3329677584828,
-166.23974488119));
#150957=CARTESIAN_POINT('Ctrl Pts',(-40.0363615889745,-52.3275249298668,
-166.349379781195));
#150958=CARTESIAN_POINT('Ctrl Pts',(-40.0883918199408,-52.3221245794599,
-166.458102843919));
#150959=CARTESIAN_POINT('Ctrl Pts',(-40.1391791878068,-52.3168532289849,
-166.564228803376));
#150960=CARTESIAN_POINT('Ctrl Pts',(-40.1920702020519,-52.3116221321699,
-166.669486100781));
#150961=CARTESIAN_POINT('Ctrl Pts',(-40.2472524480337,-52.3063985864397,
-166.773815992306));
#150962=CARTESIAN_POINT('Ctrl Pts',(-40.3015855872307,-52.3012554170705,
-166.87654052658));
#150963=CARTESIAN_POINT('Ctrl Pts',(-40.358140555795,-52.2961193585579,
-166.978366102817));
#150964=CARTESIAN_POINT('Ctrl Pts',(-40.4171056645871,-52.2909997877437,
-167.079209477833));
#150965=CARTESIAN_POINT('Ctrl Pts',(-40.4746249147384,-52.2860057517729,
-167.17758011485));
#150966=CARTESIAN_POINT('Ctrl Pts',(-40.5344381405214,-52.2810273360842,
-167.275016162333));
#150967=CARTESIAN_POINT('Ctrl Pts',(-40.5967205896074,-52.2761141036865,
-167.371413190652));
#150968=CARTESIAN_POINT('Ctrl Pts',(-40.6426385298221,-52.2724918069592,
-167.442482216489));
#150969=CARTESIAN_POINT('Ctrl Pts',(-40.6898986641975,-52.2689057716457,
-167.512985937728));
#150970=CARTESIAN_POINT('Ctrl Pts',(-40.7385684573717,-52.2653908962638,
-167.582872566557));
#150971=CARTESIAN_POINT('Origin',(-39.5,-52.58000002,-55.2499500000008));
#150972=CARTESIAN_POINT('',(-39.0000000110462,-52.5800000200017,-70.7293062304698));
#150973=CARTESIAN_POINT('Origin',(-39.5,-52.58000002,-70.7293062304687));
#150974=CARTESIAN_POINT('',(-39.,-52.58000002,-129.34995));
#150975=CARTESIAN_POINT('Ctrl Pts',(-41.4399683837798,-53.08000002,-64.1630432687404));
#150976=CARTESIAN_POINT('Ctrl Pts',(-40.5377494244216,-53.08000002,-63.4397598124973));
#150977=CARTESIAN_POINT('Ctrl Pts',(-41.1560619801497,-52.2373289603819,
-63.9347016803424));
#150978=CARTESIAN_POINT('Ctrl Pts',(-40.9682919256936,-53.08000002,-64.7596776730624));
#150979=CARTESIAN_POINT('Ctrl Pts',(-40.1178821818991,-53.08000002,-64.1644517527562));
#150980=CARTESIAN_POINT('Ctrl Pts',(-40.6320437640006,-52.2682772301857,
-64.5510855653446));
#150981=CARTESIAN_POINT('Ctrl Pts',(-40.6198991642287,-53.08000002,-65.4100287027235));
#150982=CARTESIAN_POINT('Ctrl Pts',(-39.7999900770068,-53.0800000199999,
-64.9469795070795));
#150983=CARTESIAN_POINT('Ctrl Pts',(-40.2448521881318,-52.3020649540327,
-65.2234219261584));
#150984=CARTESIAN_POINT('Ctrl Pts',(-40.2472081238925,-53.08000002,-66.3353006309098));
#150985=CARTESIAN_POINT('Ctrl Pts',(-39.4791379317096,-53.0800000199999,
-66.0432454126586));
#150986=CARTESIAN_POINT('Ctrl Pts',(-39.830683046914,-52.3501802308807,
-66.1802561999853));
#150987=CARTESIAN_POINT('Ctrl Pts',(-40.158849529204,-53.08000002,-66.5829654036754));
#150988=CARTESIAN_POINT('Ctrl Pts',(-39.4079361487702,-53.0800000199999,
-66.3190163717637));
#150989=CARTESIAN_POINT('Ctrl Pts',(-39.7324818893101,-52.3630645171375,
-66.4364231780381));
#150990=CARTESIAN_POINT('Ctrl Pts',(-39.9995673126391,-53.08000002,-67.0857801567948));
#150991=CARTESIAN_POINT('Ctrl Pts',(-39.283551683371,-53.0800000199999,
-66.871958046892));
#150992=CARTESIAN_POINT('Ctrl Pts',(-39.5554484391419,-52.3892314658149,
-66.9565858557632));
#150993=CARTESIAN_POINT('Ctrl Pts',(-39.9284899861158,-53.08000002,-67.341717845364));
#150994=CARTESIAN_POINT('Ctrl Pts',(-39.2293907876001,-53.08000002,-67.1504035968485));
#150995=CARTESIAN_POINT('Ctrl Pts',(-39.4764466553468,-52.4025551469199,
-67.2213966334271));
#150996=CARTESIAN_POINT('Ctrl Pts',(-39.7415458247801,-53.08000002,-68.1121058873989));
#150997=CARTESIAN_POINT('Ctrl Pts',(-39.0955485045717,-53.08000002,-67.9649896902694));
#150998=CARTESIAN_POINT('Ctrl Pts',(-39.2686417135216,-52.4426736449394,
-68.0186529598151));
#150999=CARTESIAN_POINT('Ctrl Pts',(-39.6510782949347,-53.08000002,-68.6301060216833));
#151000=CARTESIAN_POINT('Ctrl Pts',(-39.0344334320403,-53.08000002,-68.5169196669116));
#151001=CARTESIAN_POINT('Ctrl Pts',(-39.1680706108451,-52.4696640994698,
-68.554881198313));
#151002=CARTESIAN_POINT('Ctrl Pts',(-39.5060965949729,-53.08000002,-69.8826150276831));
#151003=CARTESIAN_POINT('Ctrl Pts',(-38.9628098506121,-53.0800000199999,
-69.8184703936588));
#151004=CARTESIAN_POINT('Ctrl Pts',(-39.0068468087641,-52.5349571571294,
-69.8519627949666));
#151005=CARTESIAN_POINT('Ctrl Pts',(-39.4806156445371,-53.08000002,-70.6208998773124));
#151006=CARTESIAN_POINT('Ctrl Pts',(-38.9718949651596,-53.0800000199999,
-70.5896094886226));
#151007=CARTESIAN_POINT('Ctrl Pts',(-38.9784724981306,-52.5734665632027,
-70.6168773255623));
#151008=CARTESIAN_POINT('Ctrl Pts',(-39.5145320287584,-53.08000002,-71.3667542047957));
#151009=CARTESIAN_POINT('Ctrl Pts',(-39.0464983325853,-53.0800000199999,
-71.3885691567561));
#151010=CARTESIAN_POINT('Ctrl Pts',(-39.0160910311445,-52.6123805775276,
-71.3900101945721));
#151011=CARTESIAN_POINT('',(-40.7385684498172,-52.2653907681885,-64.4757702925262));
#151012=CARTESIAN_POINT('Origin',(-41.0647116264214,-52.58000002,-64.687079328241));
#151013=CARTESIAN_POINT('Ctrl Pts',(-40.7385684580933,-52.265390901695,
-64.4757704085913));
#151014=CARTESIAN_POINT('Ctrl Pts',(-40.6731577382874,-52.2701147931979,
-64.5696959221107));
#151015=CARTESIAN_POINT('Ctrl Pts',(-40.6103086685504,-52.2749654591829,
-64.6647119718094));
#151016=CARTESIAN_POINT('Ctrl Pts',(-40.5498529666727,-52.2798625896157,
-64.7606962119301));
#151017=CARTESIAN_POINT('Ctrl Pts',(-40.4876384745571,-52.2849021884166,
-64.859472846139));
#151018=CARTESIAN_POINT('Ctrl Pts',(-40.4279579901574,-52.2899909785542,
-64.959274801201));
#151019=CARTESIAN_POINT('Ctrl Pts',(-40.3706215165111,-52.2950875642308,
-65.0599992822958));
#151020=CARTESIAN_POINT('Ctrl Pts',(-40.3124161847234,-52.3002613818974,
-65.1622501091852));
#151021=CARTESIAN_POINT('Ctrl Pts',(-40.2566258082699,-52.3054434096775,
-65.26545173734));
#151022=CARTESIAN_POINT('Ctrl Pts',(-40.2030547740074,-52.3106358110184,
-65.369526925024));
#151023=CARTESIAN_POINT('Ctrl Pts',(-40.1482748098001,-52.3159453885452,
-65.4759507627318));
#151024=CARTESIAN_POINT('Ctrl Pts',(-40.0958148612012,-52.3212660160675,
-65.5832881526308));
#151025=CARTESIAN_POINT('Ctrl Pts',(-40.0454787270805,-52.3266443567245,
-65.6914862715604));
#151026=CARTESIAN_POINT('Ctrl Pts',(-40.0089709584569,-52.3305451572074,
-65.7699601543962));
#151027=CARTESIAN_POINT('Ctrl Pts',(-39.9735806395691,-52.3344772730378,
-65.8488874483287));
#151028=CARTESIAN_POINT('Ctrl Pts',(-39.9392396956596,-52.3384715084012,
-65.9282567948704));
#151029=CARTESIAN_POINT('Ctrl Pts',(-39.8822675889028,-52.3450980007926,
-66.0599316520412));
#151030=CARTESIAN_POINT('Ctrl Pts',(-39.8282521243597,-52.35179330575,-66.1928019679309));
#151031=CARTESIAN_POINT('Ctrl Pts',(-39.7770250192551,-52.3585357064663,
-66.326792421969));
#151032=CARTESIAN_POINT('Ctrl Pts',(-39.7302756747203,-52.3646887540264,
-66.4490707722176));
#151033=CARTESIAN_POINT('Ctrl Pts',(-39.6858483481945,-52.3708818419249,
-66.5722825351572));
#151034=CARTESIAN_POINT('Ctrl Pts',(-39.643630310403,-52.3771272309155,
-66.6963898596616));
#151035=CARTESIAN_POINT('Ctrl Pts',(-39.5964607848755,-52.3841051022434,
-66.8350529505487));
#151036=CARTESIAN_POINT('Ctrl Pts',(-39.5519844690044,-52.3911513115055,
-66.9750591381598));
#151037=CARTESIAN_POINT('Ctrl Pts',(-39.5102573480315,-52.3982348943555,
-67.1158335539574));
#151038=CARTESIAN_POINT('Ctrl Pts',(-39.4737134245086,-52.404438579247,
-67.2391214627551));
#151039=CARTESIAN_POINT('Ctrl Pts',(-39.4392772647425,-52.4106706781818,
-67.3629983817228));
#151040=CARTESIAN_POINT('Ctrl Pts',(-39.4069537833937,-52.4169136927106,
-67.4870781002419));
#151041=CARTESIAN_POINT('Ctrl Pts',(-39.3653073114868,-52.4249573661746,
-67.6469458587845));
#151042=CARTESIAN_POINT('Ctrl Pts',(-39.3271258249076,-52.4330430184609,
-67.8072556992434));
#151043=CARTESIAN_POINT('Ctrl Pts',(-39.2922411274965,-52.4411393696389,
-67.9679723407774));
#151044=CARTESIAN_POINT('Ctrl Pts',(-39.2567093388435,-52.4493859035137,
-68.1316701843534));
#151045=CARTESIAN_POINT('Ctrl Pts',(-39.2245972902298,-52.4576442124894,
-68.2957905034026));
#151046=CARTESIAN_POINT('Ctrl Pts',(-39.1957663841659,-52.4659126791799,
-68.4603174774834));
#151047=CARTESIAN_POINT('Ctrl Pts',(-39.1662932678576,-52.4743653264855,
-68.6285093002511));
#151048=CARTESIAN_POINT('Ctrl Pts',(-39.1402487174386,-52.4828293495748,
-68.7971266032564));
#151049=CARTESIAN_POINT('Ctrl Pts',(-39.1175319575409,-52.4913245467436,
-68.9661674216048));
#151050=CARTESIAN_POINT('Ctrl Pts',(-39.1117517651853,-52.4934861170537,
-69.0091792089545));
#151051=CARTESIAN_POINT('Ctrl Pts',(-39.1061872722816,-52.4956497790532,
-69.0522184676471));
#151052=CARTESIAN_POINT('Ctrl Pts',(-39.1008373305186,-52.4978159816229,
-69.0952852526225));
#151053=CARTESIAN_POINT('Ctrl Pts',(-39.0789398766013,-52.5066823063506,
-69.2715587488873));
#151054=CARTESIAN_POINT('Ctrl Pts',(-39.060639025291,-52.5155639508941,
-69.4482775535725));
#151055=CARTESIAN_POINT('Ctrl Pts',(-39.0458873913583,-52.5244699995587,
-69.6254473411904));
#151056=CARTESIAN_POINT('Ctrl Pts',(-39.0306492988374,-52.5336697393413,
-69.8084595843056));
#151057=CARTESIAN_POINT('Ctrl Pts',(-39.019198308061,-52.5428965372875,
-69.9919537511656));
#151058=CARTESIAN_POINT('Ctrl Pts',(-39.0115396379574,-52.5521535968908,
-70.1759317271015));
#151059=CARTESIAN_POINT('Ctrl Pts',(-39.0038809678538,-52.561410656494,
-70.3599097030374));
#151060=CARTESIAN_POINT('Ctrl Pts',(-39.0000151139767,-52.5706989155813,
-70.5443721556157));
#151061=CARTESIAN_POINT('Ctrl Pts',(-39.0000000441847,-52.5800000200048,
-70.729306230472));
#151062=CARTESIAN_POINT('Ctrl Pts',(-40.7385684738022,-52.2653905871942,
-64.4757701973706));
#151063=CARTESIAN_POINT('Ctrl Pts',(-40.1851006581956,-53.08000002,-64.1171767326871));
#151064=CARTESIAN_POINT('Ctrl Pts',(-41.0647116264215,-53.08000002,-64.6870793282409));
#151065=CARTESIAN_POINT('Ctrl Pts',(-41.4350320326697,-52.2681651349568,
-63.3966889540178));
#151066=CARTESIAN_POINT('Ctrl Pts',(-40.8849497704992,-53.0800000200001,
-63.0545757298723));
#151067=CARTESIAN_POINT('Ctrl Pts',(-41.7638515954828,-53.08000002,-63.6079981134234));
#151068=CARTESIAN_POINT('Ctrl Pts',(-42.125553749702,-52.2708762823431,
-62.3137201227713));
#151069=CARTESIAN_POINT('Ctrl Pts',(-41.584202382955,-53.08000002,-61.9790488279059));
#151070=CARTESIAN_POINT('Ctrl Pts',(-42.4569204735311,-53.08000002,-62.5250292766735));
#151071=CARTESIAN_POINT('Ctrl Pts',(-42.8108476403353,-52.2735270043159,
-61.2273317382593));
#151072=CARTESIAN_POINT('Ctrl Pts',(-42.2822348911901,-53.08000002,-60.8926985768511));
#151073=CARTESIAN_POINT('Ctrl Pts',(-43.1446480925044,-53.08000002,-61.4386408691297));
#151074=CARTESIAN_POINT('',(-42.8108476403353,-52.2735270043159,-61.2273317382593));
#151075=CARTESIAN_POINT('Origin',(-43.1446480925044,-52.58000002,-61.4386408691297));
#151076=CARTESIAN_POINT('Ctrl Pts',(-42.8108476403353,-52.2735270043159,
-61.2273317382593));
#151077=CARTESIAN_POINT('Ctrl Pts',(-42.1255968220058,-52.2708764489536,
-62.3136518407425));
#151078=CARTESIAN_POINT('Ctrl Pts',(-41.4350707133446,-52.2681652890367,
-63.3966290232794));
#151079=CARTESIAN_POINT('Ctrl Pts',(-40.7385684738071,-52.2653905871969,
-64.475770197359));
#151080=CARTESIAN_POINT('Ctrl Pts',(-43.7578534463097,-53.08000002,-61.14995));
#151081=CARTESIAN_POINT('Ctrl Pts',(-43.7578534463096,-53.0800000199999,
-60.64995));
#151082=CARTESIAN_POINT('Ctrl Pts',(-43.7578534463097,-52.58000002,-60.64995));
#151083=CARTESIAN_POINT('Ctrl Pts',(-43.6407450400032,-53.08000002,-61.1499500212049));
#151084=CARTESIAN_POINT('Ctrl Pts',(-43.5651337625656,-53.08000002,-60.5880729855648));
#151085=CARTESIAN_POINT('Ctrl Pts',(-43.5763740160895,-52.5217319642193,
-60.64995));
#151086=CARTESIAN_POINT('Ctrl Pts',(-43.5216142225441,-53.08000002,-61.1725879738646));
#151087=CARTESIAN_POINT('Ctrl Pts',(-43.3529851647999,-53.0800000199999,
-60.5541186415154));
#151088=CARTESIAN_POINT('Ctrl Pts',(-43.3921532801741,-52.4622997588847,
-60.6952259861921));
#151089=CARTESIAN_POINT('Ctrl Pts',(-43.3605400154948,-53.08000002,-61.2428714356874));
#151090=CARTESIAN_POINT('Ctrl Pts',(-43.0017618884342,-53.08000002,-60.5701748148313));
#151091=CARTESIAN_POINT('Ctrl Pts',(-43.1434985367023,-52.3817526273734,
-60.8357928521433));
#151092=CARTESIAN_POINT('Ctrl Pts',(-43.3089610591665,-53.08000002,-61.2727843293231));
#151093=CARTESIAN_POINT('Ctrl Pts',(-42.8669014498658,-53.0800000199996,
-60.5905012094869));
#151094=CARTESIAN_POINT('Ctrl Pts',(-43.0639517713831,-52.3559271119108,
-60.8956186757958));
#151095=CARTESIAN_POINT('Ctrl Pts',(-43.2167397054761,-53.08000002,-61.3458748887128));
#151096=CARTESIAN_POINT('Ctrl Pts',(-42.577778492926,-53.0800000200004,
-60.6851892310921));
#151097=CARTESIAN_POINT('Ctrl Pts',(-42.9218280041301,-52.3097083637374,
-61.0417997602761));
#151098=CARTESIAN_POINT('Ctrl Pts',(-43.1765485703954,-53.08000002,-61.3882486178711));
#151099=CARTESIAN_POINT('Ctrl Pts',(-42.4244093202802,-53.0800000199984,
-60.7623557509217));
#151100=CARTESIAN_POINT('Ctrl Pts',(-42.8599235980017,-52.2895352828276,
-61.126589843371));
#151101=CARTESIAN_POINT('Ctrl Pts',(-43.1446480925044,-53.08000002,-61.4386408691297));
#151102=CARTESIAN_POINT('Ctrl Pts',(-42.2822348911901,-53.08000002,-60.8926985768511));
#151103=CARTESIAN_POINT('Ctrl Pts',(-42.8108476403352,-52.2735270043159,
-61.2273317382593));
#151104=CARTESIAN_POINT('Origin',(-43.7578534463097,-52.58000002,-61.14995));
#151105=CARTESIAN_POINT('Ctrl Pts',(-43.7578534463097,-52.58000002,-60.64995));
#151106=CARTESIAN_POINT('Ctrl Pts',(-43.5763740160895,-52.5217319642193,
-60.64995));
#151107=CARTESIAN_POINT('Ctrl Pts',(-43.3921532801741,-52.4622997588847,
-60.6952259861921));
#151108=CARTESIAN_POINT('Ctrl Pts',(-43.1434985367023,-52.3817526273734,
-60.8357928521433));
#151109=CARTESIAN_POINT('Ctrl Pts',(-43.0639517713831,-52.3559271119108,
-60.8956186757958));
#151110=CARTESIAN_POINT('Ctrl Pts',(-42.9218280041301,-52.3097083637374,
-61.0417997602761));
#151111=CARTESIAN_POINT('Ctrl Pts',(-42.8599235980017,-52.2895352828276,
-61.126589843371));
#151112=CARTESIAN_POINT('Ctrl Pts',(-42.8108476403353,-52.2735270043159,
-61.2273317382593));
#151113=CARTESIAN_POINT('Origin',(1.65582490824295E-14,-52.58000002,-61.14995));
#151114=CARTESIAN_POINT('Origin',(-59.5,-53.58000002,-55.2499500000008));
#151115=CARTESIAN_POINT('',(-60.,-53.58000002,-174.34995));
#151116=CARTESIAN_POINT('Origin',(-59.5,-53.58000002,-174.34995));
#151117=CARTESIAN_POINT('',(-60.,-53.58000002,-58.24995));
#151118=CARTESIAN_POINT('Origin',(-57.,-53.58000002,-174.34995));
#151119=CARTESIAN_POINT('Origin',(-57.,-53.58000002,-174.34995));
#151120=CARTESIAN_POINT('Origin',(0.,-12.9675000200281,-61.64995));
#151121=CARTESIAN_POINT('',(-47.3503956976423,-46.6672397853475,-61.2273317382593));
#151122=CARTESIAN_POINT('Origin',(0.,-12.9675000200281,-61.2273317382593));
#151123=CARTESIAN_POINT('Ctrl Pts',(-47.3503956976423,-46.6672397853475,
-61.2273317382593));
#151124=CARTESIAN_POINT('Ctrl Pts',(-47.4408676817955,-46.6931677917013,
-61.0370194599865));
#151125=CARTESIAN_POINT('Ctrl Pts',(-47.5839744124439,-46.7341093359256,
-60.8908220076151));
#151126=CARTESIAN_POINT('Ctrl Pts',(-47.9099463828816,-46.8268793795224,
-60.6975716107228));
#151127=CARTESIAN_POINT('Ctrl Pts',(-48.0917170178641,-46.8783971335546,
-60.64995));
#151128=CARTESIAN_POINT('Ctrl Pts',(-48.2747189347426,-46.93000002,-60.64995));
#151129=CARTESIAN_POINT('Origin',(83.2809572255632,-46.9300000199999,-61.14995));
#151130=CARTESIAN_POINT('Origin',(-48.2747189347426,-46.93000002,-61.14995));
#151131=CARTESIAN_POINT('Ctrl Pts',(-47.7195914591242,-46.43000002,-61.4386408691297));
#151132=CARTESIAN_POINT('Ctrl Pts',(-47.4775784747621,-46.4300000199999,
-61.3001247789676));
#151133=CARTESIAN_POINT('Ctrl Pts',(-47.3503956976423,-46.6672397853475,
-61.2273317382593));
#151134=CARTESIAN_POINT('Ctrl Pts',(-47.7740598678193,-46.43000002,-61.3434749301835));
#151135=CARTESIAN_POINT('Ctrl Pts',(-47.5485238823607,-46.43000002,-61.1353180501949));
#151136=CARTESIAN_POINT('Ctrl Pts',(-47.4408676817955,-46.6931677917013,
-61.0370194599865));
#151137=CARTESIAN_POINT('Ctrl Pts',(-47.8601584717208,-46.43000002,-61.2703860128396));
#151138=CARTESIAN_POINT('Ctrl Pts',(-47.6638566779936,-46.43000002,-60.997955986762));
#151139=CARTESIAN_POINT('Ctrl Pts',(-47.5839744124439,-46.7341093359256,
-60.8908220076151));
#151140=CARTESIAN_POINT('Ctrl Pts',(-48.0559929527306,-46.43000002,-61.1737607963294));
#151141=CARTESIAN_POINT('Ctrl Pts',(-47.9370084437089,-46.4300000199999,
-60.7796218648572));
#151142=CARTESIAN_POINT('Ctrl Pts',(-47.9099463828816,-46.8268793795224,
-60.6975716107228));
#151143=CARTESIAN_POINT('Ctrl Pts',(-48.1650685977726,-46.43000002,-61.1499500105546));
#151144=CARTESIAN_POINT('Ctrl Pts',(-48.1007647709628,-46.43000002,-60.6990016989097));
#151145=CARTESIAN_POINT('Ctrl Pts',(-48.0917170178641,-46.8783971335546,
-60.64995));
#151146=CARTESIAN_POINT('Ctrl Pts',(-48.2747189347426,-46.43000002,-61.14995));
#151147=CARTESIAN_POINT('Ctrl Pts',(-48.2747189347426,-46.43000002,-60.64995));
#151148=CARTESIAN_POINT('Ctrl Pts',(-48.2747189347426,-46.93000002,-60.64995));
#151149=CARTESIAN_POINT('Origin',(-47.7195914591242,-46.93000002,-61.4386408691297));
#151150=CARTESIAN_POINT('Ctrl Pts',(-47.3503956976423,-46.6672397853475,
-61.2273317382593));
#151151=CARTESIAN_POINT('Ctrl Pts',(-47.4775784747622,-46.43000002,-61.3001247789676));
#151152=CARTESIAN_POINT('Ctrl Pts',(-47.7195914591242,-46.43000002,-61.4386408691297));
#151153=CARTESIAN_POINT('Ctrl Pts',(-45.1164556950575,-46.6590534862623,
-65.1406137191269));
#151154=CARTESIAN_POINT('Ctrl Pts',(-45.2561496318399,-46.43000002,-65.1939977276857));
#151155=CARTESIAN_POINT('Ctrl Pts',(-45.4798241095785,-46.43000002,-65.3519247333759));
#151156=CARTESIAN_POINT('Ctrl Pts',(-42.8446532485491,-46.6501540216799,
-69.0311826437503));
#151157=CARTESIAN_POINT('Ctrl Pts',(-42.9872821964954,-46.43000002,-69.082946811334));
#151158=CARTESIAN_POINT('Ctrl Pts',(-43.2012981267977,-46.43000002,-69.2424952559608));
#151159=CARTESIAN_POINT('Ctrl Pts',(-40.5149864073608,-46.6403532458042,
-72.8868173744763));
#151160=CARTESIAN_POINT('Ctrl Pts',(-40.6428186202086,-46.43000002,-72.9643267243714));
#151161=CARTESIAN_POINT('Ctrl Pts',(-40.8634877666247,-46.43000002,-73.0981265053466));
#151162=CARTESIAN_POINT('',(-40.5149645407348,-46.6407620497281,-72.8871156726096));
#151163=CARTESIAN_POINT('Origin',(-40.8634877666247,-46.93000002,-73.0981265053466));
#151164=CARTESIAN_POINT('Ctrl Pts',(-40.5149864073608,-46.6403532458042,
-72.8868173744763));
#151165=CARTESIAN_POINT('Ctrl Pts',(-42.8446532485491,-46.6501540216799,
-69.0311826437503));
#151166=CARTESIAN_POINT('Ctrl Pts',(-45.1164556950575,-46.6590534862623,
-65.1406137191269));
#151167=CARTESIAN_POINT('Ctrl Pts',(-47.3503956976423,-46.6672397853475,
-61.2273317382593));
#151168=CARTESIAN_POINT('Ctrl Pts',(-39.5009150908472,-46.43000002,-78.6483012309456));
#151169=CARTESIAN_POINT('Ctrl Pts',(-38.9925996219358,-46.43000002,-78.6546392690997));
#151170=CARTESIAN_POINT('Ctrl Pts',(-39.0010185398262,-46.9382906476586,
-78.6545545088046));
#151171=CARTESIAN_POINT('Ctrl Pts',(-39.4889961719126,-46.43000002,-77.6521831848818));
#151172=CARTESIAN_POINT('Ctrl Pts',(-39.0322289013405,-46.43000002,-77.6697878581646));
#151173=CARTESIAN_POINT('Ctrl Pts',(-38.9877635814871,-46.8849139645486,
-77.6175842987478));
#151174=CARTESIAN_POINT('Ctrl Pts',(-39.5933371710426,-46.43000002,-76.6722018120623));
#151175=CARTESIAN_POINT('Ctrl Pts',(-39.1763256032396,-46.43000002,-76.6493249295432));
#151176=CARTESIAN_POINT('Ctrl Pts',(-39.1036909811623,-46.8323255651553,
-76.5984538753872));
#151177=CARTESIAN_POINT('Ctrl Pts',(-39.9334371785153,-46.43000002,-75.2543998581027));
#151178=CARTESIAN_POINT('Ctrl Pts',(-39.5965010051026,-46.4300000199999,
-75.16683002555));
#151179=CARTESIAN_POINT('Ctrl Pts',(-39.4815683506526,-46.7562077909153,
-75.125263078053));
#151180=CARTESIAN_POINT('Ctrl Pts',(-40.0729487155202,-46.43000002,-74.8007807728849));
#151181=CARTESIAN_POINT('Ctrl Pts',(-39.7579862728477,-46.43000002,-74.7028397032788));
#151182=CARTESIAN_POINT('Ctrl Pts',(-39.6365790276958,-46.7318484038351,
-74.6541180909925));
#151183=CARTESIAN_POINT('Ctrl Pts',(-40.4336795368199,-46.43000002,-73.8793270924814));
#151184=CARTESIAN_POINT('Ctrl Pts',(-40.1657218306395,-46.4300000199999,
-73.7660901072993));
#151185=CARTESIAN_POINT('Ctrl Pts',(-40.0373881727514,-46.6823634194217,
-73.6974136443781));
#151186=CARTESIAN_POINT('Ctrl Pts',(-40.6620683669064,-46.43000002,-73.411923037355));
#151187=CARTESIAN_POINT('Ctrl Pts',(-40.4182099778731,-46.4300000199999,
-73.2894241672258));
#151188=CARTESIAN_POINT('Ctrl Pts',(-40.2911698500431,-46.6572594632896,
-73.2123128660115));
#151189=CARTESIAN_POINT('Ctrl Pts',(-40.9442174875933,-46.43000002,-72.9681042608037));
#151190=CARTESIAN_POINT('Ctrl Pts',(-40.7310707477149,-46.43000002,-72.8323985218523));
#151191=CARTESIAN_POINT('Ctrl Pts',(-40.6046466716213,-46.6334277480432,
-72.7519083427877));
#151192=CARTESIAN_POINT('',(-39.,-46.93000002,-78.4955841262963));
#151193=CARTESIAN_POINT('Origin',(-39.5,-46.93000002,-78.4955841262963));
#151194=CARTESIAN_POINT('Ctrl Pts',(-39.,-46.93000002,-78.4955841262963));
#151195=CARTESIAN_POINT('Ctrl Pts',(-39.0000000114043,-46.9212366188075,
-78.325357772545));
#151196=CARTESIAN_POINT('Ctrl Pts',(-39.0036424523548,-46.9124870586774,
-78.1556109785247));
#151197=CARTESIAN_POINT('Ctrl Pts',(-39.0108614956953,-46.9037692487272,
-77.9863659895749));
#151198=CARTESIAN_POINT('Ctrl Pts',(-39.0181149087956,-46.8950099334112,
-77.8163152277052));
#151199=CARTESIAN_POINT('Ctrl Pts',(-39.0289785903128,-46.8862819126589,
-77.6467704601483));
#151200=CARTESIAN_POINT('Ctrl Pts',(-39.043431653744,-46.877583067065,-77.477738864482));
#151201=CARTESIAN_POINT('Ctrl Pts',(-39.0578119415107,-46.8689280228611,
-77.309558395414));
#151202=CARTESIAN_POINT('Ctrl Pts',(-39.0757453657993,-46.8603010136457,
-77.1418852932464));
#151203=CARTESIAN_POINT('Ctrl Pts',(-39.0972614984966,-46.851692008831,
-76.9747208445981));
#151204=CARTESIAN_POINT('Ctrl Pts',(-39.1185331932699,-46.8431808081755,
-76.809455497957));
#151205=CARTESIAN_POINT('Ctrl Pts',(-39.1433067271124,-46.8346863590143,
-76.6446866806331));
#151206=CARTESIAN_POINT('Ctrl Pts',(-39.1716605727341,-46.826203771819,
-76.4804194998339));
#151207=CARTESIAN_POINT('Ctrl Pts',(-39.1992826999361,-46.8179400919769,
-76.3203915084399));
#151208=CARTESIAN_POINT('Ctrl Pts',(-39.2303030938182,-46.8096869394463,
-76.1608390644509));
#151209=CARTESIAN_POINT('Ctrl Pts',(-39.264838514336,-46.8014558784949,
-76.001779067251));
#151210=CARTESIAN_POINT('Ctrl Pts',(-39.2940438168355,-46.7944951807135,
-75.8672680271612));
#151211=CARTESIAN_POINT('Ctrl Pts',(-39.3257637466383,-46.7875503001958,
-75.7331091835309));
#151212=CARTESIAN_POINT('Ctrl Pts',(-39.3600912437891,-46.7806433619661,
-75.5993240027414));
#151213=CARTESIAN_POINT('Ctrl Pts',(-39.4012359993546,-46.7723647425283,
-75.4389697963834));
#151214=CARTESIAN_POINT('Ctrl Pts',(-39.4461824058822,-46.7641247054021,
-75.2789598860371));
#151215=CARTESIAN_POINT('Ctrl Pts',(-39.4950323080936,-46.7559182016718,
-75.1198288925915));
#151216=CARTESIAN_POINT('Ctrl Pts',(-39.5428091296028,-46.7478919693522,
-74.9641935130659));
#151217=CARTESIAN_POINT('Ctrl Pts',(-39.5943203183166,-46.7398980605529,
-74.8093990261248));
#151218=CARTESIAN_POINT('Ctrl Pts',(-39.6496298273295,-46.7319643620929,
-74.6559650168446));
#151219=CARTESIAN_POINT('Ctrl Pts',(-39.7049393363425,-46.7240306636329,
-74.5025310075644));
#151220=CARTESIAN_POINT('Ctrl Pts',(-39.7640477566345,-46.7161574167842,
-74.3504576467527));
#151221=CARTESIAN_POINT('Ctrl Pts',(-39.8269791847324,-46.7084020374917,
-74.2002817725628));
#151222=CARTESIAN_POINT('Ctrl Pts',(-39.8745311201513,-46.7025419560283,
-74.0868066189424));
#151223=CARTESIAN_POINT('Ctrl Pts',(-39.9242976680265,-46.6967835306671,
-73.9742725680164));
#151224=CARTESIAN_POINT('Ctrl Pts',(-39.9764418349066,-46.6910703067992,
-73.8627159546544));
#151225=CARTESIAN_POINT('Ctrl Pts',(-40.0277693349268,-46.6854465617911,
-73.752906508705));
#151226=CARTESIAN_POINT('Ctrl Pts',(-40.0814011405111,-46.6798663222219,
-73.644043931816));
#151227=CARTESIAN_POINT('Ctrl Pts',(-40.1375110305611,-46.6743128514715,
-73.5361901580596));
#151228=CARTESIAN_POINT('Ctrl Pts',(-40.1949600591147,-46.6686268396217,
-73.4257623079495));
#151229=CARTESIAN_POINT('Ctrl Pts',(-40.2550075097591,-46.6629683413473,
-73.3163916130317));
#151230=CARTESIAN_POINT('Ctrl Pts',(-40.317850220895,-46.6573653423464,
-73.2081779482056));
#151231=CARTESIAN_POINT('Ctrl Pts',(-40.3769396861228,-46.6520969793389,
-73.1064272842168));
#151232=CARTESIAN_POINT('Ctrl Pts',(-40.438501162163,-46.6468778743449,
-73.005699727026));
#151233=CARTESIAN_POINT('Ctrl Pts',(-40.5026976064787,-46.6417729019327,
-72.9061082583841));
#151234=CARTESIAN_POINT('Ctrl Pts',(-40.5067752375929,-46.6414486441865,
-72.8997824053626));
#151235=CARTESIAN_POINT('Ctrl Pts',(-40.5108634973868,-46.641124861076,
-72.8934611460772));
#151236=CARTESIAN_POINT('Ctrl Pts',(-40.5149624265548,-46.6408015750335,
-72.8871445136361));
#151237=CARTESIAN_POINT('Origin',(-39.5,-46.93000002,-55.2499500000008));
#151238=CARTESIAN_POINT('',(-39.,-46.9300000199928,-153.563058845201));
#151239=CARTESIAN_POINT('Origin',(-39.5,-46.9300000199999,-153.563058845195));
#151240=CARTESIAN_POINT('',(-39.,-46.93000002,-129.34995));
#151241=CARTESIAN_POINT('Ctrl Pts',(-40.9139483721511,-46.43000002,-159.04250796345));
#151242=CARTESIAN_POINT('Ctrl Pts',(-40.6980070138923,-46.43000002,-159.177513727936));
#151243=CARTESIAN_POINT('Ctrl Pts',(-40.5710289585984,-46.6359863492877,
-159.256899712053));
#151244=CARTESIAN_POINT('Ctrl Pts',(-40.6453734355539,-46.43000002,-158.612545232755));
#151245=CARTESIAN_POINT('Ctrl Pts',(-40.4000491853353,-46.43000002,-158.734901860446));
#151246=CARTESIAN_POINT('Ctrl Pts',(-40.2726319701784,-46.6590723862912,
-158.810854977709));
#151247=CARTESIAN_POINT('Ctrl Pts',(-40.4272411167408,-46.43000002,-158.162404667172));
#151248=CARTESIAN_POINT('Ctrl Pts',(-40.1587308612842,-46.43000002,-158.276021182203));
#151249=CARTESIAN_POINT('Ctrl Pts',(-40.0302467855321,-46.6832471055803,
-158.343663631397));
#151250=CARTESIAN_POINT('Ctrl Pts',(-40.0748112905834,-46.43000002,-157.263052526127));
#151251=CARTESIAN_POINT('Ctrl Pts',(-39.7601657220121,-46.43000002,-157.361162449029));
#151252=CARTESIAN_POINT('Ctrl Pts',(-39.6386598952534,-46.7315414595573,
-157.409909939755));
#151253=CARTESIAN_POINT('Ctrl Pts',(-39.936491307137,-46.43000002,-156.81535457804));
#151254=CARTESIAN_POINT('Ctrl Pts',(-39.6001021971278,-46.43000002,-156.903067496752));
#151255=CARTESIAN_POINT('Ctrl Pts',(-39.484972353656,-46.7555812340755,
-156.944919216257));
#151256=CARTESIAN_POINT('Ctrl Pts',(-39.5977060048933,-46.43000002,-155.407958919601));
#151257=CARTESIAN_POINT('Ctrl Pts',(-39.18209163777,-46.43000002,-155.432505947607));
#151258=CARTESIAN_POINT('Ctrl Pts',(-39.1085513924158,-46.8311357158264,
-155.482548023534));
#151259=CARTESIAN_POINT('Ctrl Pts',(-39.4929946038571,-46.43000002,-154.44272705014));
#151260=CARTESIAN_POINT('Ctrl Pts',(-39.0379952988168,-46.4300000199999,
-154.42847000153));
#151261=CARTESIAN_POINT('Ctrl Pts',(-38.9922097725462,-46.8829301245063,
-154.478770282061));
#151262=CARTESIAN_POINT('Ctrl Pts',(-39.5003628921561,-46.43000002,-153.467040782265));
#151263=CARTESIAN_POINT('Ctrl Pts',(-38.9951403347308,-46.4300000199999,
-153.463084491498));
#151264=CARTESIAN_POINT('Ctrl Pts',(-39.0004039132295,-46.9352126230012,
-153.463110895003));
#151265=CARTESIAN_POINT('',(-40.5149651533753,-46.6407282068896,-159.171551992371));
#151266=CARTESIAN_POINT('Origin',(-40.8634877666247,-46.93000002,-158.96051646616));
#151267=CARTESIAN_POINT('Ctrl Pts',(-40.5149614839772,-46.640792942112,
-159.171504755847));
#151268=CARTESIAN_POINT('Ctrl Pts',(-40.4511923171114,-46.645823490987,
-159.07323460075));
#151269=CARTESIAN_POINT('Ctrl Pts',(-40.3900526489562,-46.6509693267882,
-158.973921789425));
#151270=CARTESIAN_POINT('Ctrl Pts',(-40.331374886992,-46.6561622609605,
-158.87367813627));
#151271=CARTESIAN_POINT('Ctrl Pts',(-40.2710812776531,-46.6614981963103,
-158.770674008987));
#151272=CARTESIAN_POINT('Ctrl Pts',(-40.2133863650166,-46.6668839079942,
-158.6666870514));
#151273=CARTESIAN_POINT('Ctrl Pts',(-40.1581069327706,-46.6722900646723,
-158.561806464956));
#151274=CARTESIAN_POINT('Ctrl Pts',(-40.1019927837822,-46.6777778540536,
-158.45534218675));
#151275=CARTESIAN_POINT('Ctrl Pts',(-40.0483669724133,-46.6832869376886,
-158.347956944359));
#151276=CARTESIAN_POINT('Ctrl Pts',(-39.9970465019613,-46.6888297686089,
-158.239712731665));
#151277=CARTESIAN_POINT('Ctrl Pts',(-39.944733925413,-46.6944797512428,
-158.129375986647));
#151278=CARTESIAN_POINT('Ctrl Pts',(-39.8948160656533,-46.7001650767535,
-158.018146559171));
#151279=CARTESIAN_POINT('Ctrl Pts',(-39.8471176835924,-46.7059395833958,
-157.906060277828));
#151280=CARTESIAN_POINT('Ctrl Pts',(-39.8407923129947,-46.7067053513937,
-157.891196308909));
#151281=CARTESIAN_POINT('Ctrl Pts',(-39.8345060078927,-46.7074727414294,
-157.87631723173));
#151282=CARTESIAN_POINT('Ctrl Pts',(-39.8282583922396,-46.7082419270457,
-157.861423094293));
#151283=CARTESIAN_POINT('Ctrl Pts',(-39.7717626884057,-46.7151974898055,
-157.726738948491));
#151284=CARTESIAN_POINT('Ctrl Pts',(-39.7184638218149,-46.7222433276003,
-157.590841615228));
#151285=CARTESIAN_POINT('Ctrl Pts',(-39.6682083051711,-46.7293360118737,
-157.453806541317));
#151286=CARTESIAN_POINT('Ctrl Pts',(-39.6171120060077,-46.7365473578454,
-157.314478849553));
#151287=CARTESIAN_POINT('Ctrl Pts',(-39.5691610368222,-46.7438075845872,
-157.173974722644));
#151288=CARTESIAN_POINT('Ctrl Pts',(-39.5242175974619,-46.7511105793801,
-157.03234443406));
#151289=CARTESIAN_POINT('Ctrl Pts',(-39.4783447495199,-46.758564596572,
-156.88778529963));
#151290=CARTESIAN_POINT('Ctrl Pts',(-39.4356044625501,-46.7660637202736,
-156.742052563172));
#151291=CARTESIAN_POINT('Ctrl Pts',(-39.3958849012062,-46.7736346178437,
-156.595174950523));
#151292=CARTESIAN_POINT('Ctrl Pts',(-39.3844661816561,-46.7758111261729,
-156.552950056534));
#151293=CARTESIAN_POINT('Ctrl Pts',(-39.3732973633793,-46.7779937423037,
-156.510630409542));
#151294=CARTESIAN_POINT('Ctrl Pts',(-39.3623764117127,-46.7801834881411,
-156.468216397628));
#151295=CARTESIAN_POINT('Ctrl Pts',(-39.3213886065209,-46.7884018997361,
-156.309030887905));
#151296=CARTESIAN_POINT('Ctrl Pts',(-39.2841032524674,-46.7966765801414,
-156.149349043185));
#151297=CARTESIAN_POINT('Ctrl Pts',(-39.2503661597731,-46.8049680101138,
-155.98922493615));
#151298=CARTESIAN_POINT('Ctrl Pts',(-39.2158556778871,-46.8134495128462,
-155.82543014371));
#151299=CARTESIAN_POINT('Ctrl Pts',(-39.1850574748408,-46.8219492572809,
-155.661172069128));
#151300=CARTESIAN_POINT('Ctrl Pts',(-39.157847363523,-46.830454388723,-155.496486938258));
#151301=CARTESIAN_POINT('Ctrl Pts',(-39.1298994391238,-46.8391901402154,
-155.327336304014));
#151302=CARTESIAN_POINT('Ctrl Pts',(-39.1057364276871,-46.847932409478,
-155.157734529226));
#151303=CARTESIAN_POINT('Ctrl Pts',(-39.0852736729076,-46.8566860190199,
-154.987706928931));
#151304=CARTESIAN_POINT('Ctrl Pts',(-39.064673617634,-46.8654983633181,
-154.81653848158));
#151305=CARTESIAN_POINT('Ctrl Pts',(-39.0478236262521,-46.8743231257662,
-154.644937780829));
#151306=CARTESIAN_POINT('Ctrl Pts',(-39.034690197654,-46.8831704349881,
-154.472926755722));
#151307=CARTESIAN_POINT('Ctrl Pts',(-39.0215514753255,-46.8920213103216,
-154.300846397615));
#151308=CARTESIAN_POINT('Ctrl Pts',(-39.0121325773116,-46.9008956262777,
-154.12835470933));
#151309=CARTESIAN_POINT('Ctrl Pts',(-39.0064507305479,-46.9097951391645,
-153.955480082265));
#151310=CARTESIAN_POINT('Ctrl Pts',(-39.0021584937233,-46.9165180971254,
-153.824885423315));
#151311=CARTESIAN_POINT('Ctrl Pts',(-39.0000000085995,-46.9232553328191,
-153.694072304413));
#151312=CARTESIAN_POINT('Ctrl Pts',(-39.,-46.9300000199928,-153.563058845201));
#151313=CARTESIAN_POINT('Ctrl Pts',(-40.5149864073608,-46.6403532458042,
-159.17182559703));
#151314=CARTESIAN_POINT('Ctrl Pts',(-40.6428186202086,-46.43000002,-159.094316247135));
#151315=CARTESIAN_POINT('Ctrl Pts',(-40.8634877666247,-46.43000002,-158.96051646616));
#151316=CARTESIAN_POINT('Ctrl Pts',(-42.8925295367156,-46.6503554345072,
-163.106696326736));
#151317=CARTESIAN_POINT('Ctrl Pts',(-43.0357695446718,-46.4300000199999,
-163.055969456472));
#151318=CARTESIAN_POINT('Ctrl Pts',(-43.2493416424527,-46.43000002,-162.895383432653));
#151319=CARTESIAN_POINT('Ctrl Pts',(-45.2098379840441,-46.6594189992588,
-167.077916061371));
#151320=CARTESIAN_POINT('Ctrl Pts',(-45.3499681200706,-46.4300000200635,
-167.025403443097));
#151321=CARTESIAN_POINT('Ctrl Pts',(-45.5734830336511,-46.43000002,-166.866604917879));
#151322=CARTESIAN_POINT('Ctrl Pts',(-47.4880541505298,-46.6677435098469,
-171.07256826174));
#151323=CARTESIAN_POINT('Ctrl Pts',(-47.6152001643476,-46.4300000199999,
-170.99986675708));
#151324=CARTESIAN_POINT('Ctrl Pts',(-47.8576079004676,-46.43000002,-170.861259130871));
#151325=CARTESIAN_POINT('',(-47.4880541505298,-46.6677435098469,-171.07256826174));
#151326=CARTESIAN_POINT('Origin',(-47.8576079004676,-46.93000002,-170.861259130871));
#151327=CARTESIAN_POINT('Ctrl Pts',(-47.4880541505298,-46.6677435098469,
-171.07256826174));
#151328=CARTESIAN_POINT('Ctrl Pts',(-45.2098379840441,-46.6594189992588,
-167.077916061371));
#151329=CARTESIAN_POINT('Ctrl Pts',(-42.8925295367156,-46.6503554345072,
-163.106696326736));
#151330=CARTESIAN_POINT('Ctrl Pts',(-40.5149864073608,-46.6403532458042,
-159.17182559703));
#151331=CARTESIAN_POINT('Ctrl Pts',(-48.4122058243951,-46.43000002,-171.14995));
#151332=CARTESIAN_POINT('Ctrl Pts',(-48.4122058243951,-46.43000002,-171.64995));
#151333=CARTESIAN_POINT('Ctrl Pts',(-48.4122058243951,-46.93000002,-171.64995));
#151334=CARTESIAN_POINT('Ctrl Pts',(-48.3039317427638,-46.43000002,-171.149949965311));
#151335=CARTESIAN_POINT('Ctrl Pts',(-48.2401145573434,-46.43000002,-171.601506869702));
#151336=CARTESIAN_POINT('Ctrl Pts',(-48.231362292365,-46.8790932958503,
-171.64995));
#151337=CARTESIAN_POINT('Ctrl Pts',(-48.1935717932631,-46.43000002,-171.125988974658));
#151338=CARTESIAN_POINT('Ctrl Pts',(-48.0743475333484,-46.4300000200007,
-171.520103948478));
#151339=CARTESIAN_POINT('Ctrl Pts',(-48.0473109525228,-46.8270214030016,
-171.602027929987));
#151340=CARTESIAN_POINT('Ctrl Pts',(-47.9990582077163,-46.43000002,-171.030110581883));
#151341=CARTESIAN_POINT('Ctrl Pts',(-47.8027749187994,-46.4300000199993,
-171.303307031957));
#151342=CARTESIAN_POINT('Ctrl Pts',(-47.7232867546241,-46.734966787668,
-171.410271183096));
#151343=CARTESIAN_POINT('Ctrl Pts',(-47.9126814701194,-46.43000002,-170.95757572435));
#151344=CARTESIAN_POINT('Ctrl Pts',(-47.6869922690936,-46.43000002,-171.166719195593));
#151345=CARTESIAN_POINT('Ctrl Pts',(-47.5795866952779,-46.693929642055,
-171.265147156144));
#151346=CARTESIAN_POINT('Ctrl Pts',(-47.8576079004676,-46.43000002,-170.861259130871));
#151347=CARTESIAN_POINT('Ctrl Pts',(-47.6152001643476,-46.43000002,-170.99986675708));
#151348=CARTESIAN_POINT('Ctrl Pts',(-47.4880541505298,-46.6677435098469,
-171.07256826174));
#151349=CARTESIAN_POINT('',(-48.4122058243951,-46.93000002,-171.64995));
#151350=CARTESIAN_POINT('Origin',(-48.4122058243951,-46.93000002,-171.14995));
#151351=CARTESIAN_POINT('Ctrl Pts',(-48.4122058243951,-46.93000002,-171.64995));
#151352=CARTESIAN_POINT('Ctrl Pts',(-48.231362292365,-46.8790932958503,
-171.64995));
#151353=CARTESIAN_POINT('Ctrl Pts',(-48.0473109525228,-46.8270214030016,
-171.602027929987));
#151354=CARTESIAN_POINT('Ctrl Pts',(-47.7232867546241,-46.734966787668,
-171.410271183096));
#151355=CARTESIAN_POINT('Ctrl Pts',(-47.5795866952779,-46.693929642055,
-171.265147156144));
#151356=CARTESIAN_POINT('Ctrl Pts',(-47.4880541505298,-46.6677435098469,
-171.07256826174));
#151357=CARTESIAN_POINT('Origin',(1.41965171211599E-14,-46.93000002,-171.14995));
#151358=CARTESIAN_POINT('',(-50.4241310475534,-46.93000002,-171.64995));
#151359=CARTESIAN_POINT('Origin',(-50.4241310475534,-46.93000002,-171.14995));
#151360=CARTESIAN_POINT('',(-48.7591445042216,-46.93000002,-171.64995));
#151361=CARTESIAN_POINT('Ctrl Pts',(-50.4241310475534,-46.93000002,-171.64995));
#151362=CARTESIAN_POINT('Ctrl Pts',(-50.4241310475535,-46.43000002,-171.64995));
#151363=CARTESIAN_POINT('Ctrl Pts',(-50.4241310475534,-46.43000002,-171.14995));
#151364=CARTESIAN_POINT('Ctrl Pts',(-50.5576213910783,-46.9208895200013,
-171.64995));
#151365=CARTESIAN_POINT('Ctrl Pts',(-50.5563794763166,-46.43000002,-171.640924254979));
#151366=CARTESIAN_POINT('Ctrl Pts',(-50.6224459669284,-46.43000002,-171.149950000016));
#151367=CARTESIAN_POINT('Ctrl Pts',(-50.6910111165761,-46.911785887019,
-171.675977326981));
#151368=CARTESIAN_POINT('Ctrl Pts',(-50.6936490544688,-46.43000002,-171.658003579003));
#151369=CARTESIAN_POINT('Ctrl Pts',(-50.8206114069094,-46.43000002,-171.18899099047));
#151370=CARTESIAN_POINT('Ctrl Pts',(-50.9376246396682,-46.8949549130127,
-171.776163607997));
#151371=CARTESIAN_POINT('Ctrl Pts',(-50.9520843153697,-46.4300000199999,
-171.746711574348));
#151372=CARTESIAN_POINT('Ctrl Pts',(-51.1869835328424,-46.43000002,-171.339270411997));
#151373=CARTESIAN_POINT('Ctrl Pts',(-51.0507273913534,-46.887235833176,
-171.850283164392));
#151374=CARTESIAN_POINT('Ctrl Pts',(-51.0736480315269,-46.4300000199987,
-171.817687494207));
#151375=CARTESIAN_POINT('Ctrl Pts',(-51.3550103914843,-46.43000002,-171.450449746589));
#151376=CARTESIAN_POINT('Ctrl Pts',(-51.239477210225,-46.8743539633763,
-172.035403273235));
#151377=CARTESIAN_POINT('Ctrl Pts',(-51.2780932509,-46.4300000200014,-172.003556970023));
#151378=CARTESIAN_POINT('Ctrl Pts',(-51.6354194766937,-46.43000002,-171.728129909852));
#151379=CARTESIAN_POINT('Ctrl Pts',(-51.3150500528584,-46.8691962391206,
-172.14633102856));
#151380=CARTESIAN_POINT('Ctrl Pts',(-51.3616623431659,-46.43000002,-172.118296873734));
#151381=CARTESIAN_POINT('Ctrl Pts',(-51.7476914343352,-46.43000002,-171.894521542842));
#151382=CARTESIAN_POINT('Ctrl Pts',(-51.4172007186852,-46.8622246214263,
-172.38820210671));
#151383=CARTESIAN_POINT('Ctrl Pts',(-51.4744733522994,-46.43000002,-172.371853931892));
#151384=CARTESIAN_POINT('Ctrl Pts',(-51.8994477376182,-46.43000002,-172.257328160063));
#151385=CARTESIAN_POINT('Ctrl Pts',(-51.4437383719602,-46.8604134695225,
-172.51902671195));
#151386=CARTESIAN_POINT('Ctrl Pts',(-51.5042290374097,-46.43000002,-172.511015867073));
#151387=CARTESIAN_POINT('Ctrl Pts',(-51.9388724063164,-46.43000002,-172.453565067926));
#151388=CARTESIAN_POINT('Ctrl Pts',(-51.4437383719606,-46.86041346952,-172.64995));
#151389=CARTESIAN_POINT('Ctrl Pts',(-51.5042290374232,-46.43000002,-172.64995));
#151390=CARTESIAN_POINT('Ctrl Pts',(-51.9388724063314,-46.43000002,-172.64995));
#151391=CARTESIAN_POINT('Origin',(-51.9388724063314,-46.93000002,-172.64995));
#151392=CARTESIAN_POINT('Ctrl Pts',(-51.4437383719606,-46.86041346952,-172.64995));
#151393=CARTESIAN_POINT('Ctrl Pts',(-51.4437383719602,-46.8604134695225,
-172.51902671195));
#151394=CARTESIAN_POINT('Ctrl Pts',(-51.4172007186852,-46.8622246214263,
-172.38820210671));
#151395=CARTESIAN_POINT('Ctrl Pts',(-51.3150500528584,-46.8691962391206,
-172.14633102856));
#151396=CARTESIAN_POINT('Ctrl Pts',(-51.239477210225,-46.8743539633763,
-172.035403273235));
#151397=CARTESIAN_POINT('Ctrl Pts',(-51.0507273913534,-46.887235833176,
-171.850283164392));
#151398=CARTESIAN_POINT('Ctrl Pts',(-50.9376246396682,-46.8949549130127,
-171.776163607997));
#151399=CARTESIAN_POINT('Ctrl Pts',(-50.6910111165761,-46.911785887019,
-171.675977326981));
#151400=CARTESIAN_POINT('Ctrl Pts',(-50.5576213910783,-46.9208895200013,
-171.64995));
#151401=CARTESIAN_POINT('Ctrl Pts',(-50.4241310475534,-46.93000002,-171.64995));
#151402=CARTESIAN_POINT('Origin',(-51.9388724063314,-46.93000002,-171.64995));
#151403=CARTESIAN_POINT('Origin',(-51.9388724063314,-46.93000002,-176.84995));
#151404=CARTESIAN_POINT('Origin',(83.2809572255632,-45.9300000199999,-176.84995));
#151405=CARTESIAN_POINT('',(-57.,-45.93000002,-177.34995));
#151406=CARTESIAN_POINT('Origin',(-57.,-45.93000002,-176.84995));
#151407=CARTESIAN_POINT('',(-52.0794132410337,-45.93000002,-177.34995));
#151408=CARTESIAN_POINT('',(-60.,-45.93000002,-177.34995));
#151409=CARTESIAN_POINT('Ctrl Pts',(-51.9388724063314,-46.43000002,-176.84995));
#151410=CARTESIAN_POINT('Ctrl Pts',(-51.9388724063423,-46.43000002,-176.981217345763));
#151411=CARTESIAN_POINT('Ctrl Pts',(-51.9540189315504,-46.3761134565303,
-177.110943344657));
#151412=CARTESIAN_POINT('Ctrl Pts',(-52.0060527960138,-46.1909933646562,
-177.296063436531));
#151413=CARTESIAN_POINT('Ctrl Pts',(-52.0425163963479,-46.0612673657634,
-177.34995));
#151414=CARTESIAN_POINT('Ctrl Pts',(-52.0794132410337,-45.93000002,-177.34995));
#151415=CARTESIAN_POINT('Origin',(-57.,-45.93000002,-174.34995));
#151416=CARTESIAN_POINT('',(-60.,-45.93000002,-174.34995));
#151417=CARTESIAN_POINT('Origin',(-59.5,-45.93000002,-174.34995));
#151418=CARTESIAN_POINT('Origin',(-57.,-45.93000002,-174.34995));
#151419=CARTESIAN_POINT('Origin',(-59.5,-45.93000002,-55.2499500000008));
#151420=CARTESIAN_POINT('',(-60.,-45.93000002,-58.24995));
#151421=CARTESIAN_POINT('Origin',(-59.5,-45.93000002,-58.24995));
#151422=CARTESIAN_POINT('',(-60.,-45.93000002,-174.34995));
#151423=CARTESIAN_POINT('Origin',(-57.,-45.93000002,-58.24995));
#151424=CARTESIAN_POINT('Origin',(-57.,-45.93000002,-58.24995));
#151425=CARTESIAN_POINT('Origin',(-57.,-2.42462934179819E-14,-58.24995));
#151426=CARTESIAN_POINT('',(-60.,-45.43000002,-58.24995));
#151427=CARTESIAN_POINT('Origin',(-57.,-45.43000002,-58.24995));
#151428=CARTESIAN_POINT('',(-60.,-54.58000002,-58.24995));
#151429=CARTESIAN_POINT('Origin',(-57.,-45.43000002,-58.24995));
#151430=CARTESIAN_POINT('Origin',(-59.5,-45.43000002,-58.24995));
#151431=CARTESIAN_POINT('Origin',(83.2809572255632,-44.43000002,-61.14995));
#151432=CARTESIAN_POINT('Origin',(-60.,-45.43000002,-176.84995));
#151433=CARTESIAN_POINT('',(-52.1496836583849,-45.43000002,-177.34995));
#151434=CARTESIAN_POINT('',(-57.,-45.43000002,-177.34995));
#151435=CARTESIAN_POINT('',(-60.,-45.43000002,-177.34995));
#151436=CARTESIAN_POINT('Origin',(-57.,-45.43000002,-176.84995));
#151437=CARTESIAN_POINT('Ctrl Pts',(-52.1496836583849,-45.43000002,-177.34995));
#151438=CARTESIAN_POINT('Ctrl Pts',(-52.1865805030705,-45.2987326742378,
-177.34995));
#151439=CARTESIAN_POINT('Ctrl Pts',(-52.2230441034049,-45.1690066753419,
-177.296063436528));
#151440=CARTESIAN_POINT('Ctrl Pts',(-52.2750779678683,-44.9838865834715,
-177.110943344658));
#151441=CARTESIAN_POINT('Ctrl Pts',(-52.2902244930764,-44.93000002,-176.981217345763));
#151442=CARTESIAN_POINT('Ctrl Pts',(-52.2902244930873,-44.93000002,-176.84995));
#151443=CARTESIAN_POINT('Origin',(-52.2902244930873,-44.43000002,-171.64995));
#151444=CARTESIAN_POINT('',(-51.7902244930873,-44.43000002,-172.64995));
#151445=CARTESIAN_POINT('Origin',(-52.2902244930873,-44.43000002,-172.64995));
#151446=CARTESIAN_POINT('Origin',(-52.2902244930873,-44.43000002,-176.84995));
#151447=CARTESIAN_POINT('Origin',(-52.2902244930873,-44.43000002,-172.64995));
#151448=CARTESIAN_POINT('Ctrl Pts',(-51.7950904587165,-44.36041346952,-172.64995));
#151449=CARTESIAN_POINT('Ctrl Pts',(-51.7150402894768,-44.93000002,-172.64995));
#151450=CARTESIAN_POINT('Ctrl Pts',(-52.2902244930873,-44.93000002,-172.64995));
#151451=CARTESIAN_POINT('Ctrl Pts',(-51.7950904587162,-44.3604134695225,
-172.51902671195));
#151452=CARTESIAN_POINT('Ctrl Pts',(-51.7150402894748,-44.9300000200027,
-172.529650273729));
#151453=CARTESIAN_POINT('Ctrl Pts',(-52.2902244930723,-44.93000002,-172.453565067926));
#151454=CARTESIAN_POINT('Ctrl Pts',(-51.7685528054411,-44.3622246214263,
-172.38820210671));
#151455=CARTESIAN_POINT('Ctrl Pts',(-51.6933705738162,-44.93000002,-172.409726298163));
#151456=CARTESIAN_POINT('Ctrl Pts',(-52.2507998243741,-44.93000002,-172.257328160063));
#151457=CARTESIAN_POINT('Ctrl Pts',(-51.6664021396144,-44.3691962391205,
-172.14633102856));
#151458=CARTESIAN_POINT('Ctrl Pts',(-51.6069372443981,-44.93000002,-172.182182441317));
#151459=CARTESIAN_POINT('Ctrl Pts',(-52.0990435210912,-44.93000002,-171.894521542842));
#151460=CARTESIAN_POINT('Ctrl Pts',(-51.5908292969809,-44.3743539633763,
-172.035403273235));
#151461=CARTESIAN_POINT('Ctrl Pts',(-51.5426661785871,-44.9300000199979,
-172.075215659168));
#151462=CARTESIAN_POINT('Ctrl Pts',(-51.9867715634496,-44.93000002,-171.728129909852));
#151463=CARTESIAN_POINT('Ctrl Pts',(-51.4020794781095,-44.387235833176,
-171.850283164392));
#151464=CARTESIAN_POINT('Ctrl Pts',(-51.3750094074331,-44.930000020002,
-171.888983273332));
#151465=CARTESIAN_POINT('Ctrl Pts',(-51.7063624782404,-44.93000002,-171.450449746589));
#151466=CARTESIAN_POINT('Ctrl Pts',(-51.2889767264242,-44.3949549130127,
-171.776163607997));
#151467=CARTESIAN_POINT('Ctrl Pts',(-51.2724346946947,-44.9300000200007,
-171.809929875206));
#151468=CARTESIAN_POINT('Ctrl Pts',(-51.5383356195984,-44.93000002,-171.339270411997));
#151469=CARTESIAN_POINT('Ctrl Pts',(-51.0423632033321,-44.411785887019,
-171.675977326981));
#151470=CARTESIAN_POINT('Ctrl Pts',(-51.0396558988745,-44.9300000199993,
-171.69520402023));
#151471=CARTESIAN_POINT('Ctrl Pts',(-51.1719634936654,-44.93000002,-171.18899099047));
#151472=CARTESIAN_POINT('Ctrl Pts',(-50.9089734778343,-44.4208895200012,
-171.64995));
#151473=CARTESIAN_POINT('Ctrl Pts',(-50.9102650806209,-44.93000002,-171.659148653595));
#151474=CARTESIAN_POINT('Ctrl Pts',(-50.9737980536844,-44.93000002,-171.149950000016));
#151475=CARTESIAN_POINT('Ctrl Pts',(-50.7754831343094,-44.43000002,-171.64995));
#151476=CARTESIAN_POINT('Ctrl Pts',(-50.7754831343094,-44.9300000199999,
-171.64995));
#151477=CARTESIAN_POINT('Ctrl Pts',(-50.7754831343094,-44.93000002,-171.14995));
#151478=CARTESIAN_POINT('',(-50.7754831343094,-44.43000002,-171.64995));
#151479=CARTESIAN_POINT('Origin',(-50.7754831343094,-44.43000002,-171.14995));
#151480=CARTESIAN_POINT('Ctrl Pts',(-50.7754831343094,-44.43000002,-171.64995));
#151481=CARTESIAN_POINT('Ctrl Pts',(-50.9089734778343,-44.4208895200012,
-171.64995));
#151482=CARTESIAN_POINT('Ctrl Pts',(-51.0423632033321,-44.411785887019,
-171.675977326981));
#151483=CARTESIAN_POINT('Ctrl Pts',(-51.2889767264242,-44.3949549130127,
-171.776163607997));
#151484=CARTESIAN_POINT('Ctrl Pts',(-51.4020794781095,-44.387235833176,
-171.850283164392));
#151485=CARTESIAN_POINT('Ctrl Pts',(-51.5908292969809,-44.3743539633763,
-172.035403273235));
#151486=CARTESIAN_POINT('Ctrl Pts',(-51.6664021396144,-44.3691962391205,
-172.14633102856));
#151487=CARTESIAN_POINT('Ctrl Pts',(-51.7685528054411,-44.3622246214263,
-172.38820210671));
#151488=CARTESIAN_POINT('Ctrl Pts',(-51.7950904587162,-44.3604134695225,
-172.51902671195));
#151489=CARTESIAN_POINT('Ctrl Pts',(-51.7950904587165,-44.36041346952,-172.64995));
#151490=CARTESIAN_POINT('Origin',(1.31515029790052E-14,-44.43000002,-171.14995));
#151491=CARTESIAN_POINT('',(-50.0729884546894,-44.43000002,-171.64995));
#151492=CARTESIAN_POINT('Origin',(-50.0729884546894,-44.43000002,-171.14995));
#151493=CARTESIAN_POINT('',(-50.7052127169582,-44.43000002,-171.64995));
#151494=CARTESIAN_POINT('Ctrl Pts',(-49.5369875341119,-44.93000002,-170.861259130871));
#151495=CARTESIAN_POINT('Ctrl Pts',(-48.7929216289437,-44.9300000199999,
-171.272289063137));
#151496=CARTESIAN_POINT('Ctrl Pts',(-49.1544657093286,-44.1870483688939,
-171.07256826174));
#151497=CARTESIAN_POINT('Ctrl Pts',(-49.5629323055535,-44.93000002,-170.908225431312));
#151498=CARTESIAN_POINT('Ctrl Pts',(-48.8869683938206,-44.93000002,-171.389208114715));
#151499=CARTESIAN_POINT('Ctrl Pts',(-49.1988333494309,-44.1988790013969,
-171.166486883581));
#151500=CARTESIAN_POINT('Ctrl Pts',(-49.5959607588443,-44.93000002,-170.94944826591));
#151501=CARTESIAN_POINT('Ctrl Pts',(-48.9974211832039,-44.93000002,-171.47664075754));
#151502=CARTESIAN_POINT('Ctrl Pts',(-49.2553422033029,-44.2139336491638,
-171.248946535323));
#151503=CARTESIAN_POINT('Ctrl Pts',(-49.673955990897,-44.93000002,-171.02211105853));
#151504=CARTESIAN_POINT('Ctrl Pts',(-49.2286028218105,-44.93000002,-171.604363908288));
#151505=CARTESIAN_POINT('Ctrl Pts',(-49.3888358236751,-44.249424483408,
-171.394272113556));
#151506=CARTESIAN_POINT('Ctrl Pts',(-49.7179930277929,-44.93000002,-171.052463257479));
#151507=CARTESIAN_POINT('Ctrl Pts',(-49.3448677594853,-44.9300000199992,
-171.644582495821));
#151508=CARTESIAN_POINT('Ctrl Pts',(-49.4642369070823,-44.2694386569593,
-171.45497652175));
#151509=CARTESIAN_POINT('Ctrl Pts',(-49.8597665056525,-44.93000002,-171.125547207032));
#151510=CARTESIAN_POINT('Ctrl Pts',(-49.6719308335793,-44.9300000200013,
-171.711639121533));
#151511=CARTESIAN_POINT('Ctrl Pts',(-49.7071198591548,-44.3337582466603,
-171.601144400479));
#151512=CARTESIAN_POINT('Ctrl Pts',(-49.9661358829125,-44.93000002,-171.149949988199));
#151513=CARTESIAN_POINT('Ctrl Pts',(-49.8809090309114,-44.93000002,-171.700346637809));
#151514=CARTESIAN_POINT('Ctrl Pts',(-49.8895242589787,-44.3818638633066,
-171.64995));
#151515=CARTESIAN_POINT('Ctrl Pts',(-50.0729884546894,-44.93000002,-171.14995));
#151516=CARTESIAN_POINT('Ctrl Pts',(-50.0729884546893,-44.93000002,-171.64995));
#151517=CARTESIAN_POINT('Ctrl Pts',(-50.0729884546894,-44.43000002,-171.64995));
#151518=CARTESIAN_POINT('',(-49.1544657093286,-44.1870483688939,-171.07256826174));
#151519=CARTESIAN_POINT('Origin',(-49.5369875341119,-44.43000002,-170.861259130871));
#151520=CARTESIAN_POINT('Ctrl Pts',(-49.1544657093286,-44.1870483688939,
-171.07256826174));
#151521=CARTESIAN_POINT('Ctrl Pts',(-49.1988333494309,-44.1988790013969,
-171.166486883581));
#151522=CARTESIAN_POINT('Ctrl Pts',(-49.2553422033029,-44.2139336491638,
-171.248946535323));
#151523=CARTESIAN_POINT('Ctrl Pts',(-49.3888358236751,-44.249424483408,
-171.394272113556));
#151524=CARTESIAN_POINT('Ctrl Pts',(-49.4642369070823,-44.2694386569593,
-171.45497652175));
#151525=CARTESIAN_POINT('Ctrl Pts',(-49.7071198591548,-44.3337582466603,
-171.601144400479));
#151526=CARTESIAN_POINT('Ctrl Pts',(-49.8895242589787,-44.3818638633066,
-171.64995));
#151527=CARTESIAN_POINT('Ctrl Pts',(-50.0729884546894,-44.43000002,-171.64995));
#151528=CARTESIAN_POINT('Ctrl Pts',(-49.1544657093286,-44.1870483688939,
-171.07256826174));
#151529=CARTESIAN_POINT('Ctrl Pts',(-48.7929216289437,-44.9300000199999,
-171.272289063137));
#151530=CARTESIAN_POINT('Ctrl Pts',(-49.5369875341119,-44.93000002,-170.861259130871));
#151531=CARTESIAN_POINT('Ctrl Pts',(-46.303473398785,-44.1770628106394,
-165.900085726624));
#151532=CARTESIAN_POINT('Ctrl Pts',(-45.8620651160177,-44.9300000199373,
-166.013584137672));
#151533=CARTESIAN_POINT('Ctrl Pts',(-46.6796506810215,-44.93000002,-165.688772250388));
#151534=CARTESIAN_POINT('Ctrl Pts',(-43.4017256360502,-44.1659184128467,
-160.756986066495));
#151535=CARTESIAN_POINT('Ctrl Pts',(-42.9064403928045,-44.93000002,-160.851370978315));
#151536=CARTESIAN_POINT('Ctrl Pts',(-43.7703248719811,-44.93000002,-160.54566797298));
#151537=CARTESIAN_POINT('Ctrl Pts',(-40.4124516249929,-44.1531545436406,
-155.665156257244));
#151538=CARTESIAN_POINT('Ctrl Pts',(-39.9673804148566,-44.93000002,-155.927306340695));
#151539=CARTESIAN_POINT('Ctrl Pts',(-40.7712064624936,-44.93000002,-155.453847126373));
#151540=CARTESIAN_POINT('',(-40.4124515954294,-44.1531546078393,-155.665156239121));
#151541=CARTESIAN_POINT('Origin',(-40.7712064624936,-44.43000002,-155.453847126373));
#151542=CARTESIAN_POINT('Ctrl Pts',(-40.4124516249929,-44.1531545436406,
-155.665156257244));
#151543=CARTESIAN_POINT('Ctrl Pts',(-43.4017256360502,-44.1659184128467,
-160.756986066495));
#151544=CARTESIAN_POINT('Ctrl Pts',(-46.303473398785,-44.1770628106394,
-165.900085726624));
#151545=CARTESIAN_POINT('Ctrl Pts',(-49.1544657093286,-44.1870483688939,
-171.07256826174));
#151546=CARTESIAN_POINT('Ctrl Pts',(-39.5,-44.93000002,-150.364854264666));
#151547=CARTESIAN_POINT('Ctrl Pts',(-39.0000000000006,-44.93000002,-150.364854264666));
#151548=CARTESIAN_POINT('Ctrl Pts',(-39.,-44.4300000200006,-150.364854264665));
#151549=CARTESIAN_POINT('Ctrl Pts',(-39.5000000014677,-44.93000002,-151.253598202975));
#151550=CARTESIAN_POINT('Ctrl Pts',(-38.9493378739027,-44.93000002,-151.339754274397));
#151551=CARTESIAN_POINT('Ctrl Pts',(-38.9999999999989,-44.3818073757215,
-151.292233578463));
#151552=CARTESIAN_POINT('Ctrl Pts',(-39.5994072100806,-44.93000002,-152.128156158989));
#151553=CARTESIAN_POINT('Ctrl Pts',(-39.0101446877546,-44.93000002,-152.270659170967));
#151554=CARTESIAN_POINT('Ctrl Pts',(-39.1104524571481,-44.3342708908056,
-152.203846600498));
#151555=CARTESIAN_POINT('Ctrl Pts',(-39.9069198952433,-44.93000002,-153.416428338509));
#151556=CARTESIAN_POINT('Ctrl Pts',(-39.2308584472657,-44.93000002,-153.622795365418));
#151557=CARTESIAN_POINT('Ctrl Pts',(-39.4521332161855,-44.2641615099952,
-153.545498595041));
#151558=CARTESIAN_POINT('Ctrl Pts',(-40.0374208080396,-44.93000002,-153.8438516675));
#151559=CARTESIAN_POINT('Ctrl Pts',(-39.336211428575,-44.93000002,-154.093302098276));
#151560=CARTESIAN_POINT('Ctrl Pts',(-39.5971342320646,-44.2408855884987,
-153.990424071582));
#151561=CARTESIAN_POINT('Ctrl Pts',(-40.356527124461,-44.93000002,-154.669573645042));
#151562=CARTESIAN_POINT('Ctrl Pts',(-39.6029233414186,-44.9300000199999,
-155.022603846473));
#151563=CARTESIAN_POINT('Ctrl Pts',(-39.9516968040472,-44.1959019617888,
-154.849602863721));
#151564=CARTESIAN_POINT('Ctrl Pts',(-40.5450613770689,-44.93000002,-155.069904201826));
#151565=CARTESIAN_POINT('Ctrl Pts',(-39.7696946227985,-44.93000002,-155.485741538253));
#151566=CARTESIAN_POINT('Ctrl Pts',(-40.1611888206879,-44.1740829716026,
-155.265988433439));
#151567=CARTESIAN_POINT('Ctrl Pts',(-40.7712064624936,-44.93000002,-155.453847126373));
#151568=CARTESIAN_POINT('Ctrl Pts',(-39.9673804148566,-44.93000002,-155.927306340695));
#151569=CARTESIAN_POINT('Ctrl Pts',(-40.4124516249929,-44.1531545436406,
-155.665156257244));
#151570=CARTESIAN_POINT('',(-39.,-44.4300000199906,-150.364854264666));
#151571=CARTESIAN_POINT('Origin',(-39.5,-44.43000002,-150.364854264666));
#151572=CARTESIAN_POINT('Ctrl Pts',(-39.,-44.4300000200006,-150.364854264666));
#151573=CARTESIAN_POINT('Ctrl Pts',(-38.999999999999,-44.3818073757215,
-151.292233578463));
#151574=CARTESIAN_POINT('Ctrl Pts',(-39.1104524571481,-44.3342708908056,
-152.203846600499));
#151575=CARTESIAN_POINT('Ctrl Pts',(-39.3382396298397,-44.2875313035987,
-153.098281263527));
#151576=CARTESIAN_POINT('Ctrl Pts',(-39.4521332161855,-44.2641615099952,
-153.545498595041));
#151577=CARTESIAN_POINT('Ctrl Pts',(-39.5971342320646,-44.2408855884987,
-153.990424071582));
#151578=CARTESIAN_POINT('Ctrl Pts',(-39.7744155180559,-44.2183937751437,
-154.420013467651));
#151579=CARTESIAN_POINT('Ctrl Pts',(-39.9516967998039,-44.1959019623272,
-154.849602853438));
#151580=CARTESIAN_POINT('Ctrl Pts',(-40.1611888106594,-44.1740829726471,
-155.265988413506));
#151581=CARTESIAN_POINT('Ctrl Pts',(-40.4124516069506,-44.1531545451434,
-155.665156228581));
#151582=CARTESIAN_POINT('Origin',(-39.5,-44.43000002,-55.2499500000007));
#151583=CARTESIAN_POINT('',(-39.,-44.43000002,-81.6937887068282));
#151584=CARTESIAN_POINT('Origin',(-39.5,-44.43000002,-81.6937887068282));
#151585=CARTESIAN_POINT('',(-39.,-44.43000002,-129.34995));
#151586=CARTESIAN_POINT('Ctrl Pts',(-41.0619056481271,-44.93000002,-76.1510528072502));
#151587=CARTESIAN_POINT('Ctrl Pts',(-40.2383013915693,-44.9300000200001,
-75.5735325535681));
#151588=CARTESIAN_POINT('Ctrl Pts',(-40.7356761305387,-44.1280183635067,
-75.9220149346039));
#151589=CARTESIAN_POINT('Ctrl Pts',(-40.6997637919875,-44.93000002,-76.6715445325856));
#151590=CARTESIAN_POINT('Ctrl Pts',(-39.915133580973,-44.9300000199999,
-76.1827431658708));
#151591=CARTESIAN_POINT('Ctrl Pts',(-40.3333152536302,-44.1563776140685,
-76.4629140546281));
#151592=CARTESIAN_POINT('Ctrl Pts',(-40.4205675940477,-44.93000002,-77.2240865411077));
#151593=CARTESIAN_POINT('Ctrl Pts',(-39.660816170609,-44.93000002,-76.8319017752828));
#151594=CARTESIAN_POINT('Ctrl Pts',(-40.023059761065,-44.186488846014,-77.037491401942));
#151595=CARTESIAN_POINT('Ctrl Pts',(-40.039661195993,-44.93000002,-78.208477386432));
#151596=CARTESIAN_POINT('Ctrl Pts',(-39.3372827309322,-44.93000002,-77.9582690332229));
#151597=CARTESIAN_POINT('Ctrl Pts',(-39.5997881972139,-44.2401083817187,
-78.0617130018949));
#151598=CARTESIAN_POINT('Ctrl Pts',(-39.9103339554084,-44.93000002,-78.6298739674098));
#151599=CARTESIAN_POINT('Ctrl Pts',(-39.2328733408237,-44.93000002,-78.4220178024824));
#151600=CARTESIAN_POINT('Ctrl Pts',(-39.4560716552024,-44.2630556348417,
-78.5003466592746));
#151601=CARTESIAN_POINT('Ctrl Pts',(-39.558721486255,-44.93000002,-80.0963039522294));
#151602=CARTESIAN_POINT('Ctrl Pts',(-38.9834353962971,-44.93000002,-79.9425516378539));
#151603=CARTESIAN_POINT('Ctrl Pts',(-39.0653053548081,-44.3428691652806,
-80.0275378636304));
#151604=CARTESIAN_POINT('Ctrl Pts',(-39.4642346663104,-44.93000002,-81.1617889688827));
#151605=CARTESIAN_POINT('Ctrl Pts',(-38.9290061700283,-44.9300000199999,
-81.0769866725498));
#151606=CARTESIAN_POINT('Ctrl Pts',(-38.9602847906733,-44.4007851791287,
-81.1383456746059));
#151607=CARTESIAN_POINT('Ctrl Pts',(-39.5119572736767,-44.93000002,-82.225747614569));
#151608=CARTESIAN_POINT('Ctrl Pts',(-39.0403511889319,-44.9300000199999,
-82.2482379714646));
#151609=CARTESIAN_POINT('Ctrl Pts',(-39.0132635226448,-44.4584456120789,
-82.2489957256636));
#151610=CARTESIAN_POINT('Origin',(-40.7712064624936,-44.43000002,-76.6047958451324));
#151611=CARTESIAN_POINT('Ctrl Pts',(-40.4124516186295,-44.153154649867,
-76.3934867953418));
#151612=CARTESIAN_POINT('Ctrl Pts',(-40.3492687471321,-44.1584174362915,
-76.4938623552029));
#151613=CARTESIAN_POINT('Ctrl Pts',(-40.2887972234514,-44.1637790836454,
-76.5952597648493));
#151614=CARTESIAN_POINT('Ctrl Pts',(-40.2308619735706,-44.1691773515359,
-76.6975721748967));
#151615=CARTESIAN_POINT('Ctrl Pts',(-40.1720233715351,-44.1746597916175,
-76.8014798854953));
#151616=CARTESIAN_POINT('Ctrl Pts',(-40.1158000723182,-44.1801801717817,
-76.9063314571057));
#151617=CARTESIAN_POINT('Ctrl Pts',(-40.062010544316,-44.1857172779623,
-77.0120479770336));
#151618=CARTESIAN_POINT('Ctrl Pts',(-40.0069033106055,-44.1913900290666,
-77.1203542810132));
#151619=CARTESIAN_POINT('Ctrl Pts',(-39.9543498747492,-44.1970805363738,
-77.2295685571082));
#151620=CARTESIAN_POINT('Ctrl Pts',(-39.904167438306,-44.2028090487481,
-77.3396386298012));
#151621=CARTESIAN_POINT('Ctrl Pts',(-39.859605995182,-44.2078959037604,
-77.4373796250899));
#151622=CARTESIAN_POINT('Ctrl Pts',(-39.8169140795409,-44.213013530734,
-77.5357960364665));
#151623=CARTESIAN_POINT('Ctrl Pts',(-39.7759776294699,-44.2182010663734,
-77.6348705097609));
#151624=CARTESIAN_POINT('Ctrl Pts',(-39.7206873277629,-44.2252075461762,
-77.7686842017251));
#151625=CARTESIAN_POINT('Ctrl Pts',(-39.6686277251655,-44.2322979157729,
-77.9036835094696));
#151626=CARTESIAN_POINT('Ctrl Pts',(-39.6196506088544,-44.2394333017539,
-78.0397988921473));
#151627=CARTESIAN_POINT('Ctrl Pts',(-39.5698722791269,-44.2466854150436,
-78.1781409773952));
#151628=CARTESIAN_POINT('Ctrl Pts',(-39.5232774197431,-44.2539845156844,
-78.3176362948157));
#151629=CARTESIAN_POINT('Ctrl Pts',(-39.479736648919,-44.2613273210185,
-78.4582406896765));
#151630=CARTESIAN_POINT('Ctrl Pts',(-39.435371602894,-44.2688091338215,
-78.6015068820576));
#151631=CARTESIAN_POINT('Ctrl Pts',(-39.3941767593022,-44.2763369097495,
-78.745924967725));
#151632=CARTESIAN_POINT('Ctrl Pts',(-39.3560523315242,-44.2839376143512,
-78.8914720771512));
#151633=CARTESIAN_POINT('Ctrl Pts',(-39.3509935172703,-44.284946168578,
-78.9107850435271));
#151634=CARTESIAN_POINT('Ctrl Pts',(-39.3459888245001,-44.285956042194,
-78.9301179169555));
#151635=CARTESIAN_POINT('Ctrl Pts',(-39.3410380762978,-44.2869673285108,
-78.9494706682134));
#151636=CARTESIAN_POINT('Ctrl Pts',(-39.2980051492431,-44.2957576382831,
-79.1176887837713));
#151637=CARTESIAN_POINT('Ctrl Pts',(-39.2592198938221,-44.3046155600241,
-79.2867252680673));
#151638=CARTESIAN_POINT('Ctrl Pts',(-39.224550515281,-44.3134982487801,
-79.4564303829574));
#151639=CARTESIAN_POINT('Ctrl Pts',(-39.1889042723014,-44.3226312213062,
-79.6309172072047));
#151640=CARTESIAN_POINT('Ctrl Pts',(-39.1576084892969,-44.3317911714413,
-79.8061114784507));
#151641=CARTESIAN_POINT('Ctrl Pts',(-39.1305597703672,-44.3409620370165,
-79.9818724566913));
#151642=CARTESIAN_POINT('Ctrl Pts',(-39.1026629400711,-44.3504204546697,
-80.1631444125051));
#151643=CARTESIAN_POINT('Ctrl Pts',(-39.0792832454589,-44.3598914595052,
-80.3450199391458));
#151644=CARTESIAN_POINT('Ctrl Pts',(-39.0603574905697,-44.3693756778076,
-80.5273570717227));
#151645=CARTESIAN_POINT('Ctrl Pts',(-39.0412931899528,-44.3789293251993,
-80.7110290007639));
#151646=CARTESIAN_POINT('Ctrl Pts',(-39.0267483551842,-44.3884974622236,
-80.8951701896708));
#151647=CARTESIAN_POINT('Ctrl Pts',(-39.0167110904471,-44.3980830680851,
-81.0796353183193));
#151648=CARTESIAN_POINT('Ctrl Pts',(-39.0067015411556,-44.4076422056464,
-81.2635910917448));
#151649=CARTESIAN_POINT('Ctrl Pts',(-39.0011751817154,-44.4172196919994,
-81.4478698295068));
#151650=CARTESIAN_POINT('Ctrl Pts',(-39.0001681003861,-44.4268053025559,
-81.6323145412984));
#151651=CARTESIAN_POINT('Ctrl Pts',(-39.0000562265889,-44.4278701407374,
-81.6528039791229));
#151652=CARTESIAN_POINT('Ctrl Pts',(-39.0000001661476,-44.4289350571871,
-81.6732954448402));
#151653=CARTESIAN_POINT('Ctrl Pts',(-39.0000000003688,-44.43000002,-81.6937887068282));
#151654=CARTESIAN_POINT('Ctrl Pts',(-40.4124516249929,-44.1531545436406,
-76.3934867142621));
#151655=CARTESIAN_POINT('Ctrl Pts',(-39.9673804148565,-44.93000002,-76.1313366308109));
#151656=CARTESIAN_POINT('Ctrl Pts',(-40.7712064624936,-44.93000002,-76.6047958451324));
#151657=CARTESIAN_POINT('Ctrl Pts',(-43.3552388512871,-44.1657199195518,
-71.3808409460202));
#151658=CARTESIAN_POINT('Ctrl Pts',(-42.8619820924489,-44.9300000200589,
-71.2817568775718));
#151659=CARTESIAN_POINT('Ctrl Pts',(-43.7236852143189,-44.93000002,-71.5921585277583));
#151660=CARTESIAN_POINT('Ctrl Pts',(-46.2131449010667,-44.1767154324357,
-66.3184583453296));
#151661=CARTESIAN_POINT('Ctrl Pts',(-45.7723278216974,-44.9300000200823,
-66.2016926213901));
#151662=CARTESIAN_POINT('Ctrl Pts',(-46.5890843541627,-44.93000002,-66.5297716146547));
#151663=CARTESIAN_POINT('Ctrl Pts',(-49.0214378669496,-44.1865817238571,
-61.2273317382593));
#151664=CARTESIAN_POINT('Ctrl Pts',(-48.6588221091936,-44.93000002,-61.026863396898));
#151665=CARTESIAN_POINT('Ctrl Pts',(-49.4036629110189,-44.93000002,-61.4386408691297));
#151666=CARTESIAN_POINT('Origin',(-59.5,-45.43000002,-55.2499500000007));
#151667=CARTESIAN_POINT('',(-60.,-45.43000002,-174.34995));
#151668=CARTESIAN_POINT('Origin',(-59.5,-45.43000002,-174.34995));
#151669=CARTESIAN_POINT('',(-60.,-45.43000002,-58.24995));
#151670=CARTESIAN_POINT('Origin',(-57.,-45.43000002,-174.34995));
#151671=CARTESIAN_POINT('Origin',(-57.,-45.43000002,-174.34995));
#151672=CARTESIAN_POINT('Origin',(0.,-12.9675000200281,-60.64995));
#151673=CARTESIAN_POINT('Origin',(-42.5,-55.58000002,-60.64995));
#151674=CARTESIAN_POINT('Origin',(0.,-12.9675000200281,-179.64995));
#151675=CARTESIAN_POINT('Origin',(3.54807775957937E-14,-73.08000002,3.11172719585489E-30));
#151676=CARTESIAN_POINT('',(-41.5,-73.08000002,-174.34995));
#151677=CARTESIAN_POINT('Ctrl Pts',(-30.800186642726,28.4199999800001,-78.2835659239152));
#151678=CARTESIAN_POINT('Ctrl Pts',(-29.3719438459593,28.4199999800001,
-77.079545860612));
#151679=CARTESIAN_POINT('Ctrl Pts',(-28.2935777143944,29.6448500754942,
-76.1704746152117));
#151680=CARTESIAN_POINT('Ctrl Pts',(-29.4908802242649,28.4199999800001,
-79.8367023859018));
#151681=CARTESIAN_POINT('Ctrl Pts',(-28.1162846817441,28.4199999799895,
-78.6350614606686));
#151682=CARTESIAN_POINT('Ctrl Pts',(-27.0582328538907,29.5957479131388,
-77.7235993982802));
#151683=CARTESIAN_POINT('Ctrl Pts',(-28.1443442258615,28.41999998,-81.3659786124399));
#151684=CARTESIAN_POINT('Ctrl Pts',(-26.8231903788109,28.41999998,-80.171186708314));
#151685=CARTESIAN_POINT('Ctrl Pts',(-25.7920491676122,29.54547115812,-79.2528873037006));
#151686=CARTESIAN_POINT('Ctrl Pts',(-25.359343066053,28.41999998,-84.349696566808));
#151687=CARTESIAN_POINT('Ctrl Pts',(-24.151734271497,28.41999998,-83.168456079353));
#151688=CARTESIAN_POINT('Ctrl Pts',(-23.1839068120671,29.4434760286189,
-82.2366052581402));
#151689=CARTESIAN_POINT('Ctrl Pts',(-23.928985790681,28.41999998,-85.7957524739721));
#151690=CARTESIAN_POINT('Ctrl Pts',(-22.7816855628193,28.4199999799965,
-84.621550748069));
#151691=CARTESIAN_POINT('Ctrl Pts',(-21.8495491428221,29.3920399293098,
-83.6826429630518));
#151692=CARTESIAN_POINT('Ctrl Pts',(-22.4473146057945,28.41999998,-87.1798147710383));
#151693=CARTESIAN_POINT('Ctrl Pts',(-21.3602588054756,28.41999998,-86.0160960137185));
#151694=CARTESIAN_POINT('Ctrl Pts',(-20.4734286051771,29.3409536236015,
-85.0667234623348));
#151695=CARTESIAN_POINT('Ctrl Pts',(-39.6993756576748,28.41999998,-66.758245524204));
#151696=CARTESIAN_POINT('Ctrl Pts',(-37.9544308619569,28.41999998,-65.5068366539031));
#151697=CARTESIAN_POINT('Ctrl Pts',(-36.7529144574179,29.9771506489281,
-64.6451542155005));
#151698=CARTESIAN_POINT('Ctrl Pts',(-38.3090750828473,28.41999998,-68.6968587227942));
#151699=CARTESIAN_POINT('Ctrl Pts',(-36.6139893647491,28.41999998,-67.4471428080873));
#151700=CARTESIAN_POINT('Ctrl Pts',(-35.4221830133223,29.9261764058054,
-66.5837572422386));
#151701=CARTESIAN_POINT('Ctrl Pts',(-36.8898270007225,28.4199999800001,
-70.617650456175));
#151702=CARTESIAN_POINT('Ctrl Pts',(-35.2435893151229,28.41999998,-69.3754183593105));
#151703=CARTESIAN_POINT('Ctrl Pts',(-34.0676680572731,29.8734031042169,
-68.5045591474479));
#151704=CARTESIAN_POINT('Ctrl Pts',(-33.9748337796689,28.4199999800001,
-74.4122216515051));
#151705=CARTESIAN_POINT('Ctrl Pts',(-32.4319411374915,28.41999998,-73.1856180617498));
#151706=CARTESIAN_POINT('Ctrl Pts',(-31.2955902801573,29.7642394885798,
-72.2991303428252));
#151707=CARTESIAN_POINT('Ctrl Pts',(-32.4811021033977,28.41999998,-76.2833884926716));
#151708=CARTESIAN_POINT('Ctrl Pts',(-30.9935194672858,28.4199999799959,
-75.0646492888563));
#151709=CARTESIAN_POINT('Ctrl Pts',(-29.8799523105758,29.7079117212239,
-74.1702869851635));
#151710=CARTESIAN_POINT('Ctrl Pts',(-30.9453615210646,28.41999998,-78.1110740930249));
#151711=CARTESIAN_POINT('Ctrl Pts',(-29.5115669185301,28.41999998,-76.9063064032585));
#151712=CARTESIAN_POINT('Ctrl Pts',(-28.4305705461597,29.6502955521147,
-75.9979827843214));
#151713=CARTESIAN_POINT('Ctrl Pts',(-36.7055660855173,29.9753365749746,
-64.7141089388348));
#151714=CARTESIAN_POINT('Ctrl Pts',(-35.3900556592162,29.9249246093161,
-66.6293066030352));
#151715=CARTESIAN_POINT('Ctrl Pts',(-34.0512327947874,29.8727558883661,
-68.5270566307911));
#151716=CARTESIAN_POINT('Ctrl Pts',(-32.6816291687152,29.8188212963983,
-70.4018447451366));
#151717=CARTESIAN_POINT('Ctrl Pts',(-32.0393671155873,29.7935292037721,
-71.2810080596735));
#151718=CARTESIAN_POINT('Ctrl Pts',(-31.3907503317202,29.7678616196868,
-72.1545609864309));
#151719=CARTESIAN_POINT('Ctrl Pts',(-30.7353640256462,29.7418658638091,
-73.0207789414145));
#151720=CARTESIAN_POINT('Origin',(-42.,28.91999998,-171.14995));
#151721=CARTESIAN_POINT('Origin',(-45.4220505312374,35.8460962305468,-172.64995));
#151722=CARTESIAN_POINT('Origin',(-44.489435756687,35.9771666894179,-172.64995));
#151723=CARTESIAN_POINT('Origin',(-44.2110895547669,33.9966305519348,-172.64995));
#151724=CARTESIAN_POINT('Origin',(-45.5819760525891,35.4528826626933,-172.64995));
#151725=CARTESIAN_POINT('Origin',(0.,-12.9675000200281,-172.64995));
#151726=CARTESIAN_POINT('Origin',(-48.4203826827217,32.6144760325608,-172.64995));
#151727=CARTESIAN_POINT('Origin',(-46.9641305719631,31.2435895347386,-172.64995));
#151728=CARTESIAN_POINT('Origin',(-48.9446667094463,31.5219357366587,-172.64995));
#151729=CARTESIAN_POINT('Origin',(-51.6222122422086,12.4702093225365,-172.64995));
#151730=CARTESIAN_POINT('Ctrl Pts',(-50.4704930916386,27.85041342952,-177.84995));
#151731=CARTESIAN_POINT('Ctrl Pts',(-50.4704930916386,27.85041342952,-177.34995));
#151732=CARTESIAN_POINT('Ctrl Pts',(-50.9656271260094,27.91999998,-177.34995));
#151733=CARTESIAN_POINT('Ctrl Pts',(-50.4335962469534,28.1129481210447,
-177.849949999941));
#151734=CARTESIAN_POINT('Ctrl Pts',(-50.4520556784241,27.9816024412645,
-177.367861075731));
#151735=CARTESIAN_POINT('Ctrl Pts',(-50.9287302813235,28.0512673257631,
-177.34995));
#151736=CARTESIAN_POINT('Ctrl Pts',(-50.3971326466187,28.3724001188352,
-177.742176873059));
#151737=CARTESIAN_POINT('Ctrl Pts',(-50.4311035247778,28.1306847609584,
-177.32958965968));
#151738=CARTESIAN_POINT('Ctrl Pts',(-50.8922666809894,28.1809933246567,
-177.29606343653));
#151739=CARTESIAN_POINT('Ctrl Pts',(-50.3450987821552,28.7426403025778,
-177.371936689315));
#151740=CARTESIAN_POINT('Ctrl Pts',(-50.4002116209072,28.3504920783889,
-177.142957948487));
#151741=CARTESIAN_POINT('Ctrl Pts',(-50.840232816526,28.3661134165298,-177.110943344657));
#151742=CARTESIAN_POINT('Ctrl Pts',(-50.3299522569454,28.8504134294547,
-177.112484691526));
#151743=CARTESIAN_POINT('Ctrl Pts',(-50.3904429224034,28.4199999799438,
-176.997671841187));
#151744=CARTESIAN_POINT('Ctrl Pts',(-50.8250862913143,28.41999998,-176.981217345763));
#151745=CARTESIAN_POINT('Ctrl Pts',(-50.3299522569362,28.85041342952,-176.84995));
#151746=CARTESIAN_POINT('Ctrl Pts',(-50.3904429223989,28.41999998,-176.84995));
#151747=CARTESIAN_POINT('Ctrl Pts',(-50.825086291307,28.41999998,-176.84995));
#151748=CARTESIAN_POINT('Origin',(-50.9656271260094,27.91999998,-177.84995));
#151749=CARTESIAN_POINT('Origin',(-53.107614345321,12.6789689739766,-177.84995));
#151750=CARTESIAN_POINT('Origin',(-51.0358975433606,27.41999998,-177.84995));
#151751=CARTESIAN_POINT('',(-51.0717059287548,27.1652100787588,-177.34995));
#151752=CARTESIAN_POINT('Ctrl Pts',(-50.6813043436922,26.35041342952,-176.84995));
#151753=CARTESIAN_POINT('Ctrl Pts',(-50.6012541744525,26.9199999800001,
-176.84995));
#151754=CARTESIAN_POINT('Ctrl Pts',(-51.176438378063,26.91999998,-176.84995));
#151755=CARTESIAN_POINT('Ctrl Pts',(-50.681304343683,26.3504134295853,-177.112484691526));
#151756=CARTESIAN_POINT('Ctrl Pts',(-50.6012541744552,26.9199999799806,
-176.958917254526));
#151757=CARTESIAN_POINT('Ctrl Pts',(-51.1764383780557,26.91999998,-176.981217345763));
#151758=CARTESIAN_POINT('Ctrl Pts',(-50.6661578184733,26.4581865564618,
-177.371936689315));
#151759=CARTESIAN_POINT('Ctrl Pts',(-50.5965693573617,26.9533341856637,
-177.069891898465));
#151760=CARTESIAN_POINT('Ctrl Pts',(-51.161291852844,26.9738865434699,-177.110943344657));
#151761=CARTESIAN_POINT('Ctrl Pts',(-50.6141239540097,26.8284267402052,
-177.742176873059));
#151762=CARTESIAN_POINT('Ctrl Pts',(-50.5759178325036,27.1002774203984,
-177.257255781812));
#151763=CARTESIAN_POINT('Ctrl Pts',(-51.1092579883806,27.1590066353435,
-177.29606343653));
#151764=CARTESIAN_POINT('Ctrl Pts',(-50.5776603536751,27.0878787379949,
-177.849949999941));
#151765=CARTESIAN_POINT('Ctrl Pts',(-50.5600601550379,27.2131106584802,
-177.331204220089));
#151766=CARTESIAN_POINT('Ctrl Pts',(-51.0727943880466,27.2887326342368,
-177.34995));
#151767=CARTESIAN_POINT('Ctrl Pts',(-50.5407635089898,27.3504134295199,
-177.84995));
#151768=CARTESIAN_POINT('Ctrl Pts',(-50.5407635089898,27.35041342952,-177.34995));
#151769=CARTESIAN_POINT('Ctrl Pts',(-51.0358975433606,27.41999998,-177.34995));
#151770=CARTESIAN_POINT('Origin',(-51.6222122422086,12.4702093225365,-172.64995));
#151771=CARTESIAN_POINT('',(-49.6109861057109,26.78082687904,-171.64995));
#151772=CARTESIAN_POINT('Ctrl Pts',(-51.6159008944631,19.70041342952,-177.84995));
#151773=CARTESIAN_POINT('Ctrl Pts',(-51.6159008944631,19.70041342952,-177.34995));
#151774=CARTESIAN_POINT('Ctrl Pts',(-52.1110349288339,19.76999998,-177.34995));
#151775=CARTESIAN_POINT('Ctrl Pts',(-51.5790040497779,19.9629481210451,
-177.849949999941));
#151776=CARTESIAN_POINT('Ctrl Pts',(-51.5974634812487,19.8316024412644,
-177.367861075732));
#151777=CARTESIAN_POINT('Ctrl Pts',(-52.0741380841476,19.9012673257632,
-177.34995));
#151778=CARTESIAN_POINT('Ctrl Pts',(-51.5425404494433,20.2224001188348,
-177.742176873059));
#151779=CARTESIAN_POINT('Ctrl Pts',(-51.5765113276013,19.980684760958,-177.329589659683));
#151780=CARTESIAN_POINT('Ctrl Pts',(-52.0376744838139,20.0309933246565,
-177.29606343653));
#151781=CARTESIAN_POINT('Ctrl Pts',(-51.4905065849796,20.5926403025782,
-177.371936689315));
#151782=CARTESIAN_POINT('Ctrl Pts',(-51.5456194237325,20.2004920783894,
-177.142957948484));
#151783=CARTESIAN_POINT('Ctrl Pts',(-51.9856406193506,20.2161134165301,
-177.110943344657));
#151784=CARTESIAN_POINT('Ctrl Pts',(-51.4753600597699,20.7004134294547,
-177.112484691526));
#151785=CARTESIAN_POINT('Ctrl Pts',(-51.5358507252279,20.2699999799402,
-176.997671841189));
#151786=CARTESIAN_POINT('Ctrl Pts',(-51.9704940941388,20.26999998,-176.981217345763));
#151787=CARTESIAN_POINT('Ctrl Pts',(-51.4753600597607,20.70041342952,-176.84995));
#151788=CARTESIAN_POINT('Ctrl Pts',(-51.5358507252234,20.26999998,-176.84995));
#151789=CARTESIAN_POINT('Ctrl Pts',(-51.9704940941315,20.26999998,-176.84995));
#151790=CARTESIAN_POINT('Origin',(-52.1110349288339,19.76999998,-177.84995));
#151791=CARTESIAN_POINT('Origin',(-53.107614345321,12.6789689739766,-177.84995));
#151792=CARTESIAN_POINT('Origin',(-52.1813053461851,19.26999998,-177.84995));
#151793=CARTESIAN_POINT('',(-51.0717059287548,27.1652100787588,-177.34995));
#151794=CARTESIAN_POINT('Ctrl Pts',(-51.8267121465167,18.20041342952,-176.84995));
#151795=CARTESIAN_POINT('Ctrl Pts',(-51.746661977277,18.76999998,-176.84995));
#151796=CARTESIAN_POINT('Ctrl Pts',(-52.3218461808875,18.76999998,-176.84995));
#151797=CARTESIAN_POINT('Ctrl Pts',(-51.8267121465076,18.2004134295853,
-177.112484691526));
#151798=CARTESIAN_POINT('Ctrl Pts',(-51.7466619772798,18.7699999799806,
-176.958917254526));
#151799=CARTESIAN_POINT('Ctrl Pts',(-52.3218461808802,18.76999998,-176.981217345763));
#151800=CARTESIAN_POINT('Ctrl Pts',(-51.8115656212979,18.3081865564618,
-177.371936689315));
#151801=CARTESIAN_POINT('Ctrl Pts',(-51.7419771601862,18.8033341856637,
-177.069891898465));
#151802=CARTESIAN_POINT('Ctrl Pts',(-52.3066996556685,18.8238865434699,
-177.110943344657));
#151803=CARTESIAN_POINT('Ctrl Pts',(-51.7595317568342,18.6784267402051,
-177.742176873059));
#151804=CARTESIAN_POINT('Ctrl Pts',(-51.721325635328,18.9502774203983,-177.257255781811));
#151805=CARTESIAN_POINT('Ctrl Pts',(-52.2546657912052,19.0090066353435,
-177.29606343653));
#151806=CARTESIAN_POINT('Ctrl Pts',(-51.7230681564996,18.9378787379949,
-177.849949999941));
#151807=CARTESIAN_POINT('Ctrl Pts',(-51.7054679578625,19.0631106584802,
-177.331204220089));
#151808=CARTESIAN_POINT('Ctrl Pts',(-52.2182021908711,19.1387326342368,
-177.34995));
#151809=CARTESIAN_POINT('Ctrl Pts',(-51.6861713118143,19.20041342952,-177.84995));
#151810=CARTESIAN_POINT('Ctrl Pts',(-51.6861713118143,19.2004134295199,
-177.34995));
#151811=CARTESIAN_POINT('Ctrl Pts',(-52.1813053461851,19.26999998,-177.34995));
#151812=CARTESIAN_POINT('Origin',(-51.6222122422086,12.4702093225365,-172.64995));
#151813=CARTESIAN_POINT('',(-50.9867892914963,16.9914785469432,-171.64995));
#151814=CARTESIAN_POINT('Origin',(-50.9867892914963,16.9914785469432,-172.64995));
#151815=CARTESIAN_POINT('',(-50.7563939085354,18.6308268790399,-171.64995));
#151816=CARTESIAN_POINT('Ctrl Pts',(-52.1126146143195,13.5388501432916,
-171.391638125813));
#151817=CARTESIAN_POINT('Ctrl Pts',(-52.4864722882118,13.5059760932665,
-171.679515584751));
#151818=CARTESIAN_POINT('Ctrl Pts',(-52.5050296388285,13.3739336825608,
-172.133326251627));
#151819=CARTESIAN_POINT('Ctrl Pts',(-51.9336694513028,14.1125756396742,
-171.482621144035));
#151820=CARTESIAN_POINT('Ctrl Pts',(-52.3988291636435,14.129589328176,-171.781794156641));
#151821=CARTESIAN_POINT('Ctrl Pts',(-52.4188787332531,13.9869292276479,
-172.315208572937));
#151822=CARTESIAN_POINT('Ctrl Pts',(-51.7497860966453,14.6887611591208,
-171.543915907757));
#151823=CARTESIAN_POINT('Ctrl Pts',(-52.3125022740344,14.7438370647052,
-171.821280489149));
#151824=CARTESIAN_POINT('Ctrl Pts',(-52.3315472405275,14.6083250867988,
-172.437881815118));
#151825=CARTESIAN_POINT('Ctrl Pts',(-51.3741578990745,15.8404043177988,
-171.628003076365));
#151826=CARTESIAN_POINT('Ctrl Pts',(-52.1416679592957,15.9593863754288,
-171.81403941883));
#151827=CARTESIAN_POINT('Ctrl Pts',(-52.1554800333145,15.861108362107,-172.606056153125));
#151828=CARTESIAN_POINT('Ctrl Pts',(-51.1823572933404,16.4160730441958,
-171.64995));
#151829=CARTESIAN_POINT('Ctrl Pts',(-52.0557320324868,16.5708522670934,
-171.757498535929));
#151830=CARTESIAN_POINT('Ctrl Pts',(-52.0666747393889,16.4929908616926,
-172.649949997757));
#151831=CARTESIAN_POINT('Ctrl Pts',(-50.9867892914963,16.9914785469432,
-171.64995));
#151832=CARTESIAN_POINT('Ctrl Pts',(-51.9770573602378,17.1306516479032,
-171.64995));
#151833=CARTESIAN_POINT('Ctrl Pts',(-51.9770573602378,17.1306516479033,
-172.64995));
#151834=CARTESIAN_POINT('',(-52.1126146143195,13.5388501432916,-171.391638125813));
#151835=CARTESIAN_POINT('Origin',(-51.5147615700869,13.2347605816008,-172.133326251627));
#151836=CARTESIAN_POINT('Ctrl Pts',(-52.1126146143195,13.5388501432916,
-171.391638125813));
#151837=CARTESIAN_POINT('Ctrl Pts',(-51.9336694513434,14.1125756396757,
-171.482621144061));
#151838=CARTESIAN_POINT('Ctrl Pts',(-51.7497860966928,14.6887611591254,
-171.54391590778));
#151839=CARTESIAN_POINT('Ctrl Pts',(-51.3741578991343,15.8404043178081,
-171.628003076379));
#151840=CARTESIAN_POINT('Ctrl Pts',(-51.1823572934054,16.4160730442074,
-171.649950000008));
#151841=CARTESIAN_POINT('Ctrl Pts',(-50.9867892914963,16.9914785469432,
-171.64995));
#151842=CARTESIAN_POINT('Ctrl Pts',(-53.1963133798215,12.11999998,-176.84995));
#151843=CARTESIAN_POINT('Ctrl Pts',(-52.8383133487074,12.11999998,-176.84995));
#151844=CARTESIAN_POINT('Ctrl Pts',(-52.7229737572976,12.4589111791821,
-176.84995));
#151845=CARTESIAN_POINT('Ctrl Pts',(-53.1963133903003,12.11999998,-176.935788696125));
#151846=CARTESIAN_POINT('Ctrl Pts',(-52.8383133592413,12.1199999570555,
-176.956623424753));
#151847=CARTESIAN_POINT('Ctrl Pts',(-52.7229737689762,12.4589111448658,
-177.021627393075));
#151848=CARTESIAN_POINT('Ctrl Pts',(-53.2113113817619,12.0970286741326,
-177.021779308321));
#151849=CARTESIAN_POINT('Ctrl Pts',(-52.8537691267412,12.0857563897115,
-177.064307914426));
#151850=CARTESIAN_POINT('Ctrl Pts',(-52.7396382131267,12.4078638336875,
-177.193608615338));
#151851=CARTESIAN_POINT('Ctrl Pts',(-53.2731270360347,12.0145014233151,
-177.168462633103));
#151852=CARTESIAN_POINT('Ctrl Pts',(-52.9137267746853,11.9605670475505,
-177.241607460489));
#151853=CARTESIAN_POINT('Ctrl Pts',(-52.8083222549725,12.2244699412272,
-177.486975267512));
#151854=CARTESIAN_POINT('Ctrl Pts',(-53.3209180569567,11.9546120038032,
-177.230014853822));
#151855=CARTESIAN_POINT('Ctrl Pts',(-52.9598970865314,11.8669832265648,
-177.312681927597));
#151856=CARTESIAN_POINT('Ctrl Pts',(-52.8614762873877,12.0912699189313,
-177.610143591528));
#151857=CARTESIAN_POINT('Ctrl Pts',(-53.3846587239315,11.8868850448361,
-177.272764808359));
#151858=CARTESIAN_POINT('Ctrl Pts',(-53.0160258826804,11.7628399725939,
-177.351063336446));
#151859=CARTESIAN_POINT('Ctrl Pts',(-52.9322463618642,11.9408779899289,
-177.695579616717));
#151860=CARTESIAN_POINT('Origin',(-53.3846587239314,12.1537701096722,-177.695579616717));
#151861=CARTESIAN_POINT('Ctrl Pts',(-52.5050296388285,13.3739336825608,
-172.133326251627));
#151862=CARTESIAN_POINT('Ctrl Pts',(-52.4864722882118,13.5059760932666,
-171.679515584751));
#151863=CARTESIAN_POINT('Ctrl Pts',(-52.1126146143195,13.5388501432916,
-171.391638125813));
#151864=CARTESIAN_POINT('Ctrl Pts',(-52.5511257748791,13.045942631788,-172.016544094259));
#151865=CARTESIAN_POINT('Ctrl Pts',(-52.5259488232545,13.1630178119759,
-171.621133646225));
#151866=CARTESIAN_POINT('Ctrl Pts',(-52.2275734081837,13.1702746923549,
-171.333188379966));
#151867=CARTESIAN_POINT('Ctrl Pts',(-52.6287970696452,12.7242148673197,
-171.90506362857));
#151868=CARTESIAN_POINT('Ctrl Pts',(-52.6036316644729,12.8055197818763,
-171.550813695775));
#151869=CARTESIAN_POINT('Ctrl Pts',(-52.3625569744519,12.7995634785289,
-171.277518845311));
#151870=CARTESIAN_POINT('Ctrl Pts',(-52.7423614633688,12.4030287528935,
-171.844601961512));
#151871=CARTESIAN_POINT('Ctrl Pts',(-52.7259743335333,12.4493753091149,
-171.512222020089));
#151872=CARTESIAN_POINT('Ctrl Pts',(-52.521634376552,12.4186874453849,-171.247275980756));
#151873=CARTESIAN_POINT('Ctrl Pts',(-52.5103993792155,12.4456688476555,
-171.249463186897));
#151874=CARTESIAN_POINT('Ctrl Pts',(-52.3561903484674,12.8170807700125,
-171.280152290009));
#151875=CARTESIAN_POINT('Ctrl Pts',(-52.2248583846995,13.1789834261216,
-171.33457063385));
#151876=CARTESIAN_POINT('Ctrl Pts',(-52.1126146143195,13.5388501432916,
-171.391638125813));
#151877=CARTESIAN_POINT('Ctrl Pts',(-53.3764151395101,11.8956579446144,
-177.267099525666));
#151878=CARTESIAN_POINT('Ctrl Pts',(-53.0100887119116,11.775605096064,-177.346426173794));
#151879=CARTESIAN_POINT('Ctrl Pts',(-52.9240620597106,11.958262205024,-177.68425748122));
#151880=CARTESIAN_POINT('Ctrl Pts',(-53.456953595738,11.8101639377045,-177.323569657212));
#151881=CARTESIAN_POINT('Ctrl Pts',(-53.0700075125763,11.6468244366821,
-177.3949635665));
#151882=CARTESIAN_POINT('Ctrl Pts',(-53.0038949723879,11.7887688205011,
-177.797166892916));
#151883=CARTESIAN_POINT('Ctrl Pts',(-53.5494992446435,11.7107497255641,
-177.351908350358));
#151884=CARTESIAN_POINT('Ctrl Pts',(-53.1326802282722,11.5106994843395,
-177.38870977272));
#151885=CARTESIAN_POINT('Ctrl Pts',(-53.0956839028775,11.5915634526764,
-177.853871009894));
#151886=CARTESIAN_POINT('Ctrl Pts',(-53.6420451768198,11.6097057706468,
-177.349844870837));
#151887=CARTESIAN_POINT('Ctrl Pts',(-53.1835178900119,11.3997623969134,
-177.345484998328));
#151888=CARTESIAN_POINT('Ctrl Pts',(-53.1874365908317,11.3912058852591,
-177.849739369046));
#151889=CARTESIAN_POINT('Origin',(-53.6325912458891,11.61999998,-177.84995));
#151890=CARTESIAN_POINT('Origin',(0.,-12.9675000200281,-177.84995));
#151891=CARTESIAN_POINT('Origin',(-53.8590042959267,11.11999998,-177.84995));
#151892=CARTESIAN_POINT('Origin',(0.,-12.9675000200281,-177.34995));
#151893=CARTESIAN_POINT('Ctrl Pts',(-53.8590042959257,11.1199999800011,
-177.34995));
#151894=CARTESIAN_POINT('Ctrl Pts',(-53.4025720561301,10.9158686240688,
-177.34995));
#151895=CARTESIAN_POINT('Ctrl Pts',(-53.4025720561297,10.9158686240697,
-177.84995));
#151896=CARTESIAN_POINT('Ctrl Pts',(-53.9152095126149,11.0571633006792,
-177.34995));
#151897=CARTESIAN_POINT('Ctrl Pts',(-53.4357429270681,10.8416994438452,
-177.323612898224));
#151898=CARTESIAN_POINT('Ctrl Pts',(-53.4583000366404,10.7912623535259,
-177.849949984912));
#151899=CARTESIAN_POINT('Ctrl Pts',(-53.9700011606116,10.9953079956486,
-177.338340413074));
#151900=CARTESIAN_POINT('Ctrl Pts',(-53.4634087021834,10.7796461652398,
-177.282275394088));
#151901=CARTESIAN_POINT('Ctrl Pts',(-53.5126282698489,10.6685980808388,
-177.826730821509));
#151902=CARTESIAN_POINT('Ctrl Pts',(-54.0742219292009,10.8766241714759,
-177.291358543608));
#151903=CARTESIAN_POINT('Ctrl Pts',(-53.5073796187504,10.6816635307577,
-177.18321412648));
#151904=CARTESIAN_POINT('Ctrl Pts',(-53.6159658107279,10.4332420187126,
-177.732767091856));
#151905=CARTESIAN_POINT('Ctrl Pts',(-54.1215658763003,10.8221729031368,
-177.256908861057));
#151906=CARTESIAN_POINT('Ctrl Pts',(-53.5219518286219,10.649686808137,-177.127170956772));
#151907=CARTESIAN_POINT('Ctrl Pts',(-53.6629085389549,10.3252623899094,
-177.663867719202));
#151908=CARTESIAN_POINT('Ctrl Pts',(-54.2036611796727,10.7271494012897,
-177.166153898004));
#151909=CARTESIAN_POINT('Ctrl Pts',(-53.5394251697822,10.6131024574854,
-177.020421798311));
#151910=CARTESIAN_POINT('Ctrl Pts',(-53.7443081182388,10.1368259480206,
-177.482357798918));
#151911=CARTESIAN_POINT('Ctrl Pts',(-54.2369068974943,10.6883272976786,
-177.111149481396));
#151912=CARTESIAN_POINT('Ctrl Pts',(-53.5413185515592,10.6107526879388,
-176.973405437982));
#151913=CARTESIAN_POINT('Ctrl Pts',(-53.7772720937282,10.0598397490546,
-177.372348961349));
#151914=CARTESIAN_POINT('Ctrl Pts',(-54.282897054019,10.6344777440414,-176.987189324297));
#151915=CARTESIAN_POINT('Ctrl Pts',(-53.5410688387025,10.6146700040362,
-176.899444869037));
#151916=CARTESIAN_POINT('Ctrl Pts',(-53.8228725022638,9.95305333910152,
-177.124428650036));
#151917=CARTESIAN_POINT('Ctrl Pts',(-54.2951871094022,10.61999998,-176.919796282647));
#151918=CARTESIAN_POINT('Ctrl Pts',(-53.5392499462662,10.6199999783344,
-176.8744703999));
#151919=CARTESIAN_POINT('Ctrl Pts',(-53.8350584050868,9.92434321115133,
-176.989642564215));
#151920=CARTESIAN_POINT('Ctrl Pts',(-54.2951871140408,10.61999998,-176.84995));
#151921=CARTESIAN_POINT('Ctrl Pts',(-53.5392499457278,10.61999998,-176.84995));
#151922=CARTESIAN_POINT('Ctrl Pts',(-53.8350584096845,9.92434320033874,
-176.84995));
#151923=CARTESIAN_POINT('Origin',(0.,-12.9675000200281,-171.871644662643));
#151924=CARTESIAN_POINT('Origin',(0.,-12.9675000200281,-171.449026400902));
#151925=CARTESIAN_POINT('Ctrl Pts',(-56.3647818444065,3.96926413137802,
-176.823236869191));
#151926=CARTESIAN_POINT('Ctrl Pts',(-55.9959340274937,3.96888359130611,
-176.817122088667));
#151927=CARTESIAN_POINT('Ctrl Pts',(-55.8870828276465,4.32076528003782,
-176.796522687734));
#151928=CARTESIAN_POINT('Ctrl Pts',(-56.3621914406401,3.97343752384164,
-176.898676428268));
#151929=CARTESIAN_POINT('Ctrl Pts',(-55.9940683565767,3.97509020000321,
-176.909738482033));
#151930=CARTESIAN_POINT('Ctrl Pts',(-55.8845144046578,4.32904163576369,
-176.94740476072));
#151931=CARTESIAN_POINT('Ctrl Pts',(-56.3706829146393,3.95977275889743,
-176.975561795614));
#151932=CARTESIAN_POINT('Ctrl Pts',(-56.0002448138047,3.95455861174371,
-177.005108600189));
#151933=CARTESIAN_POINT('Ctrl Pts',(-55.8929338246199,4.30194256512436,
-177.101178646029));
#151934=CARTESIAN_POINT('Ctrl Pts',(-56.4046489137991,3.9046063492797,-177.105916142434));
#151935=CARTESIAN_POINT('Ctrl Pts',(-56.0238513574191,3.87557171406294,
-177.159000770829));
#151936=CARTESIAN_POINT('Ctrl Pts',(-55.9266115295683,4.19254080857125,
-177.361891255001));
#151937=CARTESIAN_POINT('Ctrl Pts',(-56.4280565527281,3.86646604036506,
-177.161475370894));
#151938=CARTESIAN_POINT('Ctrl Pts',(-56.0401276640061,3.82096319617762,
-177.221565174049));
#151939=CARTESIAN_POINT('Ctrl Pts',(-55.9498205047936,4.11690393979646,
-177.473010794577));
#151940=CARTESIAN_POINT('Ctrl Pts',(-56.4844776989127,3.77353560122462,
-177.252565826982));
#151941=CARTESIAN_POINT('Ctrl Pts',(-56.0775874017679,3.6944039842704,-177.314195789872));
#151942=CARTESIAN_POINT('Ctrl Pts',(-56.0057627129126,3.93261288273155,
-177.655191732052));
#151943=CARTESIAN_POINT('Ctrl Pts',(-56.5179433552169,3.71797632916513,
-177.288846704038));
#151944=CARTESIAN_POINT('Ctrl Pts',(-56.0992917633819,3.62064831431513,
-177.344699390005));
#151945=CARTESIAN_POINT('Ctrl Pts',(-56.0389442880078,3.82243329271981,
-177.727752411286));
#151946=CARTESIAN_POINT('Ctrl Pts',(-56.5933952273326,3.59109438829976,
-177.340494166071));
#151947=CARTESIAN_POINT('Ctrl Pts',(-56.1453765257444,3.46307334244855,
-177.373495736382));
#151948=CARTESIAN_POINT('Ctrl Pts',(-56.1137555688082,3.57081571968701,
-177.8310434768));
#151949=CARTESIAN_POINT('Ctrl Pts',(-56.6369998249196,3.51682557412558,
-177.353132613067));
#151950=CARTESIAN_POINT('Ctrl Pts',(-56.1703907360266,3.37693361833867,
-177.366019145535));
#151951=CARTESIAN_POINT('Ctrl Pts',(-56.1569874820333,3.42354388148881,
-177.856317178204));
#151952=CARTESIAN_POINT('Ctrl Pts',(-56.6789110795914,3.44432084323002,
-177.349268724474));
#151953=CARTESIAN_POINT('Ctrl Pts',(-56.1915749927218,3.30386891072904,
-177.341992013576));
#151954=CARTESIAN_POINT('Ctrl Pts',(-56.1985461365938,3.27975188714757,
-177.848586370252));
#151955=CARTESIAN_POINT('Origin',(-56.6639973329545,3.46999998000001,-177.84995));
#151956=CARTESIAN_POINT('Origin',(0.,-12.9675000200281,-177.84995));
#151957=CARTESIAN_POINT('',(-56.8066553649227,2.96999998000001,-177.34995));
#151958=CARTESIAN_POINT('Origin',(-56.8066553649227,2.96999998000001,-177.84995));
#151959=CARTESIAN_POINT('Origin',(0.,-12.9675000200281,-177.34995));
#151960=CARTESIAN_POINT('Ctrl Pts',(-56.8066553649227,2.96999998000003,
-177.34995));
#151961=CARTESIAN_POINT('Ctrl Pts',(-56.3252430313216,2.83493642067775,
-177.34995));
#151962=CARTESIAN_POINT('Ctrl Pts',(-56.3252430313217,2.83493642067777,
-177.84995));
#151963=CARTESIAN_POINT('Ctrl Pts',(-56.8796685247676,2.83987814625872,
-177.34995));
#151964=CARTESIAN_POINT('Ctrl Pts',(-56.3657038976309,2.69072016585578,
-177.313059794074));
#151965=CARTESIAN_POINT('Ctrl Pts',(-56.3976379760506,2.57689628418379,
-177.849949962148));
#151966=CARTESIAN_POINT('Ctrl Pts',(-56.9495585329053,2.71140496526165,
-177.298153784266));
#151967=CARTESIAN_POINT('Ctrl Pts',(-56.393446522619,2.59195606221812,-177.219869815671));
#151968=CARTESIAN_POINT('Ctrl Pts',(-56.4669147992933,2.32220551629932,
-177.746434148089));
#151969=CARTESIAN_POINT('Ctrl Pts',(-57.,2.61702308584988,-177.204078948543));
#151970=CARTESIAN_POINT('Ctrl Pts',(-56.409292540301,2.5378414548249,-177.125154911669));
#151971=CARTESIAN_POINT('Ctrl Pts',(-56.5169491525424,2.13496529160036,
-177.558207897086));
#151972=CARTESIAN_POINT('Origin',(-57.,2.26404619169977,-177.558207897086));
#151973=CARTESIAN_POINT('Ctrl Pts',(-57.,2.61702308584989,-177.204078948543));
#151974=CARTESIAN_POINT('Ctrl Pts',(-56.9495585329053,2.71140496526165,
-177.298153784266));
#151975=CARTESIAN_POINT('Ctrl Pts',(-56.8796685247676,2.83987814625872,
-177.34995));
#151976=CARTESIAN_POINT('Ctrl Pts',(-56.8066553649227,2.96999998000001,
-177.34995));
#151977=CARTESIAN_POINT('Ctrl Pts',(-57.,2.61702308584989,-177.204078948543));
#151978=CARTESIAN_POINT('Ctrl Pts',(-56.409292540301,2.53784145482491,-177.125154911669));
#151979=CARTESIAN_POINT('Ctrl Pts',(-56.5169491525423,2.13496529160038,
-177.558207897086));
#151980=CARTESIAN_POINT('Ctrl Pts',(-57.043897408659,2.52469464001198,-177.112050866152));
#151981=CARTESIAN_POINT('Ctrl Pts',(-56.4267635932219,2.4778594556634,-177.032282865396));
#151982=CARTESIAN_POINT('Ctrl Pts',(-56.5659347005564,1.95164994081541,
-177.37392715461));
#151983=CARTESIAN_POINT('Ctrl Pts',(-57.0736014896981,2.46999998000001,
-176.982739539051));
#151984=CARTESIAN_POINT('Ctrl Pts',(-56.4314543935154,2.46472012384626,
-176.935564924353));
#151985=CARTESIAN_POINT('Ctrl Pts',(-56.5940537017931,1.84341101199667,
-177.116606872607));
#151986=CARTESIAN_POINT('Ctrl Pts',(-57.077763566464,2.46999998000001,-176.848740272858));
#151987=CARTESIAN_POINT('Ctrl Pts',(-56.430072632376,2.46999998,-176.848740272858));
#151988=CARTESIAN_POINT('Ctrl Pts',(-56.5940537057312,1.84341099694892,
-176.848740272858));
#151989=CARTESIAN_POINT('Origin',(0.,-12.9675000200281,-171.871644662643));
#151990=CARTESIAN_POINT('Origin',(0.,-12.9675000200281,-171.449026400902));
#151991=CARTESIAN_POINT('Ctrl Pts',(-58.2644174754153,-4.18000001999999,
-176.647241333324));
#151992=CARTESIAN_POINT('Ctrl Pts',(-57.8378063278744,-4.18000001999999,
-176.647241333323));
#151993=CARTESIAN_POINT('Ctrl Pts',(-57.7706512256236,-3.75870764711888,
-176.647241333324));
#151994=CARTESIAN_POINT('Ctrl Pts',(-58.2063099446428,-4.18000001999999,
-176.814456128226));
#151995=CARTESIAN_POINT('Ctrl Pts',(-57.8302553406283,-4.13262948514164,
-176.819875027464));
#151996=CARTESIAN_POINT('Ctrl Pts',(-57.7706512234859,-3.7587076337082,
-176.91349018761));
#151997=CARTESIAN_POINT('Ctrl Pts',(-58.1740867503666,-4.22134717274183,
-176.965019674666));
#151998=CARTESIAN_POINT('Ctrl Pts',(-57.8337414661451,-4.15737968364172,
-177.016619266697));
#151999=CARTESIAN_POINT('Ctrl Pts',(-57.7839302828914,-3.84070116554495,
-177.179630564281));
#152000=CARTESIAN_POINT('Ctrl Pts',(-58.1596733704946,-4.39698767568444,
-177.184652644663));
#152001=CARTESIAN_POINT('Ctrl Pts',(-57.8638647108401,-4.36170500598442,
-177.299461859543));
#152002=CARTESIAN_POINT('Ctrl Pts',(-57.8378689508709,-4.18900518947036,
-177.581280960616));
#152003=CARTESIAN_POINT('Ctrl Pts',(-58.1766173277935,-4.52496538336098,
-177.243973427637));
#152004=CARTESIAN_POINT('Ctrl Pts',(-57.8889218715383,-4.53236075126195,
-177.380206838676));
#152005=CARTESIAN_POINT('Ctrl Pts',(-57.8761547096863,-4.44264996470081,
-177.698192218067));
#152006=CARTESIAN_POINT('Ctrl Pts',(-58.2078173720827,-4.6591771252004,
-177.236349008085));
#152007=CARTESIAN_POINT('Ctrl Pts',(-57.9133432880527,-4.70343927025971,
-177.368016692624));
#152008=CARTESIAN_POINT('Ctrl Pts',(-57.914127722791,-4.70894021166886,
-177.693561815623));
#152009=CARTESIAN_POINT('Origin',(-58.4091202674301,-4.63835423039998,-177.693561815623));
#152010=CARTESIAN_POINT('Ctrl Pts',(-57.9826110754301,-5.20432973493151,
-177.68524973918));
#152011=CARTESIAN_POINT('Ctrl Pts',(-57.9819403936438,-5.19932045653815,
-177.367360689003));
#152012=CARTESIAN_POINT('Ctrl Pts',(-58.2670190981741,-5.15898893607704,
-177.232518219478));
#152013=CARTESIAN_POINT('Ctrl Pts',(-57.9604889110946,-5.0391007365056,
-177.687922734557));
#152014=CARTESIAN_POINT('Ctrl Pts',(-57.9597329881765,-5.03356356782781,
-177.367569378206));
#152015=CARTESIAN_POINT('Ctrl Pts',(-58.2478951756903,-4.99233199195458,
-177.233703806904));
#152016=CARTESIAN_POINT('Ctrl Pts',(-57.9376611104107,-4.87397087657654,
-177.690692163097));
#152017=CARTESIAN_POINT('Ctrl Pts',(-57.936860143276,-4.86824210971035,
-177.367787815378));
#152018=CARTESIAN_POINT('Ctrl Pts',(-58.2281612527228,-4.82572915883349,
-177.234977247299));
#152019=CARTESIAN_POINT('Ctrl Pts',(-57.9141277227909,-4.70894021166782,
-177.693561815623));
#152020=CARTESIAN_POINT('Ctrl Pts',(-57.9133432880526,-4.70343927025946,
-177.368016692624));
#152021=CARTESIAN_POINT('Ctrl Pts',(-58.207817372083,-4.65917712520044,
-177.236349008084));
#152022=CARTESIAN_POINT('Origin',(-58.4781889478697,-5.13797785215286,-177.68524973918));
#152023=CARTESIAN_POINT('Origin',(8.72896884135842,-12.9196247869585,-187.477148715837));
#152024=CARTESIAN_POINT('Ctrl Pts',(-58.250127507179,-5.06968783385529,
-177.226728198848));
#152025=CARTESIAN_POINT('Ctrl Pts',(-57.9662855289687,-5.08328249329522,
-177.360292478972));
#152026=CARTESIAN_POINT('Ctrl Pts',(-57.9585760313018,-5.02718307168404,
-177.669186903823));
#152027=CARTESIAN_POINT('Ctrl Pts',(-58.267275359726,-5.17241111264655,
-177.245973878017));
#152028=CARTESIAN_POINT('Ctrl Pts',(-57.984552359372,-5.21769695918899,
-177.385890323218));
#152029=CARTESIAN_POINT('Ctrl Pts',(-57.986638158118,-5.23110018896161,
-177.710636685369));
#152030=CARTESIAN_POINT('Ctrl Pts',(-58.2949532186373,-5.28245544896484,
-177.219964260301));
#152031=CARTESIAN_POINT('Ctrl Pts',(-58.0035760854518,-5.36150223388792,
-177.347296528341));
#152032=CARTESIAN_POINT('Ctrl Pts',(-58.0151803280234,-5.44931573531903,
-177.670490460791));
#152033=CARTESIAN_POINT('Ctrl Pts',(-58.3517502627772,-5.44113379045571,
-177.116208062583));
#152034=CARTESIAN_POINT('Ctrl Pts',(-58.0288335651954,-5.55441367376,-177.210693506391));
#152035=CARTESIAN_POINT('Ctrl Pts',(-58.0549536715593,-5.76404075854571,
-177.499799765465));
#152036=CARTESIAN_POINT('Ctrl Pts',(-58.3785597083963,-5.49933671141672,
-177.055067358297));
#152037=CARTESIAN_POINT('Ctrl Pts',(-58.0374810804384,-5.6211131042901,
-177.130197562223));
#152038=CARTESIAN_POINT('Ctrl Pts',(-58.0690822624578,-5.87947228735883,
-177.397969070777));
#152039=CARTESIAN_POINT('Ctrl Pts',(-58.4367803399072,-5.59139596273917,
-176.908361465886));
#152040=CARTESIAN_POINT('Ctrl Pts',(-58.049441388405,-5.71232355105524,
-176.947605119838));
#152041=CARTESIAN_POINT('Ctrl Pts',(-58.0910734645313,-6.0620213485957,
-177.158256835825));
#152042=CARTESIAN_POINT('Ctrl Pts',(-58.4681676012925,-5.62547497424865,
-176.823186408681));
#152043=CARTESIAN_POINT('Ctrl Pts',(-58.0527112965688,-5.73640373079481,
-176.8437834687));
#152044=CARTESIAN_POINT('Ctrl Pts',(-58.0990088104622,-6.12958052854701,
-177.021022282342));
#152045=CARTESIAN_POINT('Ctrl Pts',(-58.549399705635,-5.67884101979599,
-176.597416893918));
#152046=CARTESIAN_POINT('Ctrl Pts',(-58.0542110412498,-5.74228297193106,
-176.586646322505));
#152047=CARTESIAN_POINT('Ctrl Pts',(-58.1113726902199,-6.23532200623141,
-176.671138683684));
#152048=CARTESIAN_POINT('Ctrl Pts',(-58.5996921096123,-5.68603239881912,
-176.453921402976));
#152049=CARTESIAN_POINT('Ctrl Pts',(-58.0492158141453,-5.69790226417634,
-176.435349477229));
#152050=CARTESIAN_POINT('Ctrl Pts',(-58.1129608923341,-6.24950165634564,
-176.458921147922));
#152051=CARTESIAN_POINT('Ctrl Pts',(-58.6547670071737,-5.67538447778071,
-176.294472036962));
#152052=CARTESIAN_POINT('Ctrl Pts',(-58.0397058063333,-5.61759270411258,
-176.307417995075));
#152053=CARTESIAN_POINT('Ctrl Pts',(-58.1105363664048,-6.22828871330273,
-176.243722845542));
#152054=CARTESIAN_POINT('Origin',(0.,-12.9675000200281,-171.871644662643));
#152055=CARTESIAN_POINT('Origin',(0.,-12.9675000200281,-171.449026400902));
#152056=CARTESIAN_POINT('Ctrl Pts',(-58.9890336736409,-12.33000002,-176.26629097911));
#152057=CARTESIAN_POINT('Ctrl Pts',(-58.4985823439911,-12.33000002,-176.26629097911));
#152058=CARTESIAN_POINT('Ctrl Pts',(-58.48912660861,-11.8396398505087,-176.26629097911));
#152059=CARTESIAN_POINT('Ctrl Pts',(-58.9511729872876,-12.33000002,-176.394565470062));
#152060=CARTESIAN_POINT('Ctrl Pts',(-58.4978924302213,-12.2942221356206,
-176.390394119799));
#152061=CARTESIAN_POINT('Ctrl Pts',(-58.4891266082067,-11.8396398295935,
-176.423373313634));
#152062=CARTESIAN_POINT('Ctrl Pts',(-58.9148079297158,-12.3367286443605,
-176.512401023853));
#152063=CARTESIAN_POINT('Ctrl Pts',(-58.4973632374244,-12.2720420811237,
-176.51680491203));
#152064=CARTESIAN_POINT('Ctrl Pts',(-58.4893923301638,-11.8529830432079,
-176.578231191384));
#152065=CARTESIAN_POINT('Ctrl Pts',(-58.8482938287677,-12.3711206280572,
-176.731313674606));
#152066=CARTESIAN_POINT('Ctrl Pts',(-58.4968786243544,-12.2700692006727,
-176.761217862814));
#152067=CARTESIAN_POINT('Ctrl Pts',(-58.4906521273108,-11.9211841187055,
-176.880933630382));
#152068=CARTESIAN_POINT('Ctrl Pts',(-58.817725908538,-12.3995214017445,
-176.833790628028));
#152069=CARTESIAN_POINT('Ctrl Pts',(-58.4969059340918,-12.2890138650664,
-176.883349034336));
#152070=CARTESIAN_POINT('Ctrl Pts',(-58.4916809553489,-11.9775042760042,
-177.031063990607));
#152071=CARTESIAN_POINT('Ctrl Pts',(-58.7801197877863,-12.4620381958002,
-176.965157505607));
#152072=CARTESIAN_POINT('Ctrl Pts',(-58.4973396692349,-12.3546251483512,
-177.045101981496));
#152073=CARTESIAN_POINT('Ctrl Pts',(-58.4936040475389,-12.1014782716709,
-177.230049861356));
#152074=CARTESIAN_POINT('Ctrl Pts',(-58.7686983660461,-12.486608549538,
-177.006030037118));
#152075=CARTESIAN_POINT('Ctrl Pts',(-58.4975444264886,-12.3825831770725,
-177.096147908481));
#152076=CARTESIAN_POINT('Ctrl Pts',(-58.494315776837,-12.1502025268642,
-177.293200512009));
#152077=CARTESIAN_POINT('Ctrl Pts',(-58.7491768361659,-12.5414135007217,
-177.077379300711));
#152078=CARTESIAN_POINT('Ctrl Pts',(-58.4980148214299,-12.4487602363349,
-177.186076538859));
#152079=CARTESIAN_POINT('Ctrl Pts',(-58.4957333150688,-12.2588835334819,
-177.404811094274));
#152080=CARTESIAN_POINT('Ctrl Pts',(-58.7409598721377,-12.5716812769085,
-177.108237839695));
#152081=CARTESIAN_POINT('Ctrl Pts',(-58.4982801309887,-12.4869468894055,
-177.22572537075));
#152082=CARTESIAN_POINT('Ctrl Pts',(-58.4964422014533,-12.3189060674576,
-177.453832155185));
#152083=CARTESIAN_POINT('Ctrl Pts',(-58.7207402303504,-12.6723026604245,
-177.185595547246));
#152084=CARTESIAN_POINT('Ctrl Pts',(-58.4990784570061,-12.6167275534409,
-177.325053017822));
#152085=CARTESIAN_POINT('Ctrl Pts',(-58.4984277184057,-12.5184434004461,
-177.577650852379));
#152086=CARTESIAN_POINT('Ctrl Pts',(-58.71386124121,-12.7496539972645,-177.213921724807));
#152087=CARTESIAN_POINT('Ctrl Pts',(-58.499584494838,-12.7220101607261,
-177.363144865607));
#152088=CARTESIAN_POINT('Ctrl Pts',(-58.4994668010734,-12.6718351617761,
-177.62421726441));
#152089=CARTESIAN_POINT('Ctrl Pts',(-58.7141461350374,-12.8294402383603,
-177.213832217126));
#152090=CARTESIAN_POINT('Ctrl Pts',(-58.4998383709333,-12.8299842764724,
-177.363039831107));
#152091=CARTESIAN_POINT('Ctrl Pts',(-58.4998385375645,-12.8300551987826,
-177.624173936067));
#152092=CARTESIAN_POINT('Origin',(-58.9998371575436,-12.8288804567203,-177.624173936068));
#152093=CARTESIAN_POINT('Ctrl Pts',(-58.4988777713114,-13.3298527448209,
-177.624285947696));
#152094=CARTESIAN_POINT('Ctrl Pts',(-58.4988766126948,-13.3300397939931,
-177.363046991769));
#152095=CARTESIAN_POINT('Ctrl Pts',(-58.7133155825256,-13.3314748983275,
-177.213850156091));
#152096=CARTESIAN_POINT('Ctrl Pts',(-58.4999097084608,-13.1632549492482,
-177.624165638205));
#152097=CARTESIAN_POINT('Ctrl Pts',(-58.4999095201947,-13.1633713364571,
-177.363039299942));
#152098=CARTESIAN_POINT('Ctrl Pts',(-58.7142076600563,-13.1641303210821,
-177.213830854253));
#152099=CARTESIAN_POINT('Ctrl Pts',(-58.500229964035,-12.996655767065,-177.624128301462));
#152100=CARTESIAN_POINT('Ctrl Pts',(-58.5002301876544,-12.9966649765953,
-177.363036914652));
#152101=CARTESIAN_POINT('Ctrl Pts',(-58.7144845107404,-12.9967863561848,
-177.213824921703));
#152102=CARTESIAN_POINT('Ctrl Pts',(-58.4998385375645,-12.8300551987823,
-177.624173936067));
#152103=CARTESIAN_POINT('Ctrl Pts',(-58.4998383709332,-12.8299842764725,
-177.363039831106));
#152104=CARTESIAN_POINT('Ctrl Pts',(-58.7141461350386,-12.8294402383605,
-177.213832217124));
#152105=CARTESIAN_POINT('Origin',(-58.9988681796133,-13.3329497766555,-177.624285947696));
#152106=CARTESIAN_POINT('Origin',(9.53286718169884,-12.9674995361125,-178.689058801762));
#152107=CARTESIAN_POINT('Ctrl Pts',(-58.7171412311507,-13.2450064259713,
-177.201718344835));
#152108=CARTESIAN_POINT('Ctrl Pts',(-58.499487866025,-13.2129797427744,
-177.346623311491));
#152109=CARTESIAN_POINT('Ctrl Pts',(-58.4996466434616,-13.1583683303841,
-177.604649432751));
#152110=CARTESIAN_POINT('Ctrl Pts',(-58.7088369592429,-13.350481719734,
-177.231562795809));
#152111=CARTESIAN_POINT('Ctrl Pts',(-58.4989011425798,-13.3549568592449,
-177.387243781406));
#152112=CARTESIAN_POINT('Ctrl Pts',(-58.4990964462207,-13.3675412254732,
-177.653635589973));
#152113=CARTESIAN_POINT('Ctrl Pts',(-58.7142302220621,-13.4630034042927,
-177.204888879754));
#152114=CARTESIAN_POINT('Ctrl Pts',(-58.4976201073564,-13.5106559619976,
-177.34946224375));
#152115=CARTESIAN_POINT('Ctrl Pts',(-58.4969599356141,-13.5907093707611,
-177.608451413633));
#152116=CARTESIAN_POINT('Ctrl Pts',(-58.744734365864,-13.6207444397399,
-177.084931957504));
#152117=CARTESIAN_POINT('Ctrl Pts',(-58.4955856783522,-13.714544547136,
-177.195108413244));
#152118=CARTESIAN_POINT('Ctrl Pts',(-58.4926597506031,-13.9035447147552,
-177.415964369801));
#152119=CARTESIAN_POINT('Ctrl Pts',(-58.7643257211001,-13.6767548657761,
-177.011378635403));
#152120=CARTESIAN_POINT('Ctrl Pts',(-58.4947863265944,-13.7828140187279,
-177.100057626205));
#152121=CARTESIAN_POINT('Ctrl Pts',(-58.4906864354198,-14.0146226773921,
-177.299459860577));
#152122=CARTESIAN_POINT('Ctrl Pts',(-58.8477271879271,-13.8175445314543,
-176.717566432405));
#152123=CARTESIAN_POINT('Ctrl Pts',(-58.4932080623643,-13.9334183953258,
-176.732015957667));
#152124=CARTESIAN_POINT('Ctrl Pts',(-58.4852925969465,-14.2938175741563,
-176.853564982499));
#152125=CARTESIAN_POINT('Ctrl Pts',(-58.9364557612147,-13.8384035340429,
-176.439823404047));
#152126=CARTESIAN_POINT('Ctrl Pts',(-58.4944709305922,-13.886285675068,
-176.399510353928));
#152127=CARTESIAN_POINT('Ctrl Pts',(-58.4839076510609,-14.3351427387709,
-176.459952278612));
#152128=CARTESIAN_POINT('Ctrl Pts',(-59.0262805694248,-13.8273207647541,
-176.128850259174));
#152129=CARTESIAN_POINT('Ctrl Pts',(-58.4967342962639,-13.7830237188745,
-176.132987895578));
#152130=CARTESIAN_POINT('Ctrl Pts',(-58.4845502518446,-14.3131195259793,
-176.102153175423));
#152131=CARTESIAN_POINT('Origin',(0.,-12.9675000200281,-171.871644662643));
#152132=CARTESIAN_POINT('Origin',(0.,-12.9675000200281,-171.449026400902));
#152133=CARTESIAN_POINT('Ctrl Pts',(-58.627582591745,-20.4849178106967,
-176.310058991613));
#152134=CARTESIAN_POINT('Ctrl Pts',(-58.0107588300312,-20.5427919605405,
-176.323555907706));
#152135=CARTESIAN_POINT('Ctrl Pts',(-58.0841784519436,-19.9304621405658,
-176.259519378371));
#152136=CARTESIAN_POINT('Ctrl Pts',(-58.5358479429026,-20.4652520455798,
-176.572045320709));
#152137=CARTESIAN_POINT('Ctrl Pts',(-58.0269718314754,-20.409820708043,
-176.521171997891));
#152138=CARTESIAN_POINT('Ctrl Pts',(-58.0887038582403,-19.8911762730753,
-176.615064002266));
#152139=CARTESIAN_POINT('Ctrl Pts',(-58.453312463316,-20.5037323072241,
-176.810599719082));
#152140=CARTESIAN_POINT('Ctrl Pts',(-58.0300429255414,-20.3800147773311,
-176.815173598683));
#152141=CARTESIAN_POINT('Ctrl Pts',(-58.0801409030891,-19.9672777568629,
-176.996564457697));
#152142=CARTESIAN_POINT('Ctrl Pts',(-58.3536773083228,-20.6617143273459,
-177.059070718027));
#152143=CARTESIAN_POINT('Ctrl Pts',(-58.008419009151,-20.5399861299023,
-177.132937218036));
#152144=CARTESIAN_POINT('Ctrl Pts',(-58.0411746905458,-20.2805473548039,
-177.404658872083));
#152145=CARTESIAN_POINT('Ctrl Pts',(-58.3273152468094,-20.7187423212865,
-177.118370177225));
#152146=CARTESIAN_POINT('Ctrl Pts',(-57.9997262186439,-20.6050332455159,
-177.211134013007));
#152147=CARTESIAN_POINT('Ctrl Pts',(-58.0268899075637,-20.3936565135702,
-177.503861519498));
#152148=CARTESIAN_POINT('Ctrl Pts',(-58.2694539592074,-20.878594537362,
-177.222018588675));
#152149=CARTESIAN_POINT('Ctrl Pts',(-57.9736236814238,-20.7985247659916,
-177.347834553946));
#152150=CARTESIAN_POINT('Ctrl Pts',(-57.9855747517757,-20.7107497140498,
-177.674988342283));
#152151=CARTESIAN_POINT('Ctrl Pts',(-58.2424846982626,-20.9834338367789,
-177.246739433871));
#152152=CARTESIAN_POINT('Ctrl Pts',(-57.9549828795132,-20.9354006234089,
-177.384906431077));
#152153=CARTESIAN_POINT('Ctrl Pts',(-57.9575440958208,-20.9188769733095,
-177.71328609301));
#152154=CARTESIAN_POINT('Ctrl Pts',(-58.2224054091628,-21.0947200667586,
-177.228981500926));
#152155=CARTESIAN_POINT('Ctrl Pts',(-57.9347942321424,-21.0799781740437,
-177.361546823285));
#152156=CARTESIAN_POINT('Ctrl Pts',(-57.9264125504997,-21.1393961655747,
-177.673640454257));
#152157=CARTESIAN_POINT('Origin',(-58.4476369465814,-21.0219233613115,-177.688917160843));
#152158=CARTESIAN_POINT('Ctrl Pts',(-57.8819282087167,-21.4487963148739,
-177.697497252237));
#152159=CARTESIAN_POINT('Ctrl Pts',(-57.8810878095005,-21.4545317502846,
-177.368333266163));
#152160=CARTESIAN_POINT('Ctrl Pts',(-58.1799818947148,-21.5006430233976,
-177.238261718413));
#152161=CARTESIAN_POINT('Ctrl Pts',(-57.906096697535,-21.2838546967462,
-177.694536471641));
#152162=CARTESIAN_POINT('Ctrl Pts',(-57.9052384907138,-21.2898253143233,
-177.368094235677));
#152163=CARTESIAN_POINT('Ctrl Pts',(-58.2008748005355,-21.3341357689658,
-177.236799145875));
#152164=CARTESIAN_POINT('Ctrl Pts',(-57.9295599753438,-21.1188110827801,
-177.691677811931));
#152165=CARTESIAN_POINT('Ctrl Pts',(-57.9287492734302,-21.1245836426315,
-177.367866070024));
#152166=CARTESIAN_POINT('Ctrl Pts',(-58.2211580737071,-21.1675764425397,
-177.235439894836));
#152167=CARTESIAN_POINT('Ctrl Pts',(-57.952317989407,-20.9536655363853,
-177.688917160843));
#152168=CARTESIAN_POINT('Ctrl Pts',(-57.9515978527783,-20.958891271667,
-177.367648026607));
#152169=CARTESIAN_POINT('Ctrl Pts',(-58.2408316684984,-21.0009616906551,
-177.234173073119));
#152170=CARTESIAN_POINT('Origin',(-58.376645543834,-21.5212860267954,-177.697497252237));
#152171=CARTESIAN_POINT('Origin',(8.61202340367822,-13.0253612208376,-187.990299917396));
#152172=CARTESIAN_POINT('Ctrl Pts',(-58.1799818947148,-21.5006430233977,
-177.238261718413));
#152173=CARTESIAN_POINT('Ctrl Pts',(-57.8810878095005,-21.4545317502846,
-177.368333266163));
#152174=CARTESIAN_POINT('Ctrl Pts',(-57.8819282087167,-21.4487963148736,
-177.697497252237));
#152175=CARTESIAN_POINT('Ctrl Pts',(-58.1643305096628,-21.5659716479372,
-177.242027715059));
#152176=CARTESIAN_POINT('Ctrl Pts',(-57.868876514339,-21.5377805372773,
-177.374493960823));
#152177=CARTESIAN_POINT('Ctrl Pts',(-57.8629489711247,-21.5783230793646,
-177.699822299871));
#152178=CARTESIAN_POINT('Ctrl Pts',(-58.1516959167317,-21.6321056009482,
-177.229926261063));
#152179=CARTESIAN_POINT('Ctrl Pts',(-57.8561193903755,-21.6237742374893,
-177.3594824509));
#152180=CARTESIAN_POINT('Ctrl Pts',(-57.8432533717849,-21.7094932883126,
-177.67338127456));
#152181=CARTESIAN_POINT('Ctrl Pts',(-58.135834617463,-21.751763745641,-177.175847704912));
#152182=CARTESIAN_POINT('Ctrl Pts',(-57.833274341657,-21.7763737806991,
-177.289541220421));
#152183=CARTESIAN_POINT('Ctrl Pts',(-57.8068932864249,-21.9467814783138,
-177.56730490578));
#152184=CARTESIAN_POINT('Ctrl Pts',(-58.1325374345936,-21.8059684297317,
-177.133613057603));
#152185=CARTESIAN_POINT('Ctrl Pts',(-57.822969521998,-21.8444848229842,
-177.233860492204));
#152186=CARTESIAN_POINT('Ctrl Pts',(-57.7900355525622,-22.0542721190802,
-177.487158575097));
#152187=CARTESIAN_POINT('Ctrl Pts',(-58.1379476084663,-21.8930112710375,
-177.027055273752));
#152188=CARTESIAN_POINT('Ctrl Pts',(-57.8075855468967,-21.9461185785114,
-177.096669117024));
#152189=CARTESIAN_POINT('Ctrl Pts',(-57.7626304144021,-22.2268825024457,
-177.290851905635));
#152190=CARTESIAN_POINT('Ctrl Pts',(-58.1467121091855,-21.9264637442851,
-176.962169933093));
#152191=CARTESIAN_POINT('Ctrl Pts',(-57.8023886323833,-21.9804905067127,
-177.013273949454));
#152192=CARTESIAN_POINT('Ctrl Pts',(-57.7519076537925,-22.2932204551335,
-177.173672169064));
#152193=CARTESIAN_POINT('Ctrl Pts',(-58.1775901524469,-21.9698497118448,
-176.818815489061));
#152194=CARTESIAN_POINT('Ctrl Pts',(-57.7982009932088,-22.0095200736329,
-176.838338250264));
#152195=CARTESIAN_POINT('Ctrl Pts',(-57.7379487783882,-22.3792570371924,
-176.923566462093));
#152196=CARTESIAN_POINT('Ctrl Pts',(-58.1997838724148,-21.98000002,-176.740111438881));
#152197=CARTESIAN_POINT('Ctrl Pts',(-57.7993206334297,-22.0035077749888,
-176.744992431703));
#152198=CARTESIAN_POINT('Ctrl Pts',(-57.7346476044917,-22.3993856207533,
-176.79021969384));
#152199=CARTESIAN_POINT('Ctrl Pts',(-58.2281061322669,-21.98000002,-176.657965001855));
#152200=CARTESIAN_POINT('Ctrl Pts',(-57.8031610044997,-21.98000002,-176.657965001855));
#152201=CARTESIAN_POINT('Ctrl Pts',(-57.7346476057222,-22.3993856132206,
-176.657965001855));
#152202=CARTESIAN_POINT('Origin',(0.,-12.9675000200281,-171.871644662643));
#152203=CARTESIAN_POINT('Origin',(0.,-12.9675000200281,-171.449026400902));
#152204=CARTESIAN_POINT('Ctrl Pts',(-57.0184057454332,-28.63000002,-176.849882244789));
#152205=CARTESIAN_POINT('Ctrl Pts',(-56.3680674991214,-28.63000002,-176.849882244789));
#152206=CARTESIAN_POINT('Ctrl Pts',(-56.5351989170821,-28.0015042572884,
-176.849882244789));
#152207=CARTESIAN_POINT('Ctrl Pts',(-57.0179413444383,-28.63000002,-176.912963832989));
#152208=CARTESIAN_POINT('Ctrl Pts',(-56.3682278310667,-28.6293970924019,
-176.891072637881));
#152209=CARTESIAN_POINT('Ctrl Pts',(-56.5351989103125,-28.0015042827455,
-176.976072722839));
#152210=CARTESIAN_POINT('Ctrl Pts',(-57.0114676733044,-28.6416054347749,
-176.974087537723));
#152211=CARTESIAN_POINT('Ctrl Pts',(-56.3671971691575,-28.6322312586769,
-176.931422425923));
#152212=CARTESIAN_POINT('Ctrl Pts',(-56.5290979719196,-28.024501614784,
-177.098181890721));
#152213=CARTESIAN_POINT('Ctrl Pts',(-57.,-28.664523125878,-177.032518510534));
#152214=CARTESIAN_POINT('Ctrl Pts',(-56.364125065416,-28.6418687251214,
-176.974758823107));
#152215=CARTESIAN_POINT('Ctrl Pts',(-56.5169491525423,-28.0699653316567,
-177.215087021068));
#152216=CARTESIAN_POINT('Origin',(-57.,-28.199046231756,-177.215087021068));
#152217=CARTESIAN_POINT('Ctrl Pts',(-56.262175563026,-28.9930296810172,
-177.84995));
#152218=CARTESIAN_POINT('Ctrl Pts',(-56.262175563026,-28.9930296810172,
-177.34995));
#152219=CARTESIAN_POINT('Ctrl Pts',(-56.7430488584365,-29.13000002,-177.34995));
#152220=CARTESIAN_POINT('Ctrl Pts',(-56.3176963010821,-28.7981083537361,
-177.849949971516));
#152221=CARTESIAN_POINT('Ctrl Pts',(-56.2928119947094,-28.8854717787751,
-177.322103214377));
#152222=CARTESIAN_POINT('Ctrl Pts',(-56.799051006553,-29.0316942919675,
-177.34995));
#152223=CARTESIAN_POINT('Ctrl Pts',(-56.3721096851181,-28.6028436438479,
-177.790491903933));
#152224=CARTESIAN_POINT('Ctrl Pts',(-56.3169386704035,-28.8006430758332,
-177.261063208671));
#152225=CARTESIAN_POINT('Ctrl Pts',(-56.8539225877547,-28.933239542368,
-177.320220947896));
#152226=CARTESIAN_POINT('Ctrl Pts',(-56.4617523202342,-28.2759697513382,
-177.568612620023));
#152227=CARTESIAN_POINT('Ctrl Pts',(-56.3506671101773,-28.684579593959,
-177.121256964593));
#152228=CARTESIAN_POINT('Ctrl Pts',(-56.9443314005494,-28.7684056938368,
-177.209281314082));
#152229=CARTESIAN_POINT('Ctrl Pts',(-56.4972682976465,-28.1436156829388,
-177.404470992826));
#152230=CARTESIAN_POINT('Ctrl Pts',(-56.3596918685657,-28.6555519736166,
-177.043271150691));
#152231=CARTESIAN_POINT('Ctrl Pts',(-56.9801582405499,-28.7016493747432,
-177.12717563931));
#152232=CARTESIAN_POINT('Ctrl Pts',(-56.5169491525423,-28.0699653316567,
-177.215087021068));
#152233=CARTESIAN_POINT('Ctrl Pts',(-56.364125065416,-28.6418687251214,
-176.974758823107));
#152234=CARTESIAN_POINT('Ctrl Pts',(-57.,-28.664523125878,-177.032518510534));
#152235=CARTESIAN_POINT('',(-56.7430488584365,-29.13000002,-177.34995));
#152236=CARTESIAN_POINT('Origin',(-56.7430488584365,-29.13000002,-177.84995));
#152237=CARTESIAN_POINT('Ctrl Pts',(-56.7430488584365,-29.13000002,-177.34995));
#152238=CARTESIAN_POINT('Ctrl Pts',(-56.799051006553,-29.0316942919675,
-177.34995));
#152239=CARTESIAN_POINT('Ctrl Pts',(-56.8539225877547,-28.933239542368,
-177.320220947896));
#152240=CARTESIAN_POINT('Ctrl Pts',(-56.9443314005494,-28.7684056938368,
-177.209281314082));
#152241=CARTESIAN_POINT('Ctrl Pts',(-56.9801582405499,-28.7016493747432,
-177.12717563931));
#152242=CARTESIAN_POINT('Ctrl Pts',(-57.,-28.664523125878,-177.032518510534));
#152243=CARTESIAN_POINT('Origin',(0.,-12.9675000200281,-177.84995));
#152244=CARTESIAN_POINT('Origin',(-56.5982428503831,-29.63000002,-177.84995));
#152245=CARTESIAN_POINT('Origin',(0.,-12.9675000200281,-177.34995));
#152246=CARTESIAN_POINT('Ctrl Pts',(-56.598242850383,-29.6300000200001,
-177.34995));
#152247=CARTESIAN_POINT('Ctrl Pts',(-56.1185967245324,-29.4887923928816,
-177.34995));
#152248=CARTESIAN_POINT('Ctrl Pts',(-56.1185967245323,-29.4887923928817,
-177.84995));
#152249=CARTESIAN_POINT('Ctrl Pts',(-56.5603834356575,-29.6942993846806,
-177.34995));
#152250=CARTESIAN_POINT('Ctrl Pts',(-56.0988447287815,-29.5558848630778,
-177.36777816462));
#152251=CARTESIAN_POINT('Ctrl Pts',(-56.0810569766533,-29.6163052971279,
-177.849949980253));
#152252=CARTESIAN_POINT('Ctrl Pts',(-56.5223271856603,-29.7580969359688,
-177.337570500007));
#152253=CARTESIAN_POINT('Ctrl Pts',(-56.076826602317,-29.6305362885491,
-177.372218485688));
#152254=CARTESIAN_POINT('Ctrl Pts',(-56.04332441336,-29.7428150883777,-177.825190994024));
#152255=CARTESIAN_POINT('Ctrl Pts',(-56.4500227583409,-29.8779487295679,
-177.288930648015));
#152256=CARTESIAN_POINT('Ctrl Pts',(-56.0326216659297,-29.7794711155594,
-177.345478783924));
#152257=CARTESIAN_POINT('Ctrl Pts',(-55.9716327345056,-29.9804872937887,
-177.727911302019));
#152258=CARTESIAN_POINT('Ctrl Pts',(-56.4164036466448,-29.9329688836733,
-177.253030654974));
#152259=CARTESIAN_POINT('Ctrl Pts',(-56.010729181878,-29.8527767454272,
-177.315352245562));
#152260=CARTESIAN_POINT('Ctrl Pts',(-55.9382985315747,-30.0895950523083,
-177.656111307255));
#152261=CARTESIAN_POINT('Ctrl Pts',(-56.3301688951883,-30.0730055436657,
-177.116037754475));
#152262=CARTESIAN_POINT('Ctrl Pts',(-55.9539368540439,-30.0418512098301,
-177.177649819729));
#152263=CARTESIAN_POINT('Ctrl Pts',(-55.8527945813582,-30.367294876883,
-177.382125514336));
#152264=CARTESIAN_POINT('Ctrl Pts',(-56.2941923707649,-30.1300000200003,
-176.98587944854));
#152265=CARTESIAN_POINT('Ctrl Pts',(-55.9270363771194,-30.1300000005971,
-177.017952895974));
#152266=CARTESIAN_POINT('Ctrl Pts',(-55.8171229439391,-30.4803177904842,
-177.121808892945));
#152267=CARTESIAN_POINT('Ctrl Pts',(-56.294192362543,-30.1300000200003,
-176.84995));
#152268=CARTESIAN_POINT('Ctrl Pts',(-55.9270363712659,-30.1300000200003,
-176.84995));
#152269=CARTESIAN_POINT('Ctrl Pts',(-55.8171229357418,-30.4803178166107,
-176.84995));
#152270=CARTESIAN_POINT('Origin',(0.,-12.9675000200281,-171.871644662643));
#152271=CARTESIAN_POINT('Origin',(0.,-12.9675000200281,-171.449026400902));
#152272=CARTESIAN_POINT('Ctrl Pts',(-54.1989607257493,-36.78000002,-176.84995));
#152273=CARTESIAN_POINT('Ctrl Pts',(-53.4396057593646,-36.78000002,-176.84995));
#152274=CARTESIAN_POINT('Ctrl Pts',(-53.7396474992599,-36.0824364606782,
-176.84995));
#152275=CARTESIAN_POINT('Ctrl Pts',(-54.1989607146972,-36.78000002,-176.918317891383));
#152276=CARTESIAN_POINT('Ctrl Pts',(-53.4396057606977,-36.7800000160094,
-176.873130497251));
#152277=CARTESIAN_POINT('Ctrl Pts',(-53.7396474882981,-36.0824364861631,
-176.986685785392));
#152278=CARTESIAN_POINT('Ctrl Pts',(-54.1865253922149,-36.7944813746413,
-176.987117359946));
#152279=CARTESIAN_POINT('Ctrl Pts',(-53.4415801188845,-36.7743609339043,
-176.898046003587));
#152280=CARTESIAN_POINT('Ctrl Pts',(-53.7273175494953,-36.1111537311933,
-177.124284716345));
#152281=CARTESIAN_POINT('Ctrl Pts',(-54.1401753140075,-36.8481352183371,
-177.110787176626));
#152282=CARTESIAN_POINT('Ctrl Pts',(-53.4422054158915,-36.7696056006871,
-176.971124353297));
#152283=CARTESIAN_POINT('Ctrl Pts',(-53.6813602693863,-36.2175520155611,
-177.371624356797));
#152284=CARTESIAN_POINT('Ctrl Pts',(-54.1061105508192,-36.8874586360784,
-177.16641977034));
#152285=CARTESIAN_POINT('Ctrl Pts',(-53.4404233153528,-36.7716343519663,
-177.018743720143));
#152286=CARTESIAN_POINT('Ctrl Pts',(-53.64758418971,-36.2955323627627,-177.48288953791));
#152287=CARTESIAN_POINT('Ctrl Pts',(-54.0238234872226,-36.9816277442484,
-177.25641751247));
#152288=CARTESIAN_POINT('Ctrl Pts',(-53.4231809570326,-36.8072884980391,
-177.124958325117));
#152289=CARTESIAN_POINT('Ctrl Pts',(-53.565994475128,-36.4822744877163,
-177.662885027711));
#152290=CARTESIAN_POINT('Ctrl Pts',(-53.9751511105352,-37.0369743252984,
-177.291477883886));
#152291=CARTESIAN_POINT('Ctrl Pts',(-53.408253154931,-36.8396793680934,
-177.182243847129));
#152292=CARTESIAN_POINT('Ctrl Pts',(-53.5177345753394,-36.5920295740937,
-177.73300576859));
#152293=CARTESIAN_POINT('Ctrl Pts',(-53.8706043508049,-37.1546953024018,
-177.33811707005));
#152294=CARTESIAN_POINT('Ctrl Pts',(-53.3641465670514,-36.936877735883,
-177.281217994791));
#152295=CARTESIAN_POINT('Ctrl Pts',(-53.4140738058199,-36.825476258465,
-177.826284139284));
#152296=CARTESIAN_POINT('Ctrl Pts',(-53.8142255012181,-37.2176314844153,
-177.34995));
#152297=CARTESIAN_POINT('Ctrl Pts',(-53.3356547273387,-37.0000719000691,
-177.323538819178));
#152298=CARTESIAN_POINT('Ctrl Pts',(-53.3581698892714,-36.9502882170505,
-177.849949987733));
#152299=CARTESIAN_POINT('Ctrl Pts',(-53.7578119323263,-37.28000002,-177.34995));
#152300=CARTESIAN_POINT('Ctrl Pts',(-53.3022372549337,-37.073961884407,
-177.34995));
#152301=CARTESIAN_POINT('Ctrl Pts',(-53.3022372549337,-37.073961884407,
-177.84995));
#152302=CARTESIAN_POINT('Origin',(-53.7578119323263,-37.28000002,-177.84995));
#152303=CARTESIAN_POINT('Origin',(0.,-12.9675000200281,-177.84995));
#152304=CARTESIAN_POINT('Origin',(-53.5288692553037,-37.78000002,-177.84995));
#152305=CARTESIAN_POINT('Origin',(0.,-12.9675000200281,-177.34995));
#152306=CARTESIAN_POINT('Ctrl Pts',(-53.5288692553037,-37.78000002,-177.34995));
#152307=CARTESIAN_POINT('Ctrl Pts',(-53.0752347700892,-37.5697245962714,
-177.34995));
#152308=CARTESIAN_POINT('Ctrl Pts',(-53.0752347700893,-37.5697245962714,
-177.84995));
#152309=CARTESIAN_POINT('Ctrl Pts',(-53.4801386760123,-37.8325641065285,
-177.34995));
#152310=CARTESIAN_POINT('Ctrl Pts',(-53.0475810937503,-37.6293828354337,
-177.371580332169));
#152311=CARTESIAN_POINT('Ctrl Pts',(-53.0269261151962,-37.673942537699,
-177.849949988053));
#152312=CARTESIAN_POINT('Ctrl Pts',(-53.4320050770023,-37.884077740683,
-177.341849758034));
#152313=CARTESIAN_POINT('Ctrl Pts',(-53.0170937964823,-37.6950135347464,
-177.382936820891));
#152314=CARTESIAN_POINT('Ctrl Pts',(-52.9791793012708,-37.7761418725299,
-177.833741031442));
#152315=CARTESIAN_POINT('Ctrl Pts',(-53.3846587239314,-37.9343850848642,
-177.325518346031));
#152316=CARTESIAN_POINT('Ctrl Pts',(-52.9848137611505,-37.764168205744,
-177.380776321343));
#152317=CARTESIAN_POINT('Ctrl Pts',(-52.9322463618642,-37.8758780299853,
-177.801086692062));
#152318=CARTESIAN_POINT('Origin',(-53.3846587239314,-38.0887701497285,-177.801086692062));
#152319=CARTESIAN_POINT('Ctrl Pts',(-53.3846587239314,-37.9343850848642,
-177.325518346031));
#152320=CARTESIAN_POINT('Ctrl Pts',(-52.9848137611506,-37.764168205744,
-177.380776321343));
#152321=CARTESIAN_POINT('Ctrl Pts',(-52.9322463618642,-37.8758780299853,
-177.801086692062));
#152322=CARTESIAN_POINT('Ctrl Pts',(-53.2963306348783,-38.0282371456548,
-177.295050892481));
#152323=CARTESIAN_POINT('Ctrl Pts',(-52.9134668198848,-37.9027770181211,
-177.371916826896));
#152324=CARTESIAN_POINT('Ctrl Pts',(-52.8342434317084,-38.0841419017282,
-177.740238340822));
#152325=CARTESIAN_POINT('Ctrl Pts',(-53.2302250969522,-38.1165826570878,
-177.234494972704));
#152326=CARTESIAN_POINT('Ctrl Pts',(-52.85052657881,-38.040124740984,-177.309543897189));
#152327=CARTESIAN_POINT('Ctrl Pts',(-52.7606534316743,-38.2807615372527,
-177.619039957031));
#152328=CARTESIAN_POINT('Ctrl Pts',(-53.1455750275301,-38.2433781645652,
-177.065457314865));
#152329=CARTESIAN_POINT('Ctrl Pts',(-52.7690004592735,-38.2275535486387,
-177.113060004592));
#152330=CARTESIAN_POINT('Ctrl Pts',(-52.6665978216312,-38.5625293047724,
-177.280964618108));
#152331=CARTESIAN_POINT('Ctrl Pts',(-53.1262583407606,-38.28000002,-176.958526013972));
#152332=CARTESIAN_POINT('Ctrl Pts',(-52.7480693868922,-38.2799999991994,
-176.98145090087));
#152333=CARTESIAN_POINT('Ctrl Pts',(-52.6451348250506,-38.6439111866979,
-177.06710203648));
#152334=CARTESIAN_POINT('Ctrl Pts',(-53.1262583325313,-38.28000002,-176.84995));
#152335=CARTESIAN_POINT('Ctrl Pts',(-52.748069378376,-38.28000002,-176.84995));
#152336=CARTESIAN_POINT('Ctrl Pts',(-52.6451348158641,-38.6439112191758,
-176.84995));
#152337=CARTESIAN_POINT('Ctrl Pts',(-52.1126146143194,-39.4738501833479,
-171.391638125813));
#152338=CARTESIAN_POINT('Ctrl Pts',(-52.4864722882118,-39.4409761333229,
-171.679515584751));
#152339=CARTESIAN_POINT('Ctrl Pts',(-52.5050296388285,-39.3089337226171,
-172.133326251627));
#152340=CARTESIAN_POINT('Ctrl Pts',(-52.2029436074416,-39.18424163534,-171.345711176575));
#152341=CARTESIAN_POINT('Ctrl Pts',(-52.5176461244299,-39.1701487854048,
-171.633412526629));
#152342=CARTESIAN_POINT('Ctrl Pts',(-52.541270746464,-39.0510648426419,
-172.04151129494));
#152343=CARTESIAN_POINT('Ctrl Pts',(-52.3057718899875,-38.8932964873464,
-171.301698499895));
#152344=CARTESIAN_POINT('Ctrl Pts',(-52.5724535929286,-38.8910154875477,
-171.580271166833));
#152345=CARTESIAN_POINT('Ctrl Pts',(-52.5971684400779,-38.7973422647502,
-171.953442620307));
#152346=CARTESIAN_POINT('Ctrl Pts',(-52.4226914394942,-38.5972250898729,
-171.270067206297));
#152347=CARTESIAN_POINT('Ctrl Pts',(-52.6539547691069,-38.61136117722,-171.540761416572));
#152348=CARTESIAN_POINT('Ctrl Pts',(-52.6743159902015,-38.5446760769969,
-171.890184412595));
#152349=CARTESIAN_POINT('',(-52.1126146143194,-39.473850183348,-171.391638125813));
#152350=CARTESIAN_POINT('Origin',(-51.5147615700869,-39.1697606216571,-172.133326251627));
#152351=CARTESIAN_POINT('Ctrl Pts',(-52.1126146143194,-39.473850183348,
-171.391638125813));
#152352=CARTESIAN_POINT('Ctrl Pts',(-52.2018635968859,-39.1877043141331,
-171.34626029805));
#152353=CARTESIAN_POINT('Ctrl Pts',(-52.3033147624415,-38.900253615735,
-171.302751240844));
#152354=CARTESIAN_POINT('Ctrl Pts',(-52.418503743379,-38.6078427661481,
-171.27120723903));
#152355=CARTESIAN_POINT('Origin',(-51.6222122422086,-38.4052093625928,-172.64995));
#152356=CARTESIAN_POINT('',(-50.5139609686817,-46.2908269190399,-171.64995));
#152357=CARTESIAN_POINT('Ctrl Pts',(-50.5091418211897,-53.5104134695199,
-177.84995));
#152358=CARTESIAN_POINT('Ctrl Pts',(-50.5091418211897,-53.51041346952,-177.34995));
#152359=CARTESIAN_POINT('Ctrl Pts',(-51.0042758555605,-53.58000002,-177.34995));
#152360=CARTESIAN_POINT('Ctrl Pts',(-50.546038665875,-53.2478787779945,
-177.849949999941));
#152361=CARTESIAN_POINT('Ctrl Pts',(-50.5284384672378,-53.3731106984804,
-177.33120422009));
#152362=CARTESIAN_POINT('Ctrl Pts',(-51.0411727002473,-53.4487326742368,
-177.34995));
#152363=CARTESIAN_POINT('Ctrl Pts',(-50.5825022662094,-52.9884267802056,
-177.742176873059));
#152364=CARTESIAN_POINT('Ctrl Pts',(-50.5442961447015,-53.2602774603979,
-177.257255781812));
#152365=CARTESIAN_POINT('Ctrl Pts',(-51.0776363005805,-53.3190066753437,
-177.296063436531));
#152366=CARTESIAN_POINT('Ctrl Pts',(-50.6345361306733,-52.6181865964612,
-177.371936689315));
#152367=CARTESIAN_POINT('Ctrl Pts',(-50.5649476695633,-53.1133342256642,
-177.069891898465));
#152368=CARTESIAN_POINT('Ctrl Pts',(-51.1296701650438,-53.1338865834697,
-177.110943344657));
#152369=CARTESIAN_POINT('Ctrl Pts',(-50.6496826558828,-52.5104134695857,
-177.112484691526));
#152370=CARTESIAN_POINT('Ctrl Pts',(-50.5696324866514,-53.0800000199829,
-176.958917254526));
#152371=CARTESIAN_POINT('Ctrl Pts',(-51.1448166902519,-53.08000002,-176.981217345763));
#152372=CARTESIAN_POINT('Ctrl Pts',(-50.6496826558921,-52.5104134695199,
-176.84995));
#152373=CARTESIAN_POINT('Ctrl Pts',(-50.5696324866524,-53.08000002,-176.84995));
#152374=CARTESIAN_POINT('Ctrl Pts',(-51.1448166902628,-53.08000002,-176.84995));
#152375=CARTESIAN_POINT('Origin',(-51.0042758555605,-53.58000002,-177.84995));
#152376=CARTESIAN_POINT('Origin',(-53.1076143453209,-38.6139690140329,-177.84995));
#152377=CARTESIAN_POINT('Origin',(-50.9340054382093,-54.0800000199999,-177.84995));
#152378=CARTESIAN_POINT('',(-62.4796469926385,28.0715083218873,-177.34995));
#152379=CARTESIAN_POINT('Ctrl Pts',(-50.2983305691361,-55.0104134695199,
-176.84995));
#152380=CARTESIAN_POINT('Ctrl Pts',(-50.3588212345988,-54.58000002,-176.84995));
#152381=CARTESIAN_POINT('Ctrl Pts',(-50.7934646035069,-54.58000002,-176.84995));
#152382=CARTESIAN_POINT('Ctrl Pts',(-50.2983305691453,-55.0104134694541,
-177.112484691526));
#152383=CARTESIAN_POINT('Ctrl Pts',(-50.358821234607,-54.5800000199424,
-176.997671841189));
#152384=CARTESIAN_POINT('Ctrl Pts',(-50.7934646035178,-54.58000002,-176.981217345763));
#152385=CARTESIAN_POINT('Ctrl Pts',(-50.313477094355,-54.9026403425777,
-177.371936689315));
#152386=CARTESIAN_POINT('Ctrl Pts',(-50.3685899331079,-54.5104921183889,
-177.142957948483));
#152387=CARTESIAN_POINT('Ctrl Pts',(-50.8086111287259,-54.5261134565302,
-177.110943344657));
#152388=CARTESIAN_POINT('Ctrl Pts',(-50.3655109588186,-54.5324001588352,
-177.742176873059));
#152389=CARTESIAN_POINT('Ctrl Pts',(-50.3994818369767,-54.2906848009584,
-177.329589659683));
#152390=CARTESIAN_POINT('Ctrl Pts',(-50.8606449931892,-54.3409933646562,
-177.296063436531));
#152391=CARTESIAN_POINT('Ctrl Pts',(-50.4019745591532,-54.2729481610447,
-177.849949999941));
#152392=CARTESIAN_POINT('Ctrl Pts',(-50.420433990624,-54.1416024812641,
-177.367861075731));
#152393=CARTESIAN_POINT('Ctrl Pts',(-50.8971085935234,-54.2112673657634,
-177.34995));
#152394=CARTESIAN_POINT('Ctrl Pts',(-50.4388714038385,-54.0104134695199,
-177.84995));
#152395=CARTESIAN_POINT('Ctrl Pts',(-50.4388714038384,-54.0104134695199,
-177.34995));
#152396=CARTESIAN_POINT('Ctrl Pts',(-50.9340054382093,-54.08000002,-177.34995));
#152397=CARTESIAN_POINT('Origin',(-51.6222122422086,-38.4052093625928,-172.64995));
#152398=CARTESIAN_POINT('Origin',(-48.9446667094463,-57.4569357767149,-172.64995));
#152399=CARTESIAN_POINT('Ctrl Pts',(-50.9867892914962,-42.9264785869994,
-171.64995));
#152400=CARTESIAN_POINT('Ctrl Pts',(-51.9770573602378,-43.0656516879595,
-171.64995));
#152401=CARTESIAN_POINT('Ctrl Pts',(-51.9770573602378,-43.0656516879596,
-172.64995));
#152402=CARTESIAN_POINT('Ctrl Pts',(-51.1823572933545,-42.3510730842576,
-171.64995));
#152403=CARTESIAN_POINT('Ctrl Pts',(-52.0557320324863,-42.5058523071511,
-171.757498535929));
#152404=CARTESIAN_POINT('Ctrl Pts',(-52.0666747393887,-42.4279909017497,
-172.649949997757));
#152405=CARTESIAN_POINT('Ctrl Pts',(-51.3741578990751,-41.7754043578546,
-171.628003076365));
#152406=CARTESIAN_POINT('Ctrl Pts',(-52.1416679592955,-41.8943864154851,
-171.81403941883));
#152407=CARTESIAN_POINT('Ctrl Pts',(-52.1554800333146,-41.7961084021622,
-172.606056153133));
#152408=CARTESIAN_POINT('Ctrl Pts',(-51.7497860966445,-40.6237611991777,
-171.543915907757));
#152409=CARTESIAN_POINT('Ctrl Pts',(-52.3125022740342,-40.6788371047634,
-171.821280489149));
#152410=CARTESIAN_POINT('Ctrl Pts',(-52.3315472405273,-40.5433251268562,
-172.43788181511));
#152411=CARTESIAN_POINT('Ctrl Pts',(-51.9336694513069,-40.0475756797307,
-171.482621144039));
#152412=CARTESIAN_POINT('Ctrl Pts',(-52.3988291636532,-40.0645893682337,
-171.781794156641));
#152413=CARTESIAN_POINT('Ctrl Pts',(-52.4188787332529,-39.9219292677054,
-172.315208572937));
#152414=CARTESIAN_POINT('Ctrl Pts',(-52.1126146143194,-39.473850183348,
-171.391638125813));
#152415=CARTESIAN_POINT('Ctrl Pts',(-52.4864722882118,-39.4409761333229,
-171.679515584751));
#152416=CARTESIAN_POINT('Ctrl Pts',(-52.5050296388285,-39.3089337226171,
-172.133326251627));
#152417=CARTESIAN_POINT('',(-50.9867892914962,-42.9264785869994,-171.64995));
#152418=CARTESIAN_POINT('Origin',(-50.9867892914962,-42.9264785869994,-172.64995));
#152419=CARTESIAN_POINT('Ctrl Pts',(-50.9867892914962,-42.9264785869994,
-171.64995));
#152420=CARTESIAN_POINT('Ctrl Pts',(-51.1823574302578,-42.3510731085196,
-171.649950016858));
#152421=CARTESIAN_POINT('Ctrl Pts',(-51.3741580251093,-41.7754043773928,
-171.628003106914));
#152422=CARTESIAN_POINT('Ctrl Pts',(-51.7497861967124,-40.6237612089719,
-171.543915957081));
#152423=CARTESIAN_POINT('Ctrl Pts',(-51.9336695368887,-40.0475756828609,
-171.482621199082));
#152424=CARTESIAN_POINT('Ctrl Pts',(-52.1126146143194,-39.473850183348,
-171.391638125813));
#152425=CARTESIAN_POINT('Origin',(-51.6222122422086,-38.4052093625928,-172.64995));
#152426=CARTESIAN_POINT('',(-51.3476245933058,-40.3590020057362,-171.64995));
#152427=CARTESIAN_POINT('Ctrl Pts',(-51.6545496240141,-45.3604134695199,
-177.84995));
#152428=CARTESIAN_POINT('Ctrl Pts',(-51.6545496240142,-45.3604134695199,
-177.34995));
#152429=CARTESIAN_POINT('Ctrl Pts',(-52.1496836583849,-45.43000002,-177.34995));
#152430=CARTESIAN_POINT('Ctrl Pts',(-51.6914464686995,-45.0978787779945,
-177.849949999941));
#152431=CARTESIAN_POINT('Ctrl Pts',(-51.6738462700621,-45.2231106984802,
-177.331204220089));
#152432=CARTESIAN_POINT('Ctrl Pts',(-52.1865805030705,-45.2987326742378,
-177.34995));
#152433=CARTESIAN_POINT('Ctrl Pts',(-51.7279100690339,-44.8384267802056,
-177.742176873059));
#152434=CARTESIAN_POINT('Ctrl Pts',(-51.6897039475278,-45.1102774603978,
-177.257255781811));
#152435=CARTESIAN_POINT('Ctrl Pts',(-52.2230441034049,-45.1690066753419,
-177.296063436528));
#152436=CARTESIAN_POINT('Ctrl Pts',(-51.7799439334977,-44.4681865964612,
-177.371936689315));
#152437=CARTESIAN_POINT('Ctrl Pts',(-51.710355472386,-44.963334225664,-177.069891898465));
#152438=CARTESIAN_POINT('Ctrl Pts',(-52.2750779678683,-44.9838865834715,
-177.110943344658));
#152439=CARTESIAN_POINT('Ctrl Pts',(-51.7950904587073,-44.3604134695857,
-177.112484691526));
#152440=CARTESIAN_POINT('Ctrl Pts',(-51.7150402894787,-44.9300000199802,
-176.958917254526));
#152441=CARTESIAN_POINT('Ctrl Pts',(-52.2902244930764,-44.93000002,-176.981217345763));
#152442=CARTESIAN_POINT('Ctrl Pts',(-51.7950904587165,-44.36041346952,-176.84995));
#152443=CARTESIAN_POINT('Ctrl Pts',(-51.7150402894768,-44.93000002,-176.84995));
#152444=CARTESIAN_POINT('Ctrl Pts',(-52.2902244930873,-44.93000002,-176.84995));
#152445=CARTESIAN_POINT('Origin',(-52.1496836583849,-45.43000002,-177.84995));
#152446=CARTESIAN_POINT('Origin',(-53.1076143453209,-38.6139690140329,-177.84995));
#152447=CARTESIAN_POINT('Origin',(-52.0794132410337,-45.93000002,-177.84995));
#152448=CARTESIAN_POINT('',(-62.4796469926385,28.0715083218873,-177.34995));
#152449=CARTESIAN_POINT('Ctrl Pts',(-51.4437383719606,-46.86041346952,-176.84995));
#152450=CARTESIAN_POINT('Ctrl Pts',(-51.5042290374232,-46.43000002,-176.84995));
#152451=CARTESIAN_POINT('Ctrl Pts',(-51.9388724063314,-46.43000002,-176.84995));
#152452=CARTESIAN_POINT('Ctrl Pts',(-51.4437383719698,-46.8604134694541,
-177.112484691526));
#152453=CARTESIAN_POINT('Ctrl Pts',(-51.5042290374242,-46.4300000199415,
-176.997671841189));
#152454=CARTESIAN_POINT('Ctrl Pts',(-51.9388724063423,-46.43000002,-176.981217345763));
#152455=CARTESIAN_POINT('Ctrl Pts',(-51.4588848971795,-46.7526403425778,
-177.371936689315));
#152456=CARTESIAN_POINT('Ctrl Pts',(-51.5139977359314,-46.3604921183892,
-177.142957948483));
#152457=CARTESIAN_POINT('Ctrl Pts',(-51.9540189315504,-46.3761134565303,
-177.110943344657));
#152458=CARTESIAN_POINT('Ctrl Pts',(-51.5109187616431,-46.3824001588352,
-177.742176873059));
#152459=CARTESIAN_POINT('Ctrl Pts',(-51.5448896398021,-46.1406848009587,
-177.329589659683));
#152460=CARTESIAN_POINT('Ctrl Pts',(-52.0060527960138,-46.1909933646562,
-177.296063436531));
#152461=CARTESIAN_POINT('Ctrl Pts',(-51.5473823619777,-46.1229481610447,
-177.849949999941));
#152462=CARTESIAN_POINT('Ctrl Pts',(-51.5658417934483,-45.9916024812643,
-177.367861075732));
#152463=CARTESIAN_POINT('Ctrl Pts',(-52.0425163963479,-46.0612673657634,
-177.34995));
#152464=CARTESIAN_POINT('Ctrl Pts',(-51.584279206663,-45.86041346952,-177.84995));
#152465=CARTESIAN_POINT('Ctrl Pts',(-51.584279206663,-45.8604134695199,
-177.34995));
#152466=CARTESIAN_POINT('Ctrl Pts',(-52.0794132410337,-45.93000002,-177.34995));
#152467=CARTESIAN_POINT('Origin',(-46.9641305719631,-57.1785895747948,-172.64995));
#152468=CARTESIAN_POINT('Origin',(-48.4203826827217,-58.549476072617,-172.64995));
#152469=CARTESIAN_POINT('Origin',(0.,-12.9675000200281,-172.64995));
#152470=CARTESIAN_POINT('Origin',(-45.5819760525891,-61.3878827027496,-172.64995));
#152471=CARTESIAN_POINT('Origin',(-44.2110895547669,-59.9316305919911,-172.64995));
#152472=CARTESIAN_POINT('Origin',(-44.489435756687,-61.9121667294742,-172.64995));
#152473=CARTESIAN_POINT('Origin',(-45.4220505312374,-61.7810962706031,-172.64995));
#152474=CARTESIAN_POINT('Ctrl Pts',(-40.9304134495199,-63.4221822677665,
-177.84995));
#152475=CARTESIAN_POINT('Ctrl Pts',(-40.9304134495199,-63.4221822677665,
-177.34995));
#152476=CARTESIAN_POINT('Ctrl Pts',(-41.,-63.9173163021373,-177.34995));
#152477=CARTESIAN_POINT('Ctrl Pts',(-41.1929481410454,-63.3852854230811,
-177.849949999941));
#152478=CARTESIAN_POINT('Ctrl Pts',(-41.0616024612649,-63.4037448545523,
-177.367861075732));
#152479=CARTESIAN_POINT('Ctrl Pts',(-41.1312673457634,-63.8804194574513,
-177.34995));
#152480=CARTESIAN_POINT('Ctrl Pts',(-41.4524001388343,-63.3488218227467,
-177.742176873059));
#152481=CARTESIAN_POINT('Ctrl Pts',(-41.2106847809575,-63.3827927009057,
-177.329589659683));
#152482=CARTESIAN_POINT('Ctrl Pts',(-41.2609933446562,-63.8439558571173,
-177.296063436531));
#152483=CARTESIAN_POINT('Ctrl Pts',(-41.8226403225787,-63.2967879582829,
-177.371936689315));
#152484=CARTESIAN_POINT('Ctrl Pts',(-41.4304920983899,-63.3519007970349,
-177.142957948483));
#152485=CARTESIAN_POINT('Ctrl Pts',(-41.4461134365302,-63.7919219926539,
-177.110943344657));
#152486=CARTESIAN_POINT('Ctrl Pts',(-41.9304134494542,-63.2816414330733,
-177.112484691526));
#152487=CARTESIAN_POINT('Ctrl Pts',(-41.4999999999415,-63.342132098545,
-176.997671841189));
#152488=CARTESIAN_POINT('Ctrl Pts',(-41.5,-63.7767754674458,-176.981217345763));
#152489=CARTESIAN_POINT('Ctrl Pts',(-41.9304134495199,-63.2816414330641,
-176.84995));
#152490=CARTESIAN_POINT('Ctrl Pts',(-41.5,-63.3421320985267,-176.84995));
#152491=CARTESIAN_POINT('Ctrl Pts',(-41.5,-63.7767754674349,-176.84995));
#152492=CARTESIAN_POINT('Origin',(-41.,-63.9173163021373,-177.84995));
#152493=CARTESIAN_POINT('Origin',(-45.6308101826775,-63.2664983737155,-177.84995));
#152494=CARTESIAN_POINT('Origin',(-40.5,-63.9875867194884,-177.84995));
#152495=CARTESIAN_POINT('',(-40.227526467895,-64.0258803771248,-177.34995));
#152496=CARTESIAN_POINT('Ctrl Pts',(-39.43041344952,-63.63299351982,-176.84995));
#152497=CARTESIAN_POINT('Ctrl Pts',(-40.,-63.5529433505803,-176.84995));
#152498=CARTESIAN_POINT('Ctrl Pts',(-40.,-64.1281275541908,-176.84995));
#152499=CARTESIAN_POINT('Ctrl Pts',(-39.4304134495858,-63.6329935198108,
-177.112484691526));
#152500=CARTESIAN_POINT('Ctrl Pts',(-39.9999999999783,-63.5529433505767,
-176.958917254529));
#152501=CARTESIAN_POINT('Ctrl Pts',(-40.,-64.1281275541799,-176.981217345763));
#152502=CARTESIAN_POINT('Ctrl Pts',(-39.5381865764622,-63.6178469946011,
-177.371936689315));
#152503=CARTESIAN_POINT('Ctrl Pts',(-40.033334205665,-63.5482585334886,
-177.069891898461));
#152504=CARTESIAN_POINT('Ctrl Pts',(-40.0538865634702,-64.1129810289718,
-177.110943344657));
#152505=CARTESIAN_POINT('Ctrl Pts',(-39.9084267602046,-63.5658131301376,
-177.742176873059));
#152506=CARTESIAN_POINT('Ctrl Pts',(-40.1802774403969,-63.5276070086322,
-177.257255781815));
#152507=CARTESIAN_POINT('Ctrl Pts',(-40.2390066553433,-64.0609471645084,
-177.29606343653));
#152508=CARTESIAN_POINT('Ctrl Pts',(-40.1678787579952,-63.5293495298029,
-177.849949999941));
#152509=CARTESIAN_POINT('Ctrl Pts',(-40.293110678481,-63.5117493311661,
-177.331204220089));
#152510=CARTESIAN_POINT('Ctrl Pts',(-40.3687326542369,-64.0244835641743,
-177.34995));
#152511=CARTESIAN_POINT('Ctrl Pts',(-40.4304134495199,-63.4924526851176,
-177.84995));
#152512=CARTESIAN_POINT('Ctrl Pts',(-40.4304134495199,-63.4924526851176,
-177.34995));
#152513=CARTESIAN_POINT('Ctrl Pts',(-40.5,-63.9875867194884,-177.34995));
#152514=CARTESIAN_POINT('Origin',(-45.4220505312374,-61.7810962706031,-172.64995));
#152515=CARTESIAN_POINT('',(-39.8608268990399,-62.5626752818388,-171.64995));
#152516=CARTESIAN_POINT('Ctrl Pts',(-32.7804134495199,-64.5675900705909,
-177.84995));
#152517=CARTESIAN_POINT('Ctrl Pts',(-32.7804134495199,-64.5675900705908,
-177.34995));
#152518=CARTESIAN_POINT('Ctrl Pts',(-32.85,-65.0627241049617,-177.34995));
#152519=CARTESIAN_POINT('Ctrl Pts',(-33.0429481410447,-64.5306932259057,
-177.849949999941));
#152520=CARTESIAN_POINT('Ctrl Pts',(-32.9116024612643,-64.5491526573769,
-177.367861075732));
#152521=CARTESIAN_POINT('Ctrl Pts',(-32.9812673457631,-65.0258272602758,
-177.34995));
#152522=CARTESIAN_POINT('Ctrl Pts',(-33.3024001388352,-64.494229625571,
-177.742176873059));
#152523=CARTESIAN_POINT('Ctrl Pts',(-33.0606847809584,-64.52820050373,-177.329589659683));
#152524=CARTESIAN_POINT('Ctrl Pts',(-33.1109933446567,-64.9893636599417,
-177.29606343653));
#152525=CARTESIAN_POINT('Ctrl Pts',(-33.6726403225778,-64.4421957611075,
-177.371936689315));
#152526=CARTESIAN_POINT('Ctrl Pts',(-33.280492098389,-64.4973085998594,
-177.142957948483));
#152527=CARTESIAN_POINT('Ctrl Pts',(-33.2961134365298,-64.9373297954784,
-177.110943344657));
#152528=CARTESIAN_POINT('Ctrl Pts',(-33.7804134494542,-64.4270492358978,
-177.112484691526));
#152529=CARTESIAN_POINT('Ctrl Pts',(-33.3499999999424,-64.4875399013621,
-176.997671841189));
#152530=CARTESIAN_POINT('Ctrl Pts',(-33.35,-64.9221832702703,-176.981217345763));
#152531=CARTESIAN_POINT('Ctrl Pts',(-33.7804134495199,-64.4270492358885,
-176.84995));
#152532=CARTESIAN_POINT('Ctrl Pts',(-33.35,-64.4875399013512,-176.84995));
#152533=CARTESIAN_POINT('Ctrl Pts',(-33.35,-64.9221832702593,-176.84995));
#152534=CARTESIAN_POINT('Origin',(-32.85,-65.0627241049617,-177.84995));
#152535=CARTESIAN_POINT('Origin',(-45.6308101826775,-63.2664983737155,-177.84995));
#152536=CARTESIAN_POINT('Origin',(-32.35,-65.1329945223129,-177.84995));
#152537=CARTESIAN_POINT('',(-40.227526467895,-64.0258803771248,-177.34995));
#152538=CARTESIAN_POINT('Ctrl Pts',(-31.28041344952,-64.7784013226445,-176.84995));
#152539=CARTESIAN_POINT('Ctrl Pts',(-31.8499999999999,-64.6983511534047,
-176.84995));
#152540=CARTESIAN_POINT('Ctrl Pts',(-31.85,-65.2735353570153,-176.84995));
#152541=CARTESIAN_POINT('Ctrl Pts',(-31.2804134495858,-64.7784013226352,
-177.112484691526));
#152542=CARTESIAN_POINT('Ctrl Pts',(-31.8499999999783,-64.6983511534012,
-176.958917254529));
#152543=CARTESIAN_POINT('Ctrl Pts',(-31.85,-65.2735353570043,-176.981217345763));
#152544=CARTESIAN_POINT('Ctrl Pts',(-31.3881865764622,-64.7632547974255,
-177.371936689315));
#152545=CARTESIAN_POINT('Ctrl Pts',(-31.883334205664,-64.6936663363131,
-177.069891898462));
#152546=CARTESIAN_POINT('Ctrl Pts',(-31.9038865634697,-65.2583888317962,
-177.110943344657));
#152547=CARTESIAN_POINT('Ctrl Pts',(-31.7584267602047,-64.711220932962,
-177.742176873059));
#152548=CARTESIAN_POINT('Ctrl Pts',(-32.0302774403978,-64.6730148114567,
-177.257255781815));
#152549=CARTESIAN_POINT('Ctrl Pts',(-32.0890066553437,-65.2063549673329,
-177.296063436531));
#152550=CARTESIAN_POINT('Ctrl Pts',(-32.0178787579952,-64.6747573326273,
-177.849949999941));
#152551=CARTESIAN_POINT('Ctrl Pts',(-32.1431106784802,-64.6571571339907,
-177.331204220089));
#152552=CARTESIAN_POINT('Ctrl Pts',(-32.2187326542366,-65.1698913669989,
-177.34995));
#152553=CARTESIAN_POINT('Ctrl Pts',(-32.28041344952,-64.6378604879421,-177.84995));
#152554=CARTESIAN_POINT('Ctrl Pts',(-32.28041344952,-64.637860487942,-177.34995));
#152555=CARTESIAN_POINT('Ctrl Pts',(-32.35,-65.1329945223129,-177.34995));
#152556=CARTESIAN_POINT('Origin',(-45.4220505312374,-61.7810962706031,-172.64995));
#152557=CARTESIAN_POINT('',(-29.958978566972,-63.954289311524,-171.64995));
#152558=CARTESIAN_POINT('Origin',(-29.958978566972,-63.954289311524,-172.64995));
#152559=CARTESIAN_POINT('',(-31.7108268990399,-63.7080830846632,-171.64995));
#152560=CARTESIAN_POINT('Ctrl Pts',(-26.2234488624093,-65.1680142434972,
-171.34400271074));
#152561=CARTESIAN_POINT('Ctrl Pts',(-26.1751497442534,-65.4958993451584,
-171.625426858395));
#152562=CARTESIAN_POINT('Ctrl Pts',(-26.0394480946395,-65.5149709682656,
-172.038055421481));
#152563=CARTESIAN_POINT('Ctrl Pts',(-26.5325022452051,-65.072358231615,
-171.399245459895));
#152564=CARTESIAN_POINT('Ctrl Pts',(-26.5059850091802,-65.4494034808673,
-171.691392643103));
#152565=CARTESIAN_POINT('Ctrl Pts',(-26.3688360080808,-65.4686785159697,
-172.14852124047));
#152566=CARTESIAN_POINT('Ctrl Pts',(-26.843027692162,-64.9750314285332,
-171.444032296926));
#152567=CARTESIAN_POINT('Ctrl Pts',(-26.8344935945357,-65.4032346100804,
-171.736704292719));
#152568=CARTESIAN_POINT('Ctrl Pts',(-26.7013989289162,-65.4219398454845,
-172.23811459301));
#152569=CARTESIAN_POINT('Ctrl Pts',(-27.4650077428683,-64.7776672125821,
-171.519686348695));
#152570=CARTESIAN_POINT('Ctrl Pts',(-27.4914924972326,-65.3108994359038,
-171.799283317704));
#152571=CARTESIAN_POINT('Ctrl Pts',(-27.3705571684413,-65.3278957879536,
-172.38942269823));
#152572=CARTESIAN_POINT('Ctrl Pts',(-27.7764978537267,-64.6776202239548,
-171.550373470332));
#152573=CARTESIAN_POINT('Ctrl Pts',(-27.8213068579945,-65.2645470503453,
-171.81528847728));
#152574=CARTESIAN_POINT('Ctrl Pts',(-27.7072474293082,-65.2805770576552,
-172.450796940493));
#152575=CARTESIAN_POINT('Ctrl Pts',(-28.7113572324553,-64.3737932440126,
-171.624291948599));
#152576=CARTESIAN_POINT('Ctrl Pts',(-28.8291547927028,-65.1229032603379,
-171.822805263071));
#152577=CARTESIAN_POINT('Ctrl Pts',(-28.7226827355371,-65.1378669321315,
-172.598633897542));
#152578=CARTESIAN_POINT('Ctrl Pts',(-29.3350621276793,-64.1663451413114,
-171.64995));
#152579=CARTESIAN_POINT('Ctrl Pts',(-29.4938163229,-65.0294911740669,-171.766054775631));
#152580=CARTESIAN_POINT('Ctrl Pts',(-29.4067311934443,-65.0417301908804,
-172.64994999751));
#152581=CARTESIAN_POINT('Ctrl Pts',(-29.958978566972,-63.954289311524,-171.64995));
#152582=CARTESIAN_POINT('Ctrl Pts',(-30.098151667932,-64.9445573802655,
-171.64995));
#152583=CARTESIAN_POINT('Ctrl Pts',(-30.098151667932,-64.9445573802656,
-172.64995));
#152584=CARTESIAN_POINT('Ctrl Pts',(-26.2234488624093,-65.1680142434972,
-171.34400271074));
#152585=CARTESIAN_POINT('Ctrl Pts',(-26.5325022452051,-65.072358231615,
-171.399245459895));
#152586=CARTESIAN_POINT('Ctrl Pts',(-26.843027692162,-64.9750314285332,
-171.444032296926));
#152587=CARTESIAN_POINT('Ctrl Pts',(-27.4650077428683,-64.7776672125821,
-171.519686348695));
#152588=CARTESIAN_POINT('Ctrl Pts',(-27.7764978537267,-64.6776202239548,
-171.550373470332));
#152589=CARTESIAN_POINT('Ctrl Pts',(-28.7113572324553,-64.3737932440126,
-171.624291948599));
#152590=CARTESIAN_POINT('Ctrl Pts',(-29.3350621276793,-64.1663451413114,
-171.64995));
#152591=CARTESIAN_POINT('Ctrl Pts',(-29.958978566972,-63.954289311524,-171.64995));
#152592=CARTESIAN_POINT('Ctrl Pts',(-42.5,-54.58000002,-171.14995));
#152593=CARTESIAN_POINT('Ctrl Pts',(-41.5,-54.58000002,-171.14995));
#152594=CARTESIAN_POINT('Ctrl Pts',(-41.5,-55.58000002,-171.14995));
#152595=CARTESIAN_POINT('Ctrl Pts',(-42.5,-54.58000002,-171.64995));
#152596=CARTESIAN_POINT('Ctrl Pts',(-41.5,-54.58000002,-171.64995));
#152597=CARTESIAN_POINT('Ctrl Pts',(-41.5,-55.58000002,-171.64995));
#152598=CARTESIAN_POINT('Ctrl Pts',(-42.5,-55.08000002,-171.64995));
#152599=CARTESIAN_POINT('Ctrl Pts',(-42.,-55.08000002,-171.64995));
#152600=CARTESIAN_POINT('Ctrl Pts',(-42.,-55.58000002,-171.64995));
#152601=CARTESIAN_POINT('Ctrl Pts',(-25.1782808829885,-54.58000002,-147.977025477683));
#152602=CARTESIAN_POINT('Ctrl Pts',(-23.9800829025888,-54.5800000200001,
-149.152655882413));
#152603=CARTESIAN_POINT('Ctrl Pts',(-23.0246263600192,-55.5929437980769,
-150.090116786386));
#152604=CARTESIAN_POINT('Ctrl Pts',(-23.9836910796608,-54.58000002,-146.759504150767));
#152605=CARTESIAN_POINT('Ctrl Pts',(-22.8379194752343,-54.5800000199763,
-147.932452641776));
#152606=CARTESIAN_POINT('Ctrl Pts',(-21.9091489271198,-55.5502169050949,
-148.872607854072));
#152607=CARTESIAN_POINT('Ctrl Pts',(-22.7503247929853,-54.58000002,-145.568800995698));
#152608=CARTESIAN_POINT('Ctrl Pts',(-21.6573291961429,-54.58000002,-146.736008441848));
#152609=CARTESIAN_POINT('Ctrl Pts',(-20.7612402155903,-55.5070450251362,
-147.681892304448));
#152610=CARTESIAN_POINT('Ctrl Pts',(-20.1860325764608,-54.58000002,-143.268341382183));
#152611=CARTESIAN_POINT('Ctrl Pts',(-19.2052975266984,-54.58000002,-144.424597244368));
#152612=CARTESIAN_POINT('Ctrl Pts',(-18.3837542309683,-55.4210082419989,
-145.38143269084));
#152613=CARTESIAN_POINT('Ctrl Pts',(-18.8677311043704,-54.58000002,-142.169807438416));
#152614=CARTESIAN_POINT('Ctrl Pts',(-17.9461389525456,-54.58000002,-143.320329501862));
#152615=CARTESIAN_POINT('Ctrl Pts',(-17.165895474142,-55.3785603713206,
-144.282911778325));
#152616=CARTESIAN_POINT('Ctrl Pts',(-17.5014165897211,-54.58000002,-141.139869854338));
#152617=CARTESIAN_POINT('Ctrl Pts',(-16.6396978513013,-54.5800000199999,
-142.283025361002));
#152618=CARTESIAN_POINT('Ctrl Pts',(-15.9085533562516,-55.3376384323294,
-143.252961163042));
#152619=CARTESIAN_POINT('Ctrl Pts',(-17.55,-54.58000002,-141.176536909659));
#152620=CARTESIAN_POINT('Ctrl Pts',(-17.9693769714652,-54.5800000200003,
-141.49343498957));
#152621=CARTESIAN_POINT('Ctrl Pts',(-18.3834419174563,-54.5800000200088,
-141.816182952557));
#152622=CARTESIAN_POINT('Ctrl Pts',(-18.7928766486271,-54.5800000200341,
-142.14446893926));
#152623=CARTESIAN_POINT('Ctrl Pts',(-19.2164906824831,-54.5800000200604,
-142.48412393308));
#152624=CARTESIAN_POINT('Ctrl Pts',(-19.635148044907,-54.5800000201049,
-142.829707458939));
#152625=CARTESIAN_POINT('Ctrl Pts',(-20.0495713966389,-54.5800000201721,
-143.180920598249));
#152626=CARTESIAN_POINT('Ctrl Pts',(-20.488326023268,-54.5800000202432,
-143.552753867686));
#152627=CARTESIAN_POINT('Ctrl Pts',(-20.9223347029624,-54.58000002034,-143.930897445283));
#152628=CARTESIAN_POINT('Ctrl Pts',(-21.3524219961151,-54.5800000204563,
-144.315043885279));
#152629=CARTESIAN_POINT('Ctrl Pts',(-21.3910234228925,-54.5800000204667,
-144.349522003818));
#152630=CARTESIAN_POINT('Ctrl Pts',(-21.4295932412714,-54.5800000204773,
-144.384048506611));
#152631=CARTESIAN_POINT('Ctrl Pts',(-21.4681320362146,-54.580000020488,
-144.418623187423));
#152632=CARTESIAN_POINT('Ctrl Pts',(-21.9304021275721,-54.5800000206166,
-144.83334401305));
#152633=CARTESIAN_POINT('Ctrl Pts',(-22.3865711849682,-54.5800000207665,
-145.253534976228));
#152634=CARTESIAN_POINT('Ctrl Pts',(-22.8375326449957,-54.580000020912,
-145.679007211413));
#152635=CARTESIAN_POINT('Ctrl Pts',(-22.9587258346797,-54.5800000209511,
-145.793350324682));
#152636=CARTESIAN_POINT('Ctrl Pts',(-23.0795426741296,-54.5800000209898,
-145.90807504421));
#152637=CARTESIAN_POINT('Ctrl Pts',(-23.2,-54.5800000210274,-146.023178055809));
#152638=CARTESIAN_POINT('Origin',(3.3975957231091E-14,-70.08000002,-174.34995));
#152639=CARTESIAN_POINT('',(-41.5,-73.08000002,-174.34995));
#152640=CARTESIAN_POINT('Ctrl Pts',(-16.443141398898,-54.58000002,-140.363430177307));
#152641=CARTESIAN_POINT('Ctrl Pts',(-15.630331507009,-54.5800000199999,
-141.502754952306));
#152642=CARTESIAN_POINT('Ctrl Pts',(-14.935633130959,-55.3065630024253,
-142.47652148601));
#152643=CARTESIAN_POINT('Ctrl Pts',(-15.3397373006696,-54.58000002,-139.576246587186));
#152644=CARTESIAN_POINT('Ctrl Pts',(-14.5800220275964,-54.580000020014,
-140.713030388695));
#152645=CARTESIAN_POINT('Ctrl Pts',(-13.9222087476243,-55.2748272571858,
-141.68934947009));
#152646=CARTESIAN_POINT('Ctrl Pts',(-14.2001096642283,-54.58000002,-138.832914681508));
#152647=CARTESIAN_POINT('Ctrl Pts',(-13.4942101985199,-54.5800000200048,
-139.965671699013));
#152648=CARTESIAN_POINT('Ctrl Pts',(-12.8784929287096,-55.2441433795399,
-140.946005990295));
#152649=CARTESIAN_POINT('Ctrl Pts',(-11.8242610588971,-54.58000002,-137.462982383337));
#152650=CARTESIAN_POINT('Ctrl Pts',(-11.2325518044464,-54.5800000199952,
-138.58879503276));
#152651=CARTESIAN_POINT('Ctrl Pts',(-10.7090288904129,-55.1865297732718,
-139.576073691957));
#152652=CARTESIAN_POINT('Ctrl Pts',(-10.6074840054802,-54.58000002,-136.847973525117));
#152653=CARTESIAN_POINT('Ctrl Pts',(-10.0748797157148,-54.5800000199999,
-137.970225859417));
#152654=CARTESIAN_POINT('Ctrl Pts',(-9.6010395318864,-55.1600903081647,
-138.961065386249));
#152655=CARTESIAN_POINT('Ctrl Pts',(-9.35547519799418,-54.58000002,-136.31962263586));
#152656=CARTESIAN_POINT('Ctrl Pts',(-8.88330739463766,-54.58000002,-137.438496970103));
#152657=CARTESIAN_POINT('Ctrl Pts',(-8.46374531288877,-55.1370659744517,
-138.432713944563));
#152658=CARTESIAN_POINT('Ctrl Pts',(-9.4,-54.58000002,-136.338455187671));
#152659=CARTESIAN_POINT('Ctrl Pts',(-9.92110496058458,-54.5800000200001,
-136.559368584537));
#152660=CARTESIAN_POINT('Ctrl Pts',(-10.4350703325249,-54.5800000200483,
-136.794854049277));
#152661=CARTESIAN_POINT('Ctrl Pts',(-10.9425445776727,-54.5800000201757,
-137.043577637514));
#152662=CARTESIAN_POINT('Ctrl Pts',(-11.3976304732259,-54.58000002029,-137.266624615721));
#152663=CARTESIAN_POINT('Ctrl Pts',(-11.8474960215409,-54.5800000203574,
-137.500318485596));
#152664=CARTESIAN_POINT('Ctrl Pts',(-12.2925996107723,-54.5800000201853,
-137.743731583458));
#152665=CARTESIAN_POINT('Ctrl Pts',(-12.5336925965022,-54.5800000200921,
-137.875577724331));
#152666=CARTESIAN_POINT('Ctrl Pts',(-12.7734820900616,-54.5800000201101,
-138.010349990831));
#152667=CARTESIAN_POINT('Ctrl Pts',(-13.0121639376423,-54.580000020184,
-138.147985687537));
#152668=CARTESIAN_POINT('Ctrl Pts',(-13.3646805607945,-54.580000020293,
-138.351264116625));
#152669=CARTESIAN_POINT('Ctrl Pts',(-13.713070843513,-54.5800000206454,
-138.55976634471));
#152670=CARTESIAN_POINT('Ctrl Pts',(-14.058084756869,-54.5800000210433,
-138.77339084118));
#152671=CARTESIAN_POINT('Ctrl Pts',(-14.3916633624478,-54.580000021428,
-138.979934864164));
#152672=CARTESIAN_POINT('Ctrl Pts',(-14.7220850961472,-54.5800000217332,
-139.191268004988));
#152673=CARTESIAN_POINT('Ctrl Pts',(-15.05,-54.580000021344,-139.407335470919));
#152674=CARTESIAN_POINT('Ctrl Pts',(-1.09388780931665,-55.0499912502469,
-136.472972564846));
#152675=CARTESIAN_POINT('Ctrl Pts',(-1.14986049246831,-54.5800000199999,
-135.468532548998));
#152676=CARTESIAN_POINT('Ctrl Pts',(-1.21164037634558,-54.58000002,-134.359881256142));
#152677=CARTESIAN_POINT('Ctrl Pts',(-2.06753743423328,-55.0527136176872,
-136.533065609844));
#152678=CARTESIAN_POINT('Ctrl Pts',(-2.1734236725105,-54.580000019985,-135.528951041927));
#152679=CARTESIAN_POINT('Ctrl Pts',(-2.29002416952399,-54.58000002,-134.419974475838));
#152680=CARTESIAN_POINT('Ctrl Pts',(-3.03750542044518,-55.059063567472,
-136.673166196403));
#152681=CARTESIAN_POINT('Ctrl Pts',(-3.19311650329436,-54.58000002,-135.669893399192));
#152682=CARTESIAN_POINT('Ctrl Pts',(-3.36400336137312,-54.58000002,-134.560074887715));
#152683=CARTESIAN_POINT('Ctrl Pts',(-4.48820368733454,-55.0737025194561,
-136.999007240366));
#152684=CARTESIAN_POINT('Ctrl Pts',(-4.71607294932927,-54.5800000199999,
-135.997360222398));
#152685=CARTESIAN_POINT('Ctrl Pts',(-4.96860300664728,-54.58000002,-134.885915931654));
#152686=CARTESIAN_POINT('Ctrl Pts',(-4.97306841018422,-55.0794633322322,
-137.127585972214));
#152687=CARTESIAN_POINT('Ctrl Pts',(-5.22506238654006,-54.5800000199999,
-136.126634241129));
#152688=CARTESIAN_POINT('Ctrl Pts',(-5.50462478218054,-54.58000002,-135.014494663549));
#152689=CARTESIAN_POINT('Ctrl Pts',(-5.92682186653397,-55.0923918960893,
-137.417551068811));
#152690=CARTESIAN_POINT('Ctrl Pts',(-6.22569420503589,-54.58000002,-136.418114793059));
#152691=CARTESIAN_POINT('Ctrl Pts',(-6.5582931505392,-54.58000002,-135.304459760069));
#152692=CARTESIAN_POINT('Ctrl Pts',(-6.39676634858691,-55.099562033378,
-137.578988956132));
#152693=CARTESIAN_POINT('Ctrl Pts',(-6.71851642939749,-54.58000002,-136.580417857494));
#152694=CARTESIAN_POINT('Ctrl Pts',(-7.07711031169138,-54.58000002,-135.46589761626));
#152695=CARTESIAN_POINT('Ctrl Pts',(-6.86052929923582,-55.1073474746665,
-137.755279275981));
#152696=CARTESIAN_POINT('Ctrl Pts',(-7.20434315889942,-54.58000002,-136.757552063338));
#152697=CARTESIAN_POINT('Ctrl Pts',(-7.58869434220596,-54.58000002,-135.642187967278));
#152698=CARTESIAN_POINT('Ctrl Pts',(-1.24999999852556,-54.58000002,-134.362052703156));
#152699=CARTESIAN_POINT('Ctrl Pts',(-1.8558687299695,-54.58000002,-134.396884061811));
#152700=CARTESIAN_POINT('Ctrl Pts',(-2.45821169814561,-54.5800000199999,
-134.456836856573));
#152701=CARTESIAN_POINT('Ctrl Pts',(-3.05717008780528,-54.5800000200001,
-134.540898522254));
#152702=CARTESIAN_POINT('Ctrl Pts',(-3.40705616968019,-54.5800000200002,
-134.590003781231));
#152703=CARTESIAN_POINT('Ctrl Pts',(-3.75578723672687,-54.5800000200004,
-134.647336949705));
#152704=CARTESIAN_POINT('Ctrl Pts',(-4.10339093154591,-54.5800000200016,
-134.712704370428));
#152705=CARTESIAN_POINT('Ctrl Pts',(-4.21364342719022,-54.580000020002,
-134.733437525386));
#152706=CARTESIAN_POINT('Ctrl Pts',(-4.32374689616092,-54.5800000200024,
-134.754971981414));
#152707=CARTESIAN_POINT('Ctrl Pts',(-4.43373542753185,-54.5800000200027,
-134.777307325963));
#152708=CARTESIAN_POINT('Ctrl Pts',(-4.67988879728086,-54.5800000200034,
-134.827293631415));
#152709=CARTESIAN_POINT('Ctrl Pts',(-4.92593529130837,-54.5800000200038,
-134.881432381241));
#152710=CARTESIAN_POINT('Ctrl Pts',(-5.17124777564329,-54.5800000200039,
-134.939444408488));
#152711=CARTESIAN_POINT('Ctrl Pts',(-5.41900393393831,-54.580000020004,
-134.998034321043));
#152712=CARTESIAN_POINT('Ctrl Pts',(-5.6660135363309,-54.5800000200037,
-135.060575714351));
#152713=CARTESIAN_POINT('Ctrl Pts',(-5.91161937020563,-54.5800000200032,
-135.126829777541));
#152714=CARTESIAN_POINT('Ctrl Pts',(-5.95160365908193,-54.5800000200032,
-135.137615847073));
#152715=CARTESIAN_POINT('Ctrl Pts',(-5.99155067840898,-54.5800000200031,
-135.148500406429));
#152716=CARTESIAN_POINT('Ctrl Pts',(-6.03145750349794,-54.580000020003,
-135.159482527522));
#152717=CARTESIAN_POINT('Ctrl Pts',(-6.28934481311126,-54.5800000200026,
-135.230451582474));
#152718=CARTESIAN_POINT('Ctrl Pts',(-6.54583590336334,-54.580000020002,
-135.305503306745));
#152719=CARTESIAN_POINT('Ctrl Pts',(-6.80143368808723,-54.5800000200016,
-135.384644793435));
#152720=CARTESIAN_POINT('Ctrl Pts',(-6.83430358210449,-54.5800000200015,
-135.394822394476));
#152721=CARTESIAN_POINT('Ctrl Pts',(-6.86715867181465,-54.5800000200014,
-135.405067695209));
#152722=CARTESIAN_POINT('Ctrl Pts',(-6.9,-54.5800000200014,-135.415380765739));
#152723=CARTESIAN_POINT('Origin',(0.,-12.9675000200281,-170.64995));
#152724=CARTESIAN_POINT('Origin',(0.,-12.9675000200281,-171.64995));
#152725=CARTESIAN_POINT('Origin',(0.,-12.9675000200281,-171.07256826174));
#152726=CARTESIAN_POINT('Origin',(3.3975957231091E-14,-70.08000002,-174.34995));
#152727=CARTESIAN_POINT('Origin',(-60.,-54.58000002,-55.24995));
#152728=CARTESIAN_POINT('Origin',(-60.,-54.58000002,-55.24995));
#152729=CARTESIAN_POINT('Origin',(3.54807775957937E-14,-73.08000002,3.11172719585489E-30));
#152730=CARTESIAN_POINT('Origin',(-60.,-54.58000002,-55.24995));
#152731=CARTESIAN_POINT('Origin',(-60.,-2.55003103885676E-14,0.));
#152732=CARTESIAN_POINT('',(-60.,28.41999998,-174.34995));
#152733=CARTESIAN_POINT('Origin',(-60.,-2.55003103885676E-14,0.));
#152734=CARTESIAN_POINT('',(-60.,28.41999998,-174.34995));
#152735=CARTESIAN_POINT('Origin',(-60.,28.41999998,-177.34995));
#152736=CARTESIAN_POINT('',(-57.,-54.58000002,-177.34995));
#152737=CARTESIAN_POINT('Origin',(0.,-12.9675000200281,-171.64995));
#152738=CARTESIAN_POINT('Ctrl Pts',(-39.8501516349278,-30.4480624610812,
-139.515559008643));
#152739=CARTESIAN_POINT('Ctrl Pts',(-39.8776986028551,-31.1793494861265,
-140.199588507397));
#152740=CARTESIAN_POINT('Ctrl Pts',(-39.905579888437,-31.8977486430871,
-140.90539342064));
#152741=CARTESIAN_POINT('Ctrl Pts',(-39.9335715388522,-32.6056681732837,
-141.62920925267));
#152742=CARTESIAN_POINT('Ctrl Pts',(-39.9805442496755,-33.7936259708707,
-142.843842590218));
#152743=CARTESIAN_POINT('Ctrl Pts',(-40.0273699621533,-34.9400872995304,
-144.097130127809));
#152744=CARTESIAN_POINT('Ctrl Pts',(-40.0734472049714,-36.0537916893395,
-145.374999488024));
#152745=CARTESIAN_POINT('Ctrl Pts',(-40.0751063896396,-36.0938885093696,
-145.421033595465));
#152746=CARTESIAN_POINT('Ctrl Pts',(-39.,-37.0899493427105,-144.4917610531));
#152747=CARTESIAN_POINT('Ctrl Pts',(-39.,-38.3588510407228,-143.307942286761));
#152748=CARTESIAN_POINT('Ctrl Pts',(-40.0284942517968,-34.9676084789312,
-144.127227814579));
#152749=CARTESIAN_POINT('Ctrl Pts',(-39.,-35.9377773398718,-143.195151285356));
#152750=CARTESIAN_POINT('Ctrl Pts',(-39.,-37.1517836400886,-142.014121037894));
#152751=CARTESIAN_POINT('Ctrl Pts',(-39.98110816979,-33.8078877259523,-142.858424592381));
#152752=CARTESIAN_POINT('Ctrl Pts',(-38.9999999999999,-34.7456377245003,
-141.920028658586));
#152753=CARTESIAN_POINT('Ctrl Pts',(-39.,-35.9043030651865,-140.745333283629));
#152754=CARTESIAN_POINT('Ctrl Pts',(-39.8860349079144,-31.4034486206149,
-140.399993912959));
#152755=CARTESIAN_POINT('Ctrl Pts',(-39.,-32.2660355551645,-139.44936091542));
#152756=CARTESIAN_POINT('Ctrl Pts',(-39.,-33.3065355961441,-138.286902604304));
#152757=CARTESIAN_POINT('Ctrl Pts',(-39.838820917574,-30.1709959811911,
-139.222722930622));
#152758=CARTESIAN_POINT('Ctrl Pts',(-39.,-30.991536347315,-138.265657625916));
#152759=CARTESIAN_POINT('Ctrl Pts',(-39.,-31.969482004655,-137.109613636004));
#152760=CARTESIAN_POINT('Ctrl Pts',(-39.7930043034378,-28.8965637495112,
-138.115832334683));
#152761=CARTESIAN_POINT('Ctrl Pts',(-38.9999999999999,-29.666065684619,
-137.150287618997));
#152762=CARTESIAN_POINT('Ctrl Pts',(-39.,-30.5806161032665,-136.00274102598));
#152763=CARTESIAN_POINT('Ctrl Pts',(-39.0000000012919,-36.28000002,-141.149515588739));
#152764=CARTESIAN_POINT('Ctrl Pts',(-39.0000000010156,-35.8345332337773,
-140.70226392125));
#152765=CARTESIAN_POINT('Ctrl Pts',(-39.0000000008023,-35.3840176213637,
-140.260002181398));
#152766=CARTESIAN_POINT('Ctrl Pts',(-39.0000000006337,-34.9275493437178,
-139.822886348177));
#152767=CARTESIAN_POINT('Ctrl Pts',(-39.0000000005941,-34.8204877683556,
-139.720363758959));
#152768=CARTESIAN_POINT('Ctrl Pts',(-39.0000000005571,-34.7130985462023,
-139.618124369438));
#152769=CARTESIAN_POINT('Ctrl Pts',(-39.0000000005223,-34.6053696556425,
-139.516170434427));
#152770=CARTESIAN_POINT('Ctrl Pts',(-39.0000000003865,-34.1849244503591,
-139.118263773436));
#152771=CARTESIAN_POINT('Ctrl Pts',(-39.0000000002855,-33.7606942182181,
-138.725996583524));
#152772=CARTESIAN_POINT('Ctrl Pts',(-39.0000000002095,-33.3318521218421,
-138.33965468812));
#152773=CARTESIAN_POINT('Ctrl Pts',(-39.0000000001368,-32.9217240240916,
-137.970172149018));
#152774=CARTESIAN_POINT('Ctrl Pts',(-39.000000000087,-32.5073780349993,
-137.606108713902));
#152775=CARTESIAN_POINT('Ctrl Pts',(-39.000000000054,-32.0880629354048,
-137.247752417324));
#152776=CARTESIAN_POINT('Ctrl Pts',(-39.0000000000227,-31.6891890378919,
-136.906865640642));
#152777=CARTESIAN_POINT('Ctrl Pts',(-39.0000000000065,-31.285818826212,
-136.571142959481));
#152778=CARTESIAN_POINT('Ctrl Pts',(-39.0000000000016,-30.8772772476494,
-136.240870924102));
#152779=CARTESIAN_POINT('Ctrl Pts',(-39.0000000000006,-30.7950629150974,
-136.174407444314));
#152780=CARTESIAN_POINT('Ctrl Pts',(-39.0000000000001,-30.7126390581343,
-136.108164834603));
#152781=CARTESIAN_POINT('Ctrl Pts',(-39.,-30.63000002,-136.04214564125));
#152782=CARTESIAN_POINT('Origin',(-39.,46.91999998,-129.34995));
#152783=CARTESIAN_POINT('Origin',(-57.,-2.42462934179819E-14,-174.34995));
#152784=CARTESIAN_POINT('Origin',(-60.,28.41999998,-177.34995));
#152785=CARTESIAN_POINT('',(-57.,-54.58000002,-177.34995));
#152786=CARTESIAN_POINT('',(-60.,-29.13000002,-177.34995));
#152787=CARTESIAN_POINT('Origin',(-57.,-2.42462934179819E-14,-174.34995));
#152788=CARTESIAN_POINT('',(-60.,28.41999998,-174.34995));
#152789=CARTESIAN_POINT('Origin',(-60.,-2.55003103885676E-14,0.));
#152790=CARTESIAN_POINT('Origin',(-60.,-29.13000002,-176.84995));
#152791=CARTESIAN_POINT('Origin',(0.,-12.9675000200281,-171.64995));
#152792=CARTESIAN_POINT('Ctrl Pts',(-39.5912209089345,-22.3752378108182,
-133.464034181247));
#152793=CARTESIAN_POINT('Ctrl Pts',(-39.6121374457797,-23.2156616534414,
-133.924199547062));
#152794=CARTESIAN_POINT('Ctrl Pts',(-39.6349219111963,-24.0387135538522,
-134.431982361478));
#152795=CARTESIAN_POINT('Ctrl Pts',(-39.6912633163793,-25.928116182914,
-135.710428138755));
#152796=CARTESIAN_POINT('Ctrl Pts',(-39.7252977745181,-26.9648643074353,
-136.499221044835));
#152797=CARTESIAN_POINT('Ctrl Pts',(-39.7602371906927,-27.9700232578782,
-137.330324735012));
#152798=CARTESIAN_POINT('Ctrl Pts',(-39.7614953849933,-28.006195589491,
-137.360262497367));
#152799=CARTESIAN_POINT('Ctrl Pts',(-38.9999999999999,-28.7416759820709,
-136.390803950004));
#152800=CARTESIAN_POINT('Ctrl Pts',(-39.,-29.6092937616716,-135.247171188664));
#152801=CARTESIAN_POINT('Ctrl Pts',(-39.7261148635016,-26.9897399838167,
-136.518160398014));
#152802=CARTESIAN_POINT('Ctrl Pts',(-38.9999999999855,-27.6876355340531,
-135.545932666416));
#152803=CARTESIAN_POINT('Ctrl Pts',(-39.,-28.4992718278429,-134.405052285569));
#152804=CARTESIAN_POINT('Ctrl Pts',(-39.6916499750401,-25.9410827372237,
-135.719201830687));
#152805=CARTESIAN_POINT('Ctrl Pts',(-39.,-26.5955422649145,-134.742448815396));
#152806=CARTESIAN_POINT('Ctrl Pts',(-39.,-27.350294560115,-133.606110521891));
#152807=CARTESIAN_POINT('Ctrl Pts',(-39.6264336205064,-23.7540596888349,
-134.239374112649));
#152808=CARTESIAN_POINT('Ctrl Pts',(-38.9999999999999,-24.3121967691435,
-133.254719568795));
#152809=CARTESIAN_POINT('Ctrl Pts',(-39.,-24.9455608509554,-132.126282804037));
#152810=CARTESIAN_POINT('Ctrl Pts',(-39.5962661790751,-22.6346054925691,
-133.57169567032));
#152811=CARTESIAN_POINT('Ctrl Pts',(-38.9999999999854,-23.1403713306369,
-132.582946581795));
#152812=CARTESIAN_POINT('Ctrl Pts',(-39.,-23.7105874730482,-131.458602080542));
#152813=CARTESIAN_POINT('Ctrl Pts',(-39.5698471421185,-21.4814250807741,
-132.996116063158));
#152814=CARTESIAN_POINT('Ctrl Pts',(-39.,-21.9292251340083,-132.003415558585));
#152815=CARTESIAN_POINT('Ctrl Pts',(-39.,-22.4346253623973,-130.883024754454));
#152816=CARTESIAN_POINT('Ctrl Pts',(-39.0000000022172,-28.13000002,-134.169022080262));
#152817=CARTESIAN_POINT('Ctrl Pts',(-39.0000000027011,-27.7992138900224,
-133.937908100891));
#152818=CARTESIAN_POINT('Ctrl Pts',(-39.0000000021338,-27.4657185053518,
-133.711655036842));
#152819=CARTESIAN_POINT('Ctrl Pts',(-39.00000000154,-27.1287626917303,-133.490292823799));
#152820=CARTESIAN_POINT('Ctrl Pts',(-39.0000000009697,-26.8052287127277,
-133.277748048811));
#152821=CARTESIAN_POINT('Ctrl Pts',(-39.0000000004972,-26.4785047877958,
-133.06971193157));
#152822=CARTESIAN_POINT('Ctrl Pts',(-39.0000000003364,-26.1478973077855,
-132.866246059588));
#152823=CARTESIAN_POINT('Ctrl Pts',(-39.0000000002123,-25.8927164902428,
-132.709200043712));
#152824=CARTESIAN_POINT('Ctrl Pts',(-39.0000000001809,-25.6361572010218,
-132.555471936139));
#152825=CARTESIAN_POINT('Ctrl Pts',(-39.0000000003918,-25.3779449003587,
-132.405146018542));
#152826=CARTESIAN_POINT('Ctrl Pts',(-39.0000000007921,-24.887736647026,
-132.11975680468));
#152827=CARTESIAN_POINT('Ctrl Pts',(-39.000000000553,-24.3912688192601,
-131.846323735541));
#152828=CARTESIAN_POINT('Ctrl Pts',(-39.0000000002964,-23.8878019342432,
-131.586247706168));
#152829=CARTESIAN_POINT('Ctrl Pts',(-39.0000000000603,-23.42465277012,-131.346998613135));
#152830=CARTESIAN_POINT('Ctrl Pts',(-39.0000000000002,-22.9555805746405,
-131.119053182003));
#152831=CARTESIAN_POINT('Ctrl Pts',(-39.,-22.48000002,-130.903539806302));
#152832=CARTESIAN_POINT('Origin',(-39.,46.91999998,-129.34995));
#152833=CARTESIAN_POINT('Ctrl Pts',(-58.2228448679712,-20.997722377502,
-177.242431000705));
#152834=CARTESIAN_POINT('Ctrl Pts',(-59.9999999999999,-20.9611893120647,
-176.449983597595));
#152835=CARTESIAN_POINT('Ctrl Pts',(-60.,-20.8715629014036,-174.505875827596));
#152836=CARTESIAN_POINT('Ctrl Pts',(-58.19761253134,-21.2014273832679,-177.244315088819));
#152837=CARTESIAN_POINT('Ctrl Pts',(-59.9999999999924,-21.1661125646404,
-176.460241938351));
#152838=CARTESIAN_POINT('Ctrl Pts',(-60.,-21.0755801285197,-174.496470313984));
#152839=CARTESIAN_POINT('Ctrl Pts',(-58.1714292060953,-21.40462514847,-177.246332126402));
#152840=CARTESIAN_POINT('Ctrl Pts',(-60.0000000000095,-21.3701601153011,
-176.471395106131));
#152841=CARTESIAN_POINT('Ctrl Pts',(-60.,-21.2796010327843,-174.487167894352));
#152842=CARTESIAN_POINT('Ctrl Pts',(-58.1443031111633,-21.607263174561,
-177.248493339178));
#152843=CARTESIAN_POINT('Ctrl Pts',(-60.,-21.5731259515601,-176.483536694353));
#152844=CARTESIAN_POINT('Ctrl Pts',(-60.,-21.4836289747507,-174.478062871828));
#152845=CARTESIAN_POINT('Origin',(0.,-12.9675000200281,-171.64995));
#152846=CARTESIAN_POINT('Ctrl Pts',(-39.4710976496822,-14.3145440753934,
-130.89161549018));
#152847=CARTESIAN_POINT('Ctrl Pts',(-39.4728125648223,-14.7530413219124,
-130.92736520195));
#152848=CARTESIAN_POINT('Ctrl Pts',(-39.4753639075638,-15.1920614442498,
-130.980586110252));
#152849=CARTESIAN_POINT('Ctrl Pts',(-39.4825355718676,-16.1247177471361,
-131.130598723552));
#152850=CARTESIAN_POINT('Ctrl Pts',(-39.4873750954154,-16.6176732832087,
-131.232022056041));
#152851=CARTESIAN_POINT('Ctrl Pts',(-39.5043768621473,-18.0582508435763,
-131.589922098221));
#152852=CARTESIAN_POINT('Ctrl Pts',(-39.5191347956219,-18.9899841315148,
-131.902314804673));
#152853=CARTESIAN_POINT('Ctrl Pts',(-39.5365899624517,-19.9017174575869,
-132.27695566545));
#152854=CARTESIAN_POINT('Ctrl Pts',(-39.5372195035444,-19.9345312052232,
-132.290469469449));
#152855=CARTESIAN_POINT('Ctrl Pts',(-39.,-20.3054116348924,-131.293905860767));
#152856=CARTESIAN_POINT('Ctrl Pts',(-39.,-20.720937818584,-130.177378160746));
#152857=CARTESIAN_POINT('Ctrl Pts',(-39.5194895810462,-19.0123420478084,
-131.90982316175));
#152858=CARTESIAN_POINT('Ctrl Pts',(-39.,-19.3374585219745,-130.911526747764));
#152859=CARTESIAN_POINT('Ctrl Pts',(-39.,-19.698133940161,-129.796732169428));
#152860=CARTESIAN_POINT('Ctrl Pts',(-39.5045124277029,-18.0697294738066,
-131.592774070923));
#152861=CARTESIAN_POINT('Ctrl Pts',(-38.9999999999923,-18.3454434179522,
-130.592508390753));
#152862=CARTESIAN_POINT('Ctrl Pts',(-39.,-18.6506584423116,-129.479682762144));
#152863=CARTESIAN_POINT('Ctrl Pts',(-39.4873751859149,-16.6176732464254,
-131.23202224217));
#152864=CARTESIAN_POINT('Ctrl Pts',(-39.0000000000038,-16.8157658206047,
-130.229644160077));
#152865=CARTESIAN_POINT('Ctrl Pts',(-39.,-17.0348936577371,-129.118930933505));
#152866=CARTESIAN_POINT('Ctrl Pts',(-39.4825356614912,-16.1247177152636,
-131.130598909837));
#152867=CARTESIAN_POINT('Ctrl Pts',(-39.,-16.2963199259075,-130.127635847669));
#152868=CARTESIAN_POINT('Ctrl Pts',(-39.,-16.4860091127214,-129.017507601134));
#152869=CARTESIAN_POINT('Ctrl Pts',(-39.4749533438571,-15.1386572025492,
-130.9719965231));
#152870=CARTESIAN_POINT('Ctrl Pts',(-39.,-15.2570331695429,-129.96814976082));
#152871=CARTESIAN_POINT('Ctrl Pts',(-39.,-15.3875914977103,-128.858905214396));
#152872=CARTESIAN_POINT('Ctrl Pts',(-39.4722050319315,-14.6463890166082,
-130.914693311714));
#152873=CARTESIAN_POINT('Ctrl Pts',(-38.9999999999999,-14.7379707288414,
-129.910514022628));
#152874=CARTESIAN_POINT('Ctrl Pts',(-39.,-14.8389953875779,-128.801602009569));
#152875=CARTESIAN_POINT('Ctrl Pts',(-39.4705097325996,-14.1547657662532,
-130.879360876185));
#152876=CARTESIAN_POINT('Ctrl Pts',(-39.,-14.2195253716732,-129.874981182379));
#152877=CARTESIAN_POINT('Ctrl Pts',(-39.,-14.2910120087967,-128.766269567481));
#152878=CARTESIAN_POINT('Ctrl Pts',(-39.0000000000669,-19.98000002,-129.914446011788));
#152879=CARTESIAN_POINT('Ctrl Pts',(-39.0000000001518,-19.6367327840719,
-129.798586081307));
#152880=CARTESIAN_POINT('Ctrl Pts',(-39.0000000002631,-19.2913217887157,
-129.690298412947));
#152881=CARTESIAN_POINT('Ctrl Pts',(-39.0000000003003,-18.9438276300824,
-129.590011167477));
#152882=CARTESIAN_POINT('Ctrl Pts',(-39.0000000003366,-18.6049646905725,
-129.492214902559));
#152883=CARTESIAN_POINT('Ctrl Pts',(-39.0000000003094,-18.2641207496911,
-129.402026657411));
#152884=CARTESIAN_POINT('Ctrl Pts',(-39.0000000002472,-17.9213701519491,
-129.319797180689));
#152885=CARTESIAN_POINT('Ctrl Pts',(-39.0000000002263,-17.8056205245996,
-129.292027626528));
#152886=CARTESIAN_POINT('Ctrl Pts',(-39.0000000002019,-17.6896536077084,
-129.265165339737));
#152887=CARTESIAN_POINT('Ctrl Pts',(-39.0000000001767,-17.5734727602674,
-129.239222565105));
#152888=CARTESIAN_POINT('Ctrl Pts',(-39.0000000001494,-17.4477751466172,
-129.211154730048));
#152889=CARTESIAN_POINT('Ctrl Pts',(-39.0000000001211,-17.3216708975945,
-129.184146383705));
#152890=CARTESIAN_POINT('Ctrl Pts',(-39.0000000000953,-17.1952995452482,
-129.158233426905));
#152891=CARTESIAN_POINT('Ctrl Pts',(-39.0000000000407,-16.9274823440481,
-129.103316426838));
#152892=CARTESIAN_POINT('Ctrl Pts',(-39.0000000000228,-16.6579107580322,
-129.053205467123));
#152893=CARTESIAN_POINT('Ctrl Pts',(-39.0000000000127,-16.3874479062815,
-129.008231038422));
#152894=CARTESIAN_POINT('Ctrl Pts',(-39.0000000000071,-16.2374573286252,
-128.983289570501));
#152895=CARTESIAN_POINT('Ctrl Pts',(-39.0000000000044,-16.0871922946702,
-128.959928670237));
#152896=CARTESIAN_POINT('Ctrl Pts',(-39.0000000000028,-15.9367995435377,
-128.938211682847));
#152897=CARTESIAN_POINT('Ctrl Pts',(-39.,-15.6676875947363,-128.899351426921));
#152898=CARTESIAN_POINT('Ctrl Pts',(-39.0000000000001,-15.3983918170305,
-128.865722188253));
#152899=CARTESIAN_POINT('Ctrl Pts',(-39.,-15.1285853320425,-128.837337411665));
#152900=CARTESIAN_POINT('Ctrl Pts',(-39.,-14.8629886325447,-128.809395522211));
#152901=CARTESIAN_POINT('Ctrl Pts',(-39.,-14.5968970408721,-128.786535808696));
#152902=CARTESIAN_POINT('Ctrl Pts',(-39.,-14.3300000191853,-128.768820409992));
#152903=CARTESIAN_POINT('Origin',(-39.,46.91999998,-129.34995));
#152904=CARTESIAN_POINT('Ctrl Pts',(-58.6998841333603,-12.8234825355735,
-177.223692421544));
#152905=CARTESIAN_POINT('Ctrl Pts',(-59.9999999999999,-12.8247546893956,
-176.329633102893));
#152906=CARTESIAN_POINT('Ctrl Pts',(-60.,-12.8269998197496,-174.751773822184));
#152907=CARTESIAN_POINT('Ctrl Pts',(-58.7002617769471,-12.996381211483,
-177.22367874123));
#152908=CARTESIAN_POINT('Ctrl Pts',(-59.9999999999968,-12.9961202462228,
-176.329584396716));
#152909=CARTESIAN_POINT('Ctrl Pts',(-60.,-12.9956778161511,-174.752013833507));
#152910=CARTESIAN_POINT('Ctrl Pts',(-58.6999592969537,-13.1692782682892,
-177.223689661345));
#152911=CARTESIAN_POINT('Ctrl Pts',(-60.,-13.16751068744,-176.329623133207));
#152912=CARTESIAN_POINT('Ctrl Pts',(-60.,-13.1643444677208,-174.751821305086));
#152913=CARTESIAN_POINT('Ctrl Pts',(-58.6989770498873,-13.3421437200247,
-177.22372531347));
#152914=CARTESIAN_POINT('Ctrl Pts',(-60.,-13.338837622507,-176.329750343386));
#152915=CARTESIAN_POINT('Ctrl Pts',(-60.,-13.3329998199577,-174.75119758399));
#152916=CARTESIAN_POINT('Origin',(0.,-12.9675000200281,-171.64995));
#152917=CARTESIAN_POINT('Ctrl Pts',(-39.532390596256,-6.25584930059378,
-132.186909005141));
#152918=CARTESIAN_POINT('Ctrl Pts',(-39.5154906923694,-7.16492474321995,
-131.82486600692));
#152919=CARTESIAN_POINT('Ctrl Pts',(-39.5012062751564,-8.10027061565897,
-131.522946484679));
#152920=CARTESIAN_POINT('Ctrl Pts',(-39.4801155592828,-9.98786863920294,
-131.0794868627));
#152921=CARTESIAN_POINT('Ctrl Pts',(-39.4733327199609,-10.9147757068085,
-130.938171698301));
#152922=CARTESIAN_POINT('Ctrl Pts',(-39.4702993039609,-11.842906113671,
-130.874975449521));
#152923=CARTESIAN_POINT('Ctrl Pts',(-39.4698735679011,-11.9817787569958,
-130.866104166164));
#152924=CARTESIAN_POINT('Ctrl Pts',(-39.,-11.9280000478899,-129.861650462511));
#152925=CARTESIAN_POINT('Ctrl Pts',(-39.,-11.8686433059622,-128.75301285746));
#152926=CARTESIAN_POINT('Ctrl Pts',(-39.4726650480512,-11.0072303515572,
-130.924266220454));
#152927=CARTESIAN_POINT('Ctrl Pts',(-39.,-10.9001842769389,-129.920145931085));
#152928=CARTESIAN_POINT('Ctrl Pts',(-39.,-10.7823162329457,-128.811175087855));
#152929=CARTESIAN_POINT('Ctrl Pts',(-39.4795992973311,-10.0340735686833,
-131.068631786405));
#152930=CARTESIAN_POINT('Ctrl Pts',(-39.0000000000038,-9.87380260099891,
-130.065440410241));
#152931=CARTESIAN_POINT('Ctrl Pts',(-39.,-9.69789923172707,-128.955540477711));
#152932=CARTESIAN_POINT('Ctrl Pts',(-39.5013352696214,-8.08872573977277,
-131.525658760403));
#152933=CARTESIAN_POINT('Ctrl Pts',(-38.9999999999961,-7.82478234255028,
-130.525007038766));
#152934=CARTESIAN_POINT('Ctrl Pts',(-39.,-7.5328018765656,-129.41256745169));
#152935=CARTESIAN_POINT('Ctrl Pts',(-39.5158343666262,-7.14245811524402,
-131.8321301746));
#152936=CARTESIAN_POINT('Ctrl Pts',(-39.000000000015,-6.82873706011098,
-130.833383690437));
#152937=CARTESIAN_POINT('Ctrl Pts',(-39.,-6.48098994967646,-129.719043469502));
#152938=CARTESIAN_POINT('Ctrl Pts',(-39.5330007209533,-6.22310181331709,
-132.199981346222));
#152939=CARTESIAN_POINT('Ctrl Pts',(-39.,-5.86351575546646,-131.202920178865));
#152940=CARTESIAN_POINT('Ctrl Pts',(-39.,-5.4610240206487,-130.086890037519));
#152941=CARTESIAN_POINT('Ctrl Pts',(-39.,-11.8300000219165,-128.755118230443));
#152942=CARTESIAN_POINT('Ctrl Pts',(-39.,-11.2456383392957,-128.787506003178));
#152943=CARTESIAN_POINT('Ctrl Pts',(-38.9999999999998,-10.6643296819666,
-128.844689763199));
#152944=CARTESIAN_POINT('Ctrl Pts',(-39.0000000000002,-10.0859609278487,
-128.925742270509));
#152945=CARTESIAN_POINT('Ctrl Pts',(-39.0000000000004,-9.71348092877506,
-128.977941559687));
#152946=CARTESIAN_POINT('Ctrl Pts',(-39.0000000000007,-9.34222031417317,
-129.040041718412));
#152947=CARTESIAN_POINT('Ctrl Pts',(-39.0000000000031,-8.97214920379055,
-129.111806478628));
#152948=CARTESIAN_POINT('Ctrl Pts',(-39.0000000000039,-8.85321569986176,
-129.134870247055));
#152949=CARTESIAN_POINT('Ctrl Pts',(-39.0000000000046,-8.73429069407208,
-129.1589539896));
#152950=CARTESIAN_POINT('Ctrl Pts',(-39.0000000000049,-8.61535199981085,
-129.184060813321));
#152951=CARTESIAN_POINT('Ctrl Pts',(-39.0000000000057,-8.3170598050556,
-129.247027450022));
#152952=CARTESIAN_POINT('Ctrl Pts',(-39.0000000000046,-8.02087151391859,
-129.315956118525));
#152953=CARTESIAN_POINT('Ctrl Pts',(-39.0000000000032,-7.72648278144854,
-129.390626430169));
#152954=CARTESIAN_POINT('Ctrl Pts',(-39.0000000000018,-7.42024264682867,
-129.468302793997));
#152955=CARTESIAN_POINT('Ctrl Pts',(-39.0000000000006,-7.11594965101859,
-129.552192661458));
#152956=CARTESIAN_POINT('Ctrl Pts',(-39.0000000000002,-6.81328756599581,
-129.642098960196));
#152957=CARTESIAN_POINT('Ctrl Pts',(-39.,-6.60142553226265,-129.705032945781));
#152958=CARTESIAN_POINT('Ctrl Pts',(-39.,-6.39036319103641,-129.770916038733));
#152959=CARTESIAN_POINT('Ctrl Pts',(-39.,-6.18000018270165,-129.839693348042));
#152960=CARTESIAN_POINT('Origin',(-39.,46.91999998,-129.34995));
#152961=CARTESIAN_POINT('Ctrl Pts',(-58.1727505513103,-4.55147683639116,
-177.246631327017));
#152962=CARTESIAN_POINT('Ctrl Pts',(-59.9999999999999,-4.58657792455373,
-176.471369022158));
#152963=CARTESIAN_POINT('Ctrl Pts',(-60.,-4.67636962353871,-174.488179236421));
#152964=CARTESIAN_POINT('Ctrl Pts',(-58.1991963791488,-4.75453073304115,
-177.244581482931));
#152965=CARTESIAN_POINT('Ctrl Pts',(-60.,-4.78987454640717,-176.45995577904));
#152966=CARTESIAN_POINT('Ctrl Pts',(-60.,-4.88047860745801,-174.497420557097));
#152967=CARTESIAN_POINT('Ctrl Pts',(-58.224696806329,-4.95813196877357,
-177.242671121043));
#152968=CARTESIAN_POINT('Ctrl Pts',(-59.9999999999904,-4.99421808034748,
-176.449490545983));
#152969=CARTESIAN_POINT('Ctrl Pts',(-60.,-5.08458311893969,-174.506824441727));
#152970=CARTESIAN_POINT('Ctrl Pts',(-58.2492435654384,-5.16222748868144,
-177.240889086276));
#152971=CARTESIAN_POINT('Ctrl Pts',(-60.,-5.19940519654632,-176.439881014021));
#152972=CARTESIAN_POINT('Ctrl Pts',(-60.,-5.28868572332295,-174.51629758862));
#152973=CARTESIAN_POINT('Origin',(0.,-12.9675000200281,-171.64995));
#152974=CARTESIAN_POINT('Ctrl Pts',(-39.7525219240432,1.81208306781682,
-137.147133758372));
#152975=CARTESIAN_POINT('Ctrl Pts',(-39.7179607657458,0.808996392073229,
-136.328011452488));
#152976=CARTESIAN_POINT('Ctrl Pts',(-39.6844054587038,-0.224294744540098,
-135.552952869904));
#152977=CARTESIAN_POINT('Ctrl Pts',(-39.6367679612577,-1.84279784212966,
-134.475122839821));
#152978=CARTESIAN_POINT('Ctrl Pts',(-39.6212800791283,-2.39690688691799,
-134.128738792364));
#152979=CARTESIAN_POINT('Ctrl Pts',(-39.5994686586584,-3.23005227649636,
-133.645552385194));
#152980=CARTESIAN_POINT('Ctrl Pts',(-39.5924947647291,-3.50534889940371,
-133.491838360679));
#152981=CARTESIAN_POINT('Ctrl Pts',(-39.5857308656309,-3.78242429107441,
-133.34341275263));
#152982=CARTESIAN_POINT('Ctrl Pts',(-39.5652399075022,-4.65674474020595,
-132.895844604925));
#152983=CARTESIAN_POINT('Ctrl Pts',(-39.,-4.21888391538426,-131.902596984872));
#152984=CARTESIAN_POINT('Ctrl Pts',(-39.,-3.72521479271581,-130.782753296221));
#152985=CARTESIAN_POINT('Ctrl Pts',(-39.5781306671204,-4.08236536173137,
-133.176106520795));
#152986=CARTESIAN_POINT('Ctrl Pts',(-39.,-3.6159206095068,-132.184581657476));
#152987=CARTESIAN_POINT('Ctrl Pts',(-39.,-3.08946624372919,-131.063015115075));
#152988=CARTESIAN_POINT('Ctrl Pts',(-39.5919846958087,-3.51592220196165,
-133.479760839166));
#152989=CARTESIAN_POINT('Ctrl Pts',(-39.,-3.02226593965722,-132.489948109969));
#152990=CARTESIAN_POINT('Ctrl Pts',(-39.,-2.46339239509573,-131.366669530497));
#152991=CARTESIAN_POINT('Ctrl Pts',(-39.6212800791283,-2.39690688691799,
-134.128738792364));
#152992=CARTESIAN_POINT('Ctrl Pts',(-39.,-1.85088554063804,-133.142434340475));
#152993=CARTESIAN_POINT('Ctrl Pts',(-39.,-1.22847641296741,-132.015647483627));
#152994=CARTESIAN_POINT('Ctrl Pts',(-39.6367679612577,-1.84279784212966,
-134.475122839821));
#152995=CARTESIAN_POINT('Ctrl Pts',(-39.,-1.27148303561927,-133.490738119779));
#152996=CARTESIAN_POINT('Ctrl Pts',(-39.,-0.61794440595705,-132.362031531162));
#152997=CARTESIAN_POINT('Ctrl Pts',(-39.6847850431059,-0.21139821211329,
-135.561541219197));
#152998=CARTESIAN_POINT('Ctrl Pts',(-39.,0.433753695599259,-134.583900592971));
#152999=CARTESIAN_POINT('Ctrl Pts',(-39.,1.17663045280609,-133.448449910404));
#153000=CARTESIAN_POINT('Ctrl Pts',(-39.7187663759592,0.83378959624966,
-136.346621542847));
#153001=CARTESIAN_POINT('Ctrl Pts',(-39.,1.52263602949375,-135.373451527487));
#153002=CARTESIAN_POINT('Ctrl Pts',(-39.,2.32236925604725,-134.233515370373));
#153003=CARTESIAN_POINT('Ctrl Pts',(-39.7537665531305,1.84818159949203,
-137.176641147095));
#153004=CARTESIAN_POINT('Ctrl Pts',(-39.,2.57493359537216,-136.206226648817));
#153005=CARTESIAN_POINT('Ctrl Pts',(-39.,3.43069435955708,-135.063549838392));
#153006=CARTESIAN_POINT('Ctrl Pts',(-39.,-3.68000001999998,-130.802732351058));
#153007=CARTESIAN_POINT('Ctrl Pts',(-39.,-3.33509769381514,-130.955490419457));
#153008=CARTESIAN_POINT('Ctrl Pts',(-38.999999999995,-2.99379560771467,
-131.114791966817));
#153009=CARTESIAN_POINT('Ctrl Pts',(-39.0000000000322,-2.65562532357943,
-131.280281718424));
#153010=CARTESIAN_POINT('Ctrl Pts',(-39.0000000000621,-2.38378986674371,
-131.413309321204));
#153011=CARTESIAN_POINT('Ctrl Pts',(-39.0000000001226,-2.11397851849314,
-131.550336634986));
#153012=CARTESIAN_POINT('Ctrl Pts',(-39.0000000002374,-1.84595706992345,
-131.691201637143));
#153013=CARTESIAN_POINT('Ctrl Pts',(-39.0000000003908,-1.48773653906914,
-131.879472897226));
#153014=CARTESIAN_POINT('Ctrl Pts',(-39.0000000006483,-1.13214453284296,
-132.074954501691));
#153015=CARTESIAN_POINT('Ctrl Pts',(-39.0000000009742,-0.77990354390592,
-132.276609948051));
#153016=CARTESIAN_POINT('Ctrl Pts',(-39.0000000012103,-0.524689202150672,
-132.422718332994));
#153017=CARTESIAN_POINT('Ctrl Pts',(-39.000000001479,-0.271234086134615,
-132.572069210975));
#153018=CARTESIAN_POINT('Ctrl Pts',(-39.0000000017246,-0.0198207958907409,
-132.724283330851));
#153019=CARTESIAN_POINT('Ctrl Pts',(-39.0000000020985,0.362997438679579,
-132.956054453974));
#153020=CARTESIAN_POINT('Ctrl Pts',(-39.0000000024107,0.740951650742127,
-133.194233184148));
#153021=CARTESIAN_POINT('Ctrl Pts',(-39.0000000024159,1.11485984244746,
-133.438609986291));
#153022=CARTESIAN_POINT('Ctrl Pts',(-39.00000000242,1.40217712996276,-133.626393194792));
#153023=CARTESIAN_POINT('Ctrl Pts',(-39.0000000022332,1.68710447741373,
-133.817837252074));
#153024=CARTESIAN_POINT('Ctrl Pts',(-39.0000000018622,1.96999998000005,
-134.012863078852));
#153025=CARTESIAN_POINT('Origin',(-39.,46.91999998,-129.34995));
#153026=CARTESIAN_POINT('Origin',(83.2809572255632,2.96999998000007,-176.84995));
#153027=CARTESIAN_POINT('',(-60.,2.96999998000001,-177.34995));
#153028=CARTESIAN_POINT('Origin',(-57.,-2.42462934179819E-14,-174.34995));
#153029=CARTESIAN_POINT('',(-60.,28.41999998,-174.34995));
#153030=CARTESIAN_POINT('',(-57.,-54.58000002,-177.34995));
#153031=CARTESIAN_POINT('Origin',(-60.,-2.55003103885676E-14,0.));
#153032=CARTESIAN_POINT('Origin',(-60.,28.41999998,-177.34995));
#153033=CARTESIAN_POINT('Origin',(0.,-12.9675000200281,-171.64995));
#153034=CARTESIAN_POINT('Ctrl Pts',(-40.0642139728404,9.89540198157303,
-145.11953138824));
#153035=CARTESIAN_POINT('Ctrl Pts',(-40.0183499110469,8.78469917332298,
-143.853535251546));
#153036=CARTESIAN_POINT('Ctrl Pts',(-39.9717745968192,7.64117779462799,
-142.61251748975));
#153037=CARTESIAN_POINT('Ctrl Pts',(-39.925101121935,6.45601873886266,-141.410634166036));
#153038=CARTESIAN_POINT('Ctrl Pts',(-39.8971179105603,5.74545333844114,
-140.69004168436));
#153039=CARTESIAN_POINT('Ctrl Pts',(-39.8692646256818,5.02426042253766,
-139.987850959434));
#153040=CARTESIAN_POINT('Ctrl Pts',(-39.8417723415181,4.28998417285319,
-139.307926707528));
#153041=CARTESIAN_POINT('Ctrl Pts',(-39.,12.1842637898263,-143.052046612136));
#153042=CARTESIAN_POINT('Ctrl Pts',(-39.,10.9256789631914,-144.234640911918));
#153043=CARTESIAN_POINT('Ctrl Pts',(-40.0658654912634,9.93539056346401,
-145.16513792084));
#153044=CARTESIAN_POINT('Ctrl Pts',(-39.,10.979841755805,-141.770231455688));
#153045=CARTESIAN_POINT('Ctrl Pts',(-39.,9.77621097937933,-142.950028280238));
#153046=CARTESIAN_POINT('Ctrl Pts',(-40.0194681925347,8.81214966903568,
-143.883338323671));
#153047=CARTESIAN_POINT('Ctrl Pts',(-39.,9.73492905398707,-140.513855077087));
#153048=CARTESIAN_POINT('Ctrl Pts',(-38.9999999999938,8.58671680832509,
-141.687354928893));
#153049=CARTESIAN_POINT('Ctrl Pts',(-39.9723349230223,7.65540591189065,
-142.62694638584));
#153050=CARTESIAN_POINT('Ctrl Pts',(-39.,7.14197626750154,-138.081230637578));
#153051=CARTESIAN_POINT('Ctrl Pts',(-39.0000000000061,6.11210401876312,
-139.242594351665));
#153052=CARTESIAN_POINT('Ctrl Pts',(-39.8778673208479,5.25663156583475,
-140.194321946232));
#153053=CARTESIAN_POINT('Ctrl Pts',(-39.,5.8072721390059,-136.917329731646));
#153054=CARTESIAN_POINT('Ctrl Pts',(-39.,4.84002931498563,-138.072328953201));
#153055=CARTESIAN_POINT('Ctrl Pts',(-39.831007995706,4.02695578189988,-139.030438856635));
#153056=CARTESIAN_POINT('Ctrl Pts',(-39.,4.42069758591766,-135.824477851673));
#153057=CARTESIAN_POINT('Ctrl Pts',(-39.,3.51696512827391,-136.971103897255));
#153058=CARTESIAN_POINT('Ctrl Pts',(-39.7856126378568,2.75522939862341,
-137.937569160376));
#153059=CARTESIAN_POINT('Ctrl Pts',(-39.,4.46999998000001,-135.863383986541));
#153060=CARTESIAN_POINT('Ctrl Pts',(-39.0000000000005,4.88328157550107,
-136.189917146855));
#153061=CARTESIAN_POINT('Ctrl Pts',(-39.0000000000119,5.29116221661458,
-136.522117224196));
#153062=CARTESIAN_POINT('Ctrl Pts',(-39.0000000000389,5.69434025783345,
-136.859675625829));
#153063=CARTESIAN_POINT('Ctrl Pts',(-39.0000000000669,6.11191405992085,
-137.209286792078));
#153064=CARTESIAN_POINT('Ctrl Pts',(-39.0000000001116,6.52444323385465,
-137.564646050771));
#153065=CARTESIAN_POINT('Ctrl Pts',(-39.0000000001789,6.93266997764253,
-137.925456663921));
#153066=CARTESIAN_POINT('Ctrl Pts',(-39.0000000002504,7.36643947054107,
-138.308843198685));
#153067=CARTESIAN_POINT('Ctrl Pts',(-39.0000000003473,7.79535110451708,
-138.698384855332));
#153068=CARTESIAN_POINT('Ctrl Pts',(-39.0000000004772,8.22026082374413,
-139.093772869082));
#153069=CARTESIAN_POINT('Ctrl Pts',(-39.0000000004994,8.29309080497359,
-139.161542798356));
#153070=CARTESIAN_POINT('Ctrl Pts',(-39.0000000005226,8.36580314364496,
-139.229484583884));
#153071=CARTESIAN_POINT('Ctrl Pts',(-39.0000000005469,8.43840206333326,
-139.297596789496));
#153072=CARTESIAN_POINT('Ctrl Pts',(-39.0000000006997,8.8960899600184,-139.726998938435));
#153073=CARTESIAN_POINT('Ctrl Pts',(-39.0000000008925,9.34761173377698,
-140.161633014643));
#153074=CARTESIAN_POINT('Ctrl Pts',(-39.0000000011355,9.79388080738361,
-140.601330848477));
#153075=CARTESIAN_POINT('Ctrl Pts',(-39.0000000011949,9.90289654250056,
-140.708741344565));
#153076=CARTESIAN_POINT('Ctrl Pts',(-39.0000000012573,10.0115986221443,
-140.816454152322));
#153077=CARTESIAN_POINT('Ctrl Pts',(-39.0000000013228,10.11999998,-140.924467062102));
#153078=CARTESIAN_POINT('Origin',(-39.,46.91999998,-129.34995));
#153079=CARTESIAN_POINT('Origin',(-60.,28.41999998,-177.34995));
#153080=CARTESIAN_POINT('',(-57.,-54.58000002,-177.34995));
#153081=CARTESIAN_POINT('Origin',(-57.,-2.42462934179819E-14,-174.34995));
#153082=CARTESIAN_POINT('Ctrl Pts',(-38.9841065328395,-56.2141391785318,
-61.0006103127042));
#153083=CARTESIAN_POINT('Ctrl Pts',(-40.2048288919875,-54.58000002,-61.850776413383));
#153084=CARTESIAN_POINT('Ctrl Pts',(-42.0182169324382,-54.58000002,-63.1137016214078));
#153085=CARTESIAN_POINT('Ctrl Pts',(-36.4598290914011,-56.1197282395838,
-64.7755113243629));
#153086=CARTESIAN_POINT('Ctrl Pts',(-37.6731521867469,-54.5800000199842,
-65.6186857176609));
#153087=CARTESIAN_POINT('Ctrl Pts',(-39.3891852844759,-54.58000002,-66.8886318537073));
#153088=CARTESIAN_POINT('Ctrl Pts',(-33.8526449461492,-56.018427265929,
-68.5041285748648));
#153089=CARTESIAN_POINT('Ctrl Pts',(-35.039043742113,-54.58000002,-69.3609187351473));
#153090=CARTESIAN_POINT('Ctrl Pts',(-36.6602985783386,-54.58000002,-70.6173011253171));
#153091=CARTESIAN_POINT('Ctrl Pts',(-31.1389734555133,-55.9114071812081,
-72.1061129617773));
#153092=CARTESIAN_POINT('Ctrl Pts',(-32.2647524970408,-54.5800000199999,
-73.0003840144137));
#153093=CARTESIAN_POINT('Ctrl Pts',(-33.7990997127136,-54.58000002,-74.2192042704808));
#153094=CARTESIAN_POINT('Ctrl Pts',(-39.4999999999959,-54.58000002,-66.6681042685264));
#153095=CARTESIAN_POINT('Ctrl Pts',(-37.6706537603941,-54.58000002,-69.204359231621));
#153096=CARTESIAN_POINT('Ctrl Pts',(-35.7938421862428,-54.58000002,-71.7056198678132));
#153097=CARTESIAN_POINT('Ctrl Pts',(-33.8499999999899,-54.58000002,-74.1550953619836));
#153098=CARTESIAN_POINT('Ctrl Pts',(-33.5716649926242,-56.0068714410799,
-68.806691265109));
#153099=CARTESIAN_POINT('Ctrl Pts',(-35.3684223959548,-56.0769674434306,
-66.3189008836144));
#153100=CARTESIAN_POINT('Ctrl Pts',(-37.1195284786874,-56.1442949465457,
-63.7841134204858));
#153101=CARTESIAN_POINT('Ctrl Pts',(-38.8323589160537,-56.2084590974991,
-61.2273337386071));
#153102=CARTESIAN_POINT('Origin',(0.,-12.9675000200281,-60.64995));
#153103=CARTESIAN_POINT('Origin',(-41.5,-73.08000002,-177.34995));
#153104=CARTESIAN_POINT('',(41.5,-70.08000002,-177.34995));
#153105=CARTESIAN_POINT('Origin',(3.3975957231091E-14,-70.08000002,-174.34995));
#153106=CARTESIAN_POINT('',(-41.5,-73.08000002,-174.34995));
#153107=CARTESIAN_POINT('Origin',(3.54807775957937E-14,-73.08000002,3.11172719585489E-30));
#153108=CARTESIAN_POINT('Origin',(-60.,-54.58000002,-55.24995));
#153109=CARTESIAN_POINT('Ctrl Pts',(-33.85,-54.58000002,-157.903547609535));
#153110=CARTESIAN_POINT('Ctrl Pts',(-35.7938424480564,-54.58000002,-160.35302343361));
#153111=CARTESIAN_POINT('Ctrl Pts',(-37.6706534886586,-54.58000002,-162.854283363144));
#153112=CARTESIAN_POINT('Ctrl Pts',(-39.5,-54.58000002,-165.390538702986));
#153113=CARTESIAN_POINT('Ctrl Pts',(-42.1374590345468,-54.58000002,-169.116290576972));
#153114=CARTESIAN_POINT('Ctrl Pts',(-40.320307620846,-54.58000002,-170.379862235888));
#153115=CARTESIAN_POINT('Ctrl Pts',(-39.0986073542357,-56.2184192034566,
-171.229381885675));
#153116=CARTESIAN_POINT('Ctrl Pts',(-39.4714760509134,-54.58000002,-165.282321435755));
#153117=CARTESIAN_POINT('Ctrl Pts',(-37.7530684146655,-54.5800000201611,
-166.553337438667));
#153118=CARTESIAN_POINT('Ctrl Pts',(-36.5384467754252,-56.1227754271583,
-167.395443178417));
#153119=CARTESIAN_POINT('Ctrl Pts',(-36.7030946909167,-54.58000002,-161.495162061412));
#153120=CARTESIAN_POINT('Ctrl Pts',(-35.0808115183431,-54.5800000200163,
-162.752463904168));
#153121=CARTESIAN_POINT('Ctrl Pts',(-33.8932339485135,-56.0200282137318,
-163.608339894981));
#153122=CARTESIAN_POINT('Ctrl Pts',(-33.7983252138975,-54.58000002,-157.838463708057));
#153123=CARTESIAN_POINT('Ctrl Pts',(-32.2640061692936,-54.5800000199999,
-159.057279891091));
#153124=CARTESIAN_POINT('Ctrl Pts',(-31.1382389079697,-55.9113782125501,
-159.951555016761));
#153125=CARTESIAN_POINT('',(-38.9938267385724,-56.214502484065,-171.072567687954));
#153126=CARTESIAN_POINT('Origin',(-42.7058184423063,-60.0992226028014,-170.703547390513));
#153127=CARTESIAN_POINT('Ctrl Pts',(-38.9938273364047,-56.2145025937637,
-171.072567271539));
#153128=CARTESIAN_POINT('Ctrl Pts',(-37.2296100808616,-56.148520626844,
-168.433870605279));
#153129=CARTESIAN_POINT('Ctrl Pts',(-35.4249314550332,-56.0791684505653,
-165.817913090769));
#153130=CARTESIAN_POINT('Ctrl Pts',(-33.5716804653412,-56.0068706353672,
-163.251940550002));
#153131=CARTESIAN_POINT('Ctrl Pts',(-39.4023695343916,-56.667607408721,
-171.60507092612));
#153132=CARTESIAN_POINT('Ctrl Pts',(-39.1191457108045,-56.3534914900074,
-171.473900235605));
#153133=CARTESIAN_POINT('Ctrl Pts',(-38.9938259143948,-56.2145026772597,
-171.07256826174));
#153134=CARTESIAN_POINT('Ctrl Pts',(-39.4667323101199,-56.6069363160445,
-171.604463274963));
#153135=CARTESIAN_POINT('Ctrl Pts',(-39.1873296781659,-56.2851199488468,
-171.471360601804));
#153136=CARTESIAN_POINT('Ctrl Pts',(-39.0656324591812,-56.1451830708436,
-171.065281773562));
#153137=CARTESIAN_POINT('Ctrl Pts',(-39.532372953365,-56.5484198596326,
-171.603842231026));
#153138=CARTESIAN_POINT('Ctrl Pts',(-39.256852764825,-56.2190926208658,
-171.468759835437));
#153139=CARTESIAN_POINT('Ctrl Pts',(-39.1389029748433,-56.0783561940248,
-171.057850262871));
#153140=CARTESIAN_POINT('Ctrl Pts',(-39.59920642547,-56.4919352618991,-171.603208415545));
#153141=CARTESIAN_POINT('Ctrl Pts',(-39.3276146389594,-56.1552707341152,
-171.46610011903));
#153142=CARTESIAN_POINT('Ctrl Pts',(-39.2135563963028,-56.0138844098186,
-171.050282355671));
#153143=CARTESIAN_POINT('Origin',(-39.6007286333569,-56.8876021458077,-170.64995));
#153144=CARTESIAN_POINT('Origin',(0.,-12.9675000200281,-170.64995));
#153145=CARTESIAN_POINT('Origin',(0.,-12.9675000200281,-171.64995));
#153146=CARTESIAN_POINT('Origin',(0.,-12.9675000200281,-171.07256826174));
#153147=CARTESIAN_POINT('Origin',(0.,-12.9675000200281,-171.64995));
#153148=CARTESIAN_POINT('Ctrl Pts',(-42.5,-55.08000002,-60.64995));
#153149=CARTESIAN_POINT('Ctrl Pts',(-42.,-55.08000002,-60.64995));
#153150=CARTESIAN_POINT('Ctrl Pts',(-42.,-55.58000002,-60.64995));
#153151=CARTESIAN_POINT('Ctrl Pts',(-42.5,-54.58000002,-60.64995));
#153152=CARTESIAN_POINT('Ctrl Pts',(-41.5,-54.58000002,-60.64995));
#153153=CARTESIAN_POINT('Ctrl Pts',(-41.5,-55.58000002,-60.64995));
#153154=CARTESIAN_POINT('Ctrl Pts',(-42.5,-54.58000002,-61.14995));
#153155=CARTESIAN_POINT('Ctrl Pts',(-41.5,-54.58000002,-61.14995));
#153156=CARTESIAN_POINT('Ctrl Pts',(-41.5,-55.58000002,-61.14995));
#153157=CARTESIAN_POINT('Origin',(0.,-12.9675000200281,-171.64995));
#153158=CARTESIAN_POINT('Ctrl Pts',(-31.0842854211463,-55.9092502161047,
-159.87997642591));
#153159=CARTESIAN_POINT('Ctrl Pts',(-29.278906722612,-55.8380360188005,
-157.486006234072));
#153160=CARTESIAN_POINT('Ctrl Pts',(-27.4082502462316,-55.7634592463117,
-155.123448236681));
#153161=CARTESIAN_POINT('Ctrl Pts',(-25.4683317949416,-55.6876147613919,
-152.854279668282));
#153162=CARTESIAN_POINT('Ctrl Pts',(-33.7871193355851,-54.58000002,-157.824358608005));
#153163=CARTESIAN_POINT('Ctrl Pts',(-32.2532079260876,-54.58000002,-159.043115862826));
#153164=CARTESIAN_POINT('Ctrl Pts',(-31.1276111727346,-55.910959075446,
-159.937449916708));
#153165=CARTESIAN_POINT('Ctrl Pts',(-31.2221573047513,-54.58000002,-154.596132061548));
#153166=CARTESIAN_POINT('Ctrl Pts',(-29.7951706706339,-54.580000020057,
-155.819252869408));
#153167=CARTESIAN_POINT('Ctrl Pts',(-28.6950259327511,-55.8150212418279,
-156.709250494305));
#153168=CARTESIAN_POINT('Ctrl Pts',(-28.5157861483817,-54.58000002,-151.424072006624));
#153169=CARTESIAN_POINT('Ctrl Pts',(-27.1955413535409,-54.5800000200432,
-152.632731094419));
#153170=CARTESIAN_POINT('Ctrl Pts',(-26.143809437084,-55.7129653866513,
-153.537246733037));
#153171=CARTESIAN_POINT('Ctrl Pts',(-25.6489783375839,-54.58000002,-148.460215214005));
#153172=CARTESIAN_POINT('Ctrl Pts',(-24.4312618773724,-54.5800000199999,
-149.638058579956));
#153173=CARTESIAN_POINT('Ctrl Pts',(-23.4643533331708,-55.6098289013737,
-150.573306522708));
#153174=CARTESIAN_POINT('Ctrl Pts',(-25.7,-54.58000002,-148.513004346424));
#153175=CARTESIAN_POINT('Ctrl Pts',(-27.6634746333275,-54.58000002,-150.546045135875));
#153176=CARTESIAN_POINT('Ctrl Pts',(-29.537631721855,-54.58000002,-152.662307251431));
#153177=CARTESIAN_POINT('Ctrl Pts',(-31.35,-54.58000002,-154.831379798159));
#153178=CARTESIAN_POINT('Origin',(-60.,-54.58000002,-55.24995));
#153179=CARTESIAN_POINT('Ctrl Pts',(-31.3499999999855,-54.58000002,-77.227263173365));
#153180=CARTESIAN_POINT('Ctrl Pts',(-29.5376330958494,-54.58000002,-79.396334075655));
#153181=CARTESIAN_POINT('Ctrl Pts',(-27.6634733215002,-54.58000002,-81.5125991939361));
#153182=CARTESIAN_POINT('Ctrl Pts',(-25.7,-54.58000002,-83.5456386250818));
#153183=CARTESIAN_POINT('Ctrl Pts',(-31.127610916576,-55.9109590653435,
-72.1211933947368));
#153184=CARTESIAN_POINT('Ctrl Pts',(-32.2532076658177,-54.58000002,-73.0155274500394));
#153185=CARTESIAN_POINT('Ctrl Pts',(-33.787119065489,-54.58000002,-74.2342847034403));
#153186=CARTESIAN_POINT('Ctrl Pts',(-28.6950527991335,-55.8150223013088,
-75.3493568083322));
#153187=CARTESIAN_POINT('Ctrl Pts',(-29.7951976773991,-54.58000002,-76.2393546649833));
#153188=CARTESIAN_POINT('Ctrl Pts',(-31.2221856658751,-54.58000002,-77.4624751982426));
#153189=CARTESIAN_POINT('Ctrl Pts',(-26.1438256035288,-55.7129660087519,
-78.5213783677229));
#153190=CARTESIAN_POINT('Ctrl Pts',(-27.1955581318452,-54.5800000200432,
-79.425893713097));
#153191=CARTESIAN_POINT('Ctrl Pts',(-28.5158034471915,-54.58000002,-80.6345530934811));
#153192=CARTESIAN_POINT('Ctrl Pts',(-23.4643531971916,-55.6098288961396,
-81.485336599214));
#153193=CARTESIAN_POINT('Ctrl Pts',(-24.4312617378937,-54.58000002,-82.420584542654));
#153194=CARTESIAN_POINT('Ctrl Pts',(-25.6489781920928,-54.58000002,-83.5984279079175));
#153195=CARTESIAN_POINT('Origin',(0.,-12.9675000200281,-171.64995));
#153196=CARTESIAN_POINT('Origin',(-41.5,-73.08000002,-177.34995));
#153197=CARTESIAN_POINT('',(41.5,-70.08000002,-177.34995));
#153198=CARTESIAN_POINT('Origin',(3.3975957231091E-14,-70.08000002,-174.34995));
#153199=CARTESIAN_POINT('',(-41.5,-73.08000002,-174.34995));
#153200=CARTESIAN_POINT('Origin',(3.54807775957937E-14,-73.08000002,3.11172719585489E-30));
#153201=CARTESIAN_POINT('Origin',(0.,-12.9675000200281,-171.64995));
#153202=CARTESIAN_POINT('Origin',(0.,-12.9675000200281,-60.64995));
#153203=CARTESIAN_POINT('Origin',(0.,-12.9675000200281,-60.64995));
#153204=CARTESIAN_POINT('Ctrl Pts',(-40.5058072670198,20.4819096056616,
-73.2085628001111));
#153205=CARTESIAN_POINT('Ctrl Pts',(-40.5844085651433,22.403893278843,-70.4548680070988));
#153206=CARTESIAN_POINT('Ctrl Pts',(-40.6592141342549,24.2755389287606,
-67.6497302110104));
#153207=CARTESIAN_POINT('Ctrl Pts',(-40.7299249270772,26.1062893712319,
-64.8223085129012));
#153208=CARTESIAN_POINT('Origin',(-60.,28.41999998,-177.34995));
#153209=CARTESIAN_POINT('',(-57.,-54.58000002,-177.34995));
#153210=CARTESIAN_POINT('Origin',(-57.,-2.42462934179819E-14,-174.34995));
#153211=CARTESIAN_POINT('',(-60.,28.41999998,-174.34995));
#153212=CARTESIAN_POINT('Origin',(-60.,-2.55003103885676E-14,0.));
#153213=CARTESIAN_POINT('Ctrl Pts',(-40.7317364547463,26.153205244256,-64.7498326746213));
#153214=CARTESIAN_POINT('Ctrl Pts',(-39.,27.3939818002346,-65.5850914026758));
#153215=CARTESIAN_POINT('Ctrl Pts',(-39.,29.2922016634715,-66.8629239833248));
#153216=CARTESIAN_POINT('Ctrl Pts',(-40.6299764732755,23.5169744919048,
-68.8233420843703));
#153217=CARTESIAN_POINT('Ctrl Pts',(-39.,24.7554556194404,-69.6493391078479));
#153218=CARTESIAN_POINT('Ctrl Pts',(-39.,26.5499956507371,-70.9364700811645));
#153219=CARTESIAN_POINT('Ctrl Pts',(-40.5197426374407,20.7960159162511,
-72.851125470798));
#153220=CARTESIAN_POINT('Ctrl Pts',(-38.9999999999314,22.0110957235223,
-73.6915951012831));
#153221=CARTESIAN_POINT('Ctrl Pts',(-39.,23.7045900978902,-74.9643266004363));
#153222=CARTESIAN_POINT('Ctrl Pts',(-40.401808630759,17.9622434922255,-76.7460261035824));
#153223=CARTESIAN_POINT('Ctrl Pts',(-39.,19.1149982396193,-77.6303175298695));
#153224=CARTESIAN_POINT('Ctrl Pts',(-39.,20.7168512667374,-78.8591174122859));
#153225=CARTESIAN_POINT('Ctrl Pts',(-39.,26.4199999800115,-71.0516396909898));
#153226=CARTESIAN_POINT('Ctrl Pts',(-39.,24.5896727691867,-73.6696133337874));
#153227=CARTESIAN_POINT('Ctrl Pts',(-39.,22.7129807779577,-76.2544280814611));
#153228=CARTESIAN_POINT('Ctrl Pts',(-39.,20.769999979994,-78.7897987614735));
#153229=CARTESIAN_POINT('Origin',(-39.,46.91999998,-129.34995));
#153230=CARTESIAN_POINT('Ctrl Pts',(-39.,20.76999998,-153.26884421004));
#153231=CARTESIAN_POINT('Ctrl Pts',(-39.,22.7129810391408,-155.80421523086));
#153232=CARTESIAN_POINT('Ctrl Pts',(-39.,24.5896725049001,-158.389029259702));
#153233=CARTESIAN_POINT('Ctrl Pts',(-39.,26.4199999800001,-161.0070032805));
#153234=CARTESIAN_POINT('Ctrl Pts',(-39.,29.2922017208088,-165.195719073356));
#153235=CARTESIAN_POINT('Ctrl Pts',(-39.,27.3939818557438,-166.473551654334));
#153236=CARTESIAN_POINT('Ctrl Pts',(-40.731736456874,26.153205299378,-167.30881038206));
#153237=CARTESIAN_POINT('Ctrl Pts',(-39.,26.5499900188717,-161.122164521183));
#153238=CARTESIAN_POINT('Ctrl Pts',(-39.,24.7554502364948,-162.409295569185));
#153239=CARTESIAN_POINT('Ctrl Pts',(-40.6299762644379,23.5169690803201,
-163.235292522563));
#153240=CARTESIAN_POINT('Ctrl Pts',(-39.,23.7045860616975,-157.09431111324));
#153241=CARTESIAN_POINT('Ctrl Pts',(-39.,22.0110917831004,-158.367042514669));
#153242=CARTESIAN_POINT('Ctrl Pts',(-40.5197424781718,20.796012087217,-159.207512241208));
#153243=CARTESIAN_POINT('Ctrl Pts',(-39.,20.7168513145423,-153.199525621538));
#153244=CARTESIAN_POINT('Ctrl Pts',(-39.,19.1149982856394,-154.428325504224));
#153245=CARTESIAN_POINT('Ctrl Pts',(-40.4018086326459,17.9622435375657,
-155.312616930242));
#153246=CARTESIAN_POINT('Ctrl Pts',(-40.7299249270775,26.1062893712214,
-167.236334458579));
#153247=CARTESIAN_POINT('Ctrl Pts',(-40.6592140226013,24.2755360362191,
-164.408908292578));
#153248=CARTESIAN_POINT('Ctrl Pts',(-40.5844084705175,22.4038909152615,
-161.603771549441));
#153249=CARTESIAN_POINT('Ctrl Pts',(-40.5058072685341,20.48190961327,-158.850080166024));
#153250=CARTESIAN_POINT('Origin',(0.,-12.9675000200281,-171.64995));
#153251=CARTESIAN_POINT('Origin',(0.,-12.9675000200281,-171.07256826174));
#153252=CARTESIAN_POINT('Origin',(0.,-12.9675000200281,-170.64995));
#153253=CARTESIAN_POINT('Origin',(0.,-12.9675000200281,-171.64995));
#153254=CARTESIAN_POINT('Origin',(0.,-12.9675000200281,-171.64995));
#153255=CARTESIAN_POINT('Origin',(0.,-12.9675000200281,-170.64995));
#153256=CARTESIAN_POINT('Origin',(0.,-12.9675000200281,-171.64995));
#153257=CARTESIAN_POINT('Origin',(0.,-12.9675000200281,-171.07256826174));
#153258=CARTESIAN_POINT('Origin',(0.,-12.9675000200281,-171.64995));
#153259=CARTESIAN_POINT('Ctrl Pts',(-40.4031453084766,17.9943647936175,
-155.356778662625));
#153260=CARTESIAN_POINT('Ctrl Pts',(-40.352516489763,16.7776395477168,-153.683470409173));
#153261=CARTESIAN_POINT('Ctrl Pts',(-40.3002588807393,15.5341707784358,
-152.02728304762));
#153262=CARTESIAN_POINT('Ctrl Pts',(-40.2466286890062,14.2587895844586,
-150.39951644339));
#153263=CARTESIAN_POINT('Ctrl Pts',(-40.2205532005948,13.6386876144874,
-149.608081472651));
#153264=CARTESIAN_POINT('Ctrl Pts',(-40.194198830347,13.0122318389436,-148.824806848577));
#153265=CARTESIAN_POINT('Ctrl Pts',(-40.1676234671339,12.3782653572084,
-148.051087554039));
#153266=CARTESIAN_POINT('Ctrl Pts',(-39.,20.7969022442792,-153.303957440565));
#153267=CARTESIAN_POINT('Ctrl Pts',(-39.,19.1920625442621,-154.533208999946));
#153268=CARTESIAN_POINT('Ctrl Pts',(-40.4049679555898,18.0381725147214,
-155.417048749269));
#153269=CARTESIAN_POINT('Ctrl Pts',(-39.,19.4994946787828,-151.61013720275));
#153270=CARTESIAN_POINT('Ctrl Pts',(-38.9999999999926,17.9467387756658,
-152.837123072001));
#153271=CARTESIAN_POINT('Ctrl Pts',(-40.3537709661131,16.8074898953919,
-153.723238579969));
#153272=CARTESIAN_POINT('Ctrl Pts',(-39.,18.1688145972663,-149.933732593));
#153273=CARTESIAN_POINT('Ctrl Pts',(-39.,16.6677293129161,-151.153378312361));
#153274=CARTESIAN_POINT('Ctrl Pts',(-40.3009026952457,15.549481350471,-152.046823901733));
#153275=CARTESIAN_POINT('Ctrl Pts',(-39.,15.4269724929124,-146.639117676373));
#153276=CARTESIAN_POINT('Ctrl Pts',(-39.,14.0355026731613,-147.843763736059));
#153277=CARTESIAN_POINT('Ctrl Pts',(-40.1923546827668,12.9680978184463,
-148.752208985047));
#153278=CARTESIAN_POINT('Ctrl Pts',(-39.,14.0212803181596,-145.027145257042));
#153279=CARTESIAN_POINT('Ctrl Pts',(-39.0000000000223,12.6882757758116,
-146.224143705887));
#153280=CARTESIAN_POINT('Ctrl Pts',(-40.1368768832445,11.6498727042044,
-147.140254909589));
#153281=CARTESIAN_POINT('Ctrl Pts',(-39.,12.5683345334111,-143.463140153395));
#153282=CARTESIAN_POINT('Ctrl Pts',(-39.,11.293230102484,-144.64769997634));
#153283=CARTESIAN_POINT('Ctrl Pts',(-40.0806897728025,10.2937241351084,
-145.576231462098));
#153284=CARTESIAN_POINT('Ctrl Pts',(-39.,12.61999998,-143.518796834034));
#153285=CARTESIAN_POINT('Ctrl Pts',(-39.0000000000004,13.1830701012425,
-144.125823176785));
#153286=CARTESIAN_POINT('Ctrl Pts',(-39.000000000008,13.7383356437293,-144.739255401572));
#153287=CARTESIAN_POINT('Ctrl Pts',(-39.0000000000126,14.2868563031727,
-145.358644195211));
#153288=CARTESIAN_POINT('Ctrl Pts',(-39.0000000000176,14.874877526446,-146.022636972598));
#153289=CARTESIAN_POINT('Ctrl Pts',(-39.0000000000202,15.4551472634138,
-146.693475297455));
#153290=CARTESIAN_POINT('Ctrl Pts',(-39.0000000000369,16.0289279109256,
-147.370648869846));
#153291=CARTESIAN_POINT('Ctrl Pts',(-39.0000000000444,16.2865138368672,
-147.674650725649));
#153292=CARTESIAN_POINT('Ctrl Pts',(-39.000000000055,16.5427914446669,-147.979929896415));
#153293=CARTESIAN_POINT('Ctrl Pts',(-39.0000000000741,16.7978726164159,
-148.286442551932));
#153294=CARTESIAN_POINT('Ctrl Pts',(-39.0000000001113,17.2936331206748,
-148.88216221097));
#153295=CARTESIAN_POINT('Ctrl Pts',(-39.0000000001696,17.7841600789861,
-149.481724824065));
#153296=CARTESIAN_POINT('Ctrl Pts',(-39.0000000003777,18.2699999799999,
-150.084863924608));
#153297=CARTESIAN_POINT('Origin',(-39.,46.91999998,-129.34995));
#153298=CARTESIAN_POINT('Ctrl Pts',(-39.000000000374,18.2699999799838,-81.9737790469184));
#153299=CARTESIAN_POINT('Ctrl Pts',(-39.0000000001679,17.7841524775854,
-82.5769275834792));
#153300=CARTESIAN_POINT('Ctrl Pts',(-39.0000000001103,17.2936169434169,
-83.1765007297742));
#153301=CARTESIAN_POINT('Ctrl Pts',(-39.0000000000735,16.7978518736795,
-83.7722255217958));
#153302=CARTESIAN_POINT('Ctrl Pts',(-39.0000000000309,16.2234293967169,
-84.462467193728));
#153303=CARTESIAN_POINT('Ctrl Pts',(-39.0000000000258,15.6429390502857,
-85.1464596076279));
#153304=CARTESIAN_POINT('Ctrl Pts',(-39.0000000000195,15.0550950356354,
-85.8236901162035));
#153305=CARTESIAN_POINT('Ctrl Pts',(-39.0000000000137,14.5092314506924,
-86.4525567271254));
#153306=CARTESIAN_POINT('Ctrl Pts',(-39.0000000000098,13.957027196594,-87.0755929306387));
#153307=CARTESIAN_POINT('Ctrl Pts',(-39.0000000000048,13.3974208289947,
-87.6923562596142));
#153308=CARTESIAN_POINT('Ctrl Pts',(-39.0000000000025,13.1398841264358,
-87.9761971935281));
#153309=CARTESIAN_POINT('Ctrl Pts',(-39.0000000000002,12.8807792236243,
-88.2587090915689));
#153310=CARTESIAN_POINT('Ctrl Pts',(-39.,12.61999998,-88.5398461374725));
#153311=CARTESIAN_POINT('Ctrl Pts',(-40.4049679656207,18.0381727558475,
-76.6415938903714));
#153312=CARTESIAN_POINT('Ctrl Pts',(-39.,19.1920627889827,-77.5254336382597));
#153313=CARTESIAN_POINT('Ctrl Pts',(-39.,20.796902498477,-78.7546851990749));
#153314=CARTESIAN_POINT('Ctrl Pts',(-40.3537711092786,16.8074933352464,
-78.3353996644624));
#153315=CARTESIAN_POINT('Ctrl Pts',(-39.0000000000074,17.9467422700577,
-79.2215151478833));
#153316=CARTESIAN_POINT('Ctrl Pts',(-39.,19.4994983593746,-80.4485009715931));
#153317=CARTESIAN_POINT('Ctrl Pts',(-40.3009014559381,15.5494518783308,
-80.0118574083956));
#153318=CARTESIAN_POINT('Ctrl Pts',(-39.,16.6676992320686,-80.9053032515377));
#153319=CARTESIAN_POINT('Ctrl Pts',(-39.,18.1687833493074,-82.1249487171281));
#153320=CARTESIAN_POINT('Ctrl Pts',(-40.1923542727721,12.9680880684791,
-83.3064457069268));
#153321=CARTESIAN_POINT('Ctrl Pts',(-39.,14.0354926345166,-84.2148910918098));
#153322=CARTESIAN_POINT('Ctrl Pts',(-39.,15.4269620807205,-85.4195370156013));
#153323=CARTESIAN_POINT('Ctrl Pts',(-40.136876773061,11.6498700440212,-84.9183911253513));
#153324=CARTESIAN_POINT('Ctrl Pts',(-39.,12.6882730287539,-85.8345023651596));
#153325=CARTESIAN_POINT('Ctrl Pts',(-39.,14.0212774653657,-87.0315007804442));
#153326=CARTESIAN_POINT('Ctrl Pts',(-40.0806897769273,10.2937242346666,
-86.4824113945889));
#153327=CARTESIAN_POINT('Ctrl Pts',(-39.,11.2932302045755,-87.4109428798));
#153328=CARTESIAN_POINT('Ctrl Pts',(-39.,12.5683346400766,-88.5955027032924));
#153329=CARTESIAN_POINT('Origin',(0.,-12.9675000200281,-171.64995));
#153330=CARTESIAN_POINT('Origin',(-60.,28.41999998,-177.34995));
#153331=CARTESIAN_POINT('',(-57.,-54.58000002,-177.34995));
#153332=CARTESIAN_POINT('Origin',(-57.,-2.42462934179819E-14,-174.34995));
#153333=CARTESIAN_POINT('',(-60.,28.41999998,-174.34995));
#153334=CARTESIAN_POINT('Origin',(-60.,-2.55003103885676E-14,0.));
#153335=CARTESIAN_POINT('Ctrl Pts',(-39.,-46.9678746292626,-78.4459379002929));
#153336=CARTESIAN_POINT('Ctrl Pts',(-39.,-45.3542557512738,-77.2153536750926));
#153337=CARTESIAN_POINT('Ctrl Pts',(-40.4142759779013,-44.1970573566106,
-76.3328465915894));
#153338=CARTESIAN_POINT('Ctrl Pts',(-39.,-45.6681795295713,-80.1501792727118));
#153339=CARTESIAN_POINT('Ctrl Pts',(-38.9999999999777,-44.1065399853887,
-78.9218422882493));
#153340=CARTESIAN_POINT('Ctrl Pts',(-40.3630303964688,-42.9636869888089,
-78.0370779308685));
#153341=CARTESIAN_POINT('Ctrl Pts',(-39.,-44.3354733849924,-81.8371103170565));
#153342=CARTESIAN_POINT('Ctrl Pts',(-39.0000000000075,-42.8253754175223,
-80.6161315734671));
#153343=CARTESIAN_POINT('Ctrl Pts',(-40.3100980841279,-41.7032148714377,
-79.7240190083239));
#153344=CARTESIAN_POINT('Ctrl Pts',(-39.,-41.5900648068412,-85.1534256657242));
#153345=CARTESIAN_POINT('Ctrl Pts',(-38.9999999999925,-40.1892936959721,
-83.9475037984034));
#153346=CARTESIAN_POINT('Ctrl Pts',(-40.2013644254228,-39.117307479239,
-83.0403343570498));
#153347=CARTESIAN_POINT('Ctrl Pts',(-39.,-40.1827113458493,-86.7766805524391));
#153348=CARTESIAN_POINT('Ctrl Pts',(-39.0000000000224,-38.8402604870948,
-85.5784283533127));
#153349=CARTESIAN_POINT('Ctrl Pts',(-40.1457604305377,-37.7969103286269,
-84.6635709993291));
#153350=CARTESIAN_POINT('Ctrl Pts',(-39.,-38.7282817023213,-88.3525652913338));
#153351=CARTESIAN_POINT('Ctrl Pts',(-38.9999999999999,-37.4435485041586,
-87.1668478324999));
#153352=CARTESIAN_POINT('Ctrl Pts',(-40.0893978453286,-36.4387324215761,
-86.2394739826303));
#153353=CARTESIAN_POINT('Ctrl Pts',(-39.,-38.7800000199999,-88.296486260558));
#153354=CARTESIAN_POINT('Ctrl Pts',(-39.0000000000004,-39.3488675990385,
-87.6791933887653));
#153355=CARTESIAN_POINT('Ctrl Pts',(-39.0000000000079,-39.9098343204478,
-87.055447933957));
#153356=CARTESIAN_POINT('Ctrl Pts',(-39.0000000000125,-40.4639767641388,
-86.4257067262301));
#153357=CARTESIAN_POINT('Ctrl Pts',(-39.0000000000174,-41.0582242765977,
-85.75038912433));
#153358=CARTESIAN_POINT('Ctrl Pts',(-39.0000000000199,-41.6446237826485,
-85.0681763071405));
#153359=CARTESIAN_POINT('Ctrl Pts',(-39.0000000000371,-42.2244596706239,
-84.3795886418692));
#153360=CARTESIAN_POINT('Ctrl Pts',(-39.0000000000445,-42.4717173644235,
-84.0859562510071));
#153361=CARTESIAN_POINT('Ctrl Pts',(-39.0000000000547,-42.7177810382264,
-83.7911641691168));
#153362=CARTESIAN_POINT('Ctrl Pts',(-39.0000000000728,-42.9627483114232,
-83.4952507849665));
#153363=CARTESIAN_POINT('Ctrl Pts',(-39.0000000001092,-43.4568057616665,
-82.8984436680065));
#153364=CARTESIAN_POINT('Ctrl Pts',(-39.0000000001663,-43.9457116736056,
-82.2978701296067));
#153365=CARTESIAN_POINT('Ctrl Pts',(-39.0000000003688,-44.43000002,-81.6937887068282));
#153366=CARTESIAN_POINT('Origin',(-39.,46.91999998,-129.34995));
#153367=CARTESIAN_POINT('Ctrl Pts',(-39.0000000003644,-44.4300000199906,
-150.364854264666));
#153368=CARTESIAN_POINT('Ctrl Pts',(-39.0000000001644,-43.9457023551939,
-149.760761216984));
#153369=CARTESIAN_POINT('Ctrl Pts',(-39.000000000108,-43.4567859620687,
-149.160174741698));
#153370=CARTESIAN_POINT('Ctrl Pts',(-39.0000000000721,-42.9627229131801,
-148.563361289672));
#153371=CARTESIAN_POINT('Ctrl Pts',(-39.0000000000298,-42.3819947837029,
-147.861859000802));
#153372=CARTESIAN_POINT('Ctrl Pts',(-39.000000000025,-41.795103731089,-147.166651435239));
#153373=CARTESIAN_POINT('Ctrl Pts',(-39.0000000000189,-41.2007410723699,
-146.478263131247));
#153374=CARTESIAN_POINT('Ctrl Pts',(-39.0000000000133,-40.6489795609292,
-145.839215294884));
#153375=CARTESIAN_POINT('Ctrl Pts',(-39.0000000000093,-40.0907793123423,
-145.206044014044));
#153376=CARTESIAN_POINT('Ctrl Pts',(-39.0000000000044,-39.5250612454855,
-144.579200831309));
#153377=CARTESIAN_POINT('Ctrl Pts',(-39.0000000000023,-39.2781704674615,
-144.305633819486));
#153378=CARTESIAN_POINT('Ctrl Pts',(-39.0000000000002,-39.0298473782501,
-144.033272518857));
#153379=CARTESIAN_POINT('Ctrl Pts',(-39.,-38.7800000199999,-143.762156710948));
#153380=CARTESIAN_POINT('Ctrl Pts',(-40.4142759901646,-44.1970576517619,
-155.725796787747));
#153381=CARTESIAN_POINT('Ctrl Pts',(-38.9999999999999,-45.3542560507482,
-154.843289706001));
#153382=CARTESIAN_POINT('Ctrl Pts',(-39.,-46.9678749402838,-153.612705479043));
#153383=CARTESIAN_POINT('Ctrl Pts',(-40.3630305742695,-42.9636912658246,
-154.021570941673));
#153384=CARTESIAN_POINT('Ctrl Pts',(-39.,-44.1065443282322,-153.136806613681));
#153385=CARTESIAN_POINT('Ctrl Pts',(-39.,-45.668184102287,-151.908469685114));
#153386=CARTESIAN_POINT('Ctrl Pts',(-40.3100965640753,-41.7031787097929,
-152.33457670764));
#153387=CARTESIAN_POINT('Ctrl Pts',(-39.0000000000074,-42.8253385188873,
-151.442463829735));
#153388=CARTESIAN_POINT('Ctrl Pts',(-39.,-44.3354350613925,-150.221485398912));
#153389=CARTESIAN_POINT('Ctrl Pts',(-40.2013639252015,-39.117295594665,
-149.018294252799));
#153390=CARTESIAN_POINT('Ctrl Pts',(-38.9999999999925,-40.1892814621382,
-148.11112464401));
#153391=CARTESIAN_POINT('Ctrl Pts',(-39.,-41.5900521206853,-146.90520294412));
#153392=CARTESIAN_POINT('Ctrl Pts',(-40.1457602981154,-37.7969071359042,
-147.395068273086));
#153393=CARTESIAN_POINT('Ctrl Pts',(-39.,-38.8402571910301,-146.480210875403));
#153394=CARTESIAN_POINT('Ctrl Pts',(-39.,-40.1827079235241,-145.281958716849));
#153395=CARTESIAN_POINT('Ctrl Pts',(-40.0893978502897,-36.4387325411231,
-145.819169127587));
#153396=CARTESIAN_POINT('Ctrl Pts',(-38.9999999999999,-37.4435486267092,
-144.891795278378));
#153397=CARTESIAN_POINT('Ctrl Pts',(-39.,-38.728281830342,-143.706077818883));
#153398=CARTESIAN_POINT('Ctrl Pts',(-40.1769969654089,-38.5367854528866,
-148.32464784256));
#153399=CARTESIAN_POINT('Ctrl Pts',(-40.2034881200521,-39.168290402203,
-149.099701330404));
#153400=CARTESIAN_POINT('Ctrl Pts',(-40.2297509497426,-39.7923967253814,
-149.884082045736));
#153401=CARTESIAN_POINT('Ctrl Pts',(-40.2557302446384,-40.410237152229,
-150.67643548022));
#153402=CARTESIAN_POINT('Ctrl Pts',(-40.3094516567182,-41.6878415022836,
-152.314907407094));
#153403=CARTESIAN_POINT('Ctrl Pts',(-40.3617745388197,-42.9337816491534,
-153.981551875682));
#153404=CARTESIAN_POINT('Ctrl Pts',(-40.4124516185963,-44.1531546492747,
-155.665156176616));
#153405=CARTESIAN_POINT('Origin',(0.,-12.9675000200281,-171.64995));
#153406=CARTESIAN_POINT('Origin',(0.,-12.9675000200281,-171.07256826174));
#153407=CARTESIAN_POINT('Origin',(0.,-12.9675000200281,-170.64995));
#153408=CARTESIAN_POINT('Origin',(0.,-12.9675000200281,-171.64995));
#153409=CARTESIAN_POINT('Origin',(-60.,28.41999998,-177.34995));
#153410=CARTESIAN_POINT('',(-57.,-54.58000002,-177.34995));
#153411=CARTESIAN_POINT('Origin',(-57.,-2.42462934179819E-14,-174.34995));
#153412=CARTESIAN_POINT('',(-60.,28.41999998,-174.34995));
#153413=CARTESIAN_POINT('Origin',(-60.,-2.55003103885676E-14,0.));
#153414=CARTESIAN_POINT('Origin',(0.,-12.9675000200281,-171.64995));
#153415=CARTESIAN_POINT('Origin',(0.,-12.9675000200281,-171.64995));
#153416=CARTESIAN_POINT('Origin',(0.,-12.9675000200281,-170.64995));
#153417=CARTESIAN_POINT('Origin',(0.,-12.9675000200281,-171.07256826174));
#153418=CARTESIAN_POINT('Origin',(0.,-12.9675000200281,-171.64995));
#153419=CARTESIAN_POINT('Ctrl Pts',(-40.5149617844426,-46.6408003024225,
-159.171515337561));
#153420=CARTESIAN_POINT('Ctrl Pts',(-40.5934042533475,-48.5623552413193,
-161.934081688328));
#153421=CARTESIAN_POINT('Ctrl Pts',(-40.668031895784,-50.4341179794481,
-164.747447196893));
#153422=CARTESIAN_POINT('Ctrl Pts',(-40.7385684573717,-52.2653908962638,
-167.582872566557));
#153423=CARTESIAN_POINT('Ctrl Pts',(-40.7403779325784,-52.3123829231466,
-167.655650590757));
#153424=CARTESIAN_POINT('Ctrl Pts',(-39.,-53.5547145065899,-166.821728771562));
#153425=CARTESIAN_POINT('Ctrl Pts',(-39.,-55.460351966619,-165.542559282053));
#153426=CARTESIAN_POINT('Ctrl Pts',(-40.6387326052879,-49.6718481371244,
-163.565128292503));
#153427=CARTESIAN_POINT('Ctrl Pts',(-38.9999999999999,-50.9123394210222,
-162.740555198018));
#153428=CARTESIAN_POINT('Ctrl Pts',(-39.,-52.7145421899793,-161.452000516006));
#153429=CARTESIAN_POINT('Ctrl Pts',(-40.5285982996977,-46.9471996283483,
-159.51999555488));
#153430=CARTESIAN_POINT('Ctrl Pts',(-38.9999999999311,-48.1648205365349,
-158.680980229719));
#153431=CARTESIAN_POINT('Ctrl Pts',(-39.,-49.8662825279046,-157.406795875704));
#153432=CARTESIAN_POINT('Ctrl Pts',(-40.4106852206046,-44.110656513925,
-155.606501037481));
#153433=CARTESIAN_POINT('Ctrl Pts',(-39.,-45.2665850600662,-154.723479509065));
#153434=CARTESIAN_POINT('Ctrl Pts',(-39.,-46.8768207417856,-153.493409728778));
#153435=CARTESIAN_POINT('Ctrl Pts',(-39.,-52.5800000199845,-161.329336741015));
#153436=CARTESIAN_POINT('Ctrl Pts',(-39.,-50.7492254978239,-158.702450591995));
#153437=CARTESIAN_POINT('Ctrl Pts',(-39.,-48.8724582313882,-156.108353723945));
#153438=CARTESIAN_POINT('Ctrl Pts',(-39.,-46.9300000199928,-153.563058845201));
#153439=CARTESIAN_POINT('Origin',(-39.,46.91999998,-129.34995));
#153440=CARTESIAN_POINT('Ctrl Pts',(-39.,-46.93000002,-78.4955841262963));
#153441=CARTESIAN_POINT('Ctrl Pts',(-39.,-48.8725599414451,-75.9501559720627));
#153442=CARTESIAN_POINT('Ctrl Pts',(-39.,-50.7491289418203,-73.3563309228582));
#153443=CARTESIAN_POINT('Ctrl Pts',(-39.,-52.58000002,-70.7293062304687));
#153444=CARTESIAN_POINT('Ctrl Pts',(-39.,-55.4603726203092,-66.5160529206996));
#153445=CARTESIAN_POINT('Ctrl Pts',(-39.,-53.5547345046268,-65.2368833127815));
#153446=CARTESIAN_POINT('Ctrl Pts',(-40.7403786971506,-52.3124027851469,
-64.4029616119961));
#153447=CARTESIAN_POINT('Ctrl Pts',(-39.,-52.7124559353729,-70.609751474253));
#153448=CARTESIAN_POINT('Ctrl Pts',(-38.9999999999999,-50.9103452005084,
-69.3211688367401));
#153449=CARTESIAN_POINT('Ctrl Pts',(-40.6386554420727,-49.6698429482511,
-68.4966218848756));
#153450=CARTESIAN_POINT('Ctrl Pts',(-39.,-49.8653057974222,-74.6531246748237));
#153451=CARTESIAN_POINT('Ctrl Pts',(-39.,-48.1638674451749,-73.378963184763));
#153452=CARTESIAN_POINT('Ctrl Pts',(-40.5285598162873,-46.9462740729553,
-72.5399234557376));
#153453=CARTESIAN_POINT('Ctrl Pts',(-39.,-46.8768348378863,-78.5652147900786));
#153454=CARTESIAN_POINT('Ctrl Pts',(-39.,-45.266598631985,-77.3351449301694));
#153455=CARTESIAN_POINT('Ctrl Pts',(-40.4106857765804,-44.1106698886037,
-76.4521234813751));
#153456=CARTESIAN_POINT('Ctrl Pts',(-40.7385684580933,-52.265390901695,
-64.4757704085913));
#153457=CARTESIAN_POINT('Ctrl Pts',(-40.6679883556503,-50.4329865209081,
-67.3129485767829));
#153458=CARTESIAN_POINT('Ctrl Pts',(-40.5933737163056,-48.561586044698,
-70.1257010194362));
#153459=CARTESIAN_POINT('Ctrl Pts',(-40.5149627320849,-46.6408090593808,
-72.8871337536569));
#153460=CARTESIAN_POINT('Origin',(0.,-12.9675000200281,-60.64995));
#153461=CARTESIAN_POINT('Origin',(-60.,28.41999998,-177.34995));
#153462=CARTESIAN_POINT('',(-57.,-54.58000002,-177.34995));
#153463=CARTESIAN_POINT('Origin',(-57.,-2.42462934179819E-14,-174.34995));
#153464=CARTESIAN_POINT('',(-60.,28.41999998,-174.34995));
#153465=CARTESIAN_POINT('Origin',(-60.,-2.55003103885676E-14,0.));
#153466=CARTESIAN_POINT('Origin',(0.,-12.9675000200281,-171.64995));
#153467=CARTESIAN_POINT('Origin',(0.,-12.9675000200281,-171.64995));
#153468=CARTESIAN_POINT('',(50.9867892914962,-42.9264785869994,-171.64995));
#153469=CARTESIAN_POINT('',(50.0729884546894,-44.43000002,-171.64995));
#153470=CARTESIAN_POINT('Origin',(0.,-12.9675000200281,-171.64995));
#153471=CARTESIAN_POINT('',(50.7754831343094,-44.43000002,-171.64995));
#153472=CARTESIAN_POINT('',(50.7052127169582,-44.43000002,-171.64995));
#153473=CARTESIAN_POINT('',(51.3476245933058,-40.3590020057362,-171.64995));
#153474=CARTESIAN_POINT('Origin',(60.,-2.55003103885676E-14,0.));
#153475=CARTESIAN_POINT('',(60.,-45.43000002,-58.24995));
#153476=CARTESIAN_POINT('',(60.,-45.93000002,-58.24995));
#153477=CARTESIAN_POINT('',(60.,-54.58000002,-58.24995));
#153478=CARTESIAN_POINT('',(60.,-45.93000002,-174.34995));
#153479=CARTESIAN_POINT('',(60.,-45.93000002,-174.34995));
#153480=CARTESIAN_POINT('',(60.,-45.43000002,-174.34995));
#153481=CARTESIAN_POINT('',(60.,28.41999998,-174.34995));
#153482=CARTESIAN_POINT('',(60.,-45.43000002,-58.24995));
#153483=CARTESIAN_POINT('Origin',(57.,-2.42462934179819E-14,-174.34995));
#153484=CARTESIAN_POINT('',(57.,-45.93000002,-177.34995));
#153485=CARTESIAN_POINT('Origin',(57.,-45.93000002,-174.34995));
#153486=CARTESIAN_POINT('',(57.,-45.43000002,-177.34995));
#153487=CARTESIAN_POINT('',(57.,-54.58000002,-177.34995));
#153488=CARTESIAN_POINT('Origin',(57.,-45.43000002,-174.34995));
#153489=CARTESIAN_POINT('Origin',(60.,28.41999998,-177.34995));
#153490=CARTESIAN_POINT('',(52.0794132410337,-45.93000002,-177.34995));
#153491=CARTESIAN_POINT('',(60.,-45.93000002,-177.34995));
#153492=CARTESIAN_POINT('',(52.1496836583849,-45.43000002,-177.34995));
#153493=CARTESIAN_POINT('',(62.4796469926385,28.0715083218873,-177.34995));
#153494=CARTESIAN_POINT('',(60.,-45.43000002,-177.34995));
#153495=CARTESIAN_POINT('Origin',(0.,-12.9675000200281,-60.64995));
#153496=CARTESIAN_POINT('',(40.7385684290383,-52.2653907132467,-64.4757702425922));
#153497=CARTESIAN_POINT('',(40.5149254648566,-46.6404784163578,-72.8869718390768));
#153498=CARTESIAN_POINT('Ctrl Pts',(40.7385684580933,-52.265390901695,-64.4757704085913));
#153499=CARTESIAN_POINT('Ctrl Pts',(40.7211666822863,-51.8136050708653,
-65.175286797751));
#153500=CARTESIAN_POINT('Ctrl Pts',(40.7037330721709,-51.3649633742573,
-65.8647723839272));
#153501=CARTESIAN_POINT('Ctrl Pts',(40.6862834285501,-50.9193769960497,
-66.5441356808015));
#153502=CARTESIAN_POINT('Ctrl Pts',(40.6682155292875,-50.4580031153458,
-67.2475693942546));
#153503=CARTESIAN_POINT('Ctrl Pts',(40.6501304434355,-49.9999049480625,
-67.940150902046));
#153504=CARTESIAN_POINT('Ctrl Pts',(40.6320442475958,-49.5449972740905,
-68.6218329826322));
#153505=CARTESIAN_POINT('Ctrl Pts',(40.6135558867345,-49.0799742637535,
-69.3186729599381));
#153506=CARTESIAN_POINT('Ctrl Pts',(40.5950663659317,-48.618285303638,-70.0041236119615));
#153507=CARTESIAN_POINT('Ctrl Pts',(40.5765913348633,-48.1598519228023,
-70.6781879312868));
#153508=CARTESIAN_POINT('Ctrl Pts',(40.5575179493113,-47.6865711694347,
-71.3740833049765));
#153509=CARTESIAN_POINT('Ctrl Pts',(40.5384600096633,-47.2167603716574,
-72.057843011644));
#153510=CARTESIAN_POINT('Ctrl Pts',(40.5194331080602,-46.7503450984622,
-72.729523983642));
#153511=CARTESIAN_POINT('Ctrl Pts',(40.5179427908006,-46.7138122595236,
-72.7821346380918));
#153512=CARTESIAN_POINT('Ctrl Pts',(40.5164526631504,-46.6773002579314,
-72.8346712140457));
#153513=CARTESIAN_POINT('Ctrl Pts',(40.5149627321913,-46.6408090606421,
-72.887133751753));
#153514=CARTESIAN_POINT('',(47.3503956976423,-46.6672397853475,-61.2273317382593));
#153515=CARTESIAN_POINT('Ctrl Pts',(40.5149864073608,-46.6403532458042,
-72.8868173744763));
#153516=CARTESIAN_POINT('Ctrl Pts',(41.0609560613025,-46.6426501090734,
-71.9832291349818));
#153517=CARTESIAN_POINT('Ctrl Pts',(41.6128385796135,-46.644935702693,-71.0626686770773));
#153518=CARTESIAN_POINT('Ctrl Pts',(42.170607592867,-46.6472077166882,-70.1250927592573));
#153519=CARTESIAN_POINT('Ctrl Pts',(42.7172794741845,-46.649434527672,-69.2061704478816));
#153520=CARTESIAN_POINT('Ctrl Pts',(43.269605809916,-46.6516482924861,-68.2709029203465));
#153521=CARTESIAN_POINT('Ctrl Pts',(43.8276034398616,-46.6538471636059,
-67.3192749993308));
#153522=CARTESIAN_POINT('Ctrl Pts',(44.4025916272084,-46.6561129884974,
-66.3386708104082));
#153523=CARTESIAN_POINT('Ctrl Pts',(44.9836011759049,-46.6583629939592,
-65.3406943944767));
#153524=CARTESIAN_POINT('Ctrl Pts',(45.5707010314966,-46.6605955623318,
-64.3253600969817));
#153525=CARTESIAN_POINT('Ctrl Pts',(46.1180853657563,-46.6626771042377,
-63.3787100796264));
#153526=CARTESIAN_POINT('Ctrl Pts',(46.6707641600523,-46.6647434902106,
-62.4169713275415));
#153527=CARTESIAN_POINT('Ctrl Pts',(47.2288372631003,-46.6667937657809,
-61.440182400038));
#153528=CARTESIAN_POINT('Ctrl Pts',(47.2693283090469,-46.6669425237158,
-61.3693113884668));
#153529=CARTESIAN_POINT('Ctrl Pts',(47.3098477714336,-46.667091197001,-61.2983611610774));
#153530=CARTESIAN_POINT('Ctrl Pts',(47.3503956976423,-46.6672397853475,
-61.2273317382593));
#153531=CARTESIAN_POINT('',(42.8108476403353,-52.2735270043159,-61.2273317382593));
#153532=CARTESIAN_POINT('Origin',(0.,-12.9675000200281,-61.2273317382593));
#153533=CARTESIAN_POINT('Ctrl Pts',(42.8108476403353,-52.2735270043159,
-61.2273317382593));
#153534=CARTESIAN_POINT('Ctrl Pts',(42.1255968220058,-52.2708764489536,
-62.3136518407425));
#153535=CARTESIAN_POINT('Ctrl Pts',(41.4350707133446,-52.2681652890367,
-63.3966290232794));
#153536=CARTESIAN_POINT('Ctrl Pts',(40.7385684738071,-52.2653905871969,
-64.475770197359));
#153537=CARTESIAN_POINT('Ctrl Pts',(40.7403786971506,-52.3124027851469,
-64.4029616119961));
#153538=CARTESIAN_POINT('Ctrl Pts',(39.,-53.5547345046268,-65.2368833127815));
#153539=CARTESIAN_POINT('Ctrl Pts',(39.,-55.4603726203092,-66.5160529206996));
#153540=CARTESIAN_POINT('Ctrl Pts',(40.6386554420727,-49.6698429482511,
-68.4966218848756));
#153541=CARTESIAN_POINT('Ctrl Pts',(38.9999999999999,-50.9103452005084,
-69.3211688367401));
#153542=CARTESIAN_POINT('Ctrl Pts',(39.,-52.7124559353729,-70.609751474253));
#153543=CARTESIAN_POINT('Ctrl Pts',(40.5285598162873,-46.9462740729553,
-72.5399234557376));
#153544=CARTESIAN_POINT('Ctrl Pts',(39.,-48.1638674451749,-73.378963184763));
#153545=CARTESIAN_POINT('Ctrl Pts',(39.,-49.8653057974222,-74.6531246748237));
#153546=CARTESIAN_POINT('Ctrl Pts',(40.4106857765804,-44.1106698886037,
-76.4521234813751));
#153547=CARTESIAN_POINT('Ctrl Pts',(39.,-45.266598631985,-77.3351449301694));
#153548=CARTESIAN_POINT('Ctrl Pts',(39.,-46.8768348378863,-78.5652147900786));
#153549=CARTESIAN_POINT('',(39.,-46.93000002,-78.4955841262963));
#153550=CARTESIAN_POINT('',(39.,-52.5800000200005,-70.729306230469));
#153551=CARTESIAN_POINT('Ctrl Pts',(39.,-46.93000002,-78.4955841262963));
#153552=CARTESIAN_POINT('Ctrl Pts',(39.,-48.8725599414451,-75.9501559720627));
#153553=CARTESIAN_POINT('Ctrl Pts',(39.,-50.7491289418203,-73.3563309228582));
#153554=CARTESIAN_POINT('Ctrl Pts',(39.,-52.58000002,-70.7293062304687));
#153555=CARTESIAN_POINT('Ctrl Pts',(39.,-46.93000002,-78.4955841262963));
#153556=CARTESIAN_POINT('Ctrl Pts',(39.,-46.9255842492519,-78.4098091472741));
#153557=CARTESIAN_POINT('Ctrl Pts',(39.0008866619218,-46.920902618172,-78.3188865334045));
#153558=CARTESIAN_POINT('Ctrl Pts',(39.0030201782254,-46.9159544489267,
-78.2228086756993));
#153559=CARTESIAN_POINT('Ctrl Pts',(39.0050468444063,-46.9112540924074,
-78.1315425604054));
#153560=CARTESIAN_POINT('Ctrl Pts',(39.0081988100488,-46.9063132273459,
-78.0356246635966));
#153561=CARTESIAN_POINT('Ctrl Pts',(39.0128290773931,-46.90113159526,-77.9350548628545));
#153562=CARTESIAN_POINT('Ctrl Pts',(39.0175116979026,-46.8958913758787,
-77.8333479469085));
#153563=CARTESIAN_POINT('Ctrl Pts',(39.0237064111757,-46.8904046922954,
-77.7268790460392));
#153564=CARTESIAN_POINT('Ctrl Pts',(39.0318235339305,-46.8846730593421,
-77.6156825960158));
#153565=CARTESIAN_POINT('Ctrl Pts',(39.0384789387151,-46.8799735693215,
-77.524510217837));
#153566=CARTESIAN_POINT('Ctrl Pts',(39.046427676054,-46.8751093489263,-77.430158523236));
#153567=CARTESIAN_POINT('Ctrl Pts',(39.0559186572753,-46.8700818656153,
-77.3326586488547));
#153568=CARTESIAN_POINT('Ctrl Pts',(39.060664147886,-46.8675681239597,-77.283908711664));
#153569=CARTESIAN_POINT('Ctrl Pts',(39.065795502557,-46.8650135847254,-77.2343720793742));
#153570=CARTESIAN_POINT('Ctrl Pts',(39.0713456567497,-46.8624185135539,
-77.1840542212292));
#153571=CARTESIAN_POINT('Ctrl Pts',(39.0741207338461,-46.8611209779682,
-77.1588952921567));
#153572=CARTESIAN_POINT('Ctrl Pts',(39.0770005267778,-46.8598133115467,
-77.1335410980723));
#153573=CARTESIAN_POINT('Ctrl Pts',(39.0799892582902,-46.8584955542634,
-77.1079924524725));
#153574=CARTESIAN_POINT('Ctrl Pts',(39.0814836240464,-46.8578366756218,
-77.0952181296726));
#153575=CARTESIAN_POINT('Ctrl Pts',(39.0830052255386,-46.8571752743318,
-77.0823951952784));
#153576=CARTESIAN_POINT('Ctrl Pts',(39.0845545972427,-46.8565113557256,
-77.0695237573806));
#153577=CARTESIAN_POINT('Ctrl Pts',(39.0853292830947,-46.8561793964225,
-77.0630880384317));
#153578=CARTESIAN_POINT('Ctrl Pts',(39.0861109115594,-46.8558468077976,
-77.0566401937475));
#153579=CARTESIAN_POINT('Ctrl Pts',(39.0868995498376,-46.855513590546,-77.0501802373859));
#153580=CARTESIAN_POINT('Ctrl Pts',(39.0870967094071,-46.8554302862331,
-77.0485652482955));
#153581=CARTESIAN_POINT('Ctrl Pts',(39.0872943070911,-46.8553469426312,
-77.0469495022282));
#153582=CARTESIAN_POINT('Ctrl Pts',(39.087492343942,-46.8552635597513,-77.0453329994072));
#153583=CARTESIAN_POINT('Ctrl Pts',(39.0875504129536,-46.8552391099512,
-77.0448590031764));
#153584=CARTESIAN_POINT('Ctrl Pts',(39.0876090913764,-46.8552144165552,
-77.0443802848915));
#153585=CARTESIAN_POINT('Ctrl Pts',(39.0876650419913,-46.8551908825852,
-77.0439240441796));
#153586=CARTESIAN_POINT('Ctrl Pts',(39.0881815283767,-46.8549736378756,
-77.0397124351284));
#153587=CARTESIAN_POINT('Ctrl Pts',(39.0885201817289,-46.8548313832274,
-77.0369546251899));
#153588=CARTESIAN_POINT('Ctrl Pts',(39.0892865615655,-46.8545120536274,
-77.0307640477345));
#153589=CARTESIAN_POINT('Ctrl Pts',(39.1038378949207,-46.848448909429,-76.9132229122347));
#153590=CARTESIAN_POINT('Ctrl Pts',(39.1193530923716,-46.8426772179598,
-76.8027648546542));
#153591=CARTESIAN_POINT('Ctrl Pts',(39.1352365569654,-46.8372437726699,
-76.6993778537452));
#153592=CARTESIAN_POINT('Ctrl Pts',(39.1507083793338,-46.8319511427227,
-76.5986702717307));
#153593=CARTESIAN_POINT('Ctrl Pts',(39.1665293605593,-46.8269793809776,
-76.5046719635031));
#153594=CARTESIAN_POINT('Ctrl Pts',(39.1821968310681,-46.8223675906343,
-76.4173774322885));
#153595=CARTESIAN_POINT('Ctrl Pts',(39.1973614587387,-46.8179038143398,
-76.3328845932689));
#153596=CARTESIAN_POINT('Ctrl Pts',(39.2123821550198,-46.8137771916607,
-76.2546720979176));
#153597=CARTESIAN_POINT('Ctrl Pts',(39.2268511484975,-46.8100203816861,
-76.1827406339065));
#153598=CARTESIAN_POINT('Ctrl Pts',(39.2365066710429,-46.8075133680874,
-76.1347389623633));
#153599=CARTESIAN_POINT('Ctrl Pts',(39.2459174917404,-46.8051709836293,
-76.0895344918327));
#153600=CARTESIAN_POINT('Ctrl Pts',(39.2549753268259,-46.8030024901304,
-76.0471290191523));
#153601=CARTESIAN_POINT('Ctrl Pts',(39.2679244690509,-46.799902397176,-75.9865058689541));
#153602=CARTESIAN_POINT('Ctrl Pts',(39.2801621316059,-46.7971290289103,
-75.9315791013882));
#153603=CARTESIAN_POINT('Ctrl Pts',(39.2914380950645,-46.7946619198934,
-75.8823160645738));
#153604=CARTESIAN_POINT('Ctrl Pts',(39.3023895019119,-46.7922658217968,
-75.8344709681726));
#153605=CARTESIAN_POINT('Ctrl Pts',(39.3124339752469,-46.7901586455784,
-75.7919682881292));
#153606=CARTESIAN_POINT('Ctrl Pts',(39.3213888254142,-46.7883231875921,
-75.7547850060667));
#153607=CARTESIAN_POINT('Ctrl Pts',(39.3304763688448,-46.7864605317292,
-75.7170507409117));
#153608=CARTESIAN_POINT('Ctrl Pts',(39.3384424825747,-46.784876170525,-75.684792861159));
#153609=CARTESIAN_POINT('Ctrl Pts',(39.3451473014964,-46.7835508487111,
-75.6579881481457));
#153610=CARTESIAN_POINT('Ctrl Pts',(39.3484997109572,-46.7828881878041,
-75.6445857916391));
#153611=CARTESIAN_POINT('Ctrl Pts',(39.3515375662882,-46.7822903315084,
-75.632546809234));
#153612=CARTESIAN_POINT('Ctrl Pts',(39.3542479292085,-46.7817552642262,
-75.6218688811627));
#153613=CARTESIAN_POINT('Ctrl Pts',(39.3556031106687,-46.7814877305851,
-75.6165299171271));
#153614=CARTESIAN_POINT('Ctrl Pts',(39.3568764620696,-46.7812359081476,
-75.6115312270711));
#153615=CARTESIAN_POINT('Ctrl Pts',(39.3580666487484,-46.7809995683565,
-75.6068725597214));
#153616=CARTESIAN_POINT('Ctrl Pts',(39.3586617420878,-46.7808813984609,
-75.6045432260465));
#153617=CARTESIAN_POINT('Ctrl Pts',(39.3592360469333,-46.7807671000885,
-75.6022988986903));
#153618=CARTESIAN_POINT('Ctrl Pts',(39.3597894130148,-46.7806566486229,
-75.6001395497628));
#153619=CARTESIAN_POINT('Ctrl Pts',(39.3598612372675,-46.7806423125545,
-75.5998592766699));
#153620=CARTESIAN_POINT('Ctrl Pts',(39.3599327087539,-46.7806280413271,
-75.5995804352823));
#153621=CARTESIAN_POINT('Ctrl Pts',(39.3600038271003,-46.7806138349341,
-75.599303025727));
#153622=CARTESIAN_POINT('Ctrl Pts',(39.3602066724863,-46.7805733151326,
-75.5985117918037));
#153623=CARTESIAN_POINT('Ctrl Pts',(39.3604066500891,-46.7805333225372,
-75.5977322016091));
#153624=CARTESIAN_POINT('Ctrl Pts',(39.3606037509506,-46.7804938570154,
-75.5969642585609));
#153625=CARTESIAN_POINT('Ctrl Pts',(39.3607368535288,-46.7804672058752,
-75.5964456651928));
#153626=CARTESIAN_POINT('Ctrl Pts',(39.3608686444778,-46.7804407949061,
-75.5959323825031));
#153627=CARTESIAN_POINT('Ctrl Pts',(39.3609991215663,-46.7804146237221,
-75.5954244100684));
#153628=CARTESIAN_POINT('Ctrl Pts',(39.3610317408384,-46.7804080809262,
-75.5952974169597));
#153629=CARTESIAN_POINT('Ctrl Pts',(39.3610375440812,-46.7804069284516,
-75.5952748130406));
#153630=CARTESIAN_POINT('Ctrl Pts',(39.361036578518,-46.780407134699,-75.5952785550563));
#153631=CARTESIAN_POINT('Ctrl Pts',(39.3610358543456,-46.7804072893846,
-75.595281361568));
#153632=CARTESIAN_POINT('Ctrl Pts',(39.3610313231803,-46.7804082083531,
-75.5952989877083));
#153633=CARTESIAN_POINT('Ctrl Pts',(39.3610314438366,-46.7804081907787,
-75.5952985091008));
#153634=CARTESIAN_POINT('Ctrl Pts',(39.3610318058053,-46.7804081380554,
-75.5952970732781));
#153635=CARTESIAN_POINT('Ctrl Pts',(39.3610739620456,-46.780399656151,-75.595132688387));
#153636=CARTESIAN_POINT('Ctrl Pts',(39.3613866106273,-46.780336824024,-75.5939164234912));
#153637=CARTESIAN_POINT('Ctrl Pts',(39.3887993237504,-46.7748277663454,
-75.4872755409908));
#153638=CARTESIAN_POINT('Ctrl Pts',(39.4171239171424,-46.769455425969,-75.3838529125325));
#153639=CARTESIAN_POINT('Ctrl Pts',(39.4461119121629,-46.7642454946395,
-75.2836839374329));
#153640=CARTESIAN_POINT('Ctrl Pts',(39.4765319614061,-46.758778184207,-75.1785664516249));
#153641=CARTESIAN_POINT('Ctrl Pts',(39.5076823703915,-46.7534897219875,
-75.0770317440789));
#153642=CARTESIAN_POINT('Ctrl Pts',(39.5392965492066,-46.7484034641376,
-74.9790667613441));
#153643=CARTESIAN_POINT('Ctrl Pts',(39.5557430115697,-46.7457574694785,
-74.9281030019857));
#153644=CARTESIAN_POINT('Ctrl Pts',(39.5723153365704,-46.7431660963815,
-74.8781044890794));
#153645=CARTESIAN_POINT('Ctrl Pts',(39.5889783035331,-46.7406320190629,
-74.8290644524599));
#153646=CARTESIAN_POINT('Ctrl Pts',(39.6235154268386,-46.7353796686853,
-74.7274197816498));
#153647=CARTESIAN_POINT('Ctrl Pts',(39.6584382421912,-46.7303660691318,
-74.6299124838824));
#153648=CARTESIAN_POINT('Ctrl Pts',(39.6934473281028,-46.725573431974,-74.5365127275556));
#153649=CARTESIAN_POINT('Ctrl Pts',(39.6985874062929,-46.7248697709361,
-74.5227996574207));
#153650=CARTESIAN_POINT('Ctrl Pts',(39.7037293874539,-46.7241708730641,
-74.5091750510547));
#153651=CARTESIAN_POINT('Ctrl Pts',(39.7088723685335,-46.7234766821404,
-74.4956387342263));
#153652=CARTESIAN_POINT('Ctrl Pts',(39.7289582878229,-46.7207655185856,
-74.4427726312636));
#153653=CARTESIAN_POINT('Ctrl Pts',(39.7490592722323,-46.718125479337,-74.3912543559002));
#153654=CARTESIAN_POINT('Ctrl Pts',(39.7691234113894,-46.7155495625879,
-74.3410753456657));
#153655=CARTESIAN_POINT('Ctrl Pts',(39.7791554809679,-46.7142616042133,
-74.3159858405485));
#153656=CARTESIAN_POINT('Ctrl Pts',(39.7891783519126,-46.7129896836072,
-74.2912311569872));
#153657=CARTESIAN_POINT('Ctrl Pts',(39.7991858392501,-46.7117326802967,
-74.2668100718185));
#153658=CARTESIAN_POINT('Ctrl Pts',(39.8041895829188,-46.7111041786415,
-74.2545995292341));
#153659=CARTESIAN_POINT('Ctrl Pts',(39.8091894816777,-46.7104794068406,
-74.2424723866395));
#153660=CARTESIAN_POINT('Ctrl Pts',(39.8141847735823,-46.709858221149,-74.2304284891786));
#153661=CARTESIAN_POINT('Ctrl Pts',(39.8166824195346,-46.7095476283031,
-74.2244065404481));
#153662=CARTESIAN_POINT('Ctrl Pts',(39.819178913834,-46.7092379320185,-74.218405403026));
#153663=CARTESIAN_POINT('Ctrl Pts',(39.821674162369,-46.7089291135509,-74.2124250570812));
#153664=CARTESIAN_POINT('Ctrl Pts',(39.8234983881871,-46.7087033426052,
-74.2080529469205));
#153665=CARTESIAN_POINT('Ctrl Pts',(39.824874199419,-46.70853337947,-74.2047617703752));
#153666=CARTESIAN_POINT('Ctrl Pts',(39.826783209619,-46.7082978312743,-74.200205025373));
#153667=CARTESIAN_POINT('Ctrl Pts',(39.8274854193994,-46.7082111872916,
-74.1985288735604));
#153668=CARTESIAN_POINT('Ctrl Pts',(39.8282598940434,-46.7081156703967,
-74.1966815054939));
#153669=CARTESIAN_POINT('Ctrl Pts',(39.8291560336875,-46.7080052503693,
-74.1945463609026));
#153670=CARTESIAN_POINT('Ctrl Pts',(39.877269842631,-46.7020767902931,-74.0799102775538));
#153671=CARTESIAN_POINT('Ctrl Pts',(39.9264740604984,-46.6963385369307,
-73.968962778436));
#153672=CARTESIAN_POINT('Ctrl Pts',(39.9765878889061,-46.6907908225711,
-73.8617077695641));
#153673=CARTESIAN_POINT('Ctrl Pts',(40.0290875437083,-46.6849789918235,
-73.7493465487097));
#153674=CARTESIAN_POINT('Ctrl Pts',(40.0825853967005,-46.6793762726923,
-73.641037739188));
#153675=CARTESIAN_POINT('Ctrl Pts',(40.1368204676907,-46.6739818538525,
-73.5367631931971));
#153676=CARTESIAN_POINT('Ctrl Pts',(40.1929501737492,-46.6683989876682,
-73.4288459450216));
#153677=CARTESIAN_POINT('Ctrl Pts',(40.2498691844757,-46.6630392225076,
-73.3252496142913));
#153678=CARTESIAN_POINT('Ctrl Pts',(40.307235899747,-46.6579004797244,-73.2259317454814));
#153679=CARTESIAN_POINT('Ctrl Pts',(40.3682935377067,-46.6524311148681,
-73.1202238546246));
#153680=CARTESIAN_POINT('Ctrl Pts',(40.4298580477627,-46.6472121219459,
-73.0193625605604));
#153681=CARTESIAN_POINT('Ctrl Pts',(40.4914637898166,-46.6422397754793,
-72.9232736363168));
#153682=CARTESIAN_POINT('Ctrl Pts',(40.4992739249393,-46.6416094008342,
-72.9110918581721));
#153683=CARTESIAN_POINT('Ctrl Pts',(40.5070846601786,-46.6409829889087,
-72.8989867555173));
#153684=CARTESIAN_POINT('Ctrl Pts',(40.5148949946051,-46.6403605309214,
-72.886958154682));
#153685=CARTESIAN_POINT('Ctrl Pts',(40.7385684350658,-52.2653905899946,
-64.4757702529885));
#153686=CARTESIAN_POINT('Ctrl Pts',(40.6741963269159,-52.2700392402486,
-64.5682036154681));
#153687=CARTESIAN_POINT('Ctrl Pts',(40.6099114015966,-52.2749116374814,
-64.6650832096111));
#153688=CARTESIAN_POINT('Ctrl Pts',(40.546116711937,-52.2800128685024,-64.7665086919945));
#153689=CARTESIAN_POINT('Ctrl Pts',(40.4863184179071,-52.2847945347216,
-64.8615804111306));
#153690=CARTESIAN_POINT('Ctrl Pts',(40.4269511124508,-52.2897772674399,
-64.9606464072725));
#153691=CARTESIAN_POINT('Ctrl Pts',(40.368303754201,-52.2949643181793,-65.0637700989948));
#153692=CARTESIAN_POINT('Ctrl Pts',(40.3557054842752,-52.2960785689706,
-65.0859225052212));
#153693=CARTESIAN_POINT('Ctrl Pts',(40.3431402620066,-52.2972022442298,
-65.1082620785195));
#153694=CARTESIAN_POINT('Ctrl Pts',(40.3306106542808,-52.298335369721,-65.1307893189901));
#153695=CARTESIAN_POINT('Ctrl Pts',(40.2770643860162,-52.3031778710076,
-65.2270612604503));
#153696=CARTESIAN_POINT('Ctrl Pts',(40.2241778798164,-52.3081925187233,
-65.3267522112761));
#153697=CARTESIAN_POINT('Ctrl Pts',(40.172142097124,-52.3133789242405,-65.4298540962228));
#153698=CARTESIAN_POINT('Ctrl Pts',(40.1219281349228,-52.3183837489425,
-65.529346289589));
#153699=CARTESIAN_POINT('Ctrl Pts',(40.0725061689381,-52.3235485541602,
-65.6320155327409));
#153700=CARTESIAN_POINT('Ctrl Pts',(40.0240065700531,-52.328871683927,-65.737828636263));
#153701=CARTESIAN_POINT('Ctrl Pts',(39.9998035685206,-52.3315281124515,
-65.7906330875486));
#153702=CARTESIAN_POINT('Ctrl Pts',(39.9758295582964,-52.3342239524705,
-65.844220135671));
#153703=CARTESIAN_POINT('Ctrl Pts',(39.9520962441108,-52.3369588990613,
-65.8985836900181));
#153704=CARTESIAN_POINT('Ctrl Pts',(39.9501823456376,-52.3371794502268,
-65.9029676678667));
#153705=CARTESIAN_POINT('Ctrl Pts',(39.9478022209924,-52.3374543749929,
-65.9084324421974));
#153706=CARTESIAN_POINT('Ctrl Pts',(39.9463591924207,-52.3376214165691,
-65.9117507464063));
#153707=CARTESIAN_POINT('Ctrl Pts',(39.9439751906999,-52.3378973829726,
-65.9172328575015));
#153708=CARTESIAN_POINT('Ctrl Pts',(39.9415904249564,-52.338174107732,-65.9227302078874));
#153709=CARTESIAN_POINT('Ctrl Pts',(39.939204947652,-52.338451591336,-65.9282428006076));
#153710=CARTESIAN_POINT('Ctrl Pts',(39.8843720007904,-52.3448298719774,
-66.0549561016047));
#153711=CARTESIAN_POINT('Ctrl Pts',(39.8292508260476,-52.3516114098802,
-66.1897692462162));
#153712=CARTESIAN_POINT('Ctrl Pts',(39.77466324876,-52.3588065544525,-66.3328057530256));
#153713=CARTESIAN_POINT('Ctrl Pts',(39.7396281633994,-52.3634245008206,
-66.4246086223736));
#153714=CARTESIAN_POINT('Ctrl Pts',(39.7048123077817,-52.3682128157311,
-66.5197986983745));
#153715=CARTESIAN_POINT('Ctrl Pts',(39.6704219083266,-52.3731740475517,
-66.6184044463493));
#153716=CARTESIAN_POINT('Ctrl Pts',(39.6614376543415,-52.3744701350488,
-66.6441645159683));
#153717=CARTESIAN_POINT('Ctrl Pts',(39.6524843264061,-52.3757776790693,
-66.6701521715622));
#153718=CARTESIAN_POINT('Ctrl Pts',(39.6435649121351,-52.3770967667731,
-66.6963691459274));
#153719=CARTESIAN_POINT('Ctrl Pts',(39.6183188111944,-52.3808303999811,
-66.7705754066834));
#153720=CARTESIAN_POINT('Ctrl Pts',(39.5933299861079,-52.3846599397822,
-66.8466869090993));
#153721=CARTESIAN_POINT('Ctrl Pts',(39.5686982123625,-52.3885833393951,
-66.9246630559015));
#153722=CARTESIAN_POINT('Ctrl Pts',(39.5549282412021,-52.3907766487393,
-66.9682542850093));
#153723=CARTESIAN_POINT('Ctrl Pts',(39.541270848872,-52.3929991243851,-67.0124249390758));
#153724=CARTESIAN_POINT('Ctrl Pts',(39.5277411825347,-52.3952507861725,
-67.0571754321711));
#153725=CARTESIAN_POINT('Ctrl Pts',(39.4894213492339,-52.4016281278001,
-67.1839214577418));
#153726=CARTESIAN_POINT('Ctrl Pts',(39.4521147917285,-52.4082409660612,
-67.3153460673175));
#153727=CARTESIAN_POINT('Ctrl Pts',(39.4162038270705,-52.4150881216699,
-67.4514264537781));
#153728=CARTESIAN_POINT('Ctrl Pts',(39.4149453563048,-52.4153280747106,
-67.4561952810646));
#153729=CARTESIAN_POINT('Ctrl Pts',(39.4133617691025,-52.4156309953993,
-67.4622146571144));
#153730=CARTESIAN_POINT('Ctrl Pts',(39.4124335754226,-52.415808885988,-67.4657500795878));
#153731=CARTESIAN_POINT('Ctrl Pts',(39.4105797736013,-52.4161641716408,
-67.4728110764051));
#153732=CARTESIAN_POINT('Ctrl Pts',(39.4087222991178,-52.4165215150904,
-67.4799129639208));
#153733=CARTESIAN_POINT('Ctrl Pts',(39.4068613946353,-52.4168809133824,
-67.4870556836734));
#153734=CARTESIAN_POINT('Ctrl Pts',(39.381911700939,-52.4216994719838,-67.5828202280981));
#153735=CARTESIAN_POINT('Ctrl Pts',(39.3563089921541,-52.4268890153023,
-67.6859566474392));
#153736=CARTESIAN_POINT('Ctrl Pts',(39.3306172745555,-52.4324518255431,
-67.7965112043874));
#153737=CARTESIAN_POINT('Ctrl Pts',(39.3275224908695,-52.4331219128704,
-67.8098284315418));
#153738=CARTESIAN_POINT('Ctrl Pts',(39.3244264768482,-52.4337974167592,
-67.8232533055113));
#153739=CARTESIAN_POINT('Ctrl Pts',(39.3213302670964,-52.4344783414944,
-67.8367859134954));
#153740=CARTESIAN_POINT('Ctrl Pts',(39.2961897811093,-52.4400072882182,
-67.9466674682555));
#153741=CARTESIAN_POINT('Ctrl Pts',(39.2710330665147,-52.4458937489998,
-68.0636542200436));
#153742=CARTESIAN_POINT('Ctrl Pts',(39.2464418816062,-52.4521384400037,
-68.1877613272645));
#153743=CARTESIAN_POINT('Ctrl Pts',(39.241222042281,-52.4534639671711,-68.214104879282));
#153744=CARTESIAN_POINT('Ctrl Pts',(39.2360278299045,-52.4548056270789,
-68.2407690954401));
#153745=CARTESIAN_POINT('Ctrl Pts',(39.2308650220214,-52.4561634144658,
-68.267753883504));
#153746=CARTESIAN_POINT('Ctrl Pts',(39.2306328542106,-52.4562244732021,
-68.2689673702946));
#153747=CARTESIAN_POINT('Ctrl Pts',(39.230169613006,-52.4563464505562,-68.2713915594693));
#153748=CARTESIAN_POINT('Ctrl Pts',(39.2301687096753,-52.4563466885112,
-68.2713962886104));
#153749=CARTESIAN_POINT('Ctrl Pts',(39.2301344730456,-52.4563557071123,
-68.2715755251274));
#153750=CARTESIAN_POINT('Ctrl Pts',(39.2289672002148,-52.4566620223187,
-68.2776632593741));
#153751=CARTESIAN_POINT('Ctrl Pts',(39.2266941231712,-52.4572656889597,
-68.2896605972969));
#153752=CARTESIAN_POINT('Ctrl Pts',(39.2244113996309,-52.4578719174444,
-68.3017088495876));
#153753=CARTESIAN_POINT('Ctrl Pts',(39.2210134842536,-52.4587780266544,
-68.3197169721931));
#153754=CARTESIAN_POINT('Ctrl Pts',(39.2165803307865,-52.4599844003236,
-68.3436926461029));
#153755=CARTESIAN_POINT('Ctrl Pts',(39.2121153103965,-52.4611994457921,
-68.3678406648138));
#153756=CARTESIAN_POINT('Ctrl Pts',(39.2066001604335,-52.4627190883533,
-68.3980423412379));
#153757=CARTESIAN_POINT('Ctrl Pts',(39.2001691540676,-52.4645440491351,
-68.4343121208314));
#153758=CARTESIAN_POINT('Ctrl Pts',(39.1936237674451,-52.466401468209,-68.4712269855738));
#153759=CARTESIAN_POINT('Ctrl Pts',(39.1861293377007,-52.4685752693127,
-68.5144298402431));
#153760=CARTESIAN_POINT('Ctrl Pts',(39.1778832003543,-52.4710659880907,
-68.5639315451791));
#153761=CARTESIAN_POINT('Ctrl Pts',(39.1695997515529,-52.4735679766715,
-68.6136572314238));
#153762=CARTESIAN_POINT('Ctrl Pts',(39.1605581534571,-52.4763897165832,
-68.6697380841339));
#153763=CARTESIAN_POINT('Ctrl Pts',(39.1510103356013,-52.4795319125527,
-68.7321884721531));
#153764=CARTESIAN_POINT('Ctrl Pts',(39.1410905312248,-52.4827965296411,
-68.7970719504247));
#153765=CARTESIAN_POINT('Ctrl Pts',(39.1306246335061,-52.486407000624,-68.8688297769009));
#153766=CARTESIAN_POINT('Ctrl Pts',(39.1199512244241,-52.4903634279064,
-68.9474646303329));
#153767=CARTESIAN_POINT('Ctrl Pts',(39.1145062226234,-52.492381785257,-68.9875799220123));
#153768=CARTESIAN_POINT('Ctrl Pts',(39.1090080835936,-52.494490167789,-69.029484766641));
#153769=CARTESIAN_POINT('Ctrl Pts',(39.1035067882548,-52.4966885089909,
-69.0731779591835));
#153770=CARTESIAN_POINT('Ctrl Pts',(39.1029771369556,-52.4969001599207,
-69.077384633207));
#153771=CARTESIAN_POINT('Ctrl Pts',(39.1022508807535,-52.4971918158444,
-69.0831814548162));
#153772=CARTESIAN_POINT('Ctrl Pts',(39.1019177992675,-52.4973259667241,
-69.0858477071385));
#153773=CARTESIAN_POINT('Ctrl Pts',(39.1015249019274,-52.4974842088542,
-69.088992773704));
#153774=CARTESIAN_POINT('Ctrl Pts',(39.1011335086494,-52.4976423082182,
-69.0921350054727));
#153775=CARTESIAN_POINT('Ctrl Pts',(39.1007436120715,-52.4978002647885,
-69.0952744018884));
#153776=CARTESIAN_POINT('Ctrl Pts',(39.0832836734639,-52.5048737098396,
-69.235859551369));
#153777=CARTESIAN_POINT('Ctrl Pts',(39.0688275953131,-52.5116608692955,
-69.3707601805461));
#153778=CARTESIAN_POINT('Ctrl Pts',(39.0568219586142,-52.518159855566,-69.4999384882442));
#153779=CARTESIAN_POINT('Ctrl Pts',(39.0447636431752,-52.5246873583091,
-69.629683608905));
#153780=CARTESIAN_POINT('Ctrl Pts',(39.0351773266671,-52.5309241541674,
-69.7536560848756));
#153781=CARTESIAN_POINT('Ctrl Pts',(39.0275544970134,-52.5368686996032,
-69.8718244174154));
#153782=CARTESIAN_POINT('Ctrl Pts',(39.0199123078435,-52.5428283422574,
-69.9902928592144));
#153783=CARTESIAN_POINT('Ctrl Pts',(39.0142436155034,-52.5484942489622,
-70.1029276450134));
#153784=CARTESIAN_POINT('Ctrl Pts',(39.0100881477389,-52.5538652225379,
-70.209703776616));
#153785=CARTESIAN_POINT('Ctrl Pts',(39.0059150397578,-52.5592589962272,
-70.3169331794721));
#153786=CARTESIAN_POINT('Ctrl Pts',(39.0032680425101,-52.5643553280888,
-70.4182540860612));
#153787=CARTESIAN_POINT('Ctrl Pts',(39.0017332526658,-52.5691533557067,
-70.5136478931993));
#153788=CARTESIAN_POINT('Ctrl Pts',(39.0005167345971,-52.5729564088175,
-70.5892597370394));
#153789=CARTESIAN_POINT('Ctrl Pts',(39.,-52.5765720563163,-70.6611479548761));
#153790=CARTESIAN_POINT('Ctrl Pts',(39.,-52.58000002,-70.7293062304687));
#153791=CARTESIAN_POINT('Origin',(39.,46.91999998,-129.34995));
#153792=CARTESIAN_POINT('',(39.,-52.5800000199938,-161.329336741015));
#153793=CARTESIAN_POINT('',(39.,-46.9300000199928,-153.563058845201));
#153794=CARTESIAN_POINT('Ctrl Pts',(39.,-52.5800000199845,-161.329336741015));
#153795=CARTESIAN_POINT('Ctrl Pts',(39.,-50.7492254978239,-158.702450591995));
#153796=CARTESIAN_POINT('Ctrl Pts',(39.,-48.8724582313882,-156.108353723945));
#153797=CARTESIAN_POINT('Ctrl Pts',(39.,-46.9300000199928,-153.563058845201));
#153798=CARTESIAN_POINT('',(39.,-46.93000002,-129.34995));
#153799=CARTESIAN_POINT('',(39.,-52.58000002,-129.34995));
#153800=CARTESIAN_POINT('Ctrl Pts',(39.,-55.460351966619,-165.542559282053));
#153801=CARTESIAN_POINT('Ctrl Pts',(39.,-53.5547145065899,-166.821728771562));
#153802=CARTESIAN_POINT('Ctrl Pts',(40.7403779325784,-52.3123829231466,
-167.655650590757));
#153803=CARTESIAN_POINT('Ctrl Pts',(39.,-52.7145421899793,-161.452000516006));
#153804=CARTESIAN_POINT('Ctrl Pts',(38.9999999999999,-50.9123394210222,
-162.740555198018));
#153805=CARTESIAN_POINT('Ctrl Pts',(40.6387326052879,-49.6718481371244,
-163.565128292503));
#153806=CARTESIAN_POINT('Ctrl Pts',(39.,-49.8662825279046,-157.406795875704));
#153807=CARTESIAN_POINT('Ctrl Pts',(38.9999999999311,-48.1648205365349,
-158.680980229719));
#153808=CARTESIAN_POINT('Ctrl Pts',(40.5285982996977,-46.9471996283483,
-159.51999555488));
#153809=CARTESIAN_POINT('Ctrl Pts',(39.,-46.8768207417856,-153.493409728778));
#153810=CARTESIAN_POINT('Ctrl Pts',(39.,-45.2665850600662,-154.723479509065));
#153811=CARTESIAN_POINT('Ctrl Pts',(40.4106852206046,-44.110656513925,-155.606501037481));
#153812=CARTESIAN_POINT('',(40.5149261503614,-46.6404760392329,-159.171673926022));
#153813=CARTESIAN_POINT('',(40.7385684294474,-52.2653907112048,-167.582872729716));
#153814=CARTESIAN_POINT('Ctrl Pts',(40.5149617845453,-46.6408003036389,
-159.171515339397));
#153815=CARTESIAN_POINT('Ctrl Pts',(40.5335538982914,-47.0961591011677,
-159.826177485735));
#153816=CARTESIAN_POINT('Ctrl Pts',(40.5521766465686,-47.5547531683496,
-160.492365990833));
#153817=CARTESIAN_POINT('Ctrl Pts',(40.5708158550091,-48.0166562803791,
-161.170144960962));
#153818=CARTESIAN_POINT('Ctrl Pts',(40.5888975189152,-48.4647427350991,
-161.827649896304));
#153819=CARTESIAN_POINT('Ctrl Pts',(40.6069946714345,-48.9159431551024,
-162.496062436473));
#153820=CARTESIAN_POINT('Ctrl Pts',(40.6250928445344,-49.3703312806777,
-163.175393596044));
#153821=CARTESIAN_POINT('Ctrl Pts',(40.6427823317295,-49.8144585903571,
-163.839384363628));
#153822=CARTESIAN_POINT('Ctrl Pts',(40.6604727941326,-50.2616311860377,
-164.51380640413));
#153823=CARTESIAN_POINT('Ctrl Pts',(40.6781492466715,-50.7119252600374,
-165.198621116253));
#153824=CARTESIAN_POINT('Ctrl Pts',(40.6953050861943,-51.1489571166631,
-165.863266427761));
#153825=CARTESIAN_POINT('Ctrl Pts',(40.7124477273092,-51.5889292289694,
-166.53770137231));
#153826=CARTESIAN_POINT('Ctrl Pts',(40.729562078012,-52.0319192326658,-167.221841789087));
#153827=CARTESIAN_POINT('Ctrl Pts',(40.7325651077245,-52.1096500310188,
-167.341886892448));
#153828=CARTESIAN_POINT('Ctrl Pts',(40.7355672628713,-52.1874737695562,
-167.462230691843));
#153829=CARTESIAN_POINT('Ctrl Pts',(40.7385684573717,-52.2653908962637,
-167.582872566557));
#153830=CARTESIAN_POINT('Ctrl Pts',(40.5148965271728,-46.6403604087803,
-159.171687177116));
#153831=CARTESIAN_POINT('Ctrl Pts',(40.485505880482,-46.6427027446008,-159.126423040234));
#153832=CARTESIAN_POINT('Ctrl Pts',(40.4561230470032,-46.6450999497777,
-159.08009741564));
#153833=CARTESIAN_POINT('Ctrl Pts',(40.4267943476046,-46.6475528831212,
-159.032693440355));
#153834=CARTESIAN_POINT('Ctrl Pts',(40.3643789077675,-46.6527730571033,
-158.931811368252));
#153835=CARTESIAN_POINT('Ctrl Pts',(40.3022274691506,-46.6582166938404,
-158.826032696424));
#153836=CARTESIAN_POINT('Ctrl Pts',(40.2407519168729,-46.6639145603451,
-158.71523194619));
#153837=CARTESIAN_POINT('Ctrl Pts',(40.2154779760741,-46.6662570775797,
-158.669679340347));
#153838=CARTESIAN_POINT('Ctrl Pts',(40.1903177355716,-46.6686426274371,
-158.623278069988));
#153839=CARTESIAN_POINT('Ctrl Pts',(40.1652973161143,-46.6710736223053,
-158.57602023873));
#153840=CARTESIAN_POINT('Ctrl Pts',(40.1129408815272,-46.6761605963274,
-158.477130947318));
#153841=CARTESIAN_POINT('Ctrl Pts',(40.061187910713,-46.6814753763527,-158.374503906099));
#153842=CARTESIAN_POINT('Ctrl Pts',(40.0102983583742,-46.6870051091517,
-158.268129054487));
#153843=CARTESIAN_POINT('Ctrl Pts',(40.0055391015154,-46.6875222569265,
-158.258180740563));
#153844=CARTESIAN_POINT('Ctrl Pts',(40.000787361602,-46.6880412815843,-158.248199662502));
#153845=CARTESIAN_POINT('Ctrl Pts',(39.9960433292924,-46.688562170626,-158.238185821595));
#153846=CARTESIAN_POINT('Ctrl Pts',(39.9683079331311,-46.6916074837661,
-158.179641143458));
#153847=CARTESIAN_POINT('Ctrl Pts',(39.9408370839521,-46.6947156646751,
-158.11997668449));
#153848=CARTESIAN_POINT('Ctrl Pts',(39.9136694264136,-46.6978784774708,
-158.059195198908));
#153849=CARTESIAN_POINT('Ctrl Pts',(39.9000855976443,-46.6994598838686,
-158.028804456117));
#153850=CARTESIAN_POINT('Ctrl Pts',(39.8865774905551,-46.7010549168859,
-157.998134479889));
#153851=CARTESIAN_POINT('Ctrl Pts',(39.8731496300776,-46.7026621221226,
-157.967185912099));
#153852=CARTESIAN_POINT('Ctrl Pts',(39.8664356998389,-46.703465724741,-157.951711628204));
#153853=CARTESIAN_POINT('Ctrl Pts',(39.8597418255558,-46.7042723684712,
-157.936167697887));
#153854=CARTESIAN_POINT('Ctrl Pts',(39.8530685429161,-46.7050818534694,
-157.920554214528));
#153855=CARTESIAN_POINT('Ctrl Pts',(39.8497319015962,-46.7054865959685,
-157.912747472849));
#153856=CARTESIAN_POINT('Ctrl Pts',(39.8464004078077,-46.7058920486704,
-157.904923342997));
#153857=CARTESIAN_POINT('Ctrl Pts',(39.8430741268868,-46.7062981850526,
-157.897081837744));
#153858=CARTESIAN_POINT('Ctrl Pts',(39.8399222509519,-46.706683026718,-157.889651481654));
#153859=CARTESIAN_POINT('Ctrl Pts',(39.8360309238232,-46.7071598659057,
-157.880439145401));
#153860=CARTESIAN_POINT('Ctrl Pts',(39.8335156236791,-46.7074688074295,
-157.874466100708));
#153861=CARTESIAN_POINT('Ctrl Pts',(39.8333764427928,-46.7074859023099,
-157.874135589991));
#153862=CARTESIAN_POINT('Ctrl Pts',(39.8332414629469,-46.7075024828872,
-157.873815001909));
#153863=CARTESIAN_POINT('Ctrl Pts',(39.8331110389128,-46.7075185050603,
-157.873505188529));
#153864=CARTESIAN_POINT('Ctrl Pts',(39.8314301064126,-46.7077250022113,
-157.869512248248));
#153865=CARTESIAN_POINT('Ctrl Pts',(39.8297484996322,-46.7079318944916,
-157.86550999177));
#153866=CARTESIAN_POINT('Ctrl Pts',(39.8280662447799,-46.7081391851734,
-157.861498417039));
#153867=CARTESIAN_POINT('Ctrl Pts',(39.7687531704664,-46.7154478563873,
-157.720057998646));
#153868=CARTESIAN_POINT('Ctrl Pts',(39.7086758947724,-46.7232497705536,
-157.567010082113));
#153869=CARTESIAN_POINT('Ctrl Pts',(39.6492710002084,-46.731714411294,-157.40213520183));
#153870=CARTESIAN_POINT('Ctrl Pts',(39.6305758096956,-46.7343783007332,
-157.35024777201));
#153871=CARTESIAN_POINT('Ctrl Pts',(39.6119473744286,-46.7371081401241,
-157.297188794001));
#153872=CARTESIAN_POINT('Ctrl Pts',(39.5934307084091,-46.7399101225425,
-157.242950994996));
#153873=CARTESIAN_POINT('Ctrl Pts',(39.5539191783334,-46.7458890937288,
-157.127216422457));
#153874=CARTESIAN_POINT('Ctrl Pts',(39.5149265146814,-46.7521844764172,
-157.006122027191));
#153875=CARTESIAN_POINT('Ctrl Pts',(39.4769284603091,-46.7587734088497,
-156.879651340181));
#153876=CARTESIAN_POINT('Ctrl Pts',(39.4579294331229,-46.7620678750659,
-156.816415996676));
#153877=CARTESIAN_POINT('Ctrl Pts',(39.439179259145,-46.7654347814872,-156.751837220508));
#153878=CARTESIAN_POINT('Ctrl Pts',(39.4207374191931,-46.7688651930717,
-156.685917108977));
#153879=CARTESIAN_POINT('Ctrl Pts',(39.4115164992172,-46.7705803988639,
-156.652957053211));
#153880=CARTESIAN_POINT('Ctrl Pts',(39.4023726231759,-46.7723114718034,
-156.619661670513));
#153881=CARTESIAN_POINT('Ctrl Pts',(39.3933131608115,-46.7740568258333,
-156.586031547249));
#153882=CARTESIAN_POINT('Ctrl Pts',(39.3887834296293,-46.7749295028482,
-156.569216485616));
#153883=CARTESIAN_POINT('Ctrl Pts',(39.3842747984955,-46.7758057495308,
-156.552317739308));
#153884=CARTESIAN_POINT('Ctrl Pts',(39.3797881736941,-46.7766853518933,
-156.535335392793));
#153885=CARTESIAN_POINT('Ctrl Pts',(39.3775448612934,-46.7771251530745,
-156.526844219535));
#153886=CARTESIAN_POINT('Ctrl Pts',(39.3753070502474,-46.7775657931418,
-156.518332146253));
#153887=CARTESIAN_POINT('Ctrl Pts',(39.3730748531502,-46.7780072437074,
-156.509799184646));
#153888=CARTESIAN_POINT('Ctrl Pts',(39.3714007053272,-46.7783383316315,
-156.503399463442));
#153889=CARTESIAN_POINT('Ctrl Pts',(39.369729715331,-46.7786698754583,-156.496987992557));
#153890=CARTESIAN_POINT('Ctrl Pts',(39.3680619304574,-46.7790018628477,
-156.490564777184));
#153891=CARTESIAN_POINT('Ctrl Pts',(39.3675060021662,-46.7791125253109,
-156.488423705393));
#153892=CARTESIAN_POINT('Ctrl Pts',(39.3665115797823,-46.7793107839559,
-156.484586928693));
#153893=CARTESIAN_POINT('Ctrl Pts',(39.3663952165149,-46.779333994977,-156.484137647));
#153894=CARTESIAN_POINT('Ctrl Pts',(39.3651798359371,-46.7795764273605,
-156.479445030019));
#153895=CARTESIAN_POINT('Ctrl Pts',(39.3638113809044,-46.7798472112542,
-156.474145034342));
#153896=CARTESIAN_POINT('Ctrl Pts',(39.3622924024584,-46.7801465392495,
-156.468236627594));
#153897=CARTESIAN_POINT('Ctrl Pts',(39.3576875062211,-46.7810539743506,
-156.450324852692));
#153898=CARTESIAN_POINT('Ctrl Pts',(39.3516969630454,-46.7822232088955,
-156.42683241472));
#153899=CARTESIAN_POINT('Ctrl Pts',(39.3444292371885,-46.7836586304216,
-156.397743787219));
#153900=CARTESIAN_POINT('Ctrl Pts',(39.3394045741733,-46.7846510329414,
-156.377632881325));
#153901=CARTESIAN_POINT('Ctrl Pts',(39.3337705197713,-46.7857706667138,
-156.35484692661));
#153902=CARTESIAN_POINT('Ctrl Pts',(39.3275773655646,-46.7870189843683,
-156.329378991889));
#153903=CARTESIAN_POINT('Ctrl Pts',(39.3185244421424,-46.7888437288775,
-156.292150908258));
#153904=CARTESIAN_POINT('Ctrl Pts',(39.3082739032971,-46.7909453929226,
-156.249193109022));
#153905=CARTESIAN_POINT('Ctrl Pts',(39.2970184933079,-46.7933577839599,
-156.200472151143));
#153906=CARTESIAN_POINT('Ctrl Pts',(39.2857630833188,-46.7957701749971,
-156.151751193264));
#153907=CARTESIAN_POINT('Ctrl Pts',(39.2735027903882,-46.7984932254866,
-156.097267063491));
#153908=CARTESIAN_POINT('Ctrl Pts',(39.2604851284931,-46.8015632964374,
-156.036979329678));
#153909=CARTESIAN_POINT('Ctrl Pts',(39.247467466598,-46.8046333673881,-155.976691595865));
#153910=CARTESIAN_POINT('Ctrl Pts',(39.2336957527102,-46.8080429288287,
-155.910603676852));
#153911=CARTESIAN_POINT('Ctrl Pts',(39.2194870997902,-46.8117851407561,
-155.838698731947));
#153912=CARTESIAN_POINT('Ctrl Pts',(39.2052784468702,-46.8155273526834,
-155.766793787042));
#153913=CARTESIAN_POINT('Ctrl Pts',(39.1906327815456,-46.8196025971396,
-155.689071535734));
#153914=CARTESIAN_POINT('Ctrl Pts',(39.1759121851943,-46.824014590861,-155.605507258466));
#153915=CARTESIAN_POINT('Ctrl Pts',(39.161191588843,-46.8284265845825,-155.521942981197));
#153916=CARTESIAN_POINT('Ctrl Pts',(39.1463992322883,-46.833168409848,-155.432540854273));
#153917=CARTESIAN_POINT('Ctrl Pts',(39.1319534122398,-46.838197824685,-155.337304509702));
#153918=CARTESIAN_POINT('Ctrl Pts',(39.1247305022156,-46.8407125321035,
-155.289686337417));
#153919=CARTESIAN_POINT('Ctrl Pts',(39.1175949803997,-46.8432985882358,
-155.24060995796));
#153920=CARTESIAN_POINT('Ctrl Pts',(39.1106031571093,-46.8459469127866,
-155.190078297287));
#153921=CARTESIAN_POINT('Ctrl Pts',(39.1071072454641,-46.847271075062,-155.164812466951));
#153922=CARTESIAN_POINT('Ctrl Pts',(39.1036472844893,-46.8486108069295,
-155.139182814454));
#153923=CARTESIAN_POINT('Ctrl Pts',(39.1002305329326,-46.8499646445616,
-155.113189925138));
#153924=CARTESIAN_POINT('Ctrl Pts',(39.0985221571543,-46.8506415633776,
-155.10019348048));
#153925=CARTESIAN_POINT('Ctrl Pts',(39.096824584886,-46.8513220087368,-155.087106226545));
#153926=CARTESIAN_POINT('Ctrl Pts',(39.0951387325872,-46.8520057872307,
-155.073928243663));
#153927=CARTESIAN_POINT('Ctrl Pts',(39.0942958064377,-46.8523476764776,
-155.067339252221));
#153928=CARTESIAN_POINT('Ctrl Pts',(39.0934558103441,-46.8526903990116,
-155.060727578541));
#153929=CARTESIAN_POINT('Ctrl Pts',(39.0926188595233,-46.8530339294089,
-155.054093233508));
#153930=CARTESIAN_POINT('Ctrl Pts',(39.0917819087025,-46.8533774598063,
-155.047458888474));
#153931=CARTESIAN_POINT('Ctrl Pts',(39.0906930029478,-46.853827734122,-155.038751520483));
#153932=CARTESIAN_POINT('Ctrl Pts',(39.0901172584079,-46.854066918385,-155.034122195496));
#153933=CARTESIAN_POINT('Ctrl Pts',(39.0742562772155,-46.8606561204245,
-154.906590570869));
#153934=CARTESIAN_POINT('Ctrl Pts',(39.061129990202,-46.8670036349,-154.783735029668));
#153935=CARTESIAN_POINT('Ctrl Pts',(39.0502431981267,-46.8731065605454,
-154.665599454386));
#153936=CARTESIAN_POINT('Ctrl Pts',(39.0391497064693,-46.8793253579895,
-154.545220925085));
#153937=CARTESIAN_POINT('Ctrl Pts',(39.0303815861069,-46.8852901921471,
-154.429743243621));
#153938=CARTESIAN_POINT('Ctrl Pts',(39.0234682960032,-46.8909984573606,
-154.319202785664));
#153939=CARTESIAN_POINT('Ctrl Pts',(39.0164819666703,-46.8967670306597,
-154.207494462663));
#153940=CARTESIAN_POINT('Ctrl Pts',(39.0113899664732,-46.9022735872273,
-154.10082817691));
#153941=CARTESIAN_POINT('Ctrl Pts',(39.0077596161897,-46.9075158793827,
-153.999232157633));
#153942=CARTESIAN_POINT('Ctrl Pts',(39.004072963734,-46.9128394729037,-153.89606051173));
#153943=CARTESIAN_POINT('Ctrl Pts',(39.0018937009545,-46.9178905436415,
-153.79811756574));
#153944=CARTESIAN_POINT('Ctrl Pts',(39.000821918352,-46.9226671591535,-153.705424192369));
#153945=CARTESIAN_POINT('Ctrl Pts',(39.0002562987361,-46.9251879571451,
-153.65650644531));
#153946=CARTESIAN_POINT('Ctrl Pts',(39.,-46.9276323243641,-153.609050599416));
#153947=CARTESIAN_POINT('Ctrl Pts',(39.,-46.9300000199928,-153.563058845201));
#153948=CARTESIAN_POINT('Ctrl Pts',(39.,-52.5800000200011,-161.329336741015));
#153949=CARTESIAN_POINT('Ctrl Pts',(38.9999999999999,-52.5757636289944,
-161.413568993848));
#153950=CARTESIAN_POINT('Ctrl Pts',(39.0007875208437,-52.5712939085953,
-161.50340414571));
#153951=CARTESIAN_POINT('Ctrl Pts',(39.002705436195,-52.5665523334981,-161.598853214538));
#153952=CARTESIAN_POINT('Ctrl Pts',(39.0045946757477,-52.5618816522765,
-161.692875172275));
#153953=CARTESIAN_POINT('Ctrl Pts',(39.007580711382,-52.556947197286,-161.792344453901));
#153954=CARTESIAN_POINT('Ctrl Pts',(39.0120413122437,-52.5517104751597,
-161.897265269322));
#153955=CARTESIAN_POINT('Ctrl Pts',(39.014128447874,-52.549260188825,-161.94635820075));
#153956=CARTESIAN_POINT('Ctrl Pts',(39.0165391409009,-52.5467437004451,
-161.996644569051));
#153957=CARTESIAN_POINT('Ctrl Pts',(39.0193159959949,-52.5441569358408,
-162.048124286934));
#153958=CARTESIAN_POINT('Ctrl Pts',(39.0255457440389,-52.5383536471604,
-162.163616691443));
#153959=CARTESIAN_POINT('Ctrl Pts',(39.0336143349312,-52.5322056713611,
-162.285112131259));
#153960=CARTESIAN_POINT('Ctrl Pts',(39.0440353236384,-52.5257342581849,
-162.412568556975));
#153961=CARTESIAN_POINT('Ctrl Pts',(39.0459395812387,-52.5245517180179,
-162.435859040652));
#153962=CARTESIAN_POINT('Ctrl Pts',(39.0479225271856,-52.5233583822674,
-162.459348549214));
#153963=CARTESIAN_POINT('Ctrl Pts',(39.0499874806663,-52.522154386545,-162.483036799005));
#153964=CARTESIAN_POINT('Ctrl Pts',(39.0566701532884,-52.5182579746761,
-162.559697517917));
#153965=CARTESIAN_POINT('Ctrl Pts',(39.0642111230617,-52.5142513212459,
-162.63843891517));
#153966=CARTESIAN_POINT('Ctrl Pts',(39.0727245161976,-52.510148860684,-162.719244903039));
#153967=CARTESIAN_POINT('Ctrl Pts',(39.0769812127655,-52.5080976304031,
-162.759647896974));
#153968=CARTESIAN_POINT('Ctrl Pts',(39.0814810954767,-52.5060224564948,
-162.80056703288));
#153969=CARTESIAN_POINT('Ctrl Pts',(39.0862386725614,-52.5039259762791,
-162.841999704965));
#153970=CARTESIAN_POINT('Ctrl Pts',(39.0886174611038,-52.5028777361712,
-162.862716041008));
#153971=CARTESIAN_POINT('Ctrl Pts',(39.0910606769942,-52.501824169324,-162.883560761195));
#153972=CARTESIAN_POINT('Ctrl Pts',(39.0935701478725,-52.5007656343161,
-162.904533519597));
#153973=CARTESIAN_POINT('Ctrl Pts',(39.0948248833117,-52.5002363668122,
-162.915019898798));
#153974=CARTESIAN_POINT('Ctrl Pts',(39.0960961827068,-52.4997058572543,
-162.925538287561));
#153975=CARTESIAN_POINT('Ctrl Pts',(39.0973842749376,-52.4991741535183,
-162.936088640481));
#153976=CARTESIAN_POINT('Ctrl Pts',(39.0984281101808,-52.4987432751346,
-162.944638362265));
#153977=CARTESIAN_POINT('Ctrl Pts',(39.0996604129328,-52.4982394633436,
-162.954643068411));
#153978=CARTESIAN_POINT('Ctrl Pts',(39.1006502213987,-52.497838153136,-162.962616485939));
#153979=CARTESIAN_POINT('Ctrl Pts',(39.1008818361442,-52.497744246724,-162.964482262133));
#153980=CARTESIAN_POINT('Ctrl Pts',(39.1011000517209,-52.4976559520504,
-162.966236829985));
#153981=CARTESIAN_POINT('Ctrl Pts',(39.1012991554483,-52.4975755156648,
-162.967835546034));
#153982=CARTESIAN_POINT('Ctrl Pts',(39.1180987707534,-52.4907885993556,
-163.102729126186));
#153983=CARTESIAN_POINT('Ctrl Pts',(39.1369594452229,-52.4840212715504,
-163.23723004872));
#153984=CARTESIAN_POINT('Ctrl Pts',(39.158020961122,-52.477252165749,-163.37176382442));
#153985=CARTESIAN_POINT('Ctrl Pts',(39.179082477021,-52.4704830599476,-163.506297600119));
#153986=CARTESIAN_POINT('Ctrl Pts',(39.2023460261632,-52.4637119611059,
-163.640864383156));
#153987=CARTESIAN_POINT('Ctrl Pts',(39.2279803894119,-52.4570117183738,
-163.775880236838));
#153988=CARTESIAN_POINT('Ctrl Pts',(39.2536147526607,-52.4503114756418,
-163.910896090521));
#153989=CARTESIAN_POINT('Ctrl Pts',(39.2814446348001,-52.4435537149193,
-164.045151495395));
#153990=CARTESIAN_POINT('Ctrl Pts',(39.3114635522106,-52.4367950352887,
-164.178546542087));
#153991=CARTESIAN_POINT('Ctrl Pts',(39.3264730109159,-52.4334156954734,
-164.245244065433));
#153992=CARTESIAN_POINT('Ctrl Pts',(39.3420294553905,-52.4300359823671,
-164.311726457118));
#153993=CARTESIAN_POINT('Ctrl Pts',(39.3581260665589,-52.4266736702452,
-164.377982223013));
#153994=CARTESIAN_POINT('Ctrl Pts',(39.3661743721431,-52.4249925141843,
-164.41111010596));
#153995=CARTESIAN_POINT('Ctrl Pts',(39.3743576845704,-52.4233156920952,
-164.444181343468));
#153996=CARTESIAN_POINT('Ctrl Pts',(39.3826749315158,-52.4216453552344,
-164.477194551363));
#153997=CARTESIAN_POINT('Ctrl Pts',(39.3868335549885,-52.4208101868041,
-164.49370115531));
#153998=CARTESIAN_POINT('Ctrl Pts',(39.391025659974,-52.4199766385722,-164.510193252601));
#153999=CARTESIAN_POINT('Ctrl Pts',(39.3952510996912,-52.4191449731968,
-164.526670674556));
#154000=CARTESIAN_POINT('Ctrl Pts',(39.3973638195498,-52.4187291405091,
-164.534909385534));
#154001=CARTESIAN_POINT('Ctrl Pts',(39.3994848729635,-52.4183137784622,
-164.543144427728));
#154002=CARTESIAN_POINT('Ctrl Pts',(39.4016142407734,-52.4178989195526,
-164.551375780296));
#154003=CARTESIAN_POINT('Ctrl Pts',(39.4031446790737,-52.417600748442,-164.557291891724));
#154004=CARTESIAN_POINT('Ctrl Pts',(39.4044913051618,-52.4173392624714,
-164.562482058706));
#154005=CARTESIAN_POINT('Ctrl Pts',(39.4060594277002,-52.4170359365337,
-164.568507465127));
#154006=CARTESIAN_POINT('Ctrl Pts',(39.4066731047513,-52.4169172314182,
-164.570865478326));
#154007=CARTESIAN_POINT('Ctrl Pts',(39.4073208144597,-52.4167921189192,
-164.57335140041));
#154008=CARTESIAN_POINT('Ctrl Pts',(39.4080272966066,-52.4166558955955,
-164.576058742277));
#154009=CARTESIAN_POINT('Ctrl Pts',(39.4389568787749,-52.4106920782465,
-164.694585378933));
#154010=CARTESIAN_POINT('Ctrl Pts',(39.4709489777983,-52.4049043173862,
-164.80961245767));
#154011=CARTESIAN_POINT('Ctrl Pts',(39.5037549717153,-52.3992948524888,
-164.921096659683));
#154012=CARTESIAN_POINT('Ctrl Pts',(39.5382493737183,-52.3933966883399,
-165.038318557941));
#154013=CARTESIAN_POINT('Ctrl Pts',(39.5736433997348,-52.3876956313425,
-165.151623787289));
#154014=CARTESIAN_POINT('Ctrl Pts',(39.6096648516938,-52.3821914670209,
-165.261017822325));
#154015=CARTESIAN_POINT('Ctrl Pts',(39.6284113105696,-52.3793269631076,
-165.317949197034));
#154016=CARTESIAN_POINT('Ctrl Pts',(39.647327993138,-52.3765157420429,-165.373822126896));
#154017=CARTESIAN_POINT('Ctrl Pts',(39.6663784661277,-52.3737575148381,
-165.428642508953));
#154018=CARTESIAN_POINT('Ctrl Pts',(39.7053741027461,-52.3681115224344,
-165.540857869648));
#154019=CARTESIAN_POINT('Ctrl Pts',(39.7449238922867,-52.3626884946953,
-165.648643856583));
#154020=CARTESIAN_POINT('Ctrl Pts',(39.7847063969893,-52.3574869652637,
-165.752029633127));
#154021=CARTESIAN_POINT('Ctrl Pts',(39.8102919510438,-52.354141675332,-165.818520730005));
#154022=CARTESIAN_POINT('Ctrl Pts',(39.8359743201574,-52.3508879221915,
-165.88319338533));
#154023=CARTESIAN_POINT('Ctrl Pts',(39.8616696526033,-52.3477250660392,
-165.946060288054));
#154024=CARTESIAN_POINT('Ctrl Pts',(39.8745173188263,-52.3461436379631,
-165.977493739416));
#154025=CARTESIAN_POINT('Ctrl Pts',(39.8873682812456,-52.344584926784,-166.008475898349));
#154026=CARTESIAN_POINT('Ctrl Pts',(39.9002122316688,-52.3430488303558,
-166.039008789559));
#154027=CARTESIAN_POINT('Ctrl Pts',(39.9066342068805,-52.3422807821417,
-166.054275235164));
#154028=CARTESIAN_POINT('Ctrl Pts',(39.9130544350819,-52.3415183868975,
-166.069429378085));
#154029=CARTESIAN_POINT('Ctrl Pts',(39.9194716392171,-52.3407616305627,
-166.084471496975));
#154030=CARTESIAN_POINT('Ctrl Pts',(39.9226802412847,-52.3403832523953,
-166.09199255642));
#154031=CARTESIAN_POINT('Ctrl Pts',(39.9258880875008,-52.3400062839368,
-166.099485610224));
#154032=CARTESIAN_POINT('Ctrl Pts',(39.9290950189449,-52.3396307233536,
-166.106950694721));
#154033=CARTESIAN_POINT('Ctrl Pts',(39.930698484667,-52.339442943062,-166.11068323697));
#154034=CARTESIAN_POINT('Ctrl Pts',(39.9323017216999,-52.3392555147389,
-166.114408786899));
#154035=CARTESIAN_POINT('Ctrl Pts',(39.9339047102407,-52.3390684381484,
-166.118127349181));
#154036=CARTESIAN_POINT('Ctrl Pts',(39.9347062045111,-52.3389748998532,
-166.119986630323));
#154037=CARTESIAN_POINT('Ctrl Pts',(39.935507636658,-52.3388814494912,-166.121844164551));
#154038=CARTESIAN_POINT('Ctrl Pts',(39.9363090042075,-52.3387880870328,
-166.123699952453));
#154039=CARTESIAN_POINT('Ctrl Pts',(39.9367096879822,-52.3387414058036,
-166.124627846405));
#154040=CARTESIAN_POINT('Ctrl Pts',(39.9371103556077,-52.3386947465503,
-166.125555303774));
#154041=CARTESIAN_POINT('Ctrl Pts',(39.9375110067751,-52.3386481092691,
-166.126482324637));
#154042=CARTESIAN_POINT('Ctrl Pts',(39.9378016553992,-52.3386142766918,
-166.12715482321));
#154043=CARTESIAN_POINT('Ctrl Pts',(39.938092295362,-52.3385804556776,-166.127827092064));
#154044=CARTESIAN_POINT('Ctrl Pts',(39.9383829265455,-52.3385466462252,
-166.128499131229));
#154045=CARTESIAN_POINT('Ctrl Pts',(39.938492922488,-52.3385338502735,-166.128753479646));
#154046=CARTESIAN_POINT('Ctrl Pts',(39.9386010220686,-52.3385212764432,
-166.129003412917));
#154047=CARTESIAN_POINT('Ctrl Pts',(39.9387065331371,-52.3385090050618,
-166.129247334349));
#154048=CARTESIAN_POINT('Ctrl Pts',(39.9399964501902,-52.3383589822787,
-166.132229376132));
#154049=CARTESIAN_POINT('Ctrl Pts',(39.9409610502249,-52.3382468715858,
-166.134457830407));
#154050=CARTESIAN_POINT('Ctrl Pts',(39.9427463071851,-52.3380398161657,
-166.138573531837));
#154051=CARTESIAN_POINT('Ctrl Pts',(39.9909131807542,-52.3324533866124,
-166.249616633677));
#154052=CARTESIAN_POINT('Ctrl Pts',(40.040074614134,-52.3270302476623,-166.357417513742));
#154053=CARTESIAN_POINT('Ctrl Pts',(40.0901271983721,-52.3217716839405,
-166.461950306206));
#154054=CARTESIAN_POINT('Ctrl Pts',(40.1422107221744,-52.3162997481167,
-166.570724633593));
#154055=CARTESIAN_POINT('Ctrl Pts',(40.1952591438407,-52.3110060133846,
-166.675960294702));
#154056=CARTESIAN_POINT('Ctrl Pts',(40.249103194939,-52.3058907626207,-166.777651247629));
#154057=CARTESIAN_POINT('Ctrl Pts',(40.3044083654476,-52.3006367037243,
-166.882101699928));
#154058=CARTESIAN_POINT('Ctrl Pts',(40.360552693577,-52.2955709418491,-166.982812555586));
#154059=CARTESIAN_POINT('Ctrl Pts',(40.4173004895395,-52.2906926276812,
-167.079800199658));
#154060=CARTESIAN_POINT('Ctrl Pts',(40.4772368637466,-52.2855402079526,
-167.18223744202));
#154061=CARTESIAN_POINT('Ctrl Pts',(40.5378462972357,-52.2805968899478,
-167.280521365932));
#154062=CARTESIAN_POINT('Ctrl Pts',(40.59879608483,-52.27586045319,-167.374695481386));
#154063=CARTESIAN_POINT('Ctrl Pts',(40.645245648188,-52.2722508357007,-167.446465157953));
#154064=CARTESIAN_POINT('Ctrl Pts',(40.6918916531602,-52.268761345407,-167.515848441831));
#154065=CARTESIAN_POINT('Ctrl Pts',(40.7385684356245,-52.2653905899516,
-167.582872719316));
#154066=CARTESIAN_POINT('Origin',(0.,-12.9675000200281,-171.64995));
#154067=CARTESIAN_POINT('',(42.9629113790828,-52.2741145284007,-171.07256826174));
#154068=CARTESIAN_POINT('',(47.4880541505298,-46.6677435098469,-171.07256826174));
#154069=CARTESIAN_POINT('Origin',(0.,-12.9675000200281,-171.07256826174));
#154070=CARTESIAN_POINT('Ctrl Pts',(47.4880541505298,-46.6677435098469,
-171.07256826174));
#154071=CARTESIAN_POINT('Ctrl Pts',(46.9283768635402,-46.6656984714656,
-170.091223234496));
#154072=CARTESIAN_POINT('Ctrl Pts',(46.3741127719638,-46.6636372134722,
-169.12492957485));
#154073=CARTESIAN_POINT('Ctrl Pts',(45.8251573705305,-46.6615606438201,
-168.173728787141));
#154074=CARTESIAN_POINT('Ctrl Pts',(45.2609461023282,-46.6594263647987,
-167.196093443092));
#154075=CARTESIAN_POINT('Ctrl Pts',(44.7023427412084,-46.6572759119971,
-166.234401479565));
#154076=CARTESIAN_POINT('Ctrl Pts',(44.149280897441,-46.6551106551776,-165.288669126662));
#154077=CARTESIAN_POINT('Ctrl Pts',(43.5865485868871,-46.652907538136,-164.326400335003));
#154078=CARTESIAN_POINT('Ctrl Pts',(43.0295534282823,-46.6506890964257,
-163.380654060043));
#154079=CARTESIAN_POINT('Ctrl Pts',(42.4782718898617,-46.6484571462022,
-162.45141897123));
#154080=CARTESIAN_POINT('Ctrl Pts',(41.912450579805,-46.6461663294209,-161.497675777128));
#154081=CARTESIAN_POINT('Ctrl Pts',(41.3526483592774,-46.6438612834653,
-160.561326137806));
#154082=CARTESIAN_POINT('Ctrl Pts',(40.7988863618209,-46.6415443404656,
-159.642329260554));
#154083=CARTESIAN_POINT('Ctrl Pts',(40.7040758002953,-46.6411476525964,
-159.484986195532));
#154084=CARTESIAN_POINT('Ctrl Pts',(40.6094424040048,-46.6407506168077,
-159.32815173549));
#154085=CARTESIAN_POINT('Ctrl Pts',(40.5149864073608,-46.6403532458042,
-159.17182559703));
#154086=CARTESIAN_POINT('Ctrl Pts',(40.738568473807,-52.2653905871942,-167.582872774143));
#154087=CARTESIAN_POINT('Ctrl Pts',(41.4866208523709,-52.2683706527206,
-168.741884298091));
#154088=CARTESIAN_POINT('Ctrl Pts',(42.2277810204719,-52.2712774187735,
-169.905318536155));
#154089=CARTESIAN_POINT('Ctrl Pts',(42.9629113790828,-52.2741145284007,
-171.07256826174));
#154090=CARTESIAN_POINT('Origin',(0.,-12.9675000200281,-170.64995));
#154091=CARTESIAN_POINT('',(48.4122058243951,-46.93000002,-171.64995));
#154092=CARTESIAN_POINT('',(43.9094855672884,-52.58000002,-171.64995));
#154093=CARTESIAN_POINT('Origin',(0.,-12.9675000200281,-171.64995));
#154094=CARTESIAN_POINT('Ctrl Pts',(48.4122058243951,-46.93000002,-171.64995));
#154095=CARTESIAN_POINT('Ctrl Pts',(48.3795547379479,-46.9208088710473,
-171.64995));
#154096=CARTESIAN_POINT('Ctrl Pts',(48.3480259720962,-46.9118688891517,
-171.648414023011));
#154097=CARTESIAN_POINT('Ctrl Pts',(48.3177156961692,-46.9032522569107,
-171.645643509378));
#154098=CARTESIAN_POINT('Ctrl Pts',(48.2866802541381,-46.8944294738036,
-171.642806711868));
#154099=CARTESIAN_POINT('Ctrl Pts',(48.2569219491055,-46.8859454642817,
-171.63867615571));
#154100=CARTESIAN_POINT('Ctrl Pts',(48.2284995614569,-46.8778463555618,
-171.63356011004));
#154101=CARTESIAN_POINT('Ctrl Pts',(48.198916697874,-46.869416563126,-171.628235178053));
#154102=CARTESIAN_POINT('Ctrl Pts',(48.1707807231883,-46.8614035157324,
-171.621843200721));
#154103=CARTESIAN_POINT('Ctrl Pts',(48.1441156179165,-46.8538291316514,
-171.61470651212));
#154104=CARTESIAN_POINT('Ctrl Pts',(48.12245452578,-46.8476761677015,-171.608909105069));
#154105=CARTESIAN_POINT('Ctrl Pts',(48.101763104914,-46.8418120039883,-171.602619822146));
#154106=CARTESIAN_POINT('Ctrl Pts',(48.0820376369122,-46.8362364896225,
-171.595996656439));
#154107=CARTESIAN_POINT('Ctrl Pts',(48.0562396073805,-46.8289445316193,
-171.587334523582));
#154108=CARTESIAN_POINT('Ctrl Pts',(48.0320944146206,-46.8221467489661,
-171.578102851547));
#154109=CARTESIAN_POINT('Ctrl Pts',(48.0095649832056,-46.8158219187507,
-171.568617968669));
#154110=CARTESIAN_POINT('Ctrl Pts',(47.9927425203933,-46.811099242038,-171.561535717611));
#154111=CARTESIAN_POINT('Ctrl Pts',(47.9768201788659,-46.8066397235393,
-171.554311410389));
#154112=CARTESIAN_POINT('Ctrl Pts',(47.9617741294179,-46.8024283376171,
-171.547061058122));
#154113=CARTESIAN_POINT('Ctrl Pts',(47.944175917045,-46.7975026018549,-171.538580876037));
#154114=CARTESIAN_POINT('Ctrl Pts',(47.9277764289289,-46.7929162833264,
-171.530065584821));
#154115=CARTESIAN_POINT('Ctrl Pts',(47.9125296815332,-46.7886393940512,
-171.521677794724));
#154116=CARTESIAN_POINT('Ctrl Pts',(47.9049063078353,-46.7865009494136,
-171.517483899676));
#154117=CARTESIAN_POINT('Ctrl Pts',(47.8975710137052,-46.7844397807934,
-171.513321495654));
#154118=CARTESIAN_POINT('Ctrl Pts',(47.8905175870556,-46.7824517721236,
-171.509208644575));
#154119=CARTESIAN_POINT('Ctrl Pts',(47.8869908737309,-46.7814577677886,
-171.507152219036));
#154120=CARTESIAN_POINT('Ctrl Pts',(47.8835346346846,-46.7804820586724,
-171.505108166637));
#154121=CARTESIAN_POINT('Ctrl Pts',(47.8801480654843,-46.7795241076621,
-171.503078598546));
#154122=CARTESIAN_POINT('Ctrl Pts',(47.8784547808841,-46.7790451321569,
-171.5020638145));
#154123=CARTESIAN_POINT('Ctrl Pts',(47.8767789142175,-46.7785705965115,
-171.501052650544));
#154124=CARTESIAN_POINT('Ctrl Pts',(47.8751203661658,-46.7781004343759,
-171.500045363464));
#154125=CARTESIAN_POINT('Ctrl Pts',(47.8737467023028,-46.7777110306835,
-171.499211095286));
#154126=CARTESIAN_POINT('Ctrl Pts',(47.8732028318327,-46.7775573985475,
-171.498880505616));
#154127=CARTESIAN_POINT('Ctrl Pts',(47.8714562342584,-46.7770609996115,
-171.497809237805));
#154128=CARTESIAN_POINT('Ctrl Pts',(47.8710940073364,-46.7769580514217,
-171.497587067542));
#154129=CARTESIAN_POINT('Ctrl Pts',(47.8706801156592,-46.7768404051464,
-171.49733291326));
#154130=CARTESIAN_POINT('Ctrl Pts',(47.8701965793844,-46.7767030026997,
-171.497035384937));
#154131=CARTESIAN_POINT('Ctrl Pts',(47.836561660035,-46.7671452498347,-171.476339231072));
#154132=CARTESIAN_POINT('Ctrl Pts',(47.8047036022027,-46.7580497202331,
-171.454035671718));
#154133=CARTESIAN_POINT('Ctrl Pts',(47.7746907554855,-46.7494720426908,
-171.430440242212));
#154134=CARTESIAN_POINT('Ctrl Pts',(47.744142879704,-46.7407414537359,-171.40642418481));
#154135=CARTESIAN_POINT('Ctrl Pts',(47.7155063657762,-46.7325472033367,
-171.381070282487));
#154136=CARTESIAN_POINT('Ctrl Pts',(47.6888109308635,-46.7249172690417,
-171.354698000924));
#154137=CARTESIAN_POINT('Ctrl Pts',(47.6613862780346,-46.7170789139135,
-171.327605328767));
#154138=CARTESIAN_POINT('Ctrl Pts',(47.6360099672327,-46.709835977306,-171.299438368667));
#154139=CARTESIAN_POINT('Ctrl Pts',(47.6126733279724,-46.7031888660082,
-171.270521985313));
#154140=CARTESIAN_POINT('Ctrl Pts',(47.5889579777984,-46.6964338842684,
-171.241136342017));
#154141=CARTESIAN_POINT('Ctrl Pts',(47.5673486778549,-46.6902939779218,
-171.210977135119));
#154142=CARTESIAN_POINT('Ctrl Pts',(47.547799316212,-46.6847421919371,-171.180356754921));
#154143=CARTESIAN_POINT('Ctrl Pts',(47.5277922694594,-46.6790604288296,
-171.1490194975));
#154144=CARTESIAN_POINT('Ctrl Pts',(47.5099423764393,-46.6739943919686,
-171.117199563618));
#154145=CARTESIAN_POINT('Ctrl Pts',(47.4941672862597,-46.669490540989,-171.085196501643));
#154146=CARTESIAN_POINT('Ctrl Pts',(47.4920938454406,-46.6688985653896,
-171.080990094308));
#154147=CARTESIAN_POINT('Ctrl Pts',(47.4900562077632,-46.6683162712008,
-171.076780470406));
#154148=CARTESIAN_POINT('Ctrl Pts',(47.4880541505297,-46.6677435098468,
-171.072568261741));
#154149=CARTESIAN_POINT('Ctrl Pts',(42.9629113790828,-52.2741145284007,
-171.07256826174));
#154150=CARTESIAN_POINT('Ctrl Pts',(42.9756222718615,-52.2782546634559,
-171.098672923949));
#154151=CARTESIAN_POINT('Ctrl Pts',(42.9897028705913,-52.2828396112092,
-171.124738297516));
#154152=CARTESIAN_POINT('Ctrl Pts',(43.0052476387318,-52.2878991708896,
-171.150543690017));
#154153=CARTESIAN_POINT('Ctrl Pts',(43.013330346337,-52.290529955803,-171.163961544844));
#154154=CARTESIAN_POINT('Ctrl Pts',(43.0218083812408,-52.293288881294,-171.177309700215));
#154155=CARTESIAN_POINT('Ctrl Pts',(43.0306913485009,-52.2961789110827,
-171.190561243996));
#154156=CARTESIAN_POINT('Ctrl Pts',(43.0470490146324,-52.3015007974534,
-171.214963487364));
#154157=CARTESIAN_POINT('Ctrl Pts',(43.064778803995,-52.3072669331714,-171.23903038737));
#154158=CARTESIAN_POINT('Ctrl Pts',(43.0839005275333,-52.31348256218,-171.262607653843));
#154159=CARTESIAN_POINT('Ctrl Pts',(43.0949669386116,-52.3170797643665,
-171.276252643657));
#154160=CARTESIAN_POINT('Ctrl Pts',(43.1064988617158,-52.3208272871931,
-171.289734426472));
#154161=CARTESIAN_POINT('Ctrl Pts',(43.1184942836132,-52.3247242103712,
-171.303029756078));
#154162=CARTESIAN_POINT('Ctrl Pts',(43.1272258290788,-52.3275608060489,
-171.312707512804));
#154163=CARTESIAN_POINT('Ctrl Pts',(43.1362057486528,-52.3304774679509,
-171.322290183655));
#154164=CARTESIAN_POINT('Ctrl Pts',(43.14544820496,-52.333478680082,-171.331785371289));
#154165=CARTESIAN_POINT('Ctrl Pts',(43.1595109854538,-52.3380451487795,
-171.346232692977));
#154166=CARTESIAN_POINT('Ctrl Pts',(43.1740872867586,-52.3427767262898,
-171.360366229518));
#154167=CARTESIAN_POINT('Ctrl Pts',(43.1892239439584,-52.3476882653286,
-171.374181494434));
#154168=CARTESIAN_POINT('Ctrl Pts',(43.1988301566281,-52.3508052870011,
-171.382949108783));
#154169=CARTESIAN_POINT('Ctrl Pts',(43.2086621092605,-52.3539948050664,
-171.391588325689));
#154170=CARTESIAN_POINT('Ctrl Pts',(43.2187321357514,-52.3572607157877,
-171.400095850004));
#154171=CARTESIAN_POINT('Ctrl Pts',(43.2278830511384,-52.3602285404205,
-171.407826875858));
#154172=CARTESIAN_POINT('Ctrl Pts',(43.2372323602375,-52.3632600301537,
-171.415450206072));
#154173=CARTESIAN_POINT('Ctrl Pts',(43.2467668483314,-52.3663508159467,
-171.422945451982));
#154174=CARTESIAN_POINT('Ctrl Pts',(43.2728213692292,-52.3747968848117,
-171.443427415909));
#154175=CARTESIAN_POINT('Ctrl Pts',(43.3002828482488,-52.3836935947796,
-171.462969026633));
#154176=CARTESIAN_POINT('Ctrl Pts',(43.3291050777233,-52.3930240911597,
-171.481391787822));
#154177=CARTESIAN_POINT('Ctrl Pts',(43.332995320062,-52.3942834625797,-171.48387837567));
#154178=CARTESIAN_POINT('Ctrl Pts',(43.3369103005577,-52.3955507194566,
-171.486344636295));
#154179=CARTESIAN_POINT('Ctrl Pts',(43.3408498612603,-52.3968258055869,
-171.488790186207));
#154180=CARTESIAN_POINT('Ctrl Pts',(43.3444738260935,-52.3979987453243,
-171.491039824568));
#154181=CARTESIAN_POINT('Ctrl Pts',(43.348619785142,-52.3993405084081,-171.493577576822));
#154182=CARTESIAN_POINT('Ctrl Pts',(43.352338286152,-52.4005438861322,-171.495820868468));
#154183=CARTESIAN_POINT('Ctrl Pts',(43.3545029203103,-52.4012444029587,
-171.497126745677));
#154184=CARTESIAN_POINT('Ctrl Pts',(43.3565222632456,-52.401897888212,-171.498333988034));
#154185=CARTESIAN_POINT('Ctrl Pts',(43.3582062180294,-52.4024428669334,
-171.499335182402));
#154186=CARTESIAN_POINT('Ctrl Pts',(43.3649105815967,-52.4046126018451,
-171.503321257986));
#154187=CARTESIAN_POINT('Ctrl Pts',(43.3717389531774,-52.4068219286436,
-171.507281191728));
#154188=CARTESIAN_POINT('Ctrl Pts',(43.3786925372967,-52.4090712396164,
-171.51120960731));
#154189=CARTESIAN_POINT('Ctrl Pts',(43.4008365800392,-52.4162342849567,
-171.523719846788));
#154190=CARTESIAN_POINT('Ctrl Pts',(43.4243162170495,-52.423824032754,-171.535916815119));
#154191=CARTESIAN_POINT('Ctrl Pts',(43.4491265174689,-52.4318390452238,
-171.547571669372));
#154192=CARTESIAN_POINT('Ctrl Pts',(43.4590725867668,-52.435052140918,-171.552243921867));
#154193=CARTESIAN_POINT('Ctrl Pts',(43.4692320307583,-52.4383334238362,
-171.556828799921));
#154194=CARTESIAN_POINT('Ctrl Pts',(43.4796024564523,-52.4416821170203,
-171.561310538145));
#154195=CARTESIAN_POINT('Ctrl Pts',(43.5054793388387,-52.4500379687691,
-171.572493629016));
#154196=CARTESIAN_POINT('Ctrl Pts',(43.5326922691112,-52.4588199433374,
-171.583046072084));
#154197=CARTESIAN_POINT('Ctrl Pts',(43.5612393729964,-52.4680256720035,
-171.592719713033));
#154198=CARTESIAN_POINT('Ctrl Pts',(43.57551499012,-52.4726292023059,-171.597557233327));
#154199=CARTESIAN_POINT('Ctrl Pts',(43.5901240191453,-52.4773386219235,
-171.602174491315));
#154200=CARTESIAN_POINT('Ctrl Pts',(43.6050638744462,-52.4821528303647,
-171.606536419614));
#154201=CARTESIAN_POINT('Ctrl Pts',(43.6082649632574,-52.4831843469668,
-171.60747102839));
#154202=CARTESIAN_POINT('Ctrl Pts',(43.6114812396548,-52.4842206741277,
-171.608393905187));
#154203=CARTESIAN_POINT('Ctrl Pts',(43.614712668377,-52.4852618572514,-171.609304696318));
#154204=CARTESIAN_POINT('Ctrl Pts',(43.6171456120831,-52.4860457643543,
-171.609990431249));
#154205=CARTESIAN_POINT('Ctrl Pts',(43.6204559687148,-52.4871122872049,
-171.610908827037));
#154206=CARTESIAN_POINT('Ctrl Pts',(43.6226813902947,-52.4878292091908,
-171.611517580204));
#154207=CARTESIAN_POINT('Ctrl Pts',(43.6234117671554,-52.4880645008919,
-171.611717371216));
#154208=CARTESIAN_POINT('Ctrl Pts',(43.6240252456133,-52.4882621270372,
-171.611884340861));
#154209=CARTESIAN_POINT('Ctrl Pts',(43.6244523866038,-52.4883997220079,
-171.612000396047));
#154210=CARTESIAN_POINT('Ctrl Pts',(43.6289479545664,-52.4898478797731,
-171.61322185216));
#154211=CARTESIAN_POINT('Ctrl Pts',(43.6337045827901,-52.4913799689085,
-171.614482833112));
#154212=CARTESIAN_POINT('Ctrl Pts',(43.6387203708674,-52.49299531386,-171.615771589263));
#154213=CARTESIAN_POINT('Ctrl Pts',(43.6521489264918,-52.4973200080455,
-171.619221921174));
#154214=CARTESIAN_POINT('Ctrl Pts',(43.6674571356465,-52.5022486368226,
-171.622889155636));
#154215=CARTESIAN_POINT('Ctrl Pts',(43.6846428372704,-52.5077791164167,
-171.626522702309));
#154216=CARTESIAN_POINT('Ctrl Pts',(43.702262529913,-52.5134492573716,-171.630248007041));
#154217=CARTESIAN_POINT('Ctrl Pts',(43.7218557516377,-52.5197520367826,
-171.633937845606));
#154218=CARTESIAN_POINT('Ctrl Pts',(43.7434271305591,-52.5266870794093,
-171.6372677803));
#154219=CARTESIAN_POINT('Ctrl Pts',(43.7653502121052,-52.5337351918914,
-171.640652006691));
#154220=CARTESIAN_POINT('Ctrl Pts',(43.7893165109233,-52.5414363642839,
-171.643664337744));
#154221=CARTESIAN_POINT('Ctrl Pts',(43.8153376259069,-52.549791966158,-171.64591050217));
#154222=CARTESIAN_POINT('Ctrl Pts',(43.8419949736875,-52.5583518678077,
-171.648211586744));
#154223=CARTESIAN_POINT('Ctrl Pts',(43.8708088768737,-52.5675986046511,
-171.649708459496));
#154224=CARTESIAN_POINT('Ctrl Pts',(43.9017983937575,-52.577535306748,-171.649923358981));
#154225=CARTESIAN_POINT('Ctrl Pts',(43.9043460731332,-52.5783522130292,
-171.649941026084));
#154226=CARTESIAN_POINT('Ctrl Pts',(43.9069084601724,-52.5791737833863,
-171.64995));
#154227=CARTESIAN_POINT('Ctrl Pts',(43.9094855672884,-52.58000002,-171.64995));
#154228=CARTESIAN_POINT('Origin',(0.,-12.9675000200281,-171.64995));
#154229=CARTESIAN_POINT('',(49.6300753314849,-52.58000002,-171.64995));
#154230=CARTESIAN_POINT('',(50.4241310475534,-46.93000002,-171.64995));
#154231=CARTESIAN_POINT('',(50.5139609686817,-46.2908269190399,-171.64995));
#154232=CARTESIAN_POINT('',(48.7591445042216,-46.93000002,-171.64995));
#154233=CARTESIAN_POINT('',(49.5598049141337,-52.58000002,-171.64995));
#154234=CARTESIAN_POINT('Origin',(60.,-2.55003103885676E-14,0.));
#154235=CARTESIAN_POINT('',(60.,-53.58000002,-58.24995));
#154236=CARTESIAN_POINT('',(60.,-54.08000002,-58.24995));
#154237=CARTESIAN_POINT('',(60.,-54.58000002,-58.24995));
#154238=CARTESIAN_POINT('',(60.,-54.08000002,-174.34995));
#154239=CARTESIAN_POINT('',(60.,-54.08000002,-174.34995));
#154240=CARTESIAN_POINT('',(60.,-53.58000002,-174.34995));
#154241=CARTESIAN_POINT('',(60.,28.41999998,-174.34995));
#154242=CARTESIAN_POINT('',(60.,-53.58000002,-58.24995));
#154243=CARTESIAN_POINT('Origin',(57.,-2.42462934179819E-14,-174.34995));
#154244=CARTESIAN_POINT('',(57.,-54.08000002,-177.34995));
#154245=CARTESIAN_POINT('Origin',(57.,-54.08000002,-174.34995));
#154246=CARTESIAN_POINT('',(57.,-53.58000002,-177.34995));
#154247=CARTESIAN_POINT('',(57.,-54.58000002,-177.34995));
#154248=CARTESIAN_POINT('Origin',(57.,-53.58000002,-174.34995));
#154249=CARTESIAN_POINT('Origin',(60.,28.41999998,-177.34995));
#154250=CARTESIAN_POINT('',(50.9340054382093,-54.08000002,-177.34995));
#154251=CARTESIAN_POINT('',(60.,-54.08000002,-177.34995));
#154252=CARTESIAN_POINT('',(51.0042758555605,-53.58000002,-177.34995));
#154253=CARTESIAN_POINT('',(62.4796469926385,28.0715083218873,-177.34995));
#154254=CARTESIAN_POINT('',(60.,-53.58000002,-177.34995));
#154255=CARTESIAN_POINT('Origin',(0.,-12.9675000200281,-170.64995));
#154256=CARTESIAN_POINT('',(52.1126146143194,-39.473850183348,-171.391638125813));
#154257=CARTESIAN_POINT('',(52.4185037493065,-38.6078427690472,-171.271207233798));
#154258=CARTESIAN_POINT('Ctrl Pts',(52.1126146143194,-39.473850183348,-171.391638125813));
#154259=CARTESIAN_POINT('Ctrl Pts',(52.1380831145661,-39.3921942843444,
-171.378688901202));
#154260=CARTESIAN_POINT('Ctrl Pts',(52.1640396477339,-39.3120540081033,
-171.366154150429));
#154261=CARTESIAN_POINT('Ctrl Pts',(52.1904049108065,-39.233350279785,-171.354220830313));
#154262=CARTESIAN_POINT('Ctrl Pts',(52.21740941517,-39.1527383333408,-171.341998179841));
#154263=CARTESIAN_POINT('Ctrl Pts',(52.2448426634599,-39.0736335235921,
-171.33040624582));
#154264=CARTESIAN_POINT('Ctrl Pts',(52.2726181340388,-38.9959696675765,
-171.319592910656));
#154265=CARTESIAN_POINT('Ctrl Pts',(52.3015399982203,-38.9151003448007,
-171.308333270246));
#154266=CARTESIAN_POINT('Ctrl Pts',(52.3308328658517,-38.8357934271155,
-171.297917697251));
#154267=CARTESIAN_POINT('Ctrl Pts',(52.3603984063869,-38.7579933413912,
-171.288458976171));
#154268=CARTESIAN_POINT('Ctrl Pts',(52.3796601931508,-38.7073070141901,
-171.2822966715));
#154269=CARTESIAN_POINT('Ctrl Pts',(52.3990377034992,-38.657260644957,-171.27653939255));
#154270=CARTESIAN_POINT('Ctrl Pts',(52.4185037670893,-38.6078427777457,
-171.271207218103));
#154271=CARTESIAN_POINT('',(52.2951895046066,-38.58067735034,-171.07256826174));
#154272=CARTESIAN_POINT('Origin',(53.1718788440769,-38.7731638601678,-170.641452709883));
#154273=CARTESIAN_POINT('',(49.1544657093286,-44.1870483688939,-171.07256826174));
#154274=CARTESIAN_POINT('Origin',(0.,-12.9675000200281,-171.07256826174));
#154275=CARTESIAN_POINT('Ctrl Pts',(49.1544657093286,-44.1870483688939,
-171.07256826174));
#154276=CARTESIAN_POINT('Ctrl Pts',(49.1674099450031,-44.1904999604323,
-171.099968982618));
#154277=CARTESIAN_POINT('Ctrl Pts',(49.1818195618825,-44.1943411562328,
-171.12729943789));
#154278=CARTESIAN_POINT('Ctrl Pts',(49.1977879406042,-44.1985958890317,
-171.154324681996));
#154279=CARTESIAN_POINT('Ctrl Pts',(49.2047680888881,-44.2004557313089,
-171.166138042298));
#154280=CARTESIAN_POINT('Ctrl Pts',(49.2120456036907,-44.2023944608238,
-171.177893516791));
#154281=CARTESIAN_POINT('Ctrl Pts',(49.2196259920141,-44.2044134518367,
-171.189573569196));
#154282=CARTESIAN_POINT('Ctrl Pts',(49.2343858775653,-44.2083446589212,
-171.212315970954));
#154283=CARTESIAN_POINT('Ctrl Pts',(49.2502933549397,-44.2125799775673,
-171.234767669611));
#154284=CARTESIAN_POINT('Ctrl Pts',(49.2673661857556,-44.2171233653378,
-171.256807716226));
#154285=CARTESIAN_POINT('Ctrl Pts',(49.2780167292262,-44.2199576667771,
-171.27055695776));
#154286=CARTESIAN_POINT('Ctrl Pts',(49.2891203199703,-44.2229117312905,
-171.284146427066));
#154287=CARTESIAN_POINT('Ctrl Pts',(49.3006765847195,-44.2259852536784,
-171.297551077901));
#154288=CARTESIAN_POINT('Ctrl Pts',(49.3076450228149,-44.2278385904581,
-171.305634094477));
#154289=CARTESIAN_POINT('Ctrl Pts',(49.3147792321624,-44.2297356757576,
-171.31365165429));
#154290=CARTESIAN_POINT('Ctrl Pts',(49.322089013489,-44.2316790662859,-171.321609324439));
#154291=CARTESIAN_POINT('Ctrl Pts',(49.3361254166797,-44.2354108076054,
-171.336889818026));
#154292=CARTESIAN_POINT('Ctrl Pts',(49.3507349332876,-44.2392935037787,
-171.351849549341));
#154293=CARTESIAN_POINT('Ctrl Pts',(49.3659444071017,-44.2433339581765,
-171.366466996183));
#154294=CARTESIAN_POINT('Ctrl Pts',(49.3768819596723,-44.2462395604955,
-171.376978805811));
#154295=CARTESIAN_POINT('Ctrl Pts',(49.3881298096026,-44.2492267542621,
-171.387313431887));
#154296=CARTESIAN_POINT('Ctrl Pts',(49.3996980831345,-44.2522980875319,
-171.397460025651));
#154297=CARTESIAN_POINT('Ctrl Pts',(49.4100384253246,-44.2550434096321,
-171.406529594355));
#154298=CARTESIAN_POINT('Ctrl Pts',(49.420635347381,-44.2578561071891,-171.415448967782));
#154299=CARTESIAN_POINT('Ctrl Pts',(49.4314773883421,-44.2607330292976,
-171.424194851323));
#154300=CARTESIAN_POINT('Ctrl Pts',(49.4582917280625,-44.2678481810523,
-171.445825012401));
#154301=CARTESIAN_POINT('Ctrl Pts',(49.4866223506434,-44.275360699466,-171.466406988852));
#154302=CARTESIAN_POINT('Ctrl Pts',(49.5164137343661,-44.283254020249,-171.485716798992));
#154303=CARTESIAN_POINT('Ctrl Pts',(49.5199598905896,-44.2841935854897,
-171.488015302615));
#154304=CARTESIAN_POINT('Ctrl Pts',(49.5239976875963,-44.2852633080731,
-171.490595498519));
#154305=CARTESIAN_POINT('Ctrl Pts',(49.5276130959414,-44.2862210486011,
-171.492872353817));
#154306=CARTESIAN_POINT('Ctrl Pts',(49.5295802652792,-44.2867421620191,
-171.494111206943));
#154307=CARTESIAN_POINT('Ctrl Pts',(49.531421900296,-44.2872299980374,-171.49526124167));
#154308=CARTESIAN_POINT('Ctrl Pts',(49.5329880148365,-44.2876448451646,
-171.496233960813));
#154309=CARTESIAN_POINT('Ctrl Pts',(49.5370095623471,-44.2887101104364,
-171.498731757843));
#154310=CARTESIAN_POINT('Ctrl Pts',(49.5410793863111,-44.2897880343388,
-171.501220670594));
#154311=CARTESIAN_POINT('Ctrl Pts',(49.5451978658055,-44.2908787108092,
-171.503699197074));
#154312=CARTESIAN_POINT('Ctrl Pts',(49.5699429400149,-44.2974318259181,
-171.518590936068));
#154313=CARTESIAN_POINT('Ctrl Pts',(49.5964058211158,-44.3044348265418,
-171.533094285846));
#154314=CARTESIAN_POINT('Ctrl Pts',(49.6246582855736,-44.3119055301866,
-171.54685574217));
#154315=CARTESIAN_POINT('Ctrl Pts',(49.6332772021546,-44.3141846011545,
-171.551053919085));
#154316=CARTESIAN_POINT('Ctrl Pts',(49.6420624484702,-44.3165071389794,
-171.555182772464));
#154317=CARTESIAN_POINT('Ctrl Pts',(49.6510154288811,-44.3188734756713,
-171.559231527241));
#154318=CARTESIAN_POINT('Ctrl Pts',(49.6726079214831,-44.3245805257451,
-171.568996175831));
#154319=CARTESIAN_POINT('Ctrl Pts',(49.6951721931324,-44.3305411806568,
-171.578293225514));
#154320=CARTESIAN_POINT('Ctrl Pts',(49.7187075835833,-44.3367544577215,
-171.586960972345));
#154321=CARTESIAN_POINT('Ctrl Pts',(49.7304752788088,-44.3398610962538,
-171.59129484576));
#154322=CARTESIAN_POINT('Ctrl Pts',(49.7424854973315,-44.3430308211926,
-171.595471243433));
#154323=CARTESIAN_POINT('Ctrl Pts',(49.7547365163585,-44.3462630678917,
-171.599469109271));
#154324=CARTESIAN_POINT('Ctrl Pts',(49.760862025872,-44.3478791912413,-171.601468042189));
#154325=CARTESIAN_POINT('Ctrl Pts',(49.7670477359762,-44.3495109450574,
-171.603422339684));
#154326=CARTESIAN_POINT('Ctrl Pts',(49.7732933004513,-44.3511582236526,
-171.605329314684));
#154327=CARTESIAN_POINT('Ctrl Pts',(49.7764160826888,-44.3519818629502,
-171.606282802184));
#154328=CARTESIAN_POINT('Ctrl Pts',(49.77955382855,-44.3528093834448,-171.607224458979));
#154329=CARTESIAN_POINT('Ctrl Pts',(49.7827064904596,-44.3536407707549,
-171.608153947255));
#154330=CARTESIAN_POINT('Ctrl Pts',(49.7851118263354,-44.3542750809921,
-171.608863104012));
#154331=CARTESIAN_POINT('Ctrl Pts',(49.7883547859396,-44.3551302199853,
-171.60980415202));
#154332=CARTESIAN_POINT('Ctrl Pts',(49.7905382446473,-44.3557059426006,
-171.610428960928));
#154333=CARTESIAN_POINT('Ctrl Pts',(49.7912166345354,-44.3558848167874,
-171.610623085984));
#154334=CARTESIAN_POINT('Ctrl Pts',(49.791792643767,-44.356036692665,-171.610787142201));
#154335=CARTESIAN_POINT('Ctrl Pts',(49.7922091744941,-44.3561465181287,
-171.610905567567));
#154336=CARTESIAN_POINT('Ctrl Pts',(49.8044703717807,-44.3593793928967,
-171.614391593156));
#154337=CARTESIAN_POINT('Ctrl Pts',(49.8184706367615,-44.3630698175465,
-171.618127956761));
#154338=CARTESIAN_POINT('Ctrl Pts',(49.8342418983615,-44.3672252172811,
-171.621894685085));
#154339=CARTESIAN_POINT('Ctrl Pts',(49.8498640564744,-44.3713413313448,
-171.625625802286));
#154340=CARTESIAN_POINT('Ctrl Pts',(49.8672244691343,-44.3759138263744,
-171.629386605));
#154341=CARTESIAN_POINT('Ctrl Pts',(49.8863472451527,-44.3809478076652,
-171.632913171055));
#154342=CARTESIAN_POINT('Ctrl Pts',(49.9052048010337,-44.385911970996,-171.636390825993));
#154343=CARTESIAN_POINT('Ctrl Pts',(49.9257768087209,-44.3913250774835,
-171.639640560882));
#154344=CARTESIAN_POINT('Ctrl Pts',(49.9480705932716,-44.3971875545849,
-171.64236215772));
#154345=CARTESIAN_POINT('Ctrl Pts',(49.969627485023,-44.4028562549342,-171.644993795623));
#154346=CARTESIAN_POINT('Ctrl Pts',(49.9927947579018,-44.4089452546521,
-171.647131375962));
#154347=CARTESIAN_POINT('Ctrl Pts',(50.0175556679848,-44.4154484770367,
-171.64846219077));
#154348=CARTESIAN_POINT('Ctrl Pts',(50.0352273714949,-44.4200897853511,
-171.649411984806));
#154349=CARTESIAN_POINT('Ctrl Pts',(50.0537103637574,-44.4249419583976,
-171.64995));
#154350=CARTESIAN_POINT('Ctrl Pts',(50.0729884546894,-44.43000002,-171.64995));
#154351=CARTESIAN_POINT('Ctrl Pts',(50.9867892914962,-42.9264785869994,
-171.64995));
#154352=CARTESIAN_POINT('Ctrl Pts',(51.0240482415051,-42.8168542892489,
-171.64995));
#154353=CARTESIAN_POINT('Ctrl Pts',(51.0922171107721,-42.6180583252229,
-171.649619189927));
#154354=CARTESIAN_POINT('Ctrl Pts',(51.2371844845627,-42.18600352108,-171.638403047895));
#154355=CARTESIAN_POINT('Ctrl Pts',(51.2926025880972,-42.0196813435606,
-171.632782871465));
#154356=CARTESIAN_POINT('Ctrl Pts',(51.385977497022,-41.7369244128409,-171.619483440323));
#154357=CARTESIAN_POINT('Ctrl Pts',(51.4188123620423,-41.6371286285496,
-171.614233886791));
#154358=CARTESIAN_POINT('Ctrl Pts',(51.4706089315109,-41.4791663653461,
-171.604841992257));
#154359=CARTESIAN_POINT('Ctrl Pts',(51.4971436791054,-41.3981183730614,
-171.599766324506));
#154360=CARTESIAN_POINT('Ctrl Pts',(51.5292150542645,-41.2999588202135,
-171.593113195487));
#154361=CARTESIAN_POINT('Ctrl Pts',(51.5455297532666,-41.2499800948475,
-171.58959521104));
#154362=CARTESIAN_POINT('Ctrl Pts',(51.5525816181663,-41.2283682241181,
-171.588045568303));
#154363=CARTESIAN_POINT('Ctrl Pts',(51.5572961698944,-41.2139175755746,
-171.587003052042));
#154364=CARTESIAN_POINT('Ctrl Pts',(51.5601091265564,-41.2052942020437,
-171.586376554727));
#154365=CARTESIAN_POINT('Ctrl Pts',(51.8079906336108,-40.4453081581786,
-171.53088053051));
#154366=CARTESIAN_POINT('Ctrl Pts',(51.9887431992002,-39.8710008464974,
-171.454619407075));
#154367=CARTESIAN_POINT('Ctrl Pts',(52.1126146143194,-39.473850183348,-171.391638125813));
#154368=CARTESIAN_POINT('Origin',(0.,-12.9675000200281,-171.64995));
#154369=CARTESIAN_POINT('',(40.1769968691492,-38.5367831582149,-148.324645026283));
#154370=CARTESIAN_POINT('Ctrl Pts',(52.2951895046066,-38.58067735034,-171.07256826174));
#154371=CARTESIAN_POINT('Ctrl Pts',(51.611967682992,-38.5785901798911,-169.754773540737));
#154372=CARTESIAN_POINT('Ctrl Pts',(50.9382354286579,-38.5764745002471,
-168.460090147878));
#154373=CARTESIAN_POINT('Ctrl Pts',(50.2739302308651,-38.5743305031011,
-167.188544893716));
#154374=CARTESIAN_POINT('Ctrl Pts',(49.5884175161196,-38.5721180602227,
-165.876406373652));
#154375=CARTESIAN_POINT('Ctrl Pts',(48.9129436968084,-38.5698754660624,
-164.588907334074));
#154376=CARTESIAN_POINT('Ctrl Pts',(48.2474886948655,-38.5676040651517,
-163.32604780964));
#154377=CARTESIAN_POINT('Ctrl Pts',(47.5987203612334,-38.5653896209301,
-162.094855216772));
#154378=CARTESIAN_POINT('Ctrl Pts',(46.9594752653591,-38.5631478085241,
-160.887081815245));
#154379=CARTESIAN_POINT('Ctrl Pts',(46.3297741930984,-38.5608808096086,
-159.702700873047));
#154380=CARTESIAN_POINT('Ctrl Pts',(46.3223172763666,-38.5608539638196,
-159.68867544026));
#154381=CARTESIAN_POINT('Ctrl Pts',(46.31576784214,-38.5608303787607,-159.676357433767));
#154382=CARTESIAN_POINT('Ctrl Pts',(46.3074074634252,-38.5608002522641,
-159.660634412727));
#154383=CARTESIAN_POINT('Ctrl Pts',(46.3072537239608,-38.5607996982663,
-159.660345281227));
#154384=CARTESIAN_POINT('Ctrl Pts',(46.3070999849996,-38.5607991442668,
-159.660056150999));
#154385=CARTESIAN_POINT('Ctrl Pts',(46.3069462465417,-38.5607985902656,
-159.65976702204));
#154386=CARTESIAN_POINT('Ctrl Pts',(45.7108946304494,-38.5586507000882,
-158.538799730412));
#154387=CARTESIAN_POINT('Ctrl Pts',(45.1224208024696,-38.5564771811492,
-157.436924140047));
#154388=CARTESIAN_POINT('Ctrl Pts',(44.5414447167035,-38.55427822462,-156.354171396456));
#154389=CARTESIAN_POINT('Ctrl Pts',(43.9496124781868,-38.5520381782619,
-155.251186272456));
#154390=CARTESIAN_POINT('Ctrl Pts',(43.3655609703394,-38.5497717381949,
-154.168045243083));
#154391=CARTESIAN_POINT('Ctrl Pts',(42.7892537562729,-38.5474800295275,
-153.104754637799));
#154392=CARTESIAN_POINT('Ctrl Pts',(42.1951910911732,-38.5451177155995,
-152.008705108427));
#154393=CARTESIAN_POINT('Ctrl Pts',(41.6093573588218,-38.542728554327,-150.933747933629));
#154394=CARTESIAN_POINT('Ctrl Pts',(41.0317614677954,-38.5403147086464,
-149.879863096509));
#154395=CARTESIAN_POINT('Ctrl Pts',(40.744805903117,-38.5391154853468,-149.356282296784));
#154396=CARTESIAN_POINT('Ctrl Pts',(40.45988434067,-38.5379101834035,-148.837902175));
#154397=CARTESIAN_POINT('Ctrl Pts',(40.1770020116941,-38.5366991465431,
-148.324717991527));
#154398=CARTESIAN_POINT('',(40.4124516162331,-44.1531546061648,-155.665156220206));
#154399=CARTESIAN_POINT('Ctrl Pts',(40.1769969654164,-38.5367854529716,
-148.324647842671));
#154400=CARTESIAN_POINT('Ctrl Pts',(40.1948823687306,-38.9631265319537,
-148.847902586266));
#154401=CARTESIAN_POINT('Ctrl Pts',(40.2129052771572,-39.3918670421897,
-149.382496639157));
#154402=CARTESIAN_POINT('Ctrl Pts',(40.2310530620268,-39.8234241172529,
-149.928744356201));
#154403=CARTESIAN_POINT('Ctrl Pts',(40.2392538151749,-40.0184392701975,
-150.175586751426));
#154404=CARTESIAN_POINT('Ctrl Pts',(40.2474800182096,-40.2140300019281,
-150.424808356685));
#154405=CARTESIAN_POINT('Ctrl Pts',(40.2557302446384,-40.410237152229,-150.67643548022));
#154406=CARTESIAN_POINT('Ctrl Pts',(40.2737019599345,-40.8376410634674,
-151.224562378794));
#154407=CARTESIAN_POINT('Ctrl Pts',(40.2917665359898,-41.2674257878512,
-151.783444601094));
#154408=CARTESIAN_POINT('Ctrl Pts',(40.3099131424047,-41.6997961521597,
-152.353294054308));
#154409=CARTESIAN_POINT('Ctrl Pts',(40.326999464829,-42.106903645561,-152.889847901806));
#154410=CARTESIAN_POINT('Ctrl Pts',(40.3441585036013,-42.516303297068,-153.436124940354));
#154411=CARTESIAN_POINT('Ctrl Pts',(40.361378696468,-42.9281717249953,-153.99225788082));
#154412=CARTESIAN_POINT('Ctrl Pts',(40.3783481518696,-43.3340430745853,
-154.540293155664));
#154413=CARTESIAN_POINT('Ctrl Pts',(40.3953770040522,-43.7423116398837,
-155.097899842787));
#154414=CARTESIAN_POINT('Ctrl Pts',(40.4124516185963,-44.1531546492746,
-155.665156176616));
#154415=CARTESIAN_POINT('Ctrl Pts',(40.4124516249929,-44.1531545436406,
-155.665156257244));
#154416=CARTESIAN_POINT('Ctrl Pts',(40.9798621708435,-44.1555773238801,
-156.631664486591));
#154417=CARTESIAN_POINT('Ctrl Pts',(41.5543790914707,-44.1579855398722,
-157.617504781648));
#154418=CARTESIAN_POINT('Ctrl Pts',(42.1359452197555,-44.1603762923632,
-158.622735508298));
#154419=CARTESIAN_POINT('Ctrl Pts',(42.696413965657,-44.1626803159045,-159.59149963899));
#154420=CARTESIAN_POINT('Ctrl Pts',(43.2634297031817,-44.1649681190063,
-160.57827289928));
#154421=CARTESIAN_POINT('Ctrl Pts',(43.8369823248252,-44.167237552928,-161.58308298225));
#154422=CARTESIAN_POINT('Ctrl Pts',(44.4001337756382,-44.1694658314804,
-162.569671195192));
#154423=CARTESIAN_POINT('Ctrl Pts',(44.9695870210121,-44.1716763989756,
-163.57364806962));
#154424=CARTESIAN_POINT('Ctrl Pts',(45.5453744486588,-44.1738676841351,
-164.595014746654));
#154425=CARTESIAN_POINT('Ctrl Pts',(46.1335504926022,-44.1761061168871,
-165.638357102996));
#154426=CARTESIAN_POINT('Ctrl Pts',(46.7283357453045,-44.178324422888,-166.699845913526));
#154427=CARTESIAN_POINT('Ctrl Pts',(47.3298140619878,-44.1805214778239,
-167.779452924363));
#154428=CARTESIAN_POINT('Ctrl Pts',(47.8957945550262,-44.1825888677885,
-168.795344090068));
#154429=CARTESIAN_POINT('Ctrl Pts',(48.4677016046433,-44.1846374429551,
-169.827277858276));
#154430=CARTESIAN_POINT('Ctrl Pts',(49.0456491794116,-44.1866667637444,
-170.875204350381));
#154431=CARTESIAN_POINT('Ctrl Pts',(49.081897568424,-44.1867940410488,-170.940929424419));
#154432=CARTESIAN_POINT('Ctrl Pts',(49.1181697337045,-44.1869212427789,
-171.00671740016));
#154433=CARTESIAN_POINT('Ctrl Pts',(49.1544657093286,-44.1870483688939,
-171.07256826174));
#154434=CARTESIAN_POINT('Ctrl Pts',(39.,-46.9678749402838,-153.612705479043));
#154435=CARTESIAN_POINT('Ctrl Pts',(38.9999999999999,-45.3542560507482,
-154.843289706001));
#154436=CARTESIAN_POINT('Ctrl Pts',(40.4142759901646,-44.1970576517619,
-155.725796787747));
#154437=CARTESIAN_POINT('Ctrl Pts',(39.,-45.668184102287,-151.908469685114));
#154438=CARTESIAN_POINT('Ctrl Pts',(39.,-44.1065443282322,-153.136806613681));
#154439=CARTESIAN_POINT('Ctrl Pts',(40.3630305742695,-42.9636912658246,
-154.021570941673));
#154440=CARTESIAN_POINT('Ctrl Pts',(39.,-44.3354350613925,-150.221485398912));
#154441=CARTESIAN_POINT('Ctrl Pts',(39.0000000000074,-42.8253385188873,
-151.442463829735));
#154442=CARTESIAN_POINT('Ctrl Pts',(40.3100965640753,-41.7031787097929,
-152.33457670764));
#154443=CARTESIAN_POINT('Ctrl Pts',(39.,-41.5900521206853,-146.90520294412));
#154444=CARTESIAN_POINT('Ctrl Pts',(38.9999999999925,-40.1892814621382,
-148.11112464401));
#154445=CARTESIAN_POINT('Ctrl Pts',(40.2013639252015,-39.117295594665,-149.018294252799));
#154446=CARTESIAN_POINT('Ctrl Pts',(39.,-40.1827079235241,-145.281958716849));
#154447=CARTESIAN_POINT('Ctrl Pts',(39.,-38.8402571910301,-146.480210875403));
#154448=CARTESIAN_POINT('Ctrl Pts',(40.1457602981154,-37.7969071359042,
-147.395068273086));
#154449=CARTESIAN_POINT('Ctrl Pts',(39.,-38.728281830342,-143.706077818883));
#154450=CARTESIAN_POINT('Ctrl Pts',(38.9999999999999,-37.4435486267092,
-144.891795278378));
#154451=CARTESIAN_POINT('Ctrl Pts',(40.0893978502897,-36.4387325411231,
-145.819169127587));
#154452=CARTESIAN_POINT('',(39.,-38.78000002,-143.762156710948));
#154453=CARTESIAN_POINT('Ctrl Pts',(40.1769968691492,-38.5367831582149,
-148.324645026283));
#154454=CARTESIAN_POINT('Ctrl Pts',(40.1355273735409,-38.5405885510441,
-148.253998247274));
#154455=CARTESIAN_POINT('Ctrl Pts',(40.0931293305385,-38.5444852864301,
-148.178893064488));
#154456=CARTESIAN_POINT('Ctrl Pts',(40.050116838129,-38.5485760914372,-148.099208883115));
#154457=CARTESIAN_POINT('Ctrl Pts',(40.0079564572523,-38.5525858543579,
-148.02110330847));
#154458=CARTESIAN_POINT('Ctrl Pts',(39.9652058213465,-38.5567825344687,
-147.938597973455));
#154459=CARTESIAN_POINT('Ctrl Pts',(39.9222048827104,-38.5612440999661,
-147.851590185633));
#154460=CARTESIAN_POINT('Ctrl Pts',(39.880442017431,-38.5655772090728,-147.767087506475));
#154461=CARTESIAN_POINT('Ctrl Pts',(39.8384433132321,-38.5701605578681,
-147.678337561074));
#154462=CARTESIAN_POINT('Ctrl Pts',(39.7965596110765,-38.575041557274,-147.585261996377));
#154463=CARTESIAN_POINT('Ctrl Pts',(39.7703977220409,-38.578090384342,-147.527124046047));
#154464=CARTESIAN_POINT('Ctrl Pts',(39.744281479466,-38.581254848957,-147.467298719482));
#154465=CARTESIAN_POINT('Ctrl Pts',(39.718303767535,-38.5845404963934,-147.405771116491));
#154466=CARTESIAN_POINT('Ctrl Pts',(39.6781910428581,-38.589613932859,-147.310765066484));
#154467=CARTESIAN_POINT('Ctrl Pts',(39.6384072401214,-38.59497820995,-147.21169883425));
#154468=CARTESIAN_POINT('Ctrl Pts',(39.5993186657284,-38.60062759641,-147.108536628033));
#154469=CARTESIAN_POINT('Ctrl Pts',(39.5612326590572,-38.6061320839423,
-147.008020389331));
#154470=CARTESIAN_POINT('Ctrl Pts',(39.5238071296623,-38.6119074732402,
-146.903615357461));
#154471=CARTESIAN_POINT('Ctrl Pts',(39.4874039909042,-38.6179142095375,
-146.795314311961));
#154472=CARTESIAN_POINT('Ctrl Pts',(39.4535378615888,-38.623502324056,-146.694560988565));
#154473=CARTESIAN_POINT('Ctrl Pts',(39.4205571104765,-38.6292905412101,
-146.590435817828));
#154474=CARTESIAN_POINT('Ctrl Pts',(39.3887661995631,-38.635216720523,-146.48295663282));
#154475=CARTESIAN_POINT('Ctrl Pts',(39.3719269697633,-38.638355740212,-146.426026313963));
#154476=CARTESIAN_POINT('Ctrl Pts',(39.3554217533661,-38.6415329535104,
-146.368155370693));
#154477=CARTESIAN_POINT('Ctrl Pts',(39.3392966976341,-38.6447354631592,
-146.309349381664));
#154478=CARTESIAN_POINT('Ctrl Pts',(39.3312341697681,-38.6463367179837,
-146.27994638715));
#154479=CARTESIAN_POINT('Ctrl Pts',(39.3232666707404,-38.6479442936562,
-146.250309634084));
#154480=CARTESIAN_POINT('Ctrl Pts',(39.3154000216331,-38.6495562849387,
-146.220440057212));
#154481=CARTESIAN_POINT('Ctrl Pts',(39.3114666970794,-38.65036228058,-146.205505268776));
#154482=CARTESIAN_POINT('Ctrl Pts',(39.307558584028,-38.6511693798373,-146.190512274645));
#154483=CARTESIAN_POINT('Ctrl Pts',(39.3036764077864,-38.6519773352297,
-146.175461199439));
#154484=CARTESIAN_POINT('Ctrl Pts',(39.3017353196656,-38.6523813129259,
-146.167935661836));
#154485=CARTESIAN_POINT('Ctrl Pts',(39.2998007156842,-38.6527855046386,
-146.16039560398));
#154486=CARTESIAN_POINT('Ctrl Pts',(39.2978726865716,-38.6531898783562,
-146.152841042329));
#154487=CARTESIAN_POINT('Ctrl Pts',(39.2959446574589,-38.6535942520737,
-146.145286480678));
#154488=CARTESIAN_POINT('Ctrl Pts',(39.2936380176904,-38.6540802197939,
-146.136191881702));
#154489=CARTESIAN_POINT('Ctrl Pts',(39.2921084144363,-38.654403513146,-146.130133862755));
#154490=CARTESIAN_POINT('Ctrl Pts',(39.2559675721066,-38.6620421567188,
-145.986997459891));
#154491=CARTESIAN_POINT('Ctrl Pts',(39.2232049408543,-38.6699359481944,
-145.843120322114));
#154492=CARTESIAN_POINT('Ctrl Pts',(39.1938520119094,-38.6778211466036,
-145.698765413825));
#154493=CARTESIAN_POINT('Ctrl Pts',(39.1643011830174,-38.6857595076921,
-145.553437252449));
#154494=CARTESIAN_POINT('Ctrl Pts',(39.1382061063453,-38.6936886972171,
-145.407625253192));
#154495=CARTESIAN_POINT('Ctrl Pts',(39.1155464093657,-38.7013467251314,
-145.261596960813));
#154496=CARTESIAN_POINT('Ctrl Pts',(39.0997468350803,-38.706686319082,-145.15977808586));
#154497=CARTESIAN_POINT('Ctrl Pts',(39.0856163027924,-38.7118942339117,
-145.057854041734));
#154498=CARTESIAN_POINT('Ctrl Pts',(39.0731335090665,-38.7168854313741,
-144.9559137805));
#154499=CARTESIAN_POINT('Ctrl Pts',(39.0548053657282,-38.7242138695852,
-144.806237693489));
#154500=CARTESIAN_POINT('Ctrl Pts',(39.0398124881451,-38.7320390883622,
-144.655702496367));
#154501=CARTESIAN_POINT('Ctrl Pts',(39.0282916457397,-38.7400909159274,
-144.504532299893));
#154502=CARTESIAN_POINT('Ctrl Pts',(39.0168061959963,-38.7481180078351,
-144.353826506583));
#154503=CARTESIAN_POINT('Ctrl Pts',(39.0087717144706,-38.756369895014,-144.202489956612));
#154504=CARTESIAN_POINT('Ctrl Pts',(39.004275703363,-38.7645674845392,-144.050760362076));
#154505=CARTESIAN_POINT('Ctrl Pts',(39.001429135968,-38.7697576387672,-143.954695537878));
#154506=CARTESIAN_POINT('Ctrl Pts',(39.0000000038998,-38.7749258178196,
-143.858473458816));
#154507=CARTESIAN_POINT('Ctrl Pts',(39.,-38.78000002,-143.762156710948));
#154508=CARTESIAN_POINT('',(39.,-44.4300000199906,-150.364854264666));
#154509=CARTESIAN_POINT('Ctrl Pts',(39.0000000003644,-44.4300000199906,
-150.364854264666));
#154510=CARTESIAN_POINT('Ctrl Pts',(39.0000000001644,-43.9457023551939,
-149.760761216984));
#154511=CARTESIAN_POINT('Ctrl Pts',(39.000000000108,-43.4567859620687,-149.160174741698));
#154512=CARTESIAN_POINT('Ctrl Pts',(39.0000000000721,-42.9627229131801,
-148.563361289672));
#154513=CARTESIAN_POINT('Ctrl Pts',(39.0000000000298,-42.3819947837034,
-147.861859000803));
#154514=CARTESIAN_POINT('Ctrl Pts',(39.0000000000251,-41.7951037310901,
-147.166651435241));
#154515=CARTESIAN_POINT('Ctrl Pts',(39.000000000019,-41.2007410723715,-146.478263131248));
#154516=CARTESIAN_POINT('Ctrl Pts',(39.0000000000133,-40.6489795609409,
-145.839215294898));
#154517=CARTESIAN_POINT('Ctrl Pts',(39.0000000000093,-40.0907793123645,
-145.206044014069));
#154518=CARTESIAN_POINT('Ctrl Pts',(39.0000000000044,-39.5250612455183,
-144.579200831346));
#154519=CARTESIAN_POINT('Ctrl Pts',(39.0000000000023,-39.2781704674834,
-144.30563381951));
#154520=CARTESIAN_POINT('Ctrl Pts',(39.0000000000002,-39.0298473782612,
-144.033272518869));
#154521=CARTESIAN_POINT('Ctrl Pts',(39.,-38.7800000199999,-143.762156710948));
#154522=CARTESIAN_POINT('Ctrl Pts',(39.0000000003644,-44.4300000199906,
-150.364854264666));
#154523=CARTESIAN_POINT('Ctrl Pts',(39.0000007052026,-44.4254451266292,
-150.452504858533));
#154524=CARTESIAN_POINT('Ctrl Pts',(39.0010202384484,-44.4206877726529,
-150.544931342509));
#154525=CARTESIAN_POINT('Ctrl Pts',(39.0034067297545,-44.4156797092475,
-150.642139337907));
#154526=CARTESIAN_POINT('Ctrl Pts',(39.0057191759491,-44.4108270298623,
-150.736331283407));
#154527=CARTESIAN_POINT('Ctrl Pts',(39.0093152859151,-44.4057385176752,
-150.835012944067));
#154528=CARTESIAN_POINT('Ctrl Pts',(39.0145518042182,-44.4003915136932,
-150.938169957597));
#154529=CARTESIAN_POINT('Ctrl Pts',(39.0154416112397,-44.3994829325689,
-150.955698748607));
#154530=CARTESIAN_POINT('Ctrl Pts',(39.0163788749113,-44.3985669479675,
-150.973356707516));
#154531=CARTESIAN_POINT('Ctrl Pts',(39.0173654574034,-44.397643526823,-150.991143695347));
#154532=CARTESIAN_POINT('Ctrl Pts',(39.0229730021521,-44.3923949790017,
-151.092241506225));
#154533=CARTESIAN_POINT('Ctrl Pts',(39.0301712126243,-44.386903742455,-151.197509750464));
#154534=CARTESIAN_POINT('Ctrl Pts',(39.0393212707034,-44.3811807618817,
-151.306908428555));
#154535=CARTESIAN_POINT('Ctrl Pts',(39.0406017698706,-44.3803798629372,
-151.322218158282));
#154536=CARTESIAN_POINT('Ctrl Pts',(39.0419205457929,-44.379574476212,-151.337608737534));
#154537=CARTESIAN_POINT('Ctrl Pts',(39.0432786373157,-44.3787646832776,
-151.353080013601));
#154538=CARTESIAN_POINT('Ctrl Pts',(39.0488099378183,-44.3754665196488,
-151.416092171215));
#154539=CARTESIAN_POINT('Ctrl Pts',(39.0549931721796,-44.3720949468472,
-151.480443195579));
#154540=CARTESIAN_POINT('Ctrl Pts',(39.0619004408812,-44.3686579749138,
-151.54612071821));
#154541=CARTESIAN_POINT('Ctrl Pts',(39.0653540752321,-44.3669394889471,
-151.578959479526));
#154542=CARTESIAN_POINT('Ctrl Pts',(39.0689887775362,-44.3652046607912,
-151.612129859391));
#154543=CARTESIAN_POINT('Ctrl Pts',(39.0728138179726,-44.363454962206,-151.645629929068));
#154544=CARTESIAN_POINT('Ctrl Pts',(39.0747263381908,-44.3625801129134,
-151.662379963907));
#154545=CARTESIAN_POINT('Ctrl Pts',(39.0766864464293,-44.3617015464156,
-151.679212420879));
#154546=CARTESIAN_POINT('Ctrl Pts',(39.0786953190885,-44.3608194643872,
-151.696127044875));
#154547=CARTESIAN_POINT('Ctrl Pts',(39.0796997554181,-44.3603784233729,
-151.704584356872));
#154548=CARTESIAN_POINT('Ctrl Pts',(39.080716383072,-44.3599365035074,-151.713062210601));
#154549=CARTESIAN_POINT('Ctrl Pts',(39.0817453500286,-44.3594937318188,
-151.721560572708));
#154550=CARTESIAN_POINT('Ctrl Pts',(39.0827743169852,-44.3590509601302,
-151.730058934815));
#154551=CARTESIAN_POINT('Ctrl Pts',(39.0839942168393,-44.3585320129597,
-151.740025025291));
#154552=CARTESIAN_POINT('Ctrl Pts',(39.0848694175268,-44.3581628889547,
-151.747117150299));
#154553=CARTESIAN_POINT('Ctrl Pts',(39.105124915675,-44.3496199447983,-151.911256103819));
#154554=CARTESIAN_POINT('Ctrl Pts',(39.1291136383777,-44.3407950403259,
-152.075349215586));
#154555=CARTESIAN_POINT('Ctrl Pts',(39.1568906940477,-44.3319910570048,
-152.239164594126));
#154556=CARTESIAN_POINT('Ctrl Pts',(39.1675198003644,-44.3286221443367,
-152.301849822377));
#154557=CARTESIAN_POINT('Ctrl Pts',(39.1787031089135,-44.3252564505626,
-152.364494303024));
#154558=CARTESIAN_POINT('Ctrl Pts',(39.190441757935,-44.321911449593,-152.427084805163));
#154559=CARTESIAN_POINT('Ctrl Pts',(39.211649394889,-44.3158682016823,-152.540163971575));
#154560=CARTESIAN_POINT('Ctrl Pts',(39.2346703636018,-44.3098924130758,
-152.653066963499));
#154561=CARTESIAN_POINT('Ctrl Pts',(39.2595020395869,-44.3040887056269,
-152.765715249301));
#154562=CARTESIAN_POINT('Ctrl Pts',(39.2719178775795,-44.3011868519025,
-152.822039392202));
#154563=CARTESIAN_POINT('Ctrl Pts',(39.2847862305988,-44.2983279746361,
-152.878299892895));
#154564=CARTESIAN_POINT('Ctrl Pts',(39.298105589975,-44.2955253459415,-152.934486886189));
#154565=CARTESIAN_POINT('Ctrl Pts',(39.3047652696632,-44.2941240315943,
-152.962580382836));
#154566=CARTESIAN_POINT('Ctrl Pts',(39.311537690051,-44.2927367766557,-152.990655504777));
#154567=CARTESIAN_POINT('Ctrl Pts',(39.3184225947996,-44.2913652303238,
-153.018711029337));
#154568=CARTESIAN_POINT('Ctrl Pts',(39.3218650471739,-44.2906794571578,
-153.032738791617));
#154569=CARTESIAN_POINT('Ctrl Pts',(39.3253356199727,-44.2899976109454,
-153.046761654706));
#154570=CARTESIAN_POINT('Ctrl Pts',(39.3288342765372,-44.2893198980638,
-153.060779465937));
#154571=CARTESIAN_POINT('Ctrl Pts',(39.3305836048194,-44.2889810416229,
-153.067788371552));
#154572=CARTESIAN_POINT('Ctrl Pts',(39.3323399540012,-44.2886432185021,
-153.074796014213));
#154573=CARTESIAN_POINT('Ctrl Pts',(39.3341033192103,-44.2883064545096,
-153.081802374849));
#154574=CARTESIAN_POINT('Ctrl Pts',(39.3358666844194,-44.2879696905171,
-153.088808735485));
#154575=CARTESIAN_POINT('Ctrl Pts',(39.337254200393,-44.2877060656016,-153.094305141372));
#154576=CARTESIAN_POINT('Ctrl Pts',(39.3394144578684,-44.2872993656993,
-153.102817591642));
#154577=CARTESIAN_POINT('Ctrl Pts',(39.3748573788217,-44.2806267201212,
-153.242479694645));
#154578=CARTESIAN_POINT('Ctrl Pts',(39.412489111862,-44.2738186133137,-153.378383004324));
#154579=CARTESIAN_POINT('Ctrl Pts',(39.4519769629075,-44.2670316716111,
-153.510443256863));
#154580=CARTESIAN_POINT('Ctrl Pts',(39.4918829156408,-44.260172869027,-153.643901777807));
#154581=CARTESIAN_POINT('Ctrl Pts',(39.5336838923085,-44.2533356595528,
-153.773435489427));
#154582=CARTESIAN_POINT('Ctrl Pts',(39.5770317524979,-44.2466382972547,
-153.898989281955));
#154583=CARTESIAN_POINT('Ctrl Pts',(39.6212491945741,-44.2398065821899,
-154.027061752529));
#154584=CARTESIAN_POINT('Ctrl Pts',(39.6670756075795,-44.2331203235828,
-154.150993109346));
#154585=CARTESIAN_POINT('Ctrl Pts',(39.7141457934817,-44.2266606244434,
-154.270756794082));
#154586=CARTESIAN_POINT('Ctrl Pts',(39.7533855876433,-44.2212755328039,
-154.370597112257));
#154587=CARTESIAN_POINT('Ctrl Pts',(39.7934897051191,-44.216047010482,-154.46754169698));
#154588=CARTESIAN_POINT('Ctrl Pts',(39.8342530369782,-44.2110000715016,
-154.561590642464));
#154589=CARTESIAN_POINT('Ctrl Pts',(39.8848733950829,-44.2047327266387,
-154.678381667206));
#154590=CARTESIAN_POINT('Ctrl Pts',(39.9365093609633,-44.198746358527,-154.790706718198));
#154591=CARTESIAN_POINT('Ctrl Pts',(39.9887873165752,-44.1930504805605,
-154.898592431591));
#154592=CARTESIAN_POINT('Ctrl Pts',(40.0418796117349,-44.1872658772674,
-155.008158692779));
#154593=CARTESIAN_POINT('Ctrl Pts',(40.0956336285611,-44.1817805384754,
-155.113146519742));
#154594=CARTESIAN_POINT('Ctrl Pts',(40.1496863776524,-44.1765656542448,
-155.213609846438));
#154595=CARTESIAN_POINT('Ctrl Pts',(40.2051589771905,-44.1712137861266,
-155.31671213048));
#154596=CARTESIAN_POINT('Ctrl Pts',(40.2609458166902,-44.1661464111464,
-155.41504938527));
#154597=CARTESIAN_POINT('Ctrl Pts',(40.3166905863262,-44.161297194854,-155.508702734244));
#154598=CARTESIAN_POINT('Ctrl Pts',(40.3486445042757,-44.1585175356943,
-155.562386540784));
#154599=CARTESIAN_POINT('Ctrl Pts',(40.3805852951185,-44.1558089457943,
-155.61453170595));
#154600=CARTESIAN_POINT('Ctrl Pts',(40.4124516185963,-44.1531546492747,
-155.665156176616));
#154601=CARTESIAN_POINT('Origin',(39.,46.91999998,-129.34995));
#154602=CARTESIAN_POINT('',(39.,-38.78000002,-88.296486260558));
#154603=CARTESIAN_POINT('',(39.,-38.78000002,-129.34995));
#154604=CARTESIAN_POINT('',(39.,-44.43000002,-81.6937887068282));
#154605=CARTESIAN_POINT('Ctrl Pts',(39.,-38.7800000199999,-88.296486260558));
#154606=CARTESIAN_POINT('Ctrl Pts',(39.0000000000004,-39.3488675990358,
-87.6791933887682));
#154607=CARTESIAN_POINT('Ctrl Pts',(39.0000000000079,-39.9098343204423,
-87.055447933963));
#154608=CARTESIAN_POINT('Ctrl Pts',(39.0000000000125,-40.4639767641308,
-86.4257067262392));
#154609=CARTESIAN_POINT('Ctrl Pts',(39.0000000000174,-41.0582242765816,
-85.7503891243484));
#154610=CARTESIAN_POINT('Ctrl Pts',(39.0000000000199,-41.6446237826245,
-85.0681763071684));
#154611=CARTESIAN_POINT('Ctrl Pts',(39.0000000000371,-42.2244596705921,
-84.3795886419069));
#154612=CARTESIAN_POINT('Ctrl Pts',(39.0000000000444,-42.4717173644025,
-84.0859562510322));
#154613=CARTESIAN_POINT('Ctrl Pts',(39.0000000000547,-42.7177810382159,
-83.7911641691294));
#154614=CARTESIAN_POINT('Ctrl Pts',(39.0000000000728,-42.9627483114232,
-83.4952507849665));
#154615=CARTESIAN_POINT('Ctrl Pts',(39.0000000001092,-43.4568057616665,
-82.8984436680065));
#154616=CARTESIAN_POINT('Ctrl Pts',(39.0000000001663,-43.9457116736055,
-82.2978701296066));
#154617=CARTESIAN_POINT('Ctrl Pts',(39.0000000003688,-44.43000002,-81.6937887068282));
#154618=CARTESIAN_POINT('',(39.,-44.43000002,-129.34995));
#154619=CARTESIAN_POINT('Ctrl Pts',(40.4142759779013,-44.1970573566106,
-76.3328465915894));
#154620=CARTESIAN_POINT('Ctrl Pts',(39.,-45.3542557512738,-77.2153536750926));
#154621=CARTESIAN_POINT('Ctrl Pts',(39.,-46.9678746292626,-78.4459379002929));
#154622=CARTESIAN_POINT('Ctrl Pts',(40.3630303964688,-42.9636869888089,
-78.0370779308685));
#154623=CARTESIAN_POINT('Ctrl Pts',(39.,-44.1065399853887,-78.9218422882493));
#154624=CARTESIAN_POINT('Ctrl Pts',(39.,-45.6681795295713,-80.1501792727118));
#154625=CARTESIAN_POINT('Ctrl Pts',(40.3100980841279,-41.7032148714377,
-79.7240190083239));
#154626=CARTESIAN_POINT('Ctrl Pts',(39.0000000000075,-42.8253754175223,
-80.6161315734671));
#154627=CARTESIAN_POINT('Ctrl Pts',(39.,-44.3354733849924,-81.8371103170565));
#154628=CARTESIAN_POINT('Ctrl Pts',(40.2013644254228,-39.117307479239,-83.0403343570498));
#154629=CARTESIAN_POINT('Ctrl Pts',(38.9999999999925,-40.1892936959721,
-83.9475037984034));
#154630=CARTESIAN_POINT('Ctrl Pts',(39.,-41.5900648068412,-85.1534256657242));
#154631=CARTESIAN_POINT('Ctrl Pts',(40.1457604305377,-37.7969103286269,
-84.6635709993291));
#154632=CARTESIAN_POINT('Ctrl Pts',(39.0000000000224,-38.8402604870948,
-85.5784283533127));
#154633=CARTESIAN_POINT('Ctrl Pts',(39.,-40.1827113458493,-86.7766805524391));
#154634=CARTESIAN_POINT('Ctrl Pts',(40.0893978453286,-36.4387324215761,
-86.2394739826303));
#154635=CARTESIAN_POINT('Ctrl Pts',(38.9999999999999,-37.4435485041586,
-87.1668478324999));
#154636=CARTESIAN_POINT('Ctrl Pts',(39.,-38.7282817023213,-88.3525652913338));
#154637=CARTESIAN_POINT('',(40.1769830712292,-38.5367008846094,-83.7339572460004));
#154638=CARTESIAN_POINT('Ctrl Pts',(39.,-38.78000002,-88.296486260558));
#154639=CARTESIAN_POINT('Ctrl Pts',(39.,-38.7751322708569,-88.2040883348799));
#154640=CARTESIAN_POINT('Ctrl Pts',(39.0012719050489,-38.770015943568,-88.1070513397817));
#154641=CARTESIAN_POINT('Ctrl Pts',(39.0042443556417,-38.7646505825313,
-88.0053892224477));
#154642=CARTESIAN_POINT('Ctrl Pts',(39.006951468088,-38.7597641646792,-87.9128020541979));
#154643=CARTESIAN_POINT('Ctrl Pts',(39.0110696448286,-38.7546711367464,
-87.8163776816512));
#154644=CARTESIAN_POINT('Ctrl Pts',(39.0169597134217,-38.7493716191513,
-87.7161359772685));
#154645=CARTESIAN_POINT('Ctrl Pts',(39.0225041669748,-38.7443830644857,
-87.621776214686));
#154646=CARTESIAN_POINT('Ctrl Pts',(39.0296189198416,-38.7392117734668,
-87.5240383765513));
#154647=CARTESIAN_POINT('Ctrl Pts',(39.0386310058382,-38.7338594124382,
-87.4229686929037));
#154648=CARTESIAN_POINT('Ctrl Pts',(39.0431370488365,-38.731183231924,-87.3724338510799));
#154649=CARTESIAN_POINT('Ctrl Pts',(39.0481177945266,-38.7284618151407,
-87.3210666362513));
#154650=CARTESIAN_POINT('Ctrl Pts',(39.0536162553258,-38.7256955139037,
-87.2688755073787));
#154651=CARTESIAN_POINT('Ctrl Pts',(39.0563654857254,-38.7243123632852,
-87.2427799429424));
#154652=CARTESIAN_POINT('Ctrl Pts',(39.0592441664584,-38.7229179928732,
-87.2164784244485));
#154653=CARTESIAN_POINT('Ctrl Pts',(39.0622577885059,-38.7215124585059,
-87.1899722295901));
#154654=CARTESIAN_POINT('Ctrl Pts',(39.0630111940177,-38.721161074914,-87.1833456808756));
#154655=CARTESIAN_POINT('Ctrl Pts',(39.0637730337606,-38.7208089935898,
-87.1767063401531));
#154656=CARTESIAN_POINT('Ctrl Pts',(39.0645433942633,-38.7204562154624,
-87.1700542284318));
#154657=CARTESIAN_POINT('Ctrl Pts',(39.0651211646403,-38.7201916318669,
-87.1650651446408));
#154658=CARTESIAN_POINT('Ctrl Pts',(39.0657037279515,-38.7199266563198,
-87.1600688771641));
#154659=CARTESIAN_POINT('Ctrl Pts',(39.0662911208221,-38.7196612892144,
-87.1550654348854));
#154660=CARTESIAN_POINT('Ctrl Pts',(39.0664133853009,-38.71960605366,-87.1540239798509));
#154661=CARTESIAN_POINT('Ctrl Pts',(39.0665355793354,-38.7195509271128,
-87.1529845890894));
#154662=CARTESIAN_POINT('Ctrl Pts',(39.0666586113654,-38.7194955005559,
-87.1519395508262));
#154663=CARTESIAN_POINT('Ctrl Pts',(39.0680442608999,-38.718871258374,-87.1401697963779));
#154664=CARTESIAN_POINT('Ctrl Pts',(39.0696269835109,-38.7181701779564,
-87.1269526878292));
#154665=CARTESIAN_POINT('Ctrl Pts',(39.07096982888,-38.7175841665058,-87.1159059528804));
#154666=CARTESIAN_POINT('Ctrl Pts',(39.071226215998,-38.7174722803643,-87.1137968190948));
#154667=CARTESIAN_POINT('Ctrl Pts',(39.0714737027787,-38.7173645880403,
-87.1117667787753));
#154668=CARTESIAN_POINT('Ctrl Pts',(39.0717090468188,-38.7172624241003,
-87.1098409798219));
#154669=CARTESIAN_POINT('Ctrl Pts',(39.0875044445527,-38.7104055686412,
-86.9805886715101));
#154670=CARTESIAN_POINT('Ctrl Pts',(39.1060041069199,-38.7033702850715,
-86.8512458769073));
#154671=CARTESIAN_POINT('Ctrl Pts',(39.1272339734381,-38.6963344387826,
-86.7219659415845));
#154672=CARTESIAN_POINT('Ctrl Pts',(39.1378819023615,-38.6928055804575,
-86.6571250457942));
#154673=CARTESIAN_POINT('Ctrl Pts',(39.1492158695168,-38.6892762956135,
-86.592299827051));
#154674=CARTESIAN_POINT('Ctrl Pts',(39.1612346902753,-38.6857671564475,
-86.5275086253275));
#154675=CARTESIAN_POINT('Ctrl Pts',(39.170230183961,-38.6831407391106,-86.4790156111036));
#154676=CARTESIAN_POINT('Ctrl Pts',(39.1796091474621,-38.6805260462456,
-86.4305417811094));
#154677=CARTESIAN_POINT('Ctrl Pts',(39.1893697299427,-38.6779321756499,
-86.3820948719549));
#154678=CARTESIAN_POINT('Ctrl Pts',(39.1991303124233,-38.6753383050542,
-86.3336479628005));
#154679=CARTESIAN_POINT('Ctrl Pts',(39.2092725094359,-38.672765261147,-86.2852279785019));
#154680=CARTESIAN_POINT('Ctrl Pts',(39.2197935457867,-38.6702217598244,
-86.2368423218951));
#154681=CARTESIAN_POINT('Ctrl Pts',(39.2303145821375,-38.6676782585017,
-86.1884566652882));
#154682=CARTESIAN_POINT('Ctrl Pts',(39.2412144573617,-38.6651642995807,
-86.1401053366775));
#154683=CARTESIAN_POINT('Ctrl Pts',(39.2524893947787,-38.6626885282162,
-86.0917955706138));
#154684=CARTESIAN_POINT('Ctrl Pts',(39.2581268634872,-38.6614506425339,
-86.067640687582));
#154685=CARTESIAN_POINT('Ctrl Pts',(39.2638580840871,-38.6602222971366,
-86.0434961893031));
#154686=CARTESIAN_POINT('Ctrl Pts',(39.2696825029684,-38.6590045387141,
-86.0193629463918));
#154687=CARTESIAN_POINT('Ctrl Pts',(39.272594712409,-38.6583956595029,-86.0072963249361));
#154688=CARTESIAN_POINT('Ctrl Pts',(39.2755302206201,-38.6577894266009,
-85.9952325169264));
#154689=CARTESIAN_POINT('Ctrl Pts',(39.2784889532421,-38.6571859693317,
-85.983171629405));
#154690=CARTESIAN_POINT('Ctrl Pts',(39.2799683195532,-38.6568842406971,
-85.9771411856443));
#154691=CARTESIAN_POINT('Ctrl Pts',(39.2814534919182,-38.6565832059434,
-85.9711114719805));
#154692=CARTESIAN_POINT('Ctrl Pts',(39.2829444607249,-38.6562828811408,
-85.9650825016789));
#154693=CARTESIAN_POINT('Ctrl Pts',(39.2842286592038,-38.6560242059406,
-85.959889640195));
#154694=CARTESIAN_POINT('Ctrl Pts',(39.2852757225972,-38.6558141697005,
-85.9556680182126));
#154695=CARTESIAN_POINT('Ctrl Pts',(39.2867135640682,-38.6555118292067,
-85.9499104143363));
#154696=CARTESIAN_POINT('Ctrl Pts',(39.2869450726374,-38.6554631490033,
-85.9489833756727));
#154697=CARTESIAN_POINT('Ctrl Pts',(39.2871867538787,-38.6554120757498,
-85.9480165163723));
#154698=CARTESIAN_POINT('Ctrl Pts',(39.2874412782136,-38.6553580214243,
-85.9469993764742));
#154699=CARTESIAN_POINT('Ctrl Pts',(39.3168062531781,-38.6491216671837,
-85.8296499385384));
#154700=CARTESIAN_POINT('Ctrl Pts',(39.347813897775,-38.6430183085598,-85.7153946198998));
#154701=CARTESIAN_POINT('Ctrl Pts',(39.3802038090334,-38.6370773642453,
-85.6042576441525));
#154702=CARTESIAN_POINT('Ctrl Pts',(39.4044962424771,-38.6326216560094,
-85.5209049123421));
#154703=CARTESIAN_POINT('Ctrl Pts',(39.4295662524833,-38.6282571384398,
-85.4393063176715));
#154704=CARTESIAN_POINT('Ctrl Pts',(39.4553071010921,-38.6239848770771,
-85.3594741229853));
#154705=CARTESIAN_POINT('Ctrl Pts',(39.4939183740053,-38.6175764850329,
-85.239725830956));
#154706=CARTESIAN_POINT('Ctrl Pts',(39.5340443755693,-38.6113746546872,
-85.1239378544272));
#154707=CARTESIAN_POINT('Ctrl Pts',(39.5753182817589,-38.6053655234179,
-85.0121853429442));
#154708=CARTESIAN_POINT('Ctrl Pts',(39.6165921879486,-38.5993563921486,
-84.9004328314613));
#154709=CARTESIAN_POINT('Ctrl Pts',(39.659013902461,-38.5935399471999,-84.7927151573769));
#154710=CARTESIAN_POINT('Ctrl Pts',(39.7022266257688,-38.587902347965,-84.6890544727167));
#154711=CARTESIAN_POINT('Ctrl Pts',(39.7486087077317,-38.5818512692602,
-84.5777909835356));
#154712=CARTESIAN_POINT('Ctrl Pts',(39.7958609030512,-38.576108580013,-84.4711866585353));
#154713=CARTESIAN_POINT('Ctrl Pts',(39.8435692192616,-38.5706418472248,
-84.3691732753572));
#154714=CARTESIAN_POINT('Ctrl Pts',(39.8748801633873,-38.5670540332235,
-84.3022219428749));
#154715=CARTESIAN_POINT('Ctrl Pts',(39.9063880806255,-38.5635851184899,
-84.2372469507177));
#154716=CARTESIAN_POINT('Ctrl Pts',(39.937981857019,-38.5602263972235,-84.1742185506446));
#154717=CARTESIAN_POINT('Ctrl Pts',(39.9905251860152,-38.5546405377075,
-84.0693965781175));
#154718=CARTESIAN_POINT('Ctrl Pts',(40.043308659147,-38.5493483797232,-83.9699663358905));
#154719=CARTESIAN_POINT('Ctrl Pts',(40.0958052372803,-38.5443134355034,
-83.8758305147684));
#154720=CARTESIAN_POINT('Ctrl Pts',(40.122964392795,-38.5417086022374,-83.8271292565859));
#154721=CARTESIAN_POINT('Ctrl Pts',(40.1500471338584,-38.5391726650493,
-83.7798442200289));
#154722=CARTESIAN_POINT('Ctrl Pts',(40.1769830712292,-38.5367008846094,
-83.7339572460004));
#154723=CARTESIAN_POINT('',(40.4124515952943,-44.1531546081811,-76.3934867324882));
#154724=CARTESIAN_POINT('Ctrl Pts',(40.4124516186295,-44.153154649867,-76.3934867953418));
#154725=CARTESIAN_POINT('Ctrl Pts',(40.3952460398817,-43.7391604247703,
-76.9650940777494));
#154726=CARTESIAN_POINT('Ctrl Pts',(40.3780870787012,-43.3277837645271,
-77.5268985486059));
#154727=CARTESIAN_POINT('Ctrl Pts',(40.3609885419993,-42.9188402155611,
-78.0789845047923));
#154728=CARTESIAN_POINT('Ctrl Pts',(40.3428805261513,-42.4857530809918,
-78.6636650197566));
#154729=CARTESIAN_POINT('Ctrl Pts',(40.3248402889955,-42.055395000472,-79.2374457299862));
#154730=CARTESIAN_POINT('Ctrl Pts',(40.3068810516774,-41.6275578066968,
-79.8004867094309));
#154731=CARTESIAN_POINT('Ctrl Pts',(40.2897545069958,-41.2195575845354,
-80.3374218988947));
#154732=CARTESIAN_POINT('Ctrl Pts',(40.2727015872578,-40.8138501719484,
-80.8645911001279));
#154733=CARTESIAN_POINT('Ctrl Pts',(40.2557312547753,-40.4102611753384,
-81.3821766826868));
#154734=CARTESIAN_POINT('Ctrl Pts',(40.2374822795637,-39.97626345594,-81.9387601483187));
#154735=CARTESIAN_POINT('Ctrl Pts',(40.2193511533291,-39.5452803790655,
-82.4835699879066));
#154736=CARTESIAN_POINT('Ctrl Pts',(40.2013522628222,-39.1168809520225,
-83.0169014070057));
#154737=CARTESIAN_POINT('Ctrl Pts',(40.193206439655,-38.9229986693181,-83.258273141993));
#154738=CARTESIAN_POINT('Ctrl Pts',(40.1850876474775,-38.7296460713902,
-83.4972944027484));
#154739=CARTESIAN_POINT('Ctrl Pts',(40.1769969653824,-38.5367854415877,
-83.7339951195581));
#154740=CARTESIAN_POINT('Ctrl Pts',(40.4124516068581,-44.1531545451511,
-76.3934867430719));
#154741=CARTESIAN_POINT('Ctrl Pts',(40.3510699177843,-44.158267238669,-76.4910005227811));
#154742=CARTESIAN_POINT('Ctrl Pts',(40.2897374695193,-44.1636365976902,
-76.5934241275335));
#154743=CARTESIAN_POINT('Ctrl Pts',(40.2289388806379,-44.1692681835667,
-76.7008689731916));
#154744=CARTESIAN_POINT('Ctrl Pts',(40.1815905139172,-44.1736539168247,
-76.784544236846));
#154745=CARTESIAN_POINT('Ctrl Pts',(40.1345654049276,-44.178198675974,-76.8712646231758));
#154746=CARTESIAN_POINT('Ctrl Pts',(40.0880717165451,-44.1829046417643,
-76.9610747878389));
#154747=CARTESIAN_POINT('Ctrl Pts',(40.0366336021373,-44.1881110690267,
-77.0604359201913));
#154748=CARTESIAN_POINT('Ctrl Pts',(39.9858518633865,-44.1935143925675,
-77.1635711601288));
#154749=CARTESIAN_POINT('Ctrl Pts',(39.9359915641101,-44.199114610184,-77.2704856845705));
#154750=CARTESIAN_POINT('Ctrl Pts',(39.8861312648337,-44.2047148278006,
-77.3774002090122));
#154751=CARTESIAN_POINT('Ctrl Pts',(39.837193200328,-44.2105119454377,-77.4880941304441));
#154752=CARTESIAN_POINT('Ctrl Pts',(39.7893996906518,-44.2165040019749,
-77.6025360228382));
#154753=CARTESIAN_POINT('Ctrl Pts',(39.7863162384146,-44.2168905862676,
-77.6099193707346));
#154754=CARTESIAN_POINT('Ctrl Pts',(39.7824541929345,-44.2173769096022,
-77.6192077850968));
#154755=CARTESIAN_POINT('Ctrl Pts',(39.7801635931124,-44.2176662577561,
-77.6247328089195));
#154756=CARTESIAN_POINT('Ctrl Pts',(39.7787661541334,-44.2178427819944,
-77.6281034909458));
#154757=CARTESIAN_POINT('Ctrl Pts',(39.777367957483,-44.2180196929799,-77.6314816136799));
#154758=CARTESIAN_POINT('Ctrl Pts',(39.775969023752,-44.2181969908901,-77.6348671799205));
#154759=CARTESIAN_POINT('Ctrl Pts',(39.7180520552975,-44.225537265303,-77.7750323134183));
#154760=CARTESIAN_POINT('Ctrl Pts',(39.6589014044892,-44.2335417463499,
-77.9279743185955));
#154761=CARTESIAN_POINT('Ctrl Pts',(39.6002641254276,-44.2422288610516,
-78.0940075633862));
#154762=CARTESIAN_POINT('Ctrl Pts',(39.5860275451542,-44.2443380108582,
-78.1343188748137));
#154763=CARTESIAN_POINT('Ctrl Pts',(39.5718214669483,-44.2464874033966,
-78.1754019794697));
#154764=CARTESIAN_POINT('Ctrl Pts',(39.5576712214515,-44.2486773058874,
-78.2172615215681));
#154765=CARTESIAN_POINT('Ctrl Pts',(39.5182563748059,-44.2547771767953,
-78.3338593171923));
#154766=CARTESIAN_POINT('Ctrl Pts',(39.4792798091834,-44.2611901671226,
-78.4564714249827));
#154767=CARTESIAN_POINT('Ctrl Pts',(39.4413055250383,-44.2679169956396,
-78.5851235840438));
#154768=CARTESIAN_POINT('Ctrl Pts',(39.4103620351911,-44.273398377438,-78.6899562851032));
#154769=CARTESIAN_POINT('Ctrl Pts',(39.3800846623711,-44.2790880796353,
-78.7987983155533));
#154770=CARTESIAN_POINT('Ctrl Pts',(39.3507730694842,-44.2849849651986,
-78.9116354894448));
#154771=CARTESIAN_POINT('Ctrl Pts',(39.3486671601221,-44.2854086305573,
-78.9197423453843));
#154772=CARTESIAN_POINT('Ctrl Pts',(39.3462781123095,-44.2858919006434,
-78.9289899433011));
#154773=CARTESIAN_POINT('Ctrl Pts',(39.344470382315,-44.2862592024284,-78.9360178765697));
#154774=CARTESIAN_POINT('Ctrl Pts',(39.3433176190757,-44.2864934254578,
-78.9404994878422));
#154775=CARTESIAN_POINT('Ctrl Pts',(39.3421676157945,-44.2867279189475,
-78.9449823374088));
#154776=CARTESIAN_POINT('Ctrl Pts',(39.3410203725809,-44.2869626764882,
-78.9494664233533));
#154777=CARTESIAN_POINT('Ctrl Pts',(39.3046430590299,-44.2944064761663,
-79.0916498753526));
#154778=CARTESIAN_POINT('Ctrl Pts',(39.2711308927383,-44.3020903706652,
-79.2345947225894));
#154779=CARTESIAN_POINT('Ctrl Pts',(39.240557058843,-44.3098085083895,-79.3781902552231));
#154780=CARTESIAN_POINT('Ctrl Pts',(39.2237092792686,-44.3140616054511,
-79.4573188947637));
#154781=CARTESIAN_POINT('Ctrl Pts',(39.2077529091826,-44.3183251085781,
-79.5366446976344));
#154782=CARTESIAN_POINT('Ctrl Pts',(39.1926939224873,-44.3225650371283,
-79.6161466581915));
#154783=CARTESIAN_POINT('Ctrl Pts',(39.1818817918178,-44.3256092433848,
-79.673227895025));
#154784=CARTESIAN_POINT('Ctrl Pts',(39.1715328096908,-44.3286406374731,
-79.73039721567));
#154785=CARTESIAN_POINT('Ctrl Pts',(39.1616480262631,-44.3316460088623,
-79.7876447784984));
#154786=CARTESIAN_POINT('Ctrl Pts',(39.1517632428354,-44.3346513802515,
-79.8448923413267));
#154787=CARTESIAN_POINT('Ctrl Pts',(39.1423426585283,-44.3376307202623,
-79.9022181402485));
#154788=CARTESIAN_POINT('Ctrl Pts',(39.1333861528049,-44.3405704642751,
-79.9596120521454));
#154789=CARTESIAN_POINT('Ctrl Pts',(39.1230624498265,-44.3439589558317,
-80.0257670591857));
#154790=CARTESIAN_POINT('Ctrl Pts',(39.1132917639146,-44.3473158048929,
-80.0924491279359));
#154791=CARTESIAN_POINT('Ctrl Pts',(39.1041771551082,-44.35064350333,-80.158887585486));
#154792=CARTESIAN_POINT('Ctrl Pts',(39.0974766932732,-44.3530898086899,
-80.2077287764401));
#154793=CARTESIAN_POINT('Ctrl Pts',(39.0911296815406,-44.3555203400116,
-80.2564381655058));
#154794=CARTESIAN_POINT('Ctrl Pts',(39.0851592100358,-44.3579356581365,
-80.3047076554924));
#154795=CARTESIAN_POINT('Ctrl Pts',(39.0710671323645,-44.3636365228988,
-80.4186379207139));
#154796=CARTESIAN_POINT('Ctrl Pts',(39.0586668014923,-44.3696038383643,
-80.5331343405056));
#154797=CARTESIAN_POINT('Ctrl Pts',(39.0480243009804,-44.3755933655321,
-80.6481162160745));
#154798=CARTESIAN_POINT('Ctrl Pts',(39.0400424255965,-44.3800855109081,
-80.7343526227512));
#154799=CARTESIAN_POINT('Ctrl Pts',(39.03304753109,-44.3845906292611,-80.8208617423929));
#154800=CARTESIAN_POINT('Ctrl Pts',(39.0270467496741,-44.3891067880273,
-80.9076077919212));
#154801=CARTESIAN_POINT('Ctrl Pts',(39.0130892771956,-44.399611113601,-81.1093741145068));
#154802=CARTESIAN_POINT('Ctrl Pts',(39.0045137146899,-44.4101748983392,
-81.3124170949888));
#154803=CARTESIAN_POINT('Ctrl Pts',(39.0013677367083,-44.4207753411466,
-81.5163151311992));
#154804=CARTESIAN_POINT('Ctrl Pts',(39.0004560331356,-44.42384734662,-81.5754047272333));
#154805=CARTESIAN_POINT('Ctrl Pts',(39.,-44.426922427187,-81.6345660607426));
#154806=CARTESIAN_POINT('Ctrl Pts',(39.,-44.43000002,-81.6937887068282));
#154807=CARTESIAN_POINT('Origin',(60.,-2.55003103885676E-14,0.));
#154808=CARTESIAN_POINT('',(60.,19.76999998,-58.24995));
#154809=CARTESIAN_POINT('',(60.,19.26999998,-58.24995));
#154810=CARTESIAN_POINT('',(60.,-54.58000002,-58.24995));
#154811=CARTESIAN_POINT('',(60.,19.26999998,-174.34995));
#154812=CARTESIAN_POINT('',(60.,19.26999998,-174.34995));
#154813=CARTESIAN_POINT('',(60.,19.76999998,-174.34995));
#154814=CARTESIAN_POINT('',(60.,28.41999998,-174.34995));
#154815=CARTESIAN_POINT('',(60.,19.76999998,-58.24995));
#154816=CARTESIAN_POINT('Origin',(57.,-2.42462934179819E-14,-174.34995));
#154817=CARTESIAN_POINT('',(57.,19.26999998,-177.34995));
#154818=CARTESIAN_POINT('Origin',(57.,19.26999998,-174.34995));
#154819=CARTESIAN_POINT('',(57.,19.76999998,-177.34995));
#154820=CARTESIAN_POINT('',(57.,-54.58000002,-177.34995));
#154821=CARTESIAN_POINT('Origin',(57.,19.76999998,-174.34995));
#154822=CARTESIAN_POINT('Origin',(60.,28.41999998,-177.34995));
#154823=CARTESIAN_POINT('',(52.1813053461851,19.26999998,-177.34995));
#154824=CARTESIAN_POINT('',(60.,19.26999998,-177.34995));
#154825=CARTESIAN_POINT('',(52.1110349288339,19.76999998,-177.34995));
#154826=CARTESIAN_POINT('',(51.0717059287548,27.1652100787588,-177.34995));
#154827=CARTESIAN_POINT('',(60.,19.76999998,-177.34995));
#154828=CARTESIAN_POINT('Origin',(0.,-12.9675000200281,-171.64995));
#154829=CARTESIAN_POINT('',(50.9867892914963,16.9914785469432,-171.64995));
#154830=CARTESIAN_POINT('',(50.8071048221096,18.26999998,-171.64995));
#154831=CARTESIAN_POINT('',(50.7563939085354,18.6308268790399,-171.64995));
#154832=CARTESIAN_POINT('',(50.2136602208993,18.26999998,-171.64995));
#154833=CARTESIAN_POINT('',(49.8991400004038,18.26999998,-171.64995));
#154834=CARTESIAN_POINT('Origin',(0.,-12.9675000200281,-171.64995));
#154835=CARTESIAN_POINT('Ctrl Pts',(39.,20.796902498477,-78.7546851990749));
#154836=CARTESIAN_POINT('Ctrl Pts',(39.,19.1920627889827,-77.5254336382597));
#154837=CARTESIAN_POINT('Ctrl Pts',(40.4049679656207,18.0381727558475,-76.6415938903714));
#154838=CARTESIAN_POINT('Ctrl Pts',(39.,19.4994983593746,-80.4485009715931));
#154839=CARTESIAN_POINT('Ctrl Pts',(39.0000000000074,17.9467422700577,-79.2215151478833));
#154840=CARTESIAN_POINT('Ctrl Pts',(40.3537711092786,16.8074933352464,-78.3353996644624));
#154841=CARTESIAN_POINT('Ctrl Pts',(39.,18.1687833493074,-82.1249487171281));
#154842=CARTESIAN_POINT('Ctrl Pts',(39.,16.6676992320686,-80.9053032515377));
#154843=CARTESIAN_POINT('Ctrl Pts',(40.3009014559381,15.5494518783308,-80.0118574083956));
#154844=CARTESIAN_POINT('Ctrl Pts',(39.,15.4269620807205,-85.4195370156013));
#154845=CARTESIAN_POINT('Ctrl Pts',(39.,14.0354926345166,-84.2148910918098));
#154846=CARTESIAN_POINT('Ctrl Pts',(40.1923542727721,12.9680880684791,-83.3064457069268));
#154847=CARTESIAN_POINT('Ctrl Pts',(39.,14.0212774653657,-87.0315007804442));
#154848=CARTESIAN_POINT('Ctrl Pts',(39.,12.6882730287539,-85.8345023651596));
#154849=CARTESIAN_POINT('Ctrl Pts',(40.136876773061,11.6498700440212,-84.9183911253513));
#154850=CARTESIAN_POINT('Ctrl Pts',(39.,12.5683346400766,-88.5955027032924));
#154851=CARTESIAN_POINT('Ctrl Pts',(39.,11.2932302045755,-87.4109428798));
#154852=CARTESIAN_POINT('Ctrl Pts',(40.0806897769273,10.2937242346666,-86.4824113945889));
#154853=CARTESIAN_POINT('',(39.,18.2699999799838,-81.9737790469184));
#154854=CARTESIAN_POINT('',(39.,12.61999998,-88.5398461374725));
#154855=CARTESIAN_POINT('Ctrl Pts',(39.000000000374,18.2699999799838,-81.9737790469184));
#154856=CARTESIAN_POINT('Ctrl Pts',(39.0000000001679,17.7841524775854,-82.5769275834792));
#154857=CARTESIAN_POINT('Ctrl Pts',(39.0000000001103,17.2936169434169,-83.1765007297742));
#154858=CARTESIAN_POINT('Ctrl Pts',(39.0000000000735,16.7978518736795,-83.7722255217958));
#154859=CARTESIAN_POINT('Ctrl Pts',(39.0000000000309,16.2234293967186,-84.462467193726));
#154860=CARTESIAN_POINT('Ctrl Pts',(39.0000000000258,15.6429390502891,-85.1464596076239));
#154861=CARTESIAN_POINT('Ctrl Pts',(39.0000000000195,15.0550950356406,-85.8236901161975));
#154862=CARTESIAN_POINT('Ctrl Pts',(39.0000000000137,14.5092314506736,-86.4525567271471));
#154863=CARTESIAN_POINT('Ctrl Pts',(39.0000000000098,13.9570271965508,-87.0755929306875));
#154864=CARTESIAN_POINT('Ctrl Pts',(39.0000000000048,13.3974208289264,-87.6923562596894));
#154865=CARTESIAN_POINT('Ctrl Pts',(39.0000000000025,13.13988412639,-87.976197193578));
#154866=CARTESIAN_POINT('Ctrl Pts',(39.0000000000002,12.8807792236012,-88.2587090915938));
#154867=CARTESIAN_POINT('Ctrl Pts',(39.,12.61999998,-88.5398461374725));
#154868=CARTESIAN_POINT('',(40.4031452851324,17.9943647515726,-76.7018642453134));
#154869=CARTESIAN_POINT('Ctrl Pts',(39.,18.269999980001,-81.9737790469175));
#154870=CARTESIAN_POINT('Ctrl Pts',(38.9999999999998,18.2654156915697,-81.8856318368241));
#154871=CARTESIAN_POINT('Ctrl Pts',(39.0009991608804,18.26061957816,-81.7926846809007));
#154872=CARTESIAN_POINT('Ctrl Pts',(39.0033630480626,18.2555755018158,-81.6949391084757));
#154873=CARTESIAN_POINT('Ctrl Pts',(39.0056805350309,18.2506304345201,-81.5991121620725));
#154874=CARTESIAN_POINT('Ctrl Pts',(39.0093096132162,18.2454470421538,-81.498673282606));
#154875=CARTESIAN_POINT('Ctrl Pts',(39.0146446230652,18.2399896740651,-81.3936309537436));
#154876=CARTESIAN_POINT('Ctrl Pts',(39.0153733661184,18.2392442173188,-81.3792825514694));
#154877=CARTESIAN_POINT('Ctrl Pts',(39.0161340182114,18.2384936461679,-81.3648482669779));
#154878=CARTESIAN_POINT('Ctrl Pts',(39.0169276600567,18.2377378675041,-81.3503281331421));
#154879=CARTESIAN_POINT('Ctrl Pts',(39.0231927688791,18.2317716554125,-81.2357043653457));
#154880=CARTESIAN_POINT('Ctrl Pts',(39.0315081702222,18.2254891630288,-81.1157344332212));
#154881=CARTESIAN_POINT('Ctrl Pts',(39.0424313701074,18.2189126895613,-80.9904826023971));
#154882=CARTESIAN_POINT('Ctrl Pts',(39.04789297005,18.2156244528275,-80.927856686985));
#154883=CARTESIAN_POINT('Ctrl Pts',(39.0540073612066,18.2122635841095,-80.863911025723));
#154884=CARTESIAN_POINT('Ctrl Pts',(39.060848407193,18.2088387139701,-80.7986584961791));
#154885=CARTESIAN_POINT('Ctrl Pts',(39.0642689301862,18.2071262789005,-80.7660322314072));
#154886=CARTESIAN_POINT('Ctrl Pts',(39.0678711648011,18.2053978544484,-80.7330792582658));
#154887=CARTESIAN_POINT('Ctrl Pts',(39.0716645132203,18.203654996908,-80.6998015756023));
#154888=CARTESIAN_POINT('Ctrl Pts',(39.0735611874298,18.2027835681379,-80.6831627342706));
#154889=CARTESIAN_POINT('Ctrl Pts',(39.0755056424577,18.201908531612,-80.6664427159685));
#154890=CARTESIAN_POINT('Ctrl Pts',(39.0774990638269,18.2010300996946,-80.6496417847185));
#154891=CARTESIAN_POINT('Ctrl Pts',(39.0784957745116,18.200590883736,-80.6412413190935));
#154892=CARTESIAN_POINT('Ctrl Pts',(39.0795047269169,18.2001508189632,-80.6328206252585));
#154893=CARTESIAN_POINT('Ctrl Pts',(39.0805260696444,18.1997099337144,-80.624379737664));
#154894=CARTESIAN_POINT('Ctrl Pts',(39.0815474123718,18.1992690484656,-80.6159388500695));
#154895=CARTESIAN_POINT('Ctrl Pts',(39.0827573834569,18.1987528067232,-80.6060491570009));
#154896=CARTESIAN_POINT('Ctrl Pts',(39.0836274177688,18.1983848455065,-80.5989965285573));
#154897=CARTESIAN_POINT('Ctrl Pts',(39.1051352614155,18.1892885923952,-80.4246507265768));
#154898=CARTESIAN_POINT('Ctrl Pts',(39.1309066704761,18.1801885513109,-80.2503500624807));
#154899=CARTESIAN_POINT('Ctrl Pts',(39.1610112640735,18.1711018501782,-80.0763839135592));
#154900=CARTESIAN_POINT('Ctrl Pts',(39.1698759392603,18.1684261570551,-80.0251573989507));
#154901=CARTESIAN_POINT('Ctrl Pts',(39.1791159978341,18.1657516191816,-79.9739598404955));
#154902=CARTESIAN_POINT('Ctrl Pts',(39.1887323599578,18.1630786698777,-79.9227985019606));
#154903=CARTESIAN_POINT('Ctrl Pts',(39.220134300174,18.1543502346169,-79.7557326954332));
#154904=CARTESIAN_POINT('Ctrl Pts',(39.2555525447006,18.1456378884788,-79.589054911354));
#154905=CARTESIAN_POINT('Ctrl Pts',(39.2949852319104,18.1369559053374,-79.4230299972133));
#154906=CARTESIAN_POINT('Ctrl Pts',(39.3069784381681,18.1343153342298,-79.3725345534556));
#154907=CARTESIAN_POINT('Ctrl Pts',(39.3193426296427,18.1316775749095,-79.3220995551001));
#154908=CARTESIAN_POINT('Ctrl Pts',(39.3320767843687,18.1290430353581,-79.2717325590862));
#154909=CARTESIAN_POINT('Ctrl Pts',(39.3335084096053,18.1287468497541,-79.2660700974515));
#154910=CARTESIAN_POINT('Ctrl Pts',(39.3346928938226,18.1285025254522,-79.2613992073983));
#154911=CARTESIAN_POINT('Ctrl Pts',(39.3362385925853,18.1282026907361,-79.2553029077291));
#154912=CARTESIAN_POINT('Ctrl Pts',(39.3365946309511,18.1281336263977,-79.2538986777304));
#154913=CARTESIAN_POINT('Ctrl Pts',(39.3369699173628,18.1280616163234,-79.2524188090918));
#154914=CARTESIAN_POINT('Ctrl Pts',(39.3373720289107,18.1279853490152,-79.2508337742336));
#154915=CARTESIAN_POINT('Ctrl Pts',(39.3664342551112,18.1224732025065,-79.1362769010717));
#154916=CARTESIAN_POINT('Ctrl Pts',(39.3969619678381,18.1169261390775,-79.0242808226136));
#154917=CARTESIAN_POINT('Ctrl Pts',(39.428775919443,18.1113778371804,-78.9148742209707));
#154918=CARTESIAN_POINT('Ctrl Pts',(39.43458111554,18.1103654203351,-78.8949104395223));
#154919=CARTESIAN_POINT('Ctrl Pts',(39.4404291962516,18.1093529632644,-78.8750327509934));
#154920=CARTESIAN_POINT('Ctrl Pts',(39.4463191483709,18.108340671569,-78.8552411650393));
#154921=CARTESIAN_POINT('Ctrl Pts',(39.4749454395885,18.1034207407643,-78.7590502806814));
#154922=CARTESIAN_POINT('Ctrl Pts',(39.5045596054427,18.0985048054926,-78.6648976879518));
#154923=CARTESIAN_POINT('Ctrl Pts',(39.5350352637485,18.0936321430839,-78.5728004536459));
#154924=CARTESIAN_POINT('Ctrl Pts',(39.571899290306,18.0877380634667,-78.4613976134759));
#154925=CARTESIAN_POINT('Ctrl Pts',(39.6100411528787,18.0819102751752,-78.3529478782708));
#154926=CARTESIAN_POINT('Ctrl Pts',(39.649204178819,18.076223152307,-78.24756060623));
#154927=CARTESIAN_POINT('Ctrl Pts',(39.6883672047593,18.0705360294389,-78.1421733341892));
#154928=CARTESIAN_POINT('Ctrl Pts',(39.7285512433921,18.0649896536414,-78.039848263612));
#154929=CARTESIAN_POINT('Ctrl Pts',(39.7694967206528,18.0596550895294,-77.9406424526632));
#154930=CARTESIAN_POINT('Ctrl Pts',(39.7891552025899,18.0570938925608,-77.8930123901248));
#154931=CARTESIAN_POINT('Ctrl Pts',(39.8089883024401,18.0545801164714,-77.8460748119818));
#154932=CARTESIAN_POINT('Ctrl Pts',(39.8289779243427,18.0521207730912,-77.799822102316));
#154933=CARTESIAN_POINT('Ctrl Pts',(39.8812607387598,18.0456883656069,-77.6788482366005));
#154934=CARTESIAN_POINT('Ctrl Pts',(39.9345962223184,18.039559426019,-77.5627033684304));
#154935=CARTESIAN_POINT('Ctrl Pts',(39.9886489788594,18.0337023607363,-77.4513444300145));
#154936=CARTESIAN_POINT('Ctrl Pts',(40.0294901638302,18.0292768790051,-77.3672038367675));
#154937=CARTESIAN_POINT('Ctrl Pts',(40.0707395862103,18.0250065798345,-77.2857950222072));
#154938=CARTESIAN_POINT('Ctrl Pts',(40.112234287026,18.0208776696245,-77.2070925617702));
#154939=CARTESIAN_POINT('Ctrl Pts',(40.1739111069978,18.0147405473728,-77.090110937893));
#154940=CARTESIAN_POINT('Ctrl Pts',(40.2361301260653,18.0089161027968,-76.9791130352856));
#154941=CARTESIAN_POINT('Ctrl Pts',(40.2982915106338,18.0033979264447,-76.8739688586284));
#154942=CARTESIAN_POINT('Ctrl Pts',(40.3332999615727,18.0002901641669,-76.8147530806086));
#154943=CARTESIAN_POINT('Ctrl Pts',(40.3682890824644,17.9972795185705,-76.7573935352408));
#154944=CARTESIAN_POINT('Ctrl Pts',(40.4031452967415,17.9943646881396,-76.7018642559303));
#154945=CARTESIAN_POINT('',(40.1676094225648,12.3781800338281,-84.0075170117514));
#154946=CARTESIAN_POINT('Ctrl Pts',(40.1676234671554,12.3782653665599,-84.0075554249296));
#154947=CARTESIAN_POINT('Ctrl Pts',(40.1854904141354,12.8044715491944,-83.4873941951976));
#154948=CARTESIAN_POINT('Ctrl Pts',(40.2034989189839,13.2330557803372,-82.9558646413233));
#154949=CARTESIAN_POINT('Ctrl Pts',(40.221636439171,13.6644456562588,-82.4126443566806));
#154950=CARTESIAN_POINT('Ctrl Pts',(40.2299404179379,13.8619507359476,-82.1639394806617));
#154951=CARTESIAN_POINT('Ctrl Pts',(40.2382713875396,14.0600443482884,-81.9127845855315));
#154952=CARTESIAN_POINT('Ctrl Pts',(40.2466278643551,14.258769973405,-81.6591515576612));
#154953=CARTESIAN_POINT('Ctrl Pts',(40.2645132823419,14.6841036335584,-81.1162992505338));
#154954=CARTESIAN_POINT('Ctrl Pts',(40.2824940000457,15.1117784931431,-80.5627632534198));
#154955=CARTESIAN_POINT('Ctrl Pts',(40.3005593524997,15.5420020743483,-79.9983299955263));
#154956=CARTESIAN_POINT('Ctrl Pts',(40.3175555231764,15.9467632565014,-79.4673022167339));
#154957=CARTESIAN_POINT('Ctrl Pts',(40.3346265987071,16.3537802388756,-78.9266287711736));
#154958=CARTESIAN_POINT('Ctrl Pts',(40.351761140265,16.7632308195706,-78.3761759459867));
#154959=CARTESIAN_POINT('Ctrl Pts',(40.3688308672064,17.1711325766644,-77.8278053118314));
#154960=CARTESIAN_POINT('Ctrl Pts',(40.3859635974491,17.581449344521,-77.2697285875284));
#154961=CARTESIAN_POINT('Ctrl Pts',(40.4031453084497,17.9943647931319,-76.7018643085084));
#154962=CARTESIAN_POINT('Ctrl Pts',(40.1676094225648,12.3781800338281,-84.0075170117514));
#154963=CARTESIAN_POINT('Ctrl Pts',(40.0228549897639,12.3915973180658,-84.254864531227));
#154964=CARTESIAN_POINT('Ctrl Pts',(39.8658980290371,12.4063586860731,-84.557511956544));
#154965=CARTESIAN_POINT('Ctrl Pts',(39.6366325098753,12.4354191976067,-85.1013040029903));
#154966=CARTESIAN_POINT('Ctrl Pts',(39.5613574468262,12.4462035443194,-85.2975097823435));
#154967=CARTESIAN_POINT('Ctrl Pts',(39.4541753102143,12.4637879130523,-85.6144735095455));
#154968=CARTESIAN_POINT('Ctrl Pts',(39.4194087915838,12.4698763705169,-85.723898191007));
#154969=CARTESIAN_POINT('Ctrl Pts',(39.3692414744553,12.4792413419471,-85.8936607669787));
#154970=CARTESIAN_POINT('Ctrl Pts',(39.3446537532988,12.4839810030478,-85.9799477336672));
#154971=CARTESIAN_POINT('Ctrl Pts',(39.3169568710184,12.4895770893797,-86.0830613712933));
#154972=CARTESIAN_POINT('Ctrl Pts',(39.3033708464989,12.4923867809843,-86.1352271323001));
#154973=CARTESIAN_POINT('Ctrl Pts',(39.2976061261076,12.4935928782,-86.1577140972523));
#154974=CARTESIAN_POINT('Ctrl Pts',(39.2937760184904,12.4943973114159,-86.172734310248));
#154975=CARTESIAN_POINT('Ctrl Pts',(39.2914838099539,12.4948809191622,-86.1817797064966));
#154976=CARTESIAN_POINT('Ctrl Pts',(39.1927975915771,12.5157684085442,-86.5729597638327));
#154977=CARTESIAN_POINT('Ctrl Pts',(39.1204470384713,12.5381366398829,-86.9632929573707));
#154978=CARTESIAN_POINT('Ctrl Pts',(39.0247795673145,12.5764456511043,-87.744877974384));
#154979=CARTESIAN_POINT('Ctrl Pts',(39.0000000163315,12.5990133424068,-88.1415519987986));
#154980=CARTESIAN_POINT('Ctrl Pts',(39.,12.61999998,-88.5398461374725));
#154981=CARTESIAN_POINT('Origin',(39.,46.91999998,-129.34995));
#154982=CARTESIAN_POINT('',(39.,12.61999998,-143.518796834034));
#154983=CARTESIAN_POINT('',(39.,18.26999998,-150.084863924608));
#154984=CARTESIAN_POINT('Ctrl Pts',(39.,12.61999998,-143.518796834034));
#154985=CARTESIAN_POINT('Ctrl Pts',(39.0000000000004,13.1830701012418,-144.125823176784));
#154986=CARTESIAN_POINT('Ctrl Pts',(39.000000000008,13.738335643728,-144.73925540157));
#154987=CARTESIAN_POINT('Ctrl Pts',(39.0000000000126,14.2868563031708,-145.358644195209));
#154988=CARTESIAN_POINT('Ctrl Pts',(39.0000000000176,14.8748775264481,-146.0226369726));
#154989=CARTESIAN_POINT('Ctrl Pts',(39.0000000000202,15.4551472634197,-146.693475297462));
#154990=CARTESIAN_POINT('Ctrl Pts',(39.0000000000369,16.0289279109354,-147.370648869858));
#154991=CARTESIAN_POINT('Ctrl Pts',(39.0000000000444,16.2865138368738,-147.674650725657));
#154992=CARTESIAN_POINT('Ctrl Pts',(39.000000000055,16.5427914446702,-147.979929896419));
#154993=CARTESIAN_POINT('Ctrl Pts',(39.0000000000741,16.7978726164159,-148.286442551932));
#154994=CARTESIAN_POINT('Ctrl Pts',(39.0000000001113,17.2936331206748,-148.88216221097));
#154995=CARTESIAN_POINT('Ctrl Pts',(39.0000000001696,17.7841600789862,-149.481724824065));
#154996=CARTESIAN_POINT('Ctrl Pts',(39.0000000003777,18.26999998,-150.084863924608));
#154997=CARTESIAN_POINT('',(39.,18.26999998,-129.34995));
#154998=CARTESIAN_POINT('',(39.,12.61999998,-129.34995));
#154999=CARTESIAN_POINT('Ctrl Pts',(40.4049679555898,18.0381725147214,-155.417048749269));
#155000=CARTESIAN_POINT('Ctrl Pts',(39.,19.1920625442621,-154.533208999946));
#155001=CARTESIAN_POINT('Ctrl Pts',(39.,20.7969022442792,-153.303957440565));
#155002=CARTESIAN_POINT('Ctrl Pts',(40.3537709661131,16.8074898953919,-153.723238579969));
#155003=CARTESIAN_POINT('Ctrl Pts',(38.9999999999926,17.9467387756562,-152.837123072008));
#155004=CARTESIAN_POINT('Ctrl Pts',(39.,19.4994946787828,-151.61013720275));
#155005=CARTESIAN_POINT('Ctrl Pts',(40.3009026952457,15.549481350471,-152.046823901733));
#155006=CARTESIAN_POINT('Ctrl Pts',(38.9999999999925,16.6677293129161,-151.153378312361));
#155007=CARTESIAN_POINT('Ctrl Pts',(39.,18.1688145972663,-149.933732593));
#155008=CARTESIAN_POINT('Ctrl Pts',(40.1923546827668,12.9680978184463,-148.752208985047));
#155009=CARTESIAN_POINT('Ctrl Pts',(39.0000000000073,14.0355026731613,-147.843763736059));
#155010=CARTESIAN_POINT('Ctrl Pts',(39.,15.4269724929124,-146.639117676373));
#155011=CARTESIAN_POINT('Ctrl Pts',(40.1368768832445,11.6498727042044,-147.140254909589));
#155012=CARTESIAN_POINT('Ctrl Pts',(39.0000000000223,12.6882757758116,-146.224143705887));
#155013=CARTESIAN_POINT('Ctrl Pts',(39.,14.0212803181596,-145.027145257042));
#155014=CARTESIAN_POINT('Ctrl Pts',(40.0806897728025,10.2937241351084,-145.576231462098));
#155015=CARTESIAN_POINT('Ctrl Pts',(39.,11.293230102484,-144.64769997634));
#155016=CARTESIAN_POINT('Ctrl Pts',(39.,12.5683345334111,-143.463140153395));
#155017=CARTESIAN_POINT('',(40.4031452850214,17.9943647518538,-155.356778726108));
#155018=CARTESIAN_POINT('',(40.1676094240942,12.378180022345,-148.051125971627));
#155019=CARTESIAN_POINT('Ctrl Pts',(40.4031453084766,17.9943647936175,-155.356778662625));
#155020=CARTESIAN_POINT('Ctrl Pts',(40.3860321140814,17.5830959513313,-154.791178868832));
#155021=CARTESIAN_POINT('Ctrl Pts',(40.3689676275558,17.1744079304129,-154.235292309724));
#155022=CARTESIAN_POINT('Ctrl Pts',(40.3519656027356,16.7681166958106,-153.689035359578));
#155023=CARTESIAN_POINT('Ctrl Pts',(40.3339478834236,16.3375537774879,-153.110145227137));
#155024=CARTESIAN_POINT('Ctrl Pts',(40.316000320502,15.9096827342591,-152.542069480784));
#155025=CARTESIAN_POINT('Ctrl Pts',(40.2981360458695,15.4842945621373,-151.984648335164));
#155026=CARTESIAN_POINT('Ctrl Pts',(40.2808862495354,15.0735384870678,-151.446400831022));
#155027=CARTESIAN_POINT('Ctrl Pts',(40.2637140755375,14.665097672676,-150.918086687449));
#155028=CARTESIAN_POINT('Ctrl Pts',(40.2466286890062,14.2587895844586,-150.39951644339));
#155029=CARTESIAN_POINT('Ctrl Pts',(40.2283833140916,13.8248957777965,-149.845738599086));
#155030=CARTESIAN_POINT('Ctrl Pts',(40.210259843033,13.3940133909222,-149.30377834175));
#155031=CARTESIAN_POINT('Ctrl Pts',(40.1922726412517,12.9657005449508,-148.773332424983));
#155032=CARTESIAN_POINT('Ctrl Pts',(40.1840273016278,12.7693617856903,-148.530175830143));
#155033=CARTESIAN_POINT('Ctrl Pts',(40.1758105398716,12.5735634700978,-148.289438170232));
#155034=CARTESIAN_POINT('Ctrl Pts',(40.1676234671417,12.3782653572967,-148.051087554154));
#155035=CARTESIAN_POINT('Ctrl Pts',(40.4031452966654,17.994364688146,-155.356778715455));
#155036=CARTESIAN_POINT('Ctrl Pts',(40.3417594471859,17.9994980567657,-155.258985209779));
#155037=CARTESIAN_POINT('Ctrl Pts',(40.280419765882,18.0048901664367,-155.156247032814));
#155038=CARTESIAN_POINT('Ctrl Pts',(40.2196167541285,18.0105466339004,-155.04845145244));
#155039=CARTESIAN_POINT('Ctrl Pts',(40.173064781723,18.01487733578,-154.965921052411));
#155040=CARTESIAN_POINT('Ctrl Pts',(40.1268268322551,18.0193629844826,-154.880426356048));
#155041=CARTESIAN_POINT('Ctrl Pts',(40.081103453352,18.0240056787045,-154.791924271342));
#155042=CARTESIAN_POINT('Ctrl Pts',(40.0300289459692,18.0291917197627,-154.69306455259));
#155043=CARTESIAN_POINT('Ctrl Pts',(39.9796023466813,18.0345733014836,-154.590459987357));
#155044=CARTESIAN_POINT('Ctrl Pts',(39.9300871858588,18.0401504376233,-154.484104885994));
#155045=CARTESIAN_POINT('Ctrl Pts',(39.8805720250364,18.045727573763,-154.37774978463));
#155046=CARTESIAN_POINT('Ctrl Pts',(39.8319690807585,18.0515002708413,-154.267644023757));
#155047=CARTESIAN_POINT('Ctrl Pts',(39.7845003415924,18.0574666071742,-154.153818005325));
#155048=CARTESIAN_POINT('Ctrl Pts',(39.7814378422914,18.0578515320989,-154.146474391232));
#155049=CARTESIAN_POINT('Ctrl Pts',(39.7776001357721,18.0583360042348,-154.13723144672));
#155050=CARTESIAN_POINT('Ctrl Pts',(39.7753269786915,18.0586238608678,-154.131740764591));
#155051=CARTESIAN_POINT('Ctrl Pts',(39.77395412672,18.0587977091907,-154.128424718441));
#155052=CARTESIAN_POINT('Ctrl Pts',(39.772580519514,18.0589719361886,-154.125101397286));
#155053=CARTESIAN_POINT('Ctrl Pts',(39.7712061770303,18.0591465420297,-154.121770798376));
#155054=CARTESIAN_POINT('Ctrl Pts',(39.7147134503032,18.0663237632711,-153.984865611844));
#155055=CARTESIAN_POINT('Ctrl Pts',(39.6570058671139,18.0741420356517,-153.835646393747));
#155056=CARTESIAN_POINT('Ctrl Pts',(39.5997365496176,18.0826184704731,-153.673814403576));
#155057=CARTESIAN_POINT('Ctrl Pts',(39.5845780628911,18.0848620789243,-153.630979458405));
#155058=CARTESIAN_POINT('Ctrl Pts',(39.5694505681787,18.0871518019538,-153.587260749271));
#155059=CARTESIAN_POINT('Ctrl Pts',(39.5543851687262,18.0894879617595,-153.542652542234));
#155060=CARTESIAN_POINT('Ctrl Pts',(39.5151902756828,18.0955658313842,-153.426597610589));
#155061=CARTESIAN_POINT('Ctrl Pts',(39.4764206630589,18.1019568988266,-153.304531892792));
#155062=CARTESIAN_POINT('Ctrl Pts',(39.4386411928737,18.1086618989044,-153.176428855199));
#155063=CARTESIAN_POINT('Ctrl Pts',(39.4068074123412,18.1143116737662,-153.06848652662));
#155064=CARTESIAN_POINT('Ctrl Pts',(39.3756773812159,18.120184284672,-152.956258735352));
#155065=CARTESIAN_POINT('Ctrl Pts',(39.3455832861018,18.1262784534442,-152.839761180211));
#155066=CARTESIAN_POINT('Ctrl Pts',(39.3445386995356,18.1264899861986,-152.835717470619));
#155067=CARTESIAN_POINT('Ctrl Pts',(39.3431410854322,18.1267738816604,-152.830290388621));
#155068=CARTESIAN_POINT('Ctrl Pts',(39.3424532775621,18.1269138636721,-152.827614629636));
#155069=CARTESIAN_POINT('Ctrl Pts',(39.3413285750048,18.1271427620804,-152.823239231935));
#155070=CARTESIAN_POINT('Ctrl Pts',(39.3401977921499,18.1273735054214,-152.818828478333));
#155071=CARTESIAN_POINT('Ctrl Pts',(39.3390610558454,18.1276060961256,-152.814382322845));
#155072=CARTESIAN_POINT('Ctrl Pts',(39.3244959323229,18.130586305629,-152.757413258302));
#155073=CARTESIAN_POINT('Ctrl Pts',(39.3089685134929,18.1338668144423,-152.694689316399));
#155074=CARTESIAN_POINT('Ctrl Pts',(39.2927900726882,18.1374504392791,-152.626156872866));
#155075=CARTESIAN_POINT('Ctrl Pts',(39.2855217920503,18.1390604084554,-152.595368180778));
#155076=CARTESIAN_POINT('Ctrl Pts',(39.2781228183628,18.1407315528484,-152.563407190484));
#155077=CARTESIAN_POINT('Ctrl Pts',(39.2706247681685,18.142464101305,-152.530269443939));
#155078=CARTESIAN_POINT('Ctrl Pts',(39.2578795193265,18.1454091017568,-152.473941623395));
#155079=CARTESIAN_POINT('Ctrl Pts',(39.2448479300532,18.1485312638142,-152.414216824096));
#155080=CARTESIAN_POINT('Ctrl Pts',(39.2316997667936,18.1518310602961,-152.351082418171));
#155081=CARTESIAN_POINT('Ctrl Pts',(39.2251256851638,18.1534809585371,-152.319515215208));
#155082=CARTESIAN_POINT('Ctrl Pts',(39.2185227175705,18.1551752605691,-152.287095693681));
#155083=CARTESIAN_POINT('Ctrl Pts',(39.2119135922845,18.1569139918642,-152.253822861645));
#155084=CARTESIAN_POINT('Ctrl Pts',(39.2086090296414,18.1577833575118,-152.237186445627));
#155085=CARTESIAN_POINT('Ctrl Pts',(39.2053029411143,18.1586638305792,-152.220336699373));
#155086=CARTESIAN_POINT('Ctrl Pts',(39.2019982610058,18.1595554112169,-152.203273553159));
#155087=CARTESIAN_POINT('Ctrl Pts',(39.2003459209516,18.1600012015357,-152.194741980052));
#155088=CARTESIAN_POINT('Ctrl Pts',(39.198693933812,18.1604497687537,-152.186157056788));
#155089=CARTESIAN_POINT('Ctrl Pts',(39.1970426716466,18.1609011128083,-152.177518775964));
#155090=CARTESIAN_POINT('Ctrl Pts',(39.1962170405639,18.1611267848356,-152.173199635552));
#155091=CARTESIAN_POINT('Ctrl Pts',(39.1953915907749,18.1613531510724,-152.16886715574));
#155092=CARTESIAN_POINT('Ctrl Pts',(39.1945663691362,18.1615802114996,-152.164521335805));
#155093=CARTESIAN_POINT('Ctrl Pts',(39.1937411474975,18.1618072719268,-152.160175515869));
#155094=CARTESIAN_POINT('Ctrl Pts',(39.1931776325701,18.1619625964041,-152.157202665874));
#155095=CARTESIAN_POINT('Ctrl Pts',(39.1920914357414,18.1622634753302,-152.15144385495));
#155096=CARTESIAN_POINT('Ctrl Pts',(39.1788631156134,18.1659277492899,-152.081309794124));
#155097=CARTESIAN_POINT('Ctrl Pts',(39.1672931884971,18.1693409956331,-152.016198167235));
#155098=CARTESIAN_POINT('Ctrl Pts',(39.1570953546843,18.1724913915801,-151.956153037642));
#155099=CARTESIAN_POINT('Ctrl Pts',(39.1467171302433,18.1756975152351,-151.895045763004));
#155100=CARTESIAN_POINT('Ctrl Pts',(39.1377599277363,18.1786314258552,-151.83918548891));
#155101=CARTESIAN_POINT('Ctrl Pts',(39.1299726355725,18.1812818179602,-151.788599497983));
#155102=CARTESIAN_POINT('Ctrl Pts',(39.1253058882552,18.1828701377491,-151.758284462604));
#155103=CARTESIAN_POINT('Ctrl Pts',(39.1210602663186,18.1843566573616,-151.729863257325));
#155104=CARTESIAN_POINT('Ctrl Pts',(39.1171902972612,18.1857390937416,-151.703339248921));
#155105=CARTESIAN_POINT('Ctrl Pts',(39.1106448931655,18.188077253197,-151.658478333843));
#155106=CARTESIAN_POINT('Ctrl Pts',(39.1051703967782,18.1901236336778,-151.619046015605));
#155107=CARTESIAN_POINT('Ctrl Pts',(39.1005859920701,18.1918842844985,-151.585053901893));
#155108=CARTESIAN_POINT('Ctrl Pts',(39.0993314455262,18.1923660958879,-151.575751780573));
#155109=CARTESIAN_POINT('Ctrl Pts',(39.0981438522368,18.1928265117298,-151.566857005841));
#155110=CARTESIAN_POINT('Ctrl Pts',(39.097020173279,18.193265659932,-151.558369702141));
#155111=CARTESIAN_POINT('Ctrl Pts',(39.0944052417367,18.1942876088418,-151.538618759936));
#155112=CARTESIAN_POINT('Ctrl Pts',(39.092135864911,18.1951945362373,-151.521074619786));
#155113=CARTESIAN_POINT('Ctrl Pts',(39.0901796603349,18.1959884327771,-151.50573856626));
#155114=CARTESIAN_POINT('Ctrl Pts',(39.0892015580469,18.196385381047,-151.498070539497));
#155115=CARTESIAN_POINT('Ctrl Pts',(39.0883018748229,18.1967540904593,-151.490954519409));
#155116=CARTESIAN_POINT('Ctrl Pts',(39.0874773395217,18.1970947718093,-151.484390616359));
#155117=CARTESIAN_POINT('Ctrl Pts',(39.0870650718711,18.1972651124842,-151.481108664835));
#155118=CARTESIAN_POINT('Ctrl Pts',(39.0866715989482,18.1974284473239,-151.477964741632));
#155119=CARTESIAN_POINT('Ctrl Pts',(39.086296559352,18.1975848038151,-151.474958857364));
#155120=CARTESIAN_POINT('Ctrl Pts',(39.0861090395539,18.1976629820607,-151.473455915231));
#155121=CARTESIAN_POINT('Ctrl Pts',(39.0859261285695,18.19773941579,-151.471987482775));
#155122=CARTESIAN_POINT('Ctrl Pts',(39.0857477842125,18.197814108305,-151.470553561156));
#155123=CARTESIAN_POINT('Ctrl Pts',(39.085658612034,18.1978514545625,-151.469836600346));
#155124=CARTESIAN_POINT('Ctrl Pts',(39.0855705815424,18.1978883655208,-151.469128267242));
#155125=CARTESIAN_POINT('Ctrl Pts',(39.0854836876517,18.1979248415804,-151.468428561981));
#155126=CARTESIAN_POINT('Ctrl Pts',(39.0854619641791,18.1979339605953,-151.468253635665));
#155127=CARTESIAN_POINT('Ctrl Pts',(39.0854515340338,18.197938339297,-151.4681696234));
#155128=CARTESIAN_POINT('Ctrl Pts',(39.0854439756643,18.1979415118432,-151.468108744634));
#155129=CARTESIAN_POINT('Ctrl Pts',(39.0854326381102,18.1979462706624,-151.468017426485));
#155130=CARTESIAN_POINT('Ctrl Pts',(39.0854277616982,18.1979483155799,-151.46797815875));
#155131=CARTESIAN_POINT('Ctrl Pts',(39.0854009525399,18.1979595786092,-151.467762178707));
#155132=CARTESIAN_POINT('Ctrl Pts',(39.0853741433817,18.1979708416385,-151.467546198663));
#155133=CARTESIAN_POINT('Ctrl Pts',(39.0853253870772,18.1979913212022,-151.467153507985));
#155134=CARTESIAN_POINT('Ctrl Pts',(39.085226410725,18.1980329661159,-151.466355329862));
#155135=CARTESIAN_POINT('Ctrl Pts',(39.0849289026081,18.1981581445001,-151.463956125758));
#155136=CARTESIAN_POINT('Ctrl Pts',(39.0846323917651,18.1982832354517,-151.46155857911));
#155137=CARTESIAN_POINT('Ctrl Pts',(39.0843368746301,18.1984082389251,-151.459162690843));
#155138=CARTESIAN_POINT('Ctrl Pts',(39.0670855857401,18.2057055180914,-151.319298852997));
#155139=CARTESIAN_POINT('Ctrl Pts',(39.0531814282618,18.2127125095008,-151.184936931341));
#155140=CARTESIAN_POINT('Ctrl Pts',(39.0420026133318,18.2194266697535,-151.056136661796));
#155141=CARTESIAN_POINT('Ctrl Pts',(39.0308452663617,18.2261279360345,-150.927583742174));
#155142=CARTESIAN_POINT('Ctrl Pts',(39.0224027838946,18.2325374963608,-150.804571134108));
#155143=CARTESIAN_POINT('Ctrl Pts',(39.0161084260695,18.238653156518,-150.687152448744));
#155144=CARTESIAN_POINT('Ctrl Pts',(39.0098304711397,18.2447528794603,-150.570039752719));
#155145=CARTESIAN_POINT('Ctrl Pts',(39.0056894504988,18.2505602334755,-150.458491861449));
#155146=CARTESIAN_POINT('Ctrl Pts',(39.0031745103681,18.2560733519913,-150.352556215922));
#155147=CARTESIAN_POINT('Ctrl Pts',(39.000951854371,18.2609457407142,-150.258932318096));
#155148=CARTESIAN_POINT('Ctrl Pts',(39.,18.2655883162516,-150.169691888134));
#155149=CARTESIAN_POINT('Ctrl Pts',(39.,18.26999998,-150.084863924608));
#155150=CARTESIAN_POINT('Ctrl Pts',(39.,12.61999998,-143.518796834034));
#155151=CARTESIAN_POINT('Ctrl Pts',(39.,12.6151217916977,-143.611377351187));
#155152=CARTESIAN_POINT('Ctrl Pts',(39.001285417222,12.6099953737847,-143.708586401381));
#155153=CARTESIAN_POINT('Ctrl Pts',(39.0042875091668,12.6046202721211,-143.810409212199));
#155154=CARTESIAN_POINT('Ctrl Pts',(39.0070158061698,12.5997353871711,-143.902945641696));
#155155=CARTESIAN_POINT('Ctrl Pts',(39.0111625213286,12.5946450511523,-143.999293736081));
#155156=CARTESIAN_POINT('Ctrl Pts',(39.0170880852875,12.5893494102396,-144.099432636865));
#155157=CARTESIAN_POINT('Ctrl Pts',(39.0226020020085,12.5844216559904,-144.192614916778));
#155158=CARTESIAN_POINT('Ctrl Pts',(39.0296564835121,12.5793163599211,-144.289075241998));
#155159=CARTESIAN_POINT('Ctrl Pts',(39.0385666744866,12.5740351371479,-144.388768460183));
#155160=CARTESIAN_POINT('Ctrl Pts',(39.0430217699738,12.5713945257613,-144.438615069276));
#155161=CARTESIAN_POINT('Ctrl Pts',(39.0479411388294,12.5687099636132,-144.489269319451));
#155162=CARTESIAN_POINT('Ctrl Pts',(39.0533661791931,12.5659817900504,-144.540723001229));
#155163=CARTESIAN_POINT('Ctrl Pts',(39.056078699375,12.564617703269,-144.566449842117));
#155164=CARTESIAN_POINT('Ctrl Pts',(39.0589176574687,12.5632427150076,-144.592376515436));
#155165=CARTESIAN_POINT('Ctrl Pts',(39.0618883354043,12.5618568790563,-144.618501783899));
#155166=CARTESIAN_POINT('Ctrl Pts',(39.0626310048883,12.5615104200685,-144.625033101014));
#155167=CARTESIAN_POINT('Ctrl Pts',(39.0633819072345,12.5611632831152,-144.631576830055));
#155168=CARTESIAN_POINT('Ctrl Pts',(39.0641411256594,12.5608154690912,-144.638132950689));
#155169=CARTESIAN_POINT('Ctrl Pts',(39.0647105394781,12.5605546085733,-144.643050041165));
#155170=CARTESIAN_POINT('Ctrl Pts',(39.0652846310973,12.5602933672032,-144.647974101911));
#155171=CARTESIAN_POINT('Ctrl Pts',(39.0658634357377,12.5600317453597,-144.652905124331));
#155172=CARTESIAN_POINT('Ctrl Pts',(39.0660384936335,12.5599526185417,-144.654396498707));
#155173=CARTESIAN_POINT('Ctrl Pts',(39.0662133034635,12.559873761637,-144.655882766897));
#155174=CARTESIAN_POINT('Ctrl Pts',(39.0663916080063,12.5597934932929,-144.65739561764));
#155175=CARTESIAN_POINT('Ctrl Pts',(39.0677898358322,12.5591640453241,-144.669259084336));
#155176=CARTESIAN_POINT('Ctrl Pts',(39.0693646538055,12.5584672545937,-144.682390329012));
#155177=CARTESIAN_POINT('Ctrl Pts',(39.0706765465421,12.5578951255962,-144.693171271542));
#155178=CARTESIAN_POINT('Ctrl Pts',(39.070856771342,12.5578165278334,-144.694652332574));
#155179=CARTESIAN_POINT('Ctrl Pts',(39.0710319534679,12.5577402823252,-144.696089049905));
#155180=CARTESIAN_POINT('Ctrl Pts',(39.0712008829784,12.5576668864921,-144.697472054104));
#155181=CARTESIAN_POINT('Ctrl Pts',(39.0869456209749,12.5508261743042,-144.826372201183));
#155182=CARTESIAN_POINT('Ctrl Pts',(39.1053961392304,12.5438077204206,-144.955367405366));
#155183=CARTESIAN_POINT('Ctrl Pts',(39.126578585198,12.5367888738498,-145.084303731865));
#155184=CARTESIAN_POINT('Ctrl Pts',(39.1370708909132,12.5333122270027,-145.148169791408));
#155185=CARTESIAN_POINT('Ctrl Pts',(39.1482327304231,12.5298352050449,-145.212021539346));
#155186=CARTESIAN_POINT('Ctrl Pts',(39.1600630009103,12.5263775808316,-145.275841235295));
#155187=CARTESIAN_POINT('Ctrl Pts',(39.1689914693088,12.5237680641214,-145.324006840561));
#155188=CARTESIAN_POINT('Ctrl Pts',(39.1783005066348,12.521170027977,-145.37215406157));
#155189=CARTESIAN_POINT('Ctrl Pts',(39.187988311637,12.5185924412067,-145.42027522266));
#155190=CARTESIAN_POINT('Ctrl Pts',(39.1976761166393,12.5160148544364,-145.468396383749));
#155191=CARTESIAN_POINT('Ctrl Pts',(39.2077426849771,12.5134577213724,-145.516491480961));
#155192=CARTESIAN_POINT('Ctrl Pts',(39.2181853048246,12.5109296373551,-145.564553167133));
#155193=CARTESIAN_POINT('Ctrl Pts',(39.228627924672,12.5084015533379,-145.612614853305));
#155194=CARTESIAN_POINT('Ctrl Pts',(39.2394465955928,12.5059025182058,-145.660643128128));
#155195=CARTESIAN_POINT('Ctrl Pts',(39.2506376189685,12.5034410609666,-145.70863080923));
#155196=CARTESIAN_POINT('Ctrl Pts',(39.2562331306563,12.5022103323471,-145.732624649781));
#155197=CARTESIAN_POINT('Ctrl Pts',(39.2619217169944,12.5009889917376,-145.756608347695));
#155198=CARTESIAN_POINT('Ctrl Pts',(39.2677028352578,12.4997780721034,-145.780581038343));
#155199=CARTESIAN_POINT('Ctrl Pts',(39.2705933943894,12.4991726122863,-145.792567383666));
#155200=CARTESIAN_POINT('Ctrl Pts',(39.2735070857133,12.4985697572877,-145.804550977563));
#155201=CARTESIAN_POINT('Ctrl Pts',(39.2764438363011,12.4979696347552,-145.81653171371));
#155202=CARTESIAN_POINT('Ctrl Pts',(39.2779122115949,12.497669573489,-145.822522081783));
#155203=CARTESIAN_POINT('Ctrl Pts',(39.2793863516566,12.4973701953126,-145.828511735444));
#155204=CARTESIAN_POINT('Ctrl Pts',(39.2808662470572,12.4970715160892,-145.834500661514));
#155205=CARTESIAN_POINT('Ctrl Pts',(39.282143744699,12.4968136857024,-145.83967051266));
#155206=CARTESIAN_POINT('Ctrl Pts',(39.2831842318061,12.4966045567679,-145.843868940243));
#155207=CARTESIAN_POINT('Ctrl Pts',(39.2846166008847,12.496302858648,-145.849609262975));
#155208=CARTESIAN_POINT('Ctrl Pts',(39.2848435353867,12.4962550597157,-145.850518719414));
#155209=CARTESIAN_POINT('Ctrl Pts',(39.2850803473589,12.4962049370979,-145.851466879967));
#155210=CARTESIAN_POINT('Ctrl Pts',(39.2853295849969,12.4961519292614,-145.85246373439));
#155211=CARTESIAN_POINT('Ctrl Pts',(39.3144876655075,12.4899505915487,-145.96908481043));
#155212=CARTESIAN_POINT('Ctrl Pts',(39.3452757917139,12.4838818138653,-146.082626080962));
#155213=CARTESIAN_POINT('Ctrl Pts',(39.377433242888,12.4779746135799,-146.193064054807));
#155214=CARTESIAN_POINT('Ctrl Pts',(39.4015513312685,12.4735442133658,-146.27589253519));
#155215=CARTESIAN_POINT('Ctrl Pts',(39.4264397287502,12.4692045367127,-146.356975344281));
#155216=CARTESIAN_POINT('Ctrl Pts',(39.451991679228,12.4649566420713,-146.436300560345));
#155217=CARTESIAN_POINT('Ctrl Pts',(39.4903196049447,12.4585848001093,-146.55528838444));
#155218=CARTESIAN_POINT('Ctrl Pts',(39.5301458154197,12.452418499751,-146.670335595739));
#155219=CARTESIAN_POINT('Ctrl Pts',(39.5711029864092,12.4464465664109,-146.78136878618));
#155220=CARTESIAN_POINT('Ctrl Pts',(39.6120601573987,12.4404746330708,-146.89240197662));
#155221=CARTESIAN_POINT('Ctrl Pts',(39.6541481889008,12.4346970509066,-146.999421769204));
#155222=CARTESIAN_POINT('Ctrl Pts',(39.697010140157,12.4291022091382,-147.102407485838));
#155223=CARTESIAN_POINT('Ctrl Pts',(39.7351096523847,12.4241290164551,-147.193950345067));
#155224=CARTESIAN_POINT('Ctrl Pts',(39.7738018023959,12.4193428417345,-147.282307078856));
#155225=CARTESIAN_POINT('Ctrl Pts',(39.8128440602613,12.4147562936274,-147.367529588044));
#155226=CARTESIAN_POINT('Ctrl Pts',(39.8618865683454,12.4089949510485,-147.474580917149));
#155227=CARTESIAN_POINT('Ctrl Pts',(39.9114819117157,12.4035479278012,-147.576688885594));
#155228=CARTESIAN_POINT('Ctrl Pts',(39.9611833644274,12.3983649064512,-147.673940637116));
#155229=CARTESIAN_POINT('Ctrl Pts',(39.97083216751,12.3973586993959,-147.692820628519));
#155230=CARTESIAN_POINT('Ctrl Pts',(39.9804850491675,12.3963624584099,-147.711517731987));
#155231=CARTESIAN_POINT('Ctrl Pts',(39.9901388560831,12.3953758384233,-147.730032771159));
#155232=CARTESIAN_POINT('Ctrl Pts',(40.042584448648,12.3900158938656,-147.830618188829));
#155233=CARTESIAN_POINT('Ctrl Pts',(40.0950616995403,12.3849250467423,-147.925821963176));
#155234=CARTESIAN_POINT('Ctrl Pts',(40.1470365111874,12.380085203232,-148.015755916064));
#155235=CARTESIAN_POINT('Ctrl Pts',(40.1539032839609,12.3794457760827,-148.027637748812));
#155236=CARTESIAN_POINT('Ctrl Pts',(40.1607613212998,12.3788107298062,-148.039427662383));
#155237=CARTESIAN_POINT('Ctrl Pts',(40.1676094240942,12.378180022345,-148.051125971627));
#155238=CARTESIAN_POINT('Origin',(0.,-12.9675000200281,-171.64995));
#155239=CARTESIAN_POINT('',(52.4039495302269,12.4224147476539,-171.07256826174));
#155240=CARTESIAN_POINT('',(49.2955572616308,18.0287857662077,-171.07256826174));
#155241=CARTESIAN_POINT('Origin',(0.,-12.9675000200281,-171.07256826174));
#155242=CARTESIAN_POINT('Ctrl Pts',(49.2955572616308,18.0287857662076,-171.07256826174));
#155243=CARTESIAN_POINT('Ctrl Pts',(48.7132630683598,18.0267551266955,-170.013127987308));
#155244=CARTESIAN_POINT('Ctrl Pts',(48.1371153371835,18.0247048552528,-168.969866266346));
#155245=CARTESIAN_POINT('Ctrl Pts',(47.5669953586077,18.0226353122181,-167.942835850289));
#155246=CARTESIAN_POINT('Ctrl Pts',(46.9862239296856,18.0205271042783,-166.896617607296));
#155247=CARTESIAN_POINT('Ctrl Pts',(46.4117077069108,18.0183988996116,-165.86724275765));
#155248=CARTESIAN_POINT('Ctrl Pts',(45.8433676787677,18.0162516178655,-164.854739370262));
#155249=CARTESIAN_POINT('Ctrl Pts',(45.2580605358242,18.0140402315798,-163.812008899861));
#155250=CARTESIAN_POINT('Ctrl Pts',(44.6793039153065,18.0118086131983,-162.787172249637));
#155251=CARTESIAN_POINT('Ctrl Pts',(44.1070591167068,18.0095583137349,-161.78023170509));
#155252=CARTESIAN_POINT('Ctrl Pts',(43.5239608645021,18.0072653340743,-160.754193070863));
#155253=CARTESIAN_POINT('Ctrl Pts',(42.9476239530702,18.004952960289,-159.746735734167));
#155254=CARTESIAN_POINT('Ctrl Pts',(42.3780543128992,18.0026233653842,-158.757834162611));
#155255=CARTESIAN_POINT('Ctrl Pts',(41.7921767666784,18.0002270695668,-157.740618381898));
#155256=CARTESIAN_POINT('Ctrl Pts',(41.2134596804323,17.9978125542456,-156.743036083865));
#155257=CARTESIAN_POINT('Ctrl Pts',(40.641956554655,17.9953827110471,-155.765031415368));
#155258=CARTESIAN_POINT('Ctrl Pts',(40.5622122112717,17.9950436643444,-155.628566124808));
#155259=CARTESIAN_POINT('Ctrl Pts',(40.4826083936333,17.9947043199976,-155.492481965325));
#155260=CARTESIAN_POINT('Ctrl Pts',(40.4031453149964,17.9943646866131,-155.356778744658));
#155261=CARTESIAN_POINT('Ctrl Pts',(40.1676286103913,12.3781782553038,-148.05115874653));
#155262=CARTESIAN_POINT('Ctrl Pts',(40.7369146152135,12.3806129238374,-149.086420661532));
#155263=CARTESIAN_POINT('Ctrl Pts',(41.3145214278423,12.3830242794477,-150.142821070685));
#155264=CARTESIAN_POINT('Ctrl Pts',(41.9004187180735,12.3854095614278,-151.220396408575));
#155265=CARTESIAN_POINT('Ctrl Pts',(42.4720688158783,12.387736840799,-152.271768479359));
#155266=CARTESIAN_POINT('Ctrl Pts',(43.0516112855504,12.3900392971675,-153.343298885691));
#155267=CARTESIAN_POINT('Ctrl Pts',(43.639059311913,12.3923151748205,-154.434995860215));
#155268=CARTESIAN_POINT('Ctrl Pts',(44.2115536547062,12.394533119256,-155.498903327619));
#155269=CARTESIAN_POINT('Ctrl Pts',(44.7915556819794,12.3967258166804,-156.581963045714));
#155270=CARTESIAN_POINT('Ctrl Pts',(45.3791183645239,12.3988924598231,-157.684155326372));
#155271=CARTESIAN_POINT('Ctrl Pts',(45.69458603494,12.4000557499454,-158.275932240494));
#155272=CARTESIAN_POINT('Ctrl Pts',(46.0122339467694,12.401211543745,-158.873224061255));
#155273=CARTESIAN_POINT('Ctrl Pts',(46.3320756406617,12.402359822038,-159.476024489131));
#155274=CARTESIAN_POINT('Ctrl Pts',(46.3403466525113,12.4023895161759,-159.491612730368));
#155275=CARTESIAN_POINT('Ctrl Pts',(46.349506689406,12.4024223895878,-159.508877614243));
#155276=CARTESIAN_POINT('Ctrl Pts',(46.3569477569657,12.4024490777728,-159.522903319776));
#155277=CARTESIAN_POINT('Ctrl Pts',(46.3571037555989,12.4024496372785,-159.523197362381));
#155278=CARTESIAN_POINT('Ctrl Pts',(46.3572589987558,12.4024501940669,-159.52348998131));
#155279=CARTESIAN_POINT('Ctrl Pts',(46.3574134624099,12.4024507480515,-159.523781131265));
#155280=CARTESIAN_POINT('Ctrl Pts',(47.0115330056625,12.4047967511373,-160.756737044912));
#155281=CARTESIAN_POINT('Ctrl Pts',(47.6760241215332,12.4071159777989,-162.015036767565));
#155282=CARTESIAN_POINT('Ctrl Pts',(48.3508610839072,12.4094057510675,-163.298706080169));
#155283=CARTESIAN_POINT('Ctrl Pts',(49.0067945063899,12.411631383184,-164.54641723486));
#155284=CARTESIAN_POINT('Ctrl Pts',(49.6725021575915,12.4138291854533,-165.818096645811));
#155285=CARTESIAN_POINT('Ctrl Pts',(50.3480029624884,12.4159976714344,-167.113744493829));
#155286=CARTESIAN_POINT('Ctrl Pts',(51.0235037673853,12.4181661574155,-168.409392341847));
#155287=CARTESIAN_POINT('Ctrl Pts',(51.7087974034322,12.4203053190432,-169.729008804884));
#155288=CARTESIAN_POINT('Ctrl Pts',(52.4039495302269,12.4224147476539,-171.07256826174));
#155289=CARTESIAN_POINT('Origin',(0.,-12.9675000200281,-170.64995));
#155290=CARTESIAN_POINT('Ctrl Pts',(50.2136602208993,18.26999998,-171.64995));
#155291=CARTESIAN_POINT('Ctrl Pts',(50.0851229429831,18.23650101235,-171.64995));
#155292=CARTESIAN_POINT('Ctrl Pts',(49.9746389296368,18.2070601321017,-171.626166638551));
#155293=CARTESIAN_POINT('Ctrl Pts',(49.8399940956355,18.1718227588537,-171.580545385988));
#155294=CARTESIAN_POINT('Ctrl Pts',(49.8001480569663,18.1614733076846,-171.563607489984));
#155295=CARTESIAN_POINT('Ctrl Pts',(49.7475533787961,18.1478385799374,-171.538010641032));
#155296=CARTESIAN_POINT('Ctrl Pts',(49.7312137127225,18.1436060874251,-171.52944037697));
#155297=CARTESIAN_POINT('Ctrl Pts',(49.7084205773179,18.1376844316008,-171.516772700281));
#155298=CARTESIAN_POINT('Ctrl Pts',(49.6974529329991,18.1348302609285,-171.510485215015));
#155299=CARTESIAN_POINT('Ctrl Pts',(49.6853910445521,18.1316770648567,-171.503278490686));
#155300=CARTESIAN_POINT('Ctrl Pts',(49.6803770252153,18.1303624489092,-171.500222192265));
#155301=CARTESIAN_POINT('Ctrl Pts',(49.6770686640073,18.1294940830886,-171.498192352673));
#155302=CARTESIAN_POINT('Ctrl Pts',(49.6765960425098,18.1293702666764,-171.497905072835));
#155303=CARTESIAN_POINT('Ctrl Pts',(49.4956122808246,18.08175492675,-171.38540529848));
#155304=CARTESIAN_POINT('Ctrl Pts',(49.3699326913236,18.0484851821909,-171.23007999248));
#155305=CARTESIAN_POINT('Ctrl Pts',(49.2955572616308,18.0287857662077,-171.07256826174));
#155306=CARTESIAN_POINT('',(52.5103993912271,12.4456688534684,-171.249463176903));
#155307=CARTESIAN_POINT('Origin',(53.2802565113079,12.6131588410718,-170.642164399514));
#155308=CARTESIAN_POINT('',(52.1126146143195,13.5388501432916,-171.391638125813));
#155309=CARTESIAN_POINT('Ctrl Pts',(52.5103994272594,12.4456688709067,-171.249463146917));
#155310=CARTESIAN_POINT('Ctrl Pts',(52.4789249293047,12.5214873830577,-171.255734050496));
#155311=CARTESIAN_POINT('Ctrl Pts',(52.4475912597577,12.5988603052281,-171.263156330074));
#155312=CARTESIAN_POINT('Ctrl Pts',(52.4165030218133,12.6778243900594,-171.271682853797));
#155313=CARTESIAN_POINT('Ctrl Pts',(52.387020598463,12.7527097078642,-171.279768953194));
#155314=CARTESIAN_POINT('Ctrl Pts',(52.3577589616042,12.8290260178364,-171.288848248172));
#155315=CARTESIAN_POINT('Ctrl Pts',(52.3288066421888,12.9068196706831,-171.298836409739));
#155316=CARTESIAN_POINT('Ctrl Pts',(52.3006266608301,12.9825380839679,-171.308558125043));
#155317=CARTESIAN_POINT('Ctrl Pts',(52.2727397648527,13.0596559839818,-171.319141098433));
#155318=CARTESIAN_POINT('Ctrl Pts',(52.2452261612323,13.1382317037553,-171.330462085915));
#155319=CARTESIAN_POINT('Ctrl Pts',(52.2187662336855,13.2137982446139,-171.341349518645));
#155320=CARTESIAN_POINT('Ctrl Pts',(52.1926515942531,13.2907130439262,-171.352919627189));
#155321=CARTESIAN_POINT('Ctrl Pts',(52.1669516021167,13.3690434713394,-171.365017856694));
#155322=CARTESIAN_POINT('Ctrl Pts',(52.1486202360554,13.4249152292384,-171.373647317457));
#155323=CARTESIAN_POINT('Ctrl Pts',(52.1304997930493,13.4815075305005,-171.382544571252));
#155324=CARTESIAN_POINT('Ctrl Pts',(52.1126146143195,13.5388501432916,-171.391638125813));
#155325=CARTESIAN_POINT('Ctrl Pts',(52.1126146143195,13.5388501432916,-171.391638125814));
#155326=CARTESIAN_POINT('Ctrl Pts',(52.0803920632866,13.6421605599748,-171.408021385403));
#155327=CARTESIAN_POINT('Ctrl Pts',(52.0443154341228,13.7573997650724,-171.425325387943));
#155328=CARTESIAN_POINT('Ctrl Pts',(52.0042475791589,13.8846776632875,-171.442931430639));
#155329=CARTESIAN_POINT('Ctrl Pts',(51.9673088889449,14.0020155856068,-171.459162500599));
#155330=CARTESIAN_POINT('Ctrl Pts',(51.926977620903,14.1295858261524,-171.475647125295));
#155331=CARTESIAN_POINT('Ctrl Pts',(51.8831362090135,14.2674563385285,-171.491883525028));
#155332=CARTESIAN_POINT('Ctrl Pts',(51.8417138631109,14.3977194803224,-171.507224038415));
#155333=CARTESIAN_POINT('Ctrl Pts',(51.7971595353686,14.5371723996994,-171.522339825733));
#155334=CARTESIAN_POINT('Ctrl Pts',(51.7493757816615,14.6858287519608,-171.536828313229));
#155335=CARTESIAN_POINT('Ctrl Pts',(51.7077663335838,14.8152766979877,-171.549444692676));
#155336=CARTESIAN_POINT('Ctrl Pts',(51.6637081429747,14.9517026484988,-171.561584593079));
#155337=CARTESIAN_POINT('Ctrl Pts',(51.617135700075,15.0950969115951,-171.57301932221));
#155338=CARTESIAN_POINT('Ctrl Pts',(51.6010267119545,15.144695694415,-171.576974491925));
#155339=CARTESIAN_POINT('Ctrl Pts',(51.584616911503,15.1951280068941,-171.580845702717));
#155340=CARTESIAN_POINT('Ctrl Pts',(51.5679035198677,15.2463930815758,-171.584624968275));
#155341=CARTESIAN_POINT('Ctrl Pts',(51.5659904551147,15.2522610352249,-171.585057554304));
#155342=CARTESIAN_POINT('Ctrl Pts',(51.5645241366347,15.2567580002418,-171.58538800781));
#155343=CARTESIAN_POINT('Ctrl Pts',(51.5621523934156,15.2640296730528,-171.585919105761));
#155344=CARTESIAN_POINT('Ctrl Pts',(51.5620922592179,15.264214042173,-171.585932571447));
#155345=CARTESIAN_POINT('Ctrl Pts',(51.5620321292168,15.2643983974826,-171.585946034188));
#155346=CARTESIAN_POINT('Ctrl Pts',(51.5619720034126,15.2645827389817,-171.585959493986));
#155347=CARTESIAN_POINT('Ctrl Pts',(51.5100296192924,15.4238344458647,-171.597587346801));
#155348=CARTESIAN_POINT('Ctrl Pts',(51.4612187298276,15.5727959713245,-171.606956492029));
#155349=CARTESIAN_POINT('Ctrl Pts',(51.4156249289144,15.7114071757297,-171.614568164852));
#155350=CARTESIAN_POINT('Ctrl Pts',(51.370285212554,15.8492459293811,-171.62213741944));
#155351=CARTESIAN_POINT('Ctrl Pts',(51.3281260757772,15.9768490948217,-171.627969257248));
#155352=CARTESIAN_POINT('Ctrl Pts',(51.2891960739576,16.0941513344784,-171.632521761146));
#155353=CARTESIAN_POINT('Ctrl Pts',(51.2529325860679,16.2034189468185,-171.636762440885));
#155354=CARTESIAN_POINT('Ctrl Pts',(51.2194703342734,16.3037482407608,-171.639893258602));
#155355=CARTESIAN_POINT('Ctrl Pts',(51.1888281668638,16.3950846110292,-171.642249337767));
#155356=CARTESIAN_POINT('Ctrl Pts',(51.1597260909545,16.4818303671407,-171.644486999149));
#155357=CARTESIAN_POINT('Ctrl Pts',(51.1332014685273,16.5604778447485,-171.646031796051));
#155358=CARTESIAN_POINT('Ctrl Pts',(51.1093286900604,16.6310287376919,-171.647132271588));
#155359=CARTESIAN_POINT('Ctrl Pts',(51.0855300937576,16.701360401109,-171.648229327512));
#155360=CARTESIAN_POINT('Ctrl Pts',(51.0643670215595,16.7636457950945,-171.648884851425));
#155361=CARTESIAN_POINT('Ctrl Pts',(51.0459071806312,16.8178871170319,-171.649293646808));
#155362=CARTESIAN_POINT('Ctrl Pts',(51.0273959299895,16.8722794982784,-171.649703580665));
#155363=CARTESIAN_POINT('Ctrl Pts',(51.0116030939921,16.9185829775746,-171.649865392466));
#155364=CARTESIAN_POINT('Ctrl Pts',(50.9985891037783,16.9567994635462,-171.649923556513));
#155365=CARTESIAN_POINT('Ctrl Pts',(50.9943621183234,16.9692122998618,-171.649942448381));
#155366=CARTESIAN_POINT('Ctrl Pts',(50.9904282251185,16.9807719773071,-171.64995));
#155367=CARTESIAN_POINT('Ctrl Pts',(50.9867892914963,16.9914785469432,-171.64995));
#155368=CARTESIAN_POINT('Origin',(0.,-12.9675000200281,-171.64995));
#155369=CARTESIAN_POINT('',(50.4557527353536,20.76999998,-171.64995));
#155370=CARTESIAN_POINT('',(49.6616970192851,26.41999998,-171.64995));
#155371=CARTESIAN_POINT('',(49.6109861057109,26.78082687904,-171.64995));
#155372=CARTESIAN_POINT('',(44.1114262156583,26.41999998,-171.64995));
#155373=CARTESIAN_POINT('',(43.6598261881496,26.41999998,-171.64995));
#155374=CARTESIAN_POINT('',(48.5692718988023,20.76999998,-171.64995));
#155375=CARTESIAN_POINT('Origin',(0.,-12.9675000200281,-171.64995));
#155376=CARTESIAN_POINT('',(50.5260231527048,20.76999998,-171.64995));
#155377=CARTESIAN_POINT('Origin',(0.,-12.9675000200281,-170.64995));
#155378=CARTESIAN_POINT('',(43.1661128544364,26.1158519257145,-171.07256826174));
#155379=CARTESIAN_POINT('Ctrl Pts',(44.1114262156583,26.41999998,-171.64995));
#155380=CARTESIAN_POINT('Ctrl Pts',(44.0862354544475,26.4119589516213,-171.64995));
#155381=CARTESIAN_POINT('Ctrl Pts',(44.062424087661,26.4043528118249,-171.649077188494));
#155382=CARTESIAN_POINT('Ctrl Pts',(44.0400096738348,26.3971890622453,-171.647602355793));
#155383=CARTESIAN_POINT('Ctrl Pts',(44.0325064360514,26.3947909929969,-171.647108654707));
#155384=CARTESIAN_POINT('Ctrl Pts',(44.0251594468187,26.3924424007436,-171.646547173762));
#155385=CARTESIAN_POINT('Ctrl Pts',(44.0179685608018,26.3901433003913,-171.645927118434));
#155386=CARTESIAN_POINT('Ctrl Pts',(43.9954109094669,26.3829310731345,-171.643982018503));
#155387=CARTESIAN_POINT('Ctrl Pts',(43.9743934989977,26.3762072089724,-171.641463268277));
#155388=CARTESIAN_POINT('Ctrl Pts',(43.9549327642172,26.3699786174128,-171.638633940813));
#155389=CARTESIAN_POINT('Ctrl Pts',(43.9350172655692,26.3636044743919,-171.635738496838));
#155390=CARTESIAN_POINT('Ctrl Pts',(43.9167355998369,26.3577501595336,-171.63251895689));
#155391=CARTESIAN_POINT('Ctrl Pts',(43.900061978668,26.3524088423955,-171.629213691978));
#155392=CARTESIAN_POINT('Ctrl Pts',(43.8823343709119,26.3467298855471,-171.625699491956));
#155393=CARTESIAN_POINT('Ctrl Pts',(43.8664272902322,26.3416317152979,-171.622089275396));
#155394=CARTESIAN_POINT('Ctrl Pts',(43.8523110704409,26.337106169398,-171.618620938174));
#155395=CARTESIAN_POINT('Ctrl Pts',(43.8473291598941,26.335509009168,-171.617396889099));
#155396=CARTESIAN_POINT('Ctrl Pts',(43.8425702599821,26.3339831528831,-171.616190046819));
#155397=CARTESIAN_POINT('Ctrl Pts',(43.8380328957014,26.3325281766859,-171.615009325804));
#155398=CARTESIAN_POINT('Ctrl Pts',(43.8361555194993,26.3319261669027,-171.614520791625));
#155399=CARTESIAN_POINT('Ctrl Pts',(43.834316044768,26.3313369484831,-171.614036835203));
#155400=CARTESIAN_POINT('Ctrl Pts',(43.8325143893445,26.3307598347951,-171.613557935536));
#155401=CARTESIAN_POINT('Ctrl Pts',(43.8310448450428,26.3302891043099,-171.613167314628));
#155402=CARTESIAN_POINT('Ctrl Pts',(43.8306220292784,26.3301538547414,-171.613054933854));
#155403=CARTESIAN_POINT('Ctrl Pts',(43.8287460529606,26.3295522868089,-171.61254888948));
#155404=CARTESIAN_POINT('Ctrl Pts',(43.8283220898321,26.3294163348674,-171.61243452548));
#155405=CARTESIAN_POINT('Ctrl Pts',(43.8278239364058,26.3292565744529,-171.612299893551));
#155406=CARTESIAN_POINT('Ctrl Pts',(43.8272228179699,26.3290637741874,-171.612136790524));
#155407=CARTESIAN_POINT('Ctrl Pts',(43.7945831106783,26.3185950481281,-171.603280573905));
#155408=CARTESIAN_POINT('Ctrl Pts',(43.7634524938468,26.3086018031985,-171.593184647393));
#155409=CARTESIAN_POINT('Ctrl Pts',(43.7338613831768,26.2990964255035,-171.582169375343));
#155410=CARTESIAN_POINT('Ctrl Pts',(43.7161500744003,26.2934071264004,-171.575576351961));
#155411=CARTESIAN_POINT('Ctrl Pts',(43.6989893210903,26.287892288612,-171.568653540263));
#155412=CARTESIAN_POINT('Ctrl Pts',(43.682378199249,26.2825521351849,-171.561465632265));
#155413=CARTESIAN_POINT('Ctrl Pts',(43.6621217355773,26.2760400750766,-171.55270032438));
#155414=CARTESIAN_POINT('Ctrl Pts',(43.6426836268837,26.2697877829703,-171.543541205931));
#155415=CARTESIAN_POINT('Ctrl Pts',(43.6240553138662,26.2637931585035,-171.534100818898));
#155416=CARTESIAN_POINT('Ctrl Pts',(43.6118890679869,26.2598780388064,-171.52793525416));
#155417=CARTESIAN_POINT('Ctrl Pts',(43.6000684354351,26.2560728887536,-171.521649806639));
#155418=CARTESIAN_POINT('Ctrl Pts',(43.5885882565054,26.2523762161258,-171.515273953786));
#155419=CARTESIAN_POINT('Ctrl Pts',(43.5858376819236,26.2514905179298,-171.513746341812));
#155420=CARTESIAN_POINT('Ctrl Pts',(43.5831063120073,26.2506109376294,-171.512213345091));
#155421=CARTESIAN_POINT('Ctrl Pts',(43.58039516952,26.2497378068516,-171.510675985829));
#155422=CARTESIAN_POINT('Ctrl Pts',(43.5785452743591,26.249142043107,-171.509626998742));
#155423=CARTESIAN_POINT('Ctrl Pts',(43.5767041725523,26.2485490825943,-171.508575561719));
#155424=CARTESIAN_POINT('Ctrl Pts',(43.5748722248338,26.2479590424451,-171.507522020905));
#155425=CARTESIAN_POINT('Ctrl Pts',(43.5718287594684,26.246978792441,-171.505771744438));
#155426=CARTESIAN_POINT('Ctrl Pts',(43.5693369349477,26.2461761716096,-171.504322744292));
#155427=CARTESIAN_POINT('Ctrl Pts',(43.5663723957617,26.2452212663088,-171.502580705527));
#155428=CARTESIAN_POINT('Ctrl Pts',(43.5647615530418,26.2447023990733,-171.501634133298));
#155429=CARTESIAN_POINT('Ctrl Pts',(43.5630113134971,26.2441386224429,-171.50060039331));
#155430=CARTESIAN_POINT('Ctrl Pts',(43.5609591548336,26.243477566168,-171.499377888939));
#155431=CARTESIAN_POINT('Ctrl Pts',(43.5328624030456,26.2344268361218,-171.482640195843));
#155432=CARTESIAN_POINT('Ctrl Pts',(43.5058766871946,26.2257272700079,-171.464782106444));
#155433=CARTESIAN_POINT('Ctrl Pts',(43.4801111596735,26.2174158381575,-171.445999348312));
#155434=CARTESIAN_POINT('Ctrl Pts',(43.4531619571471,26.2087225769759,-171.426353705408));
#155435=CARTESIAN_POINT('Ctrl Pts',(43.4275474816989,26.2004538833673,-171.405696571767));
#155436=CARTESIAN_POINT('Ctrl Pts',(43.4033381150423,26.1926341561568,-171.384240314257));
#155437=CARTESIAN_POINT('Ctrl Pts',(43.3837824064608,26.1863175800693,-171.366908496987));
#155438=CARTESIAN_POINT('Ctrl Pts',(43.365142364827,26.1802935715868,-171.349055028029));
#155439=CARTESIAN_POINT('Ctrl Pts',(43.3474322736918,26.1745674931452,-171.330786171197));
#155440=CARTESIAN_POINT('Ctrl Pts',(43.3226113547606,26.1665423210721,-171.305182135005));
#155441=CARTESIAN_POINT('Ctrl Pts',(43.2997031859874,26.1591304014692,-171.278951913314));
#155442=CARTESIAN_POINT('Ctrl Pts',(43.2786212075764,26.1523059918628,-171.252199761598));
#155443=CARTESIAN_POINT('Ctrl Pts',(43.2554014801638,26.1447895753422,-171.222734895519));
#155444=CARTESIAN_POINT('Ctrl Pts',(43.2343969539159,26.1379858217079,-171.192637063565));
#155445=CARTESIAN_POINT('Ctrl Pts',(43.2154467008627,26.1318449539662,-171.162094734958));
#155446=CARTESIAN_POINT('Ctrl Pts',(43.1971455897184,26.12591444197,-171.132598635414));
#155447=CARTESIAN_POINT('Ctrl Pts',(43.1807594970827,26.1206018686274,-171.102689012713));
#155448=CARTESIAN_POINT('Ctrl Pts',(43.1661128544364,26.1158519257145,-171.07256826174));
#155449=CARTESIAN_POINT('',(47.6457075325507,20.5094809071607,-171.07256826174));
#155450=CARTESIAN_POINT('Origin',(0.,-12.9675000200281,-171.07256826174));
#155451=CARTESIAN_POINT('Ctrl Pts',(47.6457075325506,20.5094809071606,-171.072568261741));
#155452=CARTESIAN_POINT('Ctrl Pts',(47.6608054793214,20.5137743424238,-171.104353673586));
#155453=CARTESIAN_POINT('Ctrl Pts',(47.6779305040385,20.5186086512811,-171.135995650035));
#155454=CARTESIAN_POINT('Ctrl Pts',(47.6971672417547,20.5240387499795,-171.167206713736));
#155455=CARTESIAN_POINT('Ctrl Pts',(47.7160784704467,20.5293769647964,-171.197889648237));
#155456=CARTESIAN_POINT('Ctrl Pts',(47.7370309269822,20.5352912371008,-171.228155855593));
#155457=CARTESIAN_POINT('Ctrl Pts',(47.7600754969573,20.5418118265715,-171.257699199741));
#155458=CARTESIAN_POINT('Ctrl Pts',(47.7825293088982,20.548165257765,-171.286485186822));
#155459=CARTESIAN_POINT('Ctrl Pts',(47.8069696244586,20.5550945051755,-171.314584515203));
#155460=CARTESIAN_POINT('Ctrl Pts',(47.8334105302321,20.5626033659202,-171.341687271229));
#155461=CARTESIAN_POINT('Ctrl Pts',(47.8549943997946,20.568732893867,-171.363811413112));
#155462=CARTESIAN_POINT('Ctrl Pts',(47.8779108659171,20.5752482720292,-171.385270896185));
#155463=CARTESIAN_POINT('Ctrl Pts',(47.9021486191345,20.5821377906669,-171.405886271163));
#155464=CARTESIAN_POINT('Ctrl Pts',(47.9213820600628,20.5876048464848,-171.422245237825));
#155465=CARTESIAN_POINT('Ctrl Pts',(47.9414471996244,20.5933072712984,-171.438072451705));
#155466=CARTESIAN_POINT('Ctrl Pts',(47.9623296966163,20.5992329574236,-171.453274815853));
#155467=CARTESIAN_POINT('Ctrl Pts',(47.9727709451122,20.6021958004862,-171.460875997927));
#155468=CARTESIAN_POINT('Ctrl Pts',(47.9834165059242,20.6052144399543,-171.468321013392));
#155469=CARTESIAN_POINT('Ctrl Pts',(47.9942636985228,20.6082867262198,-171.475597912193));
#155470=CARTESIAN_POINT('Ctrl Pts',(47.9996872948221,20.6098228693525,-171.479236361594));
#155471=CARTESIAN_POINT('Ctrl Pts',(48.0051612966878,20.6113724225186,-171.482832785671));
#155472=CARTESIAN_POINT('Ctrl Pts',(48.0106853331332,20.6129350916101,-171.486385694791));
#155473=CARTESIAN_POINT('Ctrl Pts',(48.0142592323965,20.613946095424,-171.488684329026));
#155474=CARTESIAN_POINT('Ctrl Pts',(48.0183353267973,20.6150974528436,-171.49126815362));
#155475=CARTESIAN_POINT('Ctrl Pts',(48.0219806198629,20.6161281188114,-171.493545641964));
#155476=CARTESIAN_POINT('Ctrl Pts',(48.0239697138534,20.6166905129581,-171.494788378364));
#155477=CARTESIAN_POINT('Ctrl Pts',(48.0258300378168,20.6172166329018,-171.495940836679));
#155478=CARTESIAN_POINT('Ctrl Pts',(48.0274071543696,20.617662137765,-171.496912392695));
#155479=CARTESIAN_POINT('Ctrl Pts',(48.0507475253393,20.6242553402511,-171.511290834034));
#155480=CARTESIAN_POINT('Ctrl Pts',(48.0756840369207,20.6312829116219,-171.525353615259));
#155481=CARTESIAN_POINT('Ctrl Pts',(48.1022649324158,20.6387735189811,-171.538797793285));
#155482=CARTESIAN_POINT('Ctrl Pts',(48.127917677585,20.6460025697022,-171.551772528201));
#155483=CARTESIAN_POINT('Ctrl Pts',(48.155102381514,20.6536631594268,-171.56417076011));
#155484=CARTESIAN_POINT('Ctrl Pts',(48.1838328927653,20.6617597777488,-171.575687929238));
#155485=CARTESIAN_POINT('Ctrl Pts',(48.193709004373,20.6645429898362,-171.57964695547));
#155486=CARTESIAN_POINT('Ctrl Pts',(48.2037674836592,20.6673775162118,-171.58350160808));
#155487=CARTESIAN_POINT('Ctrl Pts',(48.2140079119365,20.6702628383739,-171.587238716541));
#155488=CARTESIAN_POINT('Ctrl Pts',(48.2258244062378,20.6735922296808,-171.59155098939));
#155489=CARTESIAN_POINT('Ctrl Pts',(48.2378831914308,20.6769892737823,-171.595706763012));
#155490=CARTESIAN_POINT('Ctrl Pts',(48.2501826687628,20.6804524954123,-171.599685179414));
#155491=CARTESIAN_POINT('Ctrl Pts',(48.2563324074288,20.6821841062273,-171.601674387615));
#155492=CARTESIAN_POINT('Ctrl Pts',(48.2625423199986,20.6839322620305,-171.603619253238));
#155493=CARTESIAN_POINT('Ctrl Pts',(48.2688120843098,20.6856966917931,-171.605517102748));
#155494=CARTESIAN_POINT('Ctrl Pts',(48.2719469664653,20.6865789066744,-171.606466027504));
#155495=CARTESIAN_POINT('Ctrl Pts',(48.2750968115901,20.6874651900693,-171.60740319812));
#155496=CARTESIAN_POINT('Ctrl Pts',(48.2782615753499,20.6883555052367,-171.608328278083));
#155497=CARTESIAN_POINT('Ctrl Pts',(48.2806789487674,20.6890355636495,-171.609034891241));
#155498=CARTESIAN_POINT('Ctrl Pts',(48.2839466163799,20.6899543743648,-171.609974943678));
#155499=CARTESIAN_POINT('Ctrl Pts',(48.2861362745438,20.6905703569427,-171.610596209647));
#155500=CARTESIAN_POINT('Ctrl Pts',(48.2868132611247,20.69076080308,-171.610788289274));
#155501=CARTESIAN_POINT('Ctrl Pts',(48.2873870926172,20.6909222321912,-171.610950345128));
#155502=CARTESIAN_POINT('Ctrl Pts',(48.2878005760434,20.6910385077935,-171.611066908152));
#155503=CARTESIAN_POINT('Ctrl Pts',(48.2998125318058,20.6944163877819,-171.614453137937));
#155504=CARTESIAN_POINT('Ctrl Pts',(48.3135201354276,20.6982563100554,-171.618084608787));
#155505=CARTESIAN_POINT('Ctrl Pts',(48.3289584082396,20.7025797409342,-171.621757482605));
#155506=CARTESIAN_POINT('Ctrl Pts',(48.3440560181388,20.7068077704313,-171.625349310317));
#155507=CARTESIAN_POINT('Ctrl Pts',(48.3608093202089,20.7114985927589,-171.628980616122));
#155508=CARTESIAN_POINT('Ctrl Pts',(48.3792439438551,20.7166665888665,-171.632412351309));
#155509=CARTESIAN_POINT('Ctrl Pts',(48.3973413375453,20.7217400453114,-171.63578130876));
#155510=CARTESIAN_POINT('Ctrl Pts',(48.4170597039694,20.7272737927182,-171.638957768871));
#155511=CARTESIAN_POINT('Ctrl Pts',(48.4384078208194,20.7332699884129,-171.641670360648));
#155512=CARTESIAN_POINT('Ctrl Pts',(48.4590004972892,20.7390539982559,-171.644286962629));
#155513=CARTESIAN_POINT('Ctrl Pts',(48.4811101375688,20.7452686573897,-171.646471581729));
#155514=CARTESIAN_POINT('Ctrl Pts',(48.5047220649505,20.7518996505501,-171.647942204836));
#155515=CARTESIAN_POINT('Ctrl Pts',(48.5251264176098,20.7576298529491,-171.649213050372));
#155516=CARTESIAN_POINT('Ctrl Pts',(48.5466525424873,20.7636708901536,-171.64995));
#155517=CARTESIAN_POINT('Ctrl Pts',(48.5692718988023,20.76999998,-171.64995));
#155518=CARTESIAN_POINT('Origin',(0.,-12.9675000200281,-171.64995));
#155519=CARTESIAN_POINT('',(40.7299248988704,26.1062891840346,-167.236334624234));
#155520=CARTESIAN_POINT('Ctrl Pts',(43.1661128544364,26.1158519257145,-171.07256826174));
#155521=CARTESIAN_POINT('Ctrl Pts',(42.3615449736022,26.1127499922191,-169.789073851883));
#155522=CARTESIAN_POINT('Ctrl Pts',(41.5498582787394,26.1095640229222,-168.510069248237));
#155523=CARTESIAN_POINT('Ctrl Pts',(40.7299249439363,26.1062890581356,-167.236334669465));
#155524=CARTESIAN_POINT('',(40.5057713939776,20.481582219525,-158.850240721809));
#155525=CARTESIAN_POINT('Ctrl Pts',(40.7299249270775,26.1062893712214,-167.236334458579));
#155526=CARTESIAN_POINT('Ctrl Pts',(40.7128753097134,25.6648631996692,-166.554593295561));
#155527=CARTESIAN_POINT('Ctrl Pts',(40.6957961482183,25.2264331174374,-165.882453706378));
#155528=CARTESIAN_POINT('Ctrl Pts',(40.6787028125346,24.7909199131761,-165.220009030196));
#155529=CARTESIAN_POINT('Ctrl Pts',(40.6609759030339,24.3392641742899,-164.533010480519));
#155530=CARTESIAN_POINT('Ctrl Pts',(40.6432337524935,23.8907456085251,-163.856438781572));
#155531=CARTESIAN_POINT('Ctrl Pts',(40.6254919034664,23.4452850207497,-163.190342549082));
#155532=CARTESIAN_POINT('Ctrl Pts',(40.607340392364,22.9895386781693,-162.508866050162));
#155533=CARTESIAN_POINT('Ctrl Pts',(40.589189196447,22.5369932474311,-161.838354137871));
#155534=CARTESIAN_POINT('Ctrl Pts',(40.5710532970034,22.0875722018093,-161.178804354429));
#155535=CARTESIAN_POINT('Ctrl Pts',(40.5522933111462,21.6226858317652,-160.496558367787));
#155536=CARTESIAN_POINT('Ctrl Pts',(40.5335496951665,21.1611426591172,-159.826041783126));
#155537=CARTESIAN_POINT('Ctrl Pts',(40.5148372507287,20.7028654660488,-159.167197042055));
#155538=CARTESIAN_POINT('Ctrl Pts',(40.5118264342186,20.6291290526335,-159.061189479517));
#155539=CARTESIAN_POINT('Ctrl Pts',(40.5088164210288,20.5554772043327,-158.955483975447));
#155540=CARTESIAN_POINT('Ctrl Pts',(40.5058072686407,20.4819096145309,-158.850080167922));
#155541=CARTESIAN_POINT('Ctrl Pts',(40.5058324224781,20.4814581622042,-158.850394545255));
#155542=CARTESIAN_POINT('Ctrl Pts',(41.0748559880981,20.4838558671134,-159.794595142241));
#155543=CARTESIAN_POINT('Ctrl Pts',(41.6503757590613,20.4862411501968,-160.757331383121));
#155544=CARTESIAN_POINT('Ctrl Pts',(42.2323582161204,20.488611368542,-161.738653725408));
#155545=CARTESIAN_POINT('Ctrl Pts',(42.7807997999503,20.4908449862182,-162.663420396849));
#155546=CARTESIAN_POINT('Ctrl Pts',(43.3349807509714,20.49306522617,-163.604692509208));
#155547=CARTESIAN_POINT('Ctrl Pts',(43.8949153576922,20.4952702209769,-164.562486402209));
#155548=CARTESIAN_POINT('Ctrl Pts',(44.4451875767377,20.4974371657787,-165.503752336773));
#155549=CARTESIAN_POINT('Ctrl Pts',(45.0010164490219,20.4995893855044,-166.460974849504));
#155550=CARTESIAN_POINT('Ctrl Pts',(45.5624581798033,20.5017254605505,-167.434143383494));
#155551=CARTESIAN_POINT('Ctrl Pts',(46.1111612276046,20.5038130696894,-168.385231468596));
#155552=CARTESIAN_POINT('Ctrl Pts',(46.6652252369269,20.5058852574484,-169.35155022864));
#155553=CARTESIAN_POINT('Ctrl Pts',(47.2247453462289,20.5079410566878,-170.333063732337));
#155554=CARTESIAN_POINT('Ctrl Pts',(47.3647237291413,20.5084553678775,-170.578614644217));
#155555=CARTESIAN_POINT('Ctrl Pts',(47.5050438144344,20.5089686551722,-170.825116431323));
#155556=CARTESIAN_POINT('Ctrl Pts',(47.6457075325507,20.5094809071607,-171.07256826174));
#155557=CARTESIAN_POINT('Ctrl Pts',(40.731736456874,26.153205299378,-167.30881038206));
#155558=CARTESIAN_POINT('Ctrl Pts',(39.,27.3939818557438,-166.473551654334));
#155559=CARTESIAN_POINT('Ctrl Pts',(39.,29.2922017208088,-165.195719073356));
#155560=CARTESIAN_POINT('Ctrl Pts',(40.6299762644379,23.5169690803201,-163.235292522563));
#155561=CARTESIAN_POINT('Ctrl Pts',(39.,24.7554502365011,-162.409295569182));
#155562=CARTESIAN_POINT('Ctrl Pts',(39.,26.5499900188717,-161.122164521183));
#155563=CARTESIAN_POINT('Ctrl Pts',(40.5197424781718,20.796012087217,-159.207512241208));
#155564=CARTESIAN_POINT('Ctrl Pts',(39.,22.0110917831,-158.367042514669));
#155565=CARTESIAN_POINT('Ctrl Pts',(39.,23.7045860616975,-157.09431111324));
#155566=CARTESIAN_POINT('Ctrl Pts',(40.4018086326459,17.9622435375657,-155.312616930242));
#155567=CARTESIAN_POINT('Ctrl Pts',(39.,19.1149982856394,-154.428325504224));
#155568=CARTESIAN_POINT('Ctrl Pts',(39.,20.7168513145423,-153.199525621538));
#155569=CARTESIAN_POINT('',(39.,26.4199999800005,-161.0070032805));
#155570=CARTESIAN_POINT('Ctrl Pts',(40.7299249051676,26.1062890609606,-167.236334613664));
#155571=CARTESIAN_POINT('Ctrl Pts',(40.6655599724143,26.1109551454916,-167.143655159795));
#155572=CARTESIAN_POINT('Ctrl Pts',(40.6012807827827,26.1158462415184,-167.04650897417));
#155573=CARTESIAN_POINT('Ctrl Pts',(40.537493215085,26.1209674811084,-166.944795556906));
#155574=CARTESIAN_POINT('Ctrl Pts',(40.4777242273763,26.1257660855567,-166.849490026288));
#155575=CARTESIAN_POINT('Ctrl Pts',(40.4183871223425,26.1307667543264,-166.750174501842));
#155576=CARTESIAN_POINT('Ctrl Pts',(40.3597727647597,26.1359727718707,-166.646784924028));
#155577=CARTESIAN_POINT('Ctrl Pts',(40.3479006562068,26.1370272303339,-166.625843769989));
#155578=CARTESIAN_POINT('Ctrl Pts',(40.3360580421242,26.1380901098204,-166.604735545593));
#155579=CARTESIAN_POINT('Ctrl Pts',(40.3242470923055,26.1391614322574,-166.583459825004));
#155580=CARTESIAN_POINT('Ctrl Pts',(40.2707276546541,26.144015959222,-166.487052286319));
#155581=CARTESIAN_POINT('Ctrl Pts',(40.2178676814488,26.149043399969,-166.387213933017));
#155582=CARTESIAN_POINT('Ctrl Pts',(40.1658599746533,26.1542433904085,-166.283952280357));
#155583=CARTESIAN_POINT('Ctrl Pts',(40.1156927673743,26.1592593585082,-166.184344951902));
#155584=CARTESIAN_POINT('Ctrl Pts',(40.0663183755085,26.1644359186199,-166.081551558006));
#155585=CARTESIAN_POINT('Ctrl Pts',(40.0178686966096,26.1697714290785,-165.975604902816));
#155586=CARTESIAN_POINT('Ctrl Pts',(39.9942719299905,26.1723700179225,-165.924005004665));
#155587=CARTESIAN_POINT('Ctrl Pts',(39.970893821805,26.1750062938622,-165.871657468398));
#155588=CARTESIAN_POINT('Ctrl Pts',(39.947745464702,26.1776799753113,-165.818567904404));
#155589=CARTESIAN_POINT('Ctrl Pts',(39.9458414957153,26.1778998875296,-165.81420124966));
#155590=CARTESIAN_POINT('Ctrl Pts',(39.9434731024443,26.1781740861158,-165.808756672598));
#155591=CARTESIAN_POINT('Ctrl Pts',(39.9420381705474,26.1783405694635,-165.805452905768));
#155592=CARTESIAN_POINT('Ctrl Pts',(39.9396836723283,26.1786137425294,-165.800031942491));
#155593=CARTESIAN_POINT('Ctrl Pts',(39.9373283981638,26.1788876628891,-165.794595981622));
#155594=CARTESIAN_POINT('Ctrl Pts',(39.9349723995142,26.1791623310232,-165.789145019958));
#155595=CARTESIAN_POINT('Ctrl Pts',(39.8799745860375,26.1855741117791,-165.661899203024));
#155596=CARTESIAN_POINT('Ctrl Pts',(39.8246694294618,26.1923956775984,-165.526432930152));
#155597=CARTESIAN_POINT('Ctrl Pts',(39.7698978587332,26.1996375838493,-165.38261840114));
#155598=CARTESIAN_POINT('Ctrl Pts',(39.7354995937025,26.2041857282102,-165.292298364332));
#155599=CARTESIAN_POINT('Ctrl Pts',(39.7013112109897,26.208899657812,-165.198685786783));
#155600=CARTESIAN_POINT('Ctrl Pts',(39.6675307141268,26.2137818117656,-165.101752901681));
#155601=CARTESIAN_POINT('Ctrl Pts',(39.6585869831338,26.2150744118065,-165.076088931958));
#155602=CARTESIAN_POINT('Ctrl Pts',(39.6496737175069,26.2163784633357,-165.050197692129));
#155603=CARTESIAN_POINT('Ctrl Pts',(39.6407939407845,26.2176940491621,-165.024077536311));
#155604=CARTESIAN_POINT('Ctrl Pts',(39.6156806967495,26.2214147089198,-164.9502061015));
#155605=CARTESIAN_POINT('Ctrl Pts',(39.5908206081619,26.2252310634679,-164.874435432396));
#155606=CARTESIAN_POINT('Ctrl Pts',(39.5663133697914,26.2291410756515,-164.796805863973));
#155607=CARTESIAN_POINT('Ctrl Pts',(39.5524797752985,26.2313481592157,-164.7529863216));
#155608=CARTESIAN_POINT('Ctrl Pts',(39.53875962603,26.2335849133149,-164.708577884265));
#155609=CARTESIAN_POINT('Ctrl Pts',(39.5251684492104,26.2358513676767,-164.663579935738));
#155610=CARTESIAN_POINT('Ctrl Pts',(39.4871369769279,26.2421934672154,-164.537664552922));
#155611=CARTESIAN_POINT('Ctrl Pts',(39.4501045438397,26.2487694405955,-164.407107098214));
#155612=CARTESIAN_POINT('Ctrl Pts',(39.4144495932088,26.2555781438501,-164.271929512584));
#155613=CARTESIAN_POINT('Ctrl Pts',(39.4131963919402,26.2558174563553,-164.267178286771));
#155614=CARTESIAN_POINT('Ctrl Pts',(39.411617445666,26.2561199480258,-164.261173555401));
#155615=CARTESIAN_POINT('Ctrl Pts',(39.4106951136031,26.2562969839952,-164.257658721375));
#155616=CARTESIAN_POINT('Ctrl Pts',(39.4088599785172,26.2566492268935,-164.250665366703));
#155617=CARTESIAN_POINT('Ctrl Pts',(39.4070210670069,26.2570035280093,-164.243631152948));
#155618=CARTESIAN_POINT('Ctrl Pts',(39.4051786186454,26.2573598846844,-164.236556132581));
#155619=CARTESIAN_POINT('Ctrl Pts',(39.3805910621168,26.2621154805938,-164.142139666509));
#155620=CARTESIAN_POINT('Ctrl Pts',(39.3553405852739,26.2672382778453,-164.040433634314));
#155621=CARTESIAN_POINT('Ctrl Pts',(39.3299788857907,26.2727306896172,-163.931389102773));
#155622=CARTESIAN_POINT('Ctrl Pts',(39.3266758216188,26.273446011891,-163.917187330312));
#155623=CARTESIAN_POINT('Ctrl Pts',(39.3233709423668,26.274167604002,-163.902861072933));
#155624=CARTESIAN_POINT('Ctrl Pts',(39.3200655291253,26.2748954716567,-163.888410214473));
#155625=CARTESIAN_POINT('Ctrl Pts',(39.3047720495629,26.2782631683074,-163.821549010632));
#155626=CARTESIAN_POINT('Ctrl Pts',(39.2894667835075,26.2817651925946,-163.752020734357));
#155627=CARTESIAN_POINT('Ctrl Pts',(39.2742814104456,26.2854018053583,-163.679819977838));
#155628=CARTESIAN_POINT('Ctrl Pts',(39.2666887239147,26.2872201117401,-163.643719599579));
#155629=CARTESIAN_POINT('Ctrl Pts',(39.2591260938889,26.2890720658277,-163.606951088395));
#155630=CARTESIAN_POINT('Ctrl Pts',(39.251610560464,26.2909576680051,-163.569514400177));
#155631=CARTESIAN_POINT('Ctrl Pts',(39.2478527937515,26.2919004690937,-163.550796056068));
#155632=CARTESIAN_POINT('Ctrl Pts',(39.2441068051003,26.2928516822406,-163.531910666905));
#155633=CARTESIAN_POINT('Ctrl Pts',(39.2403747510816,26.2938113064648,-163.512858247065));
#155634=CARTESIAN_POINT('Ctrl Pts',(39.2385087240722,26.2942911185769,-163.503332037144));
#155635=CARTESIAN_POINT('Ctrl Pts',(39.236646180934,26.29477303346,-163.493764069515));
#155636=CARTESIAN_POINT('Ctrl Pts',(39.2347873929698,26.2952570508672,-163.484154348409));
#155637=CARTESIAN_POINT('Ctrl Pts',(39.2329286050057,26.2957410682743,-163.474544627303));
#155638=CARTESIAN_POINT('Ctrl Pts',(39.2308289096148,26.2962917205444,-163.463611919718));
#155639=CARTESIAN_POINT('Ctrl Pts',(39.229222566815,26.2967154103779,-163.455199929581));
#155640=CARTESIAN_POINT('Ctrl Pts',(39.2035210820178,26.3034944477151,-163.320608087395));
#155641=CARTESIAN_POINT('Ctrl Pts',(39.1800429123288,26.3103754712095,-163.185641273895));
#155642=CARTESIAN_POINT('Ctrl Pts',(39.1587671982296,26.3172370503909,-163.050400347168));
#155643=CARTESIAN_POINT('Ctrl Pts',(39.14812934118,26.3206678399816,-162.982779883805));
#155644=CARTESIAN_POINT('Ctrl Pts',(39.1380423077006,26.324090233778,-162.915090776103));
#155645=CARTESIAN_POINT('Ctrl Pts',(39.1285006561278,26.3274858217589,-162.847345445333));
#155646=CARTESIAN_POINT('Ctrl Pts',(39.1237298303414,26.3291836157494,-162.813472779947));
#155647=CARTESIAN_POINT('Ctrl Pts',(39.1190953150477,26.3308747058532,-162.77958606057));
#155648=CARTESIAN_POINT('Ctrl Pts',(39.1145962130836,26.3325568340628,-162.745686816459));
#155649=CARTESIAN_POINT('Ctrl Pts',(39.1123466621015,26.3333978981676,-162.728737194403));
#155650=CARTESIAN_POINT('Ctrl Pts',(39.1101309623961,26.3342367217452,-162.711784441201));
#155651=CARTESIAN_POINT('Ctrl Pts',(39.1079489892389,26.3350730241177,-162.694828747083));
#155652=CARTESIAN_POINT('Ctrl Pts',(39.1068580026604,26.3354911753039,-162.686350900024));
#155653=CARTESIAN_POINT('Ctrl Pts',(39.1057754475934,26.3359086961896,-162.677872317734));
#155654=CARTESIAN_POINT('Ctrl Pts',(39.1047013076557,26.3363255518907,-162.669393023875));
#155655=CARTESIAN_POINT('Ctrl Pts',(39.1036271677181,26.3367424075918,-162.660913730015));
#155656=CARTESIAN_POINT('Ctrl Pts',(39.1027440700184,26.3370868304298,-162.653898670079));
#155657=CARTESIAN_POINT('Ctrl Pts',(39.1015019249879,26.3375872893148,-162.643953286364));
#155658=CARTESIAN_POINT('Ctrl Pts',(39.1011118171303,26.3377444633473,-162.640829840841));
#155659=CARTESIAN_POINT('Ctrl Pts',(39.1007231163658,26.337901530053,-162.63770854998));
#155660=CARTESIAN_POINT('Ctrl Pts',(39.1003358168758,26.338058489386,-162.634589414424));
#155661=CARTESIAN_POINT('Ctrl Pts',(39.0803022287851,26.3461774224188,-162.473247924084));
#155662=CARTESIAN_POINT('Ctrl Pts',(39.0640224933764,26.3540091540096,-162.317671311841));
#155663=CARTESIAN_POINT('Ctrl Pts',(39.050841126827,26.3615481992926,-162.16793193425));
#155664=CARTESIAN_POINT('Ctrl Pts',(39.038312448885,26.3687139411743,-162.025607052378));
#155665=CARTESIAN_POINT('Ctrl Pts',(39.028583270636,26.3756152663121,-161.888555596263));
#155666=CARTESIAN_POINT('Ctrl Pts',(39.0211340241148,26.3822478553176,-161.756834054055));
#155667=CARTESIAN_POINT('Ctrl Pts',(39.0132828087732,26.389238345484,-161.618004685198));
#155668=CARTESIAN_POINT('Ctrl Pts',(39.0079635979443,26.3959305221126,-161.485092013288));
#155669=CARTESIAN_POINT('Ctrl Pts',(39.004619214619,26.4023211247915,-161.358161599385));
#155670=CARTESIAN_POINT('Ctrl Pts',(39.0013874364463,26.4084965563252,-161.235504923639));
#155671=CARTESIAN_POINT('Ctrl Pts',(39.,26.4143903824311,-161.118434406696));
#155672=CARTESIAN_POINT('Ctrl Pts',(39.,26.4199999800001,-161.0070032805));
#155673=CARTESIAN_POINT('',(39.,20.76999998,-153.26884421004));
#155674=CARTESIAN_POINT('Ctrl Pts',(39.,20.76999998,-153.26884421004));
#155675=CARTESIAN_POINT('Ctrl Pts',(39.,22.7129810391408,-155.80421523086));
#155676=CARTESIAN_POINT('Ctrl Pts',(39.,24.5896725049001,-158.389029259702));
#155677=CARTESIAN_POINT('Ctrl Pts',(39.,26.4199999800001,-161.0070032805));
#155678=CARTESIAN_POINT('Ctrl Pts',(39.,20.76999998,-153.26884421004));
#155679=CARTESIAN_POINT('Ctrl Pts',(39.,20.765569632395,-153.354826102789));
#155680=CARTESIAN_POINT('Ctrl Pts',(39.000895533927,20.7608738301319,-153.445942320504));
#155681=CARTESIAN_POINT('Ctrl Pts',(39.0030485079457,20.7559119024773,-153.542200055545));
#155682=CARTESIAN_POINT('Ctrl Pts',(39.0050920925181,20.7512020830759,-153.633567076506));
#155683=CARTESIAN_POINT('Ctrl Pts',(39.0082687993418,20.7462524949737,-153.729566394896));
#155684=CARTESIAN_POINT('Ctrl Pts',(39.0129322676218,20.7410628868451,-153.830197762011));
#155685=CARTESIAN_POINT('Ctrl Pts',(39.0176588317899,20.7358030642508,-153.932190653446));
#155686=CARTESIAN_POINT('Ctrl Pts',(39.0239128232778,20.7302964639597,-154.038946012008));
#155687=CARTESIAN_POINT('Ctrl Pts',(39.0321077416871,20.7245446460313,-154.150428276652));
#155688=CARTESIAN_POINT('Ctrl Pts',(39.0387151242647,20.7199070816687,-154.2403139761));
#155689=CARTESIAN_POINT('Ctrl Pts',(39.0465852621392,20.7151100444308,-154.333273737209));
#155690=CARTESIAN_POINT('Ctrl Pts',(39.0559563911723,20.7101549630931,-154.429277186451));
#155691=CARTESIAN_POINT('Ctrl Pts',(39.0606419556888,20.7076774224243,-154.477278911072));
#155692=CARTESIAN_POINT('Ctrl Pts',(39.0657030530557,20.7051603870308,-154.526041243959));
#155693=CARTESIAN_POINT('Ctrl Pts',(39.0711711665567,20.7026041131822,-154.575558899896));
#155694=CARTESIAN_POINT('Ctrl Pts',(39.0739052233071,20.701325976258,-154.600317727865));
#155695=CARTESIAN_POINT('Ctrl Pts',(39.0767410490255,20.7000380317247,-154.625265347961));
#155696=CARTESIAN_POINT('Ctrl Pts',(39.0796826780972,20.6987403179556,-154.650400978073));
#155697=CARTESIAN_POINT('Ctrl Pts',(39.0811534926331,20.698091461071,-154.66296879313));
#155698=CARTESIAN_POINT('Ctrl Pts',(39.0826507590311,20.6974401619388,-154.675583609516));
#155699=CARTESIAN_POINT('Ctrl Pts',(39.0841749877846,20.6967864256737,-154.688245323403));
#155700=CARTESIAN_POINT('Ctrl Pts',(39.0849371021613,20.6964595575411,-154.694576180347));
#155701=CARTESIAN_POINT('Ctrl Pts',(39.085705957183,20.6961320801321,-154.700918761536));
#155702=CARTESIAN_POINT('Ctrl Pts',(39.0864816170269,20.6958039941128,-154.707273053476));
#155703=CARTESIAN_POINT('Ctrl Pts',(39.0866755319878,20.695721972608,-154.708861626461));
#155704=CARTESIAN_POINT('Ctrl Pts',(39.0868698722512,20.6956399130652,-154.710450931365));
#155705=CARTESIAN_POINT('Ctrl Pts',(39.0870646388221,20.695557815495,-154.712040967975));
#155706=CARTESIAN_POINT('Ctrl Pts',(39.0871154522388,20.695536396737,-154.71245579888));
#155707=CARTESIAN_POINT('Ctrl Pts',(39.0871666636068,20.6955148202132,-154.712873684999));
#155708=CARTESIAN_POINT('Ctrl Pts',(39.0872155866559,20.6954942166411,-154.71327272705));
#155709=CARTESIAN_POINT('Ctrl Pts',(39.0877292261227,20.6952779012655,-154.717462239963));
#155710=CARTESIAN_POINT('Ctrl Pts',(39.0880559398794,20.6951404556704,-154.720124228289));
#155711=CARTESIAN_POINT('Ctrl Pts',(39.0888290754381,20.6948179109104,-154.726371047678));
#155712=CARTESIAN_POINT('Ctrl Pts',(39.1032547849822,20.6887996428716,-154.842928617782));
#155713=CARTESIAN_POINT('Ctrl Pts',(39.1186282597997,20.6830712546896,-154.952455676747));
#155714=CARTESIAN_POINT('Ctrl Pts',(39.134360699675,20.6776783755399,-155.054965099396));
#155715=CARTESIAN_POINT('Ctrl Pts',(39.149697365566,20.6724211626496,-155.154895738147));
#155716=CARTESIAN_POINT('Ctrl Pts',(39.1653749029401,20.6674827203699,-155.248157397457));
#155717=CARTESIAN_POINT('Ctrl Pts',(39.1808956676299,20.6629012978552,-155.334756337397));
#155718=CARTESIAN_POINT('Ctrl Pts',(39.1959260131881,20.6584646373607,-155.41861895746));
#155719=CARTESIAN_POINT('Ctrl Pts',(39.2108092257903,20.6543627114732,-155.496233284115));
#155720=CARTESIAN_POINT('Ctrl Pts',(39.2251413518476,20.6506275356373,-155.567599290605));
#155721=CARTESIAN_POINT('Ctrl Pts',(39.2355153047439,20.6479239215311,-155.619255798981));
#155722=CARTESIAN_POINT('Ctrl Pts',(39.2456015006244,20.6454123949607,-155.667638558048));
#155723=CARTESIAN_POINT('Ctrl Pts',(39.2552637406475,20.643104533941,-155.712745444566));
#155724=CARTESIAN_POINT('Ctrl Pts',(39.2680118953415,20.640059591027,-155.772258514591));
#155725=CARTESIAN_POINT('Ctrl Pts',(39.2800324810176,20.6373401949117,-155.826093537767));
#155726=CARTESIAN_POINT('Ctrl Pts',(39.2910799593509,20.6349262020915,-155.874282959093));
#155727=CARTESIAN_POINT('Ctrl Pts',(39.3021027512786,20.6325176035164,-155.922364697602));
#155728=CARTESIAN_POINT('Ctrl Pts',(39.3121567697338,20.6304130796149,-155.964826035607));
#155729=CARTESIAN_POINT('Ctrl Pts',(39.3210492571792,20.6285942725498,-156.001691614201));
#155730=CARTESIAN_POINT('Ctrl Pts',(39.3299517023356,20.6267734288042,-156.038598474471));
#155731=CARTESIAN_POINT('Ctrl Pts',(39.337690840516,20.6252374529696,-156.069898858172));
#155732=CARTESIAN_POINT('Ctrl Pts',(39.3441271348021,20.6239671595869,-156.095616105163));
#155733=CARTESIAN_POINT('Ctrl Pts',(39.3473452819451,20.6233320128956,-156.108474728658));
#155734=CARTESIAN_POINT('Ctrl Pts',(39.3502385260851,20.6227633384985,-156.119937477056));
#155735=CARTESIAN_POINT('Ctrl Pts',(39.3527941980629,20.622259172562,-156.130006632794));
#155736=CARTESIAN_POINT('Ctrl Pts',(39.3540720340518,20.6220070895937,-156.135041210662));
#155737=CARTESIAN_POINT('Ctrl Pts',(39.3552655223485,20.6217711483625,-156.139727379426));
#155738=CARTESIAN_POINT('Ctrl Pts',(39.3563733761272,20.621551129286,-156.144065382332));
#155739=CARTESIAN_POINT('Ctrl Pts',(39.3569273030166,20.6214411197478,-156.146234383785));
#155740=CARTESIAN_POINT('Ctrl Pts',(39.3574598241068,20.6213350916515,-156.148316343098));
#155741=CARTESIAN_POINT('Ctrl Pts',(39.3579707959811,20.6212330217096,-156.150311286952));
#155742=CARTESIAN_POINT('Ctrl Pts',(39.3580064486167,20.6212258998647,-156.150450482492));
#155743=CARTESIAN_POINT('Ctrl Pts',(39.3580419963212,20.6212187973118,-156.150589254327));
#155744=CARTESIAN_POINT('Ctrl Pts',(39.3580774390432,20.6212117140468,-156.150727602449));
#155745=CARTESIAN_POINT('Ctrl Pts',(39.3582959780233,20.6211680388036,-156.151580653676));
#155746=CARTESIAN_POINT('Ctrl Pts',(39.358510531579,20.6211250965916,-156.152417601068));
#155747=CARTESIAN_POINT('Ctrl Pts',(39.3587210872467,20.6210828864843,-156.153238442282));
#155748=CARTESIAN_POINT('Ctrl Pts',(39.3588434390735,20.6210583586063,-156.153715425035));
#155749=CARTESIAN_POINT('Ctrl Pts',(39.3589644411211,20.6210340778222,-156.154186969809));
#155750=CARTESIAN_POINT('Ctrl Pts',(39.35908409128,20.62101004377,-156.154653077003));
#155751=CARTESIAN_POINT('Ctrl Pts',(39.3591140038197,20.621004035257,-156.154769603802));
#155752=CARTESIAN_POINT('Ctrl Pts',(39.3591165961832,20.6210035274588,-156.154779716518));
#155753=CARTESIAN_POINT('Ctrl Pts',(39.3591122924758,20.6210044063111,-156.154762971055));
#155754=CARTESIAN_POINT('Ctrl Pts',(39.3591090646952,20.6210050654502,-156.154750411958));
#155755=CARTESIAN_POINT('Ctrl Pts',(39.35910195833,20.6210065045819,-156.154722745096));
#155756=CARTESIAN_POINT('Ctrl Pts',(39.3590995907982,20.6210069880885,-156.154713533031));
#155757=CARTESIAN_POINT('Ctrl Pts',(39.3590924882029,20.6210084386082,-156.154685896836));
#155758=CARTESIAN_POINT('Ctrl Pts',(39.3591279622065,20.6210012882107,-156.15482436012));
#155759=CARTESIAN_POINT('Ctrl Pts',(39.3594389855587,20.6209386764191,-156.156035085875));
#155760=CARTESIAN_POINT('Ctrl Pts',(39.3867193814463,20.6154468879403,-156.262229934837));
#155761=CARTESIAN_POINT('Ctrl Pts',(39.4149051829703,20.6100918526737,-156.365212269418));
#155762=CARTESIAN_POINT('Ctrl Pts',(39.4437478087531,20.6048990924637,-156.464947028467));
#155763=CARTESIAN_POINT('Ctrl Pts',(39.4740165754652,20.599449573111,-156.56961323249));
#155764=CARTESIAN_POINT('Ctrl Pts',(39.5050085204789,20.5941787690805,-156.670703053005));
#155765=CARTESIAN_POINT('Ctrl Pts',(39.5364571470437,20.5891098870968,-156.768229841553));
#155766=CARTESIAN_POINT('Ctrl Pts',(39.5527864562365,20.5864779330112,-156.818869416591));
#155767=CARTESIAN_POINT('Ctrl Pts',(39.5692392444004,20.5839003179835,-156.868549206904));
#155768=CARTESIAN_POINT('Ctrl Pts',(39.585780524855,20.5813796851227,-156.917275972421));
#155769=CARTESIAN_POINT('Ctrl Pts',(39.6201299951416,20.576145362194,-157.018461523858));
#155770=CARTESIAN_POINT('Ctrl Pts',(39.6548573299948,20.5711493957629,-157.115517731783));
#155771=CARTESIAN_POINT('Ctrl Pts',(39.6896634736143,20.5663740905208,-157.20847470014));
#155772=CARTESIAN_POINT('Ctrl Pts',(39.6947578637932,20.5656751544825,-157.222080317351));
#155773=CARTESIAN_POINT('Ctrl Pts',(39.699853985679,20.5649809455337,-157.235598197776));
#155774=CARTESIAN_POINT('Ctrl Pts',(39.7049509461478,20.5642914082257,-157.249028514624));
#155775=CARTESIAN_POINT('Ctrl Pts',(39.7249112786228,20.5615910941841,-157.301623309337));
#155776=CARTESIAN_POINT('Ctrl Pts',(39.7448842807308,20.5589617603203,-157.352874077829));
#155777=CARTESIAN_POINT('Ctrl Pts',(39.7648181882144,20.5563964561493,-157.402789407317));
#155778=CARTESIAN_POINT('Ctrl Pts',(39.7747851419562,20.5551138040638,-157.427747072061));
#155779=CARTESIAN_POINT('Ctrl Pts',(39.7847423349863,20.5538471666677,-157.45237087167));
#155780=CARTESIAN_POINT('Ctrl Pts',(39.7946836004314,20.5525954318246,-157.47666203141));
#155781=CARTESIAN_POINT('Ctrl Pts',(39.7996542331539,20.5519695644031,-157.488807611281));
#155782=CARTESIAN_POINT('Ctrl Pts',(39.8046208849858,20.5513474231558,-157.500870030787));
#155783=CARTESIAN_POINT('Ctrl Pts',(39.809582796279,20.5507288654499,-157.512849444999));
#155784=CARTESIAN_POINT('Ctrl Pts',(39.8120637519256,20.5504195865969,-157.518839152105));
#155785=CARTESIAN_POINT('Ctrl Pts',(39.8145435224991,20.5501112036634,-157.524808107863));
#155786=CARTESIAN_POINT('Ctrl Pts',(39.8170220141739,20.5498036980508,-157.530756332126));
#155787=CARTESIAN_POINT('Ctrl Pts',(39.8188462490901,20.54957736585,-157.535134381284));
#155788=CARTESIAN_POINT('Ctrl Pts',(39.8202180487261,20.5494074771205,-157.538420409514));
#155789=CARTESIAN_POINT('Ctrl Pts',(39.8221344968241,20.5491704280015,-157.543001012365));
#155790=CARTESIAN_POINT('Ctrl Pts',(39.8228218255829,20.549085410997,-157.544643832787));
#155791=CARTESIAN_POINT('Ctrl Pts',(39.823579329211,20.5489917564752,-157.546453148038));
#155792=CARTESIAN_POINT('Ctrl Pts',(39.8244535178766,20.5488837732778,-157.548538842568));
#155793=CARTESIAN_POINT('Ctrl Pts',(39.8725663581697,20.5429406873756,-157.663329495599));
#155794=CARTESIAN_POINT('Ctrl Pts',(39.9217743356622,20.5371890374606,-157.774410745202));
#155795=CARTESIAN_POINT('Ctrl Pts',(39.971892926282,20.5316291232997,-157.881779625474));
#155796=CARTESIAN_POINT('Ctrl Pts',(40.0244146734342,20.5258026145705,-157.994296779528));
#155797=CARTESIAN_POINT('Ctrl Pts',(40.0779363679974,20.5201866679455,-158.102737051431));
#155798=CARTESIAN_POINT('Ctrl Pts',(40.1321925265671,20.5147804320522,-158.207119649317));
#155799=CARTESIAN_POINT('Ctrl Pts',(40.1883659720449,20.509183152311,-158.315190886312));
#155800=CARTESIAN_POINT('Ctrl Pts',(40.2453263822506,20.5038106595684,-158.418912739766));
#155801=CARTESIAN_POINT('Ctrl Pts',(40.3027268245705,20.4986608268383,-158.518328841652));
#155802=CARTESIAN_POINT('Ctrl Pts',(40.3638454627555,20.4931774063171,-158.62418476393));
#155803=CARTESIAN_POINT('Ctrl Pts',(40.4254626820068,20.4879464200038,-158.725159169806));
#155804=CARTESIAN_POINT('Ctrl Pts',(40.4871059726323,20.4829640792563,-158.821327714668));
#155805=CARTESIAN_POINT('Ctrl Pts',(40.4933177444275,20.4824620106059,-158.831018583674));
#155806=CARTESIAN_POINT('Ctrl Pts',(40.4995297413823,20.4819624659268,-158.840660668463));
#155807=CARTESIAN_POINT('Ctrl Pts',(40.5057414544625,20.4814654407574,-158.850254057419));
#155808=CARTESIAN_POINT('Origin',(39.,46.91999998,-129.34995));
#155809=CARTESIAN_POINT('',(39.,26.419999980009,-71.0516396909899));
#155810=CARTESIAN_POINT('',(39.,26.41999998,-129.34995));
#155811=CARTESIAN_POINT('',(39.,20.769999979994,-78.7897987614735));
#155812=CARTESIAN_POINT('Ctrl Pts',(39.,26.4199999800115,-71.0516396909898));
#155813=CARTESIAN_POINT('Ctrl Pts',(39.,24.5896727691867,-73.6696133337874));
#155814=CARTESIAN_POINT('Ctrl Pts',(39.,22.7129807779577,-76.2544280814611));
#155815=CARTESIAN_POINT('Ctrl Pts',(39.,20.769999979994,-78.7897987614735));
#155816=CARTESIAN_POINT('',(39.,20.76999998,-129.34995));
#155817=CARTESIAN_POINT('Ctrl Pts',(39.,29.2922016634715,-66.8629239833248));
#155818=CARTESIAN_POINT('Ctrl Pts',(39.,27.39376514223,-65.5849455541034));
#155819=CARTESIAN_POINT('Ctrl Pts',(40.7320633148745,26.1529710718006,-64.749675035773));
#155820=CARTESIAN_POINT('Ctrl Pts',(39.,26.5499956507371,-70.9364700811645));
#155821=CARTESIAN_POINT('Ctrl Pts',(39.,24.7552520476619,-69.6491930963147));
#155822=CARTESIAN_POINT('Ctrl Pts',(40.6302860195927,23.5167393131936,-68.8231852344136));
#155823=CARTESIAN_POINT('Ctrl Pts',(39.,23.7045900978902,-74.9643266004363));
#155824=CARTESIAN_POINT('Ctrl Pts',(38.9999999999314,22.0109048679673,-73.6914516653908));
#155825=CARTESIAN_POINT('Ctrl Pts',(40.5200331454484,20.7957836646288,-72.8509648236473));
#155826=CARTESIAN_POINT('Ctrl Pts',(39.,20.7168512667374,-78.8591174122859));
#155827=CARTESIAN_POINT('Ctrl Pts',(39.,19.1148189506652,-77.6301799952506));
#155828=CARTESIAN_POINT('Ctrl Pts',(40.402078446557,17.9620216308036,-76.7458559111338));
#155829=CARTESIAN_POINT('',(40.7299248988739,26.1062891840432,-64.8223083472515));
#155830=CARTESIAN_POINT('Ctrl Pts',(39.,26.4199999800114,-71.0516396909892));
#155831=CARTESIAN_POINT('Ctrl Pts',(39.,26.4157490575532,-70.9671977910182));
#155832=CARTESIAN_POINT('Ctrl Pts',(39.0007946432884,26.4112648461199,-70.8771641690186));
#155833=CARTESIAN_POINT('Ctrl Pts',(39.0027282692707,26.4065088388894,-70.7815280985075));
#155834=CARTESIAN_POINT('Ctrl Pts',(39.0046332133543,26.4018233785582,-70.687310618824));
#155835=CARTESIAN_POINT('Ctrl Pts',(39.007643552267,26.3968741379737,-70.5876556369414));
#155836=CARTESIAN_POINT('Ctrl Pts',(39.0121385956576,26.391622622828,-70.4825592333295));
#155837=CARTESIAN_POINT('Ctrl Pts',(39.0141929022949,26.389222596514,-70.4345284979758));
#155838=CARTESIAN_POINT('Ctrl Pts',(39.0165580098215,26.3867594115903,-70.3853613380078));
#155839=CARTESIAN_POINT('Ctrl Pts',(39.0192737374602,26.3842292724267,-70.3350578600083));
#155840=CARTESIAN_POINT('Ctrl Pts',(39.0255147686812,26.3784147432784,-70.2194551124234));
#155841=CARTESIAN_POINT('Ctrl Pts',(39.0336033940894,26.3722556372242,-70.0978543729413));
#155842=CARTESIAN_POINT('Ctrl Pts',(39.0440550436964,26.3657732814451,-69.9702982548804));
#155843=CARTESIAN_POINT('Ctrl Pts',(39.0459036608686,26.364626726149,-69.947736990474));
#155844=CARTESIAN_POINT('Ctrl Pts',(39.0478263334364,26.3634700624251,-69.9249894362222));
#155845=CARTESIAN_POINT('Ctrl Pts',(39.0498260809213,26.3623034136746,-69.9020558523985));
#155846=CARTESIAN_POINT('Ctrl Pts',(39.0564790072074,26.3584221095613,-69.8257584979552));
#155847=CARTESIAN_POINT('Ctrl Pts',(39.0639844336357,26.3544316715932,-69.7474029129631));
#155848=CARTESIAN_POINT('Ctrl Pts',(39.072455105127,26.3503463271069,-69.6670050750542));
#155849=CARTESIAN_POINT('Ctrl Pts',(39.0766904408726,26.3483036548637,-69.6268061560997));
#155850=CARTESIAN_POINT('Ctrl Pts',(39.0811671665333,26.3462372639141,-69.5860966794539));
#155851=CARTESIAN_POINT('Ctrl Pts',(39.0858996117955,26.3441497520647,-69.5448792292923));
#155852=CARTESIAN_POINT('Ctrl Pts',(39.0882658344266,26.34310599614,-69.5242705042115));
#155853=CARTESIAN_POINT('Ctrl Pts',(39.0906959906315,26.3420569598266,-69.503534785651));
#155854=CARTESIAN_POINT('Ctrl Pts',(39.0931918854002,26.3410029962426,-69.4826724165355));
#155855=CARTESIAN_POINT('Ctrl Pts',(39.0944398327845,26.3404760144507,-69.4722412319778));
#155856=CARTESIAN_POINT('Ctrl Pts',(39.0957042150142,26.3399478008273,-69.4617783847725));
#155857=CARTESIAN_POINT('Ctrl Pts',(39.0969852581247,26.3394184025146,-69.4512839199201));
#155858=CARTESIAN_POINT('Ctrl Pts',(39.0980249587679,26.3389887403419,-69.4427665626448));
#155859=CARTESIAN_POINT('Ctrl Pts',(39.0992517705288,26.3384865966415,-69.4328046918058));
#155860=CARTESIAN_POINT('Ctrl Pts',(39.1002372416259,26.3380865818,-69.4248647839529));
#155861=CARTESIAN_POINT('Ctrl Pts',(39.1004659959578,26.3379937276025,-69.423021717909));
#155862=CARTESIAN_POINT('Ctrl Pts',(39.1006816275985,26.3379063756034,-69.4212875849205));
#155863=CARTESIAN_POINT('Ctrl Pts',(39.1008785926738,26.3378267085406,-69.419705717698));
#155864=CARTESIAN_POINT('Ctrl Pts',(39.1176064072507,26.3310607585165,-69.2853611819927));
#155865=CARTESIAN_POINT('Ctrl Pts',(39.1363872223018,26.3243138583997,-69.1513989218022));
#155866=CARTESIAN_POINT('Ctrl Pts',(39.1573589564869,26.3175651137247,-69.0174031985853));
#155867=CARTESIAN_POINT('Ctrl Pts',(39.1783306906719,26.3108163690497,-68.8834074753684));
#155868=CARTESIAN_POINT('Ctrl Pts',(39.2014945270825,26.3040655661428,-68.7493781443013));
#155869=CARTESIAN_POINT('Ctrl Pts',(39.2270164024943,26.2973852620386,-68.6149087107991));
#155870=CARTESIAN_POINT('Ctrl Pts',(39.2525382779062,26.2907049579344,-68.4804392772969));
#155871=CARTESIAN_POINT('Ctrl Pts',(39.2802448812632,26.2839676825278,-68.346725706618));
#155872=CARTESIAN_POINT('Ctrl Pts',(39.3101294150359,26.2772295950935,-68.2138673363941));
#155873=CARTESIAN_POINT('Ctrl Pts',(39.3250716819223,26.2738605513764,-68.1474381512822));
#155874=CARTESIAN_POINT('Ctrl Pts',(39.3405581607619,26.2704911619849,-68.0812228072504));
#155875=CARTESIAN_POINT('Ctrl Pts',(39.3565820575716,26.2671390609516,-68.0152327345648));
#155876=CARTESIAN_POINT('Ctrl Pts',(39.3645940059764,26.265463010435,-67.982237698222));
#155877=CARTESIAN_POINT('Ctrl Pts',(39.3727402743783,26.2637912659535,-67.9492989688229));
#155878=CARTESIAN_POINT('Ctrl Pts',(39.3810197959113,26.2621259619583,-67.916417922894));
#155879=CARTESIAN_POINT('Ctrl Pts',(39.3851595566778,26.2612933099607,-67.8999773999296));
#155880=CARTESIAN_POINT('Ctrl Pts',(39.3893326286307,26.2604622669912,-67.8835512970938));
#155881=CARTESIAN_POINT('Ctrl Pts',(39.3935388657984,26.2596330936854,-67.8671397821491));
#155882=CARTESIAN_POINT('Ctrl Pts',(39.3956419843822,26.2592185070325,-67.8589340246768));
#155883=CARTESIAN_POINT('Ctrl Pts',(39.3977533941432,26.2588043877234,-67.8507319141284));
#155884=CARTESIAN_POINT('Ctrl Pts',(39.3998730760318,26.2583907680051,-67.8425334712319));
#155885=CARTESIAN_POINT('Ctrl Pts',(39.4014018607501,26.2580924517776,-67.8366204829287));
#155886=CARTESIAN_POINT('Ctrl Pts',(39.4027461781225,26.2578310056885,-67.8314363746657));
#155887=CARTESIAN_POINT('Ctrl Pts',(39.4043141873651,26.2575272307581,-67.8254081776661));
#155888=CARTESIAN_POINT('Ctrl Pts',(39.4049202453754,26.2574098174006,-67.823078193263));
#155889=CARTESIAN_POINT('Ctrl Pts',(39.4055598310341,26.2572860807778,-67.8206221151732));
#155890=CARTESIAN_POINT('Ctrl Pts',(39.4062569470272,26.2571514505613,-67.8179491721346));
#155891=CARTESIAN_POINT('Ctrl Pts',(39.4370469433536,26.2512051461987,-67.6998914784915));
#155892=CARTESIAN_POINT('Ctrl Pts',(39.4688929423544,26.2454344417139,-67.5853212411314));
#155893=CARTESIAN_POINT('Ctrl Pts',(39.5015465506626,26.239841569324,-67.4742814563482));
#155894=CARTESIAN_POINT('Ctrl Pts',(39.5358806442963,26.2339608653447,-67.3575271199869));
#155895=CARTESIAN_POINT('Ctrl Pts',(39.5711074099235,26.2282767546822,-67.2446756972104));
#155896=CARTESIAN_POINT('Ctrl Pts',(39.6069552370405,26.2227890155487,-67.1357214352314));
#155897=CARTESIAN_POINT('Ctrl Pts',(39.6256220886793,26.2199314138341,-67.0789862518927));
#155898=CARTESIAN_POINT('Ctrl Pts',(39.6444576394001,26.217127015129,-67.0233069304515));
#155899=CARTESIAN_POINT('Ctrl Pts',(39.6634255058615,26.2143755290716,-66.9686775345326));
#155900=CARTESIAN_POINT('Ctrl Pts',(39.7022382760887,26.2087453335856,-66.8568927855324));
#155901=CARTESIAN_POINT('Ctrl Pts',(39.7415986105878,26.2033376046449,-66.7495233055924));
#155902=CARTESIAN_POINT('Ctrl Pts',(39.781186051756,26.1981508743513,-66.6465398341847));
#155903=CARTESIAN_POINT('Ctrl Pts',(39.8066514637351,26.1948144065258,-66.5802936599174));
#155904=CARTESIAN_POINT('Ctrl Pts',(39.8322114175671,26.1915693068131,-66.5158608089899));
#155905=CARTESIAN_POINT('Ctrl Pts',(39.8577823212076,26.1884149365567,-66.4532286057725));
#155906=CARTESIAN_POINT('Ctrl Pts',(39.8705677730279,26.1868377514286,-66.4219125041639));
#155907=CARTESIAN_POINT('Ctrl Pts',(39.8833560183902,26.1852832413074,-66.3910464188101));
#155908=CARTESIAN_POINT('Ctrl Pts',(39.8961367846945,26.1837513043075,-66.3606283296588));
#155909=CARTESIAN_POINT('Ctrl Pts',(39.9025271678466,26.1829853358075,-66.3454192850831));
#155910=CARTESIAN_POINT('Ctrl Pts',(39.9089156872528,26.1822250098702,-66.3303222253317));
#155911=CARTESIAN_POINT('Ctrl Pts',(39.9153010704457,26.1814703124786,-66.3153368725879));
#155912=CARTESIAN_POINT('Ctrl Pts',(39.9184937620421,26.1810929637827,-66.307844196216));
#155913=CARTESIAN_POINT('Ctrl Pts',(39.9216856697547,26.1807170222045,-66.3003794462247));
#155914=CARTESIAN_POINT('Ctrl Pts',(39.924876635247,26.1803424859162,-66.2929425863946));
#155915=CARTESIAN_POINT('Ctrl Pts',(39.9264721179931,26.1801552177721,-66.2892241564795));
#155916=CARTESIAN_POINT('Ctrl Pts',(39.9280673651883,26.1799683009501,-66.2855126990972));
#155917=CARTESIAN_POINT('Ctrl Pts',(39.9296623571035,26.179781735215,-66.2818082095887));
#155918=CARTESIAN_POINT('Ctrl Pts',(39.9304598530611,26.1796884523475,-66.2799559648344));
#155919=CARTESIAN_POINT('Ctrl Pts',(39.931257285198,26.1795952572518,-66.2781054620504));
#155920=CARTESIAN_POINT('Ctrl Pts',(39.9320546510499,26.1795021498985,-66.2762567006511));
#155921=CARTESIAN_POINT('Ctrl Pts',(39.9324533339758,26.1794555962218,-66.2753323199515));
#155922=CARTESIAN_POINT('Ctrl Pts',(39.9328520003305,26.1794090644806,-66.2744083745979));
#155923=CARTESIAN_POINT('Ctrl Pts',(39.9332506498063,26.1793625546713,-66.2734848645166));
#155924=CARTESIAN_POINT('Ctrl Pts',(39.9334710477516,26.1793368411886,-66.2729742913521));
#155925=CARTESIAN_POINT('Ctrl Pts',(39.9336914405377,26.1793111344095,-66.2724638512311));
#155926=CARTESIAN_POINT('Ctrl Pts',(39.9339118281128,26.1792854343334,-66.2719535441411));
#155927=CARTESIAN_POINT('Ctrl Pts',(39.9340602477085,26.1792681266657,-66.271609878796));
#155928=CARTESIAN_POINT('Ctrl Pts',(39.9342090065607,26.1792507822761,-66.2712654842615));
#155929=CARTESIAN_POINT('Ctrl Pts',(39.9343519252519,26.1792341213463,-66.2709346606505));
#155930=CARTESIAN_POINT('Ctrl Pts',(39.9343806434435,26.1792307734863,-66.2708681846999));
#155931=CARTESIAN_POINT('Ctrl Pts',(39.9344091968868,26.1792274449355,-66.2708020921554));
#155932=CARTESIAN_POINT('Ctrl Pts',(39.9344375981603,26.179224134224,-66.2707363538339));
#155933=CARTESIAN_POINT('Ctrl Pts',(39.9356927533187,26.1790778218918,-66.26783113927));
#155934=CARTESIAN_POINT('Ctrl Pts',(39.936649858508,26.1789663271907,-66.2656172715509));
#155935=CARTESIAN_POINT('Ctrl Pts',(39.9383996878686,26.1787629094249,-66.2615781509511));
#155936=CARTESIAN_POINT('Ctrl Pts',(39.986566302021,26.1731635377039,-66.150395444895));
#155937=CARTESIAN_POINT('Ctrl Pts',(40.0357321248214,26.1677282386571,-66.0424674068876));
#155938=CARTESIAN_POINT('Ctrl Pts',(40.0857914406382,26.1624582752379,-65.9378193737947));
#155939=CARTESIAN_POINT('Ctrl Pts',(40.1378864073397,26.1569740099346,-65.8289158518348));
#155940=CARTESIAN_POINT('Ctrl Pts',(40.1909489716211,26.1516687995635,-65.7235645048982));
#155941=CARTESIAN_POINT('Ctrl Pts',(40.2448072385024,26.1465429026494,-65.6217708150873));
#155942=CARTESIAN_POINT('Ctrl Pts',(40.3001348611089,26.1412771615403,-65.5172000002484));
#155943=CARTESIAN_POINT('Ctrl Pts',(40.3563019551941,26.1362006462319,-65.4163835080774));
#155944=CARTESIAN_POINT('Ctrl Pts',(40.4130699166274,26.1313124810063,-65.3193043818183));
#155945=CARTESIAN_POINT('Ctrl Pts',(40.4730292450883,26.1261495141332,-65.2167676855708));
#155946=CARTESIAN_POINT('Ctrl Pts',(40.5336587646811,26.1211966671277,-65.1184003258764));
#155947=CARTESIAN_POINT('Ctrl Pts',(40.594622373623,26.1164516892111,-65.0241581730242));
#155948=CARTESIAN_POINT('Ctrl Pts',(40.6395930973415,26.1129514848327,-64.9546390305044));
#155949=CARTESIAN_POINT('Ctrl Pts',(40.6847443924467,26.1095643652524,-64.8873640810613));
#155950=CARTESIAN_POINT('Ctrl Pts',(40.7299249051783,26.1062890609598,-64.8223083578266));
#155951=CARTESIAN_POINT('',(40.5057713943428,20.4815822174724,-73.2084022473292));
#155952=CARTESIAN_POINT('Ctrl Pts',(40.5058072671264,20.4819096069224,-73.2085627982137));
#155953=CARTESIAN_POINT('Ctrl Pts',(40.524433110837,20.9372732015992,-72.5561415754388));
#155954=CARTESIAN_POINT('Ctrl Pts',(40.5430920718079,21.3958644703476,-71.8921575025155));
#155955=CARTESIAN_POINT('Ctrl Pts',(40.5617698100191,21.8577586494764,-71.2165453906544));
#155956=CARTESIAN_POINT('Ctrl Pts',(40.579811750967,22.3039297762911,-70.5639313702585));
#155957=CARTESIAN_POINT('Ctrl Pts',(40.5978712100053,22.753182702484,-69.9004673459997));
#155958=CARTESIAN_POINT('Ctrl Pts',(40.6159337007597,23.2055915895099,-69.2261421324262));
#155959=CARTESIAN_POINT('Ctrl Pts',(40.6335867547941,23.6477453675777,-68.5671023801613));
#155960=CARTESIAN_POINT('Ctrl Pts',(40.6512427049893,24.0929135723843,-67.8976880494934));
#155961=CARTESIAN_POINT('Ctrl Pts',(40.6688865216948,24.5411727272614,-67.2179375596961));
#155962=CARTESIAN_POINT('Ctrl Pts',(40.6860071352838,24.9761393734549,-66.5583441357168));
#155963=CARTESIAN_POINT('Ctrl Pts',(40.7031163227297,25.4140163111681,-65.8890183497114));
#155964=CARTESIAN_POINT('Ctrl Pts',(40.7201989295779,25.8548813945471,-65.2100441331028));
#155965=CARTESIAN_POINT('Ctrl Pts',(40.7234419274554,25.9385761457275,-65.0811462451561));
#155966=CARTESIAN_POINT('Ctrl Pts',(40.7266839631706,26.0223786149058,-64.9519007760722));
#155967=CARTESIAN_POINT('Ctrl Pts',(40.7299249270772,26.1062893712319,-64.8223085129012));
#155968=CARTESIAN_POINT('Ctrl Pts',(40.5057175975614,20.4815025603645,-73.2083776836381));
#155969=CARTESIAN_POINT('Ctrl Pts',(40.5054644120188,20.4815748935818,-73.2086976157026));
#155970=CARTESIAN_POINT('Ctrl Pts',(40.5049011999628,20.4816397337449,-73.2095404184828));
#155971=CARTESIAN_POINT('Ctrl Pts',(40.5040075187888,20.4817138168114,-73.2109184929233));
#155972=CARTESIAN_POINT('Ctrl Pts',(40.5039405013756,20.4817193723222,-73.2110218351295));
#155973=CARTESIAN_POINT('Ctrl Pts',(40.5038716257255,20.4817249801809,-73.2111281875613));
#155974=CARTESIAN_POINT('Ctrl Pts',(40.5038008833269,20.4817306475902,-73.2112375555082));
#155975=CARTESIAN_POINT('Ctrl Pts',(40.5036682413297,20.4817412739827,-73.2114426204088));
#155976=CARTESIAN_POINT('Ctrl Pts',(40.5035290365313,20.4817521097208,-73.2116582867215));
#155977=CARTESIAN_POINT('Ctrl Pts',(40.5033832129991,20.4817632024457,-73.2118845894146));
#155978=CARTESIAN_POINT('Ctrl Pts',(40.5023624482738,20.4818408515203,-73.2134687082665));
#155979=CARTESIAN_POINT('Ctrl Pts',(40.5010173195751,20.4819310487397,-73.2155739780529));
#155980=CARTESIAN_POINT('Ctrl Pts',(40.4993289612953,20.4820504367294,-73.2182126034611));
#155981=CARTESIAN_POINT('Ctrl Pts',(40.4972707721543,20.4821959763739,-73.2214292134824));
#155982=CARTESIAN_POINT('Ctrl Pts',(40.4947024442687,20.482384902843,-73.225438450215));
#155983=CARTESIAN_POINT('Ctrl Pts',(40.4916267542034,20.482620024983,-73.2302425124976));
#155984=CARTESIAN_POINT('Ctrl Pts',(40.4900889091707,20.4827375860529,-73.232644543639));
#155985=CARTESIAN_POINT('Ctrl Pts',(40.4884242433347,20.4828667122259,-73.2352452930148));
#155986=CARTESIAN_POINT('Ctrl Pts',(40.4866332081492,20.4830078607953,-73.2380451199897));
#155987=CARTESIAN_POINT('Ctrl Pts',(40.4848421729637,20.4831490093648,-73.2408449469647));
#155988=CARTESIAN_POINT('Ctrl Pts',(40.4819068550032,20.483384737091,-73.2454372432251));
#155989=CARTESIAN_POINT('Ctrl Pts',(40.4808815266029,20.4834678959463,-73.2470422411145));
#155990=CARTESIAN_POINT('Ctrl Pts',(40.4726788994003,20.4841331667888,-73.2598822242301));
#155991=CARTESIAN_POINT('Ctrl Pts',(40.4643047119547,20.484816592624,-73.2730804680188));
#155992=CARTESIAN_POINT('Ctrl Pts',(40.4561952554549,20.4854831988743,-73.2859475813571));
#155993=CARTESIAN_POINT('Ctrl Pts',(40.442730688993,20.4865900010578,-73.3073115411638));
#155994=CARTESIAN_POINT('Ctrl Pts',(40.4290118058235,20.4877298937745,-73.3293255323986));
#155995=CARTESIAN_POINT('Ctrl Pts',(40.4157123730281,20.4888477046274,-73.3509081883742));
#155996=CARTESIAN_POINT('Ctrl Pts',(40.4129918066602,20.4890763669064,-73.3553231922979));
#155997=CARTESIAN_POINT('Ctrl Pts',(40.4102886284986,20.4893041021319,-73.3597200850662));
#155998=CARTESIAN_POINT('Ctrl Pts',(40.4076083565512,20.4895304334342,-73.3640895164659));
#155999=CARTESIAN_POINT('Ctrl Pts',(40.3918256302552,20.4908631806573,-73.3898188234937));
#156000=CARTESIAN_POINT('Ctrl Pts',(40.3760899149249,20.4922092776769,-73.4158150871827));
#156001=CARTESIAN_POINT('Ctrl Pts',(40.3604066409036,20.4935692425358,-73.442079018916));
#156002=CARTESIAN_POINT('Ctrl Pts',(40.3491586948822,20.4945446008253,-73.4609153464609));
#156003=CARTESIAN_POINT('Ctrl Pts',(40.337580168363,20.4955585440772,-73.4804966048277));
#156004=CARTESIAN_POINT('Ctrl Pts',(40.3264437516604,20.496543538312,-73.4995169658499));
#156005=CARTESIAN_POINT('Ctrl Pts',(40.3220524022774,20.4969319445598,-73.5070171387395));
#156006=CARTESIAN_POINT('Ctrl Pts',(40.3177292467201,20.4973158389473,-73.5144298906698));
#156007=CARTESIAN_POINT('Ctrl Pts',(40.3135195919864,20.4976910410416,-73.5216743800284));
#156008=CARTESIAN_POINT('Ctrl Pts',(40.2837490006234,20.5003444625053,-73.5729072591995));
#156009=CARTESIAN_POINT('Ctrl Pts',(40.2541443566281,20.5030513930188,-73.6252024652474));
#156010=CARTESIAN_POINT('Ctrl Pts',(40.2247473538148,20.5058144906767,-73.6785646287757));
#156011=CARTESIAN_POINT('Ctrl Pts',(40.2100488524082,20.5071960395057,-73.7052457105399));
#156012=CARTESIAN_POINT('Ctrl Pts',(40.1954022357644,20.5085916032087,-73.7321935119101));
#156013=CARTESIAN_POINT('Ctrl Pts',(40.1808127130061,20.5100011562159,-73.7594083654028));
#156014=CARTESIAN_POINT('Ctrl Pts',(40.173517951627,20.5107059327196,-73.7730157921491));
#156015=CARTESIAN_POINT('Ctrl Pts',(40.1662374614079,20.5114142046086,-73.7866899804991));
#156016=CARTESIAN_POINT('Ctrl Pts',(40.1589718843034,20.5121259510964,-73.8004309595697));
#156017=CARTESIAN_POINT('Ctrl Pts',(40.1528035177503,20.5127302132447,-73.8120968457736));
#156018=CARTESIAN_POINT('Ctrl Pts',(40.1461485986819,20.5133861915882,-73.8247609414863));
#156019=CARTESIAN_POINT('Ctrl Pts',(40.1402744482112,20.5139685326086,-73.8360036008295));
#156020=CARTESIAN_POINT('Ctrl Pts',(40.1392295719346,20.5140721176836,-73.838003411371));
#156021=CARTESIAN_POINT('Ctrl Pts',(40.1382092722869,20.5141733704156,-73.8399581997929));
#156022=CARTESIAN_POINT('Ctrl Pts',(40.1372205265763,20.5142715823243,-73.8418542900697));
#156023=CARTESIAN_POINT('Ctrl Pts',(40.0848418236023,20.5194743481513,-73.9422994787208));
#156024=CARTESIAN_POINT('Ctrl Pts',(40.0326909735655,20.5249042925461,-74.0473968589734));
#156025=CARTESIAN_POINT('Ctrl Pts',(39.9811106489698,20.53059114945,-74.15719227979));
#156026=CARTESIAN_POINT('Ctrl Pts',(39.955320486672,20.533434577902,-74.2120899901983));
#156027=CARTESIAN_POINT('Ctrl Pts',(39.9296729235851,20.5363414040528,-74.2681616497415));
#156028=CARTESIAN_POINT('Ctrl Pts',(39.9042093277617,20.5393099926147,-74.3254093376965));
#156029=CARTESIAN_POINT('Ctrl Pts',(39.89147752985,20.5407942868957,-74.354033181674));
#156030=CARTESIAN_POINT('Ctrl Pts',(39.8787916677988,20.5422939996947,-74.3829510163953));
#156031=CARTESIAN_POINT('Ctrl Pts',(39.8661567482737,20.5438085282331,-74.4121628275136));
#156032=CARTESIAN_POINT('Ctrl Pts',(39.8598392885112,20.5445657925023,-74.4267687330727));
#156033=CARTESIAN_POINT('Ctrl Pts',(39.8535345599658,20.5453267592658,-74.4414481316369));
#156034=CARTESIAN_POINT('Ctrl Pts',(39.8472431670729,20.546091336907,-74.4562010097231));
#156035=CARTESIAN_POINT('Ctrl Pts',(39.8440974706264,20.5464736257276,-74.4635774487662));
#156036=CARTESIAN_POINT('Ctrl Pts',(39.8409551077943,20.5468568171812,-74.4709722576226));
#156037=CARTESIAN_POINT('Ctrl Pts',(39.8378161530651,20.5472408983346,-74.4783854335678));
#156038=CARTESIAN_POINT('Ctrl Pts',(39.834677198336,20.5476249794881,-74.485798609513));
#156039=CARTESIAN_POINT('Ctrl Pts',(39.8308803749233,20.5480914147653,-74.4948030605568));
#156040=CARTESIAN_POINT('Ctrl Pts',(39.8284095866455,20.5483957973263,-74.5006800594813));
#156041=CARTESIAN_POINT('Ctrl Pts',(39.8267548791063,20.5485996448687,-74.5046159347301));
#156042=CARTESIAN_POINT('Ctrl Pts',(39.8250994988266,20.5488038771736,-74.5085609314176));
#156043=CARTESIAN_POINT('Ctrl Pts',(39.8234434712545,20.5490084974887,-74.5125150515796));
#156044=CARTESIAN_POINT('Ctrl Pts',(39.7650787544711,20.5562200964616,-74.6518733009648));
#156045=CARTESIAN_POINT('Ctrl Pts',(39.705949287917,20.5639116601681,-74.8025864915926));
#156046=CARTESIAN_POINT('Ctrl Pts',(39.6474445414473,20.5722505834299,-74.9648672153215));
#156047=CARTESIAN_POINT('Ctrl Pts',(39.6282911439158,20.5749805963238,-75.0179949938496));
#156048=CARTESIAN_POINT('Ctrl Pts',(39.6092048952496,20.5777803184013,-75.0723627785656));
#156049=CARTESIAN_POINT('Ctrl Pts',(39.590234879732,20.5806566307811,-75.1279785331065));
#156050=CARTESIAN_POINT('Ctrl Pts',(39.5509555186119,20.5866123303195,-75.2431366522207));
#156051=CARTESIAN_POINT('Ctrl Pts',(39.5121846907435,20.5928834855924,-75.3636377971847));
#156052=CARTESIAN_POINT('Ctrl Pts',(39.4743970636933,20.5994474513941,-75.4894988803743));
#156053=CARTESIAN_POINT('Ctrl Pts',(39.4555032501681,20.602729434295,-75.5524294219692));
#156054=CARTESIAN_POINT('Ctrl Pts',(39.4368554442729,20.6060836803313,-75.616699311578));
#156055=CARTESIAN_POINT('Ctrl Pts',(39.4185130435008,20.6095013265868,-75.682306527728));
#156056=CARTESIAN_POINT('Ctrl Pts',(39.4093418431147,20.6112101497145,-75.715110135803));
#156057=CARTESIAN_POINT('Ctrl Pts',(39.4002469552407,20.6129348140017,-75.7482480687642));
#156058=CARTESIAN_POINT('Ctrl Pts',(39.3912357431359,20.6146737452512,-75.7817197508287));
#156059=CARTESIAN_POINT('Ctrl Pts',(39.3867301370835,20.615543210876,-75.798455591861));
#156060=CARTESIAN_POINT('Ctrl Pts',(39.3822454466591,20.616416242651,-75.8152748697134));
#156061=CARTESIAN_POINT('Ctrl Pts',(39.3777825776534,20.6172926281855,-75.8321775012889));
#156062=CARTESIAN_POINT('Ctrl Pts',(39.3755511431506,20.6177308209527,-75.8406288170767));
#156063=CARTESIAN_POINT('Ctrl Pts',(39.3733251637777,20.6181698521267,-75.8491009712693));
#156064=CARTESIAN_POINT('Ctrl Pts',(39.3711047520856,20.6186096935286,-75.8575939523402));
#156065=CARTESIAN_POINT('Ctrl Pts',(39.3694394433164,20.6189395745801,-75.8639636881434));
#156066=CARTESIAN_POINT('Ctrl Pts',(39.3677772663487,20.6192699113821,-75.8703451390635));
#156067=CARTESIAN_POINT('Ctrl Pts',(39.3661182684645,20.6196006916848,-75.876738299984));
#156068=CARTESIAN_POINT('Ctrl Pts',(39.3655652691698,20.6197109517858,-75.8788693536241));
#156069=CARTESIAN_POINT('Ctrl Pts',(39.364566060937,20.6199104927054,-75.882726903527));
#156070=CARTESIAN_POINT('Ctrl Pts',(39.3644603320247,20.6199316193372,-75.883135364027));
#156071=CARTESIAN_POINT('Ctrl Pts',(39.3632886423492,20.6201657450447,-75.8876619305092));
#156072=CARTESIAN_POINT('Ctrl Pts',(39.3619401943855,20.6204326391343,-75.8928872274733));
#156073=CARTESIAN_POINT('Ctrl Pts',(39.3604179112815,20.6207325043951,-75.8988123848571));
#156074=CARTESIAN_POINT('Ctrl Pts',(39.3561202061195,20.6215790831136,-75.915540271678));
#156075=CARTESIAN_POINT('Ctrl Pts',(39.3504345352844,20.6226880046764,-75.9378370320484));
#156076=CARTESIAN_POINT('Ctrl Pts',(39.3434643999225,20.6240629515274,-75.9657169873842));
#156077=CARTESIAN_POINT('Ctrl Pts',(39.338645331914,20.6250135732928,-75.9849928541872));
#156078=CARTESIAN_POINT('Ctrl Pts',(39.3332133533839,20.6260913571462,-76.0069377298266));
#156079=CARTESIAN_POINT('Ctrl Pts',(39.3272171126794,20.6272975187254,-76.0315582073714));
#156080=CARTESIAN_POINT('Ctrl Pts',(39.3183466318018,20.6290818422292,-76.0679802734658));
#156081=CARTESIAN_POINT('Ctrl Pts',(39.3082381023201,20.6311490838876,-76.1102569728201));
#156082=CARTESIAN_POINT('Ctrl Pts',(39.2970861361385,20.6335337862126,-76.1584224289575));
#156083=CARTESIAN_POINT('Ctrl Pts',(39.2859341699569,20.6359184885376,-76.2065878850949));
#156084=CARTESIAN_POINT('Ctrl Pts',(39.2737387538673,20.638620581188,-76.2606421223469));
#156085=CARTESIAN_POINT('Ctrl Pts',(39.2607519274271,20.6416772034245,-76.320626599082));
#156086=CARTESIAN_POINT('Ctrl Pts',(39.2477651009869,20.6447338256609,-76.3806110758172));
#156087=CARTESIAN_POINT('Ctrl Pts',(39.2339901728747,20.6481374432729,-76.4465224823002));
#156088=CARTESIAN_POINT('Ctrl Pts',(39.2197517386379,20.6518811490863,-76.5183784626765));
#156089=CARTESIAN_POINT('Ctrl Pts',(39.2055133044011,20.6556248548996,-76.5902344430528));
#156090=CARTESIAN_POINT('Ctrl Pts',(39.1908112827616,20.6597090490522,-76.668035292015));
#156091=CARTESIAN_POINT('Ctrl Pts',(39.1760175660153,20.6641379750649,-76.7518070063022));
#156092=CARTESIAN_POINT('Ctrl Pts',(39.1612238492691,20.6685669010776,-76.8355787205894));
#156093=CARTESIAN_POINT('Ctrl Pts',(39.1463417152349,20.6733334101818,-76.9253169916379));
#156094=CARTESIAN_POINT('Ctrl Pts',(39.1318020793478,20.6783942558663,-77.0210185553126));
#156095=CARTESIAN_POINT('Ctrl Pts',(39.1245322614042,20.6809246787086,-77.0688693371499));
#156096=CARTESIAN_POINT('Ctrl Pts',(39.1173488620745,20.6835281179723,-77.1182105829694));
#156097=CARTESIAN_POINT('Ctrl Pts',(39.1103099921676,20.6861952262397,-77.1690393189886));
#156098=CARTESIAN_POINT('Ctrl Pts',(39.1067905572142,20.6875287803734,-77.1944536869981));
#156099=CARTESIAN_POINT('Ctrl Pts',(39.1033072823559,20.6888782545145,-77.2202399296267));
#156100=CARTESIAN_POINT('Ctrl Pts',(39.0998676643283,20.6902421382148,-77.2463974463625));
#156101=CARTESIAN_POINT('Ctrl Pts',(39.0981478553145,20.6909240800649,-77.2594762047304));
#156102=CARTESIAN_POINT('Ctrl Pts',(39.0964389617509,20.6916096244217,-77.2726477817081));
#156103=CARTESIAN_POINT('Ctrl Pts',(39.0947419304685,20.6922985716316,-77.2859120947703));
#156104=CARTESIAN_POINT('Ctrl Pts',(39.0938934148273,20.6926430452366,-77.2925442513014));
#156105=CARTESIAN_POINT('Ctrl Pts',(39.0930478648249,20.6929883695589,-77.2991995918563));
#156106=CARTESIAN_POINT('Ctrl Pts',(39.0922053995177,20.6933345183431,-77.305878105238));
#156107=CARTESIAN_POINT('Ctrl Pts',(39.0913629342106,20.6936806671272,-77.3125566186197));
#156108=CARTESIAN_POINT('Ctrl Pts',(39.0902593691714,20.6941375164164,-77.3213829757033));
#156109=CARTESIAN_POINT('Ctrl Pts',(39.0896873770723,20.6943754114281,-77.3259831523947));
#156110=CARTESIAN_POINT('Ctrl Pts',(39.073847709233,20.700963226138,-77.4533717490315));
#156111=CARTESIAN_POINT('Ctrl Pts',(39.0607443555278,20.70730974043,-77.576098400105));
#156112=CARTESIAN_POINT('Ctrl Pts',(39.0498825952953,20.7134119697754,-77.6941169307647));
#156113=CARTESIAN_POINT('Ctrl Pts',(39.0388132758123,20.7196308076743,-77.8143906978918));
#156114=CARTESIAN_POINT('Ctrl Pts',(39.0300720643756,20.7255959375135,-77.9297747532434));
#156115=CARTESIAN_POINT('Ctrl Pts',(39.0231884656326,20.7313047362494,-78.0402316284843));
#156116=CARTESIAN_POINT('Ctrl Pts',(39.0162316052384,20.7370742933238,-78.1518640883824));
#156117=CARTESIAN_POINT('Ctrl Pts',(39.0111722044164,20.7425820371733,-78.2584640096062));
#156118=CARTESIAN_POINT('Ctrl Pts',(39.007577304562,20.7478257600228,-78.3600031367658));
#156119=CARTESIAN_POINT('Ctrl Pts',(39.0039265968346,20.7531508873704,-78.4631185756265));
#156120=CARTESIAN_POINT('Ctrl Pts',(39.0017862622086,20.7582037355828,-78.5610149408692));
#156121=CARTESIAN_POINT('Ctrl Pts',(39.0007559038223,20.7629824596714,-78.6536722122545));
#156122=CARTESIAN_POINT('Ctrl Pts',(39.0002365147002,20.7653913470468,-78.7003794351757));
#156123=CARTESIAN_POINT('Ctrl Pts',(39.,20.7677305858192,-78.745755534165));
#156124=CARTESIAN_POINT('Ctrl Pts',(39.,20.769999979994,-78.7897987614735));
#156125=CARTESIAN_POINT('Origin',(60.,-2.55003103885676E-14,0.));
#156126=CARTESIAN_POINT('',(60.,27.41999998,-174.34995));
#156127=CARTESIAN_POINT('',(60.,27.91999998,-174.34995));
#156128=CARTESIAN_POINT('',(60.,28.41999998,-174.34995));
#156129=CARTESIAN_POINT('',(60.,27.91999998,-58.24995));
#156130=CARTESIAN_POINT('',(60.,27.91999998,-58.24995));
#156131=CARTESIAN_POINT('',(60.,27.41999998,-58.24995));
#156132=CARTESIAN_POINT('',(60.,-54.58000002,-58.24995));
#156133=CARTESIAN_POINT('',(60.,27.41999998,-174.34995));
#156134=CARTESIAN_POINT('Origin',(57.,-2.42462934179819E-14,-174.34995));
#156135=CARTESIAN_POINT('',(57.,27.91999998,-177.34995));
#156136=CARTESIAN_POINT('',(57.,27.41999998,-177.34995));
#156137=CARTESIAN_POINT('',(57.,-54.58000002,-177.34995));
#156138=CARTESIAN_POINT('Origin',(57.,27.91999998,-174.34995));
#156139=CARTESIAN_POINT('Origin',(57.,27.41999998,-174.34995));
#156140=CARTESIAN_POINT('Origin',(60.,28.41999998,-177.34995));
#156141=CARTESIAN_POINT('',(51.0358975433606,27.41999998,-177.34995));
#156142=CARTESIAN_POINT('',(60.,27.41999998,-177.34995));
#156143=CARTESIAN_POINT('',(50.9656271260094,27.91999998,-177.34995));
#156144=CARTESIAN_POINT('',(51.0717059287548,27.1652100787588,-177.34995));
#156145=CARTESIAN_POINT('',(60.,27.91999998,-177.34995));
#156146=CARTESIAN_POINT('Origin',(0.,-12.9675000200281,-60.64995));
#156147=CARTESIAN_POINT('',(43.0147613882085,26.1152677387813,-61.2273317382593));
#156148=CARTESIAN_POINT('Ctrl Pts',(40.7299249439368,26.1062890581501,-64.8223083020179));
#156149=CARTESIAN_POINT('Ctrl Pts',(41.4984715481572,26.1093587748547,-63.6284010127));
#156150=CARTESIAN_POINT('Ctrl Pts',(42.2597732523974,26.1123503129199,-62.4298580866994));
#156151=CARTESIAN_POINT('Ctrl Pts',(43.0147613882085,26.1152677387813,-61.2273317382593));
#156152=CARTESIAN_POINT('',(47.508501172308,20.508980519813,-61.2273317382593));
#156153=CARTESIAN_POINT('Origin',(0.,-12.9675000200281,-61.2273317382593));
#156154=CARTESIAN_POINT('Ctrl Pts',(47.508501172308,20.508980519813,-61.2273317382593));
#156155=CARTESIAN_POINT('Ctrl Pts',(46.9479652028759,20.506933294733,-62.2124897267371));
#156156=CARTESIAN_POINT('Ctrl Pts',(46.3928886767053,20.5048696025693,-63.1825198713977));
#156157=CARTESIAN_POINT('Ctrl Pts',(45.8431672210077,20.5027903324153,-64.1373805839133));
#156158=CARTESIAN_POINT('Ctrl Pts',(45.2781159650936,20.5006530787213,-65.1188690072553));
#156159=CARTESIAN_POINT('Ctrl Pts',(44.718722664361,20.4984993668521,-66.0843301889488));
#156160=CARTESIAN_POINT('Ctrl Pts',(44.1649210893552,20.4963305571374,-67.0337477577078));
#156161=CARTESIAN_POINT('Ctrl Pts',(43.6014124126742,20.494123732261,-67.9998068336205));
#156162=CARTESIAN_POINT('Ctrl Pts',(43.0436933549281,20.4919012772471,-68.9492550300463));
#156163=CARTESIAN_POINT('Ctrl Pts',(42.4917405921862,20.4896650090889,-69.8821034900559));
#156164=CARTESIAN_POINT('Ctrl Pts',(41.9251450970919,20.4873694150639,-70.8396994488505));
#156165=CARTESIAN_POINT('Ctrl Pts',(41.3646260097972,20.4850592665968,-71.7798033059479));
#156166=CARTESIAN_POINT('Ctrl Pts',(40.810204740074,20.4827369083245,-72.7024556292253));
#156167=CARTESIAN_POINT('Ctrl Pts',(40.7085420530185,20.4823110639438,-72.8716398209669));
#156168=CARTESIAN_POINT('Ctrl Pts',(40.6070845166736,20.4818848099951,-73.0402373040993));
#156169=CARTESIAN_POINT('Ctrl Pts',(40.5058324224785,20.4814581622114,-73.2082484262411));
#156170=CARTESIAN_POINT('Origin',(0.,-12.9675000200281,-60.64995));
#156171=CARTESIAN_POINT('',(36.7055660333102,29.9753365541058,-64.7141088836342));
#156172=CARTESIAN_POINT('',(30.7353086514483,29.741858118838,-73.0207560182717));
#156173=CARTESIAN_POINT('Ctrl Pts',(36.7055660855173,29.9753365749746,-64.7141089388348));
#156174=CARTESIAN_POINT('Ctrl Pts',(36.2220584843733,29.9568079733785,-65.4180278206773));
#156175=CARTESIAN_POINT('Ctrl Pts',(35.7419772179904,29.9382942623995,-66.1100086426196));
#156176=CARTESIAN_POINT('Ctrl Pts',(35.2650854674007,29.9198082912173,-66.7901977895291));
#156177=CARTESIAN_POINT('Ctrl Pts',(34.7683249631423,29.9005521385268,-67.4987256749291));
#156178=CARTESIAN_POINT('Ctrl Pts',(34.2750253842728,29.8813260904984,-68.1944589405539));
#156179=CARTESIAN_POINT('Ctrl Pts',(33.7849656074347,29.8621435250255,-68.8775972447204));
#156180=CARTESIAN_POINT('Ctrl Pts',(33.4153693887468,29.8476763028648,-69.3928105839785));
#156181=CARTESIAN_POINT('Ctrl Pts',(33.0476169663231,29.8332337892929,-69.9008606940659));
#156182=CARTESIAN_POINT('Ctrl Pts',(32.6816291687152,29.8188212963983,-70.4018447451366));
#156183=CARTESIAN_POINT('Ctrl Pts',(32.2720987954213,29.8026941095528,-70.9624322477535));
#156184=CARTESIAN_POINT('Ctrl Pts',(31.8649468060184,29.7866101193311,-71.5139406969673));
#156185=CARTESIAN_POINT('Ctrl Pts',(31.4601541744911,29.7705870470778,-72.0562568439028));
#156186=CARTESIAN_POINT('Ctrl Pts',(31.2177120993998,29.760990363285,-72.3810657504347));
#156187=CARTESIAN_POINT('Ctrl Pts',(30.9761164695227,29.7514154886983,-72.7025782839012));
#156188=CARTESIAN_POINT('Ctrl Pts',(30.7353640256726,29.7418658638113,-73.0207789413775));
#156189=CARTESIAN_POINT('',(30.7601599624812,36.3431985357226,-61.2273317382593));
#156190=CARTESIAN_POINT('Ctrl Pts',(30.7353076117298,29.7418701453522,-73.0207363867594));
#156191=CARTESIAN_POINT('Ctrl Pts',(30.7376555198548,30.3201755188477,-72.011174247587));
#156192=CARTESIAN_POINT('Ctrl Pts',(30.7399863123607,30.9057127448615,-70.982250645273));
#156193=CARTESIAN_POINT('Ctrl Pts',(30.7422975783267,31.4984542632869,-69.933929106915));
#156194=CARTESIAN_POINT('Ctrl Pts',(30.7445647962615,32.0798993332709,-68.9055864460945));
#156195=CARTESIAN_POINT('Ctrl Pts',(30.7468132224327,32.6682765545812,-67.8585780816147));
#156196=CARTESIAN_POINT('Ctrl Pts',(30.7490411044641,33.2636023728865,-66.792894370105));
#156197=CARTESIAN_POINT('Ctrl Pts',(30.7512077501492,33.8425648571132,-65.7565024145669));
#156198=CARTESIAN_POINT('Ctrl Pts',(30.7533549642696,34.4280991321017,-64.7024475949364));
#156199=CARTESIAN_POINT('Ctrl Pts',(30.7554816601947,35.0202624568943,-63.6307456284999));
#156200=CARTESIAN_POINT('Ctrl Pts',(30.7570523555171,35.4576113761063,-62.839228023281));
#156201=CARTESIAN_POINT('Ctrl Pts',(30.7586118691448,35.8985771000441,-62.0380848686548));
#156202=CARTESIAN_POINT('Ctrl Pts',(30.7601599624812,36.3431985357226,-61.2273317382593));
#156203=CARTESIAN_POINT('',(36.7137393100582,32.0861766206928,-61.2273317382593));
#156204=CARTESIAN_POINT('Origin',(0.,-12.9675000200281,-61.2273317382593));
#156205=CARTESIAN_POINT('Ctrl Pts',(36.7137393100582,32.0861766206928,-61.2273317382593));
#156206=CARTESIAN_POINT('Ctrl Pts',(36.7110837808245,31.3874382843756,-62.3925373065787));
#156207=CARTESIAN_POINT('Ctrl Pts',(36.7083607806502,30.6840320430885,-63.5549321813014));
#156208=CARTESIAN_POINT('Ctrl Pts',(36.7055659807394,29.9753365781839,-64.7141088636381));
#156209=CARTESIAN_POINT('Origin',(0.,-12.9675000200281,-171.64995));
#156210=CARTESIAN_POINT('',(38.9938267385724,-56.214502484065,-171.072567687954));
#156211=CARTESIAN_POINT('',(33.5713998621727,-56.0068402847832,-163.25208226359));
#156212=CARTESIAN_POINT('Ctrl Pts',(38.9938273364047,-56.2145025937637,
-171.072567271539));
#156213=CARTESIAN_POINT('Ctrl Pts',(38.5540171403421,-56.1980536322107,
-170.41475390162));
#156214=CARTESIAN_POINT('Ctrl Pts',(38.1169660650788,-56.1815933299574,
-169.766247994682));
#156215=CARTESIAN_POINT('Ctrl Pts',(37.6825967520171,-56.165136805697,-169.127138796781));
#156216=CARTESIAN_POINT('Ctrl Pts',(37.2317386940273,-56.1480555885249,
-168.463768887479));
#156217=CARTESIAN_POINT('Ctrl Pts',(36.7837699246781,-56.1309784443151,
-167.810522543182));
#156218=CARTESIAN_POINT('Ctrl Pts',(36.3386107368843,-56.1139204163073,
-167.167443811692));
#156219=CARTESIAN_POINT('Ctrl Pts',(35.871378908884,-56.0960165881337,-166.492478856456));
#156220=CARTESIAN_POINT('Ctrl Pts',(35.4072422564642,-56.0781338251636,
-165.828714783957));
#156221=CARTESIAN_POINT('Ctrl Pts',(34.9461149698614,-56.0602874301248,
-165.176142950611));
#156222=CARTESIAN_POINT('Ctrl Pts',(34.4849876832587,-56.042441035086,-164.523571117264));
#156223=CARTESIAN_POINT('Ctrl Pts',(34.0268698769957,-56.0246309977758,
-163.882191037155));
#156224=CARTESIAN_POINT('Ctrl Pts',(33.5716804663548,-56.0068706354489,
-163.251940551477));
#156225=CARTESIAN_POINT('',(33.5886122085038,-60.5345771657123,-171.07256826174));
#156226=CARTESIAN_POINT('Ctrl Pts',(33.5712930253539,-56.0068938993568,
-163.252219719633));
#156227=CARTESIAN_POINT('Ctrl Pts',(33.5735544942697,-56.5714984856234,
-164.209913770145));
#156228=CARTESIAN_POINT('Ctrl Pts',(33.5758020709476,-57.1422670958701,
-165.18499894682));
#156229=CARTESIAN_POINT('Ctrl Pts',(33.5780337735611,-57.7192031690627,
-166.177497602729));
#156230=CARTESIAN_POINT('Ctrl Pts',(33.5802053064641,-58.2805842680772,
-167.143237157098));
#156231=CARTESIAN_POINT('Ctrl Pts',(33.5823618086959,-58.8478046711717,
-168.125463912336));
#156232=CARTESIAN_POINT('Ctrl Pts',(33.5845018265016,-59.4209095564351,
-169.124173270749));
#156233=CARTESIAN_POINT('Ctrl Pts',(33.5858788715011,-59.7896874303229,
-169.766816394718));
#156234=CARTESIAN_POINT('Ctrl Pts',(33.5872490985137,-60.1609026711095,
-170.416283768652));
#156235=CARTESIAN_POINT('Ctrl Pts',(33.5886122085038,-60.5345771657124,
-171.07256826174));
#156236=CARTESIAN_POINT('Origin',(0.,-12.9675000200281,-171.07256826174));
#156237=CARTESIAN_POINT('Origin',(-3.54807775957937E-14,-73.08000002,3.11172719585489E-30));
#156238=CARTESIAN_POINT('',(32.85,-73.08000002,-58.24995));
#156239=CARTESIAN_POINT('',(32.35,-73.08000002,-58.24995));
#156240=CARTESIAN_POINT('',(-41.5,-73.0800000199999,-58.24995));
#156241=CARTESIAN_POINT('',(32.35,-73.08000002,-174.34995));
#156242=CARTESIAN_POINT('',(32.35,-73.08000002,-174.34995));
#156243=CARTESIAN_POINT('',(32.85,-73.08000002,-174.34995));
#156244=CARTESIAN_POINT('',(41.5,-73.08000002,-174.34995));
#156245=CARTESIAN_POINT('',(32.85,-73.08000002,-58.24995));
#156246=CARTESIAN_POINT('Origin',(-3.3975957231091E-14,-70.08000002,-174.34995));
#156247=CARTESIAN_POINT('',(32.35,-70.08000002,-177.34995));
#156248=CARTESIAN_POINT('Origin',(32.35,-70.08000002,-174.34995));
#156249=CARTESIAN_POINT('',(32.85,-70.08000002,-177.34995));
#156250=CARTESIAN_POINT('',(-41.5,-70.08000002,-177.34995));
#156251=CARTESIAN_POINT('Origin',(32.85,-70.08000002,-174.34995));
#156252=CARTESIAN_POINT('Origin',(41.5,-73.08000002,-177.34995));
#156253=CARTESIAN_POINT('',(32.35,-65.1329945223129,-177.34995));
#156254=CARTESIAN_POINT('',(32.35,-73.08000002,-177.34995));
#156255=CARTESIAN_POINT('',(32.85,-65.0627241049617,-177.34995));
#156256=CARTESIAN_POINT('',(40.227526467895,-64.0258803771248,-177.34995));
#156257=CARTESIAN_POINT('',(32.85,-73.08000002,-177.34995));
#156258=CARTESIAN_POINT('Origin',(0.,-12.9675000200281,-171.64995));
#156259=CARTESIAN_POINT('',(29.958978566972,-63.954289311524,-171.64995));
#156260=CARTESIAN_POINT('',(31.35,-63.7587939982373,-171.64995));
#156261=CARTESIAN_POINT('',(31.7108268990399,-63.7080830846632,-171.64995));
#156262=CARTESIAN_POINT('',(31.35,-63.1109998882233,-171.64995));
#156263=CARTESIAN_POINT('',(31.35,-62.7949079300497,-171.64995));
#156264=CARTESIAN_POINT('Origin',(0.,-12.9675000200281,-171.64995));
#156265=CARTESIAN_POINT('Ctrl Pts',(33.787119065489,-54.58000002,-74.2342847034403));
#156266=CARTESIAN_POINT('Ctrl Pts',(32.2532076658177,-54.58000002,-73.0155274500394));
#156267=CARTESIAN_POINT('Ctrl Pts',(31.127610916576,-55.9109590653435,-72.1211933947368));
#156268=CARTESIAN_POINT('Ctrl Pts',(31.2221856658751,-54.58000002,-77.4624751982426));
#156269=CARTESIAN_POINT('Ctrl Pts',(29.795197677401,-54.58000002,-76.2393546649806));
#156270=CARTESIAN_POINT('Ctrl Pts',(28.6950527991335,-55.8150223013088,
-75.3493568083322));
#156271=CARTESIAN_POINT('Ctrl Pts',(28.5158034471915,-54.58000002,-80.6345530934811));
#156272=CARTESIAN_POINT('Ctrl Pts',(27.1955581318591,-54.5800000200432,
-79.4258937131132));
#156273=CARTESIAN_POINT('Ctrl Pts',(26.1438256035288,-55.7129660087519,
-78.5213783677229));
#156274=CARTESIAN_POINT('Ctrl Pts',(25.6489781920928,-54.58000002,-83.5984279079175));
#156275=CARTESIAN_POINT('Ctrl Pts',(24.4312617378937,-54.58000002,-82.420584542654));
#156276=CARTESIAN_POINT('Ctrl Pts',(23.4643531971916,-55.6098288961396,
-81.485336599214));
#156277=CARTESIAN_POINT('',(31.3499999999941,-54.58000002,-77.227263173365));
#156278=CARTESIAN_POINT('',(25.7,-54.58000002,-83.5456386250818));
#156279=CARTESIAN_POINT('Ctrl Pts',(31.3499999999855,-54.58000002,-77.227263173365));
#156280=CARTESIAN_POINT('Ctrl Pts',(29.5376330958494,-54.58000002,-79.396334075655));
#156281=CARTESIAN_POINT('Ctrl Pts',(27.6634733215002,-54.58000002,-81.5125991939361));
#156282=CARTESIAN_POINT('Ctrl Pts',(25.7,-54.58000002,-83.5456386250818));
#156283=CARTESIAN_POINT('',(31.0842852491211,-55.9092501930853,-72.1786663403249));
#156284=CARTESIAN_POINT('Ctrl Pts',(31.3500000000008,-54.58000002,-77.2272631733646));
#156285=CARTESIAN_POINT('Ctrl Pts',(31.3453107206565,-54.5800000199999,
-77.1375720242367));
#156286=CARTESIAN_POINT('Ctrl Pts',(31.3403970685239,-54.5810786430591,
-77.0428817158067));
#156287=CARTESIAN_POINT('Ctrl Pts',(31.3352210588623,-54.5836402116848,
-76.9431962742989));
#156288=CARTESIAN_POINT('Ctrl Pts',(31.3300450492006,-54.5862017803106,
-76.843510832791));
#156289=CARTESIAN_POINT('Ctrl Pts',(31.3246066855266,-54.5902459987653,
-76.7388301777383));
#156290=CARTESIAN_POINT('Ctrl Pts',(31.3188661644989,-54.5962369768836,
-76.6291669959942));
#156291=CARTESIAN_POINT('Ctrl Pts',(31.3131256434712,-54.6022279550019,
-76.51950381425));
#156292=CARTESIAN_POINT('Ctrl Pts',(31.3070902307353,-54.6101659107058,
-76.4048625539582));
#156293=CARTESIAN_POINT('Ctrl Pts',(31.3007798943886,-54.6205652232166,
-76.2853053463729));
#156294=CARTESIAN_POINT('Ctrl Pts',(31.2976247262152,-54.6257648794721,
-76.2255267425802));
#156295=CARTESIAN_POINT('Ctrl Pts',(31.2944015900026,-54.6315806184543,
-76.164519829024));
#156296=CARTESIAN_POINT('Ctrl Pts',(31.2911181260652,-54.6380804273865,
-76.1022968571952));
#156297=CARTESIAN_POINT('Ctrl Pts',(31.2894763940964,-54.6413303318526,
-76.0711853712808));
#156298=CARTESIAN_POINT('Ctrl Pts',(31.2878195895528,-54.6447512961395,
-76.0397698784925));
#156299=CARTESIAN_POINT('Ctrl Pts',(31.2861490867532,-54.6483519686845,
-76.0080522698309));
#156300=CARTESIAN_POINT('Ctrl Pts',(31.2853138353534,-54.650152304957,-75.9921934655001));
#156301=CARTESIAN_POINT('Ctrl Pts',(31.284475159829,-54.6519975703892,-75.9762591325628));
#156302=CARTESIAN_POINT('Ctrl Pts',(31.2836332475183,-54.6538888551562,
-75.9602495203746));
#156303=CARTESIAN_POINT('Ctrl Pts',(31.283212291363,-54.6548344975397,-75.9522447142805));
#156304=CARTESIAN_POINT('Ctrl Pts',(31.2827905260398,-54.6557916448769,
-75.9442210883976));
#156305=CARTESIAN_POINT('Ctrl Pts',(31.2823679765381,-54.656760433808,-75.9361786752311));
#156306=CARTESIAN_POINT('Ctrl Pts',(31.2819454270365,-54.657729222739,-75.9281362620647));
#156307=CARTESIAN_POINT('Ctrl Pts',(31.2814519788643,-54.6588736933179,
-75.9187392181045));
#156308=CARTESIAN_POINT('Ctrl Pts',(31.2810980010362,-54.6597018623565,
-75.9119951068502));
#156309=CARTESIAN_POINT('Ctrl Pts',(31.2722272916116,-54.6804558370728,
-75.7429872015412));
#156310=CARTESIAN_POINT('Ctrl Pts',(31.2633507615356,-54.705371481956,-75.574005469165));
#156311=CARTESIAN_POINT('Ctrl Pts',(31.2544854003494,-54.7345127723453,
-75.4053367307167));
#156312=CARTESIAN_POINT('Ctrl Pts',(31.2520303003698,-54.7425829208636,
-75.3586270019613));
#156313=CARTESIAN_POINT('Ctrl Pts',(31.2495760556688,-54.7509768357141,
-75.3119412323424));
#156314=CARTESIAN_POINT('Ctrl Pts',(31.2471230238481,-54.7596951726748,
-75.2652854092562));
#156315=CARTESIAN_POINT('Ctrl Pts',(31.2385625508759,-54.7901200074795,
-75.1024681521939));
#156316=CARTESIAN_POINT('Ctrl Pts',(31.2300160506949,-54.8244995244996,
-74.940017336389));
#156317=CARTESIAN_POINT('Ctrl Pts',(31.2214979294548,-54.862827933893,-74.7781981331342));
#156318=CARTESIAN_POINT('Ctrl Pts',(31.2191128026884,-54.8735601261897,
-74.7328877528154));
#156319=CARTESIAN_POINT('Ctrl Pts',(31.2167299031896,-54.8846016101691,
-74.6876269284716));
#156320=CARTESIAN_POINT('Ctrl Pts',(31.2143495510005,-54.8959515162524,
-74.6424215363045));
#156321=CARTESIAN_POINT('Ctrl Pts',(31.2140609162468,-54.8973277736659,
-74.6369400586917));
#156322=CARTESIAN_POINT('Ctrl Pts',(31.2138228813912,-54.8984661601923,
-74.632419632326));
#156323=CARTESIAN_POINT('Ctrl Pts',(31.2135285145844,-54.8999595685782,
-74.6264903392875));
#156324=CARTESIAN_POINT('Ctrl Pts',(31.2134648969398,-54.9002823193833,
-74.6252089188002));
#156325=CARTESIAN_POINT('Ctrl Pts',(31.2133986476546,-54.9006217246293,
-74.6238616838906));
#156326=CARTESIAN_POINT('Ctrl Pts',(31.2133286878654,-54.9009838833262,
-74.6224247205651));
#156327=CARTESIAN_POINT('Ctrl Pts',(31.2078839743254,-54.9291693650911,
-74.5105911405694));
#156328=CARTESIAN_POINT('Ctrl Pts',(31.2024129074911,-54.9587960031325,
-74.4012817764876));
#156329=CARTESIAN_POINT('Ctrl Pts',(31.1969474187156,-54.9896805561478,
-74.2945231806525));
#156330=CARTESIAN_POINT('Ctrl Pts',(31.1960901136078,-54.994525042367,-74.2777772511894));
#156331=CARTESIAN_POINT('Ctrl Pts',(31.1952329460617,-54.999400523412,-74.2610939879282));
#156332=CARTESIAN_POINT('Ctrl Pts',(31.1943760394873,-55.0043063412549,
-74.2444733920645));
#156333=CARTESIAN_POINT('Ctrl Pts',(31.1896361485215,-55.0314423702774,
-74.1525382680613));
#156334=CARTESIAN_POINT('Ctrl Pts',(31.1849043296596,-55.0595054546659,
-74.0625245652527));
#156335=CARTESIAN_POINT('Ctrl Pts',(31.1802158006127,-55.0883755446775,
-73.9744474139547));
#156336=CARTESIAN_POINT('Ctrl Pts',(31.1743848787859,-55.1242800333362,
-73.8649096508721));
#156337=CARTESIAN_POINT('Ctrl Pts',(31.1686235363137,-55.1614471793065,
-73.7583217249963));
#156338=CARTESIAN_POINT('Ctrl Pts',(31.1630045098354,-55.1996179865692,
-73.6547813901237));
#156339=CARTESIAN_POINT('Ctrl Pts',(31.1576629693929,-55.2359037936395,
-73.5563542180359));
#156340=CARTESIAN_POINT('Ctrl Pts',(31.152450076667,-55.2730964685128,-73.4606804383564));
#156341=CARTESIAN_POINT('Ctrl Pts',(31.1474257337304,-55.3109734535205,
-73.3678004487643));
#156342=CARTESIAN_POINT('Ctrl Pts',(31.1449858887296,-55.3293666989023,
-73.3226974808467));
#156343=CARTESIAN_POINT('Ctrl Pts',(31.1425895372687,-55.3479189876124,
-73.2782350785174));
#156344=CARTESIAN_POINT('Ctrl Pts',(31.1402427759134,-55.3666136886743,
-73.2344049908577));
#156345=CARTESIAN_POINT('Ctrl Pts',(31.1336254850984,-55.4193281555054,
-73.1108149053839));
#156346=CARTESIAN_POINT('Ctrl Pts',(31.1273335379019,-55.4731591730317,
-72.9923884427035));
#156347=CARTESIAN_POINT('Ctrl Pts',(31.1213310258052,-55.5277148075479,
-72.8790684585829));
#156348=CARTESIAN_POINT('Ctrl Pts',(31.1174456970023,-55.5630277856362,
-72.8057182693366));
#156349=CARTESIAN_POINT('Ctrl Pts',(31.1136816088053,-55.5986432025572,
-72.7345071180142));
#156350=CARTESIAN_POINT('Ctrl Pts',(31.1100289108462,-55.6344440246039,
-72.6654155838679));
#156351=CARTESIAN_POINT('Ctrl Pts',(31.103673361896,-55.6967360289041,-72.5451990665901));
#156352=CARTESIAN_POINT('Ctrl Pts',(31.0976553569188,-55.7595906037036,
-72.4314038795334));
#156353=CARTESIAN_POINT('Ctrl Pts',(31.0919676912673,-55.8223273129114,
-72.3238825741213));
#156354=CARTESIAN_POINT('Ctrl Pts',(31.0893364096103,-55.8513511624607,
-72.2741400512662));
#156355=CARTESIAN_POINT('Ctrl Pts',(31.0867758098859,-55.8803490121959,
-72.2257399755741));
#156356=CARTESIAN_POINT('Ctrl Pts',(31.0842850954296,-55.9092502064055,
-72.1786663566349));
#156357=CARTESIAN_POINT('',(25.4680306998147,-55.6875937661705,-79.20421297481));
#156358=CARTESIAN_POINT('Ctrl Pts',(25.4683317135053,-55.6876147553279,
-79.2043632295083));
#156359=CARTESIAN_POINT('Ctrl Pts',(25.860615391601,-55.7029545756699,-78.7454945043951));
#156360=CARTESIAN_POINT('Ctrl Pts',(26.2547029404868,-55.7184229037236,
-78.2773837565957));
#156361=CARTESIAN_POINT('Ctrl Pts',(26.6507273376328,-55.7340096395059,
-77.7999327473883));
#156362=CARTESIAN_POINT('Ctrl Pts',(27.0210025496724,-55.7485829383693,
-77.3535252155626));
#156363=CARTESIAN_POINT('Ctrl Pts',(27.3929707792159,-55.7632597430092,
-76.8989523765739));
#156364=CARTESIAN_POINT('Ctrl Pts',(27.7667262123628,-55.778029204186,-76.4361762559085));
#156365=CARTESIAN_POINT('Ctrl Pts',(28.1285322965327,-55.7923264703655,
-75.9881955679608));
#156366=CARTESIAN_POINT('Ctrl Pts',(28.4920130741863,-55.8067105712765,
-75.5325274217445));
#156367=CARTESIAN_POINT('Ctrl Pts',(28.8572413086363,-55.8211691061762,
-75.0691821389535));
#156368=CARTESIAN_POINT('Ctrl Pts',(29.2247961803246,-55.8357197472236,
-74.6028851774929));
#156369=CARTESIAN_POINT('Ctrl Pts',(29.5941208661498,-55.8503458004071,
-74.1288122836977));
#156370=CARTESIAN_POINT('Ctrl Pts',(29.96527663479,-55.8650317084468,-73.6470279022662));
#156371=CARTESIAN_POINT('Ctrl Pts',(30.3095833935785,-55.8786552536649,
-73.2000952857711));
#156372=CARTESIAN_POINT('Ctrl Pts',(30.6554657752219,-55.8923302944832,
-72.7465266201201));
#156373=CARTESIAN_POINT('Ctrl Pts',(31.0029626442895,-55.9060418772438,
-72.286422310765));
#156374=CARTESIAN_POINT('Ctrl Pts',(31.0300604186516,-55.9071111052251,
-72.250543418413));
#156375=CARTESIAN_POINT('Ctrl Pts',(31.0571680056025,-55.9081805540986,
-72.2146248096625));
#156376=CARTESIAN_POINT('Ctrl Pts',(31.0842854210862,-55.9092502160976,
-72.1786665455479));
#156377=CARTESIAN_POINT('Ctrl Pts',(25.4680306998147,-55.6875937661705,
-79.20421297481));
#156378=CARTESIAN_POINT('Ctrl Pts',(25.4683278290903,-55.6871423789816,
-79.205235636863));
#156379=CARTESIAN_POINT('Ctrl Pts',(25.4685596245448,-55.6842213655928,
-79.2103525600497));
#156380=CARTESIAN_POINT('Ctrl Pts',(25.4692817313297,-55.6758960492355,
-79.224980571896));
#156381=CARTESIAN_POINT('Ctrl Pts',(25.4697672929732,-55.6704183548359,
-79.2346152157047));
#156382=CARTESIAN_POINT('Ctrl Pts',(25.4705320388274,-55.66214441212,-79.2492396837741));
#156383=CARTESIAN_POINT('Ctrl Pts',(25.4709043683141,-55.658198381398,-79.2562346877634));
#156384=CARTESIAN_POINT('Ctrl Pts',(25.4711627415284,-55.6554792098156,
-79.2610599241439));
#156385=CARTESIAN_POINT('Ctrl Pts',(25.4713670581236,-55.6533481293772,
-79.2648467294586));
#156386=CARTESIAN_POINT('Ctrl Pts',(25.472547099263,-55.6410978948656,-79.2866308125499));
#156387=CARTESIAN_POINT('Ctrl Pts',(25.4736967231167,-55.6293072323705,
-79.307839175783));
#156388=CARTESIAN_POINT('Ctrl Pts',(25.4770338679804,-55.5955045885169,
-79.3693302774191));
#156389=CARTESIAN_POINT('Ctrl Pts',(25.4793891057231,-55.5722204188109,
-79.4126816839331));
#156390=CARTESIAN_POINT('Ctrl Pts',(25.4838233290034,-55.5293901492856,
-79.4942352738236));
#156391=CARTESIAN_POINT('Ctrl Pts',(25.4872055392468,-55.497440282494,-79.5564379815909));
#156392=CARTESIAN_POINT('Ctrl Pts',(25.490671225521,-55.4658071514793,-79.6202024646101));
#156393=CARTESIAN_POINT('Ctrl Pts',(25.4929998345068,-55.4447953387203,
-79.6630595960062));
#156394=CARTESIAN_POINT('Ctrl Pts',(25.494272991468,-55.4334480988312,-79.6864995491182));
#156395=CARTESIAN_POINT('Ctrl Pts',(25.4996853335514,-55.3857186867812,
-79.7861924995833));
#156396=CARTESIAN_POINT('Ctrl Pts',(25.504170022895,-55.3477170112747,-79.8690767460442));
#156397=CARTESIAN_POINT('Ctrl Pts',(25.5111409036076,-55.291348542635,-79.9981497038913));
#156398=CARTESIAN_POINT('Ctrl Pts',(25.5146868706228,-55.2633232496154,
-80.0638724996628));
#156399=CARTESIAN_POINT('Ctrl Pts',(25.5189273312081,-55.2309885305297,
-80.1426326343882));
#156400=CARTESIAN_POINT('Ctrl Pts',(25.5210727305464,-55.2149222425954,
-80.1825342051072));
#156401=CARTESIAN_POINT('Ctrl Pts',(25.5219974942784,-55.2080595018384,
-80.1997466864495));
#156402=CARTESIAN_POINT('Ctrl Pts',(25.5226151719892,-55.2034895393514,
-80.2112465257512));
#156403=CARTESIAN_POINT('Ctrl Pts',(25.5230043996644,-55.20062028382,-80.2184954847682));
#156404=CARTESIAN_POINT('Ctrl Pts',(25.530600911193,-55.1447563858798,-80.3600047810412));
#156405=CARTESIAN_POINT('Ctrl Pts',(25.5388664494851,-55.0868589761765,
-80.5174942954816));
#156406=CARTESIAN_POINT('Ctrl Pts',(25.5531250311004,-54.9992784182683,
-80.7851227928128));
#156407=CARTESIAN_POINT('Ctrl Pts',(25.5581822585155,-54.9699767299778,
-80.8795612335467));
#156408=CARTESIAN_POINT('Ctrl Pts',(25.5662146791705,-54.9265911279604,
-81.0291346039942));
#156409=CARTESIAN_POINT('Ctrl Pts',(25.5703415777611,-54.9050412831635,
-81.105899507708));
#156410=CARTESIAN_POINT('Ctrl Pts',(25.5753363913883,-54.880321616272,-81.1989275171106));
#156411=CARTESIAN_POINT('Ctrl Pts',(25.5778761532825,-54.8680895188335,
-81.246308880565));
#156412=CARTESIAN_POINT('Ctrl Pts',(25.5789733849926,-54.8628769662688,
-81.2668010318613));
#156413=CARTESIAN_POINT('Ctrl Pts',(25.5797067823245,-54.85940881693,-81.28050376331));
#156414=CARTESIAN_POINT('Ctrl Pts',(25.58013492075,-54.8573947781028,-81.2885068528041));
#156415=CARTESIAN_POINT('Ctrl Pts',(25.6001616759959,-54.7635577145736,
-81.6630099302082));
#156416=CARTESIAN_POINT('Ctrl Pts',(25.6214848628736,-54.6947552928938,
-82.036220275339));
#156417=CARTESIAN_POINT('Ctrl Pts',(25.6583907318718,-54.6035691563163,
-82.7847463047849));
#156418=CARTESIAN_POINT('Ctrl Pts',(25.6799145825718,-54.5800000497493,
-83.1644838191851));
#156419=CARTESIAN_POINT('Ctrl Pts',(25.7,-54.58000002,-83.5456386250818));
#156420=CARTESIAN_POINT('Origin',(60.,-54.58000002,-55.24995));
#156421=CARTESIAN_POINT('',(25.7,-54.58000002,-148.513004346424));
#156422=CARTESIAN_POINT('',(31.3500000000003,-54.58000002,-154.831379798158));
#156423=CARTESIAN_POINT('Ctrl Pts',(25.7,-54.58000002,-148.513004346424));
#156424=CARTESIAN_POINT('Ctrl Pts',(27.6634746333275,-54.58000002,-150.546045135875));
#156425=CARTESIAN_POINT('Ctrl Pts',(29.537631721855,-54.58000002,-152.662307251431));
#156426=CARTESIAN_POINT('Ctrl Pts',(31.35,-54.58000002,-154.831379798159));
#156427=CARTESIAN_POINT('',(31.35,-54.58000002,-76.6255854122387));
#156428=CARTESIAN_POINT('',(25.7,-54.58000002,-147.999168907581));
#156429=CARTESIAN_POINT('Ctrl Pts',(31.1276111727346,-55.910959075446,-159.937449916708));
#156430=CARTESIAN_POINT('Ctrl Pts',(32.2532079260876,-54.58000002,-159.043115862826));
#156431=CARTESIAN_POINT('Ctrl Pts',(33.7871193355851,-54.58000002,-157.824358608005));
#156432=CARTESIAN_POINT('Ctrl Pts',(28.6950259327511,-55.8150212418279,
-156.709250494305));
#156433=CARTESIAN_POINT('Ctrl Pts',(29.7951706706344,-54.5800000200427,
-155.819252869409));
#156434=CARTESIAN_POINT('Ctrl Pts',(31.2221573047513,-54.58000002,-154.596132061548));
#156435=CARTESIAN_POINT('Ctrl Pts',(26.143809437084,-55.7129653866513,-153.537246733037));
#156436=CARTESIAN_POINT('Ctrl Pts',(27.1955413535444,-54.5800000200432,
-152.632731094415));
#156437=CARTESIAN_POINT('Ctrl Pts',(28.5157861483817,-54.58000002,-151.424072006624));
#156438=CARTESIAN_POINT('Ctrl Pts',(23.4643533331708,-55.6098289013737,
-150.573306522708));
#156439=CARTESIAN_POINT('Ctrl Pts',(24.4312618773724,-54.5800000199999,
-149.638058579956));
#156440=CARTESIAN_POINT('Ctrl Pts',(25.6489783375839,-54.58000002,-148.460215214005));
#156441=CARTESIAN_POINT('',(31.0842852491456,-55.9092501930801,-159.879976631169));
#156442=CARTESIAN_POINT('',(25.4680827049418,-55.6876414657738,-152.854491724755));
#156443=CARTESIAN_POINT('Ctrl Pts',(31.0842854211464,-55.9092502161047,
-159.87997642591));
#156444=CARTESIAN_POINT('Ctrl Pts',(30.7346533861529,-55.8954587801339,
-159.4163569811));
#156445=CARTESIAN_POINT('Ctrl Pts',(30.386656089505,-55.8817029991764,-158.959334162683));
#156446=CARTESIAN_POINT('Ctrl Pts',(30.0402547234154,-55.8679982667367,
-158.509013875888));
#156447=CARTESIAN_POINT('Ctrl Pts',(29.6827133608912,-55.8538528008432,
-158.044211641617));
#156448=CARTESIAN_POINT('Ctrl Pts',(29.3268722787328,-55.8397617134658,
-157.586549708062));
#156449=CARTESIAN_POINT('Ctrl Pts',(28.9726777824063,-55.8257391217459,
-157.136090072484));
#156450=CARTESIAN_POINT('Ctrl Pts',(28.5999643590844,-55.8109833640537,
-156.662078323047));
#156451=CARTESIAN_POINT('Ctrl Pts',(28.2290743062977,-55.7963034531147,
-156.196041547281));
#156452=CARTESIAN_POINT('Ctrl Pts',(27.8599317931223,-55.781712801269,-155.737995624991));
#156453=CARTESIAN_POINT('Ctrl Pts',(27.4782730833951,-55.7666274367858,
-155.264419134997));
#156454=CARTESIAN_POINT('Ctrl Pts',(27.0984824976563,-55.7516374773747,
-154.799384179417));
#156455=CARTESIAN_POINT('Ctrl Pts',(26.7204611045877,-55.7367546582871,
-154.342854013806));
#156456=CARTESIAN_POINT('Ctrl Pts',(26.3230166169315,-55.7211071459622,
-153.86286689906));
#156457=CARTESIAN_POINT('Ctrl Pts',(25.9275279292449,-55.7055780633222,
-153.392280661765));
#156458=CARTESIAN_POINT('Ctrl Pts',(25.5338619724156,-55.6901777816033,
-152.930999011426));
#156459=CARTESIAN_POINT('Ctrl Pts',(25.512012978637,-55.68932304511,-152.90539725508));
#156460=CARTESIAN_POINT('Ctrl Pts',(25.4901695948933,-55.688468704589,-152.879824148347));
#156461=CARTESIAN_POINT('Ctrl Pts',(25.468331796778,-55.6876147615411,-152.854279670573));
#156462=CARTESIAN_POINT('Ctrl Pts',(31.0842850954302,-55.909250206398,-159.879976614859));
#156463=CARTESIAN_POINT('Ctrl Pts',(31.0895854115311,-55.8477481146612,
-159.779803440199));
#156464=CARTESIAN_POINT('Ctrl Pts',(31.0951600653657,-55.7862957665143,
-159.6744189526));
#156465=CARTESIAN_POINT('Ctrl Pts',(31.1010151755717,-55.7254297048882,
-159.563699979791));
#156466=CARTESIAN_POINT('Ctrl Pts',(31.1048957464655,-55.6850897183029,
-159.490319153784));
#156467=CARTESIAN_POINT('Ctrl Pts',(31.1088994942666,-55.6450065439528,
-159.414595376028));
#156468=CARTESIAN_POINT('Ctrl Pts',(31.1130279364408,-55.6053242693568,
-159.336497304981));
#156469=CARTESIAN_POINT('Ctrl Pts',(31.1182320407174,-55.5553028118145,
-159.238050847847));
#156470=CARTESIAN_POINT('Ctrl Pts',(31.1236338630895,-55.505924294484,-159.135838743465));
#156471=CARTESIAN_POINT('Ctrl Pts',(31.1292335128526,-55.4574651316412,
-159.029851363251));
#156472=CARTESIAN_POINT('Ctrl Pts',(31.134430377709,-55.412491654549,-158.93148769503));
#156473=CARTESIAN_POINT('Ctrl Pts',(31.1397976024776,-55.3683104260197,
-158.829872916478));
#156474=CARTESIAN_POINT('Ctrl Pts',(31.1453337206069,-55.3251129589623,
-158.725027925676));
#156475=CARTESIAN_POINT('Ctrl Pts',(31.1457047307718,-55.3222180244603,
-158.718001602099));
#156476=CARTESIAN_POINT('Ctrl Pts',(31.1461718442569,-55.3185888253415,
-158.709155023414));
#156477=CARTESIAN_POINT('Ctrl Pts',(31.1464490733754,-55.3164414031806,
-158.703905479327));
#156478=CARTESIAN_POINT('Ctrl Pts',(31.1466037171372,-55.315243529584,-158.700977182148));
#156479=CARTESIAN_POINT('Ctrl Pts',(31.1467586734147,-55.3140450063871,
-158.698042922972));
#156480=CARTESIAN_POINT('Ctrl Pts',(31.1469139423337,-55.3128458487235,
-158.695102699558));
#156481=CARTESIAN_POINT('Ctrl Pts',(31.1533714787286,-55.2629736379607,
-158.572820662532));
#156482=CARTESIAN_POINT('Ctrl Pts',(31.1603704172416,-55.2120214585731,
-158.440211131639));
#156483=CARTESIAN_POINT('Ctrl Pts',(31.1679235634068,-55.1612687635298,
-158.297038080203));
#156484=CARTESIAN_POINT('Ctrl Pts',(31.1706072274891,-55.1432361210005,
-158.246168102674));
#156485=CARTESIAN_POINT('Ctrl Pts',(31.1733608621816,-55.1252291692777,
-158.193964379686));
#156486=CARTESIAN_POINT('Ctrl Pts',(31.1761850567432,-55.1073066058283,
-158.140415804507));
#156487=CARTESIAN_POINT('Ctrl Pts',(31.182154073824,-55.0694267483942,-158.027239338468));
#156488=CARTESIAN_POINT('Ctrl Pts',(31.1884373070365,-55.0319283050599,
-157.908064907983));
#156489=CARTESIAN_POINT('Ctrl Pts',(31.1950355152709,-54.9953865838879,
-157.782861954481));
#156490=CARTESIAN_POINT('Ctrl Pts',(31.200367630056,-54.9658566501828,-157.681683498786));
#156491=CARTESIAN_POINT('Ctrl Pts',(31.2059053736433,-54.9369522328227,
-157.576569309603));
#156492=CARTESIAN_POINT('Ctrl Pts',(31.211647603869,-54.9089746582482,-157.467531218779));
#156493=CARTESIAN_POINT('Ctrl Pts',(31.211851539337,-54.9079810338998,-157.463658727915));
#156494=CARTESIAN_POINT('Ctrl Pts',(31.2121280280077,-54.9066380554768,
-157.458408449884));
#156495=CARTESIAN_POINT('Ctrl Pts',(31.2122601928806,-54.9059973007545,
-157.45589890854));
#156496=CARTESIAN_POINT('Ctrl Pts',(31.212464012248,-54.9050091545155,-157.452028794511));
#156497=CARTESIAN_POINT('Ctrl Pts',(31.2126695003386,-54.9040153265436,
-157.448126913748));
#156498=CARTESIAN_POINT('Ctrl Pts',(31.2128766588162,-54.9030159233487,
-157.444193233984));
#156499=CARTESIAN_POINT('Ctrl Pts',(31.2156323833892,-54.8897213675319,
-157.391865479322));
#156500=CARTESIAN_POINT('Ctrl Pts',(31.2186822770619,-54.8754481380802,
-157.333937612989));
#156501=CARTESIAN_POINT('Ctrl Pts',(31.2220286788944,-54.8604870397,-157.270362719997));
#156502=CARTESIAN_POINT('Ctrl Pts',(31.2236506557137,-54.8532355032798,
-157.239548428142));
#156503=CARTESIAN_POINT('Ctrl Pts',(31.2253422855029,-54.8458231472352,
-157.207407563133));
#156504=CARTESIAN_POINT('Ctrl Pts',(31.2271037881024,-54.8382874305316,
-157.173935514171));
#156505=CARTESIAN_POINT('Ctrl Pts',(31.230750984607,-54.8226847061137,-157.104631534711));
#156506=CARTESIAN_POINT('Ctrl Pts',(31.2346975404456,-54.8065505635224,
-157.02962198736));
#156507=CARTESIAN_POINT('Ctrl Pts',(31.2389443632973,-54.7902552512034,
-156.948879688243));
#156508=CARTESIAN_POINT('Ctrl Pts',(31.2404734082391,-54.7843882146574,
-156.919808872633));
#156509=CARTESIAN_POINT('Ctrl Pts',(31.242041368692,-54.7785007447406,-156.889995055113));
#156510=CARTESIAN_POINT('Ctrl Pts',(31.243648253759,-54.7726116560897,-156.859437531544));
#156511=CARTESIAN_POINT('Ctrl Pts',(31.2440818183164,-54.7710226811428,
-156.851192598878));
#156512=CARTESIAN_POINT('Ctrl Pts',(31.2445182165278,-54.7694335927254,
-156.842893526154));
#156513=CARTESIAN_POINT('Ctrl Pts',(31.244957689739,-54.7678447199691,-156.834540313013));
#156514=CARTESIAN_POINT('Ctrl Pts',(31.2453971629501,-54.7662558472127,
-156.826187099872));
#156515=CARTESIAN_POINT('Ctrl Pts',(31.2457373617316,-54.7650314393738,
-156.819720368753));
#156516=CARTESIAN_POINT('Ctrl Pts',(31.2462842962207,-54.7630793515511,
-156.809318204654));
#156517=CARTESIAN_POINT('Ctrl Pts',(31.2499077279959,-54.7501468026159,
-156.740404042759));
#156518=CARTESIAN_POINT('Ctrl Pts',(31.2532865764462,-54.7388343038513,
-156.676335804936));
#156519=CARTESIAN_POINT('Ctrl Pts',(31.2564089347118,-54.7288613645528,
-156.617160899623));
#156520=CARTESIAN_POINT('Ctrl Pts',(31.2595996255425,-54.718670168262,-156.55669095616));
#156521=CARTESIAN_POINT('Ctrl Pts',(31.2625225020072,-54.709877696298,-156.501330429004));
#156522=CARTESIAN_POINT('Ctrl Pts',(31.2651663049396,-54.7022330407062,
-156.451105263779));
#156523=CARTESIAN_POINT('Ctrl Pts',(31.2661836254125,-54.6992914203054,
-156.431778903174));
#156524=CARTESIAN_POINT('Ctrl Pts',(31.2671596373143,-54.6965202625494,
-156.413212698865));
#156525=CARTESIAN_POINT('Ctrl Pts',(31.2680937422418,-54.6939071725389,
-156.395407391056));
#156526=CARTESIAN_POINT('Ctrl Pts',(31.2705597707236,-54.6870086387644,
-156.348401540974));
#156527=CARTESIAN_POINT('Ctrl Pts',(31.2727389909105,-54.6812076253658,
-156.306702425142));
#156528=CARTESIAN_POINT('Ctrl Pts',(31.2746373151085,-54.6763099699925,
-156.270323611698));
#156529=CARTESIAN_POINT('Ctrl Pts',(31.2749472115869,-54.6755104405157,
-156.264384865203));
#156530=CARTESIAN_POINT('Ctrl Pts',(31.2752496232857,-54.6747350947099,
-156.258587876625));
#156531=CARTESIAN_POINT('Ctrl Pts',(31.2755445770089,-54.6739832155616,
-156.252932676198));
#156532=CARTESIAN_POINT('Ctrl Pts',(31.2765954487601,-54.6713043934435,
-156.232784124375));
#156533=CARTESIAN_POINT('Ctrl Pts',(31.2775517837798,-54.6689230091112,
-156.214435590985));
#156534=CARTESIAN_POINT('Ctrl Pts',(31.2784152401867,-54.6668102998059,
-156.197888377381));
#156535=CARTESIAN_POINT('Ctrl Pts',(31.2788469683902,-54.6657539451532,
-156.189614770579));
#156536=CARTESIAN_POINT('Ctrl Pts',(31.2792554896595,-54.6647648470439,
-156.181791483242));
#156537=CARTESIAN_POINT('Ctrl Pts',(31.2796409993958,-54.6638399472217,
-156.174418629354));
#156538=CARTESIAN_POINT('Ctrl Pts',(31.2798337542639,-54.6633774973106,
-156.170732202409));
#156539=CARTESIAN_POINT('Ctrl Pts',(31.2800207570482,-54.6629311023795,
-156.167158383168));
#156540=CARTESIAN_POINT('Ctrl Pts',(31.2802020332021,-54.6625004132038,
-156.163697183383));
#156541=CARTESIAN_POINT('Ctrl Pts',(31.280292671279,-54.662285068616,-156.161966583491));
#156542=CARTESIAN_POINT('Ctrl Pts',(31.2803818777461,-54.6620736508037,
-156.160264138423));
#156543=CARTESIAN_POINT('Ctrl Pts',(31.2804696557356,-54.6618661181874,
-156.158589849491));
#156544=CARTESIAN_POINT('Ctrl Pts',(31.2805135447303,-54.6617623518792,
-156.157752705025));
#156545=CARTESIAN_POINT('Ctrl Pts',(31.2805570766087,-54.661659556891,-156.15692259959));
#156546=CARTESIAN_POINT('Ctrl Pts',(31.2806002517564,-54.6615577281553,
-156.156099533342));
#156547=CARTESIAN_POINT('Ctrl Pts',(31.2806218393302,-54.6615068137874,
-156.155688000219));
#156548=CARTESIAN_POINT('Ctrl Pts',(31.2806273357613,-54.6614938621523,
-156.155583237424));
#156549=CARTESIAN_POINT('Ctrl Pts',(31.2806407410667,-54.6614622698096,
-156.155327731628));
#156550=CARTESIAN_POINT('Ctrl Pts',(31.2806541463722,-54.6614306774669,
-156.155072225832));
#156551=CARTESIAN_POINT('Ctrl Pts',(31.2806754569608,-54.6613804188924,
-156.154665979994));
#156552=CARTESIAN_POINT('Ctrl Pts',(31.2807287078847,-54.6612551356553,
-156.153651452317));
#156553=CARTESIAN_POINT('Ctrl Pts',(31.2808487333909,-54.6609727521238,
-156.151364746491));
#156554=CARTESIAN_POINT('Ctrl Pts',(31.2809686760916,-54.6606913107074,
-156.149079596605));
#156555=CARTESIAN_POINT('Ctrl Pts',(31.2810885359334,-54.6604108081993,
-156.146796003748));
#156556=CARTESIAN_POINT('Ctrl Pts',(31.2882968648863,-54.6435414854894,
-156.009461528184));
#156557=CARTESIAN_POINT('Ctrl Pts',(31.2952156728382,-54.6300150587062,
-155.877565569711));
#156558=CARTESIAN_POINT('Ctrl Pts',(31.3018424173055,-54.6192049768191,
-155.751171162578));
#156559=CARTESIAN_POINT('Ctrl Pts',(31.3084520725614,-54.6084227722368,
-155.625102704447));
#156560=CARTESIAN_POINT('Ctrl Pts',(31.3147711704004,-54.6003428938458,
-155.504507460173));
#156561=CARTESIAN_POINT('Ctrl Pts',(31.3207975017896,-54.5943950305198,
-155.389442427711));
#156562=CARTESIAN_POINT('Ctrl Pts',(31.3268022969577,-54.5884684229948,
-155.274788601642));
#156563=CARTESIAN_POINT('Ctrl Pts',(31.332516415975,-54.5846586070994,-155.165625531183));
#156564=CARTESIAN_POINT('Ctrl Pts',(31.3379379616093,-54.5824527478572,
-155.062004084437));
#156565=CARTESIAN_POINT('Ctrl Pts',(31.3421341584728,-54.5807454451325,
-154.981802603317));
#156566=CARTESIAN_POINT('Ctrl Pts',(31.3461550941912,-54.58000002,-154.904920740243));
#156567=CARTESIAN_POINT('Ctrl Pts',(31.35,-54.58000002,-154.831379798159));
#156568=CARTESIAN_POINT('Ctrl Pts',(25.7,-54.58000002,-148.513004346424));
#156569=CARTESIAN_POINT('Ctrl Pts',(25.6952401431873,-54.58000002,-148.603330686833));
#156570=CARTESIAN_POINT('Ctrl Pts',(25.690234948237,-54.5812733325853,-148.69822201173));
#156571=CARTESIAN_POINT('Ctrl Pts',(25.6849838077408,-54.5842510816626,
-148.797663422931));
#156572=CARTESIAN_POINT('Ctrl Pts',(25.6802258199289,-54.5869491800714,
-148.887765948818));
#156573=CARTESIAN_POINT('Ctrl Pts',(25.6752658344534,-54.5910472446749,
-148.981605501865));
#156574=CARTESIAN_POINT('Ctrl Pts',(25.6701039419043,-54.5969022494087,
-149.079159958141));
#156575=CARTESIAN_POINT('Ctrl Pts',(25.6654607472659,-54.6021689081641,
-149.166911557778));
#156576=CARTESIAN_POINT('Ctrl Pts',(25.660654398054,-54.608857531153,-149.257664908944));
#156577=CARTESIAN_POINT('Ctrl Pts',(25.6556862558358,-54.6172494896974,
-149.351379263024));
#156578=CARTESIAN_POINT('Ctrl Pts',(25.6532021847266,-54.6214454689696,
-149.398236440063));
#156579=CARTESIAN_POINT('Ctrl Pts',(25.6506776946647,-54.6260675732657,
-149.445833314481));
#156580=CARTESIAN_POINT('Ctrl Pts',(25.6481130758643,-54.6311526793434,
-149.494162543797));
#156581=CARTESIAN_POINT('Ctrl Pts',(25.6468307664641,-54.6336952323822,
-149.518327158455));
#156582=CARTESIAN_POINT('Ctrl Pts',(25.6455384263384,-54.636353552382,-149.542674834613));
#156583=CARTESIAN_POINT('Ctrl Pts',(25.6442361017532,-54.6391323395035,
-149.567204468556));
#156584=CARTESIAN_POINT('Ctrl Pts',(25.6439105206068,-54.6398270362839,
-149.573336877041));
#156585=CARTESIAN_POINT('Ctrl Pts',(25.6435843154472,-54.6405292625706,
-149.579480657608));
#156586=CARTESIAN_POINT('Ctrl Pts',(25.6432574870445,-54.6412390923846,
-149.585635792139));
#156587=CARTESIAN_POINT('Ctrl Pts',(25.6430123657424,-54.6417714647451,
-149.590252143037));
#156588=CARTESIAN_POINT('Ctrl Pts',(25.6427668938662,-54.6423081140951,
-149.594874880539));
#156589=CARTESIAN_POINT('Ctrl Pts',(25.6425210717417,-54.642849071759,-149.599503996986));
#156590=CARTESIAN_POINT('Ctrl Pts',(25.6424595871068,-54.6429843752208,
-149.600661824155));
#156591=CARTESIAN_POINT('Ctrl Pts',(25.642398181581,-54.6431197234208,-149.601818148208));
#156592=CARTESIAN_POINT('Ctrl Pts',(25.6423358274055,-54.6432573912261,
-149.602992322239));
#156593=CARTESIAN_POINT('Ctrl Pts',(25.6417248072865,-54.6446064235565,
-149.614498271108));
#156594=CARTESIAN_POINT('Ctrl Pts',(25.6410477023583,-54.646127792578,-149.627247027373));
#156595=CARTESIAN_POINT('Ctrl Pts',(25.6404953939238,-54.6473869011259,
-149.637644969131));
#156596=CARTESIAN_POINT('Ctrl Pts',(25.6404280329281,-54.6475404653307,
-149.638913129577));
#156597=CARTESIAN_POINT('Ctrl Pts',(25.6403625279329,-54.6476900650441,
-149.640146332103));
#156598=CARTESIAN_POINT('Ctrl Pts',(25.6402992249769,-54.6478348634309,
-149.641338064999));
#156599=CARTESIAN_POINT('Ctrl Pts',(25.6335671479497,-54.6632337318913,
-149.768075237438));
#156600=CARTESIAN_POINT('Ctrl Pts',(25.6266648637635,-54.68134375949,-149.894901757786));
#156601=CARTESIAN_POINT('Ctrl Pts',(25.6197654985376,-54.7021891456976,
-150.021659611439));
#156602=CARTESIAN_POINT('Ctrl Pts',(25.6166209067786,-54.7116900530323,
-150.079433289006));
#156603=CARTESIAN_POINT('Ctrl Pts',(25.6134766834941,-54.7217585222176,
-150.137192825257));
#156604=CARTESIAN_POINT('Ctrl Pts',(25.6103479373083,-54.7323935724098,
-150.194923995243));
#156605=CARTESIAN_POINT('Ctrl Pts',(25.6078496009172,-54.7408857706705,
-150.241022935302));
#156606=CARTESIAN_POINT('Ctrl Pts',(25.6053615108759,-54.749739102678,-150.287103673156));
#156607=CARTESIAN_POINT('Ctrl Pts',(25.6028917781346,-54.7589519149327,
-150.333158921312));
#156608=CARTESIAN_POINT('Ctrl Pts',(25.6004220453934,-54.7681647271875,
-150.379214169468));
#156609=CARTESIAN_POINT('Ctrl Pts',(25.5979706737284,-54.7777370159852,
-150.42524392434));
#156610=CARTESIAN_POINT('Ctrl Pts',(25.5955454527164,-54.787666304305,-150.471241193469));
#156611=CARTESIAN_POINT('Ctrl Pts',(25.5931202317043,-54.7975955926248,
-150.517238462598));
#156612=CARTESIAN_POINT('Ctrl Pts',(25.5907211611064,-54.8078818802587,
-150.563203245825));
#156613=CARTESIAN_POINT('Ctrl Pts',(25.5883559904803,-54.8185217967351,
-150.609128693392));
#156614=CARTESIAN_POINT('Ctrl Pts',(25.586849990668,-54.8252966619559,-150.63837128361));
#156615=CARTESIAN_POINT('Ctrl Pts',(25.5853907429839,-54.832056830242,-150.666933522216));
#156616=CARTESIAN_POINT('Ctrl Pts',(25.5838882239385,-54.8391074038692,
-150.696081713571));
#156617=CARTESIAN_POINT('Ctrl Pts',(25.5830751710654,-54.8429226561036,
-150.711854572358));
#156618=CARTESIAN_POINT('Ctrl Pts',(25.5822494632555,-54.8468237998395,
-150.727798866652));
#156619=CARTESIAN_POINT('Ctrl Pts',(25.5813969566317,-54.8508654682067,
-150.744114196661));
#156620=CARTESIAN_POINT('Ctrl Pts',(25.5813506829308,-54.8510848482654,
-150.74499978591));
#156621=CARTESIAN_POINT('Ctrl Pts',(25.5813043298756,-54.8513046489268,
-150.74588647576));
#156622=CARTESIAN_POINT('Ctrl Pts',(25.5812578952138,-54.8515248793833,
-150.746774298036));
#156623=CARTESIAN_POINT('Ctrl Pts',(25.5762922628235,-54.8750758959192,
-150.841716284895));
#156624=CARTESIAN_POINT('Ctrl Pts',(25.5712705869925,-54.9000065217402,
-150.935491566644));
#156625=CARTESIAN_POINT('Ctrl Pts',(25.5663110036503,-54.9262266483463,
-151.02805147902));
#156626=CARTESIAN_POINT('Ctrl Pts',(25.5573185100371,-54.9737678034748,
-151.195876952141));
#156627=CARTESIAN_POINT('Ctrl Pts',(25.5485269899804,-55.025545197899,-151.359704657308));
#156628=CARTESIAN_POINT('Ctrl Pts',(25.539955871748,-55.0811644018053,-151.519223093345));
#156629=CARTESIAN_POINT('Ctrl Pts',(25.5367090290684,-55.1022336252313,
-151.579650595599));
#156630=CARTESIAN_POINT('Ctrl Pts',(25.5334937784768,-55.1238542107661,
-151.639460298851));
#156631=CARTESIAN_POINT('Ctrl Pts',(25.5303111060527,-55.1460043862931,
-151.698636298518));
#156632=CARTESIAN_POINT('Ctrl Pts',(25.5291526668546,-55.1540666773987,
-151.720175366468));
#156633=CARTESIAN_POINT('Ctrl Pts',(25.5279985351647,-55.1621991258492,
-151.741630495981));
#156634=CARTESIAN_POINT('Ctrl Pts',(25.5268458420758,-55.1704017042082,
-151.763000564696));
#156635=CARTESIAN_POINT('Ctrl Pts',(25.5259639599703,-55.1766771882415,
-151.779350000099));
#156636=CARTESIAN_POINT('Ctrl Pts',(25.5251276462376,-55.1826745046545,
-151.794830293532));
#156637=CARTESIAN_POINT('Ctrl Pts',(25.5242386556593,-55.1891234263154,
-151.811322522395));
#156638=CARTESIAN_POINT('Ctrl Pts',(25.523965661785,-55.1911037803844,-151.81638700515));
#156639=CARTESIAN_POINT('Ctrl Pts',(25.5236877053738,-55.1931270620186,
-151.821546800661));
#156640=CARTESIAN_POINT('Ctrl Pts',(25.5234019553268,-55.1952153541429,
-151.826856060969));
#156641=CARTESIAN_POINT('Ctrl Pts',(25.516907746872,-55.2426757290784,-151.947519009381));
#156642=CARTESIAN_POINT('Ctrl Pts',(25.5103427225298,-55.2927227172219,
-152.066203784139));
#156643=CARTESIAN_POINT('Ctrl Pts',(25.5038940014195,-55.3452199311413,
-152.182765043397));
#156644=CARTESIAN_POINT('Ctrl Pts',(25.5006806324233,-55.3713790589293,
-152.240846999532));
#156645=CARTESIAN_POINT('Ctrl Pts',(25.4974956403295,-55.3981463157476,
-152.298402283602));
#156646=CARTESIAN_POINT('Ctrl Pts',(25.4943591646552,-55.4255036723978,
-152.355416512223));
#156647=CARTESIAN_POINT('Ctrl Pts',(25.4920014436296,-55.4460684787852,
-152.398274694317));
#156648=CARTESIAN_POINT('Ctrl Pts',(25.489671651699,-55.4669661314315,-152.440826470802));
#156649=CARTESIAN_POINT('Ctrl Pts',(25.4873785634058,-55.4881875528084,
-152.483065297136));
#156650=CARTESIAN_POINT('Ctrl Pts',(25.4839389309659,-55.5200196848738,
-152.546423536637));
#156651=CARTESIAN_POINT('Ctrl Pts',(25.4805819867172,-55.5525804217012,
-152.609077547121));
#156652=CARTESIAN_POINT('Ctrl Pts',(25.4773357259928,-55.5858365512146,
-152.671006667056));
#156653=CARTESIAN_POINT('Ctrl Pts',(25.4740921888675,-55.6190647789758,
-152.73288382872));
#156654=CARTESIAN_POINT('Ctrl Pts',(25.4709591638032,-55.6529871939301,
-152.794037301754));
#156655=CARTESIAN_POINT('Ctrl Pts',(25.4679623650184,-55.6875680621891,
-152.854448417611));
#156656=CARTESIAN_POINT('Origin',(0.,-12.9675000200281,-171.64995));
#156657=CARTESIAN_POINT('',(25.5015460489969,-65.317216804244,-171.07256826174));
#156658=CARTESIAN_POINT('',(31.1079170675507,-62.1926886331265,-171.07256826174));
#156659=CARTESIAN_POINT('Origin',(0.,-12.9675000200281,-171.07256826174));
#156660=CARTESIAN_POINT('Ctrl Pts',(31.1079170675507,-62.1926886331265,
-171.07256826174));
#156661=CARTESIAN_POINT('Ctrl Pts',(31.1058138200187,-61.5908885288768,
-169.979184151723));
#156662=CARTESIAN_POINT('Ctrl Pts',(31.1036899128493,-60.9957468863196,
-168.903399109055));
#156663=CARTESIAN_POINT('Ctrl Pts',(31.1015460971806,-60.4071760243875,
-167.845246182439));
#156664=CARTESIAN_POINT('Ctrl Pts',(31.0993650427809,-59.8083815073155,
-166.768712817194));
#156665=CARTESIAN_POINT('Ctrl Pts',(31.0971633844274,-59.216388176699,-165.710429350991));
#156666=CARTESIAN_POINT('Ctrl Pts',(31.094942488845,-58.6311510745784,-164.670402894343));
#156667=CARTESIAN_POINT('Ctrl Pts',(31.0926579405937,-58.0291406023887,
-163.600568435817));
#156668=CARTESIAN_POINT('Ctrl Pts',(31.0903530381058,-57.4342792756791,
-162.550052453581));
#156669=CARTESIAN_POINT('Ctrl Pts',(31.0880298460936,-56.8465661337348,
-161.518834639248));
#156670=CARTESIAN_POINT('Ctrl Pts',(31.0867866957293,-56.5320782211154,
-160.967025406579));
#156671=CARTESIAN_POINT('Ctrl Pts',(31.0855383179793,-56.2196378961364,
-160.420741481362));
#156672=CARTESIAN_POINT('Ctrl Pts',(31.0842850915597,-55.9092502513102,
-159.879976688011));
#156673=CARTESIAN_POINT('Ctrl Pts',(25.4679548160676,-55.6876551762764,
-152.854600597735));
#156674=CARTESIAN_POINT('Ctrl Pts',(25.4704574246668,-56.3163380661018,
-154.015391793635));
#156675=CARTESIAN_POINT('Ctrl Pts',(25.4729351017059,-56.9553314098175,
-155.201562547543));
#156676=CARTESIAN_POINT('Ctrl Pts',(25.4753841249239,-57.6045621956431,
-156.413167418875));
#156677=CARTESIAN_POINT('Ctrl Pts',(25.4777340045614,-58.2275102316101,
-157.575723002255));
#156678=CARTESIAN_POINT('Ctrl Pts',(25.4800575016275,-58.8598835484616,
-158.761695122599));
#156679=CARTESIAN_POINT('Ctrl Pts',(25.4823522232456,-59.5016591213111,
-159.97110891368));
#156680=CARTESIAN_POINT('Ctrl Pts',(25.4846007074484,-60.1305032590741,
-161.156153662694));
#156681=CARTESIAN_POINT('Ctrl Pts',(25.4868215599701,-60.7683743984617,
-162.363705019834));
#156682=CARTESIAN_POINT('Ctrl Pts',(25.4890134549808,-61.4152933901963,
-163.593762998944));
#156683=CARTESIAN_POINT('Ctrl Pts',(25.4911578809512,-62.0482023022682,
-164.797182078134));
#156684=CARTESIAN_POINT('Ctrl Pts',(25.49327458673,-62.6897712831155,-166.022143574981));
#156685=CARTESIAN_POINT('Ctrl Pts',(25.4953632798875,-63.3400631788034,
-167.268623429998));
#156686=CARTESIAN_POINT('Ctrl Pts',(25.497451973045,-63.9903550744914,-168.515103285014));
#156687=CARTESIAN_POINT('Ctrl Pts',(25.4995126467204,-64.6493695892343,
-169.783101662045));
#156688=CARTESIAN_POINT('Ctrl Pts',(25.5015460489969,-65.317216804244,-171.07256826174));
#156689=CARTESIAN_POINT('Ctrl Pts',(42.,-55.58000002,-60.64995));
#156690=CARTESIAN_POINT('Ctrl Pts',(42.,-55.08000002,-60.64995));
#156691=CARTESIAN_POINT('Ctrl Pts',(42.5,-55.08000002,-60.64995));
#156692=CARTESIAN_POINT('Ctrl Pts',(41.5,-55.58000002,-60.64995));
#156693=CARTESIAN_POINT('Ctrl Pts',(41.5,-54.58000002,-60.64995));
#156694=CARTESIAN_POINT('Ctrl Pts',(42.5,-54.58000002,-60.64995));
#156695=CARTESIAN_POINT('Ctrl Pts',(41.5,-55.58000002,-61.14995));
#156696=CARTESIAN_POINT('Ctrl Pts',(41.5,-54.58000002,-61.14995));
#156697=CARTESIAN_POINT('Ctrl Pts',(42.5,-54.58000002,-61.14995));
#156698=CARTESIAN_POINT('',(42.,-55.58000002,-60.64995));
#156699=CARTESIAN_POINT('',(41.5,-55.58000002,-61.14995));
#156700=CARTESIAN_POINT('Origin',(42.,-55.58000002,-61.14995));
#156701=CARTESIAN_POINT('',(42.5,-54.58000002,-61.14995));
#156702=CARTESIAN_POINT('Origin',(42.5,-55.58000002,-61.14995));
#156703=CARTESIAN_POINT('',(42.5,-55.08000002,-60.64995));
#156704=CARTESIAN_POINT('Origin',(42.5,-55.08000002,-61.14995));
#156705=CARTESIAN_POINT('Origin',(42.5,-55.58000002,-60.64995));
#156706=CARTESIAN_POINT('Origin',(0.,-12.9675000200281,-171.64995));
#156707=CARTESIAN_POINT('',(33.85,-63.4074419114814,-171.64995));
#156708=CARTESIAN_POINT('',(39.5,-62.6133861954129,-171.64995));
#156709=CARTESIAN_POINT('',(39.8608268990399,-62.5626752818388,-171.64995));
#156710=CARTESIAN_POINT('',(39.5,-56.978215522411,-171.64995));
#156711=CARTESIAN_POINT('',(39.5,-56.5665827677457,-171.64995));
#156712=CARTESIAN_POINT('',(33.85,-61.4584329769396,-171.64995));
#156713=CARTESIAN_POINT('Origin',(0.,-12.9675000200281,-171.64995));
#156714=CARTESIAN_POINT('',(33.85,-63.4777123288326,-171.64995));
#156715=CARTESIAN_POINT('Origin',(0.,-12.9675000200281,-170.64995));
#156716=CARTESIAN_POINT('',(39.3992713666431,-56.66417131427,-171.60362375617));
#156717=CARTESIAN_POINT('Origin',(39.9831889404834,-58.6893018970301,-160.044295853358));
#156718=CARTESIAN_POINT('Origin',(39.6007286333569,-56.8876021458077,-170.64995));
#156719=CARTESIAN_POINT('Ctrl Pts',(33.5886122085037,-60.5345771657122,
-171.072568261741));
#156720=CARTESIAN_POINT('Ctrl Pts',(33.5929196926425,-60.5496789454406,
-171.104351697009));
#156721=CARTESIAN_POINT('Ctrl Pts',(33.5977697943261,-60.5668084312768,
-171.13599186684));
#156722=CARTESIAN_POINT('Ctrl Pts',(33.6032176264056,-60.5860501581706,
-171.167201320259));
#156723=CARTESIAN_POINT('Ctrl Pts',(33.6085732655045,-60.6049662597278,
-171.197882620002));
#156724=CARTESIAN_POINT('Ctrl Pts',(33.6145068364652,-60.6259240920045,
-171.228147383835));
#156725=CARTESIAN_POINT('Ctrl Pts',(33.6210487151924,-60.6489745030752,
-171.257689498379));
#156726=CARTESIAN_POINT('Ctrl Pts',(33.6274228563078,-60.6714338880711,
-171.28647413576));
#156727=CARTESIAN_POINT('Ctrl Pts',(33.6343746980392,-60.695880197154,-171.314572324815));
#156728=CARTESIAN_POINT('Ctrl Pts',(33.6419080665843,-60.722327544365,-171.341674173059));
#156729=CARTESIAN_POINT('Ctrl Pts',(33.6480621691508,-60.7439327116121,
-171.363814010349));
#156730=CARTESIAN_POINT('Ctrl Pts',(33.6546039728895,-60.7668727584721,
-171.38528835636));
#156731=CARTESIAN_POINT('Ctrl Pts',(33.6615217079334,-60.7911363934354,
-171.405917367214));
#156732=CARTESIAN_POINT('Ctrl Pts',(33.6670079528816,-60.8103791432507,
-171.42227760736));
#156733=CARTESIAN_POINT('Ctrl Pts',(33.6727304167729,-60.8304540680111,
-171.438105942042));
#156734=CARTESIAN_POINT('Ctrl Pts',(33.6786769452906,-60.8513468520672,
-171.453309230289));
#156735=CARTESIAN_POINT('Ctrl Pts',(33.6816502095495,-60.8617932440953,
-171.460910874412));
#156736=CARTESIAN_POINT('Ctrl Pts',(33.6846794709728,-60.8724440739407,
-171.468356302772));
#156737=CARTESIAN_POINT('Ctrl Pts',(33.6877625715685,-60.883296665184,-171.475633559578));
#156738=CARTESIAN_POINT('Ctrl Pts',(33.6893041218664,-60.8887229608057,
-171.479272187981));
#156739=CARTESIAN_POINT('Ctrl Pts',(33.690859130285,-60.8941996943994,-171.482868777341));
#156740=CARTESIAN_POINT('Ctrl Pts',(33.692427301567,-60.8997264955286,-171.486421837307));
#156741=CARTESIAN_POINT('Ctrl Pts',(33.6934416044798,-60.9033012647824,
-171.488719978534));
#156742=CARTESIAN_POINT('Ctrl Pts',(33.6945967894686,-60.907378611323,-171.491303411206));
#156743=CARTESIAN_POINT('Ctrl Pts',(33.6956308892224,-60.9110250428065,
-171.49358056745));
#156744=CARTESIAN_POINT('Ctrl Pts',(33.6961955678179,-60.9130162064263,
-171.49482402717));
#156745=CARTESIAN_POINT('Ctrl Pts',(33.6967238009515,-60.9148783795049,
-171.495977094956));
#156746=CARTESIAN_POINT('Ctrl Pts',(33.6971709938997,-60.9164567102561,
-171.496948943728));
#156747=CARTESIAN_POINT('Ctrl Pts',(33.7037454599816,-60.9396607478684,
-171.51123670657));
#156748=CARTESIAN_POINT('Ctrl Pts',(33.7107503112399,-60.964441558183,-171.525212483463));
#156749=CARTESIAN_POINT('Ctrl Pts',(33.7182138182058,-60.9908464908231,
-171.538579075089));
#156750=CARTESIAN_POINT('Ctrl Pts',(33.722249158874,-61.0051230097589,-171.545806073206));
#156751=CARTESIAN_POINT('Ctrl Pts',(33.7264182463428,-61.0198738554632,
-171.552854348258));
#156752=CARTESIAN_POINT('Ctrl Pts',(33.7307227872848,-61.0351027074787,
-171.559672544505));
#156753=CARTESIAN_POINT('Ctrl Pts',(33.7368557590083,-61.0568002868611,
-171.569386891599));
#156754=CARTESIAN_POINT('Ctrl Pts',(33.7432641867585,-61.0794688883045,
-171.578634643421));
#156755=CARTESIAN_POINT('Ctrl Pts',(33.7499446944048,-61.1031075981544,
-171.587257169257));
#156756=CARTESIAN_POINT('Ctrl Pts',(33.7532849482279,-61.1149269530793,
-171.591568432174));
#156757=CARTESIAN_POINT('Ctrl Pts',(33.7566930603084,-61.1269886097382,
-171.595723207788));
#156758=CARTESIAN_POINT('Ctrl Pts',(33.7601675497484,-61.1392909724596,
-171.599700645306));
#156759=CARTESIAN_POINT('Ctrl Pts',(33.7619047944684,-61.1454421538202,
-171.601689364065));
#156760=CARTESIAN_POINT('Ctrl Pts',(33.7636586341358,-61.1516535125633,
-171.603633745029));
#156761=CARTESIAN_POINT('Ctrl Pts',(33.7654287967637,-61.1579247271646,
-171.605531115606));
#156762=CARTESIAN_POINT('Ctrl Pts',(33.7663138780777,-61.1610603344652,
-171.606479800894));
#156763=CARTESIAN_POINT('Ctrl Pts',(33.7672030401555,-61.1642109057643,
-171.607416733475));
#156764=CARTESIAN_POINT('Ctrl Pts',(33.7680962461282,-61.1673763968156,
-171.608341576954));
#156765=CARTESIAN_POINT('Ctrl Pts',(33.7687784745082,-61.1697941905808,
-171.609047969978));
#156766=CARTESIAN_POINT('Ctrl Pts',(33.7697003191667,-61.1730627912301,
-171.609987833509));
#156767=CARTESIAN_POINT('Ctrl Pts',(33.7703182663326,-61.1752528272204,
-171.610608904528));
#156768=CARTESIAN_POINT('Ctrl Pts',(33.7705093651044,-61.1759300909268,
-171.610800969345));
#156769=CARTESIAN_POINT('Ctrl Pts',(33.7706713306159,-61.1765040977548,
-171.610962995654));
#156770=CARTESIAN_POINT('Ctrl Pts',(33.7707879573347,-61.1769175828282,
-171.611079502341));
#156771=CARTESIAN_POINT('Ctrl Pts',(33.7741748768774,-61.1889254716733,
-171.614462936079));
#156772=CARTESIAN_POINT('Ctrl Pts',(33.778025386712,-61.2026296218794,-171.618091850388));
#156773=CARTESIAN_POINT('Ctrl Pts',(33.7823610153952,-61.2180649959048,
-171.621762516496));
#156774=CARTESIAN_POINT('Ctrl Pts',(33.7866010646012,-61.2331600951773,
-171.62535226231));
#156775=CARTESIAN_POINT('Ctrl Pts',(33.7913054677371,-61.2499114871387,
-171.62898182177));
#156776=CARTESIAN_POINT('Ctrl Pts',(33.7964886563819,-61.2683447777054,
-171.632412230725));
#156777=CARTESIAN_POINT('Ctrl Pts',(33.801577086152,-61.2864410714946,-171.635779925064));
#156778=CARTESIAN_POINT('Ctrl Pts',(33.8071273721981,-61.3061589305378,
-171.638955522725));
#156779=CARTESIAN_POINT('Ctrl Pts',(33.8131416925086,-61.3275071544742,
-171.641667715949));
#156780=CARTESIAN_POINT('Ctrl Pts',(33.8189432281165,-61.348100085169,-171.644283952655));
#156781=CARTESIAN_POINT('Ctrl Pts',(33.8251768962949,-61.370210572944,-171.646468631973));
#156782=CARTESIAN_POINT('Ctrl Pts',(33.8318283554853,-61.3938240136231,
-171.647939780786));
#156783=CARTESIAN_POINT('Ctrl Pts',(33.8375807854589,-61.4142457977842,
-171.649212085146));
#156784=CARTESIAN_POINT('Ctrl Pts',(33.8436456332876,-61.4357916287887,
-171.64995));
#156785=CARTESIAN_POINT('Ctrl Pts',(33.85,-61.4584329769396,-171.64995));
#156786=CARTESIAN_POINT('Ctrl Pts',(38.9938259143948,-56.2145026772597,
-171.07256826174));
#156787=CARTESIAN_POINT('Ctrl Pts',(39.1191457108045,-56.3534914900074,
-171.473900235605));
#156788=CARTESIAN_POINT('Ctrl Pts',(39.4023695343915,-56.6676074087211,
-171.60507092612));
#156789=CARTESIAN_POINT('Ctrl Pts',(39.0656324591812,-56.1451830708436,
-171.065281773562));
#156790=CARTESIAN_POINT('Ctrl Pts',(39.1873296781658,-56.2851199488468,
-171.471360601804));
#156791=CARTESIAN_POINT('Ctrl Pts',(39.4667323101199,-56.6069363160446,
-171.604463274963));
#156792=CARTESIAN_POINT('Ctrl Pts',(39.1389029748433,-56.0783561940248,
-171.057850262871));
#156793=CARTESIAN_POINT('Ctrl Pts',(39.2568527648251,-56.2190926208658,
-171.468759835437));
#156794=CARTESIAN_POINT('Ctrl Pts',(39.532372953365,-56.5484198596326,-171.603842231026));
#156795=CARTESIAN_POINT('Ctrl Pts',(39.2135563963028,-56.0138844098186,
-171.050282355671));
#156796=CARTESIAN_POINT('Ctrl Pts',(39.3276146389594,-56.1552707341152,
-171.46610011903));
#156797=CARTESIAN_POINT('Ctrl Pts',(39.59920642547,-56.4919352618992,-171.603208415545));
#156798=CARTESIAN_POINT('',(39.2122208303137,-56.0150382731948,-171.050417727856));
#156799=CARTESIAN_POINT('Ctrl Pts',(39.3992713666431,-56.6641713142699,
-171.60362375617));
#156800=CARTESIAN_POINT('Ctrl Pts',(39.3906770785271,-56.6361858077295,
-171.595251703632));
#156801=CARTESIAN_POINT('Ctrl Pts',(39.3823718010794,-56.6088835146842,
-171.585840100202));
#156802=CARTESIAN_POINT('Ctrl Pts',(39.3743756985557,-56.5823930069001,
-171.575551092327));
#156803=CARTESIAN_POINT('Ctrl Pts',(39.3659748533384,-56.5545616159241,
-171.564741280628));
#156804=CARTESIAN_POINT('Ctrl Pts',(39.3579151925546,-56.527625972385,-171.552963121434));
#156805=CARTESIAN_POINT('Ctrl Pts',(39.3502074591453,-56.5016806847487,
-171.540389654922));
#156806=CARTESIAN_POINT('Ctrl Pts',(39.344062169692,-56.48099479773,-171.530364971004));
#156807=CARTESIAN_POINT('Ctrl Pts',(39.3381395186297,-56.4609345535854,
-171.519832885525));
#156808=CARTESIAN_POINT('Ctrl Pts',(39.3324428773758,-56.4415362262102,
-171.508879279698));
#156809=CARTESIAN_POINT('Ctrl Pts',(39.3245733723685,-56.4147388156646,
-171.493747651769));
#156810=CARTESIAN_POINT('Ctrl Pts',(39.3171386020042,-56.3892165372729,
-171.477816990192));
#156811=CARTESIAN_POINT('Ctrl Pts',(39.3101422442096,-56.3650383608604,
-171.461323930839));
#156812=CARTESIAN_POINT('Ctrl Pts',(39.3066440653122,-56.3529492726542,
-171.453077401162));
#156813=CARTESIAN_POINT('Ctrl Pts',(39.3032553172147,-56.3411954690074,
-171.444690285293));
#156814=CARTESIAN_POINT('Ctrl Pts',(39.2999755567523,-56.3297816523997,
-171.436192546601));
#156815=CARTESIAN_POINT('Ctrl Pts',(39.2983356765211,-56.3240747440958,
-171.431943677255));
#156816=CARTESIAN_POINT('Ctrl Pts',(39.2967230252678,-56.318452762688,-171.427667134469));
#156817=CARTESIAN_POINT('Ctrl Pts',(39.2951374873227,-56.3129160426783,
-171.423366671635));
#156818=CARTESIAN_POINT('Ctrl Pts',(39.2942934323989,-56.3099685914361,
-171.421077337065));
#156819=CARTESIAN_POINT('Ctrl Pts',(39.2934570590603,-56.3070452947652,
-171.418781220015));
#156820=CARTESIAN_POINT('Ctrl Pts',(39.2926283405029,-56.3041461672385,
-171.416478873257));
#156821=CARTESIAN_POINT('Ctrl Pts',(39.2923552884053,-56.3031909420352,
-171.415720279636));
#156822=CARTESIAN_POINT('Ctrl Pts',(39.2920830672967,-56.3022383405622,
-171.414961009691));
#156823=CARTESIAN_POINT('Ctrl Pts',(39.2918116761374,-56.301288363005,-171.414201083151));
#156824=CARTESIAN_POINT('Ctrl Pts',(39.2916633249908,-56.3007690746823,
-171.413785682834));
#156825=CARTESIAN_POINT('Ctrl Pts',(39.2915170891402,-56.3002571066252,
-171.413375314105));
#156826=CARTESIAN_POINT('Ctrl Pts',(39.2913732225394,-56.2997533552218,
-171.412970764343));
#156827=CARTESIAN_POINT('Ctrl Pts',(39.2910785677092,-56.2987216162118,
-171.412142201349));
#156828=CARTESIAN_POINT('Ctrl Pts',(39.2907927013265,-56.2977203215939,
-171.411334858269));
#156829=CARTESIAN_POINT('Ctrl Pts',(39.2905105668222,-56.2967317999291,
-171.410534859845));
#156830=CARTESIAN_POINT('Ctrl Pts',(39.2895637803088,-56.2934145205245,
-171.407850226428));
#156831=CARTESIAN_POINT('Ctrl Pts',(39.2886580158514,-56.2902380779171,
-171.405249914464));
#156832=CARTESIAN_POINT('Ctrl Pts',(39.287606731647,-56.2865471065203,-171.402183331585));
#156833=CARTESIAN_POINT('Ctrl Pts',(39.2872325193817,-56.2852332783835,
-171.401091759087));
#156834=CARTESIAN_POINT('Ctrl Pts',(39.2868399324184,-56.2838544292433,
-171.399940714715));
#156835=CARTESIAN_POINT('Ctrl Pts',(39.2864208072506,-56.282381690366,-171.398703860458));
#156836=CARTESIAN_POINT('Ctrl Pts',(39.2793207216785,-56.2574331240225,
-171.377751238812));
#156837=CARTESIAN_POINT('Ctrl Pts',(39.2725972793437,-56.2336227224313,
-171.355722284568));
#156838=CARTESIAN_POINT('Ctrl Pts',(39.2662721784007,-56.2110893945002,
-171.33284252015));
#156839=CARTESIAN_POINT('Ctrl Pts',(39.2598102321418,-56.1880685517593,
-171.309467745673));
#156840=CARTESIAN_POINT('Ctrl Pts',(39.2537640388237,-56.1663806024417,
-171.285204989219));
#156841=CARTESIAN_POINT('Ctrl Pts',(39.2481450730767,-56.1461217644991,
-171.260281430404));
#156842=CARTESIAN_POINT('Ctrl Pts',(39.2424446265433,-56.1255691525555,
-171.234996454334));
#156843=CARTESIAN_POINT('Ctrl Pts',(39.2371838522641,-56.1064872560232,
-171.209031394905));
#156844=CARTESIAN_POINT('Ctrl Pts',(39.23236323362,-56.0889251572901,-171.182609447624));
#156845=CARTESIAN_POINT('Ctrl Pts',(39.2274123917834,-56.0708886396635,
-171.155473743339));
#156846=CARTESIAN_POINT('Ctrl Pts',(39.2229257811129,-56.0544550420533,
-171.127856183048));
#156847=CARTESIAN_POINT('Ctrl Pts',(39.2188923243667,-56.0396254214308,
-171.099983271027));
#156848=CARTESIAN_POINT('Ctrl Pts',(39.2165122517984,-56.0308747206147,
-171.083535951155));
#156849=CARTESIAN_POINT('Ctrl Pts',(39.2142897493854,-56.0226815447907,
-171.066999426818));
#156850=CARTESIAN_POINT('Ctrl Pts',(39.2122207971109,-56.0150382320577,
-171.050417750961));
#156851=CARTESIAN_POINT('Origin',(42.7058184422067,-60.0992226026716,-170.70354739068));
#156852=CARTESIAN_POINT('Ctrl Pts',(39.0986073542357,-56.2184192034566,
-171.229381885675));
#156853=CARTESIAN_POINT('Ctrl Pts',(40.320307620846,-54.58000002,-170.379862235888));
#156854=CARTESIAN_POINT('Ctrl Pts',(42.1374590345468,-54.58000002,-169.116290576972));
#156855=CARTESIAN_POINT('Ctrl Pts',(36.5384467754252,-56.1227754271583,
-167.395443178417));
#156856=CARTESIAN_POINT('Ctrl Pts',(37.7530684146654,-54.5800000200966,
-166.553337438667));
#156857=CARTESIAN_POINT('Ctrl Pts',(39.4714760509134,-54.58000002,-165.282321435755));
#156858=CARTESIAN_POINT('Ctrl Pts',(33.8932339485135,-56.0200282137318,
-163.608339894981));
#156859=CARTESIAN_POINT('Ctrl Pts',(35.0808115183432,-54.5800000200163,
-162.752463904168));
#156860=CARTESIAN_POINT('Ctrl Pts',(36.7030946909167,-54.58000002,-161.495162061412));
#156861=CARTESIAN_POINT('Ctrl Pts',(31.1382389079697,-55.9113782125501,
-159.951555016761));
#156862=CARTESIAN_POINT('Ctrl Pts',(32.2640061692936,-54.5800000199999,
-159.057279891091));
#156863=CARTESIAN_POINT('Ctrl Pts',(33.7983252138975,-54.58000002,-157.838463708057));
#156864=CARTESIAN_POINT('',(39.5000000000002,-54.58000002,-165.390538702985));
#156865=CARTESIAN_POINT('Ctrl Pts',(39.2122207971107,-56.015038232057,-171.050417750959));
#156866=CARTESIAN_POINT('Ctrl Pts',(39.217277668066,-55.9551243221841,-170.951014902235));
#156867=CARTESIAN_POINT('Ctrl Pts',(39.2225737764226,-55.8953485378391,
-170.846909763433));
#156868=CARTESIAN_POINT('Ctrl Pts',(39.2281136244437,-55.8361395590084,
-170.738013265696));
#156869=CARTESIAN_POINT('Ctrl Pts',(39.2329744614731,-55.7841877372847,
-170.642464050889));
#156870=CARTESIAN_POINT('Ctrl Pts',(39.2380229477203,-55.732672178747,-170.543226083457));
#156871=CARTESIAN_POINT('Ctrl Pts',(39.2432615363417,-55.6818511882625,
-170.440250573425));
#156872=CARTESIAN_POINT('Ctrl Pts',(39.2486908746011,-55.6291796830242,
-170.333525476877));
#156873=CARTESIAN_POINT('Ctrl Pts',(39.2543239888344,-55.5772600009846,
-170.22279399802));
#156874=CARTESIAN_POINT('Ctrl Pts',(39.2601606430054,-55.5263531464095,
-170.108059909242));
#156875=CARTESIAN_POINT('Ctrl Pts',(39.2655922070714,-55.4789794569764,
-170.001288883325));
#156876=CARTESIAN_POINT('Ctrl Pts',(39.2712000221776,-55.4324830581944,
-169.891051881756));
#156877=CARTESIAN_POINT('Ctrl Pts',(39.2769824136889,-55.3870332559345,
-169.777380931684));
#156878=CARTESIAN_POINT('Ctrl Pts',(39.2774136687668,-55.3836435757349,
-169.768903267325));
#156879=CARTESIAN_POINT('Ctrl Pts',(39.2778458943164,-55.3802596954691,
-169.76040651352));
#156880=CARTESIAN_POINT('Ctrl Pts',(39.2782790893708,-55.3768816747099,
-169.751890688863));
#156881=CARTESIAN_POINT('Ctrl Pts',(39.2786817731338,-55.3737415785869,
-169.743974660545));
#156882=CARTESIAN_POINT('Ctrl Pts',(39.2791846505417,-55.3698374844174,
-169.734088992016));
#156883=CARTESIAN_POINT('Ctrl Pts',(39.2794897333218,-55.3674765853668,
-169.728093195798));
#156884=CARTESIAN_POINT('Ctrl Pts',(39.2796754514722,-55.3660393957464,
-169.724443274347));
#156885=CARTESIAN_POINT('Ctrl Pts',(39.279861545757,-55.3646017242543,-169.720785919229));
#156886=CARTESIAN_POINT('Ctrl Pts',(39.2800480163202,-55.3631635898699,
-169.717121128618));
#156887=CARTESIAN_POINT('Ctrl Pts',(39.2896637468172,-55.2890032912071,
-169.528138812898));
#156888=CARTESIAN_POINT('Ctrl Pts',(39.3002819901101,-55.2136805673814,
-169.319346539255));
#156889=CARTESIAN_POINT('Ctrl Pts',(39.3119342062424,-55.1403994795761,
-169.090262204253));
#156890=CARTESIAN_POINT('Ctrl Pts',(39.3182997955631,-55.1003661241485,
-168.965113753532));
#156891=CARTESIAN_POINT('Ctrl Pts',(39.3249727388327,-55.0609470669007,
-168.833918228421));
#156892=CARTESIAN_POINT('Ctrl Pts',(39.331953351763,-55.0226701436895,-168.69666675457));
#156893=CARTESIAN_POINT('Ctrl Pts',(39.3377950222373,-54.9906384045853,
-168.581808949051));
#156894=CARTESIAN_POINT('Ctrl Pts',(39.3438520987461,-54.9594069518665,
-168.462711233961));
#156895=CARTESIAN_POINT('Ctrl Pts',(39.3501233117751,-54.9292733027628,
-168.339396616846));
#156896=CARTESIAN_POINT('Ctrl Pts',(39.3503418056772,-54.9282234231705,
-168.33510024041));
#156897=CARTESIAN_POINT('Ctrl Pts',(39.3506232405128,-54.9268751667346,
-168.329566206783));
#156898=CARTESIAN_POINT('Ctrl Pts',(39.3507795876923,-54.9261276645024,
-168.326492141633));
#156899=CARTESIAN_POINT('Ctrl Pts',(39.3510206043589,-54.9249753540039,
-168.321753322947));
#156900=CARTESIAN_POINT('Ctrl Pts',(39.3512629457232,-54.9238198292848,
-168.316988402192));
#156901=CARTESIAN_POINT('Ctrl Pts',(39.3515066134264,-54.9226611781907,
-168.312197349974));
#156902=CARTESIAN_POINT('Ctrl Pts',(39.3552892899169,-54.9046743781474,
-168.23782146695));
#156903=CARTESIAN_POINT('Ctrl Pts',(39.3593881459255,-54.8859547368179,
-168.157216109233));
#156904=CARTESIAN_POINT('Ctrl Pts',(39.3638064495819,-54.8668806041018,
-168.070327443506));
#156905=CARTESIAN_POINT('Ctrl Pts',(39.3650116256491,-54.861677772871,-168.046626913035));
#156906=CARTESIAN_POINT('Ctrl Pts',(39.3662405652956,-54.8564488546796,
-168.022458966405));
#156907=CARTESIAN_POINT('Ctrl Pts',(39.3674933237398,-54.8512021679473,
-167.997822720973));
#156908=CARTESIAN_POINT('Ctrl Pts',(39.3705640006804,-54.8383418435663,
-167.93743601905));
#156909=CARTESIAN_POINT('Ctrl Pts',(39.3737775356156,-54.8253747693599,
-167.874238194184));
#156910=CARTESIAN_POINT('Ctrl Pts',(39.3771341911808,-54.8124307390108,
-167.808223412464));
#156911=CARTESIAN_POINT('Ctrl Pts',(39.3788125189633,-54.8059587238362,
-167.775216021605));
#156912=CARTESIAN_POINT('Ctrl Pts',(39.3805266279187,-54.7994925927265,
-167.741504369649));
#156913=CARTESIAN_POINT('Ctrl Pts',(39.3822765218251,-54.7930494106325,
-167.707088286477));
#156914=CARTESIAN_POINT('Ctrl Pts',(39.3831514687782,-54.7898278195855,
-167.689880244891));
#156915=CARTESIAN_POINT('Ctrl Pts',(39.3840353620358,-54.7866119728371,
-167.672496094056));
#156916=CARTESIAN_POINT('Ctrl Pts',(39.3849282011879,-54.7834040498743,
-167.654935829232));
#156917=CARTESIAN_POINT('Ctrl Pts',(39.3853746207639,-54.7818000883929,
-167.64615569682));
#156918=CARTESIAN_POINT('Ctrl Pts',(39.3858232768172,-54.7801981082895,
-167.637331535831));
#156919=CARTESIAN_POINT('Ctrl Pts',(39.386274169183,-54.778598385049,-167.62846334785));
#156920=CARTESIAN_POINT('Ctrl Pts',(39.3867250615487,-54.7769986618084,
-167.61959515987));
#156921=CARTESIAN_POINT('Ctrl Pts',(39.3872461308566,-54.7751632308417,
-167.609346669943));
#156922=CARTESIAN_POINT('Ctrl Pts',(39.3876335550243,-54.7738062632412,
-167.601726705049));
#156923=CARTESIAN_POINT('Ctrl Pts',(39.3938323417077,-54.752094781634,-167.479807266749));
#156924=CARTESIAN_POINT('Ctrl Pts',(39.4001106304159,-54.7322517188799,
-167.357667971969));
#156925=CARTESIAN_POINT('Ctrl Pts',(39.4063626742351,-54.7142658021284,
-167.235386059973));
#156926=CARTESIAN_POINT('Ctrl Pts',(39.4094886961447,-54.7052728437527,
-167.174245103974));
#156927=CARTESIAN_POINT('Ctrl Pts',(39.4126074508743,-54.6967440843976,
-167.113068500334));
#156928=CARTESIAN_POINT('Ctrl Pts',(39.4157054315454,-54.6886767990617,
-167.051865706899));
#156929=CARTESIAN_POINT('Ctrl Pts',(39.4172544218809,-54.6846431563937,
-167.021264310181));
#156930=CARTESIAN_POINT('Ctrl Pts',(39.4187982167228,-54.6807248694948,
-166.990656367443));
#156931=CARTESIAN_POINT('Ctrl Pts',(39.4203351387637,-54.6769215183548,
-166.960043055177));
#156932=CARTESIAN_POINT('Ctrl Pts',(39.4211035997842,-54.6750198427849,
-166.944736399044));
#156933=CARTESIAN_POINT('Ctrl Pts',(39.4218703425289,-54.6731469003953,
-166.929428400584));
#156934=CARTESIAN_POINT('Ctrl Pts',(39.4226351589158,-54.6713026337753,
-166.914119205984));
#156935=CARTESIAN_POINT('Ctrl Pts',(39.4230175671092,-54.6703805004653,
-166.906464608684));
#156936=CARTESIAN_POINT('Ctrl Pts',(39.4233994937091,-54.6694655360523,
-166.898809712353));
#156937=CARTESIAN_POINT('Ctrl Pts',(39.4237809128189,-54.6685577330597,
-166.891154535198));
#156938=CARTESIAN_POINT('Ctrl Pts',(39.4241623319288,-54.6676499300671,
-166.883499358043));
#156939=CARTESIAN_POINT('Ctrl Pts',(39.4244844603489,-54.6668873637392,
-166.877027058665));
#156940=CARTESIAN_POINT('Ctrl Pts',(39.4249334045403,-54.6658543237986,
-166.868188340615));
#156941=CARTESIAN_POINT('Ctrl Pts',(39.4250682094824,-54.6655441318147,
-166.865534329497));
#156942=CARTESIAN_POINT('Ctrl Pts',(39.4252029319403,-54.6652349867371,
-166.862881953684));
#156943=CARTESIAN_POINT('Ctrl Pts',(39.425337571846,-54.6649268850763,-166.860231214349));
#156944=CARTESIAN_POINT('Ctrl Pts',(39.4335179130109,-54.6462074966023,
-166.699179763937));
#156945=CARTESIAN_POINT('Ctrl Pts',(39.4414032837231,-54.6312933688463,
-166.54397705278));
#156946=CARTESIAN_POINT('Ctrl Pts',(39.4489876210276,-54.6195031874319,
-166.394706763715));
#156947=CARTESIAN_POINT('Ctrl Pts',(39.4545816663594,-54.6108070012453,
-166.284608184209));
#156948=CARTESIAN_POINT('Ctrl Pts',(39.4600119506171,-54.6038113708886,
-166.177736867599));
#156949=CARTESIAN_POINT('Ctrl Pts',(39.4652761839798,-54.5982610012924,
-166.074124550311));
#156950=CARTESIAN_POINT('Ctrl Pts',(39.4723661788121,-54.590785631368,-165.934577014416));
#156951=CARTESIAN_POINT('Ctrl Pts',(39.4791552957939,-54.5859295459294,
-165.80093473994));
#156952=CARTESIAN_POINT('Ctrl Pts',(39.4856401196765,-54.5831141206687,
-165.673267756554));
#156953=CARTESIAN_POINT('Ctrl Pts',(39.4906056246988,-54.5809583168219,
-165.575511663456));
#156954=CARTESIAN_POINT('Ctrl Pts',(39.4953927244241,-54.58000002,-165.481258862479));
#156955=CARTESIAN_POINT('Ctrl Pts',(39.5,-54.58000002,-165.390538702986));
#156956=CARTESIAN_POINT('',(33.85,-54.58000002,-157.903547609535));
#156957=CARTESIAN_POINT('Ctrl Pts',(33.85,-54.58000002,-157.903547609535));
#156958=CARTESIAN_POINT('Ctrl Pts',(35.7938424480564,-54.58000002,-160.35302343361));
#156959=CARTESIAN_POINT('Ctrl Pts',(37.6706534886586,-54.58000002,-162.854283363144));
#156960=CARTESIAN_POINT('Ctrl Pts',(39.5,-54.58000002,-165.390538702986));
#156961=CARTESIAN_POINT('Ctrl Pts',(33.85,-54.58000002,-157.903547609535));
#156962=CARTESIAN_POINT('Ctrl Pts',(33.8455842717013,-54.58000002,-157.988668869387));
#156963=CARTESIAN_POINT('Ctrl Pts',(33.840905459912,-54.5809154547948,-158.078838729506));
#156964=CARTESIAN_POINT('Ctrl Pts',(33.8359628860556,-54.5831131147122,
-158.174062541897));
#156965=CARTESIAN_POINT('Ctrl Pts',(33.8312850893789,-54.5851930444324,
-158.264185147261));
#156966=CARTESIAN_POINT('Ctrl Pts',(33.826371034481,-54.5884217416172,-158.358834689519));
#156967=CARTESIAN_POINT('Ctrl Pts',(33.8212204663112,-54.5931538081737,
-158.458009249791));
#156968=CARTESIAN_POINT('Ctrl Pts',(33.8159363095128,-54.5980086088171,
-158.559756068707));
#156969=CARTESIAN_POINT('Ctrl Pts',(33.8104030224301,-54.6044458578897,
-158.666269301579));
#156970=CARTESIAN_POINT('Ctrl Pts',(33.8046223261081,-54.6128946576057,
-158.777508335281));
#156971=CARTESIAN_POINT('Ctrl Pts',(33.8003719093108,-54.6191068711921,
-158.859299910384));
#156972=CARTESIAN_POINT('Ctrl Pts',(33.7959876687427,-54.6264077104841,
-158.943647679002));
#156973=CARTESIAN_POINT('Ctrl Pts',(33.791470801607,-54.634983652183,-159.030525674615));
#156974=CARTESIAN_POINT('Ctrl Pts',(33.7892123680392,-54.6392716230325,
-159.073964672421));
#156975=CARTESIAN_POINT('Ctrl Pts',(33.7869207854566,-54.6438785762368,
-159.118036081396));
#156976=CARTESIAN_POINT('Ctrl Pts',(33.7845962600292,-54.64882901054,-159.162735578489));
#156977=CARTESIAN_POINT('Ctrl Pts',(33.7834339973156,-54.6513042276916,
-159.185085327036));
#156978=CARTESIAN_POINT('Ctrl Pts',(33.7822635001811,-54.6538653257679,
-159.207592072923));
#156979=CARTESIAN_POINT('Ctrl Pts',(33.7810847987406,-54.6565154364382,
-159.230255193116));
#156980=CARTESIAN_POINT('Ctrl Pts',(33.7804954480203,-54.6578404917734,
-159.241586753212));
#156981=CARTESIAN_POINT('Ctrl Pts',(33.7799040462578,-54.6591878009921,
-159.252957406234));
#156982=CARTESIAN_POINT('Ctrl Pts',(33.7793105974546,-54.6605577598491,
-159.264367069807));
#156983=CARTESIAN_POINT('Ctrl Pts',(33.779013873053,-54.6612427392777,-159.270071901593));
#156984=CARTESIAN_POINT('Ctrl Pts',(33.7787166368952,-54.6619333811565,
-159.275786485939));
#156985=CARTESIAN_POINT('Ctrl Pts',(33.7784188895009,-54.6626297352091,
-159.28151081218));
#156986=CARTESIAN_POINT('Ctrl Pts',(33.7783816710766,-54.6627167794657,
-159.28222635296));
#156987=CARTESIAN_POINT('Ctrl Pts',(33.7783444446642,-54.6628039129752,
-159.282942045957));
#156988=CARTESIAN_POINT('Ctrl Pts',(33.7783072102649,-54.6628911358349,
-159.283657891149));
#156989=CARTESIAN_POINT('Ctrl Pts',(33.778284912608,-54.6629433688623,-159.284086571907));
#156990=CARTESIAN_POINT('Ctrl Pts',(33.7782626120867,-54.6629956339321,
-159.284515307244));
#156991=CARTESIAN_POINT('Ctrl Pts',(33.7782403087015,-54.6630479310653,
-159.284944097156));
#156992=CARTESIAN_POINT('Ctrl Pts',(33.7782180028459,-54.6631002339908,
-159.28537293456));
#156993=CARTESIAN_POINT('Ctrl Pts',(33.77819542865,-54.6631531926069,-159.285806930388));
#156994=CARTESIAN_POINT('Ctrl Pts',(33.7781740983071,-54.663203256122,-159.28621701232));
#156995=CARTESIAN_POINT('Ctrl Pts',(33.7779674505323,-54.6636882700773,
-159.290189874781));
#156996=CARTESIAN_POINT('Ctrl Pts',(33.7778502780355,-54.6639632537656,
-159.292442549935));
#156997=CARTESIAN_POINT('Ctrl Pts',(33.7775241141409,-54.6647359837781,
-159.298713005671));
#156998=CARTESIAN_POINT('Ctrl Pts',(33.7717564466018,-54.678400432493,-159.409595615936));
#156999=CARTESIAN_POINT('Ctrl Pts',(33.7662716229799,-54.6929414485542,
-159.513746318479));
#157000=CARTESIAN_POINT('Ctrl Pts',(33.7611094668565,-54.7078021960704,
-159.611181297637));
#157001=CARTESIAN_POINT('Ctrl Pts',(33.7560582805545,-54.7223434851163,
-159.706521736841));
#157002=CARTESIAN_POINT('Ctrl Pts',(33.7513159805723,-54.7371906836515,
-159.795432098454));
#157003=CARTESIAN_POINT('Ctrl Pts',(33.7469165106161,-54.7518701986928,
-159.877921548684));
#157004=CARTESIAN_POINT('Ctrl Pts',(33.7426426249294,-54.7661306823073,
-159.958056311314));
#157005=CARTESIAN_POINT('Ctrl Pts',(33.7386922093325,-54.7802328295328,
-160.032131525696));
#157006=CARTESIAN_POINT('Ctrl Pts',(33.7350940886263,-54.7937904986563,
-160.10014960274));
#157007=CARTESIAN_POINT('Ctrl Pts',(33.7318108902886,-54.8061615446452,
-160.16221445707));
#157008=CARTESIAN_POINT('Ctrl Pts',(33.728820953291,-54.8180796425581,-160.219236030609));
#157009=CARTESIAN_POINT('Ctrl Pts',(33.7261451708852,-54.82928903124,-160.271211282608));
#157010=CARTESIAN_POINT('Ctrl Pts',(33.7232172313475,-54.8415547566755,
-160.328084515266));
#157011=CARTESIAN_POINT('Ctrl Pts',(33.7206338516712,-54.8529843457977,
-160.378943028466));
#157012=CARTESIAN_POINT('Ctrl Pts',(33.7183743345158,-54.8633229976481,
-160.423822117226));
#157013=CARTESIAN_POINT('Ctrl Pts',(33.7161148173604,-54.8736616494985,
-160.468701205986));
#157014=CARTESIAN_POINT('Ctrl Pts',(33.7141792010275,-54.8829093403809,
-160.507600869464));
#157015=CARTESIAN_POINT('Ctrl Pts',(33.7125484587061,-54.8908716103222,
-160.540547336014));
#157016=CARTESIAN_POINT('Ctrl Pts',(33.7109177163846,-54.8988338802635,
-160.573493802564));
#157017=CARTESIAN_POINT('Ctrl Pts',(33.7095906356586,-54.905511485582,-160.600488868346));
#157018=CARTESIAN_POINT('Ctrl Pts',(33.7085494778909,-54.910771945989,-160.621555337921));
#157019=CARTESIAN_POINT('Ctrl Pts',(33.7080288990071,-54.9134021761925,
-160.632088572709));
#157020=CARTESIAN_POINT('Ctrl Pts',(33.7075798767493,-54.9156790556679,
-160.64113953553));
#157021=CARTESIAN_POINT('Ctrl Pts',(33.7072007704359,-54.9175915601511,
-160.648710248803));
#157022=CARTESIAN_POINT('Ctrl Pts',(33.7070112172792,-54.9185478123928,
-160.65249560544));
#157023=CARTESIAN_POINT('Ctrl Pts',(33.7068391595856,-54.9194130241989,
-160.655910886927));
#157024=CARTESIAN_POINT('Ctrl Pts',(33.7066844261339,-54.9201861620642,
-160.658956291836));
#157025=CARTESIAN_POINT('Ctrl Pts',(33.7066271536549,-54.9204723285113,
-160.66008350697));
#157026=CARTESIAN_POINT('Ctrl Pts',(33.7065722544831,-54.9207458838973,
-160.661160051605));
#157027=CARTESIAN_POINT('Ctrl Pts',(33.7065197237176,-54.9210067805742,
-160.662185924984));
#157028=CARTESIAN_POINT('Ctrl Pts',(33.7065012931173,-54.9210983170736,
-160.6625458562));
#157029=CARTESIAN_POINT('Ctrl Pts',(33.7064831539969,-54.9211882964876,
-160.662899551137));
#157030=CARTESIAN_POINT('Ctrl Pts',(33.7064653061515,-54.9212767167715,
-160.663247009611));
#157031=CARTESIAN_POINT('Ctrl Pts',(33.7064309473279,-54.9214469343443,
-160.663915900679));
#157032=CARTESIAN_POINT('Ctrl Pts',(33.7063976681466,-54.9216113735066,
-160.664561678743));
#157033=CARTESIAN_POINT('Ctrl Pts',(33.7063654665511,-54.9217700215039,
-160.66518434624));
#157034=CARTESIAN_POINT('Ctrl Pts',(33.7063493657534,-54.9218493455026,
-160.665495679988));
#157035=CARTESIAN_POINT('Ctrl Pts',(33.7063335343563,-54.9219272217235,
-160.665801236091));
#157036=CARTESIAN_POINT('Ctrl Pts',(33.7063179721145,-54.9220036486581,
-160.666101014837));
#157037=CARTESIAN_POINT('Ctrl Pts',(33.7063101909937,-54.9220418621254,
-160.66625090421));
#157038=CARTESIAN_POINT('Ctrl Pts',(33.7063255851885,-54.921966662831,-160.665956043164));
#157039=CARTESIAN_POINT('Ctrl Pts',(33.7063294920643,-54.921947622701,-160.665881391093));
#157040=CARTESIAN_POINT('Ctrl Pts',(33.7063333989402,-54.9219285825709,
-160.665806739022));
#157041=CARTESIAN_POINT('Ctrl Pts',(33.7063258183025,-54.9219656412912,
-160.66595230046));
#157042=CARTESIAN_POINT('Ctrl Pts',(33.706272088182,-54.9222285814461,-160.666983018974));
#157043=CARTESIAN_POINT('Ctrl Pts',(33.7009078975708,-54.9484794272874,
-160.769885646496));
#157044=CARTESIAN_POINT('Ctrl Pts',(33.6956802612108,-54.975601534076,-160.869638762938));
#157045=CARTESIAN_POINT('Ctrl Pts',(33.6906131147999,-55.0033469705025,
-160.966209592634));
#157046=CARTESIAN_POINT('Ctrl Pts',(33.6852952359268,-55.0324653061955,
-161.067558938667));
#157047=CARTESIAN_POINT('Ctrl Pts',(33.6801541162865,-55.0622699904258,
-161.16540357318));
#157048=CARTESIAN_POINT('Ctrl Pts',(33.675211508873,-55.0924969827791,-161.259758725589));
#157049=CARTESIAN_POINT('Ctrl Pts',(33.6727873622862,-55.1073220850409,
-161.306036064963));
#157050=CARTESIAN_POINT('Ctrl Pts',(33.6704108807543,-55.1222491269139,
-161.351474766905));
#157051=CARTESIAN_POINT('Ctrl Pts',(33.6680841619286,-55.1372490025288,
-161.396080607222));
#157052=CARTESIAN_POINT('Ctrl Pts',(33.6629744949401,-55.1701899700473,
-161.494038721992));
#157053=CARTESIAN_POINT('Ctrl Pts',(33.6580979013176,-55.2034782520868,
-161.587960992612));
#157054=CARTESIAN_POINT('Ctrl Pts',(33.6534377421645,-55.2368194787995,
-161.677878398062));
#157055=CARTESIAN_POINT('Ctrl Pts',(33.6528122575655,-55.241294524208,-161.689947074355));
#157056=CARTESIAN_POINT('Ctrl Pts',(33.652190671613,-55.2457705620805,-161.701943669366));
#157057=CARTESIAN_POINT('Ctrl Pts',(33.651572943776,-55.2502469164948,-161.713868317027));
#157058=CARTESIAN_POINT('Ctrl Pts',(33.6489628960728,-55.2691605834178,
-161.764252802516));
#157059=CARTESIAN_POINT('Ctrl Pts',(33.6464211319758,-55.2880796832181,
-161.813351747981));
#157060=CARTESIAN_POINT('Ctrl Pts',(33.6439413334603,-55.306954917264,-161.861173480295));
#157061=CARTESIAN_POINT('Ctrl Pts',(33.6427014342026,-55.3163925342869,
-161.885084346451));
#157062=CARTESIAN_POINT('Ctrl Pts',(33.6414770339499,-55.3258191988819,
-161.908675903486));
#157063=CARTESIAN_POINT('Ctrl Pts',(33.6402671210953,-55.3352290373697,
-161.93194933418));
#157064=CARTESIAN_POINT('Ctrl Pts',(33.639662164668,-55.3399339566135,-161.943586049527));
#157065=CARTESIAN_POINT('Ctrl Pts',(33.6390608306291,-55.3446346703723,
-161.955143232875));
#157066=CARTESIAN_POINT('Ctrl Pts',(33.6384629894247,-55.349330455341,-161.96662103369));
#157067=CARTESIAN_POINT('Ctrl Pts',(33.6381640688225,-55.3516783478254,
-161.972359934098));
#157068=CARTESIAN_POINT('Ctrl Pts',(33.6378660214631,-55.3540250081756,
-161.978078988847));
#157069=CARTESIAN_POINT('Ctrl Pts',(33.6375688304508,-55.3563703470497,
-161.983778217058));
#157070=CARTESIAN_POINT('Ctrl Pts',(33.6373398167457,-55.3581776518568,
-161.988170009928));
#157071=CARTESIAN_POINT('Ctrl Pts',(33.6371703141945,-55.3595177060693,
-161.991420282418));
#157072=CARTESIAN_POINT('Ctrl Pts',(33.6369239026404,-55.361468542626,-161.996140872168));
#157073=CARTESIAN_POINT('Ctrl Pts',(33.636850545999,-55.3620493060492,-161.997546190237));
#157074=CARTESIAN_POINT('Ctrl Pts',(33.636770374559,-55.3626842991758,-161.999081790039));
#157075=CARTESIAN_POINT('Ctrl Pts',(33.6366797957947,-55.3634022825266,
-162.00081644943));
#157076=CARTESIAN_POINT('Ctrl Pts',(33.6303630969412,-55.4134723474333,
-162.121786536301));
#157077=CARTESIAN_POINT('Ctrl Pts',(33.6242642048687,-55.4647929755218,
-162.238561065914));
#157078=CARTESIAN_POINT('Ctrl Pts',(33.6183832363913,-55.5171199863229,
-162.351143940503));
#157079=CARTESIAN_POINT('Ctrl Pts',(33.6124477006515,-55.5699325194892,
-162.464771428624));
#157080=CARTESIAN_POINT('Ctrl Pts',(33.6067341407565,-55.6237697200541,
-162.574129314741));
#157081=CARTESIAN_POINT('Ctrl Pts',(33.6012414339651,-55.67832637603,-162.679244507083));
#157082=CARTESIAN_POINT('Ctrl Pts',(33.5953685243728,-55.7366594202596,
-162.791635727812));
#157083=CARTESIAN_POINT('Ctrl Pts',(33.5897480982937,-55.7958148333295,
-162.899176624726));
#157084=CARTESIAN_POINT('Ctrl Pts',(33.5843774549044,-55.8553619694533,
-163.001924469437));
#157085=CARTESIAN_POINT('Ctrl Pts',(33.5798407181868,-55.90566314555,-163.088718524814));
#157086=CARTESIAN_POINT('Ctrl Pts',(33.5754821883936,-55.956242546843,-163.172092965307));
#157087=CARTESIAN_POINT('Ctrl Pts',(33.5712996217319,-56.0068141405006,
-163.252093549704));
#157088=CARTESIAN_POINT('Origin',(60.,-54.58000002,-55.24995));
#157089=CARTESIAN_POINT('',(39.4999999999985,-54.58000002,-66.6681042685273));
#157090=CARTESIAN_POINT('',(39.5,-54.58000002,-65.9723506080548));
#157091=CARTESIAN_POINT('',(33.8499999999899,-54.58000002,-74.1550953619836));
#157092=CARTESIAN_POINT('Ctrl Pts',(39.4999999999959,-54.58000002,-66.6681042685264));
#157093=CARTESIAN_POINT('Ctrl Pts',(37.6706537603941,-54.58000002,-69.204359231621));
#157094=CARTESIAN_POINT('Ctrl Pts',(35.7938421862428,-54.58000002,-71.7056198678132));
#157095=CARTESIAN_POINT('Ctrl Pts',(33.8499999999899,-54.58000002,-74.1550953619836));
#157096=CARTESIAN_POINT('',(33.85,-54.58000002,-157.276549545042));
#157097=CARTESIAN_POINT('Origin',(-3.54807775957937E-14,-73.08000002,3.11172719585489E-30));
#157098=CARTESIAN_POINT('',(40.5,-73.08000002,-174.34995));
#157099=CARTESIAN_POINT('',(41.,-73.08000002,-174.34995));
#157100=CARTESIAN_POINT('',(41.5,-73.08000002,-174.34995));
#157101=CARTESIAN_POINT('',(41.,-73.08000002,-58.24995));
#157102=CARTESIAN_POINT('',(41.,-73.08000002,-58.24995));
#157103=CARTESIAN_POINT('',(40.5,-73.08000002,-58.24995));
#157104=CARTESIAN_POINT('',(-41.5,-73.0800000199999,-58.24995));
#157105=CARTESIAN_POINT('',(40.5,-73.08000002,-174.34995));
#157106=CARTESIAN_POINT('Origin',(-3.3975957231091E-14,-70.08000002,-174.34995));
#157107=CARTESIAN_POINT('',(41.,-70.08000002,-177.34995));
#157108=CARTESIAN_POINT('',(40.5,-70.08000002,-177.34995));
#157109=CARTESIAN_POINT('',(-41.5,-70.08000002,-177.34995));
#157110=CARTESIAN_POINT('Origin',(41.,-70.08000002,-174.34995));
#157111=CARTESIAN_POINT('Origin',(40.5,-70.08000002,-174.34995));
#157112=CARTESIAN_POINT('Origin',(41.5,-73.08000002,-177.34995));
#157113=CARTESIAN_POINT('',(40.5,-63.9875867194884,-177.34995));
#157114=CARTESIAN_POINT('',(40.5,-73.08000002,-177.34995));
#157115=CARTESIAN_POINT('',(41.,-63.9173163021373,-177.34995));
#157116=CARTESIAN_POINT('',(40.227526467895,-64.0258803771248,-177.34995));
#157117=CARTESIAN_POINT('',(41.,-73.08000002,-177.34995));
#157118=CARTESIAN_POINT('Origin',(0.,-12.9675000200281,-60.64995));
#157119=CARTESIAN_POINT('',(38.8323576630952,-56.2084583512428,-61.2273323469212));
#157120=CARTESIAN_POINT('',(33.5881101525803,-60.3971457002532,-61.2273317382593));
#157121=CARTESIAN_POINT('Origin',(0.,-12.9675000200281,-61.2273317382593));
#157122=CARTESIAN_POINT('',(33.5713955981572,-56.0068423841383,-68.80655523181));
#157123=CARTESIAN_POINT('Ctrl Pts',(33.5881101525803,-60.3971457002532,
-61.2273317382593));
#157124=CARTESIAN_POINT('Ctrl Pts',(33.5859966234634,-59.8194297837461,
-62.2410161014668));
#157125=CARTESIAN_POINT('Ctrl Pts',(33.5838660751903,-59.2475976035343,
-63.2383627339802));
#157126=CARTESIAN_POINT('Ctrl Pts',(33.5817197112415,-58.6815774556952,
-64.2193509751279));
#157127=CARTESIAN_POINT('Ctrl Pts',(33.579516248939,-58.1004998341978,-65.2264358219469));
#157128=CARTESIAN_POINT('Ctrl Pts',(33.5772961193852,-57.5255476663152,
-66.2162804051611));
#157129=CARTESIAN_POINT('Ctrl Pts',(33.5750610470281,-56.9566908458864,
-67.1888908421399));
#157130=CARTESIAN_POINT('Ctrl Pts',(33.5738095983383,-56.6381798498937,
-67.7334692103161));
#157131=CARTESIAN_POINT('Ctrl Pts',(33.5725534724423,-56.3215806067112,
-68.2726451091889));
#157132=CARTESIAN_POINT('Ctrl Pts',(33.5712930253538,-56.006893899348,-68.8064232518886));
#157133=CARTESIAN_POINT('Ctrl Pts',(33.5716649935586,-56.0068714411552,
-68.8066912637494));
#157134=CARTESIAN_POINT('Ctrl Pts',(34.023338992169,-56.0244950519456,-68.1812988971121));
#157135=CARTESIAN_POINT('Ctrl Pts',(34.477894463698,-56.042167524175,-67.5449502682449));
#157136=CARTESIAN_POINT('Ctrl Pts',(34.9354108072308,-56.0598757513079,
-66.8975869283598));
#157137=CARTESIAN_POINT('Ctrl Pts',(35.3815636085019,-56.0771441511205,
-66.2663024472423));
#157138=CARTESIAN_POINT('Ctrl Pts',(35.8305319442804,-56.094446553343,-65.6245433868767));
#157139=CARTESIAN_POINT('Ctrl Pts',(36.2823935541714,-56.1117690245108,
-64.9723033619553));
#157140=CARTESIAN_POINT('Ctrl Pts',(36.7172567195688,-56.1284398469034,
-64.3445997561884));
#157141=CARTESIAN_POINT('Ctrl Pts',(37.1547995097133,-56.1451292541387,
-63.7071888252589));
#157142=CARTESIAN_POINT('Ctrl Pts',(37.5950960941535,-56.1618231713757,
-63.0601118262641));
#157143=CARTESIAN_POINT('Ctrl Pts',(38.0051074962401,-56.177368820955,-62.4575431101039));
#157144=CARTESIAN_POINT('Ctrl Pts',(38.41750687348,-56.1929183711655,-61.846592510695));
#157145=CARTESIAN_POINT('Ctrl Pts',(38.8323589160537,-56.2084590974991,
-61.2273337386071));
#157146=CARTESIAN_POINT('Ctrl Pts',(42.0182169324382,-54.58000002,-63.1137016214078));
#157147=CARTESIAN_POINT('Ctrl Pts',(40.2048288919875,-54.58000002,-61.850776413383));
#157148=CARTESIAN_POINT('Ctrl Pts',(38.9841065328395,-56.2141391785318,
-61.0006103127042));
#157149=CARTESIAN_POINT('Ctrl Pts',(39.3891852844759,-54.58000002,-66.8886318537073));
#157150=CARTESIAN_POINT('Ctrl Pts',(37.6731521867469,-54.58000002,-65.6186857176609));
#157151=CARTESIAN_POINT('Ctrl Pts',(36.4598290914011,-56.1197282395838,
-64.7755113243629));
#157152=CARTESIAN_POINT('Ctrl Pts',(36.6602985783386,-54.58000002,-70.6173011253171));
#157153=CARTESIAN_POINT('Ctrl Pts',(35.039043742113,-54.58000002,-69.3609187351473));
#157154=CARTESIAN_POINT('Ctrl Pts',(33.8526449461492,-56.018427265929,-68.5041285748648));
#157155=CARTESIAN_POINT('Ctrl Pts',(33.7990997127136,-54.58000002,-74.2192042704808));
#157156=CARTESIAN_POINT('Ctrl Pts',(32.2647524970408,-54.5800000199999,
-73.0003840144137));
#157157=CARTESIAN_POINT('Ctrl Pts',(31.1389734555133,-55.9114071812081,
-72.1061129617773));
#157158=CARTESIAN_POINT('',(39.2253966502056,-55.8655297208509,-61.2672223984388));
#157159=CARTESIAN_POINT('Ctrl Pts',(39.4999999999998,-54.58000002,-66.6681042685264));
#157160=CARTESIAN_POINT('Ctrl Pts',(39.495523236403,-54.58000002,-66.5799539738083));
#157161=CARTESIAN_POINT('Ctrl Pts',(39.4908202961929,-54.5808808281515,
-66.4866281324533));
#157162=CARTESIAN_POINT('Ctrl Pts',(39.4858571267135,-54.5829895419112,
-66.3881202588974));
#157163=CARTESIAN_POINT('Ctrl Pts',(39.480993916126,-54.5850557858959,-66.2915963469858));
#157164=CARTESIAN_POINT('Ctrl Pts',(39.4758808544998,-54.5883008850007,
-66.1900969985362));
#157165=CARTESIAN_POINT('Ctrl Pts',(39.4704844413006,-54.5931012842766,
-66.0836227128787));
#157166=CARTESIAN_POINT('Ctrl Pts',(39.4697336068659,-54.5937691918188,
-66.0688083246691));
#157167=CARTESIAN_POINT('Ctrl Pts',(39.4689772847685,-54.5944672898739,
-66.0538976389502));
#157168=CARTESIAN_POINT('Ctrl Pts',(39.468215382555,-54.595196672676,-66.0388906681808));
#157169=CARTESIAN_POINT('Ctrl Pts',(39.4623021949749,-54.6008574743503,
-65.9224202975833));
#157170=CARTESIAN_POINT('Ctrl Pts',(39.4560603818811,-54.6083970407844,
-65.8001528088562));
#157171=CARTESIAN_POINT('Ctrl Pts',(39.4495103135196,-54.6183556248677,
-65.6721332133175));
#157172=CARTESIAN_POINT('Ctrl Pts',(39.4462352793388,-54.6233349169094,
-65.6081234155481));
#157173=CARTESIAN_POINT('Ctrl Pts',(39.4428839973304,-54.6289198642788,
-65.5426762103419));
#157174=CARTESIAN_POINT('Ctrl Pts',(39.4394645933395,-54.6351826677793,
-65.4758013974786));
#157175=CARTESIAN_POINT('Ctrl Pts',(39.437754891344,-54.6383140695295,-65.442363991047));
#157176=CARTESIAN_POINT('Ctrl Pts',(39.4360281696955,-54.6416149880493,
-65.4085696904452));
#157177=CARTESIAN_POINT('Ctrl Pts',(39.4342859048123,-54.6450946615458,
-65.3744200607822));
#157178=CARTESIAN_POINT('Ctrl Pts',(39.4334147723707,-54.646834498294,-65.3573452459507));
#157179=CARTESIAN_POINT('Ctrl Pts',(39.4325397546503,-54.6486190265432,
-65.3401815992333));
#157180=CARTESIAN_POINT('Ctrl Pts',(39.4316610537463,-54.6504494140905,
-65.3229293289581));
#157181=CARTESIAN_POINT('Ctrl Pts',(39.4312217032943,-54.6513646078642,
-65.3143031938205));
#157182=CARTESIAN_POINT('Ctrl Pts',(39.4307814320818,-54.6522912666236,
-65.305654902819));
#157183=CARTESIAN_POINT('Ctrl Pts',(39.4303402670448,-54.6532295369723,
-65.2969844832221));
#157184=CARTESIAN_POINT('Ctrl Pts',(39.430009393267,-54.6539332397338,-65.2904816685244));
#157185=CARTESIAN_POINT('Ctrl Pts',(39.4296780167157,-54.6546434740272,
-65.2839664064937));
#157186=CARTESIAN_POINT('Ctrl Pts',(39.4293461491344,-54.6553603018509,
-65.2774387089119));
#157187=CARTESIAN_POINT('Ctrl Pts',(39.4292355266072,-54.6555992444588,
-65.2752628097179));
#157188=CARTESIAN_POINT('Ctrl Pts',(39.4291942240796,-54.6556882995562,
-65.274450489437));
#157189=CARTESIAN_POINT('Ctrl Pts',(39.4290141183437,-54.6560793298168,
-65.2709068666062));
#157190=CARTESIAN_POINT('Ctrl Pts',(39.4232507347946,-54.6685922981555,
-65.1575109360216));
#157191=CARTESIAN_POINT('Ctrl Pts',(39.4178450815666,-54.6819071044714,
-65.0511646649134));
#157192=CARTESIAN_POINT('Ctrl Pts',(39.4127966639773,-54.6954925733759,
-64.9518535498794));
#157193=CARTESIAN_POINT('Ctrl Pts',(39.4079368016429,-54.7085706334722,
-64.8562516431812));
#157194=CARTESIAN_POINT('Ctrl Pts',(39.4034079875762,-54.7218995863115,
-64.7671691893792));
#157195=CARTESIAN_POINT('Ctrl Pts',(39.3992100712441,-54.7350554540221,
-64.6845997089738));
#157196=CARTESIAN_POINT('Ctrl Pts',(39.3950616267999,-54.7480562815743,
-64.6030032989584));
#157197=CARTESIAN_POINT('Ctrl Pts',(39.3912363253505,-54.7608879647296,
-64.5277672359874));
#157198=CARTESIAN_POINT('Ctrl Pts',(39.3877343287418,-54.7731916269955,
-64.4588918939396));
#157199=CARTESIAN_POINT('Ctrl Pts',(39.3842823576569,-54.7853195331948,
-64.3910004263623));
#157200=CARTESIAN_POINT('Ctrl Pts',(39.3811445195931,-54.796934330417,-64.3292892396896));
#157201=CARTESIAN_POINT('Ctrl Pts',(39.3783212885897,-54.8077427493247,
-64.2737654283553));
#157202=CARTESIAN_POINT('Ctrl Pts',(39.3778747135099,-54.809452411244,-64.2649827426853));
#157203=CARTESIAN_POINT('Ctrl Pts',(39.3774360107346,-54.8111420022469,
-64.2563548824163));
#157204=CARTESIAN_POINT('Ctrl Pts',(39.3770051829108,-54.8128104810774,
-64.2478818916985));
#157205=CARTESIAN_POINT('Ctrl Pts',(39.3743361892215,-54.8231467667669,
-64.1953914128839));
#157206=CARTESIAN_POINT('Ctrl Pts',(39.371967988214,-54.8326738045252,-64.1488179262381));
#157207=CARTESIAN_POINT('Ctrl Pts',(39.369899295881,-54.8411825869057,-64.1081353024567));
#157208=CARTESIAN_POINT('Ctrl Pts',(39.3678433023701,-54.8496391374912,
-64.0677024119946));
#157209=CARTESIAN_POINT('Ctrl Pts',(39.3660831513506,-54.857089892747,-64.03308828041));
#157210=CARTESIAN_POINT('Ctrl Pts',(39.3646179182847,-54.8633802441861,
-64.0042741362313));
#157211=CARTESIAN_POINT('Ctrl Pts',(39.3631516508793,-54.8696750361198,
-63.9754396515278));
#157212=CARTESIAN_POINT('Ctrl Pts',(39.3619807133368,-54.8748077492079,
-63.9524132576399));
#157213=CARTESIAN_POINT('Ctrl Pts',(39.3611042771126,-54.8786758154394,
-63.9351782941354));
#157214=CARTESIAN_POINT('Ctrl Pts',(39.3602895559443,-54.8822715082603,
-63.9191569463013));
#157215=CARTESIAN_POINT('Ctrl Pts',(39.3597293339265,-54.8847748380768,
-63.9081403809706));
#157216=CARTESIAN_POINT('Ctrl Pts',(39.3594232718812,-54.8861432861055,
-63.9021217828994));
#157217=CARTESIAN_POINT('Ctrl Pts',(39.3593226039518,-54.8865933870957,
-63.9001421849207));
#157218=CARTESIAN_POINT('Ctrl Pts',(39.359249433704,-54.8869210418335,-63.8987033204161));
#157219=CARTESIAN_POINT('Ctrl Pts',(39.3592037570943,-54.8871256249942,
-63.8978051077709));
#157220=CARTESIAN_POINT('Ctrl Pts',(39.3591935404627,-54.8871713847563,
-63.8976042017099));
#157221=CARTESIAN_POINT('Ctrl Pts',(39.3591846993252,-54.8872109892174,
-63.8974303442201));
#157222=CARTESIAN_POINT('Ctrl Pts',(39.3591772336508,-54.8872444346251,
-63.8972835346803));
#157223=CARTESIAN_POINT('Ctrl Pts',(39.3591735008137,-54.8872611573289,
-63.8972101299104));
#157224=CARTESIAN_POINT('Ctrl Pts',(39.3591701118425,-54.8872763402874,
-63.8971434871318));
#157225=CARTESIAN_POINT('Ctrl Pts',(39.3591670667343,-54.887289983141,-63.8970836062849));
#157226=CARTESIAN_POINT('Ctrl Pts',(39.3591655441802,-54.8872968045678,
-63.8970536658614));
#157227=CARTESIAN_POINT('Ctrl Pts',(39.3591900763927,-54.8871869022241,
-63.8975360766884));
#157228=CARTESIAN_POINT('Ctrl Pts',(39.3592017106449,-54.8871347946242,
-63.897764848134));
#157229=CARTESIAN_POINT('Ctrl Pts',(39.359213344897,-54.8870826870244,-63.8979936195796));
#157230=CARTESIAN_POINT('Ctrl Pts',(39.3592120810124,-54.8870883035032,
-63.8979687479432));
#157231=CARTESIAN_POINT('Ctrl Pts',(39.3591589665828,-54.8873262900705,
-63.8969242492737));
#157232=CARTESIAN_POINT('Ctrl Pts',(39.3534773448721,-54.9127835840158,
-63.7851947934758));
#157233=CARTESIAN_POINT('Ctrl Pts',(39.3479856206203,-54.9391109216136,
-63.6772073597653));
#157234=CARTESIAN_POINT('Ctrl Pts',(39.3426855452689,-54.966034304412,-63.5729933103322));
#157235=CARTESIAN_POINT('Ctrl Pts',(39.337116117579,-54.9943259462696,-63.4634830535726));
#157236=CARTESIAN_POINT('Ctrl Pts',(39.3317582956126,-55.0232755056928,
-63.3581391118471));
#157237=CARTESIAN_POINT('Ctrl Pts',(39.3266113718449,-55.052586215412,-63.2569443988532));
#157238=CARTESIAN_POINT('Ctrl Pts',(39.3249343634493,-55.0621364455105,
-63.2239723963631));
#157239=CARTESIAN_POINT('Ctrl Pts',(39.3232797251223,-55.071725193134,-63.1914405077103));
#157240=CARTESIAN_POINT('Ctrl Pts',(39.3216473789753,-55.0813427108627,
-63.159347100086));
#157241=CARTESIAN_POINT('Ctrl Pts',(39.3163246960283,-55.1127030921774,
-63.0546983196863));
#157242=CARTESIAN_POINT('Ctrl Pts',(39.3112522088888,-55.1443595066673,
-62.954726789106));
#157243=CARTESIAN_POINT('Ctrl Pts',(39.3064521227518,-55.1759617601416,
-62.8593924163544));
#157244=CARTESIAN_POINT('Ctrl Pts',(39.306107452178,-55.1782309625117,-62.8525469239979));
#157245=CARTESIAN_POINT('Ctrl Pts',(39.3057641849582,-55.1804998949383,
-62.845725320774));
#157246=CARTESIAN_POINT('Ctrl Pts',(39.3054223287976,-55.1827684321607,
-62.8389275828999));
#157247=CARTESIAN_POINT('Ctrl Pts',(39.3028709552403,-55.1996991958884,
-62.7881940561616));
#157248=CARTESIAN_POINT('Ctrl Pts',(39.3003875354856,-55.2166118918502,
-62.7387919172498));
#157249=CARTESIAN_POINT('Ctrl Pts',(39.2979654360815,-55.2334594185815,
-62.6907137704932));
#157250=CARTESIAN_POINT('Ctrl Pts',(39.2967543863794,-55.2418831819471,
-62.6666746971149));
#157251=CARTESIAN_POINT('Ctrl Pts',(39.2955586742956,-55.250290669231,-62.6429666270713));
#157252=CARTESIAN_POINT('Ctrl Pts',(39.2943772688074,-55.2586762672058,
-62.6195885146807));
#157253=CARTESIAN_POINT('Ctrl Pts',(39.2937865660632,-55.2628690661932,
-62.6078994584855));
#157254=CARTESIAN_POINT('Ctrl Pts',(39.2931994405157,-55.2670563940624,
-62.5962928920887));
#157255=CARTESIAN_POINT('Ctrl Pts',(39.2926157608318,-55.2712375603914,
-62.58476868362));
#157256=CARTESIAN_POINT('Ctrl Pts',(39.2923239209898,-55.2733281435559,
-62.5790065793857));
#157257=CARTESIAN_POINT('Ctrl Pts',(39.2920329426495,-55.2754171864107,
-62.5732650646585));
#157258=CARTESIAN_POINT('Ctrl Pts',(39.2917428087709,-55.2775046036935,
-62.5675441225895));
#157259=CARTESIAN_POINT('Ctrl Pts',(39.2915090535797,-55.2791863949705,
-62.5629348714603));
#157260=CARTESIAN_POINT('Ctrl Pts',(39.2913400018075,-55.2804046703665,
-62.5596019669335));
#157261=CARTESIAN_POINT('Ctrl Pts',(39.2910805711966,-55.2822769572449,
-62.554492614977));
#157262=CARTESIAN_POINT('Ctrl Pts',(39.2910179999347,-55.2827285282922,
-62.5532603062746));
#157263=CARTESIAN_POINT('Ctrl Pts',(39.29095017263,-55.2832182167915,-62.5519246872481));
#157264=CARTESIAN_POINT('Ctrl Pts',(39.2908749168058,-55.2837618804591,
-62.5504429930271));
#157265=CARTESIAN_POINT('Ctrl Pts',(39.2844820573665,-55.3299452216857,
-62.4245754872765));
#157266=CARTESIAN_POINT('Ctrl Pts',(39.2782741629842,-55.3774330170781,
-62.3027126717482));
#157267=CARTESIAN_POINT('Ctrl Pts',(39.2722610566445,-55.4260061918257,
-62.1848677196681));
#157268=CARTESIAN_POINT('Ctrl Pts',(39.2660766425471,-55.4759631707472,
-62.0636654754735));
#157269=CARTESIAN_POINT('Ctrl Pts',(39.26009828666,-55.5270679896246,-61.946713217043));
#157270=CARTESIAN_POINT('Ctrl Pts',(39.254335463863,-55.5790290546349,-61.8340043906321));
#157271=CARTESIAN_POINT('Ctrl Pts',(39.2482258756724,-55.6341167643111,
-61.7145135544448));
#157272=CARTESIAN_POINT('Ctrl Pts',(39.2423585567611,-55.6901667039142,
-61.5997921748508));
#157273=CARTESIAN_POINT('Ctrl Pts',(39.2367431964852,-55.7467753028942,
-61.4898098101459));
#157274=CARTESIAN_POINT('Ctrl Pts',(39.2328382758321,-55.7861409137256,
-61.4133280910202));
#157275=CARTESIAN_POINT('Ctrl Pts',(39.2290551619518,-55.8257754618418,
-61.3391375767458));
#157276=CARTESIAN_POINT('Ctrl Pts',(39.2253966502057,-55.8655297208508,
-61.2672223984388));
#157277=CARTESIAN_POINT('Ctrl Pts',(39.2253966502054,-55.865529720851,-61.2672223984388));
#157278=CARTESIAN_POINT('Ctrl Pts',(39.0894849099381,-55.973106721351,-61.2534405956196));
#157279=CARTESIAN_POINT('Ctrl Pts',(38.9583675005087,-56.087272628509,-61.2401323247394));
#157280=CARTESIAN_POINT('Ctrl Pts',(38.8323573704738,-56.2084579968516,
-61.2273318724241));
#157281=CARTESIAN_POINT('Ctrl Pts',(33.5713705761603,-56.0068466996901,
-68.8065662520943));
#157282=CARTESIAN_POINT('Ctrl Pts',(33.5716407255132,-56.0065270796914,
-68.8073048104027));
#157283=CARTESIAN_POINT('Ctrl Pts',(33.571763596338,-56.0045950124546,-68.8104067087827));
#157284=CARTESIAN_POINT('Ctrl Pts',(33.5721706506023,-55.9991005135222,
-68.8191908544081));
#157285=CARTESIAN_POINT('Ctrl Pts',(33.5724492473124,-55.9954676511144,
-68.8249939058348));
#157286=CARTESIAN_POINT('Ctrl Pts',(33.5728282689527,-55.9907549991229,
-68.8325305810644));
#157287=CARTESIAN_POINT('Ctrl Pts',(33.5731041457865,-55.9873742312304,
-68.8379409991175));
#157288=CARTESIAN_POINT('Ctrl Pts',(33.5733343137518,-55.9846017185724,
-68.8423820318139));
#157289=CARTESIAN_POINT('Ctrl Pts',(33.5740628471358,-55.9759052979108,
-68.8563203448581));
#157290=CARTESIAN_POINT('Ctrl Pts',(33.5747259271068,-55.9680435604782,
-68.8690049728665));
#157291=CARTESIAN_POINT('Ctrl Pts',(33.5766727727727,-55.9451279534846,
-68.9062215166601));
#157292=CARTESIAN_POINT('Ctrl Pts',(33.5780152783015,-55.9295406414513,
-68.9318763717004));
#157293=CARTESIAN_POINT('Ctrl Pts',(33.5806116739953,-55.8998032246295,
-68.9814610011427));
#157294=CARTESIAN_POINT('Ctrl Pts',(33.5819227551623,-55.8849811468815,
-69.0064972151006));
#157295=CARTESIAN_POINT('Ctrl Pts',(33.5845705352917,-55.8554389192834,
-69.0570579760427));
#157296=CARTESIAN_POINT('Ctrl Pts',(33.5859648027717,-55.8400931028538,
-69.0836819419351));
#157297=CARTESIAN_POINT('Ctrl Pts',(33.5898400697109,-55.7979757190093,
-69.1576904032815));
#157298=CARTESIAN_POINT('Ctrl Pts',(33.5937887266916,-55.7560919721939,
-69.2331703700131));
#157299=CARTESIAN_POINT('Ctrl Pts',(33.5985250010602,-55.7077292668964,
-69.3238132173549));
#157300=CARTESIAN_POINT('Ctrl Pts',(33.6005822539447,-55.6871201048491,
-69.3632141538798));
#157301=CARTESIAN_POINT('Ctrl Pts',(33.6019597992385,-55.6734079620416,
-69.3896046055977));
#157302=CARTESIAN_POINT('Ctrl Pts',(33.6027160054383,-55.6659325257803,
-69.4040961057493));
#157303=CARTESIAN_POINT('Ctrl Pts',(33.6083893848232,-55.6101758456577,
-69.5128495384139));
#157304=CARTESIAN_POINT('Ctrl Pts',(33.6136342702573,-55.5608215111131,
-69.613836091737));
#157305=CARTESIAN_POINT('Ctrl Pts',(33.6218546903343,-55.4875927031781,
-69.7718651036816));
#157306=CARTESIAN_POINT('Ctrl Pts',(33.6260524855428,-55.4511796496671,
-69.8525164490197));
#157307=CARTESIAN_POINT('Ctrl Pts',(33.6311062438331,-55.4091644471695,
-69.9494849851258));
#157308=CARTESIAN_POINT('Ctrl Pts',(33.633671936046,-55.3882882683558,-69.9986889872937));
#157309=CARTESIAN_POINT('Ctrl Pts',(33.6347797887555,-55.3793710855899,
-70.0199307304866));
#157310=CARTESIAN_POINT('Ctrl Pts',(33.6355201880339,-55.3734330861315,
-70.0341261927124));
#157311=CARTESIAN_POINT('Ctrl Pts',(33.6359696672266,-55.3698435365156,
-70.0427433731727));
#157312=CARTESIAN_POINT('Ctrl Pts',(33.6456605291765,-55.2926836875688,
-70.228524654433));
#157313=CARTESIAN_POINT('Ctrl Pts',(33.6559356302676,-55.2164164760441,
-70.4286045583069));
#157314=CARTESIAN_POINT('Ctrl Pts',(33.673171806379,-55.1046321197711,-70.7593432066334));
#157315=CARTESIAN_POINT('Ctrl Pts',(33.6792132916678,-55.0678175042389,
-70.8746875304398));
#157316=CARTESIAN_POINT('Ctrl Pts',(33.6886934938914,-55.0139506128507,
-71.0553819190524));
#157317=CARTESIAN_POINT('Ctrl Pts',(33.6935370007537,-54.987356742398,-71.1476478424839));
#157318=CARTESIAN_POINT('Ctrl Pts',(33.6993504871532,-54.9570822780224,
-71.2586472129303));
#157319=CARTESIAN_POINT('Ctrl Pts',(33.7022946123362,-54.9421531363248,
-71.3149848772055));
#157320=CARTESIAN_POINT('Ctrl Pts',(33.7038813586064,-54.9342138292439,
-71.3453900726014));
#157321=CARTESIAN_POINT('Ctrl Pts',(33.704624367107,-54.9305251002979,-71.3596402001894));
#157322=CARTESIAN_POINT('Ctrl Pts',(33.7050495491287,-54.9284213105411,
-71.3677980732163));
#157323=CARTESIAN_POINT('Ctrl Pts',(33.7052491662678,-54.9274352281448,
-71.371628851342));
#157324=CARTESIAN_POINT('Ctrl Pts',(33.7069422801926,-54.9190764485954,
-71.4041231748996));
#157325=CARTESIAN_POINT('Ctrl Pts',(33.7130531741981,-54.884534886557,-71.5342184997344));
#157326=CARTESIAN_POINT('Ctrl Pts',(33.7307728610088,-54.8097058756137,
-71.8787180674662));
#157327=CARTESIAN_POINT('Ctrl Pts',(33.7381334527421,-54.7811877769103,
-72.0184836933547));
#157328=CARTESIAN_POINT('Ctrl Pts',(33.7513335591963,-54.7374161896249,
-72.2658215103054));
#157329=CARTESIAN_POINT('Ctrl Pts',(33.7560887124468,-54.7226759772122,
-72.354546583101));
#157330=CARTESIAN_POINT('Ctrl Pts',(33.7636849639329,-54.7010223535207,
-72.4970490085014));
#157331=CARTESIAN_POINT('Ctrl Pts',(33.7675980837435,-54.6903110456761,
-72.5706533552747));
#157332=CARTESIAN_POINT('Ctrl Pts',(33.7723387369823,-54.678178773344,-72.660635090891));
#157333=CARTESIAN_POINT('Ctrl Pts',(33.7747487362382,-54.6722248501104,
-72.7066518276824));
#157334=CARTESIAN_POINT('Ctrl Pts',(33.7759631018253,-54.6692786047312,
-72.7299164371522));
#157335=CARTESIAN_POINT('Ctrl Pts',(33.7764854891564,-54.6680227978837,
-72.7399418666397));
#157336=CARTESIAN_POINT('Ctrl Pts',(33.7768341725156,-54.6671871520272,
-72.7466376793895));
#157337=CARTESIAN_POINT('Ctrl Pts',(33.7770694365511,-54.6666255109262,
-72.7511589231412));
#157338=CARTESIAN_POINT('Ctrl Pts',(33.8063811783703,-54.5968113004879,
-73.3147231974228));
#157339=CARTESIAN_POINT('Ctrl Pts',(33.8306904602248,-54.5800000405386,
-73.7828685758946));
#157340=CARTESIAN_POINT('Ctrl Pts',(33.8499999999899,-54.58000002,-74.1550953619836));
#157341=CARTESIAN_POINT('Origin',(57.,-2.42462934179819E-14,-174.34995));
#157342=CARTESIAN_POINT('',(60.,11.11999998,-174.34995));
#157343=CARTESIAN_POINT('',(60.,11.61999998,-174.34995));
#157344=CARTESIAN_POINT('',(60.,28.41999998,-174.34995));
#157345=CARTESIAN_POINT('',(57.,11.11999998,-177.34995));
#157346=CARTESIAN_POINT('Origin',(57.,11.11999998,-174.34995));
#157347=CARTESIAN_POINT('',(57.,11.61999998,-177.34995));
#157348=CARTESIAN_POINT('',(57.,-54.58000002,-177.34995));
#157349=CARTESIAN_POINT('Origin',(57.,11.61999998,-174.34995));
#157350=CARTESIAN_POINT('Origin',(60.,28.41999998,-177.34995));
#157351=CARTESIAN_POINT('',(53.8590042959267,11.11999998,-177.34995));
#157352=CARTESIAN_POINT('',(60.,11.11999998,-177.34995));
#157353=CARTESIAN_POINT('',(53.6325912458891,11.61999998,-177.34995));
#157354=CARTESIAN_POINT('Origin',(0.,-12.9675000200281,-177.34995));
#157355=CARTESIAN_POINT('',(60.,11.61999998,-177.34995));
#157356=CARTESIAN_POINT('Origin',(39.,46.91999998,-129.34995));
#157357=CARTESIAN_POINT('',(39.,4.46999998000001,-135.863383986541));
#157358=CARTESIAN_POINT('',(39.0000000003307,10.11999998,-140.924467062102));
#157359=CARTESIAN_POINT('Ctrl Pts',(39.,4.46999998000001,-135.863383986541));
#157360=CARTESIAN_POINT('Ctrl Pts',(39.0000000000005,4.88328157550195,-136.189917146856));
#157361=CARTESIAN_POINT('Ctrl Pts',(39.0000000000119,5.29116221661631,-136.522117224197));
#157362=CARTESIAN_POINT('Ctrl Pts',(39.0000000000389,5.69434025783604,-136.859675625831));
#157363=CARTESIAN_POINT('Ctrl Pts',(39.0000000000669,6.11191405993836,-137.209286792093));
#157364=CARTESIAN_POINT('Ctrl Pts',(39.0000000001116,6.52444323388668,-137.564646050799));
#157365=CARTESIAN_POINT('Ctrl Pts',(39.0000000001789,6.93266997768885,-137.925456663962));
#157366=CARTESIAN_POINT('Ctrl Pts',(39.0000000002504,7.36643947058691,-138.308843198726));
#157367=CARTESIAN_POINT('Ctrl Pts',(39.0000000003473,7.7953511045625,-138.698384855374));
#157368=CARTESIAN_POINT('Ctrl Pts',(39.0000000004772,8.2202608237891,-139.093772869124));
#157369=CARTESIAN_POINT('Ctrl Pts',(39.0000000004994,8.29309080500349,-139.161542798384));
#157370=CARTESIAN_POINT('Ctrl Pts',(39.0000000005226,8.36580314365992,-139.229484583898));
#157371=CARTESIAN_POINT('Ctrl Pts',(39.0000000005469,8.43840206333325,-139.297596789496));
#157372=CARTESIAN_POINT('Ctrl Pts',(39.0000000006997,8.89608996002628,-139.726998938443));
#157373=CARTESIAN_POINT('Ctrl Pts',(39.0000000008925,9.34761173379244,-140.161633014658));
#157374=CARTESIAN_POINT('Ctrl Pts',(39.0000000011356,9.79388080740657,-140.6013308485));
#157375=CARTESIAN_POINT('Ctrl Pts',(39.0000000011949,9.90289654251582,-140.70874134458));
#157376=CARTESIAN_POINT('Ctrl Pts',(39.0000000012573,10.011598622152,-140.816454152329));
#157377=CARTESIAN_POINT('Ctrl Pts',(39.0000000013228,10.1199999800001,-140.924467062102));
#157378=CARTESIAN_POINT('',(39.0000000003509,10.11999998,-91.1341759094044));
#157379=CARTESIAN_POINT('',(39.,10.11999998,-129.34995));
#157380=CARTESIAN_POINT('',(39.,4.46999998000002,-96.1952589849652));
#157381=CARTESIAN_POINT('Ctrl Pts',(39.0000000014036,10.11999998,-91.1341759094044));
#157382=CARTESIAN_POINT('Ctrl Pts',(39.0000000011199,9.67730365007889,-91.575285870475));
#157383=CARTESIAN_POINT('Ctrl Pts',(39.0000000008904,9.22960685190676,-92.0113795711832));
#157384=CARTESIAN_POINT('Ctrl Pts',(39.0000000007062,8.77598048492635,-92.4423316322574));
#157385=CARTESIAN_POINT('Ctrl Pts',(39.0000000006606,8.66387047835803,-92.5488378715646));
#157386=CARTESIAN_POINT('Ctrl Pts',(39.0000000006178,8.55139809477872,-92.6550299299106));
#157387=CARTESIAN_POINT('Ctrl Pts',(39.0000000005776,8.43854888592038,-92.7609056252127));
#157388=CARTESIAN_POINT('Ctrl Pts',(39.0000000004289,8.02088208266706,-93.1527627205917));
#157389=CARTESIAN_POINT('Ctrl Pts',(39.000000000316,7.59947404051456,-93.5389725674448));
#157390=CARTESIAN_POINT('Ctrl Pts',(39.0000000002313,7.17350510090081,-93.9192513866299));
#157391=CARTESIAN_POINT('Ctrl Pts',(39.0000000001502,6.7660803065941,-94.2829751356576));
#157392=CARTESIAN_POINT('Ctrl Pts',(39.000000000095,6.35448332392143,-94.6412733529686));
#157393=CARTESIAN_POINT('Ctrl Pts',(39.0000000000588,5.93796915862382,-94.9938596181638));
#157394=CARTESIAN_POINT('Ctrl Pts',(39.0000000000244,5.54178994073892,-95.3292320074371));
#157395=CARTESIAN_POINT('Ctrl Pts',(39.0000000000072,5.14116207564722,-95.659436734842));
#157396=CARTESIAN_POINT('Ctrl Pts',(39.0000000000019,4.73541621354422,-95.9841886225431));
#157397=CARTESIAN_POINT('Ctrl Pts',(39.0000000000007,4.64718860206996,-96.0548044588332));
#157398=CARTESIAN_POINT('Ctrl Pts',(39.0000000000001,4.55871888397169,-96.1251623138121));
#157399=CARTESIAN_POINT('Ctrl Pts',(39.,4.46999998000004,-96.1952589849652));
#157400=CARTESIAN_POINT('',(39.,4.46999998000002,-129.34995));
#157401=CARTESIAN_POINT('Ctrl Pts',(40.0658656066501,9.93539045625896,-145.165138021572));
#157402=CARTESIAN_POINT('Ctrl Pts',(39.,10.925678886939,-144.234640983567));
#157403=CARTESIAN_POINT('Ctrl Pts',(39.,12.1842637898263,-143.052046612136));
#157404=CARTESIAN_POINT('Ctrl Pts',(40.0194683031852,8.81214956439894,-143.88333842497));
#157405=CARTESIAN_POINT('Ctrl Pts',(39.,9.77621090664518,-142.950028351532));
#157406=CARTESIAN_POINT('Ctrl Pts',(39.,10.979841755805,-141.770231455688));
#157407=CARTESIAN_POINT('Ctrl Pts',(39.9723350288336,7.65540581054358,-142.626946488088));
#157408=CARTESIAN_POINT('Ctrl Pts',(38.9999999999938,8.58671673912124,-141.687354999621));
#157409=CARTESIAN_POINT('Ctrl Pts',(39.,9.73492905398707,-140.513855077087));
#157410=CARTESIAN_POINT('Ctrl Pts',(39.8778674168776,5.25663147225476,-140.194322050342));
#157411=CARTESIAN_POINT('Ctrl Pts',(39.0000000000061,6.11210395701397,-139.242594421298));
#157412=CARTESIAN_POINT('Ctrl Pts',(39.,7.14197626750154,-138.081230637578));
#157413=CARTESIAN_POINT('Ctrl Pts',(39.8310080868429,4.02695569272985,-139.030438961711));
#157414=CARTESIAN_POINT('Ctrl Pts',(39.,4.84002925713993,-138.072329022275));
#157415=CARTESIAN_POINT('Ctrl Pts',(39.,5.8072721390059,-136.917329731646));
#157416=CARTESIAN_POINT('Ctrl Pts',(39.785612724228,2.75522931487726,-137.937569266631));
#157417=CARTESIAN_POINT('Ctrl Pts',(39.,3.51696507435961,-136.97110396566));
#157418=CARTESIAN_POINT('Ctrl Pts',(39.,4.42069758591766,-135.824477851673));
#157419=CARTESIAN_POINT('',(40.0642139599405,9.89540189006471,-145.119531500823));
#157420=CARTESIAN_POINT('',(39.8417543169614,4.28989009289605,-139.307982736423));
#157421=CARTESIAN_POINT('Ctrl Pts',(40.0642139728404,9.89540198157303,-145.11953138824));
#157422=CARTESIAN_POINT('Ctrl Pts',(40.0490672312073,9.52858910434629,-144.701432431427));
#157423=CARTESIAN_POINT('Ctrl Pts',(40.0340775687819,9.16386888011769,-144.292528978177));
#157424=CARTESIAN_POINT('Ctrl Pts',(40.0192554498771,8.80086505585303,-143.892595037891));
#157425=CARTESIAN_POINT('Ctrl Pts',(40.0026735092318,8.39476199416364,-143.445177168527));
#157426=CARTESIAN_POINT('Ctrl Pts',(39.9863012938639,7.99080764660249,-143.008984945727));
#157427=CARTESIAN_POINT('Ctrl Pts',(39.9701472616296,7.5884884611955,-142.583631867571));
#157428=CARTESIAN_POINT('Ctrl Pts',(39.9549376693659,7.20969072938624,-142.183146911676));
#157429=CARTESIAN_POINT('Ctrl Pts',(39.9399213864914,6.83234320991116,-141.792269106813));
#157430=CARTESIAN_POINT('Ctrl Pts',(39.925101121935,6.45601873886265,-141.410634166036));
#157431=CARTESIAN_POINT('Ctrl Pts',(39.9070625690653,5.9979736856591,-140.946125450285));
#157432=CARTESIAN_POINT('Ctrl Pts',(39.8893840622469,5.54324262799147,-140.497110855627));
#157433=CARTESIAN_POINT('Ctrl Pts',(39.872080343996,5.09074233509129,-140.062917663929));
#157434=CARTESIAN_POINT('Ctrl Pts',(39.8618462222629,4.82311528437996,-139.806118176378));
#157435=CARTESIAN_POINT('Ctrl Pts',(39.8517430061508,4.55626932041237,-139.554502279586));
#157436=CARTESIAN_POINT('Ctrl Pts',(39.8417723415372,4.28998417309766,-139.307926707773));
#157437=CARTESIAN_POINT('Ctrl Pts',(40.0642139578498,9.89540181780599,-145.119531498084));
#157438=CARTESIAN_POINT('Ctrl Pts',(39.9837119096533,9.9031049697781,-144.977776866857));
#157439=CARTESIAN_POINT('Ctrl Pts',(39.9033047333671,9.91139396310649,-144.824952312001));
#157440=CARTESIAN_POINT('Ctrl Pts',(39.7852935726608,9.9248259446457,-144.578638079069));
#157441=CARTESIAN_POINT('Ctrl Pts',(39.7463938137604,9.92946595900602,-144.493689828532));
#157442=CARTESIAN_POINT('Ctrl Pts',(39.6890397168151,9.9366461072912,-144.36197286233));
#157443=CARTESIAN_POINT('Ctrl Pts',(39.6606118595104,9.94029076562729,-144.2950410825));
#157444=CARTESIAN_POINT('Ctrl Pts',(39.6279593144707,9.94462815869065,-144.215073303383));
#157445=CARTESIAN_POINT('Ctrl Pts',(39.6117712025815,9.94681650242244,-144.174619255621));
#157446=CARTESIAN_POINT('Ctrl Pts',(39.6048641034372,9.94775838423618,-144.15718106888));
#157447=CARTESIAN_POINT('Ctrl Pts',(39.6002663026222,9.94838717661874,-144.145533226968));
#157448=CARTESIAN_POINT('Ctrl Pts',(39.5972217602901,9.94880504951511,-144.137787256445));
#157449=CARTESIAN_POINT('Ctrl Pts',(39.5463093096446,9.95580814360903,-144.007917527242));
#157450=CARTESIAN_POINT('Ctrl Pts',(39.4916542170312,9.96362771148659,-143.859230612069));
#157451=CARTESIAN_POINT('Ctrl Pts',(39.4071494540781,9.97745077382445,-143.600799527875));
#157452=CARTESIAN_POINT('Ctrl Pts',(39.3785796317958,9.98240180929145,-143.508758121777));
#157453=CARTESIAN_POINT('Ctrl Pts',(39.3359627083911,9.99033143895586,-143.361740135451));
#157454=CARTESIAN_POINT('Ctrl Pts',(39.314715370758,9.99442093206169,-143.285992920656));
#157455=CARTESIAN_POINT('Ctrl Pts',(39.2902343489268,9.99939423749642,-143.193690016968));
#157456=CARTESIAN_POINT('Ctrl Pts',(39.2780969557419,10.0019282957381,-143.14655487039));
#157457=CARTESIAN_POINT('Ctrl Pts',(39.2720573444652,10.0032067423246,-143.122741292126));
#157458=CARTESIAN_POINT('Ctrl Pts',(39.2694755295604,10.0037570444933,-143.112482751614));
#157459=CARTESIAN_POINT('Ctrl Pts',(39.2677558239374,10.004124439372,-143.105632008287));
#157460=CARTESIAN_POINT('Ctrl Pts',(39.2672057147562,10.0042420820058,-143.103438103034));
#157461=CARTESIAN_POINT('Ctrl Pts',(39.1913299145855,10.0205271473602,-142.799601273041));
#157462=CARTESIAN_POINT('Ctrl Pts',(39.1470186327352,10.0338725753239,-142.55835026003));
#157463=CARTESIAN_POINT('Ctrl Pts',(39.1029770738426,10.0481832824593,-142.288135290547));
#157464=CARTESIAN_POINT('Ctrl Pts',(39.0921521568062,10.0520678385991,-142.213264213691));
#157465=CARTESIAN_POINT('Ctrl Pts',(39.0799075063914,10.0566771044917,-142.123910676051));
#157466=CARTESIAN_POINT('Ctrl Pts',(39.0764992482883,10.0580114078987,-142.097949836939));
#157467=CARTESIAN_POINT('Ctrl Pts',(39.0722428292861,10.0597256940649,-142.064751310274));
#157468=CARTESIAN_POINT('Ctrl Pts',(39.0703293336654,10.0605110264876,-142.049587644647));
#157469=CARTESIAN_POINT('Ctrl Pts',(39.0684465687074,10.0613046863452,-142.034409863244));
#157470=CARTESIAN_POINT('Ctrl Pts',(39.0675898962216,10.0616712186324,-142.027449333261));
#157471=CARTESIAN_POINT('Ctrl Pts',(39.0671824151856,10.0618469512748,-142.024126166792));
#157472=CARTESIAN_POINT('Ctrl Pts',(39.0670122165204,10.0619206551731,-142.022735617363));
#157473=CARTESIAN_POINT('Ctrl Pts',(39.0668997329735,10.0619694337677,-142.021816065555));
#157474=CARTESIAN_POINT('Ctrl Pts',(39.0669853751627,10.0619321550857,-142.022517281932));
#157475=CARTESIAN_POINT('Ctrl Pts',(39.0164452565529,10.0839111803066,-141.608863850399));
#157476=CARTESIAN_POINT('Ctrl Pts',(39.0000054549653,10.1032655307119,-141.242483723391));
#157477=CARTESIAN_POINT('Ctrl Pts',(39.,10.11999998,-140.924467062102));
#157478=CARTESIAN_POINT('Ctrl Pts',(39.,4.46999998000002,-135.863383986541));
#157479=CARTESIAN_POINT('Ctrl Pts',(39.,4.4649048304607,-135.964102536252));
#157480=CARTESIAN_POINT('Ctrl Pts',(39.0019791923666,4.45957150846498,-136.069213666802));
#157481=CARTESIAN_POINT('Ctrl Pts',(39.0065120981555,4.45399949430044,-136.178648033205));
#157482=CARTESIAN_POINT('Ctrl Pts',(39.0102594534973,4.44939310757717,-136.269117475238));
#157483=CARTESIAN_POINT('Ctrl Pts',(39.0157536191668,4.44462331813979,-136.362546776375));
#157484=CARTESIAN_POINT('Ctrl Pts',(39.0233429014063,4.4396914744795,-136.458863808463));
#157485=CARTESIAN_POINT('Ctrl Pts',(39.027137542526,4.43722555264935,-136.507022324508));
#157486=CARTESIAN_POINT('Ctrl Pts',(39.0314562808131,4.43471912489781,-136.555902622014));
#157487=CARTESIAN_POINT('Ctrl Pts',(39.0363440945682,4.43217253088145,-136.605492393808));
#157488=CARTESIAN_POINT('Ctrl Pts',(39.0387880014458,4.43089923387327,-136.630287279704));
#157489=CARTESIAN_POINT('Ctrl Pts',(39.0413741920377,4.4296158957776,-136.655259525851));
#157490=CARTESIAN_POINT('Ctrl Pts',(39.0441083522793,4.42832257012126,-136.680407386378));
#157491=CARTESIAN_POINT('Ctrl Pts',(39.0454754324001,4.42767590729309,-136.692981316641));
#157492=CARTESIAN_POINT('Ctrl Pts',(39.0468795052976,4.42702674778821,-136.705599146449));
#157493=CARTESIAN_POINT('Ctrl Pts',(39.0483212846087,4.42637509905493,-136.718260643517));
#157494=CARTESIAN_POINT('Ctrl Pts',(39.0490421742642,4.42604927468829,-136.724591392051));
#157495=CARTESIAN_POINT('Ctrl Pts',(39.0497724905614,4.42572282801754,-136.730933057349));
#157496=CARTESIAN_POINT('Ctrl Pts',(39.050512322863,4.425395760019,-136.737285609543));
#157497=CARTESIAN_POINT('Ctrl Pts',(39.0506203872579,4.42534798648262,-136.738213501861));
#157498=CARTESIAN_POINT('Ctrl Pts',(39.0507286546797,4.42530019969011,-136.739141626453));
#157499=CARTESIAN_POINT('Ctrl Pts',(39.0508371254071,4.42525239964456,-136.740069983224));
#157500=CARTESIAN_POINT('Ctrl Pts',(39.050905139878,4.42522242755084,-136.740652091375));
#157501=CARTESIAN_POINT('Ctrl Pts',(39.0509725129255,4.42519276704729,-136.741228138368));
#157502=CARTESIAN_POINT('Ctrl Pts',(39.0510428967244,4.42516181331133,-136.741829291024));
#157503=CARTESIAN_POINT('Ctrl Pts',(39.051628747135,4.42490416511385,-136.746833077913));
#157504=CARTESIAN_POINT('Ctrl Pts',(39.0523841686075,4.42457546869017,-136.75321552608));
#157505=CARTESIAN_POINT('Ctrl Pts',(39.0527604572301,4.42441269305049,-136.756375896314));
#157506=CARTESIAN_POINT('Ctrl Pts',(39.0588994248826,4.42175708688442,-136.807935814608));
#157507=CARTESIAN_POINT('Ctrl Pts',(39.0661343773194,4.41885667205721,-136.864171648229));
#157508=CARTESIAN_POINT('Ctrl Pts',(39.0747889848578,4.41571105540969,-136.925046284492));
#157509=CARTESIAN_POINT('Ctrl Pts',(39.0830014682778,4.41272613385796,-136.982811115398));
#157510=CARTESIAN_POINT('Ctrl Pts',(39.0924926835029,4.40952042207355,-137.044752833922));
#157511=CARTESIAN_POINT('Ctrl Pts',(39.1035844904071,4.40609375716194,-137.110831569558));
#157512=CARTESIAN_POINT('Ctrl Pts',(39.1155719987269,4.40239037731665,-137.182246389528));
#157513=CARTESIAN_POINT('Ctrl Pts',(39.1294289734821,4.39842885436704,-137.258494527262));
#157514=CARTESIAN_POINT('Ctrl Pts',(39.1456101803986,4.39421132377648,-137.339475634449));
#157515=CARTESIAN_POINT('Ctrl Pts',(39.1617913873151,4.38999379318591,-137.420456741636));
#157516=CARTESIAN_POINT('Ctrl Pts',(39.180298150752,4.38552005634583,-137.506174477798));
#157517=CARTESIAN_POINT('Ctrl Pts',(39.2016291583746,4.38079442929467,-137.596483472856));
#157518=CARTESIAN_POINT('Ctrl Pts',(39.2042389185241,4.38021626846057,-137.607532403155));
#157519=CARTESIAN_POINT('Ctrl Pts',(39.2066394307158,4.37968903599853,-137.617605342405));
#157520=CARTESIAN_POINT('Ctrl Pts',(39.2095655036944,4.37905318437206,-137.629749427704));
#157521=CARTESIAN_POINT('Ctrl Pts',(39.2096485574449,4.37903513633884,-137.630094125816));
#157522=CARTESIAN_POINT('Ctrl Pts',(39.2097320395475,4.3790170007186,-137.630440493425));
#157523=CARTESIAN_POINT('Ctrl Pts',(39.2098159675572,4.37899877386231,-137.630788600126));
#157524=CARTESIAN_POINT('Ctrl Pts',(39.2281276302169,4.37502198416818,-137.70673955509));
#157525=CARTESIAN_POINT('Ctrl Pts',(39.2466813967273,4.37123554737574,-137.778431463205));
#157526=CARTESIAN_POINT('Ctrl Pts',(39.2651044416888,4.36766070800654,-137.845883960537));
#157527=CARTESIAN_POINT('Ctrl Pts',(39.2840409735794,4.3639862307494,-137.915216493215));
#157528=CARTESIAN_POINT('Ctrl Pts',(39.3028391507201,4.36053526087973,-137.980070624068));
#157529=CARTESIAN_POINT('Ctrl Pts',(39.3211407154263,4.35732730003464,-138.040497223528));
#157530=CARTESIAN_POINT('Ctrl Pts',(39.3323413059184,4.35536402223205,-138.077478410997));
#157531=CARTESIAN_POINT('Ctrl Pts',(39.3433568176487,4.35349169612979,-138.11280181407));
#157532=CARTESIAN_POINT('Ctrl Pts',(39.3541139348103,4.35171428876002,-138.146482817966));
#157533=CARTESIAN_POINT('Ctrl Pts',(39.3720039620678,4.34875830475286,-138.202497275065));
#157534=CARTESIAN_POINT('Ctrl Pts',(39.3891776151373,4.34605561713149,-138.253964698044));
#157535=CARTESIAN_POINT('Ctrl Pts',(39.4053429559131,4.34359270394892,-138.300951862157));
#157536=CARTESIAN_POINT('Ctrl Pts',(39.4097047527134,4.34292815087899,-138.313630126409));
#157537=CARTESIAN_POINT('Ctrl Pts',(39.4139934300582,4.34228105444557,-138.325982248389));
#157538=CARTESIAN_POINT('Ctrl Pts',(39.4182038966227,4.34165114941491,-138.338009611435));
#157539=CARTESIAN_POINT('Ctrl Pts',(39.4281113763137,4.34016894519766,-138.366310716144));
#157540=CARTESIAN_POINT('Ctrl Pts',(39.4375853042781,4.33878145855264,-138.392813478883));
#157541=CARTESIAN_POINT('Ctrl Pts',(39.4465655554463,4.33748325874983,-138.417535049933));
#157542=CARTESIAN_POINT('Ctrl Pts',(39.4510556810304,4.33683415884842,-138.429895835458));
#157543=CARTESIAN_POINT('Ctrl Pts',(39.4554224959828,4.33620741251945,-138.441811284974));
#157544=CARTESIAN_POINT('Ctrl Pts',(39.4596592959402,4.33560223077118,-138.453283494151));
#157545=CARTESIAN_POINT('Ctrl Pts',(39.4617776959189,4.33529963989704,-138.45901959874));
#157546=CARTESIAN_POINT('Ctrl Pts',(39.4638635991141,4.33500244217455,-138.464644890844));
#157547=CARTESIAN_POINT('Ctrl Pts',(39.4659162115836,4.33471054561932,-138.470159619889));
#157548=CARTESIAN_POINT('Ctrl Pts',(39.4669425178184,4.3345645973417,-138.472916984412));
#157549=CARTESIAN_POINT('Ctrl Pts',(39.4679605018047,4.33441997448555,-138.475646708015));
#157550=CARTESIAN_POINT('Ctrl Pts',(39.4689700673648,4.33427666540267,-138.478348821464));
#157551=CARTESIAN_POINT('Ctrl Pts',(39.4694748501449,4.33420501086123,-138.479699878188));
#157552=CARTESIAN_POINT('Ctrl Pts',(39.4699775283455,4.33413368477126,-138.481044032364));
#157553=CARTESIAN_POINT('Ctrl Pts',(39.4704780901355,4.33406268566851,-138.482381287809));
#157554=CARTESIAN_POINT('Ctrl Pts',(39.4709786519255,4.33399168656576,-138.483718543254));
#157555=CARTESIAN_POINT('Ctrl Pts',(39.4710360424286,4.33398352830646,-138.483872798879));
#157556=CARTESIAN_POINT('Ctrl Pts',(39.4719734145588,4.33385066787384,-138.486372361736));
#157557=CARTESIAN_POINT('Ctrl Pts',(39.5076868319688,4.32878875069687,-138.581604477941));
#157558=CARTESIAN_POINT('Ctrl Pts',(39.5441541767506,4.3239356277841,-138.67269332793));
#157559=CARTESIAN_POINT('Ctrl Pts',(39.580948614012,4.31929192751637,-138.759679041817));
#157560=CARTESIAN_POINT('Ctrl Pts',(39.6188258809332,4.31451156701532,-138.849224672855));
#157561=CARTESIAN_POINT('Ctrl Pts',(39.65704958739,4.30995310473825,-138.934422681979));
#157562=CARTESIAN_POINT('Ctrl Pts',(39.6951901830099,4.30561446676912,-139.01535983076));
#157563=CARTESIAN_POINT('Ctrl Pts',(39.7348091235138,4.30110766144076,-139.099434136102));
#157564=CARTESIAN_POINT('Ctrl Pts',(39.7743381098534,4.29683801816509,-139.17891148334));
#157565=CARTESIAN_POINT('Ctrl Pts',(39.8133377650709,4.29280078440236,-139.253925691597));
#157566=CARTESIAN_POINT('Ctrl Pts',(39.8228431850076,4.29181678590074,-139.272208969916));
#157567=CARTESIAN_POINT('Ctrl Pts',(39.8323173603756,4.29084658406392,-139.290227256414));
#157568=CARTESIAN_POINT('Ctrl Pts',(39.8417543169614,4.28989009289605,-139.307982736423));
#157569=CARTESIAN_POINT('Origin',(0.,-12.9675000200281,-171.64995));
#157570=CARTESIAN_POINT('',(55.7843555297028,4.33575017898885,-171.449026400902));
#157571=CARTESIAN_POINT('',(53.7255998841352,9.94225131873297,-171.449026400902));
#157572=CARTESIAN_POINT('Origin',(0.,-12.9675000200281,-171.449026400902));
#157573=CARTESIAN_POINT('Ctrl Pts',(53.7255998841352,9.94225131873298,-171.449026400902));
#157574=CARTESIAN_POINT('Ctrl Pts',(53.0048383941293,9.94024676411936,-170.025533543412));
#157575=CARTESIAN_POINT('Ctrl Pts',(52.294948227473,9.93824451327994,-168.627760176666));
#157576=CARTESIAN_POINT('Ctrl Pts',(51.5958827203954,9.9362037934586,-167.255727365281));
#157577=CARTESIAN_POINT('Ctrl Pts',(51.1460015352648,9.93489049528776,-166.372760402993));
#157578=CARTESIAN_POINT('Ctrl Pts',(50.7006043959427,9.93356129347437,-165.50045341864));
#157579=CARTESIAN_POINT('Ctrl Pts',(50.2596888381369,9.93220562599593,-164.638806639518));
#157580=CARTESIAN_POINT('Ctrl Pts',(49.6966641013534,9.93047451374166,-163.53853144526));
#157581=CARTESIAN_POINT('Ctrl Pts',(49.1409444411495,9.92870584879501,-162.455639719489));
#157582=CARTESIAN_POINT('Ctrl Pts',(48.5925279246073,9.92691158097371,-161.390127665526));
#157583=CARTESIAN_POINT('Ctrl Pts',(48.3183196663362,9.92601444706306,-160.857371638545));
#157584=CARTESIAN_POINT('Ctrl Pts',(48.0459373244593,9.92511126710263,-160.328960426286));
#157585=CARTESIAN_POINT('Ctrl Pts',(47.7753813036175,9.92420565463034,-159.804892982715));
#157586=CARTESIAN_POINT('Ctrl Pts',(47.6401032931966,9.9237528483942,-159.542859260929));
#157587=CARTESIAN_POINT('Ctrl Pts',(47.5052818754017,9.92329944091239,-159.281911474732));
#157588=CARTESIAN_POINT('Ctrl Pts',(47.3709171228666,9.92284603234586,-159.022049462581));
#157589=CARTESIAN_POINT('Ctrl Pts',(47.3037347465991,9.92261932806259,-158.892118456506));
#157590=CARTESIAN_POINT('Ctrl Pts',(47.236666537344,9.9223926239238,-158.762458893565));
#157591=CARTESIAN_POINT('Ctrl Pts',(47.1697125068932,9.92216600042275,-158.6330707515));
#157592=CARTESIAN_POINT('Ctrl Pts',(47.1069431033455,9.92195354089051,-158.511769368315));
#157593=CARTESIAN_POINT('Ctrl Pts',(47.0442740522902,9.92174115224678,-158.39070653862));
#157594=CARTESIAN_POINT('Ctrl Pts',(46.9817053643811,9.92152890466437,-158.269882243086));
#157595=CARTESIAN_POINT('Ctrl Pts',(46.9775341185205,9.92151475482554,-158.26182729005));
#157596=CARTESIAN_POINT('Ctrl Pts',(46.9739449851603,9.92150257901683,-158.25489657829));
#157597=CARTESIAN_POINT('Ctrl Pts',(46.969192963075,9.92148646200742,-158.245720565411));
#157598=CARTESIAN_POINT('Ctrl Pts',(46.9690340241742,9.92148592294852,-158.245413659135));
#157599=CARTESIAN_POINT('Ctrl Pts',(46.9688750858378,9.9214853838877,-158.245106754236));
#157600=CARTESIAN_POINT('Ctrl Pts',(46.9687161480657,9.92148484482495,-158.244799850712));
#157601=CARTESIAN_POINT('Ctrl Pts',(46.3446685940074,9.91936828820202,-157.039784889644));
#157602=CARTESIAN_POINT('Ctrl Pts',(45.7293385706448,9.91722214649627,-155.855973727983));
#157603=CARTESIAN_POINT('Ctrl Pts',(45.1226444261086,9.91504615189965,-154.693400464412));
#157604=CARTESIAN_POINT('Ctrl Pts',(44.5040721429633,9.91282755467424,-153.508065803699));
#157605=CARTESIAN_POINT('Ctrl Pts',(43.8944773759627,9.91057792895297,-152.344808699876));
#157606=CARTESIAN_POINT('Ctrl Pts',(43.2938225298004,9.90829822225579,-151.203638927001));
#157607=CARTESIAN_POINT('Ctrl Pts',(42.6723312127876,9.90593943346604,-150.022882441624));
#157608=CARTESIAN_POINT('Ctrl Pts',(42.0604109072536,9.90354844326633,-148.865772219977));
#157609=CARTESIAN_POINT('Ctrl Pts',(41.4580700145246,9.90112755266097,-147.732292127205));
#157610=CARTESIAN_POINT('Ctrl Pts',(40.9875983364426,9.89923666250341,-146.8469624281));
#157611=CARTESIAN_POINT('Ctrl Pts',(40.5229718710177,9.89732755761719,-145.976048274262));
#157612=CARTESIAN_POINT('Ctrl Pts',(40.064213984323,9.8954018152728,-145.1195315447));
#157613=CARTESIAN_POINT('Ctrl Pts',(39.8417798628559,4.28988750369336,-139.308030800137));
#157614=CARTESIAN_POINT('Ctrl Pts',(40.4868859579449,4.29232172358473,-140.57956955374));
#157615=CARTESIAN_POINT('Ctrl Pts',(41.1456653359953,4.2947194009918,-141.882651683976));
#157616=CARTESIAN_POINT('Ctrl Pts',(41.8180607265059,4.29707616997945,-143.217318051408));
#157617=CARTESIAN_POINT('Ctrl Pts',(42.4709012105623,4.29936439834689,-144.5131690487));
#157618=CARTESIAN_POINT('Ctrl Pts',(43.1365771358385,4.30161405421269,-145.838794161371));
#157619=CARTESIAN_POINT('Ctrl Pts',(43.8150777647377,4.30382299667252,-147.194208617093));
#157620=CARTESIAN_POINT('Ctrl Pts',(44.4699896786601,4.30595514316214,-148.502500809534));
#157621=CARTESIAN_POINT('Ctrl Pts',(45.136849288454,4.30804935037138,-149.838545750742));
#157622=CARTESIAN_POINT('Ctrl Pts',(45.8156861354303,4.31010554107007,-151.202330462395));
#157623=CARTESIAN_POINT('Ctrl Pts',(46.4845297539595,4.31213146236976,-152.546038756222));
#157624=CARTESIAN_POINT('Ctrl Pts',(47.1650003076918,4.3141204676528,-153.916676154632));
#157625=CARTESIAN_POINT('Ctrl Pts',(47.8571688879798,4.31607443802584,-155.314205466087));
#157626=CARTESIAN_POINT('Ctrl Pts',(47.8626439628392,4.31608989399187,-155.325259966127));
#157627=CARTESIAN_POINT('Ctrl Pts',(47.8688897641185,4.31610752027897,-155.337870868679));
#157628=CARTESIAN_POINT('Ctrl Pts',(47.8736561032779,4.31612096323088,-155.347494742445));
#157629=CARTESIAN_POINT('Ctrl Pts',(47.8737827560485,4.31612132044153,-155.347750471263));
#157630=CARTESIAN_POINT('Ctrl Pts',(47.8739083642008,4.31612167469916,-155.348004090965));
#157631=CARTESIAN_POINT('Ctrl Pts',(47.8740328855181,4.31612202588467,-155.348255516304));
#157632=CARTESIAN_POINT('Ctrl Pts',(48.6583351081591,4.31833398113315,-156.931867517586));
#157633=CARTESIAN_POINT('Ctrl Pts',(49.4602813144816,4.32050804470002,-158.555378883432));
#157634=CARTESIAN_POINT('Ctrl Pts',(50.2798261127653,4.32264044202089,-160.218817015509));
#157635=CARTESIAN_POINT('Ctrl Pts',(51.0778218667667,4.32471677026001,-161.838516840608));
#157636=CARTESIAN_POINT('Ctrl Pts',(51.8925026843305,4.32675358286625,-163.496071488855));
#157637=CARTESIAN_POINT('Ctrl Pts',(52.7238700838759,4.32874953207866,-165.191483761551));
#157638=CARTESIAN_POINT('Ctrl Pts',(53.5277706787544,4.33067953890847,-166.83088282306));
#157639=CARTESIAN_POINT('Ctrl Pts',(54.3472733569927,4.33257133103891,-168.505679408003));
#157640=CARTESIAN_POINT('Ctrl Pts',(55.1824230680481,4.33442584374162,-170.215853479615));
#157641=CARTESIAN_POINT('Ctrl Pts',(55.3821715796289,4.33486940032455,-170.624887597482));
#157642=CARTESIAN_POINT('Ctrl Pts',(55.582815395474,4.33531083454817,-171.035945398186));
#157643=CARTESIAN_POINT('Ctrl Pts',(55.7843555297028,4.33575017898885,-171.449026400902));
#157644=CARTESIAN_POINT('Origin',(60.,28.41999998,-177.34995));
#157645=CARTESIAN_POINT('',(57.,2.96999998000001,-177.34995));
#157646=CARTESIAN_POINT('',(56.8066553649227,2.96999998000001,-177.34995));
#157647=CARTESIAN_POINT('',(60.,2.96999998000001,-177.34995));
#157648=CARTESIAN_POINT('',(56.6639973329545,3.46999998000001,-177.34995));
#157649=CARTESIAN_POINT('Origin',(0.,-12.9675000200281,-177.34995));
#157650=CARTESIAN_POINT('',(57.,3.46999998000002,-177.34995));
#157651=CARTESIAN_POINT('',(60.,3.46999998000001,-177.34995));
#157652=CARTESIAN_POINT('',(57.,-54.58000002,-177.34995));
#157653=CARTESIAN_POINT('Origin',(60.,-2.55003103885676E-14,0.));
#157654=CARTESIAN_POINT('',(60.,3.46999998000001,-58.24995));
#157655=CARTESIAN_POINT('',(60.,2.96999998000001,-58.24995));
#157656=CARTESIAN_POINT('',(60.,-54.58000002,-58.24995));
#157657=CARTESIAN_POINT('',(60.,2.96999998000001,-174.34995));
#157658=CARTESIAN_POINT('',(60.,2.96999998000001,-174.34995));
#157659=CARTESIAN_POINT('',(60.,3.46999998000001,-174.34995));
#157660=CARTESIAN_POINT('',(60.,28.41999998,-174.34995));
#157661=CARTESIAN_POINT('',(60.,3.46999998000001,-58.24995));
#157662=CARTESIAN_POINT('Origin',(57.,-2.42462934179819E-14,-174.34995));
#157663=CARTESIAN_POINT('Origin',(57.,2.96999998000001,-174.34995));
#157664=CARTESIAN_POINT('Origin',(57.,3.46999998000001,-174.34995));
#157665=CARTESIAN_POINT('Origin',(-83.2809572255632,2.96999998000007,-176.84995));
#157666=CARTESIAN_POINT('',(57.,2.61702308584989,-177.204078948543));
#157667=CARTESIAN_POINT('Origin',(57.,2.96999998000001,-176.84995));
#157668=CARTESIAN_POINT('Ctrl Pts',(57.,2.61702308584994,-177.204078948543));
#157669=CARTESIAN_POINT('Ctrl Pts',(56.9920596731222,2.63188036382227,-177.218887892731));
#157670=CARTESIAN_POINT('Ctrl Pts',(56.9834056339598,2.64801985224532,-177.233109037942));
#157671=CARTESIAN_POINT('Ctrl Pts',(56.9740378825128,2.66543214066919,-177.246483014067));
#157672=CARTESIAN_POINT('Ctrl Pts',(56.9691180761738,2.67457682041948,-177.253506831137));
#157673=CARTESIAN_POINT('Ctrl Pts',(56.9640014139196,2.68407181613746,-177.260296610627));
#157674=CARTESIAN_POINT('Ctrl Pts',(56.9586878957502,2.69391033186455,-177.266812694652));
#157675=CARTESIAN_POINT('Ctrl Pts',(56.9548301627084,2.70105331434672,-177.271543517403));
#157676=CARTESIAN_POINT('Ctrl Pts',(56.9508686652447,2.70837729051018,-177.276130042922));
#157677=CARTESIAN_POINT('Ctrl Pts',(56.9468034033591,2.71587828894132,-177.280556741858));
#157678=CARTESIAN_POINT('Ctrl Pts',(56.9445388538477,2.72005671158906,-177.283022629467));
#157679=CARTESIAN_POINT('Ctrl Pts',(56.942637304404,2.7235662490483,-177.285018059377));
#157680=CARTESIAN_POINT('Ctrl Pts',(56.9408724773909,2.72681209002593,-177.286824867863));
#157681=CARTESIAN_POINT('Ctrl Pts',(56.9394691316813,2.72939310050244,-177.288261596175));
#157682=CARTESIAN_POINT('Ctrl Pts',(56.9381522359377,2.73180827092145,-177.289577706413));
#157683=CARTESIAN_POINT('Ctrl Pts',(56.9368080197773,2.73427291767105,-177.290895293756));
#157684=CARTESIAN_POINT('Ctrl Pts',(56.9307386543405,2.74540121848779,-177.296844425536));
#157685=CARTESIAN_POINT('Ctrl Pts',(56.9241477932597,2.75741692047087,-177.302727797935));
#157686=CARTESIAN_POINT('Ctrl Pts',(56.9170354365348,2.7703598532817,-177.308364462909));
#157687=CARTESIAN_POINT('Ctrl Pts',(56.9095156481655,2.78404422252536,-177.314324024465));
#157688=CARTESIAN_POINT('Ctrl Pts',(56.9014129050262,2.79876611353917,-177.320008025187));
#157689=CARTESIAN_POINT('Ctrl Pts',(56.8927272071169,2.81454408608465,-177.325169386228));
#157690=CARTESIAN_POINT('Ctrl Pts',(56.8843005955034,2.82985141637389,-177.330176788667));
#157691=CARTESIAN_POINT('Ctrl Pts',(56.8753252884202,2.84615339254148,-177.334691867768));
#157692=CARTESIAN_POINT('Ctrl Pts',(56.8658012858673,2.8634291514813,-177.338460653424));
#157693=CARTESIAN_POINT('Ctrl Pts',(56.8567116437613,2.87991701622107,-177.342057556365));
#157694=CARTESIAN_POINT('Ctrl Pts',(56.8471222135273,2.89729223915623,-177.344974141857));
#157695=CARTESIAN_POINT('Ctrl Pts',(56.8370329951653,2.91549476483612,-177.346970302925));
#157696=CARTESIAN_POINT('Ctrl Pts',(56.8273659549057,2.93293561528255,-177.34888293567));
#157697=CARTESIAN_POINT('Ctrl Pts',(56.8172400781582,2.95113622605794,-177.34995));
#157698=CARTESIAN_POINT('Ctrl Pts',(56.8066553649227,2.96999998000001,-177.34995));
#157699=CARTESIAN_POINT('Origin',(39.,46.91999998,-129.34995));
#157700=CARTESIAN_POINT('',(39.0000000012314,1.96999998000004,-98.0457798926543));
#157701=CARTESIAN_POINT('',(39.,-3.68000001999999,-101.255910620448));
#157702=CARTESIAN_POINT('Ctrl Pts',(39.0000000024628,1.96999998000006,-98.0457798926544));
#157703=CARTESIAN_POINT('Ctrl Pts',(39.0000000032442,1.50691588071896,-98.3650262521902));
#157704=CARTESIAN_POINT('Ctrl Pts',(39.0000000016551,1.03814546724657,-98.6748799794054));
#157705=CARTESIAN_POINT('Ctrl Pts',(39.0000000008071,0.562698589411684,
-98.9745405549561));
#157706=CARTESIAN_POINT('Ctrl Pts',(39.0000000004711,0.374284444249737,
-99.0932926044768));
#157707=CARTESIAN_POINT('Ctrl Pts',(39.0000000002453,0.184822272624995,
-99.2104442275613));
#157708=CARTESIAN_POINT('Ctrl Pts',(39.0000000001311,-0.00574774121676395,
-99.3259468990426));
#157709=CARTESIAN_POINT('Ctrl Pts',(38.9999999999777,-0.261894757938799,
-99.4811951677863));
#157710=CARTESIAN_POINT('Ctrl Pts',(39.,-0.520415976845901,-99.6335997492721));
#157711=CARTESIAN_POINT('Ctrl Pts',(39.,-0.780592906922143,-99.7825242060483));
#157712=CARTESIAN_POINT('Ctrl Pts',(39.,-1.12946683952905,-99.9822185482085));
#157713=CARTESIAN_POINT('Ctrl Pts',(39.,-1.48228932648713,-100.176247523887));
#157714=CARTESIAN_POINT('Ctrl Pts',(39.,-1.83764512720228,-100.363126009317));
#157715=CARTESIAN_POINT('Ctrl Pts',(39.0000000000001,-2.17904755464558,
-100.542666538652));
#157716=CARTESIAN_POINT('Ctrl Pts',(39.0000000000001,-2.52330369641992,
-100.715959269876));
#157717=CARTESIAN_POINT('Ctrl Pts',(39.0000000000001,-2.87085998622341,
-100.88265759943));
#157718=CARTESIAN_POINT('Ctrl Pts',(39.0000000000001,-3.13854475841823,
-101.011047174532));
#157719=CARTESIAN_POINT('Ctrl Pts',(39.,-3.40818747901783,-101.135524193408));
#157720=CARTESIAN_POINT('Ctrl Pts',(39.,-3.68000001999998,-101.255910620448));
#157721=CARTESIAN_POINT('',(39.,-3.68000001999998,-130.802732351058));
#157722=CARTESIAN_POINT('',(39.,-3.68000001999999,-129.34995));
#157723=CARTESIAN_POINT('',(39.0000000004655,1.96999998000006,-134.012863078852));
#157724=CARTESIAN_POINT('Ctrl Pts',(39.,-3.68000001999998,-130.802732351058));
#157725=CARTESIAN_POINT('Ctrl Pts',(39.,-3.3350976938153,-130.955490419457));
#157726=CARTESIAN_POINT('Ctrl Pts',(38.999999999995,-2.99379560771499,-131.114791966817));
#157727=CARTESIAN_POINT('Ctrl Pts',(39.0000000000322,-2.6556253235799,-131.280281718424));
#157728=CARTESIAN_POINT('Ctrl Pts',(39.0000000000621,-2.38378986674403,
-131.413309321204));
#157729=CARTESIAN_POINT('Ctrl Pts',(39.0000000001226,-2.1139785184933,-131.550336634986));
#157730=CARTESIAN_POINT('Ctrl Pts',(39.0000000002374,-1.84595706992345,
-131.691201637143));
#157731=CARTESIAN_POINT('Ctrl Pts',(39.0000000003908,-1.48773653906918,
-131.879472897226));
#157732=CARTESIAN_POINT('Ctrl Pts',(39.0000000006483,-1.13214453284304,
-132.074954501691));
#157733=CARTESIAN_POINT('Ctrl Pts',(39.0000000009742,-0.779903543906046,
-132.276609948051));
#157734=CARTESIAN_POINT('Ctrl Pts',(39.0000000012103,-0.524689202150759,
-132.422718332994));
#157735=CARTESIAN_POINT('Ctrl Pts',(39.000000001479,-0.271234086134657,
-132.572069210975));
#157736=CARTESIAN_POINT('Ctrl Pts',(39.0000000017246,-0.0198207958907458,
-132.724283330851));
#157737=CARTESIAN_POINT('Ctrl Pts',(39.0000000020985,0.362997438679328,
-132.956054453973));
#157738=CARTESIAN_POINT('Ctrl Pts',(39.0000000024107,0.740951650741639,
-133.194233184148));
#157739=CARTESIAN_POINT('Ctrl Pts',(39.0000000024159,1.11485984244673,-133.43860998629));
#157740=CARTESIAN_POINT('Ctrl Pts',(39.00000000242,1.40217712996228,-133.626393194792));
#157741=CARTESIAN_POINT('Ctrl Pts',(39.0000000022332,1.68710447741349,-133.817837252074));
#157742=CARTESIAN_POINT('Ctrl Pts',(39.0000000018622,1.96999998000005,-134.012863078852));
#157743=CARTESIAN_POINT('',(39.,1.96999998000002,-129.34995));
#157744=CARTESIAN_POINT('Ctrl Pts',(39.,-3.72521479271581,-130.782753296221));
#157745=CARTESIAN_POINT('Ctrl Pts',(39.,-4.21888391538426,-131.902596984872));
#157746=CARTESIAN_POINT('Ctrl Pts',(39.5652399075022,-4.65674474020595,
-132.895844604925));
#157747=CARTESIAN_POINT('Ctrl Pts',(39.,-3.08946624372919,-131.063015115075));
#157748=CARTESIAN_POINT('Ctrl Pts',(38.9999999999904,-3.61592060950642,
-132.184581657476));
#157749=CARTESIAN_POINT('Ctrl Pts',(39.5781306671204,-4.08236536173137,
-133.176106520795));
#157750=CARTESIAN_POINT('Ctrl Pts',(39.,-2.46339239509573,-131.366669530497));
#157751=CARTESIAN_POINT('Ctrl Pts',(39.,-3.02226593965722,-132.489948109969));
#157752=CARTESIAN_POINT('Ctrl Pts',(39.5919846958087,-3.51592220196165,
-133.479760839166));
#157753=CARTESIAN_POINT('Ctrl Pts',(39.,-1.22847641296741,-132.015647483627));
#157754=CARTESIAN_POINT('Ctrl Pts',(39.,-1.85088554063804,-133.142434340475));
#157755=CARTESIAN_POINT('Ctrl Pts',(39.6212800791283,-2.39690688691799,
-134.128738792364));
#157756=CARTESIAN_POINT('Ctrl Pts',(39.,-0.61794440595705,-132.362031531162));
#157757=CARTESIAN_POINT('Ctrl Pts',(39.,-1.27148303561927,-133.490738119779));
#157758=CARTESIAN_POINT('Ctrl Pts',(39.6367679612577,-1.84279784212966,
-134.475122839821));
#157759=CARTESIAN_POINT('Ctrl Pts',(39.,1.17663045280609,-133.448449910404));
#157760=CARTESIAN_POINT('Ctrl Pts',(39.,0.433753695599258,-134.583900592971));
#157761=CARTESIAN_POINT('Ctrl Pts',(39.6847850431059,-0.21139821211329,
-135.561541219197));
#157762=CARTESIAN_POINT('Ctrl Pts',(39.,2.32236925604725,-134.233515370373));
#157763=CARTESIAN_POINT('Ctrl Pts',(39.,1.52263602949357,-135.373451527488));
#157764=CARTESIAN_POINT('Ctrl Pts',(39.7187663759592,0.83378959624966,-136.346621542847));
#157765=CARTESIAN_POINT('Ctrl Pts',(39.,3.43069435955708,-135.063549838392));
#157766=CARTESIAN_POINT('Ctrl Pts',(39.,2.57493359537216,-136.206226648817));
#157767=CARTESIAN_POINT('Ctrl Pts',(39.7537665531305,1.84818159949203,-137.176641147095));
#157768=CARTESIAN_POINT('',(39.7525218945665,1.81208317188674,-137.147133694481));
#157769=CARTESIAN_POINT('',(39.585730149821,-3.78242344375788,-133.343410042124));
#157770=CARTESIAN_POINT('Ctrl Pts',(39.7525219099498,1.81208323948034,-137.14713352867));
#157771=CARTESIAN_POINT('Ctrl Pts',(39.7388044572068,1.41395416292999,-136.822020786323));
#157772=CARTESIAN_POINT('Ctrl Pts',(39.7254997729288,1.01842473737008,-136.509864953903));
#157773=CARTESIAN_POINT('Ctrl Pts',(39.712614901004,0.624517733625811,-136.210149947402));
#157774=CARTESIAN_POINT('Ctrl Pts',(39.693784203698,0.0488392482247798,
-135.772129096404));
#157775=CARTESIAN_POINT('Ctrl Pts',(39.6758506543709,-0.523370028522445,
-135.360673152285));
#157776=CARTESIAN_POINT('Ctrl Pts',(39.6588130338047,-1.09508430367974,
-134.974099746561));
#157777=CARTESIAN_POINT('Ctrl Pts',(39.6567872693803,-1.16306084036945,
-134.928136365132));
#157778=CARTESIAN_POINT('Ctrl Pts',(39.6547741490203,-1.23103038514879,
-134.882524801265));
#157779=CARTESIAN_POINT('Ctrl Pts',(39.6527736552071,-1.29899796545754,
-134.837262299613));
#157780=CARTESIAN_POINT('Ctrl Pts',(39.6459517210492,-1.53077591681986,
-134.682911506796));
#157781=CARTESIAN_POINT('Ctrl Pts',(39.6392813566793,-1.76247360775619,
-134.53272279422));
#157782=CARTESIAN_POINT('Ctrl Pts',(39.6327764980427,-1.99382554704971,
-134.386891929138));
#157783=CARTESIAN_POINT('Ctrl Pts',(39.6258782044137,-2.23917040356775,
-134.23224073936));
#157784=CARTESIAN_POINT('Ctrl Pts',(39.619166022538,-2.48412652209771,-134.082490044296));
#157785=CARTESIAN_POINT('Ctrl Pts',(39.6126548834015,-2.72843126504667,
-133.937850299462));
#157786=CARTESIAN_POINT('Ctrl Pts',(39.6106277671319,-2.80449078532386,
-133.892819533902));
#157787=CARTESIAN_POINT('Ctrl Pts',(39.6086201268254,-2.88048753715528,
-133.848284024339));
#157788=CARTESIAN_POINT('Ctrl Pts',(39.6066323874685,-2.95641454443982,
-133.804249815765));
#157789=CARTESIAN_POINT('Ctrl Pts',(39.5994131121229,-3.23217402459558,
-133.644321867863));
#157790=CARTESIAN_POINT('Ctrl Pts',(39.5924450145065,-3.50738674925618,
-133.490746661292));
#157791=CARTESIAN_POINT('Ctrl Pts',(39.5857305518838,-3.78242124043357,
-133.343407072386));
#157792=CARTESIAN_POINT('Ctrl Pts',(39.7525218896124,1.81208307130645,-137.147133691772));
#157793=CARTESIAN_POINT('Ctrl Pts',(39.7139087968672,1.81599661082028,-137.07244305817));
#157794=CARTESIAN_POINT('Ctrl Pts',(39.6744474421853,1.82016969113522,-136.992602940359));
#157795=CARTESIAN_POINT('Ctrl Pts',(39.634725153328,1.82460721687045,-136.907430510093));
#157796=CARTESIAN_POINT('Ctrl Pts',(39.6193838930589,1.82632104654174,-136.874535819026));
#157797=CARTESIAN_POINT('Ctrl Pts',(39.6040042538397,1.82807431955759,-136.840845596339));
#157798=CARTESIAN_POINT('Ctrl Pts',(39.5886220325896,1.82986730990165,-136.806348725811));
#157799=CARTESIAN_POINT('Ctrl Pts',(39.5610167425994,1.83308505183843,-136.744439844176));
#157800=CARTESIAN_POINT('Ctrl Pts',(39.5334042639744,1.8364305250442,-136.679936254232));
#157801=CARTESIAN_POINT('Ctrl Pts',(39.5060076808651,1.839904013326,-136.612794432445));
#157802=CARTESIAN_POINT('Ctrl Pts',(39.4923093893105,1.8416407574669,-136.579223521551));
#157803=CARTESIAN_POINT('Ctrl Pts',(39.4786652963206,1.84340948973778,-136.544993284572));
#157804=CARTESIAN_POINT('Ctrl Pts',(39.4651044746358,1.84521014365973,-136.510099833943));
#157805=CARTESIAN_POINT('Ctrl Pts',(39.4583240637933,1.8461104706207,-136.492653108628));
#157806=CARTESIAN_POINT('Ctrl Pts',(39.4515644747565,1.84701877781338,-136.475040579033));
#157807=CARTESIAN_POINT('Ctrl Pts',(39.4448294099773,1.84793504887911,-136.457261889256));
#157808=CARTESIAN_POINT('Ctrl Pts',(39.4414618775878,1.84839318441198,-136.448372544368));
#157809=CARTESIAN_POINT('Ctrl Pts',(39.4381004763634,1.84885331090119,-136.439441659398));
#157810=CARTESIAN_POINT('Ctrl Pts',(39.4347456711397,1.84931542601312,-136.430469193862));
#157811=CARTESIAN_POINT('Ctrl Pts',(39.4330682685279,1.84954648356909,-136.425982961093));
#157812=CARTESIAN_POINT('Ctrl Pts',(39.4313925149198,1.84977803827995,-136.421486333182));
#157813=CARTESIAN_POINT('Ctrl Pts',(39.4297184686102,1.85001008982501,-136.41697930553));
#157814=CARTESIAN_POINT('Ctrl Pts',(39.4288814454554,1.85012611559753,-136.414725791704));
#157815=CARTESIAN_POINT('Ctrl Pts',(39.4280448491253,1.85024226557856,-136.412469677942));
#157816=CARTESIAN_POINT('Ctrl Pts',(39.4272086869189,1.85035853972607,-136.410210963702));
#157817=CARTESIAN_POINT('Ctrl Pts',(39.4263725247124,1.85047481387359,-136.407952249462));
#157818=CARTESIAN_POINT('Ctrl Pts',(39.424817695823,1.85069152670635,-136.403741922849));
#157819=CARTESIAN_POINT('Ctrl Pts',(39.4247015099726,1.8507077346254,-136.403427019011));
#157820=CARTESIAN_POINT('Ctrl Pts',(39.422629125099,1.85099683218914,-136.397810139249));
#157821=CARTESIAN_POINT('Ctrl Pts',(39.4190350978131,1.85149872607394,-136.388058312145));
#157822=CARTESIAN_POINT('Ctrl Pts',(39.4139781513362,1.85221396905478,-136.374151811247));
#157823=CARTESIAN_POINT('Ctrl Pts',(39.4089011553785,1.85293204778847,-136.360190174681));
#157824=CARTESIAN_POINT('Ctrl Pts',(39.4023496341151,1.85386517241038,-136.342040848675));
#157825=CARTESIAN_POINT('Ctrl Pts',(39.3944335185994,1.85501428022268,-136.319668562829));
#157826=CARTESIAN_POINT('Ctrl Pts',(39.3864697665656,1.85617030297894,-136.2971616481));
#157827=CARTESIAN_POINT('Ctrl Pts',(39.3771249826558,1.85754491903973,-136.270380783999));
#157828=CARTESIAN_POINT('Ctrl Pts',(39.3665617445024,1.85913943038351,-136.239274722874));
#157829=CARTESIAN_POINT('Ctrl Pts',(39.3565727512439,1.86064725997442,-136.209859667532));
#157830=CARTESIAN_POINT('Ctrl Pts',(39.3454941464808,1.86235181612195,-136.176575105897));
#157831=CARTESIAN_POINT('Ctrl Pts',(39.3335058501688,1.86425413539818,-136.139371406299));
#157832=CARTESIAN_POINT('Ctrl Pts',(39.3205136229093,1.86631575981201,-136.099052172649));
#157833=CARTESIAN_POINT('Ctrl Pts',(39.3064535772128,1.86860950825767,-136.054132995381));
#157834=CARTESIAN_POINT('Ctrl Pts',(39.2916080338993,1.87113616999862,-136.00455070594));
#157835=CARTESIAN_POINT('Ctrl Pts',(39.2764341215566,1.87371871904832,-135.953871704315));
#157836=CARTESIAN_POINT('Ctrl Pts',(39.2604385453299,1.8765448407645,-135.898316363799));
#157837=CARTESIAN_POINT('Ctrl Pts',(39.2439796575266,1.87961420051954,-135.837827876053));
#157838=CARTESIAN_POINT('Ctrl Pts',(39.2275207697233,1.88268356027457,-135.777339388308));
#157839=CARTESIAN_POINT('Ctrl Pts',(39.2105986989925,1.88599627399723,-135.711915499126));
#157840=CARTESIAN_POINT('Ctrl Pts',(39.1936207585355,1.88955053178332,-135.641515239685));
#157841=CARTESIAN_POINT('Ctrl Pts',(39.1927210714146,1.88973887735814,-135.637784621893));
#157842=CARTESIAN_POINT('Ctrl Pts',(39.1915408777627,1.88998700014396,-135.632869094502));
#157843=CARTESIAN_POINT('Ctrl Pts',(39.1909213209675,1.89011760234143,-135.630281476236));
#157844=CARTESIAN_POINT('Ctrl Pts',(39.1908306970963,1.89013670579862,-135.629902979888));
#157845=CARTESIAN_POINT('Ctrl Pts',(39.1907401153123,1.89015580793797,-135.629524521743));
#157846=CARTESIAN_POINT('Ctrl Pts',(39.1906495755884,1.89017490875729,-135.629146101804));
#157847=CARTESIAN_POINT('Ctrl Pts',(39.1688106141026,1.89478219094973,-135.537867952023));
#157848=CARTESIAN_POINT('Ctrl Pts',(39.1494516718396,1.89931800089657,-135.448695842305));
#157849=CARTESIAN_POINT('Ctrl Pts',(39.1322641903651,1.90374697366022,-135.361758548468));
#157850=CARTESIAN_POINT('Ctrl Pts',(39.1183456696376,1.90733358111656,-135.291356231057));
#157851=CARTESIAN_POINT('Ctrl Pts',(39.1058515634338,1.910850196318,-135.222418328487));
#157852=CARTESIAN_POINT('Ctrl Pts',(39.0946282203871,1.9142795706683,-135.154990566977));
#157853=CARTESIAN_POINT('Ctrl Pts',(39.0794701304433,1.9189112356398,-135.06392357656));
#157854=CARTESIAN_POINT('Ctrl Pts',(39.0666297867406,1.92338527749994,-134.975613379054));
#157855=CARTESIAN_POINT('Ctrl Pts',(39.0557624151109,1.92766357312286,-134.89020734062));
#157856=CARTESIAN_POINT('Ctrl Pts',(39.0486059555491,1.93048094706223,-134.833965143223));
#157857=CARTESIAN_POINT('Ctrl Pts',(39.0423054581754,1.93321351492931,-134.77898124839));
#157858=CARTESIAN_POINT('Ctrl Pts',(39.0367670376279,1.93585124621579,-134.725286427561));
#157859=CARTESIAN_POINT('Ctrl Pts',(39.0280343318381,1.94001028958918,-134.640623107267));
#157860=CARTESIAN_POINT('Ctrl Pts',(39.0211901513801,1.94394587338376,-134.55913268505));
#157861=CARTESIAN_POINT('Ctrl Pts',(39.015888450433,1.94769256523156,-134.480886044911));
#157862=CARTESIAN_POINT('Ctrl Pts',(39.0104340250084,1.95154718688547,-134.400385377742));
#157863=CARTESIAN_POINT('Ctrl Pts',(39.006612106687,1.95520190735825,-134.323317581055));
#157864=CARTESIAN_POINT('Ctrl Pts',(39.0040807323282,1.95869471836818,-134.249716322542));
#157865=CARTESIAN_POINT('Ctrl Pts',(39.0014556000694,1.96231689729392,-134.173388995717));
#157866=CARTESIAN_POINT('Ctrl Pts',(39.0002182001485,1.96576496763912,-134.100789292161));
#157867=CARTESIAN_POINT('Ctrl Pts',(39.000026518969,1.96908130239247,-134.031915960005));
#157868=CARTESIAN_POINT('Ctrl Pts',(39.000008754634,1.96938864858968,-134.025533022726));
#157869=CARTESIAN_POINT('Ctrl Pts',(39.,1.96969486323497,-134.019182067323));
#157870=CARTESIAN_POINT('Ctrl Pts',(39.,1.96999998000015,-134.012863078852));
#157871=CARTESIAN_POINT('Ctrl Pts',(39.,-3.68000001999999,-130.802732351058));
#157872=CARTESIAN_POINT('Ctrl Pts',(39.,-3.68320699217295,-130.887923832903));
#157873=CARTESIAN_POINT('Ctrl Pts',(39.0018493117517,-3.68659779226474,
-130.977410061787));
#157874=CARTESIAN_POINT('Ctrl Pts',(39.006160362258,-3.69017516856669,-131.071072933503));
#157875=CARTESIAN_POINT('Ctrl Pts',(39.009621104999,-3.69304694635053,-131.146261823757));
#157876=CARTESIAN_POINT('Ctrl Pts',(39.0146693161162,-3.6960389628621,-131.224142051601));
#157877=CARTESIAN_POINT('Ctrl Pts',(39.021645013605,-3.69915270994247,-131.304648061783));
#157878=CARTESIAN_POINT('Ctrl Pts',(39.0263019739025,-3.70123144064329,
-131.358393697072));
#157879=CARTESIAN_POINT('Ctrl Pts',(39.0318189308278,-3.70336458614086,
-131.413313609595));
#157880=CARTESIAN_POINT('Ctrl Pts',(39.0382997789448,-3.70555193766198,
-131.469370363117));
#157881=CARTESIAN_POINT('Ctrl Pts',(39.0486691056802,-3.70905168988551,
-131.559060907086));
#157882=CARTESIAN_POINT('Ctrl Pts',(39.0615053548553,-3.7126900014574,-131.651656352322));
#157883=CARTESIAN_POINT('Ctrl Pts',(39.0772366782264,-3.71646510502138,
-131.746979581721));
#157884=CARTESIAN_POINT('Ctrl Pts',(39.0925140114832,-3.72013126290684,
-131.839551878932));
#157885=CARTESIAN_POINT('Ctrl Pts',(39.1105225354627,-3.72392632174515,
-131.934693626701));
#157886=CARTESIAN_POINT('Ctrl Pts',(39.131639726789,-3.72784618719993,-132.032183000023));
#157887=CARTESIAN_POINT('Ctrl Pts',(39.1362592325343,-3.72870368006957,
-132.053509355086));
#157888=CARTESIAN_POINT('Ctrl Pts',(39.1410274043101,-3.72956713592367,
-132.074947836959));
#157889=CARTESIAN_POINT('Ctrl Pts',(39.1459480171903,-3.7304364973889,-132.096495803533));
#157890=CARTESIAN_POINT('Ctrl Pts',(39.1463940915734,-3.73051530868512,
-132.098449217901));
#157891=CARTESIAN_POINT('Ctrl Pts',(39.1471435285986,-3.73064731141171,
-132.101720321296));
#157892=CARTESIAN_POINT('Ctrl Pts',(39.1472900013385,-3.73067307710898,
-132.102358743601));
#157893=CARTESIAN_POINT('Ctrl Pts',(39.1473069993462,-3.73067606719111,
-132.10243283184));
#157894=CARTESIAN_POINT('Ctrl Pts',(39.1473240236054,-3.73067906164339,
-132.10250702793));
#157895=CARTESIAN_POINT('Ctrl Pts',(39.1473410741282,-3.73068206046583,
-132.102581331868));
#157896=CARTESIAN_POINT('Ctrl Pts',(39.1506177864137,-3.73125836410335,
-132.116860813524));
#157897=CARTESIAN_POINT('Ctrl Pts',(39.1548622386872,-3.73199618726408,
-132.135127161461));
#157898=CARTESIAN_POINT('Ctrl Pts',(39.1601911467889,-3.73289584576598,
-132.157352936904));
#157899=CARTESIAN_POINT('Ctrl Pts',(39.1655157741583,-3.73379478156875,
-132.179560858298));
#157900=CARTESIAN_POINT('Ctrl Pts',(39.1719231966379,-3.73485530708176,
-132.205722138333));
#157901=CARTESIAN_POINT('Ctrl Pts',(39.1795804315515,-3.73607783719616,
-132.235797617303));
#157902=CARTESIAN_POINT('Ctrl Pts',(39.1862116453768,-3.73713655600104,
-132.261843172155));
#157903=CARTESIAN_POINT('Ctrl Pts',(39.1937810024339,-3.73831678222952,
-132.290824222945));
#157904=CARTESIAN_POINT('Ctrl Pts',(39.2024269115509,-3.73961870163836,
-132.322705237269));
#157905=CARTESIAN_POINT('Ctrl Pts',(39.2123357614401,-3.74111079735848,
-132.359243232403));
#157906=CARTESIAN_POINT('Ctrl Pts',(39.2236573987929,-3.74276269105182,
-132.399589405842));
#157907=CARTESIAN_POINT('Ctrl Pts',(39.2366415304428,-3.74457397905163,
-132.443662692744));
#157908=CARTESIAN_POINT('Ctrl Pts',(39.2493021068547,-3.74634013105502,
-132.486637704982));
#157909=CARTESIAN_POINT('Ctrl Pts',(39.2635438263983,-3.74825787607168,
-132.533157316448));
#157910=CARTESIAN_POINT('Ctrl Pts',(39.2796379042396,-3.75032602419857,
-132.583117096287));
#157911=CARTESIAN_POINT('Ctrl Pts',(39.2888298631554,-3.75150722468746,
-132.611651085513));
#157912=CARTESIAN_POINT('Ctrl Pts',(39.2986267896565,-3.75273747274754,
-132.64130675528));
#157913=CARTESIAN_POINT('Ctrl Pts',(39.3090846344843,-3.7540163764884,-132.672059341533));
#157914=CARTESIAN_POINT('Ctrl Pts',(39.3124808338629,-3.75443170222344,
-132.682046285884));
#157915=CARTESIAN_POINT('Ctrl Pts',(39.3159467643173,-3.75485215835433,
-132.692148877582));
#157916=CARTESIAN_POINT('Ctrl Pts',(39.3194844958346,-3.75527819196887,
-132.702366145836));
#157917=CARTESIAN_POINT('Ctrl Pts',(39.3212533615932,-3.75549120877614,
-132.707474779963));
#157918=CARTESIAN_POINT('Ctrl Pts',(39.3230401941007,-3.75570572694133,
-132.712612077562));
#157919=CARTESIAN_POINT('Ctrl Pts',(39.3248451944342,-3.75592137730407,
-132.717777933179));
#157920=CARTESIAN_POINT('Ctrl Pts',(39.3266501947677,-3.75613702766681,
-132.722943788797));
#157921=CARTESIAN_POINT('Ctrl Pts',(39.3288894696748,-3.7564030433275,-132.72931830416));
#157922=CARTESIAN_POINT('Ctrl Pts',(39.3303149522011,-3.75657170342897,
-132.733361050105));
#157923=CARTESIAN_POINT('Ctrl Pts',(39.3540564862143,-3.75938075191748,
-132.800693331353));
#157924=CARTESIAN_POINT('Ctrl Pts',(39.3778323091587,-3.76204300277362,
-132.864162372071));
#157925=CARTESIAN_POINT('Ctrl Pts',(39.401268547416,-3.76455722155949,-132.923846293981));
#157926=CARTESIAN_POINT('Ctrl Pts',(39.4251684250805,-3.76712117916839,
-132.984710943696));
#157927=CARTESIAN_POINT('Ctrl Pts',(39.4487151410444,-3.76953121903715,
-133.041639875485));
#157928=CARTESIAN_POINT('Ctrl Pts',(39.4715634783474,-3.77178764461923,
-133.094737153497));
#157929=CARTESIAN_POINT('Ctrl Pts',(39.4949245826598,-3.77409470936084,
-133.149026051368));
#157930=CARTESIAN_POINT('Ctrl Pts',(39.517555574636,-3.77624121630412,-133.199310024175));
#157931=CARTESIAN_POINT('Ctrl Pts',(39.5391409289902,-3.77822871249156,
-133.245712369463));
#157932=CARTESIAN_POINT('Ctrl Pts',(39.5552925697658,-3.7797158932872,-133.280433782879));
#157933=CARTESIAN_POINT('Ctrl Pts',(39.5708598736309,-3.78111407042952,
-133.312982141961));
#157934=CARTESIAN_POINT('Ctrl Pts',(39.5857296458368,-3.78242418360352,
-133.343410256559));
#157935=CARTESIAN_POINT('Origin',(0.,-12.9675000200281,-171.64995));
#157936=CARTESIAN_POINT('',(57.6746235421417,-3.75150367745622,-171.449026400902));
#157937=CARTESIAN_POINT('',(56.4941621559325,1.85499746228791,-171.449026400902));
#157938=CARTESIAN_POINT('Origin',(0.,-12.9675000200281,-171.449026400902));
#157939=CARTESIAN_POINT('Ctrl Pts',(56.4941621559325,1.85499746228791,-171.449026400902));
#157940=CARTESIAN_POINT('Ctrl Pts',(55.5872148662684,1.85328258784851,-169.566813619198));
#157941=CARTESIAN_POINT('Ctrl Pts',(54.6987069265873,1.85157789414912,-167.72566026361));
#157942=CARTESIAN_POINT('Ctrl Pts',(53.8286007394999,1.84982266457049,-165.9255866409));
#157943=CARTESIAN_POINT('Ctrl Pts',(53.2735091105652,1.84870290095956,-164.777214391328));
#157944=CARTESIAN_POINT('Ctrl Pts',(52.7259078414064,1.84756262081415,-163.645560727361));
#157945=CARTESIAN_POINT('Ctrl Pts',(52.1857969712753,1.8463865543554,-162.53062597535));
#157946=CARTESIAN_POINT('Ctrl Pts',(51.492429613171,1.84487677897675,-161.099328428474));
#157947=CARTESIAN_POINT('Ctrl Pts',(50.8114042047774,1.84331606104898,-159.69558475759));
#157948=CARTESIAN_POINT('Ctrl Pts',(50.1427245048726,1.84172122826594,-158.319391243539));
#157949=CARTESIAN_POINT('Ctrl Pts',(49.8083846549203,1.84092381187443,-157.631294486514));
#157950=CARTESIAN_POINT('Ctrl Pts',(49.4771313616882,1.84011838355358,-156.950085170635));
#157951=CARTESIAN_POINT('Ctrl Pts',(49.1489657089356,1.83931015210421,-156.27576229937));
#157952=CARTESIAN_POINT('Ctrl Pts',(48.9848828825593,1.83890603637952,-155.938600863737));
#157953=CARTESIAN_POINT('Ctrl Pts',(48.8215719791454,1.83850122447541,-155.60316103291));
#157954=CARTESIAN_POINT('Ctrl Pts',(48.6590331509111,1.83809659258963,-155.269442654971));
#157955=CARTESIAN_POINT('Ctrl Pts',(48.5777637367939,1.83789427664674,-155.102583466001));
#157956=CARTESIAN_POINT('Ctrl Pts',(48.4966873421834,1.83769200598395,-154.936154639899));
#157957=CARTESIAN_POINT('Ctrl Pts',(48.4158039886763,1.83748989727043,-154.770156155779));
#157958=CARTESIAN_POINT('Ctrl Pts',(48.3753623119227,1.83738884291367,-154.687156913718));
#157959=CARTESIAN_POINT('Ctrl Pts',(48.3349688954873,1.83728782906129,-154.604265257132));
#157960=CARTESIAN_POINT('Ctrl Pts',(48.2946237421284,1.837186871069,-154.521481183311));
#157961=CARTESIAN_POINT('Ctrl Pts',(48.2593217329394,1.83709853282574,-154.449045118718));
#157962=CARTESIAN_POINT('Ctrl Pts',(48.224056675171,1.8370102373514,-154.376691422179));
#157963=CARTESIAN_POINT('Ctrl Pts',(48.1888285707055,1.83692199521058,-154.304420091836));
#157964=CARTESIAN_POINT('Ctrl Pts',(48.1837959843533,1.83690938919046,-154.294095616072));
#157965=CARTESIAN_POINT('Ctrl Pts',(48.1796675061752,1.83689904733514,-154.285626026406));
#157966=CARTESIAN_POINT('Ctrl Pts',(48.1737330726839,1.83688418615863,-154.273451708059));
#157967=CARTESIAN_POINT('Ctrl Pts',(48.1736305779674,1.83688392948846,-154.273241443119));
#157968=CARTESIAN_POINT('Ctrl Pts',(48.1735280835149,1.83688367281755,-154.273031178774));
#157969=CARTESIAN_POINT('Ctrl Pts',(48.1734255893264,1.83688341614592,-154.272820915026));
#157970=CARTESIAN_POINT('Ctrl Pts',(47.4138476394261,1.83498123889893,-152.714569574048));
#157971=CARTESIAN_POINT('Ctrl Pts',(46.6687914400752,1.83303990966285,-151.189068021751));
#157972=CARTESIAN_POINT('Ctrl Pts',(45.938183755171,1.83105643289783,-149.696350512763));
#157973=CARTESIAN_POINT('Ctrl Pts',(45.1949410991184,1.82903865431501,-148.177818270302));
#157974=CARTESIAN_POINT('Ctrl Pts',(44.4666512921154,1.82697727414329,-146.693213656769));
#157975=CARTESIAN_POINT('Ctrl Pts',(43.7532878193704,1.82487206350732,-145.24254696461));
#157976=CARTESIAN_POINT('Ctrl Pts',(43.0079230141743,1.82267241357356,-143.726803675645));
#157977=CARTESIAN_POINT('Ctrl Pts',(42.278853870262,1.82042491917042,-142.248111447343));
#157978=CARTESIAN_POINT('Ctrl Pts',(41.5661022554074,1.81813232414976,-140.806455468107));
#157979=CARTESIAN_POINT('Ctrl Pts',(40.9493421409949,1.81614848975672,-139.558957899297));
#157980=CARTESIAN_POINT('Ctrl Pts',(40.3448013391909,1.81413094379836,-138.339191935329));
#157981=CARTESIAN_POINT('Ctrl Pts',(39.7525219240432,1.81208306781681,-137.147133758372));
#157982=CARTESIAN_POINT('Ctrl Pts',(39.5857308656309,-3.78242429107441,
-133.34341275263));
#157983=CARTESIAN_POINT('Ctrl Pts',(40.9519549067385,-3.77910503324588,
-136.199077491809));
#157984=CARTESIAN_POINT('Ctrl Pts',(42.3907152118192,-3.77572283235729,
-139.21370723183));
#157985=CARTESIAN_POINT('Ctrl Pts',(44.6577376745155,-3.77119731722451,
-143.974099343123));
#157986=CARTESIAN_POINT('Ctrl Pts',(45.4315569217728,-3.76976624204378,
-145.600637963764));
#157987=CARTESIAN_POINT('Ctrl Pts',(46.6194990079656,-3.76769078813001,
-148.100057770041));
#157988=CARTESIAN_POINT('Ctrl Pts',(47.2202732321399,-3.76666954253768,
-149.364670642009));
#157989=CARTESIAN_POINT('Ctrl Pts',(47.933079937314,-3.76548325423015,-150.866132521422));
#157990=CARTESIAN_POINT('Ctrl Pts',(48.2924588112532,-3.76488740822001,
-151.623383509991));
#157991=CARTESIAN_POINT('Ctrl Pts',(48.4954462437539,-3.76455089104309,
-152.051170954804));
#157992=CARTESIAN_POINT('Ctrl Pts',(48.5955948730132,-3.76438477362141,
-152.262252292382));
#157993=CARTESIAN_POINT('Ctrl Pts',(48.6473508980734,-3.76429887944539,
-152.37134303568));
#157994=CARTESIAN_POINT('Ctrl Pts',(48.651123012323,-3.76429261899403,-152.379293884756));
#157995=CARTESIAN_POINT('Ctrl Pts',(51.416797493966,-3.75970237622441,-158.208789756719));
#157996=CARTESIAN_POINT('Ctrl Pts',(54.4237264557334,-3.75540420604071,
-164.563471491086));
#157997=CARTESIAN_POINT('Ctrl Pts',(57.6746235421417,-3.75150367745622,
-171.449026400902));
#157998=CARTESIAN_POINT('Ctrl Pts',(60.,-4.67636962353871,-174.488179236421));
#157999=CARTESIAN_POINT('Ctrl Pts',(60.,-4.58657792455374,-176.471369022159));
#158000=CARTESIAN_POINT('Ctrl Pts',(58.1727505513102,-4.55147683639116,
-177.246631327017));
#158001=CARTESIAN_POINT('Ctrl Pts',(60.,-4.88047860745801,-174.497420557097));
#158002=CARTESIAN_POINT('Ctrl Pts',(60.0000000000001,-4.78987454640719,
-176.45995577904));
#158003=CARTESIAN_POINT('Ctrl Pts',(58.1991963791505,-4.75453073304092,
-177.244581482931));
#158004=CARTESIAN_POINT('Ctrl Pts',(60.,-5.08458311893969,-174.506824441727));
#158005=CARTESIAN_POINT('Ctrl Pts',(59.9999999999904,-4.99421808034747,
-176.449490545983));
#158006=CARTESIAN_POINT('Ctrl Pts',(58.2246968063274,-4.95813196877381,
-177.242671121044));
#158007=CARTESIAN_POINT('Ctrl Pts',(60.,-5.28868572332295,-174.51629758862));
#158008=CARTESIAN_POINT('Ctrl Pts',(60.,-5.19940519654632,-176.439881014021));
#158009=CARTESIAN_POINT('Ctrl Pts',(58.2492435654384,-5.16222748868145,
-177.240889086276));
#158010=CARTESIAN_POINT('',(60.,-5.18000001999999,-174.511260182693));
#158011=CARTESIAN_POINT('',(58.2670184333942,-5.15898900219891,-177.232516794804));
#158012=CARTESIAN_POINT('Ctrl Pts',(60.,-5.18000001999999,-174.511260182693));
#158013=CARTESIAN_POINT('Ctrl Pts',(60.,-5.1799272377721,-174.520713255673));
#158014=CARTESIAN_POINT('Ctrl Pts',(59.9999613146273,-5.17983454997278,
-174.533245214993));
#158015=CARTESIAN_POINT('Ctrl Pts',(59.9997683044872,-5.17971977325836,
-174.548915860866));
#158016=CARTESIAN_POINT('Ctrl Pts',(59.9995874353749,-5.17961221640953,
-174.563600767101));
#158017=CARTESIAN_POINT('Ctrl Pts',(59.9992707239901,-5.17948526269027,
-174.581041858777));
#158018=CARTESIAN_POINT('Ctrl Pts',(59.99867265545,-5.17933717776086,-174.6012798489));
#158019=CARTESIAN_POINT('Ctrl Pts',(59.99808144442,-5.17919079078715,-174.621285788327));
#158020=CARTESIAN_POINT('Ctrl Pts',(59.9972154017306,-5.1790237543439,-174.644024877617));
#158021=CARTESIAN_POINT('Ctrl Pts',(59.9958839884361,-5.17883445369421,
-174.669527960362));
#158022=CARTESIAN_POINT('Ctrl Pts',(59.9945723442879,-5.17864796382631,
-174.69465236717));
#158023=CARTESIAN_POINT('Ctrl Pts',(59.9928091104631,-5.17843986597539,
-174.722459311834));
#158024=CARTESIAN_POINT('Ctrl Pts',(59.9903620933743,-5.17820867615274,
-174.752969724891));
#158025=CARTESIAN_POINT('Ctrl Pts',(59.9897615851697,-5.17815194120554,
-174.760457107571));
#158026=CARTESIAN_POINT('Ctrl Pts',(59.9891196557456,-5.17809381587359,
-174.768107260234));
#158027=CARTESIAN_POINT('Ctrl Pts',(59.988432396927,-5.17803427879222,-174.775920410068));
#158028=CARTESIAN_POINT('Ctrl Pts',(59.9856554152033,-5.17779370947197,
-174.807490720562));
#158029=CARTESIAN_POINT('Ctrl Pts',(59.9821408038309,-5.17752962562884,
-174.841740394733));
#158030=CARTESIAN_POINT('Ctrl Pts',(59.9775984010229,-5.17724229616848,
-174.878666355715));
#158031=CARTESIAN_POINT('Ctrl Pts',(59.9730975147709,-5.17695759283578,
-174.915254821588));
#158032=CARTESIAN_POINT('Ctrl Pts',(59.9675875782563,-5.17665006670961,
-174.954470891117));
#158033=CARTESIAN_POINT('Ctrl Pts',(59.9607357962623,-5.17632004513401,
-174.996302707221));
#158034=CARTESIAN_POINT('Ctrl Pts',(59.9592196006012,-5.17624701635385,
-175.005559455047));
#158035=CARTESIAN_POINT('Ctrl Pts',(59.9576374998204,-5.17617288630168,
-175.014944252933));
#158036=CARTESIAN_POINT('Ctrl Pts',(59.9559855465045,-5.17609765897697,
-175.024456911882));
#158037=CARTESIAN_POINT('Ctrl Pts',(59.9481389578712,-5.17574033781949,
-175.069640949992));
#158038=CARTESIAN_POINT('Ctrl Pts',(59.9387215277951,-5.17535866288732,
-175.117704292394));
#158039=CARTESIAN_POINT('Ctrl Pts',(59.9272892750181,-5.17495659188962,
-175.168559246422));
#158040=CARTESIAN_POINT('Ctrl Pts',(59.9265912438941,-5.17493204221635,
-175.171664351024));
#158041=CARTESIAN_POINT('Ctrl Pts',(59.9258856855017,-5.17490741653123,
-175.174779860105));
#158042=CARTESIAN_POINT('Ctrl Pts',(59.9251724926247,-5.17488271574553,
-175.177905752576));
#158043=CARTESIAN_POINT('Ctrl Pts',(59.9189756112986,-5.17466809240504,
-175.205066406175));
#158044=CARTESIAN_POINT('Ctrl Pts',(59.9122028334488,-5.17444785344947,
-175.233010001163));
#158045=CARTESIAN_POINT('Ctrl Pts',(59.904783763042,-5.1742229673739,-175.261715234116));
#158046=CARTESIAN_POINT('Ctrl Pts',(59.9010742278385,-5.17411052433611,
-175.276067850593));
#158047=CARTESIAN_POINT('Ctrl Pts',(59.8972030676678,-5.17399691988581,
-175.290610868415));
#158048=CARTESIAN_POINT('Ctrl Pts',(59.8931613792453,-5.17388230573763,
-175.305340960976));
#158049=CARTESIAN_POINT('Ctrl Pts',(59.891140535034,-5.17382499866353,-175.312706007257));
#158050=CARTESIAN_POINT('Ctrl Pts',(59.889077056277,-5.17376743915838,-175.320117822345));
#158051=CARTESIAN_POINT('Ctrl Pts',(59.8869698226738,-5.17370964723968,
-175.327575967589));
#158052=CARTESIAN_POINT('Ctrl Pts',(59.8859162058722,-5.17368075128032,
-175.331305040212));
#158053=CARTESIAN_POINT('Ctrl Pts',(59.8848516502199,-5.17365179721695,
-175.335045695386));
#158054=CARTESIAN_POINT('Ctrl Pts',(59.8837760155946,-5.17362278766247,
-175.338797875885));
#158055=CARTESIAN_POINT('Ctrl Pts',(59.8827003809693,-5.17359377810799,
-175.342550056383));
#158056=CARTESIAN_POINT('Ctrl Pts',(59.8812553100241,-5.17355521136971,
-175.347545951429));
#158057=CARTESIAN_POINT('Ctrl Pts',(59.8805157344353,-5.17353559732074,
-175.350088935428));
#158058=CARTESIAN_POINT('Ctrl Pts',(59.8800176333053,-5.17352238733908,
-175.351801624737));
#158059=CARTESIAN_POINT('Ctrl Pts',(59.8795184251299,-5.17350919095032,
-175.353512540531));
#158060=CARTESIAN_POINT('Ctrl Pts',(59.8790181177072,-5.17349600812921,
-175.355221686178));
#158061=CARTESIAN_POINT('Ctrl Pts',(59.8654362414286,-5.17313813327622,
-175.401619967842));
#158062=CARTESIAN_POINT('Ctrl Pts',(59.8509971474762,-5.17279016162673,
-175.446725987013));
#158063=CARTESIAN_POINT('Ctrl Pts',(59.8359110132716,-5.17245277034999,
-175.490454018024));
#158064=CARTESIAN_POINT('Ctrl Pts',(59.8203336981495,-5.17210439414134,
-175.535605765283));
#158065=CARTESIAN_POINT('Ctrl Pts',(59.8040664089156,-5.17176729583692,
-175.579288675368));
#158066=CARTESIAN_POINT('Ctrl Pts',(59.7873050482715,-5.17144188203371,
-175.621452071484));
#158067=CARTESIAN_POINT('Ctrl Pts',(59.7697421073717,-5.17110090593307,
-175.665631851983));
#158068=CARTESIAN_POINT('Ctrl Pts',(59.7516366599007,-5.17077275638255,
-175.70814359908));
#158069=CARTESIAN_POINT('Ctrl Pts',(59.7331769155636,-5.1704575724523,-175.748971379014));
#158070=CARTESIAN_POINT('Ctrl Pts',(59.7318411535293,-5.17043476548812,
-175.7519257102));
#158071=CARTESIAN_POINT('Ctrl Pts',(59.7305035211752,-5.1704120262858,-175.754871240386));
#158072=CARTESIAN_POINT('Ctrl Pts',(59.7291640828256,-5.17038935484021,
-175.757807970983));
#158073=CARTESIAN_POINT('Ctrl Pts',(59.7245308271502,-5.17031093196695,
-175.767966425615));
#158074=CARTESIAN_POINT('Ctrl Pts',(59.7198743116007,-5.17023326574134,
-175.778026603707));
#158075=CARTESIAN_POINT('Ctrl Pts',(59.7151963681919,-5.17015634142143,
-175.787990446344));
#158076=CARTESIAN_POINT('Ctrl Pts',(59.6859083951819,-5.16967472862527,
-175.850372721789));
#158077=CARTESIAN_POINT('Ctrl Pts',(59.6559202772399,-5.16922449040161,
-175.908679583196));
#158078=CARTESIAN_POINT('Ctrl Pts',(59.6259391187632,-5.16880507771954,
-175.962986478089));
#158079=CARTESIAN_POINT('Ctrl Pts',(59.6006389687672,-5.16845114864189,
-176.008814346537));
#158080=CARTESIAN_POINT('Ctrl Pts',(59.5753448613497,-5.16811915863265,
-176.051795357692));
#158081=CARTESIAN_POINT('Ctrl Pts',(59.5504391432744,-5.16780833955879,
-176.092031152333));
#158082=CARTESIAN_POINT('Ctrl Pts',(59.5458311121938,-5.16775083212421,
-176.099475538867));
#158083=CARTESIAN_POINT('Ctrl Pts',(59.5412362469768,-5.16769404861673,
-176.106826053089));
#158084=CARTESIAN_POINT('Ctrl Pts',(59.5366567934599,-5.16763798325383,
-176.11408345595));
#158085=CARTESIAN_POINT('Ctrl Pts',(59.5348607551479,-5.16761599470447,
-176.116929772335));
#158086=CARTESIAN_POINT('Ctrl Pts',(59.5337373392218,-5.16760226626031,
-176.118706848888));
#158087=CARTESIAN_POINT('Ctrl Pts',(59.5313782454486,-5.16757359498196,
-176.122418507681));
#158088=CARTESIAN_POINT('Ctrl Pts',(59.5312518004227,-5.16757205823061,
-176.122617448815));
#158089=CARTESIAN_POINT('Ctrl Pts',(59.5311217942244,-5.16757047859849,
-176.122821941482));
#158090=CARTESIAN_POINT('Ctrl Pts',(59.5309879284935,-5.16756885253193,
-176.123032445711));
#158091=CARTESIAN_POINT('Ctrl Pts',(59.5290762516248,-5.16754563139973,
-176.126038562844));
#158092=CARTESIAN_POINT('Ctrl Pts',(59.5271600421084,-5.16752244583908,
-176.12904004279));
#158093=CARTESIAN_POINT('Ctrl Pts',(59.5252393170933,-5.16749929577026,
-176.132036896267));
#158094=CARTESIAN_POINT('Ctrl Pts',(59.4885613142581,-5.16705722400919,
-176.189264557424));
#158095=CARTESIAN_POINT('Ctrl Pts',(59.4500653841475,-5.16662664608057,
-176.244992491202));
#158096=CARTESIAN_POINT('Ctrl Pts',(59.4101077057974,-5.16620977760933,
-176.298936679342));
#158097=CARTESIAN_POINT('Ctrl Pts',(59.3694359516207,-5.16578545936345,
-176.353844893479));
#158098=CARTESIAN_POINT('Ctrl Pts',(59.3272496939177,-5.16537534434658,
-176.4069051164));
#158099=CARTESIAN_POINT('Ctrl Pts',(59.2838905709168,-5.16498144614305,
-176.457859440189));
#158100=CARTESIAN_POINT('Ctrl Pts',(59.2787049812111,-5.1649343373842,-176.463953387636));
#158101=CARTESIAN_POINT('Ctrl Pts',(59.2735025769242,-5.16488746021233,
-176.470017261057));
#158102=CARTESIAN_POINT('Ctrl Pts',(59.2682839111567,-5.16484081777635,
-176.476050657348));
#158103=CARTESIAN_POINT('Ctrl Pts',(59.198184488061,-5.16421429597941,-176.557093900619));
#158104=CARTESIAN_POINT('Ctrl Pts',(59.1254281377786,-5.16363128018837,
-176.63248959021));
#158105=CARTESIAN_POINT('Ctrl Pts',(59.0504291615598,-5.16308787519053,
-176.702751972211));
#158106=CARTESIAN_POINT('Ctrl Pts',(59.0228175280704,-5.16288781513113,
-176.728619780516));
#158107=CARTESIAN_POINT('Ctrl Pts',(58.994901582676,-5.16269312687973,-176.753791426191));
#158108=CARTESIAN_POINT('Ctrl Pts',(58.966700826357,-5.16250362596014,-176.778291252628));
#158109=CARTESIAN_POINT('Ctrl Pts',(58.9580740402192,-5.16244565645437,
-176.785785901378));
#158110=CARTESIAN_POINT('Ctrl Pts',(58.9494150826379,-5.16238815490271,
-176.79321994001));
#158111=CARTESIAN_POINT('Ctrl Pts',(58.9407254879922,-5.16233112230567,
-176.800593251677));
#158112=CARTESIAN_POINT('Ctrl Pts',(58.8901282302924,-5.16199903627317,
-176.843526134708));
#158113=CARTESIAN_POINT('Ctrl Pts',(58.8387753737899,-5.16168474946931,
-176.884162608041));
#158114=CARTESIAN_POINT('Ctrl Pts',(58.7869638405979,-5.1613877473488,-176.922564128275));
#158115=CARTESIAN_POINT('Ctrl Pts',(58.7327825694257,-5.16107716104806,
-176.962722043955));
#158116=CARTESIAN_POINT('Ctrl Pts',(58.6780996195717,-5.1607854754869,-177.000436045426));
#158117=CARTESIAN_POINT('Ctrl Pts',(58.6231983985429,-5.16051201831244,
-177.035786965185));
#158118=CARTESIAN_POINT('Ctrl Pts',(58.5639650113499,-5.16021698307657,
-177.073927368595));
#158119=CARTESIAN_POINT('Ctrl Pts',(58.5044777230962,-5.15994316516394,
-177.109317211894));
#158120=CARTESIAN_POINT('Ctrl Pts',(58.4450274076812,-5.15968964438824,
-177.142067473344));
#158121=CARTESIAN_POINT('Ctrl Pts',(58.3855770922661,-5.15943612361254,
-177.174817734794));
#158122=CARTESIAN_POINT('Ctrl Pts',(58.3261631370263,-5.15920289782321,
-177.204928688562));
#158123=CARTESIAN_POINT('Ctrl Pts',(58.2670184333942,-5.15898900219891,
-177.232516794804));
#158124=CARTESIAN_POINT('',(58.2078173715129,-4.65917712431111,-177.236349007278));
#158125=CARTESIAN_POINT('Origin',(-8.73110974027571,-12.9198662892988,-187.475563684127));
#158126=CARTESIAN_POINT('',(60.,-4.68000001999999,-174.488343624884));
#158127=CARTESIAN_POINT('Ctrl Pts',(58.2078173713336,-4.65917712527795,
-177.236349006383));
#158128=CARTESIAN_POINT('Ctrl Pts',(58.2680396583105,-4.65937904897621,
-177.209843370633));
#158129=CARTESIAN_POINT('Ctrl Pts',(58.3286061602997,-4.6595903192446,-177.180819390645));
#158130=CARTESIAN_POINT('Ctrl Pts',(58.389247772245,-4.65981829367543,-177.149112865983));
#158131=CARTESIAN_POINT('Ctrl Pts',(58.4488949403758,-4.66004252962116,
-177.117926287218));
#158132=CARTESIAN_POINT('Ctrl Pts',(58.5086145427696,-4.66028295223093,
-177.084143855486));
#158133=CARTESIAN_POINT('Ctrl Pts',(58.5681109624229,-4.66054518977293,
-177.047638867556));
#158134=CARTESIAN_POINT('Ctrl Pts',(58.6261911081638,-4.6608011849193,-177.01200285733));
#158135=CARTESIAN_POINT('Ctrl Pts',(58.6840581776048,-4.66107798952929,
-176.973771908009));
#158136=CARTESIAN_POINT('Ctrl Pts',(58.7414038465745,-4.66137918120361,
-176.932863994594));
#158137=CARTESIAN_POINT('Ctrl Pts',(58.7956818748661,-4.66166426097535,
-176.89414440301));
#158138=CARTESIAN_POINT('Ctrl Pts',(58.8494922433316,-4.66197119389585,
-176.853026464809));
#158139=CARTESIAN_POINT('Ctrl Pts',(58.9025503147113,-4.66230134010155,
-176.809476916618));
#158140=CARTESIAN_POINT('Ctrl Pts',(58.9569411261647,-4.66263977909037,
-176.764833468356));
#158141=CARTESIAN_POINT('Ctrl Pts',(59.0105409839596,-4.66300263959302,
-176.717634115967));
#158142=CARTESIAN_POINT('Ctrl Pts',(59.0630247791536,-4.66338930132797,
-176.667888366361));
#158143=CARTESIAN_POINT('Ctrl Pts',(59.114910853718,-4.66377155949998,-176.618709154687));
#158144=CARTESIAN_POINT('Ctrl Pts',(59.1657055368162,-4.66417709024071,
-176.567040982309));
#158145=CARTESIAN_POINT('Ctrl Pts',(59.2150845173184,-4.66460301486336,
-176.512942701094));
#158146=CARTESIAN_POINT('Ctrl Pts',(59.2637965700052,-4.66502318681605,
-176.459575088032));
#158147=CARTESIAN_POINT('Ctrl Pts',(59.3111302557302,-4.66546320851134,
-176.40384249302));
#158148=CARTESIAN_POINT('Ctrl Pts',(59.356773551464,-4.66591798745967,-176.345852268448));
#158149=CARTESIAN_POINT('Ctrl Pts',(59.3632118699717,-4.66598213733476,
-176.337672325915));
#158150=CARTESIAN_POINT('Ctrl Pts',(59.3696165628679,-4.6660465769791,-176.329447547331));
#158151=CARTESIAN_POINT('Ctrl Pts',(59.3759867651245,-4.6661112882857,-176.321178317415));
#158152=CARTESIAN_POINT('Ctrl Pts',(59.3999226589537,-4.66635443958636,
-176.290106869232));
#158153=CARTESIAN_POINT('Ctrl Pts',(59.4233715104119,-4.66660144104085,
-176.258407507797));
#158154=CARTESIAN_POINT('Ctrl Pts',(59.4462880189083,-4.66685121140858,
-176.226103284235));
#158155=CARTESIAN_POINT('Ctrl Pts',(59.4577462731564,-4.66697609659244,
-176.209951172454));
#158156=CARTESIAN_POINT('Ctrl Pts',(59.4690714829495,-4.66710167269257,
-176.193647874009));
#158157=CARTESIAN_POINT('Ctrl Pts',(59.4802580714741,-4.6672277849629,-176.177196699382));
#158158=CARTESIAN_POINT('Ctrl Pts',(59.4858513657365,-4.66729084109807,
-176.168971112068));
#158159=CARTESIAN_POINT('Ctrl Pts',(59.4914100075004,-4.66735403118273,
-176.160708557756));
#158160=CARTESIAN_POINT('Ctrl Pts',(59.496933313017,-4.66741733507178,-176.152409467875));
#158161=CARTESIAN_POINT('Ctrl Pts',(59.4996949657753,-4.66744898701631,
-176.148259922935));
#158162=CARTESIAN_POINT('Ctrl Pts',(59.5024477846533,-4.66748066740648,
-176.144101244222));
#158163=CARTESIAN_POINT('Ctrl Pts',(59.5051916847113,-4.66751237365184,
-176.139933487251));
#158164=CARTESIAN_POINT('Ctrl Pts',(59.5076606481011,-4.66754090295588,
-176.136183336312));
#158165=CARTESIAN_POINT('Ctrl Pts',(59.5107552332661,-4.66757679218943,
-176.131455884057));
#158166=CARTESIAN_POINT('Ctrl Pts',(59.5127669604926,-4.66760023191263,
-176.128369384483));
#158167=CARTESIAN_POINT('Ctrl Pts',(59.5129909806557,-4.66760284209285,
-176.128025680759));
#158168=CARTESIAN_POINT('Ctrl Pts',(59.5132016187169,-4.66760529661482,
-176.127702354121));
#158169=CARTESIAN_POINT('Ctrl Pts',(59.5133965440667,-4.66760756732954,
-176.127403037814));
#158170=CARTESIAN_POINT('Ctrl Pts',(59.5371312287591,-4.6678840562422,-176.09095740269));
#158171=CARTESIAN_POINT('Ctrl Pts',(59.5613327018925,-4.66817509409086,
-176.052066438838));
#158172=CARTESIAN_POINT('Ctrl Pts',(59.5856916606812,-4.66848486559977,
-176.010634488638));
#158173=CARTESIAN_POINT('Ctrl Pts',(59.6095513371242,-4.66878828776317,
-175.970051763623));
#158174=CARTESIAN_POINT('Ctrl Pts',(59.6335618236263,-4.66910971421667,
-175.927030471272));
#158175=CARTESIAN_POINT('Ctrl Pts',(59.6573936723734,-4.66945172336169,
-175.881509967927));
#158176=CARTESIAN_POINT('Ctrl Pts',(59.6811736782573,-4.66979298851353,
-175.836088488089));
#158177=CARTESIAN_POINT('Ctrl Pts',(59.7047754709015,-4.67015478183408,
-175.788177887775));
#158178=CARTESIAN_POINT('Ctrl Pts',(59.7278372729539,-4.67053780712503,
-175.737758277064));
#158179=CARTESIAN_POINT('Ctrl Pts',(59.7508990750064,-4.67092083241598,
-175.687338666353));
#158180=CARTESIAN_POINT('Ctrl Pts',(59.773420321916,-4.67132512407299,-175.634409283462));
#158181=CARTESIAN_POINT('Ctrl Pts',(59.7950115476719,-4.6717490027353,-175.57900221117));
#158182=CARTESIAN_POINT('Ctrl Pts',(59.8094968549156,-4.67203337809809,
-175.541830237949));
#158183=CARTESIAN_POINT('Ctrl Pts',(59.8235629763428,-4.6723265191891,-175.503544172828));
#158184=CARTESIAN_POINT('Ctrl Pts',(59.8370875679768,-4.67262720060425,
-175.464169412071));
#158185=CARTESIAN_POINT('Ctrl Pts',(59.8438498637937,-4.67277754131183,
-175.444482031693));
#158186=CARTESIAN_POINT('Ctrl Pts',(59.8504767991258,-4.67292976676747,
-175.424522484744));
#158187=CARTESIAN_POINT('Ctrl Pts',(59.856952806083,-4.67308365370076,-175.404295481212));
#158188=CARTESIAN_POINT('Ctrl Pts',(59.8601908095616,-4.6731605971674,-175.394181979446));
#158189=CARTESIAN_POINT('Ctrl Pts',(59.863391084221,-4.67323795595347,-175.384001614636));
#158190=CARTESIAN_POINT('Ctrl Pts',(59.8665516908483,-4.67331569985915,
-175.37375502587));
#158191=CARTESIAN_POINT('Ctrl Pts',(59.868131994162,-4.67335457181198,-175.368631731487));
#158192=CARTESIAN_POINT('Ctrl Pts',(59.8697023806881,-4.67339354004155,
-175.363491881185));
#158193=CARTESIAN_POINT('Ctrl Pts',(59.8712626078616,-4.67343260052121,
-175.35833556037));
#158194=CARTESIAN_POINT('Ctrl Pts',(59.8720427214483,-4.67345213076104,
-175.355757399962));
#158195=CARTESIAN_POINT('Ctrl Pts',(59.8728202952122,-4.67347168406318,
-175.353175121931));
#158196=CARTESIAN_POINT('Ctrl Pts',(59.8735952988247,-4.67349125990757,
-175.350588737318));
#158197=CARTESIAN_POINT('Ctrl Pts',(59.8743703024372,-4.67351083575196,
-175.348002352706));
#158198=CARTESIAN_POINT('Ctrl Pts',(59.8747992527727,-4.67352167993367,
-175.346569510899));
#158199=CARTESIAN_POINT('Ctrl Pts',(59.8759125689141,-4.67355005454189,
-175.342817274903));
#158200=CARTESIAN_POINT('Ctrl Pts',(59.8902666875517,-4.67391589177132,
-175.294439245841));
#158201=CARTESIAN_POINT('Ctrl Pts',(59.9027576717863,-4.67427372815143,
-175.247880000389));
#158202=CARTESIAN_POINT('Ctrl Pts',(59.9136927181814,-4.67461859932685,
-175.203252216413));
#158203=CARTESIAN_POINT('Ctrl Pts',(59.9249587511274,-4.67497390920703,
-175.157273620035));
#158204=CARTESIAN_POINT('Ctrl Pts',(59.9345737413699,-4.6753154806694,-175.113344667922));
#158205=CARTESIAN_POINT('Ctrl Pts',(59.9428469848154,-4.67564005948804,
-175.071540483632));
#158206=CARTESIAN_POINT('Ctrl Pts',(59.9514972186274,-4.67597942852633,
-175.02783139048));
#158207=CARTESIAN_POINT('Ctrl Pts',(59.9586811510616,-4.67630024501819,
-174.986444595862));
#158208=CARTESIAN_POINT('Ctrl Pts',(59.9647154213307,-4.67660076426343,
-174.947422139622));
#158209=CARTESIAN_POINT('Ctrl Pts',(59.970910334806,-4.67690928387539,-174.907360834903));
#158210=CARTESIAN_POINT('Ctrl Pts',(59.9758938379629,-4.67719644344746,
-174.86979072386));
#158211=CARTESIAN_POINT('Ctrl Pts',(59.9799644784539,-4.67746194092389,
-174.834721935552));
#158212=CARTESIAN_POINT('Ctrl Pts',(59.9841355348749,-4.67773398778144,
-174.798788058567));
#158213=CARTESIAN_POINT('Ctrl Pts',(59.9873482802513,-4.67798332297327,
-174.765479724316));
#158214=CARTESIAN_POINT('Ctrl Pts',(59.9898750007537,-4.67821076220642,
-174.734782194308));
#158215=CARTESIAN_POINT('Ctrl Pts',(59.9924851917468,-4.67844571491974,
-174.703070568006));
#158216=CARTESIAN_POINT('Ctrl Pts',(59.9943634066945,-4.67865733157614,
-174.674144423609));
#158217=CARTESIAN_POINT('Ctrl Pts',(59.9957560933403,-4.67884722582315,
-174.647971186912));
#158218=CARTESIAN_POINT('Ctrl Pts',(59.9971686015776,-4.67903982276443,
-174.621425436262));
#158219=CARTESIAN_POINT('Ctrl Pts',(59.9980815614673,-4.67921010288986,
-174.597710889651));
#158220=CARTESIAN_POINT('Ctrl Pts',(59.9986978258392,-4.67936001600106,
-174.576787075096));
#158221=CARTESIAN_POINT('Ctrl Pts',(59.9993246130872,-4.67951248891803,
-174.555505980908));
#158222=CARTESIAN_POINT('Ctrl Pts',(59.9996443925775,-4.67964391657227,
-174.537111225911));
#158223=CARTESIAN_POINT('Ctrl Pts',(59.9998163358512,-4.67975622902168,
-174.521562257855));
#158224=CARTESIAN_POINT('Ctrl Pts',(59.9999609781594,-4.67985070862284,
-174.508482137991));
#158225=CARTESIAN_POINT('Ctrl Pts',(59.9999999999999,-4.67993166335616,
-174.49741579048));
#158226=CARTESIAN_POINT('Ctrl Pts',(60.,-4.68000001999999,-174.488343624884));
#158227=CARTESIAN_POINT('Ctrl Pts',(60.,-5.18000001999999,-174.511260182693));
#158228=CARTESIAN_POINT('Ctrl Pts',(60.,-5.01333573888012,-174.503547232447));
#158229=CARTESIAN_POINT('Ctrl Pts',(60.,-4.84666961885575,-174.495891400547));
#158230=CARTESIAN_POINT('Ctrl Pts',(60.,-4.68000001999999,-174.488343624884));
#158231=CARTESIAN_POINT('Origin',(39.,46.91999998,-129.34995));
#158232=CARTESIAN_POINT('',(39.,-11.8300000206964,-128.75511820843));
#158233=CARTESIAN_POINT('',(39.,-6.180000128392,-129.839693182379));
#158234=CARTESIAN_POINT('Ctrl Pts',(39.,-11.8300000219165,-128.755118230443));
#158235=CARTESIAN_POINT('Ctrl Pts',(39.,-11.2456383392948,-128.787506003178));
#158236=CARTESIAN_POINT('Ctrl Pts',(38.9999999999998,-10.6643296819649,
-128.844689763199));
#158237=CARTESIAN_POINT('Ctrl Pts',(39.0000000000002,-10.0859609278462,
-128.92574227051));
#158238=CARTESIAN_POINT('Ctrl Pts',(39.0000000000004,-9.71348092877341,
-128.977941559688));
#158239=CARTESIAN_POINT('Ctrl Pts',(39.0000000000007,-9.34222031417234,
-129.040041718412));
#158240=CARTESIAN_POINT('Ctrl Pts',(39.0000000000031,-8.97214920379055,
-129.111806478628));
#158241=CARTESIAN_POINT('Ctrl Pts',(39.0000000000039,-8.85321569986176,
-129.134870247055));
#158242=CARTESIAN_POINT('Ctrl Pts',(39.0000000000046,-8.73429069407208,
-129.1589539896));
#158243=CARTESIAN_POINT('Ctrl Pts',(39.0000000000049,-8.61535199981085,
-129.184060813321));
#158244=CARTESIAN_POINT('Ctrl Pts',(39.0000000000057,-8.31705980505462,
-129.247027450022));
#158245=CARTESIAN_POINT('Ctrl Pts',(39.0000000000046,-8.02087151391665,
-129.315956118525));
#158246=CARTESIAN_POINT('Ctrl Pts',(39.0000000000032,-7.72648278144565,
-129.39062643017));
#158247=CARTESIAN_POINT('Ctrl Pts',(39.0000000000018,-7.4202426468251,-129.468302793998));
#158248=CARTESIAN_POINT('Ctrl Pts',(39.0000000000006,-7.11594965101434,
-129.552192661459));
#158249=CARTESIAN_POINT('Ctrl Pts',(39.0000000000002,-6.81328756599089,
-129.642098960197));
#158250=CARTESIAN_POINT('Ctrl Pts',(39.,-6.60142553225938,-129.705032945782));
#158251=CARTESIAN_POINT('Ctrl Pts',(39.,-6.39036319103478,-129.770916038734));
#158252=CARTESIAN_POINT('Ctrl Pts',(39.,-6.18000018270164,-129.839693348042));
#158253=CARTESIAN_POINT('',(39.,-6.18000001999998,-102.218950121094));
#158254=CARTESIAN_POINT('',(39.,-6.18000001999998,-129.34995));
#158255=CARTESIAN_POINT('',(39.,-11.8300000202903,-103.303524781275));
#158256=CARTESIAN_POINT('Ctrl Pts',(39.0000000000558,-6.18000001999998,
-102.218950121094));
#158257=CARTESIAN_POINT('Ctrl Pts',(39.0000000001314,-6.52925246371981,
-102.333137272009));
#158258=CARTESIAN_POINT('Ctrl Pts',(39.0000000002528,-6.88066423663777,
-102.439420790159));
#158259=CARTESIAN_POINT('Ctrl Pts',(39.0000000003133,-7.23418430799431,
-102.537367117889));
#158260=CARTESIAN_POINT('Ctrl Pts',(39.0000000003723,-7.57920291835191,
-102.63295802947));
#158261=CARTESIAN_POINT('Ctrl Pts',(39.0000000003716,-7.92622968242249,
-102.720607819344));
#158262=CARTESIAN_POINT('Ctrl Pts',(39.0000000003073,-8.27519962485344,
-102.799960112761));
#158263=CARTESIAN_POINT('Ctrl Pts',(39.0000000002873,-8.38389527497297,
-102.824676422313));
#158264=CARTESIAN_POINT('Ctrl Pts',(39.0000000002619,-8.49277931386329,
-102.848588085812));
#158265=CARTESIAN_POINT('Ctrl Pts',(39.0000000002334,-8.60184941027751,
-102.871685311886));
#158266=CARTESIAN_POINT('Ctrl Pts',(39.0000000002017,-8.723199010669,-102.897382906795));
#158267=CARTESIAN_POINT('Ctrl Pts',(39.0000000001662,-8.84492476936504,
-102.922084618583));
#158268=CARTESIAN_POINT('Ctrl Pts',(39.0000000001318,-8.96688496783026,
-102.945759157014));
#158269=CARTESIAN_POINT('Ctrl Pts',(39.0000000000546,-9.24095711310763,
-102.998961198483));
#158270=CARTESIAN_POINT('Ctrl Pts',(39.0000000000303,-9.51689579309186,
-103.04710594614));
#158271=CARTESIAN_POINT('Ctrl Pts',(39.0000000000166,-9.7935384256358,-103.08982360864));
#158272=CARTESIAN_POINT('Ctrl Pts',(39.0000000000094,-9.93973590489214,
-103.112398634476));
#158273=CARTESIAN_POINT('Ctrl Pts',(39.0000000000059,-10.0861301614977,
-103.133457170461));
#158274=CARTESIAN_POINT('Ctrl Pts',(39.0000000000038,-10.2325489057379,
-103.152938666286));
#158275=CARTESIAN_POINT('Ctrl Pts',(38.9999999999998,-10.5104673644924,
-103.189916631927));
#158276=CARTESIAN_POINT('Ctrl Pts',(39.0000000000001,-10.7886085240243,
-103.221310636521));
#158277=CARTESIAN_POINT('Ctrl Pts',(39.,-11.0672887212858,-103.24709706551));
#158278=CARTESIAN_POINT('Ctrl Pts',(39.,-11.3209998818248,-103.270573096062));
#158279=CARTESIAN_POINT('Ctrl Pts',(39.,-11.5751577965224,-103.289400790235));
#158280=CARTESIAN_POINT('Ctrl Pts',(39.,-11.8300000206635,-103.303524774541));
#158281=CARTESIAN_POINT('',(39.,-11.83000002,-129.34995));
#158282=CARTESIAN_POINT('Ctrl Pts',(39.,-11.8686433059622,-128.75301285746));
#158283=CARTESIAN_POINT('Ctrl Pts',(39.,-11.928001403163,-129.861675775672));
#158284=CARTESIAN_POINT('Ctrl Pts',(39.4698940168252,-11.9817810974188,
-130.866147879494));
#158285=CARTESIAN_POINT('Ctrl Pts',(39.,-10.7823162329457,-128.811175087855));
#158286=CARTESIAN_POINT('Ctrl Pts',(39.,-10.9001869685749,-129.920171255555));
#158287=CARTESIAN_POINT('Ctrl Pts',(39.4726856154538,-11.0072350094688,
-130.924309912886));
#158288=CARTESIAN_POINT('Ctrl Pts',(39.,-9.69789923172707,-128.955540477711));
#158289=CARTESIAN_POINT('Ctrl Pts',(39.0000000000038,-9.87380661939344,
-130.065465765161));
#158290=CARTESIAN_POINT('Ctrl Pts',(39.4796201588693,-10.0340805400384,
-131.068675422521));
#158291=CARTESIAN_POINT('Ctrl Pts',(39.,-7.5328018765656,-129.41256745169));
#158292=CARTESIAN_POINT('Ctrl Pts',(38.9999999999961,-7.82478902027571,
-130.525032480762));
#158293=CARTESIAN_POINT('Ctrl Pts',(39.5013570517183,-8.08873720748368,
-131.525702236331));
#158294=CARTESIAN_POINT('Ctrl Pts',(39.,-6.48098994967646,-129.719043469502));
#158295=CARTESIAN_POINT('Ctrl Pts',(39.000000000015,-6.82874501931943,-130.833409195368));
#158296=CARTESIAN_POINT('Ctrl Pts',(39.5158567615765,-7.14247173527162,
-131.832173534627));
#158297=CARTESIAN_POINT('Ctrl Pts',(39.,-5.4610240206487,-130.086890037519));
#158298=CARTESIAN_POINT('Ctrl Pts',(39.,-5.86352497601848,-131.202945745636));
#158299=CARTESIAN_POINT('Ctrl Pts',(39.5330238402174,-6.22311741040379,
-132.200024593865));
#158300=CARTESIAN_POINT('',(39.5323905961839,-6.25584930016544,-132.186909003948));
#158301=CARTESIAN_POINT('',(39.4702993039609,-11.842906113671,-130.874975449521));
#158302=CARTESIAN_POINT('Ctrl Pts',(39.5323905962552,-6.25584930063541,
-132.186909005125));
#158303=CARTESIAN_POINT('Ctrl Pts',(39.523857640195,-6.71485178464417,-132.004109523071));
#158304=CARTESIAN_POINT('Ctrl Pts',(39.5161290340393,-7.17254264947844,
-131.839797338281));
#158305=CARTESIAN_POINT('Ctrl Pts',(39.5092514743187,-7.62950902695592,
-131.693972450754));
#158306=CARTESIAN_POINT('Ctrl Pts',(39.5058126944584,-7.85799221570156,
-131.621060006988));
#158307=CARTESIAN_POINT('Ctrl Pts',(39.5025859571867,-8.08629451480858,
-131.55276938753));
#158308=CARTESIAN_POINT('Ctrl Pts',(39.4995726887182,-8.31449060038593,
-131.489100581947));
#158309=CARTESIAN_POINT('Ctrl Pts',(39.498066054484,-8.42858864317462,-131.457266179156));
#158310=CARTESIAN_POINT('Ctrl Pts',(39.4966127484778,-8.54266013706068,
-131.426587248127));
#158311=CARTESIAN_POINT('Ctrl Pts',(39.4952126570643,-8.656714496533,-131.397063765538));
#158312=CARTESIAN_POINT('Ctrl Pts',(39.4945126113576,-8.71374167626916,
-131.382302024243));
#158313=CARTESIAN_POINT('Ctrl Pts',(39.4938258668266,-8.77076457270839,
-131.367829146221));
#158314=CARTESIAN_POINT('Ctrl Pts',(39.4931523927028,-8.82778436533119,
-131.353645131744));
#158315=CARTESIAN_POINT('Ctrl Pts',(39.492815655641,-8.85629426164259,-131.346553124506));
#158316=CARTESIAN_POINT('Ctrl Pts',(39.4924822360254,-8.88480338201596,
-131.339533333227));
#158317=CARTESIAN_POINT('Ctrl Pts',(39.4921521288706,-8.91331187415817,
-131.332585757904));
#158318=CARTESIAN_POINT('Ctrl Pts',(39.4918220217157,-8.94182036630037,
-131.325638182582));
#158319=CARTESIAN_POINT('Ctrl Pts',(39.4915087745014,-8.96913435998962,
-131.319047734368));
#158320=CARTESIAN_POINT('Ctrl Pts',(39.4911717391153,-8.99883561371038,
-131.311959679951));
#158321=CARTESIAN_POINT('Ctrl Pts',(39.4857791729374,-9.47405567324245,
-131.19855080929));
#158322=CARTESIAN_POINT('Ctrl Pts',(39.4813196690077,-9.94820234418142,
-131.105431021423));
#158323=CARTESIAN_POINT('Ctrl Pts',(39.4778365952643,-10.4219783954996,
-131.032600316352));
#158324=CARTESIAN_POINT('Ctrl Pts',(39.4743535215209,-10.8957544468178,
-130.95976961128));
#158325=CARTESIAN_POINT('Ctrl Pts',(39.4718469693993,-11.3691601359334,
-130.907227989003));
#158326=CARTESIAN_POINT('Ctrl Pts',(39.4702993039608,-11.842906113671,-130.874975449521));
#158327=CARTESIAN_POINT('Ctrl Pts',(39.5323905963862,-6.25584929916185,
-132.186909001152));
#158328=CARTESIAN_POINT('Ctrl Pts',(39.5179944370568,-6.25479880330938,
-132.156848952689));
#158329=CARTESIAN_POINT('Ctrl Pts',(39.5020197274459,-6.25361968902792,
-132.122785753625));
#158330=CARTESIAN_POINT('Ctrl Pts',(39.4847061343331,-6.2523014792109,-132.084599485537));
#158331=CARTESIAN_POINT('Ctrl Pts',(39.4684261104329,-6.25106196253827,
-132.048692822312));
#158332=CARTESIAN_POINT('Ctrl Pts',(39.450962599556,-6.24969928622832,-132.0091400591));
#158333=CARTESIAN_POINT('Ctrl Pts',(39.4325663511067,-6.24820853511762,
-131.965832371443));
#158334=CARTESIAN_POINT('Ctrl Pts',(39.4313984292324,-6.24811389186272,
-131.963082898044));
#158335=CARTESIAN_POINT('Ctrl Pts',(39.4302267652109,-6.24801873425826,
-131.960318288634));
#158336=CARTESIAN_POINT('Ctrl Pts',(39.4290514303077,-6.24792306186184,
-131.957538514917));
#158337=CARTESIAN_POINT('Ctrl Pts',(39.4108228025833,-6.2464392494667,-131.914426155958));
#158338=CARTESIAN_POINT('Ctrl Pts',(39.3917069600447,-6.24483093357756,
-131.867665934195));
#158339=CARTESIAN_POINT('Ctrl Pts',(39.3719967225372,-6.24310057463505,
-131.817153403871));
#158340=CARTESIAN_POINT('Ctrl Pts',(39.3704183573035,-6.24296201017607,
-131.813108438826));
#158341=CARTESIAN_POINT('Ctrl Pts',(39.3688362077372,-6.24282266780877,
-131.809039414516));
#158342=CARTESIAN_POINT('Ctrl Pts',(39.3672504385086,-6.24268255138138,
-131.804946279015));
#158343=CARTESIAN_POINT('Ctrl Pts',(39.3557827352194,-6.24166928060638,
-131.775346219556));
#158344=CARTESIAN_POINT('Ctrl Pts',(39.3439645144113,-6.24060098426729,
-131.744058170279));
#158345=CARTESIAN_POINT('Ctrl Pts',(39.3321251353788,-6.23950301199643,
-131.711747849603));
#158346=CARTESIAN_POINT('Ctrl Pts',(39.3218828342703,-6.23855315114849,
-131.683796042978));
#158347=CARTESIAN_POINT('Ctrl Pts',(39.3116243197905,-6.23758115645557,
-131.655079514983));
#158348=CARTESIAN_POINT('Ctrl Pts',(39.3015342098243,-6.23660444805766,
-131.626042903635));
#158349=CARTESIAN_POINT('Ctrl Pts',(39.280893042025,-6.23460641215916,-131.566643197469));
#158350=CARTESIAN_POINT('Ctrl Pts',(39.2624581975365,-6.23271275158796,
-131.510276774682));
#158351=CARTESIAN_POINT('Ctrl Pts',(39.245910507631,-6.23093757224289,-131.457104348278));
#158352=CARTESIAN_POINT('Ctrl Pts',(39.229157708339,-6.22914038946722,-131.403272847174));
#158353=CARTESIAN_POINT('Ctrl Pts',(39.2143386414709,-6.2274644078617,-131.352714546923));
#158354=CARTESIAN_POINT('Ctrl Pts',(39.2011526186406,-6.22591312153527,
-131.30555355468));
#158355=CARTESIAN_POINT('Ctrl Pts',(39.1877850185983,-6.22434047332816,
-131.257743135267));
#158356=CARTESIAN_POINT('Ctrl Pts',(39.1760953442301,-6.22289575183262,
-131.213423757931));
#158357=CARTESIAN_POINT('Ctrl Pts',(39.1658083189928,-6.22157474435082,
-131.172688346465));
#158358=CARTESIAN_POINT('Ctrl Pts',(39.164576028932,-6.22141649992618,-131.167808622589));
#158359=CARTESIAN_POINT('Ctrl Pts',(39.1633639148167,-6.22126002397052,
-131.162980290591));
#158360=CARTESIAN_POINT('Ctrl Pts',(39.162171543294,-6.22110530414493,-131.158203480778));
#158361=CARTESIAN_POINT('Ctrl Pts',(39.1570610239266,-6.22044217302339,
-131.137730013747));
#158362=CARTESIAN_POINT('Ctrl Pts',(39.1523129371346,-6.21981132039893,
-131.118203146671));
#158363=CARTESIAN_POINT('Ctrl Pts',(39.1478950036551,-6.21921161678299,
-131.09963198434));
#158364=CARTESIAN_POINT('Ctrl Pts',(39.1456860369154,-6.21891176497502,
-131.090346403175));
#158365=CARTESIAN_POINT('Ctrl Pts',(39.1435596592823,-6.21861969634864,
-131.081299736341));
#158366=CARTESIAN_POINT('Ctrl Pts',(39.1415121166505,-6.2183352522959,-131.072492943193));
#158367=CARTESIAN_POINT('Ctrl Pts',(39.1404883453346,-6.21819303026953,
-131.068089546618));
#158368=CARTESIAN_POINT('Ctrl Pts',(39.1394842859575,-6.21805271412436,
-131.063746117702));
#158369=CARTESIAN_POINT('Ctrl Pts',(39.1384994880882,-6.21791428326854,
-131.059462770329));
#158370=CARTESIAN_POINT('Ctrl Pts',(39.1380070891535,-6.21784506784063,
-131.057321096642));
#158371=CARTESIAN_POINT('Ctrl Pts',(39.137519505795,-6.21777632371958,-131.055194443296));
#158372=CARTESIAN_POINT('Ctrl Pts',(39.1370366828335,-6.21770804828387,
-131.053082823924));
#158373=CARTESIAN_POINT('Ctrl Pts',(39.1365538598719,-6.21763977284816,
-131.050971204551));
#158374=CARTESIAN_POINT('Ctrl Pts',(39.1364094970497,-6.21761943893419,
-131.050342030326));
#158375=CARTESIAN_POINT('Ctrl Pts',(39.1356024407393,-6.21750462536783,
-131.046793081091));
#158376=CARTESIAN_POINT('Ctrl Pts',(39.1150883146437,-6.21458624167215,
-130.956584267683));
#158377=CARTESIAN_POINT('Ctrl Pts',(39.0973860303671,-6.21172537375338,
-130.868122645569));
#158378=CARTESIAN_POINT('Ctrl Pts',(39.0821843947385,-6.20895207399527,
-130.781623452936));
#158379=CARTESIAN_POINT('Ctrl Pts',(39.0664755042733,-6.20608623355601,
-130.692237917354));
#158380=CARTESIAN_POINT('Ctrl Pts',(39.0534363138107,-6.20331381068036,
-130.604947964263));
#158381=CARTESIAN_POINT('Ctrl Pts',(39.0427217194077,-6.20064908714807,
-130.519937966199));
#158382=CARTESIAN_POINT('Ctrl Pts',(39.0318057827407,-6.19793428972137,
-130.433330510982));
#158383=CARTESIAN_POINT('Ctrl Pts',(39.0233020474348,-6.19533110598602,
-130.349089264251));
#158384=CARTESIAN_POINT('Ctrl Pts',(39.0168531430717,-6.19283746461102,
-130.267356945417));
#158385=CARTESIAN_POINT('Ctrl Pts',(39.0101961559517,-6.19026336247201,
-130.182987421057));
#158386=CARTESIAN_POINT('Ctrl Pts',(39.0057281795345,-6.18780581569125,
-130.10129110459));
#158387=CARTESIAN_POINT('Ctrl Pts',(39.0030730286528,-6.18544701429272,
-130.022373375295));
#158388=CARTESIAN_POINT('Ctrl Pts',(39.0009650480001,-6.18357431178611,
-129.959718914618));
#158389=CARTESIAN_POINT('Ctrl Pts',(39.0000000000003,-6.18176350020245,
-129.898814707424));
#158390=CARTESIAN_POINT('Ctrl Pts',(39.,-6.18000018270164,-129.839693348042));
#158391=CARTESIAN_POINT('Origin',(46.4017469067786,-11.845764450772,-128.222607383819));
#158392=CARTESIAN_POINT('Origin',(0.,-12.9675000200281,-171.64995));
#158393=CARTESIAN_POINT('',(58.3953999019963,-11.8387575339013,-171.449026400902));
#158394=CARTESIAN_POINT('',(58.0166638356104,-6.23225639415715,-171.449026400902));
#158395=CARTESIAN_POINT('Origin',(0.,-12.9675000200281,-171.449026400902));
#158396=CARTESIAN_POINT('Ctrl Pts',(58.0166638356104,-6.23225639415715,
-171.449026400902));
#158397=CARTESIAN_POINT('Ctrl Pts',(56.349577545528,-6.23372673672702,-167.897434994591));
#158398=CARTESIAN_POINT('Ctrl Pts',(54.7469618912178,-6.23517242645505,
-164.485193986989));
#158399=CARTESIAN_POINT('Ctrl Pts',(52.439761917831,-6.23757483085028,-159.575858073651));
#158400=CARTESIAN_POINT('Ctrl Pts',(51.686815584278,-6.23840909492504,-157.974250368882));
#158401=CARTESIAN_POINT('Ctrl Pts',(50.5815758482561,-6.23969494579187,
-155.624095211246));
#158402=CARTESIAN_POINT('Ctrl Pts',(50.0350008862545,-6.24034596867499,
-154.462081732306));
#158403=CARTESIAN_POINT('Ctrl Pts',(49.4079081179195,-6.24111077357991,
-153.129261514999));
#158404=CARTESIAN_POINT('Ctrl Pts',(49.0553674761703,-6.24154416602389,
-152.380081070807));
#158405=CARTESIAN_POINT('Ctrl Pts',(48.8814612455038,-6.24175878610164,
-152.010550217392));
#158406=CARTESIAN_POINT('Ctrl Pts',(48.7933718888155,-6.24186763099907,
-151.823379333081));
#158407=CARTESIAN_POINT('Ctrl Pts',(48.7911832326025,-6.24187033541698,
-151.818728915993));
#158408=CARTESIAN_POINT('Ctrl Pts',(45.3920876839696,-6.24607063796648,
-144.596406262261));
#158409=CARTESIAN_POINT('Ctrl Pts',(42.3069257173847,-6.25073126772922,
-138.054815014792));
#158410=CARTESIAN_POINT('Ctrl Pts',(39.532390596256,-6.25584930059378,-132.186909005141));
#158411=CARTESIAN_POINT('Ctrl Pts',(39.4702993039609,-11.842906113671,-130.874975449521));
#158412=CARTESIAN_POINT('Ctrl Pts',(41.7583572470671,-11.8421670407155,
-135.779786235607));
#158413=CARTESIAN_POINT('Ctrl Pts',(44.2894937407195,-11.8414658913629,
-141.205977562808));
#158414=CARTESIAN_POINT('Ctrl Pts',(47.0636808807324,-11.8408304355432,
-147.153562779003));
#158415=CARTESIAN_POINT('Ctrl Pts',(49.4731957341661,-11.840278511625,-152.319326369276));
#158416=CARTESIAN_POINT('Ctrl Pts',(52.0660617843129,-11.8397764603368,
-157.878417006278));
#158417=CARTESIAN_POINT('Ctrl Pts',(54.8422877286471,-11.8393150124165,
-163.830830224675));
#158418=CARTESIAN_POINT('Ctrl Pts',(55.995043971226,-11.8391234080653,-166.302416339601));
#158419=CARTESIAN_POINT('Ctrl Pts',(57.1794138783212,-11.8389384233643,
-168.841815469919));
#158420=CARTESIAN_POINT('Ctrl Pts',(58.3953999019963,-11.8387575339013,
-171.449026400902));
#158421=CARTESIAN_POINT('Ctrl Pts',(60.,-12.8269998197496,-174.751773822184));
#158422=CARTESIAN_POINT('Ctrl Pts',(60.,-12.8247546893956,-176.329633102893));
#158423=CARTESIAN_POINT('Ctrl Pts',(58.6998841333603,-12.8234825355735,
-177.223692421544));
#158424=CARTESIAN_POINT('Ctrl Pts',(60.,-12.9956778161511,-174.752013833507));
#158425=CARTESIAN_POINT('Ctrl Pts',(59.9999999999984,-12.9961202462228,
-176.329584396716));
#158426=CARTESIAN_POINT('Ctrl Pts',(58.7002617769476,-12.996381211483,-177.22367874123));
#158427=CARTESIAN_POINT('Ctrl Pts',(60.,-13.1643444677208,-174.751821305086));
#158428=CARTESIAN_POINT('Ctrl Pts',(60.,-13.16751068744,-176.329623133207));
#158429=CARTESIAN_POINT('Ctrl Pts',(58.6999592969537,-13.1692782682892,
-177.223689661345));
#158430=CARTESIAN_POINT('Ctrl Pts',(60.,-13.3329998199577,-174.75119758399));
#158431=CARTESIAN_POINT('Ctrl Pts',(60.,-13.338837622507,-176.329750343386));
#158432=CARTESIAN_POINT('Ctrl Pts',(58.6989770498873,-13.3421437200247,
-177.22372531347));
#158433=CARTESIAN_POINT('',(60.,-13.33000002,-174.751208632418));
#158434=CARTESIAN_POINT('',(58.7133156820334,-13.3314748988427,-177.213850299147));
#158435=CARTESIAN_POINT('Ctrl Pts',(60.,-13.33000002,-174.751208632418));
#158436=CARTESIAN_POINT('Ctrl Pts',(60.,-13.3300406632064,-174.817693892478));
#158437=CARTESIAN_POINT('Ctrl Pts',(59.9978175504489,-13.3300830974903,
-174.883676399972));
#158438=CARTESIAN_POINT('Ctrl Pts',(59.9935259312227,-13.33012663432,-174.948960491235));
#158439=CARTESIAN_POINT('Ctrl Pts',(59.9891899816022,-13.3301706208645,
-175.014918936243));
#158440=CARTESIAN_POINT('Ctrl Pts',(59.9827011519673,-13.3302157328684,
-175.080164469868));
#158441=CARTESIAN_POINT('Ctrl Pts',(59.9741881323204,-13.3302612676316,
-175.144504391241));
#158442=CARTESIAN_POINT('Ctrl Pts',(59.965483642566,-13.3303078265375,-175.210291410374));
#158443=CARTESIAN_POINT('Ctrl Pts',(59.9546629379879,-13.3303548274467,
-175.275131623486));
#158444=CARTESIAN_POINT('Ctrl Pts',(59.9419179227273,-13.3304015266371,
-175.338828443807));
#158445=CARTESIAN_POINT('Ctrl Pts',(59.9330492512272,-13.3304340224615,
-175.383152139265));
#158446=CARTESIAN_POINT('Ctrl Pts',(59.9232499582355,-13.3304663723483,
-175.426922389111));
#158447=CARTESIAN_POINT('Ctrl Pts',(59.9125992990762,-13.3304983276908,
-175.470075512945));
#158448=CARTESIAN_POINT('Ctrl Pts',(59.8981332593431,-13.3305417303804,
-175.528687359843));
#158449=CARTESIAN_POINT('Ctrl Pts',(59.8820111888294,-13.3305844310845,
-175.586206570858));
#158450=CARTESIAN_POINT('Ctrl Pts',(59.864531922907,-13.3306256977267,-175.642287543161));
#158451=CARTESIAN_POINT('Ctrl Pts',(59.8603213155855,-13.3306356385117,
-175.655796975057));
#158452=CARTESIAN_POINT('Ctrl Pts',(59.856032061966,-13.3306454962089,-175.66922315738));
#158453=CARTESIAN_POINT('Ctrl Pts',(59.8516685359687,-13.3306552608383,
-175.682561672477));
#158454=CARTESIAN_POINT('Ctrl Pts',(59.8315974156507,-13.3307001756736,
-175.743915481654));
#158455=CARTESIAN_POINT('Ctrl Pts',(59.8098453629079,-13.3307433634398,
-175.803746308069));
#158456=CARTESIAN_POINT('Ctrl Pts',(59.7867216622384,-13.3307845551397,
-175.861801089472));
#158457=CARTESIAN_POINT('Ctrl Pts',(59.7637846813986,-13.3308254142239,
-175.919387088692));
#158458=CARTESIAN_POINT('Ctrl Pts',(59.7394982842042,-13.3308643093334,
-175.975225576071));
#158459=CARTESIAN_POINT('Ctrl Pts',(59.7141598494433,-13.3309010082065,
-176.029120623913));
#158460=CARTESIAN_POINT('Ctrl Pts',(59.6948604672771,-13.3309289604295,
-176.070170559908));
#158461=CARTESIAN_POINT('Ctrl Pts',(59.6749506878815,-13.3309556391615,
-176.110094083364));
#158462=CARTESIAN_POINT('Ctrl Pts',(59.6545592887383,-13.3309809536881,
-176.148824764904));
#158463=CARTESIAN_POINT('Ctrl Pts',(59.6248502631807,-13.3310178354102,
-176.205253007011));
#158464=CARTESIAN_POINT('Ctrl Pts',(59.5939431737811,-13.3310520515032,
-176.259532914652));
#158465=CARTESIAN_POINT('Ctrl Pts',(59.5622506861511,-13.3310833724742,
-176.31154208023));
#158466=CARTESIAN_POINT('Ctrl Pts',(59.5406769550353,-13.3311046933062,
-176.34694579378));
#158467=CARTESIAN_POINT('Ctrl Pts',(59.5187390405221,-13.3311246732112,
-176.381298364634));
#158468=CARTESIAN_POINT('Ctrl Pts',(59.4965632307964,-13.3311432473675,
-176.414574433984));
#158469=CARTESIAN_POINT('Ctrl Pts',(59.4634357414712,-13.3311709945014,
-176.464284124219));
#158470=CARTESIAN_POINT('Ctrl Pts',(59.4297640859701,-13.3311957856679,
-176.511615559249));
#158471=CARTESIAN_POINT('Ctrl Pts',(59.3958538673844,-13.3312180275919,
-176.556637376878));
#158472=CARTESIAN_POINT('Ctrl Pts',(59.3604749618748,-13.3312412328368,
-176.60360913637));
#158473=CARTESIAN_POINT('Ctrl Pts',(59.3248363486428,-13.3312616634009,
-176.648067167108));
#158474=CARTESIAN_POINT('Ctrl Pts',(59.2892362542711,-13.3312797965956,
-176.690119079622));
#158475=CARTESIAN_POINT('Ctrl Pts',(59.2732699473442,-13.3312879291625,
-176.708978966201));
#158476=CARTESIAN_POINT('Ctrl Pts',(59.2573107554705,-13.3312955998131,
-176.727355236389));
#158477=CARTESIAN_POINT('Ctrl Pts',(59.2413826308639,-13.3313028524118,
-176.74525917353));
#158478=CARTESIAN_POINT('Ctrl Pts',(59.1984116798147,-13.3313224184983,
-176.79356047864));
#158479=CARTESIAN_POINT('Ctrl Pts',(59.1558409640565,-13.3313388818287,
-176.83831965251));
#158480=CARTESIAN_POINT('Ctrl Pts',(59.1139642014224,-13.3313532051975,
-176.879933610363));
#158481=CARTESIAN_POINT('Ctrl Pts',(59.1028928301105,-13.3313569920074,
-176.890935501393));
#158482=CARTESIAN_POINT('Ctrl Pts',(59.0918697733653,-13.3313606290969,
-176.901717342555));
#158483=CARTESIAN_POINT('Ctrl Pts',(59.0809000521733,-13.3313641339516,
-176.91228602047));
#158484=CARTESIAN_POINT('Ctrl Pts',(59.037658448174,-13.3313779497574,-176.953946749782));
#158485=CARTESIAN_POINT('Ctrl Pts',(58.9953543728595,-13.3313897838346,
-176.992195992816));
#158486=CARTESIAN_POINT('Ctrl Pts',(58.9543294737028,-13.3314009374072,
-177.027413076148));
#158487=CARTESIAN_POINT('Ctrl Pts',(58.9133506411377,-13.3314120784555,
-177.062590614446));
#158488=CARTESIAN_POINT('Ctrl Pts',(58.8736481149678,-13.3314225404819,
-177.094742812638));
#158489=CARTESIAN_POINT('Ctrl Pts',(58.8355275097074,-13.3314335944421,
-177.12420916681));
#158490=CARTESIAN_POINT('Ctrl Pts',(58.7974621106597,-13.331444632394,-177.153632847846));
#158491=CARTESIAN_POINT('Ctrl Pts',(58.7609740532324,-13.3314562605222,
-177.18037846857));
#158492=CARTESIAN_POINT('Ctrl Pts',(58.7263328221663,-13.331469719106,-177.204745412345));
#158493=CARTESIAN_POINT('Ctrl Pts',(58.7219643842158,-13.3314714163028,
-177.207818209663));
#158494=CARTESIAN_POINT('Ctrl Pts',(58.7176252699974,-13.3314731425762,
-177.210853129469));
#158495=CARTESIAN_POINT('Ctrl Pts',(58.7133159805679,-13.3314749003853,
-177.213850728308));
#158496=CARTESIAN_POINT('',(58.7141461350309,-12.8294402383603,-177.213832217122));
#158497=CARTESIAN_POINT('Origin',(-9.53286718169884,-12.9674995361125,-178.689058801762));
#158498=CARTESIAN_POINT('',(60.,-12.83000002,-174.751778045593));
#158499=CARTESIAN_POINT('Ctrl Pts',(58.7141461350221,-12.8294402383603,
-177.213832217103));
#158500=CARTESIAN_POINT('Ctrl Pts',(58.7755886331233,-12.8294220721977,
-177.171054260417));
#158501=CARTESIAN_POINT('Ctrl Pts',(58.8359427968261,-12.8294076339433,
-177.125614758351));
#158502=CARTESIAN_POINT('Ctrl Pts',(58.8948831125148,-12.8293968304697,
-177.077594979963));
#158503=CARTESIAN_POINT('Ctrl Pts',(58.9533625385092,-12.8293861114749,
-177.029950697036));
#158504=CARTESIAN_POINT('Ctrl Pts',(59.0104494931047,-12.8293789706229,
-176.979766371684));
#158505=CARTESIAN_POINT('Ctrl Pts',(59.0658331174558,-12.8293752468593,
-176.927171986301));
#158506=CARTESIAN_POINT('Ctrl Pts',(59.120872654405,-12.8293715462306,-176.874904359335));
#158507=CARTESIAN_POINT('Ctrl Pts',(59.174229327996,-12.8293712201624,-176.820256697794));
#158508=CARTESIAN_POINT('Ctrl Pts',(59.2256146190754,-12.8293740426676,
-176.763405201032));
#158509=CARTESIAN_POINT('Ctrl Pts',(59.2767636605023,-12.829376852196,-176.706815085418));
#158510=CARTESIAN_POINT('Ctrl Pts',(59.3259588177311,-12.8293827810321,
-176.648041653612));
#158511=CARTESIAN_POINT('Ctrl Pts',(59.3729411440154,-12.8293915431069,
-176.587303496293));
#158512=CARTESIAN_POINT('Ctrl Pts',(59.4197836406822,-12.8294002791039,
-176.526746108936));
#158513=CARTESIAN_POINT('Ctrl Pts',(59.464425943485,-12.829411830954,-176.464236091621));
#158514=CARTESIAN_POINT('Ctrl Pts',(59.5066452026437,-12.8294258590997,
-176.400029364887));
#158515=CARTESIAN_POINT('Ctrl Pts',(59.5488389306529,-12.8294398787623,
-176.335861465731));
#158516=CARTESIAN_POINT('Ctrl Pts',(59.5886121199466,-12.8294563710419,
-176.269999423512));
#158517=CARTESIAN_POINT('Ctrl Pts',(59.6257832108178,-12.8294749501596,
-176.202730993732));
#158518=CARTESIAN_POINT('Ctrl Pts',(59.6629837603696,-12.8294935440016,
-176.135409252651));
#158519=CARTESIAN_POINT('Ctrl Pts',(59.6975777773869,-12.8295142271887,
-176.066679489299));
#158520=CARTESIAN_POINT('Ctrl Pts',(59.7294297692503,-12.8295365772786,
-175.996854153079));
#158521=CARTESIAN_POINT('Ctrl Pts',(59.7613529583115,-12.8295589773266,
-175.926872739705));
#158522=CARTESIAN_POINT('Ctrl Pts',(59.7905216739406,-12.8295830508558,
-175.855791497974));
#158523=CARTESIAN_POINT('Ctrl Pts',(59.8168498754468,-12.8296083493863,
-175.783939712998));
#158524=CARTESIAN_POINT('Ctrl Pts',(59.843274872218,-12.8296337409265,-175.711823765938));
#158525=CARTESIAN_POINT('Ctrl Pts',(59.8668383938283,-12.8296603655722,
-175.638932268924));
#158526=CARTESIAN_POINT('Ctrl Pts',(59.8875057522723,-12.8296877601467,
-175.565603027702));
#158527=CARTESIAN_POINT('Ctrl Pts',(59.908361509043,-12.829715404443,-175.491605335967));
#158528=CARTESIAN_POINT('Ctrl Pts',(59.926268131564,-12.8297438318391,-175.417162555197));
#158529=CARTESIAN_POINT('Ctrl Pts',(59.9412429556759,-12.8297725705227,
-175.342616582038));
#158530=CARTESIAN_POINT('Ctrl Pts',(59.9563048455964,-12.8298014762971,
-175.267637187735));
#158531=CARTESIAN_POINT('Ctrl Pts',(59.9684009949618,-12.8298306961103,
-175.192554025529));
#158532=CARTESIAN_POINT('Ctrl Pts',(59.9775999311467,-12.8298597677861,
-175.117699848986));
#158533=CARTESIAN_POINT('Ctrl Pts',(59.986908142556,-12.8298891848077,-175.041956471043));
#158534=CARTESIAN_POINT('Ctrl Pts',(59.9932502385466,-12.8299184493296,
-174.966448134161));
#158535=CARTESIAN_POINT('Ctrl Pts',(59.9967447710968,-12.8299471137923,
-174.891494881111));
#158536=CARTESIAN_POINT('Ctrl Pts',(59.9989272876026,-12.8299650162334,
-174.844682693903));
#158537=CARTESIAN_POINT('Ctrl Pts',(59.9999999999993,-12.8299826852913,
-174.798086493521));
#158538=CARTESIAN_POINT('Ctrl Pts',(60.,-12.83000002,-174.751778045593));
#158539=CARTESIAN_POINT('Origin',(60.,-12.9674774176428,-75.9457339865586));
#158540=CARTESIAN_POINT('Origin',(39.,46.91999998,-129.34995));
#158541=CARTESIAN_POINT('',(39.,-19.98000002,-129.914446011788));
#158542=CARTESIAN_POINT('',(39.,-14.3300000196436,-128.768820403088));
#158543=CARTESIAN_POINT('Ctrl Pts',(39.0000000000669,-19.98000002,-129.914446011788));
#158544=CARTESIAN_POINT('Ctrl Pts',(39.0000000001518,-19.6367327840738,
-129.798586081307));
#158545=CARTESIAN_POINT('Ctrl Pts',(39.0000000002631,-19.2913217887197,
-129.690298412948));
#158546=CARTESIAN_POINT('Ctrl Pts',(39.0000000003003,-18.9438276300884,
-129.590011167479));
#158547=CARTESIAN_POINT('Ctrl Pts',(39.0000000003366,-18.6049646905776,
-129.49221490256));
#158548=CARTESIAN_POINT('Ctrl Pts',(39.0000000003094,-18.2641207496953,
-129.402026657412));
#158549=CARTESIAN_POINT('Ctrl Pts',(39.0000000002472,-17.9213701519525,
-129.31979718069));
#158550=CARTESIAN_POINT('Ctrl Pts',(39.0000000002263,-17.8056205246018,
-129.292027626528));
#158551=CARTESIAN_POINT('Ctrl Pts',(39.0000000002019,-17.6896536077095,
-129.265165339738));
#158552=CARTESIAN_POINT('Ctrl Pts',(39.0000000001767,-17.5734727602674,
-129.239222565105));
#158553=CARTESIAN_POINT('Ctrl Pts',(39.0000000001494,-17.4477751466172,
-129.211154730048));
#158554=CARTESIAN_POINT('Ctrl Pts',(39.0000000001211,-17.3216708975945,
-129.184146383705));
#158555=CARTESIAN_POINT('Ctrl Pts',(39.0000000000953,-17.1952995452482,
-129.158233426905));
#158556=CARTESIAN_POINT('Ctrl Pts',(39.0000000000407,-16.9274823440487,
-129.103316426838));
#158557=CARTESIAN_POINT('Ctrl Pts',(39.0000000000228,-16.6579107580334,
-129.053205467123));
#158558=CARTESIAN_POINT('Ctrl Pts',(39.0000000000127,-16.3874479062833,
-129.008231038422));
#158559=CARTESIAN_POINT('Ctrl Pts',(39.0000000000071,-16.2374573286264,
-128.983289570501));
#158560=CARTESIAN_POINT('Ctrl Pts',(39.0000000000044,-16.0871922946708,
-128.959928670237));
#158561=CARTESIAN_POINT('Ctrl Pts',(39.0000000000028,-15.9367995435377,
-128.938211682847));
#158562=CARTESIAN_POINT('Ctrl Pts',(39.,-15.6676875947363,-128.899351426921));
#158563=CARTESIAN_POINT('Ctrl Pts',(39.0000000000001,-15.3983918170305,
-128.865722188253));
#158564=CARTESIAN_POINT('Ctrl Pts',(39.,-15.1285853320425,-128.837337411665));
#158565=CARTESIAN_POINT('Ctrl Pts',(39.,-14.8629886325448,-128.809395522211));
#158566=CARTESIAN_POINT('Ctrl Pts',(39.,-14.5968970408721,-128.786535808696));
#158567=CARTESIAN_POINT('Ctrl Pts',(39.,-14.3300000191853,-128.768820409992));
#158568=CARTESIAN_POINT('',(39.0000000000001,-14.330000015482,-103.28982244638));
#158569=CARTESIAN_POINT('',(39.,-14.33000002,-129.34995));
#158570=CARTESIAN_POINT('',(39.,-19.9800000199999,-102.144196959718));
#158571=CARTESIAN_POINT('Ctrl Pts',(39.,-14.3300000071456,-103.289822320808));
#158572=CARTESIAN_POINT('Ctrl Pts',(39.,-14.6503224302969,-103.268556852662));
#158573=CARTESIAN_POINT('Ctrl Pts',(38.9999999999999,-14.9696787697451,
-103.239819970848));
#158574=CARTESIAN_POINT('Ctrl Pts',(39.0000000000001,-15.2880843675587,
-103.203826801699));
#158575=CARTESIAN_POINT('Ctrl Pts',(39.0000000000004,-15.6115732353083,
-103.167259010131));
#158576=CARTESIAN_POINT('Ctrl Pts',(38.9999999999999,-15.9340810135561,
-103.123201376371));
#158577=CARTESIAN_POINT('Ctrl Pts',(39.0000000000089,-16.2556315657715,
-103.071825704718));
#158578=CARTESIAN_POINT('Ctrl Pts',(39.0000000000177,-16.5680888803951,
-103.021902903184));
#158579=CARTESIAN_POINT('Ctrl Pts',(39.0000000000333,-16.8796426042176,
-102.965069752024));
#158580=CARTESIAN_POINT('Ctrl Pts',(39.000000000099,-17.1903180517835,-102.90143687879));
#158581=CARTESIAN_POINT('Ctrl Pts',(39.0000000001251,-17.3140185734884,
-102.87610040731));
#158582=CARTESIAN_POINT('Ctrl Pts',(39.0000000001567,-17.4376802476524,
-102.849665441423));
#158583=CARTESIAN_POINT('Ctrl Pts',(39.0000000001917,-17.5613085289994,
-102.822130971399));
#158584=CARTESIAN_POINT('Ctrl Pts',(39.000000000283,-17.8840119032272,-102.750258530179));
#158585=CARTESIAN_POINT('Ctrl Pts',(39.0000000004,-18.2040368478246,-102.671531783398));
#158586=CARTESIAN_POINT('Ctrl Pts',(39.0000000004561,-18.5218724866243,
-102.586181685713));
#158587=CARTESIAN_POINT('Ctrl Pts',(39.0000000005153,-18.8564962428645,
-102.496323385396));
#158588=CARTESIAN_POINT('Ctrl Pts',(39.0000000004874,-19.1886932216449,
-102.399123389358));
#158589=CARTESIAN_POINT('Ctrl Pts',(39.0000000003521,-19.5190105422359,
-102.294797669285));
#158590=CARTESIAN_POINT('Ctrl Pts',(39.000000000289,-19.6730648764638,-102.246141942362));
#158591=CARTESIAN_POINT('Ctrl Pts',(39.0000000002054,-19.8267100435463,
-102.195935559143));
#158592=CARTESIAN_POINT('Ctrl Pts',(39.000000000131,-19.98000002,-102.144196959718));
#158593=CARTESIAN_POINT('',(39.,-19.98000002,-129.34995));
#158594=CARTESIAN_POINT('Ctrl Pts',(39.,-20.720937818584,-130.177378160746));
#158595=CARTESIAN_POINT('Ctrl Pts',(39.,-20.3054116348924,-131.293905860767));
#158596=CARTESIAN_POINT('Ctrl Pts',(39.5372195035444,-19.9345312052232,
-132.290469469449));
#158597=CARTESIAN_POINT('Ctrl Pts',(39.,-19.698133940161,-129.796732169428));
#158598=CARTESIAN_POINT('Ctrl Pts',(39.,-19.3374585219745,-130.911526747764));
#158599=CARTESIAN_POINT('Ctrl Pts',(39.5194895810462,-19.0123420478084,
-131.90982316175));
#158600=CARTESIAN_POINT('Ctrl Pts',(39.,-18.6506584423116,-129.479682762144));
#158601=CARTESIAN_POINT('Ctrl Pts',(38.9999999999923,-18.3454434179522,
-130.592508390753));
#158602=CARTESIAN_POINT('Ctrl Pts',(39.5045124277029,-18.0697294738066,
-131.592774070923));
#158603=CARTESIAN_POINT('Ctrl Pts',(39.,-17.0348936577371,-129.118930933505));
#158604=CARTESIAN_POINT('Ctrl Pts',(39.0000000000038,-16.8157658206047,
-130.229644160077));
#158605=CARTESIAN_POINT('Ctrl Pts',(39.4873751859149,-16.6176732464254,
-131.23202224217));
#158606=CARTESIAN_POINT('Ctrl Pts',(39.,-16.4860091127214,-129.017507601134));
#158607=CARTESIAN_POINT('Ctrl Pts',(39.,-16.2963199259075,-130.127635847669));
#158608=CARTESIAN_POINT('Ctrl Pts',(39.4825356614912,-16.1247177152636,
-131.130598909837));
#158609=CARTESIAN_POINT('Ctrl Pts',(39.,-15.3875914977103,-128.858905214396));
#158610=CARTESIAN_POINT('Ctrl Pts',(39.,-15.2570331695429,-129.96814976082));
#158611=CARTESIAN_POINT('Ctrl Pts',(39.4749533438571,-15.1386572025492,
-130.9719965231));
#158612=CARTESIAN_POINT('Ctrl Pts',(39.,-14.8389953875779,-128.801602009569));
#158613=CARTESIAN_POINT('Ctrl Pts',(38.9999999999999,-14.7379707288414,
-129.910514022628));
#158614=CARTESIAN_POINT('Ctrl Pts',(39.4722050319315,-14.6463890166082,
-130.914693311714));
#158615=CARTESIAN_POINT('Ctrl Pts',(39.,-14.2910120087967,-128.766269567481));
#158616=CARTESIAN_POINT('Ctrl Pts',(39.,-14.2195253716732,-129.874981182379));
#158617=CARTESIAN_POINT('Ctrl Pts',(39.4705097325996,-14.1547657662532,
-130.879360876185));
#158618=CARTESIAN_POINT('',(39.4710976354407,-14.3145440749074,-130.891615496825));
#158619=CARTESIAN_POINT('',(39.5365899598451,-19.9017174806626,-132.276955615329));
#158620=CARTESIAN_POINT('Ctrl Pts',(39.4710975927162,-14.3145440734493,
-130.89161551676));
#158621=CARTESIAN_POINT('Ctrl Pts',(39.471847193384,-14.5062549022323,-130.907244870022));
#158622=CARTESIAN_POINT('Ctrl Pts',(39.4727537671787,-14.6975339673999,
-130.926164753854));
#158623=CARTESIAN_POINT('Ctrl Pts',(39.4738171268208,-14.888760940223,-130.948378536857));
#158624=CARTESIAN_POINT('Ctrl Pts',(39.474880959685,-15.0800730138931,-130.970602205556));
#158625=CARTESIAN_POINT('Ctrl Pts',(39.4761017195622,-15.2713329311122,
-130.996122712195));
#158626=CARTESIAN_POINT('Ctrl Pts',(39.4774817130348,-15.4629223698792,
-131.024995466283));
#158627=CARTESIAN_POINT('Ctrl Pts',(39.477886687669,-15.5191464494941,-131.033468501305));
#158628=CARTESIAN_POINT('Ctrl Pts',(39.4783053917035,-15.5753989181463,
-131.042230571371));
#158629=CARTESIAN_POINT('Ctrl Pts',(39.4787379239733,-15.6316894498703,
-131.051283927837));
#158630=CARTESIAN_POINT('Ctrl Pts',(39.4802253119557,-15.8252608114915,
-131.082416526602));
#158631=CARTESIAN_POINT('Ctrl Pts',(39.4818769063609,-16.0191549692742,
-131.117009241646));
#158632=CARTESIAN_POINT('Ctrl Pts',(39.4836882348007,-16.2132119285899,
-131.15498469469));
#158633=CARTESIAN_POINT('Ctrl Pts',(39.4854164288744,-16.3983622744101,
-131.191217192038));
#158634=CARTESIAN_POINT('Ctrl Pts',(39.4872900662569,-16.5836618542002,
-131.230529742924));
#158635=CARTESIAN_POINT('Ctrl Pts',(39.4893069555753,-16.7689438009247,
-131.272891706083));
#158636=CARTESIAN_POINT('Ctrl Pts',(39.4905145726718,-16.8798817906742,
-131.298256028499));
#158637=CARTESIAN_POINT('Ctrl Pts',(39.4917735763949,-16.9908128539619,
-131.324714234321));
#158638=CARTESIAN_POINT('Ctrl Pts',(39.4930837333765,-17.1016937426839,
-131.3522649967));
#158639=CARTESIAN_POINT('Ctrl Pts',(39.4933071500142,-17.1206018855207,
-131.356963135003));
#158640=CARTESIAN_POINT('Ctrl Pts',(39.4935320777091,-17.1395124913016,
-131.361693525097));
#158641=CARTESIAN_POINT('Ctrl Pts',(39.4937585203661,-17.1584259087636,
-131.366456272776));
#158642=CARTESIAN_POINT('Ctrl Pts',(39.495180807944,-17.2772211881662,-131.396371117214));
#158643=CARTESIAN_POINT('Ctrl Pts',(39.4966613081908,-17.396083803422,-131.427549347277));
#158644=CARTESIAN_POINT('Ctrl Pts',(39.4981991234424,-17.5150239674286,
-131.459993872874));
#158645=CARTESIAN_POINT('Ctrl Pts',(39.4989402647689,-17.5723465039512,
-131.475630327717));
#158646=CARTESIAN_POINT('Ctrl Pts',(39.4996676909946,-17.6275909302336,
-131.490985006607));
#158647=CARTESIAN_POINT('Ctrl Pts',(39.5003975533504,-17.6821327275196,
-131.506398539652));
#158648=CARTESIAN_POINT('Ctrl Pts',(39.501014492288,-17.7282358841042,-131.519427309566));
#158649=CARTESIAN_POINT('Ctrl Pts',(39.5016332183093,-17.7738366805642,
-131.532499125543));
#158650=CARTESIAN_POINT('Ctrl Pts',(39.5022647440593,-17.8197567988279,
-131.54584706425));
#158651=CARTESIAN_POINT('Ctrl Pts',(39.5023846973585,-17.8284789604902,
-131.548382399168));
#158652=CARTESIAN_POINT('Ctrl Pts',(39.5025051156569,-17.8372126194999,
-131.55092776617));
#158653=CARTESIAN_POINT('Ctrl Pts',(39.5026260789289,-17.8459633741104,
-131.553484861057));
#158654=CARTESIAN_POINT('Ctrl Pts',(39.5027441884728,-17.8545076836315,
-131.555981629755));
#158655=CARTESIAN_POINT('Ctrl Pts',(39.5028628740704,-17.8630723274425,
-131.558490774156));
#158656=CARTESIAN_POINT('Ctrl Pts',(39.5029817892779,-17.8716322053535,
-131.561004974254));
#158657=CARTESIAN_POINT('Ctrl Pts',(39.508478276978,-18.2672860888239,-131.67721609819));
#158658=CARTESIAN_POINT('Ctrl Pts',(39.5146109899203,-18.6633075913778,
-131.807303922318));
#158659=CARTESIAN_POINT('Ctrl Pts',(39.5213644858589,-19.0600784979616,
-131.951274464432));
#158660=CARTESIAN_POINT('Ctrl Pts',(39.5261325711292,-19.3402056398967,
-132.052920164296));
#158661=CARTESIAN_POINT('Ctrl Pts',(39.5312100096328,-19.6207057232028,
-132.161484957873));
#158662=CARTESIAN_POINT('Ctrl Pts',(39.5365899584985,-19.9017174949438,
-132.276955564612));
#158663=CARTESIAN_POINT('Origin',(46.4751157297648,-14.311069215956,-128.224481951383));
#158664=CARTESIAN_POINT('Ctrl Pts',(39.0000000000669,-19.98000002,-129.914446011788));
#158665=CARTESIAN_POINT('Ctrl Pts',(39.0000003661163,-19.9777368568499,
-129.988373295946));
#158666=CARTESIAN_POINT('Ctrl Pts',(39.0015009625459,-19.9753955019565,
-130.065171376428));
#158667=CARTESIAN_POINT('Ctrl Pts',(39.0048608917524,-19.9729474378609,
-130.144774766188));
#158668=CARTESIAN_POINT('Ctrl Pts',(39.0081523964114,-19.9705492282913,
-130.222757042648));
#158669=CARTESIAN_POINT('Ctrl Pts',(39.0132286832547,-19.9680484121296,
-130.303431904837));
#158670=CARTESIAN_POINT('Ctrl Pts',(39.0204492557753,-19.9654302366679,
-130.386695447003));
#158671=CARTESIAN_POINT('Ctrl Pts',(39.0274582141761,-19.9628887923649,
-130.467518775301));
#158672=CARTESIAN_POINT('Ctrl Pts',(39.036488107848,-19.9602366117811,-130.5507814907));
#158673=CARTESIAN_POINT('Ctrl Pts',(39.0478819729243,-19.9574742277174,
-130.636344073164));
#158674=CARTESIAN_POINT('Ctrl Pts',(39.0545620631387,-19.9558546741568,
-130.686508417397));
#158675=CARTESIAN_POINT('Ctrl Pts',(39.062054969042,-19.9541975163494,-130.737462445253));
#158676=CARTESIAN_POINT('Ctrl Pts',(39.0704310879636,-19.9525055342341,
-130.789170171557));
#158677=CARTESIAN_POINT('Ctrl Pts',(39.079165226721,-19.9507412318516,-130.843088037409));
#158678=CARTESIAN_POINT('Ctrl Pts',(39.0888597435241,-19.948939029304,-130.897825485729));
#158679=CARTESIAN_POINT('Ctrl Pts',(39.0995946815592,-19.9471047139459,
-130.953334379507));
#158680=CARTESIAN_POINT('Ctrl Pts',(39.1049621505767,-19.9461875562668,
-130.981088826396));
#158681=CARTESIAN_POINT('Ctrl Pts',(39.1105897492738,-19.9452623720647,
-131.009036129875));
#158682=CARTESIAN_POINT('Ctrl Pts',(39.116487410739,-19.9443302068421,-131.037169407258));
#158683=CARTESIAN_POINT('Ctrl Pts',(39.1194362414716,-19.9438641242308,
-131.05123604595));
#158684=CARTESIAN_POINT('Ctrl Pts',(39.1224525886999,-19.9433962964075,
-131.065349177994));
#158685=CARTESIAN_POINT('Ctrl Pts',(39.1255376923908,-19.9429268649362,
-131.079507915865));
#158686=CARTESIAN_POINT('Ctrl Pts',(39.1270802442362,-19.9426921492006,
-131.0865872848));
#158687=CARTESIAN_POINT('Ctrl Pts',(39.1286399852446,-19.9424570325568,
-131.093678055182));
#158688=CARTESIAN_POINT('Ctrl Pts',(39.1302170699468,-19.9422215338507,
-131.100780113065));
#158689=CARTESIAN_POINT('Ctrl Pts',(39.1310056122978,-19.9421037844977,
-131.104331142007));
#158690=CARTESIAN_POINT('Ctrl Pts',(39.1317984905748,-19.9419859396293,
-131.107884992824));
#158691=CARTESIAN_POINT('Ctrl Pts',(39.1325957240583,-19.941868001679,-131.111441651072));
#158692=CARTESIAN_POINT('Ctrl Pts',(39.1333929575419,-19.9417500637286,
-131.114998309321));
#158693=CARTESIAN_POINT('Ctrl Pts',(39.134531130502,-19.941582703029,-131.120045436292));
#158694=CARTESIAN_POINT('Ctrl Pts',(39.1350005094029,-19.9415139110393,
-131.122120033608));
#158695=CARTESIAN_POINT('Ctrl Pts',(39.1425105718177,-19.9404132392045,
-131.155313590669));
#158696=CARTESIAN_POINT('Ctrl Pts',(39.1512549053093,-19.939183276348,-131.192549999964));
#158697=CARTESIAN_POINT('Ctrl Pts',(39.1614907401956,-19.9378138682254,
-131.233761736226));
#158698=CARTESIAN_POINT('Ctrl Pts',(39.171726575082,-19.9364444601029,-131.274973472488));
#158699=CARTESIAN_POINT('Ctrl Pts',(39.1834541487602,-19.9349353410833,
-131.320161159432));
#158700=CARTESIAN_POINT('Ctrl Pts',(39.1969827572539,-19.9332812983121,
-131.369224668865));
#158701=CARTESIAN_POINT('Ctrl Pts',(39.207442020742,-19.9320025216239,-131.407156742445));
#158702=CARTESIAN_POINT('Ctrl Pts',(39.2188983592693,-19.9306465353236,
-131.447121602909));
#158703=CARTESIAN_POINT('Ctrl Pts',(39.2315999854523,-19.9292039335511,
-131.48938673147));
#158704=CARTESIAN_POINT('Ctrl Pts',(39.2436716909817,-19.9278328757399,
-131.529555775874));
#158705=CARTESIAN_POINT('Ctrl Pts',(39.2568682353366,-19.9263834726761,
-131.571802875789));
#158706=CARTESIAN_POINT('Ctrl Pts',(39.2714424595273,-19.9248510153574,
-131.616333969799));
#158707=CARTESIAN_POINT('Ctrl Pts',(39.2812031361056,-19.9238246951867,
-131.646157417045));
#158708=CARTESIAN_POINT('Ctrl Pts',(39.2915825498145,-19.9227611873571,
-131.677004826585));
#158709=CARTESIAN_POINT('Ctrl Pts',(39.3026674122468,-19.9216604123578,
-131.708930511829));
#158710=CARTESIAN_POINT('Ctrl Pts',(39.3230244720018,-19.9196388678799,
-131.767561197254));
#158711=CARTESIAN_POINT('Ctrl Pts',(39.3432099268556,-19.9177236323538,
-131.822474694915));
#158712=CARTESIAN_POINT('Ctrl Pts',(39.3628888866153,-19.9159285670117,
-131.873757669544));
#158713=CARTESIAN_POINT('Ctrl Pts',(39.3830325254433,-19.9140911148106,
-131.92625158851));
#158714=CARTESIAN_POINT('Ctrl Pts',(39.4026453461985,-19.9123793539091,
-131.974942141252));
#158715=CARTESIAN_POINT('Ctrl Pts',(39.4214203923536,-19.9107967575629,
-132.019933390249));
#158716=CARTESIAN_POINT('Ctrl Pts',(39.4403970415853,-19.9091971675812,
-132.065407747205));
#158717=CARTESIAN_POINT('Ctrl Pts',(39.4585178974063,-19.9077292958912,
-132.107103532241));
#158718=CARTESIAN_POINT('Ctrl Pts',(39.4755189459911,-19.9063887570054,
-132.145129888499));
#158719=CARTESIAN_POINT('Ctrl Pts',(39.4927238794532,-19.9050321417226,
-132.183612275391));
#158720=CARTESIAN_POINT('Ctrl Pts',(39.5087820945746,-19.9038057193559,
-132.218337222793));
#158721=CARTESIAN_POINT('Ctrl Pts',(39.5234725234859,-19.9027002333108,
-132.249410952062));
#158722=CARTESIAN_POINT('Ctrl Pts',(39.5279749265633,-19.9023614178956,
-132.258934598726));
#158723=CARTESIAN_POINT('Ctrl Pts',(39.5323492112491,-19.9020339414172,
-132.268115196008));
#158724=CARTESIAN_POINT('Ctrl Pts',(39.5365899584985,-19.9017174949438,
-132.276955564612));
#158725=CARTESIAN_POINT('Origin',(0.,-12.9675000200281,-171.64995));
#158726=CARTESIAN_POINT('',(57.9903087491627,-19.9260113903464,-171.449026400902));
#158727=CARTESIAN_POINT('',(58.3906572805143,-14.3195102506022,-171.449026400902));
#158728=CARTESIAN_POINT('Origin',(0.,-12.9675000200281,-171.449026400902));
#158729=CARTESIAN_POINT('Ctrl Pts',(58.3906572805143,-14.3195102506022,
-171.449026400902));
#158730=CARTESIAN_POINT('Ctrl Pts',(56.6764429446617,-14.3192048286978,
-167.77385178941));
#158731=CARTESIAN_POINT('Ctrl Pts',(55.0310749604167,-14.318890449637,-164.246346972861));
#158732=CARTESIAN_POINT('Ctrl Pts',(53.4545452629458,-14.318560171184,-160.866515925776));
#158733=CARTESIAN_POINT('Ctrl Pts',(52.6662804142103,-14.3183950319575,
-159.176600402234));
#158734=CARTESIAN_POINT('Ctrl Pts',(51.895225247074,-14.3182260159383,-157.523603253589));
#158735=CARTESIAN_POINT('Ctrl Pts',(51.1413794916545,-14.3180481994016,
-155.907524626682));
#158736=CARTESIAN_POINT('Ctrl Pts',(50.7644566139448,-14.3179592911332,
-155.099485313228));
#158737=CARTESIAN_POINT('Ctrl Pts',(50.391836093189,-14.3178683195607,-154.300675628705));
#158738=CARTESIAN_POINT('Ctrl Pts',(50.0235178752065,-14.317777011786,-153.51109559057));
#158739=CARTESIAN_POINT('Ctrl Pts',(49.8393587662153,-14.3177313578986,
-153.116305571502));
#158740=CARTESIAN_POINT('Ctrl Pts',(49.6562752331921,-14.3176856199487,
-152.723822963869));
#158741=CARTESIAN_POINT('Ctrl Pts',(49.4742672731976,-14.3176399235889,
-152.333647768291));
#158742=CARTESIAN_POINT('Ctrl Pts',(49.3832632932003,-14.317617075409,-152.138560170502));
#158743=CARTESIAN_POINT('Ctrl Pts',(49.2925282064789,-14.317594237627,-151.944049425717));
#158744=CARTESIAN_POINT('Ctrl Pts',(49.2020620127266,-14.3175714278585,
-151.750115533972));
#158745=CARTESIAN_POINT('Ctrl Pts',(49.1144228875291,-14.3175493308953,
-151.562242076344));
#158746=CARTESIAN_POINT('Ctrl Pts',(49.0270361120814,-14.317527260222,-151.374909981773));
#158747=CARTESIAN_POINT('Ctrl Pts',(48.9399016861439,-14.3175052327755,
-151.188119250263));
#158748=CARTESIAN_POINT('Ctrl Pts',(48.9370908982105,-14.3175045222127,
-151.182093742795));
#158749=CARTESIAN_POINT('Ctrl Pts',(48.9348754797666,-14.3175039621476,
-151.177344533669));
#158750=CARTESIAN_POINT('Ctrl Pts',(48.9314701101151,-14.3175031012272,
-151.170044417858));
#158751=CARTESIAN_POINT('Ctrl Pts',(46.2622647123347,-14.3168282924576,
-145.448049298071));
#158752=CARTESIAN_POINT('Ctrl Pts',(43.7885373821752,-14.3160934996481,
-140.145481122769));
#158753=CARTESIAN_POINT('Ctrl Pts',(41.5103050054923,-14.3152949524359,
-135.26233262387));
#158754=CARTESIAN_POINT('Ctrl Pts',(40.812213131252,-14.315050263033,-133.766047028652));
#158755=CARTESIAN_POINT('Ctrl Pts',(40.1324769686662,-14.3147998235171,
-132.309141494925));
#158756=CARTESIAN_POINT('Ctrl Pts',(39.4710976496822,-14.3145440753934,
-130.89161549018));
#158757=CARTESIAN_POINT('Ctrl Pts',(39.5365899624517,-19.9017174575869,
-132.27695566545));
#158758=CARTESIAN_POINT('Ctrl Pts',(40.9222207127391,-19.9043502993893,
-135.204751179876));
#158759=CARTESIAN_POINT('Ctrl Pts',(42.3851075877766,-19.9070565011848,
-138.300261437352));
#158760=CARTESIAN_POINT('Ctrl Pts',(44.6953683528657,-19.9106521746941,
-143.195098938138));
#158761=CARTESIAN_POINT('Ctrl Pts',(45.484775776705,-19.911785330507,-144.868640124163));
#158762=CARTESIAN_POINT('Ctrl Pts',(46.6978643305816,-19.9134223042145,
-147.441844931843));
#158763=CARTESIAN_POINT('Ctrl Pts',(47.3116528834097,-19.914226217965,-148.744170592844));
#158764=CARTESIAN_POINT('Ctrl Pts',(48.0404155449538,-19.9151581515399,
-150.29106623071));
#158765=CARTESIAN_POINT('Ctrl Pts',(48.4079656496442,-19.915625950211,-151.07139297465));
#158766=CARTESIAN_POINT('Ctrl Pts',(48.6156037677501,-19.9158900971054,
-151.512261465775));
#158767=CARTESIAN_POINT('Ctrl Pts',(48.7180581100362,-19.916020478077,-151.729811584573));
#158768=CARTESIAN_POINT('Ctrl Pts',(48.7710084967803,-19.9160878923004,
-151.842249064289));
#158769=CARTESIAN_POINT('Ctrl Pts',(48.774880162121,-19.9160928217188,-151.850470369442));
#158770=CARTESIAN_POINT('Ctrl Pts',(51.5915976683688,-19.919679174478,-157.83165200233));
#158771=CARTESIAN_POINT('Ctrl Pts',(54.6624934339681,-19.9229803733939,
-164.362558913099));
#158772=CARTESIAN_POINT('Ctrl Pts',(57.9903087491627,-19.9260113903464,
-171.449026400902));
#158773=CARTESIAN_POINT('Ctrl Pts',(60.,-20.8715629014036,-174.505875827596));
#158774=CARTESIAN_POINT('Ctrl Pts',(59.9999999999999,-20.9611893120647,
-176.449983597595));
#158775=CARTESIAN_POINT('Ctrl Pts',(58.2228448679712,-20.997722377502,-177.242431000704));
#158776=CARTESIAN_POINT('Ctrl Pts',(60.,-21.0755801285197,-174.496470313984));
#158777=CARTESIAN_POINT('Ctrl Pts',(59.9999999999923,-21.1661125646405,
-176.460241938351));
#158778=CARTESIAN_POINT('Ctrl Pts',(58.1976125313383,-21.2014273832677,
-177.244315088819));
#158779=CARTESIAN_POINT('Ctrl Pts',(60.,-21.2796010327843,-174.487167894352));
#158780=CARTESIAN_POINT('Ctrl Pts',(60.0000000000095,-21.3701601153012,
-176.47139510613));
#158781=CARTESIAN_POINT('Ctrl Pts',(58.1714292060958,-21.40462514847,-177.246332126403));
#158782=CARTESIAN_POINT('Ctrl Pts',(60.,-21.4836289747507,-174.478062871828));
#158783=CARTESIAN_POINT('Ctrl Pts',(60.,-21.57312595156,-176.483536694353));
#158784=CARTESIAN_POINT('Ctrl Pts',(58.1443031111632,-21.607263174561,-177.248493339177));
#158785=CARTESIAN_POINT('',(60.,-21.48000002,-174.47822483969));
#158786=CARTESIAN_POINT('',(58.1799818944376,-21.5006430239275,-177.23826171807));
#158787=CARTESIAN_POINT('Ctrl Pts',(60.,-21.48000002,-174.47822483969));
#158788=CARTESIAN_POINT('Ctrl Pts',(60.,-21.4803505539985,-174.525420140524));
#158789=CARTESIAN_POINT('Ctrl Pts',(60.0001399779557,-21.4809879986116,
-174.619372716533));
#158790=CARTESIAN_POINT('Ctrl Pts',(59.9796633935931,-21.4825721374009,
-174.834540579974));
#158791=CARTESIAN_POINT('Ctrl Pts',(59.9691516993081,-21.4832061865197,
-174.91866280707));
#158792=CARTESIAN_POINT('Ctrl Pts',(59.9428873533568,-21.4843111756952,
-175.063261197871));
#158793=CARTESIAN_POINT('Ctrl Pts',(59.9323654277428,-21.4847047157807,
-175.114519734261));
#158794=CARTESIAN_POINT('Ctrl Pts',(59.9131593178258,-21.4853260452443,
-175.195833730679));
#158795=CARTESIAN_POINT('Ctrl Pts',(59.9026989428284,-21.4856443826443,
-175.237595425077));
#158796=CARTESIAN_POINT('Ctrl Pts',(59.8888111932657,-21.4860267073919,
-175.288192398583));
#158797=CARTESIAN_POINT('Ctrl Pts',(59.8814224077432,-21.4862202024632,
-175.313950381331));
#158798=CARTESIAN_POINT('Ctrl Pts',(59.8781578694836,-21.4863035832901,
-175.325086930002));
#158799=CARTESIAN_POINT('Ctrl Pts',(59.875959462847,-21.4863592661649,-175.332532820678));
#158800=CARTESIAN_POINT('Ctrl Pts',(59.8745119134935,-21.4863955582652,
-175.337392867869));
#158801=CARTESIAN_POINT('Ctrl Pts',(59.8235471264794,-21.4876651097968,
-175.507567331279));
#158802=CARTESIAN_POINT('Ctrl Pts',(59.7625865562566,-21.4888125164959,
-175.657773599687));
#158803=CARTESIAN_POINT('Ctrl Pts',(59.6668100439519,-21.4902869942187,
-175.855173103668));
#158804=CARTESIAN_POINT('Ctrl Pts',(59.6341488192349,-21.4907398771631,
-175.916376608615));
#158805=CARTESIAN_POINT('Ctrl Pts',(59.5853331656683,-21.4913676068731,
-176.001447175398));
#158806=CARTESIAN_POINT('Ctrl Pts',(59.5609666819441,-21.491668721715,-176.042302052764));
#158807=CARTESIAN_POINT('Ctrl Pts',(59.5328610248443,-21.4920003992658,
-176.087088941708));
#158808=CARTESIAN_POINT('Ctrl Pts',(59.5189174770905,-21.4921617429715,
-176.108772671461));
#158809=CARTESIAN_POINT('Ctrl Pts',(59.5129681152444,-21.4922299719197,
-176.117914660496));
#158810=CARTESIAN_POINT('Ctrl Pts',(59.5090080803609,-21.4922752589613,
-176.123975875479));
#158811=CARTESIAN_POINT('Ctrl Pts',(59.5078278775364,-21.4922887416491,
-176.125779857974));
#158812=CARTESIAN_POINT('Ctrl Pts',(59.3277545680046,-21.4943367985525,
-176.399243062079));
#158813=CARTESIAN_POINT('Ctrl Pts',(59.112894255709,-21.4961971427573,-176.62948927359));
#158814=CARTESIAN_POINT('Ctrl Pts',(58.6562287443494,-21.4989602174682,
-176.998436545936));
#158815=CARTESIAN_POINT('Ctrl Pts',(58.4150195201894,-21.4998854333264,
-177.137642938512));
#158816=CARTESIAN_POINT('Ctrl Pts',(58.1799818947148,-21.5006430233981,
-177.238261718413));
#158817=CARTESIAN_POINT('',(58.2408314794355,-21.0009616714991,-177.234172657581));
#158818=CARTESIAN_POINT('Origin',(-8.61422153796722,-13.0251077027817,-187.988562411664));
#158819=CARTESIAN_POINT('',(60.,-20.98000002,-174.500886972636));
#158820=CARTESIAN_POINT('Ctrl Pts',(58.2408309122627,-21.0009616140329,
-177.234171411));
#158821=CARTESIAN_POINT('Ctrl Pts',(58.2980225092941,-21.0007609899858,
-177.208159469229));
#158822=CARTESIAN_POINT('Ctrl Pts',(58.3554746487018,-21.0005425919237,
-177.179810838538));
#158823=CARTESIAN_POINT('Ctrl Pts',(58.4129879890245,-21.0003055852495,
-177.149025012205));
#158824=CARTESIAN_POINT('Ctrl Pts',(58.4687033405938,-21.0000759879055,
-177.119201615964));
#158825=CARTESIAN_POINT('Ctrl Pts',(58.5244764048851,-20.999828925583,-177.087090811604));
#158826=CARTESIAN_POINT('Ctrl Pts',(58.5800794173198,-20.9995636500946,
-177.052602282868));
#158827=CARTESIAN_POINT('Ctrl Pts',(58.63402128412,-20.9993062997384,-177.019144102425));
#158828=CARTESIAN_POINT('Ctrl Pts',(58.6878033716843,-20.9990318066526,
-176.983447946087));
#158829=CARTESIAN_POINT('Ctrl Pts',(58.7411692944488,-20.9987395210302,
-176.945435343265));
#158830=CARTESIAN_POINT('Ctrl Pts',(58.7924353414766,-20.9984587364454,
-176.908918484136));
#158831=CARTESIAN_POINT('Ctrl Pts',(58.8433174795946,-20.9981615307026,
-176.870263722897));
#158832=CARTESIAN_POINT('Ctrl Pts',(58.8935402105985,-20.9978473791949,
-176.829407837885));
#158833=CARTESIAN_POINT('Ctrl Pts',(58.9036719315393,-20.9977840036009,
-176.821165744764));
#158834=CARTESIAN_POINT('Ctrl Pts',(58.9137766493985,-20.9977199385699,
-176.812834097921));
#158835=CARTESIAN_POINT('Ctrl Pts',(58.9238518425652,-20.9976551801365,
-176.804412420825));
#158836=CARTESIAN_POINT('Ctrl Pts',(58.9326728926055,-20.9975984827241,
-176.797039059952));
#158837=CARTESIAN_POINT('Ctrl Pts',(58.9414695595589,-20.9975412674908,
-176.789598141511));
#158838=CARTESIAN_POINT('Ctrl Pts',(58.9502388844965,-20.997483541128,-176.782090523443));
#158839=CARTESIAN_POINT('Ctrl Pts',(58.9984162702457,-20.9971664009531,
-176.74084477029));
#158840=CARTESIAN_POINT('Ctrl Pts',(59.0459429298583,-20.9968333060902,
-176.697517295804));
#158841=CARTESIAN_POINT('Ctrl Pts',(59.0925361026031,-20.9964844704348,
-176.652133568374));
#158842=CARTESIAN_POINT('Ctrl Pts',(59.1264706681046,-20.9962304077535,
-176.619079861566));
#158843=CARTESIAN_POINT('Ctrl Pts',(59.159910744717,-20.9959680013015,-176.58493618398));
#158844=CARTESIAN_POINT('Ctrl Pts',(59.1927590407498,-20.9956974369349,
-176.549725798655));
#158845=CARTESIAN_POINT('Ctrl Pts',(59.2141973373912,-20.9955208542851,
-176.526745894775));
#158846=CARTESIAN_POINT('Ctrl Pts',(59.2353825316704,-20.9953408095841,
-176.503313294377));
#158847=CARTESIAN_POINT('Ctrl Pts',(59.256294110943,-20.995157339527,-176.479432519626));
#158848=CARTESIAN_POINT('Ctrl Pts',(59.2962851015841,-20.9948064741407,
-176.433763284073));
#158849=CARTESIAN_POINT('Ctrl Pts',(59.3352429768689,-20.9944429709512,
-176.38644039433));
#158850=CARTESIAN_POINT('Ctrl Pts',(59.3730217009492,-20.9940675205211,
-176.337552001638));
#158851=CARTESIAN_POINT('Ctrl Pts',(59.3981850918781,-20.9938174430985,
-176.304988759571));
#158852=CARTESIAN_POINT('Ctrl Pts',(59.422824079193,-20.9935620676181,-176.271731280423));
#158853=CARTESIAN_POINT('Ctrl Pts',(59.4468837816017,-20.9933015806725,
-176.237803245043));
#158854=CARTESIAN_POINT('Ctrl Pts',(59.458913632806,-20.9931713371996,-176.220839227352));
#158855=CARTESIAN_POINT('Ctrl Pts',(59.4707984783363,-20.9930398159737,
-176.203707584064));
#158856=CARTESIAN_POINT('Ctrl Pts',(59.4825305150169,-20.9929070384393,
-176.186411021836));
#158857=CARTESIAN_POINT('Ctrl Pts',(59.4883965333572,-20.9928406496721,
-176.177762740722));
#158858=CARTESIAN_POINT('Ctrl Pts',(59.4942243293403,-20.9927739469164,
-176.16907324131));
#158859=CARTESIAN_POINT('Ctrl Pts',(59.5000128525514,-20.9927069328473,
-176.160342860609));
#158860=CARTESIAN_POINT('Ctrl Pts',(59.5029071141569,-20.9926734258127,
-176.155977670259));
#158861=CARTESIAN_POINT('Ctrl Pts',(59.5057915568634,-20.9926398409485,
-176.151602259423));
#158862=CARTESIAN_POINT('Ctrl Pts',(59.5086660442441,-20.9926061785915,
-176.147216670479));
#158863=CARTESIAN_POINT('Ctrl Pts',(59.5101859584498,-20.9925883792806,
-176.144897746075));
#158864=CARTESIAN_POINT('Ctrl Pts',(59.5117030892688,-20.992570558303,-176.142575975924));
#158865=CARTESIAN_POINT('Ctrl Pts',(59.5132174161754,-20.9925527157083,
-176.140251366253));
#158866=CARTESIAN_POINT('Ctrl Pts',(59.5136029453564,-20.9925481732011,
-176.139659548952));
#158867=CARTESIAN_POINT('Ctrl Pts',(59.5139882928002,-20.9925436292928,
-176.139067547608));
#158868=CARTESIAN_POINT('Ctrl Pts',(59.5143734581649,-20.9925390839842,
-176.138475362326));
#158869=CARTESIAN_POINT('Ctrl Pts',(59.5146391908111,-20.9925359480924,
-176.138066802843));
#158870=CARTESIAN_POINT('Ctrl Pts',(59.5149048367898,-20.9925328115342,
-176.137658155807));
#158871=CARTESIAN_POINT('Ctrl Pts',(59.5151703959885,-20.9925296743097,
-176.137249421253));
#158872=CARTESIAN_POINT('Ctrl Pts',(59.5154011012622,-20.9925269488374,
-176.136894332001));
#158873=CARTESIAN_POINT('Ctrl Pts',(59.5156369697105,-20.9925241610901,
-176.13653112869));
#158874=CARTESIAN_POINT('Ctrl Pts',(59.5158771919828,-20.9925213204693,
-176.136161036115));
#158875=CARTESIAN_POINT('Ctrl Pts',(59.5163626876872,-20.9925155794979,
-176.135413069019));
#158876=CARTESIAN_POINT('Ctrl Pts',(59.5168650831917,-20.9925096329291,
-176.13463831307));
#158877=CARTESIAN_POINT('Ctrl Pts',(59.5173723671556,-20.9925036221267,
-176.133855185661));
#158878=CARTESIAN_POINT('Ctrl Pts',(59.5189847061201,-20.992484517539,-176.131366112625));
#158879=CARTESIAN_POINT('Ctrl Pts',(59.5206462689632,-20.9924647590044,
-176.128791809003));
#158880=CARTESIAN_POINT('Ctrl Pts',(59.521976211733,-20.9924489032738,-176.126725977334));
#158881=CARTESIAN_POINT('Ctrl Pts',(59.5223775029386,-20.9924441190339,
-176.126102642179));
#158882=CARTESIAN_POINT('Ctrl Pts',(59.5227486471359,-20.9924396903121,
-176.125525625579));
#158883=CARTESIAN_POINT('Ctrl Pts',(59.5230792754666,-20.9924357426811,
-176.125011289112));
#158884=CARTESIAN_POINT('Ctrl Pts',(59.5232128115734,-20.9924341482888,
-176.124803555886));
#158885=CARTESIAN_POINT('Ctrl Pts',(59.5233389910641,-20.9924326413239,
-176.124607213406));
#158886=CARTESIAN_POINT('Ctrl Pts',(59.5234673634073,-20.992431107786,-176.124407408557));
#158887=CARTESIAN_POINT('Ctrl Pts',(59.5564258070327,-20.9920373857261,
-176.073109311956));
#158888=CARTESIAN_POINT('Ctrl Pts',(59.5902891109346,-20.9916067368321,
-176.016989055202));
#158889=CARTESIAN_POINT('Ctrl Pts',(59.624130621386,-20.9911378554161,-175.955869202696));
#158890=CARTESIAN_POINT('Ctrl Pts',(59.6410513766116,-20.9909034147081,
-175.925309276443));
#158891=CARTESIAN_POINT('Ctrl Pts',(59.6579660208221,-20.9906594132553,
-175.893499084123));
#158892=CARTESIAN_POINT('Ctrl Pts',(59.6747556984726,-20.9904056762572,
-175.860414770979));
#158893=CARTESIAN_POINT('Ctrl Pts',(59.6835884223126,-20.9902721901427,
-175.843009755379));
#158894=CARTESIAN_POINT('Ctrl Pts',(59.6923865345141,-20.9901360095157,
-175.82525209878));
#158895=CARTESIAN_POINT('Ctrl Pts',(59.7011325951197,-20.9899971084505,
-175.807138253296));
#158896=CARTESIAN_POINT('Ctrl Pts',(59.7083460854132,-20.9898825469889,
-175.792198493047));
#158897=CARTESIAN_POINT('Ctrl Pts',(59.7155249023031,-20.9897661213385,
-175.777014659413));
#158898=CARTESIAN_POINT('Ctrl Pts',(59.7226512817366,-20.98964795287,-175.761602485893));
#158899=CARTESIAN_POINT('Ctrl Pts',(59.7233086393773,-20.9896370526721,
-175.760180822885));
#158900=CARTESIAN_POINT('Ctrl Pts',(59.7239655678023,-20.9896261373806,
-175.758757182504));
#158901=CARTESIAN_POINT('Ctrl Pts',(59.7246220603473,-20.9896152069761,
-175.757331562141));
#158902=CARTESIAN_POINT('Ctrl Pts',(59.7426945533578,-20.9893143053719,
-175.718085855172));
#158903=CARTESIAN_POINT('Ctrl Pts',(59.7604642712953,-20.9890011177224,
-175.677230878131));
#158904=CARTESIAN_POINT('Ctrl Pts',(59.7777374148834,-20.9886761769839,
-175.63483458625));
#158905=CARTESIAN_POINT('Ctrl Pts',(59.786590310033,-20.9885096371603,-175.613105482637));
#158906=CARTESIAN_POINT('Ctrl Pts',(59.7953115318292,-20.9883400331687,
-175.590974522494));
#158907=CARTESIAN_POINT('Ctrl Pts',(59.803875922402,-20.988167406105,-175.568446835027));
#158908=CARTESIAN_POINT('Ctrl Pts',(59.8214736860823,-20.98781269899,-175.522157853114));
#158909=CARTESIAN_POINT('Ctrl Pts',(59.8384192713474,-20.9874450703999,
-175.474173290825));
#158910=CARTESIAN_POINT('Ctrl Pts',(59.8544690713476,-20.9870649116206,
-175.424541860454));
#158911=CARTESIAN_POINT('Ctrl Pts',(59.8619224947127,-20.986888368341,-175.401493345036));
#158912=CARTESIAN_POINT('Ctrl Pts',(59.8691821364436,-20.9867091261014,
-175.378090090578));
#158913=CARTESIAN_POINT('Ctrl Pts',(59.8762202767283,-20.9865272376599,
-175.35433870977));
#158914=CARTESIAN_POINT('Ctrl Pts',(59.8764969529595,-20.986520087446,-175.353405019581));
#158915=CARTESIAN_POINT('Ctrl Pts',(59.8767260835289,-20.9865141545933,
-175.352630294314));
#158916=CARTESIAN_POINT('Ctrl Pts',(59.8769595354051,-20.986508101865,-175.351839913648));
#158917=CARTESIAN_POINT('Ctrl Pts',(59.8773656835597,-20.9864975716242,
-175.350464848027));
#158918=CARTESIAN_POINT('Ctrl Pts',(59.8777854130835,-20.9864866791224,
-175.349042476302));
#158919=CARTESIAN_POINT('Ctrl Pts',(59.8784867712533,-20.9864683764864,
-175.346652423526));
#158920=CARTESIAN_POINT('Ctrl Pts',(59.8951524677523,-20.9860334686325,
-175.289859908819));
#158921=CARTESIAN_POINT('Ctrl Pts',(59.9092622647949,-20.9856141796718,
-175.235700841717));
#158922=CARTESIAN_POINT('Ctrl Pts',(59.9213105226927,-20.9852134475942,
-175.184255041104));
#158923=CARTESIAN_POINT('Ctrl Pts',(59.9333080963485,-20.9848144013041,
-175.133025661109));
#158924=CARTESIAN_POINT('Ctrl Pts',(59.9432614521596,-20.9844337557669,
-175.084486756453));
#158925=CARTESIAN_POINT('Ctrl Pts',(59.9516078878375,-20.984074329303,-175.038707777574));
#158926=CARTESIAN_POINT('Ctrl Pts',(59.9599375046911,-20.9837156271159,
-174.993021047486));
#158927=CARTESIAN_POINT('Ctrl Pts',(59.9666666937355,-20.9833780582865,
-174.950083123863));
#158928=CARTESIAN_POINT('Ctrl Pts',(59.9721790686904,-20.9830643460922,
-174.909953824021));
#158929=CARTESIAN_POINT('Ctrl Pts',(59.9776790706391,-20.9827513380522,
-174.869914597891));
#158930=CARTESIAN_POINT('Ctrl Pts',(59.9819677270108,-20.9824620793983,
-174.832671393466));
#158931=CARTESIAN_POINT('Ctrl Pts',(59.9853749488932,-20.9821992015194,
-174.798274559429));
#158932=CARTESIAN_POINT('Ctrl Pts',(59.9862696517874,-20.9821301723786,
-174.789242289731));
#158933=CARTESIAN_POINT('Ctrl Pts',(59.9871033020603,-20.9820629619045,
-174.780406239223));
#158934=CARTESIAN_POINT('Ctrl Pts',(59.9878812857174,-20.9819976169342,
-174.771767216616));
#158935=CARTESIAN_POINT('Ctrl Pts',(59.9907884757324,-20.9817534341119,
-174.739484687239));
#158936=CARTESIAN_POINT('Ctrl Pts',(59.9929279440318,-20.9815324672645,
-174.709892376057));
#158937=CARTESIAN_POINT('Ctrl Pts',(59.9945472810677,-20.9813332116831,
-174.682970861426));
#158938=CARTESIAN_POINT('Ctrl Pts',(59.996197019977,-20.9811302152234,-174.655543914966));
#158939=CARTESIAN_POINT('Ctrl Pts',(59.9973068774898,-20.9809497528969,
-174.630888979004));
#158940=CARTESIAN_POINT('Ctrl Pts',(59.9980852070704,-20.9807901713966,
-174.608976344373));
#158941=CARTESIAN_POINT('Ctrl Pts',(59.9988728010901,-20.9806286904015,
-174.586802884156));
#158942=CARTESIAN_POINT('Ctrl Pts',(59.9993208127642,-20.9804885902046,
-174.567437372749));
#158943=CARTESIAN_POINT('Ctrl Pts',(59.9995921509242,-20.9803680953684,
-174.550840012396));
#158944=CARTESIAN_POINT('Ctrl Pts',(59.9998684942221,-20.9802453778693,
-174.533936495053));
#158945=CARTESIAN_POINT('Ctrl Pts',(59.9999615061132,-20.9801429956864,
-174.519904176989));
#158946=CARTESIAN_POINT('Ctrl Pts',(59.9999900624123,-20.9800590094608,
-174.50869202207));
#158947=CARTESIAN_POINT('Ctrl Pts',(59.9999971274817,-20.9800382305599,
-174.505918040328));
#158948=CARTESIAN_POINT('Ctrl Pts',(60.,-20.9800185773921,-174.503316641764));
#158949=CARTESIAN_POINT('Ctrl Pts',(60.,-20.98000002,-174.500886972636));
#158950=CARTESIAN_POINT('Ctrl Pts',(60.,-21.48000002,-174.47822483969));
#158951=CARTESIAN_POINT('Ctrl Pts',(60.,-21.3133292808184,-174.485664661366));
#158952=CARTESIAN_POINT('Ctrl Pts',(60.,-21.1466632268706,-174.493235890728));
#158953=CARTESIAN_POINT('Ctrl Pts',(60.,-20.98000002,-174.500886972636));
#158954=CARTESIAN_POINT('Origin',(39.,46.91999998,-129.34995));
#158955=CARTESIAN_POINT('',(39.0000000011086,-28.13000002,-134.169022080262));
#158956=CARTESIAN_POINT('',(39.,-22.48000002,-130.903539806302));
#158957=CARTESIAN_POINT('Ctrl Pts',(39.0000000022172,-28.13000002,-134.169022080262));
#158958=CARTESIAN_POINT('Ctrl Pts',(39.0000000027011,-27.7992138900219,
-133.93790810089));
#158959=CARTESIAN_POINT('Ctrl Pts',(39.0000000021338,-27.4657185053507,
-133.711655036841));
#158960=CARTESIAN_POINT('Ctrl Pts',(39.0000000015399,-27.1287626917287,
-133.490292823798));
#158961=CARTESIAN_POINT('Ctrl Pts',(39.0000000009697,-26.8052287127266,
-133.277748048811));
#158962=CARTESIAN_POINT('Ctrl Pts',(39.0000000004972,-26.4785047877952,
-133.069711931569));
#158963=CARTESIAN_POINT('Ctrl Pts',(39.0000000003364,-26.1478973077855,
-132.866246059588));
#158964=CARTESIAN_POINT('Ctrl Pts',(39.0000000002123,-25.8927164902428,
-132.709200043712));
#158965=CARTESIAN_POINT('Ctrl Pts',(39.0000000001809,-25.6361572010218,
-132.555471936139));
#158966=CARTESIAN_POINT('Ctrl Pts',(39.0000000003918,-25.3779449003587,
-132.405146018542));
#158967=CARTESIAN_POINT('Ctrl Pts',(39.0000000007921,-24.8877366470251,
-132.119756804679));
#158968=CARTESIAN_POINT('Ctrl Pts',(39.000000000553,-24.3912688192582,-131.84632373554));
#158969=CARTESIAN_POINT('Ctrl Pts',(39.0000000002964,-23.8878019342404,
-131.586247706167));
#158970=CARTESIAN_POINT('Ctrl Pts',(39.0000000000603,-23.4246527701181,
-131.346998613135));
#158971=CARTESIAN_POINT('Ctrl Pts',(39.0000000000002,-22.9555805746395,
-131.119053182003));
#158972=CARTESIAN_POINT('Ctrl Pts',(39.,-22.48000002,-130.903539806302));
#158973=CARTESIAN_POINT('',(39.,-22.48000002,-101.155103165204));
#158974=CARTESIAN_POINT('',(39.,-22.48000002,-129.34995));
#158975=CARTESIAN_POINT('',(39.,-28.13000002,-97.8896208912436));
#158976=CARTESIAN_POINT('Ctrl Pts',(39.,-22.48000002,-101.155103165204));
#158977=CARTESIAN_POINT('Ctrl Pts',(39.0000000000003,-23.0421399014191,
-100.900364693921));
#158978=CARTESIAN_POINT('Ctrl Pts',(39.0000000001808,-23.5949958654216,
-100.628353151271));
#158979=CARTESIAN_POINT('Ctrl Pts',(39.0000000005377,-24.1395638864455,
-100.340934396652));
#158980=CARTESIAN_POINT('Ctrl Pts',(39.0000000008113,-24.5569439995021,
-100.120644427969));
#158981=CARTESIAN_POINT('Ctrl Pts',(39.0000000009101,-24.9694552602945,
-99.8913025435709));
#158982=CARTESIAN_POINT('Ctrl Pts',(39.0000000004916,-25.3775420853185,
-99.6537285981461));
#158983=CARTESIAN_POINT('Ctrl Pts',(39.0000000002285,-25.6341396980635,
-99.5043463992897));
#158984=CARTESIAN_POINT('Ctrl Pts',(39.0000000001306,-25.8888446969123,
-99.35177201821));
#158985=CARTESIAN_POINT('Ctrl Pts',(39.0000000000752,-26.1419870362595,
-99.1960691366333));
#158986=CARTESIAN_POINT('Ctrl Pts',(39.0000000000073,-26.4522179455436,
-99.0052521968269));
#158987=CARTESIAN_POINT('Ctrl Pts',(39.0000000000056,-26.7601021070994,
-98.8096624723066));
#158988=CARTESIAN_POINT('Ctrl Pts',(39.0000000000023,-27.0653588164942,
-98.6099244013));
#158989=CARTESIAN_POINT('Ctrl Pts',(38.9999999999992,-27.3493059604978,
-98.4241297797058));
#158990=CARTESIAN_POINT('Ctrl Pts',(39.0000000000001,-27.6309803020602,
-98.2347441815217));
#158991=CARTESIAN_POINT('Ctrl Pts',(39.0000000000002,-27.9101240577928,
-98.0422452092007));
#158992=CARTESIAN_POINT('Ctrl Pts',(39.0000000000002,-27.9835605023139,
-97.9916030586567));
#158993=CARTESIAN_POINT('Ctrl Pts',(39.0000000000002,-28.0568495646841,
-97.9407287002963));
#158994=CARTESIAN_POINT('Ctrl Pts',(39.0000000000003,-28.13000002,-97.8896208912436));
#158995=CARTESIAN_POINT('',(39.,-28.13000002,-129.34995));
#158996=CARTESIAN_POINT('Ctrl Pts',(39.,-29.6092937616716,-135.247171188664));
#158997=CARTESIAN_POINT('Ctrl Pts',(38.9999999999999,-28.7416759820709,
-136.390803950004));
#158998=CARTESIAN_POINT('Ctrl Pts',(39.7614953849933,-28.006195589491,-137.360262497367));
#158999=CARTESIAN_POINT('Ctrl Pts',(39.,-28.4992718278429,-134.405052285569));
#159000=CARTESIAN_POINT('Ctrl Pts',(38.9999999999855,-27.6876355340531,
-135.545932666416));
#159001=CARTESIAN_POINT('Ctrl Pts',(39.7261148635016,-26.9897399838167,
-136.518160398014));
#159002=CARTESIAN_POINT('Ctrl Pts',(39.,-27.350294560115,-133.606110521891));
#159003=CARTESIAN_POINT('Ctrl Pts',(39.,-26.5955422649145,-134.742448815396));
#159004=CARTESIAN_POINT('Ctrl Pts',(39.6916499750401,-25.9410827372237,
-135.719201830687));
#159005=CARTESIAN_POINT('Ctrl Pts',(39.,-24.9455608509554,-132.126282804037));
#159006=CARTESIAN_POINT('Ctrl Pts',(38.9999999999999,-24.3121967691435,
-133.254719568795));
#159007=CARTESIAN_POINT('Ctrl Pts',(39.6264336205064,-23.7540596888349,
-134.239374112649));
#159008=CARTESIAN_POINT('Ctrl Pts',(39.,-23.7105874730482,-131.458602080542));
#159009=CARTESIAN_POINT('Ctrl Pts',(38.9999999999854,-23.1403713306369,
-132.582946581795));
#159010=CARTESIAN_POINT('Ctrl Pts',(39.5962661790751,-22.6346054925691,
-133.57169567032));
#159011=CARTESIAN_POINT('Ctrl Pts',(39.,-22.4346253623973,-130.883024754454));
#159012=CARTESIAN_POINT('Ctrl Pts',(39.,-21.9292251340083,-132.003415558585));
#159013=CARTESIAN_POINT('Ctrl Pts',(39.5698471421185,-21.4814250807741,
-132.996116063158));
#159014=CARTESIAN_POINT('',(39.5912209089345,-22.3752378108182,-133.464034181247));
#159015=CARTESIAN_POINT('',(39.7602371761935,-27.9700233746923,-137.330324614952));
#159016=CARTESIAN_POINT('Ctrl Pts',(39.5912176877287,-22.3752677013603,
-133.463979745435));
#159017=CARTESIAN_POINT('Ctrl Pts',(39.5991937056478,-22.6956823003948,
-133.639446472636));
#159018=CARTESIAN_POINT('Ctrl Pts',(39.607504589464,-23.0161431501768,-133.823227767823));
#159019=CARTESIAN_POINT('Ctrl Pts',(39.6161482430768,-23.3372484672009,
-134.015540725654));
#159020=CARTESIAN_POINT('Ctrl Pts',(39.625740246586,-23.6935842790838,-134.228953554191));
#159021=CARTESIAN_POINT('Ctrl Pts',(39.6357421466937,-24.050713523311,-134.452873202772));
#159022=CARTESIAN_POINT('Ctrl Pts',(39.6461511970428,-24.4094330557747,
-134.687659604986));
#159023=CARTESIAN_POINT('Ctrl Pts',(39.6503809255142,-24.5551991121233,
-134.78306530453));
#159024=CARTESIAN_POINT('Ctrl Pts',(39.6546778750575,-24.7012275599844,
-134.880265972657));
#159025=CARTESIAN_POINT('Ctrl Pts',(39.6590417977732,-24.8475712130293,
-134.979287971668));
#159026=CARTESIAN_POINT('Ctrl Pts',(39.6744840567571,-25.3654256156315,
-135.32968907944));
#159027=CARTESIAN_POINT('Ctrl Pts',(39.6906347977313,-25.8829878852576,
-135.699934267346));
#159028=CARTESIAN_POINT('Ctrl Pts',(39.7075008936637,-26.402609425732,-136.091336282031));
#159029=CARTESIAN_POINT('Ctrl Pts',(39.7200778526961,-26.7900884756006,
-136.383202705867));
#159030=CARTESIAN_POINT('Ctrl Pts',(39.7330525286025,-27.1787101201886,
-136.686837180687));
#159031=CARTESIAN_POINT('Ctrl Pts',(39.7464218716113,-27.5694625249137,
-137.00277640538));
#159032=CARTESIAN_POINT('Ctrl Pts',(39.7509812362623,-27.7027213320365,
-137.110521575203));
#159033=CARTESIAN_POINT('Ctrl Pts',(39.755586444335,-27.8362282160821,-137.219697552064));
#159034=CARTESIAN_POINT('Ctrl Pts',(39.7602371757582,-27.9700234449751,
-137.330324487883));
#159035=CARTESIAN_POINT('Ctrl Pts',(39.5912176308748,-22.3752654174111,
-133.46397849469));
#159036=CARTESIAN_POINT('Ctrl Pts',(39.5704459682015,-22.3771166985369,
-133.421559237108));
#159037=CARTESIAN_POINT('Ctrl Pts',(39.5485259522618,-22.3791109149648,
-133.375464310273));
#159038=CARTESIAN_POINT('Ctrl Pts',(39.5257329435558,-22.3812642489227,
-133.325575012736));
#159039=CARTESIAN_POINT('Ctrl Pts',(39.5072761806346,-22.3830079228213,
-133.285176882378));
#159040=CARTESIAN_POINT('Ctrl Pts',(39.4882478794602,-22.3848559043229,
-133.242290536397));
#159041=CARTESIAN_POINT('Ctrl Pts',(39.4688188799045,-22.3868120470417,
-133.196854321189));
#159042=CARTESIAN_POINT('Ctrl Pts',(39.4471075484527,-22.3889979785824,
-133.146080696666));
#159043=CARTESIAN_POINT('Ctrl Pts',(39.4248951791589,-22.3913193770836,
-133.09212240113));
#159044=CARTESIAN_POINT('Ctrl Pts',(39.4024537571075,-22.3937724613011,
-133.034900572149));
#159045=CARTESIAN_POINT('Ctrl Pts',(39.3912330460818,-22.3949990034098,
-133.006289657658));
#159046=CARTESIAN_POINT('Ctrl Pts',(39.3799556321572,-22.3962582955159,
-132.976863015288));
#159047=CARTESIAN_POINT('Ctrl Pts',(39.3686588779053,-22.3975486744013,
-132.946612030522));
#159048=CARTESIAN_POINT('Ctrl Pts',(39.3630105007794,-22.3981938638439,
-132.931486538139));
#159049=CARTESIAN_POINT('Ctrl Pts',(39.3573573118174,-22.3988468290841,
-132.916154951723));
#159050=CARTESIAN_POINT('Ctrl Pts',(39.3517042042225,-22.3995072548015,
-132.900616324401));
#159051=CARTESIAN_POINT('Ctrl Pts',(39.3488776504251,-22.3998374676602,
-132.892847010739));
#159052=CARTESIAN_POINT('Ctrl Pts',(39.3460511183112,-22.4001695458829,
-132.88502593635));
#159053=CARTESIAN_POINT('Ctrl Pts',(39.3432252304613,-22.4005034472795,
-132.877152986039));
#159054=CARTESIAN_POINT('Ctrl Pts',(39.3418122865364,-22.4006703979778,
-132.873216510883));
#159055=CARTESIAN_POINT('Ctrl Pts',(39.3403995037615,-22.4008378044838,
-132.869267066718));
#159056=CARTESIAN_POINT('Ctrl Pts',(39.3389869607814,-22.4010056611205,
-132.865304639651));
#159057=CARTESIAN_POINT('Ctrl Pts',(39.3375744178012,-22.4011735177572,
-132.861342212583));
#159058=CARTESIAN_POINT('Ctrl Pts',(39.3367132897538,-22.4012759517441,
-132.858923697129));
#159059=CARTESIAN_POINT('Ctrl Pts',(39.3347501303002,-22.4015105756498,
-132.853378395947));
#159060=CARTESIAN_POINT('Ctrl Pts',(39.3150826350157,-22.4038611053285,
-132.79782397593));
#159061=CARTESIAN_POINT('Ctrl Pts',(39.2975369800321,-22.4060800233942,
-132.745592029857));
#159062=CARTESIAN_POINT('Ctrl Pts',(39.281813765163,-22.4081460611799,-132.696818181293));
#159063=CARTESIAN_POINT('Ctrl Pts',(39.2659071443645,-22.4102361985906,
-132.647475402449));
#159064=CARTESIAN_POINT('Ctrl Pts',(39.2518653111442,-22.4121701620292,
-132.601671421479));
#159065=CARTESIAN_POINT('Ctrl Pts',(39.2394145627136,-22.4139389110504,
-132.559509824754));
#159066=CARTESIAN_POINT('Ctrl Pts',(39.2268139559692,-22.4157289488919,
-132.516840767305));
#159067=CARTESIAN_POINT('Ctrl Pts',(39.2158426385727,-22.4173500443747,
-132.477901869192));
#159068=CARTESIAN_POINT('Ctrl Pts',(39.2062595192933,-22.418801719556,-132.442769697218));
#159069=CARTESIAN_POINT('Ctrl Pts',(39.1966374578557,-22.4202592937941,
-132.407494761436));
#159070=CARTESIAN_POINT('Ctrl Pts',(39.1884147146853,-22.4215463105877,
-132.376057135563));
#159071=CARTESIAN_POINT('Ctrl Pts',(39.1813937185977,-22.4226672718763,
-132.348509965414));
#159072=CARTESIAN_POINT('Ctrl Pts',(39.174347612458,-22.4237922421966,-132.320864274931));
#159073=CARTESIAN_POINT('Ctrl Pts',(39.1685117471268,-22.424750159556,-132.297136577662));
#159074=CARTESIAN_POINT('Ctrl Pts',(39.1637353846615,-22.4255473035123,
-132.277361832726));
#159075=CARTESIAN_POINT('Ctrl Pts',(39.1614455703549,-22.4259294586877,
-132.267881711778));
#159076=CARTESIAN_POINT('Ctrl Pts',(39.1593999930064,-22.4262746704984,
-132.259309852597));
#159077=CARTESIAN_POINT('Ctrl Pts',(39.1575861139129,-22.4265835945122,
-132.251648900436));
#159078=CARTESIAN_POINT('Ctrl Pts',(39.1561218222149,-22.4268329798601,
-132.245464437157));
#159079=CARTESIAN_POINT('Ctrl Pts',(39.1548085749677,-22.42705871667,-132.239873584309));
#159080=CARTESIAN_POINT('Ctrl Pts',(39.153641039373,-22.4272611070789,-132.234877417562));
#159081=CARTESIAN_POINT('Ctrl Pts',(39.1530572715757,-22.4273623022833,
-132.232379334188));
#159082=CARTESIAN_POINT('Ctrl Pts',(39.1525099491287,-22.427457662781,-132.23002991835));
#159083=CARTESIAN_POINT('Ctrl Pts',(39.1519985118524,-22.42754721861,-132.227829279993));
#159084=CARTESIAN_POINT('Ctrl Pts',(39.1517427932143,-22.4275919965244,
-132.226728960814));
#159085=CARTESIAN_POINT('Ctrl Pts',(39.1514960469557,-22.4276353233905,
-132.225665835756));
#159086=CARTESIAN_POINT('Ctrl Pts',(39.1512582096618,-22.4276772030782,
-132.224639917171));
#159087=CARTESIAN_POINT('Ctrl Pts',(39.1511392910149,-22.4276981429221,
-132.224126957879));
#159088=CARTESIAN_POINT('Ctrl Pts',(39.1510226000849,-22.427718720953,-132.223623300112));
#159089=CARTESIAN_POINT('Ctrl Pts',(39.1509092053933,-22.4277387590788,
-132.223133603284));
#159090=CARTESIAN_POINT('Ctrl Pts',(39.1507958107018,-22.4277587972047,
-132.222643906455));
#159091=CARTESIAN_POINT('Ctrl Pts',(39.1506832277566,-22.4277786733366,
-132.222158917573));
#159092=CARTESIAN_POINT('Ctrl Pts',(39.1502251980778,-22.42785987834,-132.22017626939));
#159093=CARTESIAN_POINT('Ctrl Pts',(39.1289904035728,-22.4316246377878,
-132.128258368202));
#159094=CARTESIAN_POINT('Ctrl Pts',(39.1105424377617,-22.435323922588,-132.038287095715));
#159095=CARTESIAN_POINT('Ctrl Pts',(39.0945601802243,-22.4389133364673,
-131.950468295162));
#159096=CARTESIAN_POINT('Ctrl Pts',(39.0782303612054,-22.4425808082807,
-131.860739724832));
#159097=CARTESIAN_POINT('Ctrl Pts',(39.0644740620208,-22.4461337419189,
-131.773258146502));
#159098=CARTESIAN_POINT('Ctrl Pts',(39.0529498734261,-22.4495490877257,
-131.688194391823));
#159099=CARTESIAN_POINT('Ctrl Pts',(39.0410276477678,-22.4530823970842,
-131.600192597137));
#159100=CARTESIAN_POINT('Ctrl Pts',(39.0314937928809,-22.4564686204929,
-131.514778400783));
#159101=CARTESIAN_POINT('Ctrl Pts',(39.0239807694142,-22.4597054491932,
-131.432091105995));
#159102=CARTESIAN_POINT('Ctrl Pts',(39.0163143777417,-22.4630083533707,
-131.347715861994));
#159103=CARTESIAN_POINT('Ctrl Pts',(39.0107516622859,-22.4661559629513,
-131.266179646715));
#159104=CARTESIAN_POINT('Ctrl Pts',(39.0069213198967,-22.4691661594339,
-131.187583251473));
#159105=CARTESIAN_POINT('Ctrl Pts',(39.0029761663714,-22.4722665839021,
-131.106630998577));
#159106=CARTESIAN_POINT('Ctrl Pts',(39.0008683301356,-22.475221500718,-131.02879708224));
#159107=CARTESIAN_POINT('Ctrl Pts',(39.0002198458126,-22.4780677464764,
-130.954147392188));
#159108=CARTESIAN_POINT('Ctrl Pts',(39.0000718620453,-22.4787172581995,
-130.937112373806));
#159109=CARTESIAN_POINT('Ctrl Pts',(39.0000000007212,-22.4793611705732,
-130.920243010183));
#159110=CARTESIAN_POINT('Ctrl Pts',(39.,-22.48000002,-130.903539806302));
#159111=CARTESIAN_POINT('Ctrl Pts',(39.0000000022172,-28.13000002,-134.169022080262));
#159112=CARTESIAN_POINT('Ctrl Pts',(39.0000022444212,-28.1256876822484,
-134.257859743399));
#159113=CARTESIAN_POINT('Ctrl Pts',(39.0017029362504,-28.1212246324348,
-134.349811093215));
#159114=CARTESIAN_POINT('Ctrl Pts',(39.0054625728427,-28.1165865787746,
-134.444817027622));
#159115=CARTESIAN_POINT('Ctrl Pts',(39.0069704165467,-28.1147264362214,
-134.48292020502));
#159116=CARTESIAN_POINT('Ctrl Pts',(39.0088097443042,-28.1128384071593,
-134.521514303064));
#159117=CARTESIAN_POINT('Ctrl Pts',(39.0110049637423,-28.1109220758294,
-134.560593760958));
#159118=CARTESIAN_POINT('Ctrl Pts',(39.0148393383217,-28.1075748331758,
-134.628853579237));
#159119=CARTESIAN_POINT('Ctrl Pts',(39.0197592533743,-28.104140802429,-134.698594823325));
#159120=CARTESIAN_POINT('Ctrl Pts',(39.0258989313664,-28.1006234906337,
-134.769779548678));
#159121=CARTESIAN_POINT('Ctrl Pts',(39.0289687703624,-28.0988648347361,
-134.805371911355));
#159122=CARTESIAN_POINT('Ctrl Pts',(39.0323436499559,-28.097085364818,-134.841325135559));
#159123=CARTESIAN_POINT('Ctrl Pts',(39.036040744954,-28.0952864067033,-134.877633224531));
#159124=CARTESIAN_POINT('Ctrl Pts',(39.0378892924531,-28.0943869276459,
-134.895787269017));
#159125=CARTESIAN_POINT('Ctrl Pts',(39.0398183990165,-28.0934825767865,
-134.914030029345));
#159126=CARTESIAN_POINT('Ctrl Pts',(39.0418302364931,-28.0925735524499,
-134.932360712653));
#159127=CARTESIAN_POINT('Ctrl Pts',(39.0428361552314,-28.0921190402817,
-134.941526054307));
#159128=CARTESIAN_POINT('Ctrl Pts',(39.0438627570247,-28.0916633597697,
-134.950713376669));
#159129=CARTESIAN_POINT('Ctrl Pts',(39.0449103145788,-28.0912065389918,
-134.959922576108));
#159130=CARTESIAN_POINT('Ctrl Pts',(39.0454340933558,-28.0909781286029,
-134.964527175827));
#159131=CARTESIAN_POINT('Ctrl Pts',(39.0459631110927,-28.090749433149,-134.969137244813));
#159132=CARTESIAN_POINT('Ctrl Pts',(39.0464974019454,-28.0905204563639,
-134.973752769806));
#159133=CARTESIAN_POINT('Ctrl Pts',(39.0470316927981,-28.0902914795789,
-134.9783682948));
#159134=CARTESIAN_POINT('Ctrl Pts',(39.0477179000727,-28.0900004456395,
-134.984234402956));
#159135=CARTESIAN_POINT('Ctrl Pts',(39.0481161280684,-28.0898326858219,
-134.987615699453));
#159136=CARTESIAN_POINT('Ctrl Pts',(39.0550934125024,-28.08689339482,-135.046858815623));
#159137=CARTESIAN_POINT('Ctrl Pts',(39.0632889714829,-28.0837723561849,
-135.109990104035));
#159138=CARTESIAN_POINT('Ctrl Pts',(39.0730296264029,-28.0804454103404,
-135.176965171389));
#159139=CARTESIAN_POINT('Ctrl Pts',(39.0824823950805,-28.0772167927854,
-135.241960782471));
#159140=CARTESIAN_POINT('Ctrl Pts',(39.0933906084473,-28.0737939047369,
-135.310576693437));
#159141=CARTESIAN_POINT('Ctrl Pts',(39.1060896137435,-28.0701698336421,
-135.382744720427));
#159142=CARTESIAN_POINT('Ctrl Pts',(39.1161545441063,-28.0672974808596,
-135.439943386712));
#159143=CARTESIAN_POINT('Ctrl Pts',(39.1273451751191,-28.0642989515184,
-135.499372979695));
#159144=CARTESIAN_POINT('Ctrl Pts',(39.1398433469704,-28.0611802471452,
-135.56098419753));
#159145=CARTESIAN_POINT('Ctrl Pts',(39.1472627659542,-28.0593288584215,
-135.597559101817));
#159146=CARTESIAN_POINT('Ctrl Pts',(39.1551432186097,-28.0574352910613,
-135.634902556301));
#159147=CARTESIAN_POINT('Ctrl Pts',(39.163524700022,-28.0555025618695,-135.673001567496));
#159148=CARTESIAN_POINT('Ctrl Pts',(39.1677154407281,-28.0545361972736,
-135.692051073094));
#159149=CARTESIAN_POINT('Ctrl Pts',(39.1720314685517,-28.0535600468933,
-135.711289461438));
#159150=CARTESIAN_POINT('Ctrl Pts',(39.176477895301,-28.052574648591,-135.730714871549));
#159151=CARTESIAN_POINT('Ctrl Pts',(39.1787011086756,-28.0520819494398,
-135.740427576604));
#159152=CARTESIAN_POINT('Ctrl Pts',(39.180956923569,-28.051586938574,-135.750187036735));
#159153=CARTESIAN_POINT('Ctrl Pts',(39.1832459874,-28.0510896896912,-135.759993010319));
#159154=CARTESIAN_POINT('Ctrl Pts',(39.1843905193155,-28.0508410652498,
-135.764895997111));
#159155=CARTESIAN_POINT('Ctrl Pts',(39.1855433635767,-28.0505918813225,
-135.769810612242));
#159156=CARTESIAN_POINT('Ctrl Pts',(39.1867046015345,-28.050342147721,-135.774736824644));
#159157=CARTESIAN_POINT('Ctrl Pts',(39.1872852205135,-28.0502172809202,
-135.777199930845));
#159158=CARTESIAN_POINT('Ctrl Pts',(39.1878679379234,-28.050092276702,-135.779665936363));
#159159=CARTESIAN_POINT('Ctrl Pts',(39.1884527639581,-28.0499671363333,
-135.782134837256));
#159160=CARTESIAN_POINT('Ctrl Pts',(39.1890375899928,-28.0498419959645,
-135.784603738149));
#159161=CARTESIAN_POINT('Ctrl Pts',(39.1893301170433,-28.0497793997691,
-135.7858386911));
#159162=CARTESIAN_POINT('Ctrl Pts',(39.1902135781519,-28.0495913080571,
-135.7895502221));
#159163=CARTESIAN_POINT('Ctrl Pts',(39.2059227393946,-28.0462467770936,
-135.855546380124));
#159164=CARTESIAN_POINT('Ctrl Pts',(39.221650020651,-28.0430713006495,-135.917319405468));
#159165=CARTESIAN_POINT('Ctrl Pts',(39.2370526053371,-28.0400995402759,
-135.974902972362));
#159166=CARTESIAN_POINT('Ctrl Pts',(39.2526423857115,-28.0370916625402,
-136.033186382538));
#159167=CARTESIAN_POINT('Ctrl Pts',(39.267899310265,-28.034292087431,-136.087178424114));
#159168=CARTESIAN_POINT('Ctrl Pts',(39.2825152847821,-28.0317169129634,
-136.136928250427));
#159169=CARTESIAN_POINT('Ctrl Pts',(39.2973176181395,-28.0291089041111,
-136.187312404608));
#159170=CARTESIAN_POINT('Ctrl Pts',(39.311462418526,-28.0267306714006,-136.233345984635));
#159171=CARTESIAN_POINT('Ctrl Pts',(39.324680631343,-28.024584655685,-136.275086526027));
#159172=CARTESIAN_POINT('Ctrl Pts',(39.3379570787827,-28.0224291854071,
-136.317010961014));
#159173=CARTESIAN_POINT('Ctrl Pts',(39.3502987596337,-28.020507625517,-136.354604895132));
#159174=CARTESIAN_POINT('Ctrl Pts',(39.3614850041212,-28.0188137834241,
-136.387925840271));
#159175=CARTESIAN_POINT('Ctrl Pts',(39.3727121720073,-28.0171137446335,
-136.421368685688));
#159176=CARTESIAN_POINT('Ctrl Pts',(39.3827754798058,-28.0156427969912,
-136.450507583106));
#159177=CARTESIAN_POINT('Ctrl Pts',(39.3915036402467,-28.0143909018923,
-136.475393771548));
#159178=CARTESIAN_POINT('Ctrl Pts',(39.3940272651179,-28.0140289340264,
-136.482589263029));
#159179=CARTESIAN_POINT('Ctrl Pts',(39.3964395993417,-28.0136852698651,
-136.489429167449));
#159180=CARTESIAN_POINT('Ctrl Pts',(39.3987372963114,-28.0133596580246,
-136.495914555584));
#159181=CARTESIAN_POINT('Ctrl Pts',(39.405657219105,-28.0123790200961,-136.515446454598));
#159182=CARTESIAN_POINT('Ctrl Pts',(39.4115352343368,-28.0115620234741,
-136.531763419977));
#159183=CARTESIAN_POINT('Ctrl Pts',(39.4162991112997,-28.010902423024,-136.544889594268));
#159184=CARTESIAN_POINT('Ctrl Pts',(39.4186810497811,-28.010572622799,-136.551452681414));
#159185=CARTESIAN_POINT('Ctrl Pts',(39.420784901807,-28.0102821911499,-136.557217945173));
#159186=CARTESIAN_POINT('Ctrl Pts',(39.4226043068137,-28.010030508285,-136.562187596028));
#159187=CARTESIAN_POINT('Ctrl Pts',(39.423514009317,-28.0099046668525,-136.564672421456));
#159188=CARTESIAN_POINT('Ctrl Pts',(39.4243526262731,-28.0097885194934,
-136.5669583344));
#159189=CARTESIAN_POINT('Ctrl Pts',(39.4251195294557,-28.0096819964926,
-136.56904555736));
#159190=CARTESIAN_POINT('Ctrl Pts',(39.425502981047,-28.0096287349923,-136.57008916884));
#159191=CARTESIAN_POINT('Ctrl Pts',(39.4258685058372,-28.0095778800107,
-136.571083107247));
#159192=CARTESIAN_POINT('Ctrl Pts',(39.4262160353219,-28.0095294246206,
-136.572027396811));
#159193=CARTESIAN_POINT('Ctrl Pts',(39.4263898000642,-28.0095051969255,
-136.572499541593));
#159194=CARTESIAN_POINT('Ctrl Pts',(39.4265590665073,-28.0094815691999,
-136.572959273977));
#159195=CARTESIAN_POINT('Ctrl Pts',(39.4267215489531,-28.0094588375901,
-136.573400400812));
#159196=CARTESIAN_POINT('Ctrl Pts',(39.4268840313989,-28.0094361059803,
-136.573841527647));
#159197=CARTESIAN_POINT('Ctrl Pts',(39.4270438833707,-28.0094136336851,
-136.574276585042));
#159198=CARTESIAN_POINT('Ctrl Pts',(39.4278967242282,-28.009294249711,-136.576588215794));
#159199=CARTESIAN_POINT('Ctrl Pts',(39.4596149084087,-28.0048542151545,
-136.662560562586));
#159200=CARTESIAN_POINT('Ctrl Pts',(39.4919257606152,-28.0005742974956,
-136.744743249651));
#159201=CARTESIAN_POINT('Ctrl Pts',(39.5244183422418,-27.9964886368414,
-136.82314195696));
#159202=CARTESIAN_POINT('Ctrl Pts',(39.557501220046,-27.9923287515567,-136.902964941902));
#159203=CARTESIAN_POINT('Ctrl Pts',(39.5907720426126,-27.9883699287563,
-136.978865697753));
#159204=CARTESIAN_POINT('Ctrl Pts',(39.6238294631346,-27.9846169757305,
-137.050881414756));
#159205=CARTESIAN_POINT('Ctrl Pts',(39.6577842812835,-27.9807621426705,
-137.124852115921));
#159206=CARTESIAN_POINT('Ctrl Pts',(39.6915135537608,-27.9771241573282,
-137.194724506443));
#159207=CARTESIAN_POINT('Ctrl Pts',(39.7246228724876,-27.973680678008,-137.260563754943));
#159208=CARTESIAN_POINT('Ctrl Pts',(39.7365804986175,-27.972437045101,-137.284341988641));
#159209=CARTESIAN_POINT('Ctrl Pts',(39.7484576652078,-27.9712185539927,
-137.307594356029));
#159210=CARTESIAN_POINT('Ctrl Pts',(39.7602371757582,-27.9700234449751,
-137.330324487883));
#159211=CARTESIAN_POINT('Origin',(0.,-12.9675000200281,-171.64995));
#159212=CARTESIAN_POINT('',(56.4351108624337,-28.0132652467914,-171.449026400902));
#159213=CARTESIAN_POINT('',(57.638503474757,-22.4067641070473,-171.449026400902));
#159214=CARTESIAN_POINT('Origin',(0.,-12.9675000200281,-171.449026400902));
#159215=CARTESIAN_POINT('Ctrl Pts',(57.638503474757,-22.4067641070473,-171.449026400902));
#159216=CARTESIAN_POINT('Ctrl Pts',(56.0174734274339,-22.4047732541902,
-168.017725527675));
#159217=CARTESIAN_POINT('Ctrl Pts',(54.4570351795732,-22.4027901572724,
-164.718389532589));
#159218=CARTESIAN_POINT('Ctrl Pts',(52.2072906835069,-22.399520061464,-159.96733285717));
#159219=CARTESIAN_POINT('Ctrl Pts',(51.4725275267282,-22.3983876189532,
-158.416638518232));
#159220=CARTESIAN_POINT('Ctrl Pts',(50.3931082416263,-22.3966483219777,
-156.140083839128));
#159221=CARTESIAN_POINT('Ctrl Pts',(49.8590798993526,-22.3957691535144,
-155.014178206902));
#159222=CARTESIAN_POINT('Ctrl Pts',(49.2459879385832,-22.3947385586366,
-153.722272123792));
#159223=CARTESIAN_POINT('Ctrl Pts',(48.9419270289921,-22.3942240082935,
-153.081731704191));
#159224=CARTESIAN_POINT('Ctrl Pts',(48.7715916624419,-22.3939350767465,
-152.722950018091));
#159225=CARTESIAN_POINT('Ctrl Pts',(48.6879979444904,-22.3937931129051,
-152.546890421963));
#159226=CARTESIAN_POINT('Ctrl Pts',(48.6449082650321,-22.3937199051624,
-152.456141770449));
#159227=CARTESIAN_POINT('Ctrl Pts',(48.6427494969204,-22.3937162374209,
-152.451595325367));
#159228=CARTESIAN_POINT('Ctrl Pts',(45.3353322790861,-22.3880967559532,
-145.486078532289));
#159229=CARTESIAN_POINT('Ctrl Pts',(42.3192392814167,-22.3819993338137,
-139.159156692962));
#159230=CARTESIAN_POINT('Ctrl Pts',(39.5912209089345,-22.3752378108182,
-133.464034181247));
#159231=CARTESIAN_POINT('Ctrl Pts',(39.7602371906927,-27.9700232578782,
-137.330324735012));
#159232=CARTESIAN_POINT('Ctrl Pts',(41.0440760495002,-27.9745032276897,
-139.909644963587));
#159233=CARTESIAN_POINT('Ctrl Pts',(42.3849915594275,-27.9790517553505,
-142.618821730253));
#159234=CARTESIAN_POINT('Ctrl Pts',(44.4821817835909,-27.9852985070288,
-146.877371687389));
#159235=CARTESIAN_POINT('Ctrl Pts',(45.1955448675102,-27.987298498321,-148.329352474291));
#159236=CARTESIAN_POINT('Ctrl Pts',(46.2870402618014,-27.9902150737621,
-150.556019856428));
#159237=CARTESIAN_POINT('Ctrl Pts',(46.8381504361392,-27.9916538177842,
-151.681527597942));
#159238=CARTESIAN_POINT('Ctrl Pts',(47.4904948539634,-27.9933207698379,
-153.015924551323));
#159239=CARTESIAN_POINT('Ctrl Pts',(47.8190123404997,-27.9941552160743,
-153.688449175084));
#159240=CARTESIAN_POINT('Ctrl Pts',(48.0015193211533,-27.9946179773477,
-154.06221379323));
#159241=CARTESIAN_POINT('Ctrl Pts',(48.0900254381751,-27.9948422372974,
-154.243513467762));
#159242=CARTESIAN_POINT('Ctrl Pts',(48.137277552473,-27.9949619482672,-154.34031758891));
#159243=CARTESIAN_POINT('Ctrl Pts',(48.144080578613,-27.9949791830011,-154.354255016688));
#159244=CARTESIAN_POINT('Ctrl Pts',(50.7155543787194,-28.0014936334107,
-159.622532560907));
#159245=CARTESIAN_POINT('Ctrl Pts',(53.477513591401,-28.0075945743212,-165.317366506688));
#159246=CARTESIAN_POINT('Ctrl Pts',(56.4351108624337,-28.0132652467914,
-171.449026400902));
#159247=CARTESIAN_POINT('Origin',(60.,-29.13000002,-176.84995));
#159248=CARTESIAN_POINT('',(56.7430488584365,-29.13000002,-177.34995));
#159249=CARTESIAN_POINT('',(57.,-29.13000002,-177.34995));
#159250=CARTESIAN_POINT('',(60.,-29.13000002,-177.34995));
#159251=CARTESIAN_POINT('',(57.,-28.664523125878,-177.032518510534));
#159252=CARTESIAN_POINT('Ctrl Pts',(56.7430488584365,-29.13000002,-177.34995));
#159253=CARTESIAN_POINT('Ctrl Pts',(56.7774215329782,-29.0696624994766,
-177.34995));
#159254=CARTESIAN_POINT('Ctrl Pts',(56.8073315614797,-29.0157589594499,
-177.339097737931));
#159255=CARTESIAN_POINT('Ctrl Pts',(56.8455026351718,-28.947352143821,-177.316017469029));
#159256=CARTESIAN_POINT('Ctrl Pts',(56.8571106648925,-28.9265627510565,
-177.30717515183));
#159257=CARTESIAN_POINT('Ctrl Pts',(56.8728492172084,-28.8983280728031,
-177.293163830275));
#159258=CARTESIAN_POINT('Ctrl Pts',(56.8803001203001,-28.8849448328683,
-177.285968499567));
#159259=CARTESIAN_POINT('Ctrl Pts',(56.8882606877078,-28.8705728009652,
-177.277425887854));
#159260=CARTESIAN_POINT('Ctrl Pts',(56.8915154695541,-28.8646735743065,
-177.273750819397));
#159261=CARTESIAN_POINT('Ctrl Pts',(56.8936504596961,-28.8607979147461,
-177.271299598116));
#159262=CARTESIAN_POINT('Ctrl Pts',(56.8941472201129,-28.8598965492813,
-177.270730233962));
#159263=CARTESIAN_POINT('Ctrl Pts',(56.9464830121473,-28.7645629228455,
-177.208602031531));
#159264=CARTESIAN_POINT('Ctrl Pts',(56.9812386277457,-28.6996278422223,
-177.122021537563));
#159265=CARTESIAN_POINT('Ctrl Pts',(57.,-28.664523125878,-177.032518510534));
#159266=CARTESIAN_POINT('Origin',(57.,-29.13000002,-176.84995));
#159267=CARTESIAN_POINT('Origin',(60.,-2.55003103885676E-14,0.));
#159268=CARTESIAN_POINT('',(60.,-29.13000002,-58.24995));
#159269=CARTESIAN_POINT('',(60.,-29.63000002,-58.24995));
#159270=CARTESIAN_POINT('',(60.,-54.58000002,-58.24995));
#159271=CARTESIAN_POINT('',(60.,-29.63000002,-174.34995));
#159272=CARTESIAN_POINT('',(60.,-29.63000002,-174.34995));
#159273=CARTESIAN_POINT('',(60.,-29.13000002,-174.34995));
#159274=CARTESIAN_POINT('',(60.,28.41999998,-174.34995));
#159275=CARTESIAN_POINT('',(60.,-29.13000002,-58.24995));
#159276=CARTESIAN_POINT('Origin',(57.,-2.42462934179819E-14,-174.34995));
#159277=CARTESIAN_POINT('',(57.,-29.63000002,-177.34995));
#159278=CARTESIAN_POINT('Origin',(57.,-29.63000002,-174.34995));
#159279=CARTESIAN_POINT('',(57.,-54.58000002,-177.34995));
#159280=CARTESIAN_POINT('Origin',(57.,-29.13000002,-174.34995));
#159281=CARTESIAN_POINT('Origin',(60.,28.41999998,-177.34995));
#159282=CARTESIAN_POINT('',(56.5982428503831,-29.63000002,-177.34995));
#159283=CARTESIAN_POINT('',(60.,-29.63000002,-177.34995));
#159284=CARTESIAN_POINT('Origin',(0.,-12.9675000200281,-177.34995));
#159285=CARTESIAN_POINT('Origin',(57.,-2.42462934179819E-14,-174.34995));
#159286=CARTESIAN_POINT('',(60.,-37.78000002,-174.34995));
#159287=CARTESIAN_POINT('',(60.,-37.28000002,-174.34995));
#159288=CARTESIAN_POINT('',(60.,28.41999998,-174.34995));
#159289=CARTESIAN_POINT('',(57.,-37.78000002,-177.34995));
#159290=CARTESIAN_POINT('Origin',(57.,-37.78000002,-174.34995));
#159291=CARTESIAN_POINT('',(57.,-37.28000002,-177.34995));
#159292=CARTESIAN_POINT('',(57.,-54.58000002,-177.34995));
#159293=CARTESIAN_POINT('Origin',(57.,-37.28000002,-174.34995));
#159294=CARTESIAN_POINT('Origin',(39.,46.91999998,-129.34995));
#159295=CARTESIAN_POINT('',(39.,-30.63000002,-96.0164973302555));
#159296=CARTESIAN_POINT('',(39.0000000003234,-36.28000002,-90.9091273827666));
#159297=CARTESIAN_POINT('Ctrl Pts',(39.,-30.63000002,-96.0164973302555));
#159298=CARTESIAN_POINT('Ctrl Pts',(39.0000000000004,-31.0448154973607,
-95.6851069386958));
#159299=CARTESIAN_POINT('Ctrl Pts',(39.0000000000118,-31.454211737686,-95.3480909235777));
#159300=CARTESIAN_POINT('Ctrl Pts',(39.0000000000377,-31.8588908811793,
-95.0057530542704));
#159301=CARTESIAN_POINT('Ctrl Pts',(39.0000000000646,-32.2780518714171,
-94.6511642828895));
#159302=CARTESIAN_POINT('Ctrl Pts',(39.0000000001072,-32.6921518967125,
-94.2908656551258));
#159303=CARTESIAN_POINT('Ctrl Pts',(39.0000000001713,-33.1019373671843,
-93.9251487646761));
#159304=CARTESIAN_POINT('Ctrl Pts',(39.0000000002394,-33.5373888366211,
-93.5365260124815));
#159305=CARTESIAN_POINT('Ctrl Pts',(39.0000000003318,-33.9679681800838,
-93.1417847771912));
#159306=CARTESIAN_POINT('Ctrl Pts',(39.0000000004578,-34.394536385264,-92.7412278681602));
#159307=CARTESIAN_POINT('Ctrl Pts',(39.0000000004786,-34.4649233358098,
-92.6751329764071));
#159308=CARTESIAN_POINT('Ctrl Pts',(39.0000000005003,-34.5352010051139,
-92.6088796459859));
#159309=CARTESIAN_POINT('Ctrl Pts',(39.000000000523,-34.605373184231,-92.5424691324455));
#159310=CARTESIAN_POINT('Ctrl Pts',(39.0000000006715,-35.0646606142243,
-92.1078023674648));
#159311=CARTESIAN_POINT('Ctrl Pts',(39.0000000008613,-35.5177770523147,
-91.6679502775283));
#159312=CARTESIAN_POINT('Ctrl Pts',(39.0000000011092,-35.965637218633,-91.2230746458943));
#159313=CARTESIAN_POINT('Ctrl Pts',(39.0000000011674,-36.0707105045093,
-91.1187015671131));
#159314=CARTESIAN_POINT('Ctrl Pts',(39.0000000012288,-36.1754942796337,
-91.0140518532023));
#159315=CARTESIAN_POINT('Ctrl Pts',(39.0000000012937,-36.28000002,-90.9091273827667));
#159316=CARTESIAN_POINT('',(39.000000000323,-36.28000002,-141.149515588739));
#159317=CARTESIAN_POINT('',(39.,-36.28000002,-129.34995));
#159318=CARTESIAN_POINT('',(39.,-30.63000002,-136.04214564125));
#159319=CARTESIAN_POINT('Ctrl Pts',(39.0000000012919,-36.28000002,-141.149515588739));
#159320=CARTESIAN_POINT('Ctrl Pts',(39.0000000010156,-35.8345332337807,
-140.702263921253));
#159321=CARTESIAN_POINT('Ctrl Pts',(39.0000000008023,-35.3840176213704,
-140.260002181405));
#159322=CARTESIAN_POINT('Ctrl Pts',(39.0000000006337,-34.9275493437281,
-139.822886348187));
#159323=CARTESIAN_POINT('Ctrl Pts',(39.0000000005941,-34.8204877683625,
-139.720363758965));
#159324=CARTESIAN_POINT('Ctrl Pts',(39.0000000005571,-34.7130985462057,
-139.618124369441));
#159325=CARTESIAN_POINT('Ctrl Pts',(39.0000000005223,-34.6053696556424,
-139.516170434427));
#159326=CARTESIAN_POINT('Ctrl Pts',(39.0000000003866,-34.1849244503587,
-139.118263773436));
#159327=CARTESIAN_POINT('Ctrl Pts',(39.0000000002855,-33.7606942182172,
-138.725996583523));
#159328=CARTESIAN_POINT('Ctrl Pts',(39.0000000002095,-33.3318521218407,
-138.339654688119));
#159329=CARTESIAN_POINT('Ctrl Pts',(39.0000000001368,-32.9217240241196,
-137.970172149043));
#159330=CARTESIAN_POINT('Ctrl Pts',(39.000000000087,-32.5073780350574,-137.606108713954));
#159331=CARTESIAN_POINT('Ctrl Pts',(39.0000000000541,-32.0880629354937,
-137.2477524174));
#159332=CARTESIAN_POINT('Ctrl Pts',(39.0000000000227,-31.6891890379909,
-136.906865640726));
#159333=CARTESIAN_POINT('Ctrl Pts',(39.0000000000065,-31.2858188263214,
-136.571142959571));
#159334=CARTESIAN_POINT('Ctrl Pts',(39.0000000000016,-30.8772772477696,
-136.240870924199));
#159335=CARTESIAN_POINT('Ctrl Pts',(39.0000000000006,-30.7950629151777,
-136.174407444378));
#159336=CARTESIAN_POINT('Ctrl Pts',(39.0000000000001,-30.7126390581746,
-136.108164834635));
#159337=CARTESIAN_POINT('Ctrl Pts',(39.,-30.63000002,-136.04214564125));
#159338=CARTESIAN_POINT('',(39.,-30.63000002,-129.34995));
#159339=CARTESIAN_POINT('Ctrl Pts',(39.,-38.3588510407228,-143.307942286761));
#159340=CARTESIAN_POINT('Ctrl Pts',(39.,-37.0899493427105,-144.4917610531));
#159341=CARTESIAN_POINT('Ctrl Pts',(40.0751063896396,-36.0938885093696,
-145.421033595465));
#159342=CARTESIAN_POINT('Ctrl Pts',(39.,-37.1517836400886,-142.014121037894));
#159343=CARTESIAN_POINT('Ctrl Pts',(39.,-35.9377773398718,-143.195151285356));
#159344=CARTESIAN_POINT('Ctrl Pts',(40.0284942517968,-34.9676084789312,
-144.127227814579));
#159345=CARTESIAN_POINT('Ctrl Pts',(39.,-35.9043030651865,-140.745333283629));
#159346=CARTESIAN_POINT('Ctrl Pts',(38.9999999999999,-34.7456377245003,
-141.920028658586));
#159347=CARTESIAN_POINT('Ctrl Pts',(39.98110816979,-33.8078877259523,-142.858424592381));
#159348=CARTESIAN_POINT('Ctrl Pts',(39.,-33.3065355961441,-138.286902604304));
#159349=CARTESIAN_POINT('Ctrl Pts',(39.,-32.2660355551645,-139.44936091542));
#159350=CARTESIAN_POINT('Ctrl Pts',(39.8860349079144,-31.4034486206149,
-140.399993912959));
#159351=CARTESIAN_POINT('Ctrl Pts',(39.,-31.969482004655,-137.109613636004));
#159352=CARTESIAN_POINT('Ctrl Pts',(39.,-30.9915363473202,-138.26565762591));
#159353=CARTESIAN_POINT('Ctrl Pts',(39.838820917574,-30.1709959811911,-139.222722930622));
#159354=CARTESIAN_POINT('Ctrl Pts',(39.,-30.5806161032665,-136.00274102598));
#159355=CARTESIAN_POINT('Ctrl Pts',(38.9999999999999,-29.666065684619,-137.150287618997));
#159356=CARTESIAN_POINT('Ctrl Pts',(39.7930043034378,-28.8965637495112,
-138.115832334683));
#159357=CARTESIAN_POINT('',(39.8501336360982,-30.4479678253697,-139.515614761957));
#159358=CARTESIAN_POINT('',(40.073447192122,-36.0537915982708,-145.374999599156));
#159359=CARTESIAN_POINT('Ctrl Pts',(39.8501516349467,-30.4480624613224,
-139.515559008888));
#159360=CARTESIAN_POINT('Ctrl Pts',(39.8682496030913,-30.928479243834,-139.964932207816));
#159361=CARTESIAN_POINT('Ctrl Pts',(39.8867711495951,-31.4107613119204,
-140.430651260819));
#159362=CARTESIAN_POINT('Ctrl Pts',(39.9057043691656,-31.8961926581865,
-140.913553018237));
#159363=CARTESIAN_POINT('Ctrl Pts',(39.9148973085922,-32.131891660429,-141.148023790015));
#159364=CARTESIAN_POINT('Ctrl Pts',(39.9241871517812,-32.3683334399629,
-141.386545178378));
#159365=CARTESIAN_POINT('Ctrl Pts',(39.9335715388522,-32.6056681732837,
-141.62920925267));
#159366=CARTESIAN_POINT('Ctrl Pts',(39.9498531623278,-33.0174366496215,
-142.050223971987));
#159367=CARTESIAN_POINT('Ctrl Pts',(39.9663641156002,-33.4304553032117,
-142.482261868868));
#159368=CARTESIAN_POINT('Ctrl Pts',(39.9831005766346,-33.8452748182043,
-142.925794853778));
#159369=CARTESIAN_POINT('Ctrl Pts',(39.9978992507961,-34.2120655528516,
-143.317974545175));
#159370=CARTESIAN_POINT('Ctrl Pts',(40.0128742075591,-34.5802637197622,
-143.719141833042));
#159371=CARTESIAN_POINT('Ctrl Pts',(40.028018889995,-34.950251571756,-144.129584741671));
#159372=CARTESIAN_POINT('Ctrl Pts',(40.0429991025759,-35.3162213897886,
-144.535570278154));
#159373=CARTESIAN_POINT('Ctrl Pts',(40.058145417947,-35.6839417083337,-144.950631978182));
#159374=CARTESIAN_POINT('Ctrl Pts',(40.0734472049714,-36.0537916893395,
-145.374999488024));
#159375=CARTESIAN_POINT('Ctrl Pts',(39.8501336360982,-30.4479678253697,
-139.515614761957));
#159376=CARTESIAN_POINT('Ctrl Pts',(39.8191622083133,-30.4511037081781,
-139.457491138984));
#159377=CARTESIAN_POINT('Ctrl Pts',(39.7879243927985,-30.4543702018603,
-139.396870134181));
#159378=CARTESIAN_POINT('Ctrl Pts',(39.7566167914735,-30.4577697087166,
-139.333684763231));
#159379=CARTESIAN_POINT('Ctrl Pts',(39.725300593464,-30.461170149036,-139.27048204235));
#159380=CARTESIAN_POINT('Ctrl Pts',(39.6939201493324,-30.4646865160787,
-139.204710898193));
#159381=CARTESIAN_POINT('Ctrl Pts',(39.6626726151794,-30.4683465195869,
-139.136305569412));
#159382=CARTESIAN_POINT('Ctrl Pts',(39.6314250810264,-30.472006523095,-139.067900240632));
#159383=CARTESIAN_POINT('Ctrl Pts',(39.6003118730321,-30.4758126014794,
-138.996864100184));
#159384=CARTESIAN_POINT('Ctrl Pts',(39.5695612146119,-30.4797609358057,
-138.923160316523));
#159385=CARTESIAN_POINT('Ctrl Pts',(39.5541858854018,-30.4817351029688,
-138.886308424692));
#159386=CARTESIAN_POINT('Ctrl Pts',(39.5389014254943,-30.4837445705845,
-138.848789863091));
#159387=CARTESIAN_POINT('Ctrl Pts',(39.5237375144895,-30.4857871269164,
-138.810601657135));
#159388=CARTESIAN_POINT('Ctrl Pts',(39.5161555589871,-30.4868084050824,
-138.791507554157));
#159389=CARTESIAN_POINT('Ctrl Pts',(39.5086037389925,-30.4878379536194,
-138.772246042189));
#159390=CARTESIAN_POINT('Ctrl Pts',(39.5010858288046,-30.4888753565829,
-138.752816883547));
#159391=CARTESIAN_POINT('Ctrl Pts',(39.4973268737106,-30.4893940580646,
-138.743102304227));
#159392=CARTESIAN_POINT('Ctrl Pts',(39.4935763957452,-30.4899147229967,
-138.733345813422));
#159393=CARTESIAN_POINT('Ctrl Pts',(39.4898348670455,-30.4904372946442,
-138.723547386211));
#159394=CARTESIAN_POINT('Ctrl Pts',(39.4879641026957,-30.4906985804679,
-138.718648172605));
#159395=CARTESIAN_POINT('Ctrl Pts',(39.486095575638,-30.4909603429601,-138.713738474911));
#159396=CARTESIAN_POINT('Ctrl Pts',(39.4842293450209,-30.491222574526,-138.708818290504));
#159397=CARTESIAN_POINT('Ctrl Pts',(39.4832962297124,-30.491353690309,-138.7063581983));
#159398=CARTESIAN_POINT('Ctrl Pts',(39.4823636885123,-30.4914849233598,
-138.70389548442));
#159399=CARTESIAN_POINT('Ctrl Pts',(39.4814317288226,-30.4916162726957,
-138.701430148567));
#159400=CARTESIAN_POINT('Ctrl Pts',(39.480499769133,-30.4917476220316,-138.698964812714));
#159401=CARTESIAN_POINT('Ctrl Pts',(39.4791346823167,-30.491940398823,-138.69534566852));
#159402=CARTESIAN_POINT('Ctrl Pts',(39.4786376016852,-30.4920106685648,
-138.694026274808));
#159403=CARTESIAN_POINT('Ctrl Pts',(39.4658888577959,-30.4938128931618,
-138.660187473907));
#159404=CARTESIAN_POINT('Ctrl Pts',(39.4517135693882,-30.4958331216217,
-138.621772379626));
#159405=CARTESIAN_POINT('Ctrl Pts',(39.436343196791,-30.4980914029818,-138.578720983754));
#159406=CARTESIAN_POINT('Ctrl Pts',(39.4206728558649,-30.5003937569811,
-138.534829396455));
#159407=CARTESIAN_POINT('Ctrl Pts',(39.4037603945031,-30.5029435136479,
-138.486118765703));
#159408=CARTESIAN_POINT('Ctrl Pts',(39.3859029566423,-30.5057633173538,
-138.432509027361));
#159409=CARTESIAN_POINT('Ctrl Pts',(39.3775676371762,-30.5070795176342,
-138.407485600201));
#159410=CARTESIAN_POINT('Ctrl Pts',(39.3690271533864,-30.5084545769865,
-138.381394552734));
#159411=CARTESIAN_POINT('Ctrl Pts',(39.3603153951006,-30.5098909286504,
-138.354226571495));
#159412=CARTESIAN_POINT('Ctrl Pts',(39.3401293576112,-30.5132191027784,
-138.291275572419));
#159413=CARTESIAN_POINT('Ctrl Pts',(39.3190231670336,-30.5168728189609,
-138.222549326763));
#159414=CARTESIAN_POINT('Ctrl Pts',(39.2974832707415,-30.5208429798159,
-138.147968464029));
#159415=CARTESIAN_POINT('Ctrl Pts',(39.2946500754201,-30.5213651847981,
-138.138158660467));
#159416=CARTESIAN_POINT('Ctrl Pts',(39.2918094470411,-30.5218928638335,
-138.128247546444));
#159417=CARTESIAN_POINT('Ctrl Pts',(39.2889625545045,-30.5224259954821,
-138.118234922939));
#159418=CARTESIAN_POINT('Ctrl Pts',(39.2767170922724,-30.5247191777443,
-138.075167191581));
#159419=CARTESIAN_POINT('Ctrl Pts',(39.2643559286661,-30.5271124131941,
-138.030222414249));
#159420=CARTESIAN_POINT('Ctrl Pts',(39.2519774397925,-30.5295977664338,
-137.983390722815));
#159421=CARTESIAN_POINT('Ctrl Pts',(39.2457881953557,-30.5308404430536,
-137.959974877098));
#159422=CARTESIAN_POINT('Ctrl Pts',(39.2395946713538,-30.5321061642718,
-137.936087285073));
#159423=CARTESIAN_POINT('Ctrl Pts',(39.2334097009524,-30.5333933219195,
-137.9117272282));
#159424=CARTESIAN_POINT('Ctrl Pts',(39.2285848334955,-30.534397427783,-137.89272405793));
#159425=CARTESIAN_POINT('Ctrl Pts',(39.2235931574876,-30.5354511329446,
-137.872738003284));
#159426=CARTESIAN_POINT('Ctrl Pts',(39.2188441690707,-30.5364681053083,
-137.853395850005));
#159427=CARTESIAN_POINT('Ctrl Pts',(39.2175054560001,-30.5367547840863,
-137.847943406003));
#159428=CARTESIAN_POINT('Ctrl Pts',(39.2161857199312,-30.5370385409,-137.842542224786));
#159429=CARTESIAN_POINT('Ctrl Pts',(39.2148934224204,-30.5373174350074,
-137.837228967863));
#159430=CARTESIAN_POINT('Ctrl Pts',(39.2146990458272,-30.5373593839286,
-137.836429792154));
#159431=CARTESIAN_POINT('Ctrl Pts',(39.214504847708,-30.5374013226796,-137.835630793376));
#159432=CARTESIAN_POINT('Ctrl Pts',(39.2143108278165,-30.5374432512608,
-137.834831971547));
#159433=CARTESIAN_POINT('Ctrl Pts',(39.1922239238158,-30.5422163316834,
-137.743895413848));
#159434=CARTESIAN_POINT('Ctrl Pts',(39.1724858756577,-30.5468621133865,
-137.655159254419));
#159435=CARTESIAN_POINT('Ctrl Pts',(39.1547975358758,-30.5513764763546,
-137.568736391554));
#159436=CARTESIAN_POINT('Ctrl Pts',(39.1364521564366,-30.5560585269369,
-137.479103320783));
#159437=CARTESIAN_POINT('Ctrl Pts',(39.1203114766778,-30.5605992305923,
-137.391958310255));
#159438=CARTESIAN_POINT('Ctrl Pts',(39.1060690480999,-30.5649963940464,
-137.307379213395));
#159439=CARTESIAN_POINT('Ctrl Pts',(39.1049881432084,-30.5653301092874,
-137.300960226703));
#159440=CARTESIAN_POINT('Ctrl Pts',(39.1039181848734,-30.5656629988024,
-137.29455599823));
#159441=CARTESIAN_POINT('Ctrl Pts',(39.102859045528,-30.5659950621301,-137.288166551949));
#159442=CARTESIAN_POINT('Ctrl Pts',(39.0868430811912,-30.5710164169082,
-137.191547401492));
#159443=CARTESIAN_POINT('Ctrl Pts',(39.0733000498566,-30.5758480119611,
-137.098324767538));
#159444=CARTESIAN_POINT('Ctrl Pts',(39.061819755875,-30.5804857187884,-137.008629087097));
#159445=CARTESIAN_POINT('Ctrl Pts',(39.0536432573057,-30.5837887877951,
-136.944746001525));
#159446=CARTESIAN_POINT('Ctrl Pts',(39.0465142325881,-30.586993461715,-136.882652782168));
#159447=CARTESIAN_POINT('Ctrl Pts',(39.0402963664581,-30.5900982170105,
-136.822396589877));
#159448=CARTESIAN_POINT('Ctrl Pts',(39.0363915886327,-30.5920479823123,
-136.784556109142));
#159449=CARTESIAN_POINT('Ctrl Pts',(39.0328458135265,-30.593958569049,-136.747435703989));
#159450=CARTESIAN_POINT('Ctrl Pts',(39.0296261138438,-30.5958302989186,
-136.711033325134));
#159451=CARTESIAN_POINT('Ctrl Pts',(39.0222574437438,-30.6001139779211,
-136.627722101395));
#159452=CARTESIAN_POINT('Ctrl Pts',(39.0165956522317,-30.6041933284833,
-136.548187569322));
#159453=CARTESIAN_POINT('Ctrl Pts',(39.01228209515,-30.6080685835929,-136.472473348208));
#159454=CARTESIAN_POINT('Ctrl Pts',(39.0077058481702,-30.6121798365926,
-136.392148231571));
#159455=CARTESIAN_POINT('Ctrl Pts',(39.004646624077,-30.6160614012094,-136.316122548143));
#159456=CARTESIAN_POINT('Ctrl Pts',(39.0027201584472,-30.6197156000662,
-136.244404502519));
#159457=CARTESIAN_POINT('Ctrl Pts',(39.0007936928175,-30.623369798923,-136.172686456895));
#159458=CARTESIAN_POINT('Ctrl Pts',(39.,-30.6267966711481,-136.105275326978));
#159459=CARTESIAN_POINT('Ctrl Pts',(39.,-30.63000002,-136.04214564125));
#159460=CARTESIAN_POINT('Ctrl Pts',(39.,-36.28000002,-141.149515588739));
#159461=CARTESIAN_POINT('Ctrl Pts',(39.0000026845439,-36.271636952727,-141.308381696112));
#159462=CARTESIAN_POINT('Ctrl Pts',(39.0041560645674,-36.2626979527457,
-141.479433937643));
#159463=CARTESIAN_POINT('Ctrl Pts',(39.0196751709712,-36.2481955286276,
-141.754045307826));
#159464=CARTESIAN_POINT('Ctrl Pts',(39.0264019740874,-36.2431828057576,
-141.848583729441));
#159465=CARTESIAN_POINT('Ctrl Pts',(39.0392524022158,-36.2354101945438,
-141.994816669982));
#159466=CARTESIAN_POINT('Ctrl Pts',(39.046368127812,-36.2314610334767,-142.06903892383));
#159467=CARTESIAN_POINT('Ctrl Pts',(39.0559766116434,-36.2267529476897,
-142.157543704131));
#159468=CARTESIAN_POINT('Ctrl Pts',(39.0611201501891,-36.2243753882432,
-142.202270756544));
#159469=CARTESIAN_POINT('Ctrl Pts',(39.0639681937629,-36.2230956375407,
-142.22635834997));
#159470=CARTESIAN_POINT('Ctrl Pts',(39.0653227137038,-36.2224968063035,
-142.237633644024));
#159471=CARTESIAN_POINT('Ctrl Pts',(39.0661029962005,-36.2221542283202,
-142.244085085566));
#159472=CARTESIAN_POINT('Ctrl Pts',(39.0664357352188,-36.2220086145544,
-142.246827511015));
#159473=CARTESIAN_POINT('Ctrl Pts',(39.0740430194889,-36.2186840002108,
-142.309443989598));
#159474=CARTESIAN_POINT('Ctrl Pts',(39.0887631405107,-36.2125697575084,
-142.430607476474));
#159475=CARTESIAN_POINT('Ctrl Pts',(39.1326226546473,-36.1982650817826,
-142.700184720785));
#159476=CARTESIAN_POINT('Ctrl Pts',(39.1509869144791,-36.1926373593803,
-142.804670073255));
#159477=CARTESIAN_POINT('Ctrl Pts',(39.1865588623926,-36.1829503810533,
-142.982962068645));
#159478=CARTESIAN_POINT('Ctrl Pts',(39.1997609500423,-36.179515996477,-143.0459837673));
#159479=CARTESIAN_POINT('Ctrl Pts',(39.2219443680061,-36.1740903581866,
-143.145821485805));
#159480=CARTESIAN_POINT('Ctrl Pts',(39.2336317728787,-36.1713093947294,
-143.197066214847));
#159481=CARTESIAN_POINT('Ctrl Pts',(39.2483952962438,-36.1679576185287,
-143.259149252828));
#159482=CARTESIAN_POINT('Ctrl Pts',(39.2560702744332,-36.1662567791381,
-143.290761895407));
#159483=CARTESIAN_POINT('Ctrl Pts',(39.259423588014,-36.1655227139119,-143.304432193872));
#159484=CARTESIAN_POINT('Ctrl Pts',(39.261673495937,-36.1650322209503,-143.313572801173));
#159485=CARTESIAN_POINT('Ctrl Pts',(39.2630923672526,-36.1647244206623,
-143.319313599113));
#159486=CARTESIAN_POINT('Ctrl Pts',(39.3185147861829,-36.1527413890172,
-143.542939666575));
#159487=CARTESIAN_POINT('Ctrl Pts',(39.376487191619,-36.1419772728173,-143.740335575647));
#159488=CARTESIAN_POINT('Ctrl Pts',(39.4618196356428,-36.1278685716875,
-144.002760783506));
#159489=CARTESIAN_POINT('Ctrl Pts',(39.4900070416244,-36.1234910906176,
-144.084635066894));
#159490=CARTESIAN_POINT('Ctrl Pts',(39.5312015397534,-36.117374661997,-144.199178928827));
#159491=CARTESIAN_POINT('Ctrl Pts',(39.5515286748293,-36.1144280945784,
-144.254384472605));
#159492=CARTESIAN_POINT('Ctrl Pts',(39.5746338810447,-36.111170400366,-144.315208007352));
#159493=CARTESIAN_POINT('Ctrl Pts',(39.5860181263649,-36.1095842181069,
-144.34472838493));
#159494=CARTESIAN_POINT('Ctrl Pts',(39.5908593359132,-36.1089133141243,
-144.35718942879));
#159495=CARTESIAN_POINT('Ctrl Pts',(39.5940782365116,-36.1084679908687,
-144.365454499774));
#159496=CARTESIAN_POINT('Ctrl Pts',(39.5949354491578,-36.1083494362718,
-144.367654752919));
#159497=CARTESIAN_POINT('Ctrl Pts',(39.7476034322303,-36.0872982613274,
-144.757746156936));
#159498=CARTESIAN_POINT('Ctrl Pts',(39.9115823286905,-36.0692299855258,
-145.090746526247));
#159499=CARTESIAN_POINT('Ctrl Pts',(40.0734471901674,-36.0537915266759,
-145.374999596381));
#159500=CARTESIAN_POINT('Origin',(0.,-12.9675000200281,-171.64995));
#159501=CARTESIAN_POINT('',(53.6298444656516,-36.1005191032365,-171.449026400902));
#159502=CARTESIAN_POINT('',(55.7146117108563,-30.4940179634924,-171.449026400902));
#159503=CARTESIAN_POINT('Origin',(0.,-12.9675000200281,-171.449026400902));
#159504=CARTESIAN_POINT('Ctrl Pts',(55.7146117108563,-30.4940179634924,
-171.449026400902));
#159505=CARTESIAN_POINT('Ctrl Pts',(54.8724055325709,-30.4921606112015,
-169.724950356757));
#159506=CARTESIAN_POINT('Ctrl Pts',(54.0458152036748,-30.4902665003795,
-168.036186540547));
#159507=CARTESIAN_POINT('Ctrl Pts',(53.234784597893,-30.4883339514173,-166.382763547322));
#159508=CARTESIAN_POINT('Ctrl Pts',(52.4060857875293,-30.4863593021075,
-164.693320932276));
#159509=CARTESIAN_POINT('Ctrl Pts',(51.5936324329536,-30.4843445334443,
-163.040775976074));
#159510=CARTESIAN_POINT('Ctrl Pts',(50.7974127390484,-30.482290227048,-161.425132437527));
#159511=CARTESIAN_POINT('Ctrl Pts',(49.9722431291296,-30.4801612277018,
-159.750745382452));
#159512=CARTESIAN_POINT('Ctrl Pts',(49.1645092733571,-30.4779897715322,
-158.115991828474));
#159513=CARTESIAN_POINT('Ctrl Pts',(48.3742448639459,-30.4757788795041,
-156.520846084462));
#159514=CARTESIAN_POINT('Ctrl Pts',(48.2015166730246,-30.4752956445566,
-156.17219487945));
#159515=CARTESIAN_POINT('Ctrl Pts',(48.0296232101336,-30.4748105340451,
-155.825435739396));
#159516=CARTESIAN_POINT('Ctrl Pts',(47.8585650914879,-30.4743235932024,
-155.480568209344));
#159517=CARTESIAN_POINT('Ctrl Pts',(47.8537746537233,-30.4743099565518,
-155.470910284583));
#159518=CARTESIAN_POINT('Ctrl Pts',(47.8497874336421,-30.4742986041782,
-155.462871822295));
#159519=CARTESIAN_POINT('Ctrl Pts',(47.8441957454454,-30.4742826727293,
-155.451598884702));
#159520=CARTESIAN_POINT('Ctrl Pts',(47.8440689808494,-30.4742823115604,
-155.451343325141));
#159521=CARTESIAN_POINT('Ctrl Pts',(47.8439422166437,-30.4742819503903,
-155.451087766482));
#159522=CARTESIAN_POINT('Ctrl Pts',(47.8438154528283,-30.4742815892191,
-155.450832208722));
#159523=CARTESIAN_POINT('Ctrl Pts',(47.1281154616227,-30.4722424406397,
-154.00797025836));
#159524=CARTESIAN_POINT('Ctrl Pts',(46.4248779163233,-30.4701660906363,
-152.59381081989));
#159525=CARTESIAN_POINT('Ctrl Pts',(45.7340209887441,-30.4680503695182,
-151.208391024834));
#159526=CARTESIAN_POINT('Ctrl Pts',(45.0434297046247,-30.4659354619224,
-149.823503941679));
#159527=CARTESIAN_POINT('Ctrl Pts',(44.3652099140242,-30.4637812311311,
-148.467334199979));
#159528=CARTESIAN_POINT('Ctrl Pts',(43.6993304940745,-30.4615877238109,
-147.139892688189));
#159529=CARTESIAN_POINT('Ctrl Pts',(43.0059147757672,-30.4593035077674,
-145.757557115364));
#159530=CARTESIAN_POINT('Ctrl Pts',(42.3258812524105,-30.4569767040243,
-144.406374866656));
#159531=CARTESIAN_POINT('Ctrl Pts',(41.6592463874673,-30.4546096167241,
-143.086331517643));
#159532=CARTESIAN_POINT('Ctrl Pts',(41.0448183892133,-30.4524279055834,
-141.869666090743));
#159533=CARTESIAN_POINT('Ctrl Pts',(40.4417734418195,-30.4502120095389,
-140.679452889206));
#159534=CARTESIAN_POINT('Ctrl Pts',(39.850159149164,-30.447965242174,-139.5156626415));
#159535=CARTESIAN_POINT('Ctrl Pts',(40.0734472163172,-36.0537915241817,
-145.374999642303));
#159536=CARTESIAN_POINT('Ctrl Pts',(41.1513629919691,-36.0583266065864,
-147.382840909586));
#159537=CARTESIAN_POINT('Ctrl Pts',(42.2612453872436,-36.0628720322864,
-149.46995218686));
#159538=CARTESIAN_POINT('Ctrl Pts',(43.9743253442819,-36.0693743353693,
-152.719524117757));
#159539=CARTESIAN_POINT('Ctrl Pts',(44.5533923517989,-36.0714955758215,
-153.822532263887));
#159540=CARTESIAN_POINT('Ctrl Pts',(45.4340727076594,-36.0746257587657,
-155.506770736829));
#159541=CARTESIAN_POINT('Ctrl Pts',(45.8774326678813,-36.0761785538904,
-156.356321536736));
#159542=CARTESIAN_POINT('Ctrl Pts',(46.3999730275242,-36.0779791102198,
-157.360469372642));
#159543=CARTESIAN_POINT('Ctrl Pts',(46.6625651604514,-36.0788784372191,
-157.865794599598));
#159544=CARTESIAN_POINT('Ctrl Pts',(46.8082945827096,-36.0793762814646,
-158.146428123263));
#159545=CARTESIAN_POINT('Ctrl Pts',(46.878919483461,-36.0796172170613,-158.282490689921));
#159546=CARTESIAN_POINT('Ctrl Pts',(46.9166136408414,-36.0797457363095,
-158.355125127742));
#159547=CARTESIAN_POINT('Ctrl Pts',(46.9218982679862,-36.0797637527598,
-158.36530862072));
#159548=CARTESIAN_POINT('Ctrl Pts',(49.0459171851673,-36.0870044798771,
-162.458404893256));
#159549=CARTESIAN_POINT('Ctrl Pts',(51.2803555380598,-36.0939327197443,
-166.816984571593));
#159550=CARTESIAN_POINT('Ctrl Pts',(53.6298444656516,-36.1005191032365,
-171.449026400902));
#159551=CARTESIAN_POINT('Origin',(60.,28.41999998,-177.34995));
#159552=CARTESIAN_POINT('',(53.5288692553037,-37.78000002,-177.34995));
#159553=CARTESIAN_POINT('',(60.,-37.78000002,-177.34995));
#159554=CARTESIAN_POINT('',(53.7578119323263,-37.28000002,-177.34995));
#159555=CARTESIAN_POINT('Origin',(0.,-12.9675000200281,-177.34995));
#159556=CARTESIAN_POINT('',(60.,-37.28000002,-177.34995));
#159557=CARTESIAN_POINT('Origin',(60.,-2.55003103885676E-14,0.));
#159558=CARTESIAN_POINT('',(60.,-37.28000002,-58.24995));
#159559=CARTESIAN_POINT('',(60.,-37.78000002,-58.24995));
#159560=CARTESIAN_POINT('',(60.,-54.58000002,-58.24995));
#159561=CARTESIAN_POINT('',(60.,-37.78000002,-174.34995));
#159562=CARTESIAN_POINT('',(60.,-37.28000002,-58.24995));
#159563=CARTESIAN_POINT('Origin',(60.,-2.55003103885676E-14,0.));
#159564=CARTESIAN_POINT('',(60.,11.61999998,-58.24995));
#159565=CARTESIAN_POINT('',(60.,11.11999998,-58.24995));
#159566=CARTESIAN_POINT('',(60.,-54.58000002,-58.24995));
#159567=CARTESIAN_POINT('',(60.,11.11999998,-174.34995));
#159568=CARTESIAN_POINT('',(60.,11.61999998,-58.24995));
#159569=CARTESIAN_POINT('Origin',(60.,-54.58000002,-55.24995));
#159570=CARTESIAN_POINT('',(17.55,-54.58000002,-141.176536909659));
#159571=CARTESIAN_POINT('',(23.2,-54.5800000202568,-146.023178055809));
#159572=CARTESIAN_POINT('Ctrl Pts',(17.55,-54.58000002,-141.176536909659));
#159573=CARTESIAN_POINT('Ctrl Pts',(17.9693769714657,-54.5800000200003,
-141.49343498957));
#159574=CARTESIAN_POINT('Ctrl Pts',(18.3834419174572,-54.5800000200088,
-141.816182952558));
#159575=CARTESIAN_POINT('Ctrl Pts',(18.7928766486286,-54.5800000200341,
-142.144468939261));
#159576=CARTESIAN_POINT('Ctrl Pts',(19.2164906824758,-54.5800000200604,
-142.484123933074));
#159577=CARTESIAN_POINT('Ctrl Pts',(19.635148044891,-54.5800000201049,-142.829707458926));
#159578=CARTESIAN_POINT('Ctrl Pts',(20.0495713966145,-54.5800000201721,
-143.180920598229));
#159579=CARTESIAN_POINT('Ctrl Pts',(20.4883260232375,-54.5800000202432,
-143.55275386766));
#159580=CARTESIAN_POINT('Ctrl Pts',(20.9223347029258,-54.58000002034,-143.930897445251));
#159581=CARTESIAN_POINT('Ctrl Pts',(21.3524219960725,-54.5800000204563,
-144.315043885241));
#159582=CARTESIAN_POINT('Ctrl Pts',(21.3910234228641,-54.5800000204667,
-144.349522003793));
#159583=CARTESIAN_POINT('Ctrl Pts',(21.4295932412572,-54.5800000204773,
-144.384048506598));
#159584=CARTESIAN_POINT('Ctrl Pts',(21.4681320362146,-54.580000020488,-144.418623187422));
#159585=CARTESIAN_POINT('Ctrl Pts',(21.9304021275721,-54.5800000206166,
-144.83334401305));
#159586=CARTESIAN_POINT('Ctrl Pts',(22.3865711849682,-54.5800000207665,
-145.253534976228));
#159587=CARTESIAN_POINT('Ctrl Pts',(22.8375326449957,-54.580000020912,-145.679007211413));
#159588=CARTESIAN_POINT('Ctrl Pts',(22.9587258346798,-54.5800000209511,
-145.793350324682));
#159589=CARTESIAN_POINT('Ctrl Pts',(23.0795426741296,-54.5800000209898,
-145.90807504421));
#159590=CARTESIAN_POINT('Ctrl Pts',(23.2,-54.5800000210274,-146.023178055809));
#159591=CARTESIAN_POINT('',(23.2,-54.58000002,-86.035464915697));
#159592=CARTESIAN_POINT('',(23.2,-54.58000002,-85.5535812563546));
#159593=CARTESIAN_POINT('',(17.55,-54.58000002,-90.8821060618472));
#159594=CARTESIAN_POINT('Ctrl Pts',(23.2,-54.5800000205323,-86.035464915697));
#159595=CARTESIAN_POINT('Ctrl Pts',(22.7416005580064,-54.5800000204569,
-86.473488555251));
#159596=CARTESIAN_POINT('Ctrl Pts',(22.2778852069184,-54.580000020382,-86.9061566638687));
#159597=CARTESIAN_POINT('Ctrl Pts',(21.8082168240834,-54.5800000203146,
-87.3329667340019));
#159598=CARTESIAN_POINT('Ctrl Pts',(21.6948114073334,-54.5800000202983,
-87.4360236474446));
#159599=CARTESIAN_POINT('Ctrl Pts',(21.5810587192868,-54.5800000202825,
-87.5387388946999));
#159600=CARTESIAN_POINT('Ctrl Pts',(21.4669494079305,-54.5800000202671,
-87.6411051232898));
#159601=CARTESIAN_POINT('Ctrl Pts',(21.0322856597372,-54.5800000202087,
-88.0310372688657));
#159602=CARTESIAN_POINT('Ctrl Pts',(20.5935852018712,-54.5800000201577,
-88.4149271477261));
#159603=CARTESIAN_POINT('Ctrl Pts',(20.150033972245,-54.580000020117,-88.7924150855438));
#159604=CARTESIAN_POINT('Ctrl Pts',(19.7265254012934,-54.5800000200782,
-89.152845553139));
#159605=CARTESIAN_POINT('Ctrl Pts',(19.2985947426908,-54.5800000200487,
-89.5074398670458));
#159606=CARTESIAN_POINT('Ctrl Pts',(18.8655062292501,-54.5800000200292,
-89.8558463488876));
#159607=CARTESIAN_POINT('Ctrl Pts',(18.4324177158094,-54.5800000200098,
-90.2042528307294));
#159608=CARTESIAN_POINT('Ctrl Pts',(17.994171750171,-54.5800000200003,-90.5464720515007));
#159609=CARTESIAN_POINT('Ctrl Pts',(17.55,-54.58000002,-90.8821060618472));
#159610=CARTESIAN_POINT('',(17.55,-54.58000002,-140.803447286915));
#159611=CARTESIAN_POINT('Origin',(-3.54807775957937E-14,-73.08000002,3.11172719585489E-30));
#159612=CARTESIAN_POINT('',(16.55,-73.08000002,-58.24995));
#159613=CARTESIAN_POINT('',(16.05,-73.08000002,-58.24995));
#159614=CARTESIAN_POINT('',(-41.5,-73.0800000199999,-58.24995));
#159615=CARTESIAN_POINT('',(16.05,-73.08000002,-174.34995));
#159616=CARTESIAN_POINT('',(16.05,-73.08000002,-174.34995));
#159617=CARTESIAN_POINT('',(16.55,-73.08000002,-174.34995));
#159618=CARTESIAN_POINT('',(41.5,-73.08000002,-174.34995));
#159619=CARTESIAN_POINT('',(16.55,-73.08000002,-58.24995));
#159620=CARTESIAN_POINT('Origin',(60.,-54.58000002,-55.24995));
#159621=CARTESIAN_POINT('',(9.4,-54.58000002,-136.338455187671));
#159622=CARTESIAN_POINT('',(15.05,-54.580000020336,-139.407335470919));
#159623=CARTESIAN_POINT('Ctrl Pts',(9.4,-54.58000002,-136.338455187671));
#159624=CARTESIAN_POINT('Ctrl Pts',(9.92110496058178,-54.5800000200001,
-136.559368584536));
#159625=CARTESIAN_POINT('Ctrl Pts',(10.4350703325194,-54.5800000200483,
-136.794854049275));
#159626=CARTESIAN_POINT('Ctrl Pts',(10.9425445776645,-54.5800000201757,
-137.04357763751));
#159627=CARTESIAN_POINT('Ctrl Pts',(11.3976304732205,-54.58000002029,-137.266624615718));
#159628=CARTESIAN_POINT('Ctrl Pts',(11.8474960215382,-54.5800000203574,
-137.500318485595));
#159629=CARTESIAN_POINT('Ctrl Pts',(12.2925996107723,-54.5800000201853,
-137.743731583458));
#159630=CARTESIAN_POINT('Ctrl Pts',(12.5336925965022,-54.5800000200921,
-137.875577724331));
#159631=CARTESIAN_POINT('Ctrl Pts',(12.7734820900616,-54.5800000201101,
-138.010349990831));
#159632=CARTESIAN_POINT('Ctrl Pts',(13.0121639376423,-54.5800000201839,
-138.147985687537));
#159633=CARTESIAN_POINT('Ctrl Pts',(13.3646805607937,-54.580000020293,-138.351264116624));
#159634=CARTESIAN_POINT('Ctrl Pts',(13.7130708435113,-54.5800000206454,
-138.559766344709));
#159635=CARTESIAN_POINT('Ctrl Pts',(14.0580847568665,-54.5800000210433,
-138.773390841178));
#159636=CARTESIAN_POINT('Ctrl Pts',(14.3916633624461,-54.580000021428,-138.979934864163));
#159637=CARTESIAN_POINT('Ctrl Pts',(14.7220850961464,-54.5800000217332,
-139.191268004987));
#159638=CARTESIAN_POINT('Ctrl Pts',(15.05,-54.5800000213439,-139.407335470919));
#159639=CARTESIAN_POINT('',(15.05,-54.5800000206722,-92.6513075005872));
#159640=CARTESIAN_POINT('',(15.05,-54.58000002,-92.3169104578858));
#159641=CARTESIAN_POINT('',(9.4,-54.58000002,-95.7201877838351));
#159642=CARTESIAN_POINT('Ctrl Pts',(15.05,-54.5800000213444,-92.6513075005872));
#159643=CARTESIAN_POINT('Ctrl Pts',(14.7116749748805,-54.5800000217462,
-92.8742343330664));
#159644=CARTESIAN_POINT('Ctrl Pts',(14.3706840440917,-54.5800000214065,
-93.0921200800065));
#159645=CARTESIAN_POINT('Ctrl Pts',(14.0263093380892,-54.580000021009,-93.3049061919411));
#159646=CARTESIAN_POINT('Ctrl Pts',(13.691663333917,-54.5800000206227,-93.5116810242999));
#159647=CARTESIAN_POINT('Ctrl Pts',(13.3538223587281,-54.5800000202949,
-93.7136406704411));
#159648=CARTESIAN_POINT('Ctrl Pts',(13.0120992871415,-54.5800000201906,
-93.9106936784565));
#159649=CARTESIAN_POINT('Ctrl Pts',(12.7734325857322,-54.5800000201177,
-94.0483197135013));
#159650=CARTESIAN_POINT('Ctrl Pts',(12.5336633488411,-54.5800000201,-94.1830804413658));
#159651=CARTESIAN_POINT('Ctrl Pts',(12.2925916871682,-54.5800000202013,
-94.3149150255473));
#159652=CARTESIAN_POINT('Ctrl Pts',(11.7801234903754,-54.5800000204166,
-94.5951679228046));
#159653=CARTESIAN_POINT('Ctrl Pts',(11.2613422805864,-54.5800000202694,
-94.8625400041996));
#159654=CARTESIAN_POINT('Ctrl Pts',(10.7355463256496,-54.580000020136,-95.1156089775454));
#159655=CARTESIAN_POINT('Ctrl Pts',(10.2954190750541,-54.5800000200243,
-95.3274450527451));
#159656=CARTESIAN_POINT('Ctrl Pts',(9.85037652346006,-54.5800000200001,
-95.5292584793922));
#159657=CARTESIAN_POINT('Ctrl Pts',(9.4,-54.58000002,-95.7201877838351));
#159658=CARTESIAN_POINT('',(9.4,-54.58000002,-136.131917111522));
#159659=CARTESIAN_POINT('Origin',(60.,-54.58000002,-55.24995));
#159660=CARTESIAN_POINT('',(1.24999999943729,-54.58000002,-134.362052687297));
#159661=CARTESIAN_POINT('',(6.9,-54.58000002,-135.415380765739));
#159662=CARTESIAN_POINT('Ctrl Pts',(1.24999999852555,-54.58000002,-134.362052703156));
#159663=CARTESIAN_POINT('Ctrl Pts',(1.85586872996852,-54.58000002,-134.396884061811));
#159664=CARTESIAN_POINT('Ctrl Pts',(2.45821169814366,-54.5800000199999,
-134.456836856573));
#159665=CARTESIAN_POINT('Ctrl Pts',(3.05717008780238,-54.5800000200001,
-134.540898522253));
#159666=CARTESIAN_POINT('Ctrl Pts',(3.40705616967825,-54.5800000200002,
-134.590003781231));
#159667=CARTESIAN_POINT('Ctrl Pts',(3.75578723672591,-54.5800000200004,
-134.647336949705));
#159668=CARTESIAN_POINT('Ctrl Pts',(4.10339093154591,-54.5800000200016,
-134.712704370428));
#159669=CARTESIAN_POINT('Ctrl Pts',(4.21364342719022,-54.580000020002,-134.733437525386));
#159670=CARTESIAN_POINT('Ctrl Pts',(4.32374689616092,-54.5800000200024,
-134.754971981414));
#159671=CARTESIAN_POINT('Ctrl Pts',(4.43373542753185,-54.5800000200027,
-134.777307325963));
#159672=CARTESIAN_POINT('Ctrl Pts',(4.6798887972806,-54.5800000200034,-134.827293631415));
#159673=CARTESIAN_POINT('Ctrl Pts',(4.92593529130785,-54.5800000200038,
-134.881432381241));
#159674=CARTESIAN_POINT('Ctrl Pts',(5.17124777564251,-54.5800000200039,
-134.939444408488));
#159675=CARTESIAN_POINT('Ctrl Pts',(5.41900393393866,-54.580000020004,-134.998034321043));
#159676=CARTESIAN_POINT('Ctrl Pts',(5.66601353633239,-54.5800000200037,
-135.060575714351));
#159677=CARTESIAN_POINT('Ctrl Pts',(5.91161937020824,-54.5800000200032,
-135.126829777541));
#159678=CARTESIAN_POINT('Ctrl Pts',(5.95160365908367,-54.5800000200032,
-135.137615847074));
#159679=CARTESIAN_POINT('Ctrl Pts',(5.99155067840985,-54.5800000200031,
-135.148500406429));
#159680=CARTESIAN_POINT('Ctrl Pts',(6.03145750349794,-54.580000020003,-135.159482527522));
#159681=CARTESIAN_POINT('Ctrl Pts',(6.28934481311032,-54.5800000200026,
-135.230451582474));
#159682=CARTESIAN_POINT('Ctrl Pts',(6.54583590336147,-54.580000020002,-135.305503306744));
#159683=CARTESIAN_POINT('Ctrl Pts',(6.80143368808444,-54.5800000200016,
-135.384644793434));
#159684=CARTESIAN_POINT('Ctrl Pts',(6.83430358210263,-54.5800000200015,
-135.394822394476));
#159685=CARTESIAN_POINT('Ctrl Pts',(6.86715867181372,-54.5800000200014,
-135.405067695209));
#159686=CARTESIAN_POINT('Ctrl Pts',(6.9,-54.5800000200014,-135.415380765739));
#159687=CARTESIAN_POINT('',(6.9,-54.58000002,-96.6432622057672));
#159688=CARTESIAN_POINT('',(6.9,-54.58000002,-96.4806904787158));
#159689=CARTESIAN_POINT('',(1.24999998181185,-54.5800000199993,-97.6965897229033));
#159690=CARTESIAN_POINT('Ctrl Pts',(6.9,-54.5800000200288,-96.6432622057672));
#159691=CARTESIAN_POINT('Ctrl Pts',(6.49061970139211,-54.5800000200775,
-96.7718187571058));
#159692=CARTESIAN_POINT('Ctrl Pts',(6.07861873660016,-54.5800000205753,
-96.8899526380549));
#159693=CARTESIAN_POINT('Ctrl Pts',(5.66396816650171,-54.5800000217474,
-96.9971605311362));
#159694=CARTESIAN_POINT('Ctrl Pts',(5.26447645459898,-54.5800000228767,
-97.100449101863));
#159695=CARTESIAN_POINT('Ctrl Pts',(4.86252531660943,-54.5800000241933,
-97.1935960044572));
#159696=CARTESIAN_POINT('Ctrl Pts',(4.45809517257588,-54.5800000232613,
-97.2761964906685));
#159697=CARTESIAN_POINT('Ctrl Pts',(4.34240961804981,-54.5800000229947,
-97.2998240149577));
#159698=CARTESIAN_POINT('Ctrl Pts',(4.22645442245894,-54.5800000225654,
-97.3225679069059));
#159699=CARTESIAN_POINT('Ctrl Pts',(4.1103033922506,-54.5800000220553,-97.3444205163838));
#159700=CARTESIAN_POINT('Ctrl Pts',(3.87438492650356,-54.5800000210192,
-97.3888061244265));
#159701=CARTESIAN_POINT('Ctrl Pts',(3.63765702198835,-54.580000020604,-97.4294862943975));
#159702=CARTESIAN_POINT('Ctrl Pts',(3.40027293016165,-54.5800000203617,
-97.466451043988));
#159703=CARTESIAN_POINT('Ctrl Pts',(3.16793216733981,-54.5800000201245,
-97.5026304612829));
#159704=CARTESIAN_POINT('Ctrl Pts',(2.93496148468427,-54.5800000200661,
-97.5352507112807));
#159705=CARTESIAN_POINT('Ctrl Pts',(2.70149448625451,-54.5800000200335,
-97.5642527645725));
#159706=CARTESIAN_POINT('Ctrl Pts',(2.47413670469376,-54.5800000200018,
-97.5924959104624));
#159707=CARTESIAN_POINT('Ctrl Pts',(2.2463071385321,-54.580000020002,-97.6173077624549));
#159708=CARTESIAN_POINT('Ctrl Pts',(2.01813705517291,-54.5800000200007,
-97.6385856637381));
#159709=CARTESIAN_POINT('Ctrl Pts',(1.80087152564896,-54.5800000199995,
-97.658846665625));
#159710=CARTESIAN_POINT('Ctrl Pts',(1.58329647023807,-54.58000002,-97.6759032884729));
#159711=CARTESIAN_POINT('Ctrl Pts',(1.36554569823627,-54.58000002,-97.6896238013575));
#159712=CARTESIAN_POINT('Ctrl Pts',(1.32703559408638,-54.58000002,-97.6920503295177));
#159713=CARTESIAN_POINT('Ctrl Pts',(1.2885200646298,-54.58000002,-97.6943724020827));
#159714=CARTESIAN_POINT('Ctrl Pts',(1.24999994858788,-54.58000002,-97.6965891455738));
#159715=CARTESIAN_POINT('',(1.24999999999997,-54.58000002,-134.339054731985));
#159716=CARTESIAN_POINT('Origin',(-3.3975957231091E-14,-70.08000002,-174.34995));
#159717=CARTESIAN_POINT('',(24.2,-73.08000002,-174.34995));
#159718=CARTESIAN_POINT('',(24.7,-73.08000002,-174.34995));
#159719=CARTESIAN_POINT('',(41.5,-73.08000002,-174.34995));
#159720=CARTESIAN_POINT('',(24.2,-70.08000002,-177.34995));
#159721=CARTESIAN_POINT('Origin',(24.2,-70.08000002,-174.34995));
#159722=CARTESIAN_POINT('',(24.7,-70.08000002,-177.34995));
#159723=CARTESIAN_POINT('',(-41.5,-70.08000002,-177.34995));
#159724=CARTESIAN_POINT('Origin',(24.7,-70.08000002,-174.34995));
#159725=CARTESIAN_POINT('Origin',(0.,-12.9675000200281,-170.64995));
#159726=CARTESIAN_POINT('Ctrl Pts',(31.35,-63.1109998882233,-171.64995));
#159727=CARTESIAN_POINT('Ctrl Pts',(31.3163826919509,-62.9824421580757,
-171.64995));
#159728=CARTESIAN_POINT('Ctrl Pts',(31.2868383330336,-62.8719447893433,
-171.626170015677));
#159729=CARTESIAN_POINT('Ctrl Pts',(31.2514775435999,-62.7372823365182,
-171.580557425965));
#159730=CARTESIAN_POINT('Ctrl Pts',(31.2410919380176,-62.6974310527944,
-171.563623005043));
#159731=CARTESIAN_POINT('Ctrl Pts',(31.2274097259629,-62.6448298616196,
-171.538032015327));
#159732=CARTESIAN_POINT('Ctrl Pts',(31.2231625215576,-62.6284882571325,
-171.529463812056));
#159733=CARTESIAN_POINT('Ctrl Pts',(31.2172203289157,-62.6056926604661,
-171.516799359085));
#159734=CARTESIAN_POINT('Ctrl Pts',(31.2143562722305,-62.5947238974589,
-171.51051351882));
#159735=CARTESIAN_POINT('Ctrl Pts',(31.211192177598,-62.5826609240819,-171.503308765418));
#159736=CARTESIAN_POINT('Ctrl Pts',(31.2098730231894,-62.5776464897022,
-171.500253322111));
#159737=CARTESIAN_POINT('Ctrl Pts',(31.2090016607235,-62.5743378631998,
-171.49822405484));
#159738=CARTESIAN_POINT('Ctrl Pts',(31.2088776499101,-62.5738660850072,
-171.497937403819));
#159739=CARTESIAN_POINT('Ctrl Pts',(31.1610829776623,-62.392811385933,-171.385434173695));
#159740=CARTESIAN_POINT('Ctrl Pts',(31.1276890220452,-62.2670868673818,
-171.23009267792));
#159741=CARTESIAN_POINT('Ctrl Pts',(31.1079170675507,-62.1926886331265,
-171.07256826174));
#159742=CARTESIAN_POINT('',(25.5241645866138,-65.4203114476559,-171.244965289362));
#159743=CARTESIAN_POINT('Origin',(25.6930085000554,-66.193075224377,-170.642186607387));
#159744=CARTESIAN_POINT('',(26.2234488624093,-65.1680142434972,-171.34400271074));
#159745=CARTESIAN_POINT('Ctrl Pts',(25.5241645593467,-65.420311391623,-171.244965335496));
#159746=CARTESIAN_POINT('Ctrl Pts',(25.5856266066318,-65.3950097001748,
-171.250561299215));
#159747=CARTESIAN_POINT('Ctrl Pts',(25.6482431903754,-65.3700416388738,
-171.257283842693));
#159748=CARTESIAN_POINT('Ctrl Pts',(25.7120492724639,-65.3455045252255,
-171.26508922401));
#159749=CARTESIAN_POINT('Ctrl Pts',(25.7739841159747,-65.3216870105894,
-171.272665697202));
#159750=CARTESIAN_POINT('Ctrl Pts',(25.8370396117807,-65.2982756083868,
-171.281262680318));
#159751=CARTESIAN_POINT('Ctrl Pts',(25.9012641559865,-65.2753562048817,
-171.290795412438));
#159752=CARTESIAN_POINT('Ctrl Pts',(25.9628302885007,-65.2533854918032,
-171.299933561353));
#159753=CARTESIAN_POINT('Ctrl Pts',(26.0254706465919,-65.231866942171,-171.309931710469));
#159754=CARTESIAN_POINT('Ctrl Pts',(26.0892441669414,-65.2108724395197,
-171.320670985522));
#159755=CARTESIAN_POINT('Ctrl Pts',(26.1334266108244,-65.1963273990365,
-171.328111180366));
#159756=CARTESIAN_POINT('Ctrl Pts',(26.1781532742408,-65.1820338125062,
-171.335906203664));
#159757=CARTESIAN_POINT('Ctrl Pts',(26.2234488624093,-65.1680142434972,
-171.34400271074));
#159758=CARTESIAN_POINT('Ctrl Pts',(26.2234488624093,-65.1680142434972,
-171.34400271074));
#159759=CARTESIAN_POINT('Ctrl Pts',(26.3217167386875,-65.1375990677912,
-171.361567921566));
#159760=CARTESIAN_POINT('Ctrl Pts',(26.4303514143194,-65.1038537466012,
-171.379899641242));
#159761=CARTESIAN_POINT('Ctrl Pts',(26.5494548896309,-65.0666619993164,
-171.39847124772));
#159762=CARTESIAN_POINT('Ctrl Pts',(26.6414327590449,-65.0379406067114,
-171.412813203661));
#159763=CARTESIAN_POINT('Ctrl Pts',(26.7396537921653,-65.0071635777161,
-171.427297276244));
#159764=CARTESIAN_POINT('Ctrl Pts',(26.8441476657696,-64.9742759706334,
-171.441710877444));
#159765=CARTESIAN_POINT('Ctrl Pts',(26.8973144353205,-64.9575426659283,
-171.449044557276));
#159766=CARTESIAN_POINT('Ctrl Pts',(26.9521048251731,-64.9402629709406,
-171.456360592174));
#159767=CARTESIAN_POINT('Ctrl Pts',(27.0085205474515,-64.9224297399861,
-171.46363596587));
#159768=CARTESIAN_POINT('Ctrl Pts',(27.0558749625435,-64.9074608237524,
-171.469742793046));
#159769=CARTESIAN_POINT('Ctrl Pts',(27.104374200011,-64.8921020024936,-171.475820972803));
#159770=CARTESIAN_POINT('Ctrl Pts',(27.1540177175151,-64.8763493205577,
-171.48185932281));
#159771=CARTESIAN_POINT('Ctrl Pts',(27.2981145026722,-64.8306251064268,
-171.499386421359));
#159772=CARTESIAN_POINT('Ctrl Pts',(27.4518624274715,-64.7815805088472,
-171.51653998626));
#159773=CARTESIAN_POINT('Ctrl Pts',(27.6152854898679,-64.729100640996,-171.532829362194));
#159774=CARTESIAN_POINT('Ctrl Pts',(27.762285103335,-64.6818948171925,-171.547481712545));
#159775=CARTESIAN_POINT('Ctrl Pts',(27.9171113129778,-64.6319098298976,
-171.561433561531));
#159776=CARTESIAN_POINT('Ctrl Pts',(28.0797524083188,-64.5790629606593,
-171.574350075366));
#159777=CARTESIAN_POINT('Ctrl Pts',(28.0826324162796,-64.5781271614765,
-171.574578797772));
#159778=CARTESIAN_POINT('Ctrl Pts',(28.0845605503282,-64.5775006128595,
-171.574731707236));
#159779=CARTESIAN_POINT('Ctrl Pts',(28.0881176467749,-64.5763445655939,
-171.575012963699));
#159780=CARTESIAN_POINT('Ctrl Pts',(28.0885065052652,-64.5762181875771,
-171.575043710395));
#159781=CARTESIAN_POINT('Ctrl Pts',(28.088914830995,-64.5760854809111,-171.575075987216));
#159782=CARTESIAN_POINT('Ctrl Pts',(28.0893459957261,-64.5759453491265,
-171.575110057511));
#159783=CARTESIAN_POINT('Ctrl Pts',(28.2453251126488,-64.5252509615012,
-171.587435403764));
#159784=CARTESIAN_POINT('Ctrl Pts',(28.3917855167039,-64.4774693308856,
-171.597568849547));
#159785=CARTESIAN_POINT('Ctrl Pts',(28.5286691085897,-64.4326571475584,
-171.605956388818));
#159786=CARTESIAN_POINT('Ctrl Pts',(28.6375214539492,-64.3970216766547,
-171.612626314036));
#159787=CARTESIAN_POINT('Ctrl Pts',(28.7403173603302,-64.363262690218,-171.618191806933));
#159788=CARTESIAN_POINT('Ctrl Pts',(28.8370242459599,-64.331388662323,-171.622865882341));
#159789=CARTESIAN_POINT('Ctrl Pts',(28.9570429382945,-64.2918311983175,
-171.628666673203));
#159790=CARTESIAN_POINT('Ctrl Pts',(29.0676861505517,-64.2551849334993,
-171.63309896429));
#159791=CARTESIAN_POINT('Ctrl Pts',(29.1688978658542,-64.2215000860559,
-171.636547403149));
#159792=CARTESIAN_POINT('Ctrl Pts',(29.2517930969775,-64.1939112520377,
-171.639371771211));
#159793=CARTESIAN_POINT('Ctrl Pts',(29.3283616429728,-64.1683085580936,
-171.641535544552));
#159794=CARTESIAN_POINT('Ctrl Pts',(29.3985739176396,-64.1447118415866,
-171.643225082614));
#159795=CARTESIAN_POINT('Ctrl Pts',(29.4774723478353,-64.1181959097354,
-171.645123638124));
#159796=CARTESIAN_POINT('Ctrl Pts',(29.5483631757519,-64.0942438437233,
-171.646429379742));
#159797=CARTESIAN_POINT('Ctrl Pts',(29.6112478721861,-64.0729216658316,
-171.647365040175));
#159798=CARTESIAN_POINT('Ctrl Pts',(29.674111806394,-64.051606527743,-171.648300391687));
#159799=CARTESIAN_POINT('Ctrl Pts',(29.7289749630295,-64.0329196552157,
-171.648865922478));
#159800=CARTESIAN_POINT('Ctrl Pts',(29.7758403385976,-64.016920223518,-171.64923249186));
#159801=CARTESIAN_POINT('Ctrl Pts',(29.823015394053,-64.0008150697996,-171.649601483481));
#159802=CARTESIAN_POINT('Ctrl Pts',(29.8620866579719,-63.9874330870119,
-171.649768868419));
#159803=CARTESIAN_POINT('Ctrl Pts',(29.8930579659894,-63.976826170643,-171.649856428699));
#159804=CARTESIAN_POINT('Ctrl Pts',(29.9222033403128,-63.9668445919568,
-171.649938826806));
#159805=CARTESIAN_POINT('Ctrl Pts',(29.9441756977843,-63.9593204895971,
-171.64995));
#159806=CARTESIAN_POINT('Ctrl Pts',(29.958978566972,-63.954289311524,-171.64995));
#159807=CARTESIAN_POINT('Ctrl Pts',(1.21164037634558,-54.58000002,-134.359881256142));
#159808=CARTESIAN_POINT('Ctrl Pts',(1.14985954526071,-54.5800000199999,
-135.468549546812));
#159809=CARTESIAN_POINT('Ctrl Pts',(1.09388617364344,-55.0500049847781,
-136.4730019173));
#159810=CARTESIAN_POINT('Ctrl Pts',(2.29002416952399,-54.58000002,-134.419974475838));
#159811=CARTESIAN_POINT('Ctrl Pts',(2.17342188453964,-54.580000019985,-135.528968047153));
#159812=CARTESIAN_POINT('Ctrl Pts',(2.06753434039226,-55.0527274298038,
-136.533094948603));
#159813=CARTESIAN_POINT('Ctrl Pts',(3.36400336137312,-54.58000002,-134.560074887715));
#159814=CARTESIAN_POINT('Ctrl Pts',(3.19311388201375,-54.58000002,-135.669910423004));
#159815=CARTESIAN_POINT('Ctrl Pts',(3.03750087523273,-55.0590775604595,
-136.673195500792));
#159816=CARTESIAN_POINT('Ctrl Pts',(4.96860300664728,-54.58000002,-134.885915931654));
#159817=CARTESIAN_POINT('Ctrl Pts',(4.71606907271929,-54.5800000199999,
-135.997377284272));
#159818=CARTESIAN_POINT('Ctrl Pts',(4.48819703666783,-55.0737169289411,
-136.999036474763));
#159819=CARTESIAN_POINT('Ctrl Pts',(5.50462478218054,-54.58000002,-135.014494663549));
#159820=CARTESIAN_POINT('Ctrl Pts',(5.22505809365354,-54.5800000199999,
-136.126651318852));
#159821=CARTESIAN_POINT('Ctrl Pts',(4.97306105763453,-55.0794779054381,
-137.127615177464));
#159822=CARTESIAN_POINT('Ctrl Pts',(6.5582931505392,-54.58000002,-135.304459760069));
#159823=CARTESIAN_POINT('Ctrl Pts',(6.22568909425541,-54.58000002,-136.4181319057));
#159824=CARTESIAN_POINT('Ctrl Pts',(5.92681315212766,-55.0924068363451,
-137.417580209995));
#159825=CARTESIAN_POINT('Ctrl Pts',(7.07711031169138,-54.58000002,-135.46589761626));
#159826=CARTESIAN_POINT('Ctrl Pts',(6.71851091709043,-54.58000002,-136.580434989905));
#159827=CARTESIAN_POINT('Ctrl Pts',(6.39675697066589,-55.0995771769741,
-137.579018061084));
#159828=CARTESIAN_POINT('Ctrl Pts',(7.58869434220596,-54.58000002,-135.642187967278));
#159829=CARTESIAN_POINT('Ctrl Pts',(7.2043372482231,-54.58000002,-136.757569215766));
#159830=CARTESIAN_POINT('Ctrl Pts',(6.86051928234731,-55.1073628388699,
-137.755308344391));
#159831=CARTESIAN_POINT('',(6.82752390438729,-55.1067946098355,-137.742762001241));
#159832=CARTESIAN_POINT('',(1.23668893165473,-55.0504165218146,-136.482360813851));
#159833=CARTESIAN_POINT('Ctrl Pts',(6.82752390105444,-55.106794611208,-137.742762010959));
#159834=CARTESIAN_POINT('Ctrl Pts',(6.36691608500268,-55.099096087914,-137.56848291046));
#159835=CARTESIAN_POINT('Ctrl Pts',(5.90746653899706,-55.0921186415656,
-137.411614134422));
#159836=CARTESIAN_POINT('Ctrl Pts',(5.21924575097325,-55.0827917577677,
-137.202426457053));
#159837=CARTESIAN_POINT('Ctrl Pts',(4.87537346097248,-55.0784122257285,
-137.10436149004));
#159838=CARTESIAN_POINT('Ctrl Pts',(4.47443163044212,-55.0738024150764,
-137.001377887286));
#159839=CARTESIAN_POINT('Ctrl Pts',(4.30263256796571,-55.0719335078804,
-136.959690384411));
#159840=CARTESIAN_POINT('Ctrl Pts',(4.1881051325322,-55.0707112308887,-136.932442788467));
#159841=CARTESIAN_POINT('Ctrl Pts',(4.13281892637863,-55.0701321878583,
-136.91954214536));
#159842=CARTESIAN_POINT('Ctrl Pts',(3.12583467092903,-55.059800011716,-136.689517799435));
#159843=CARTESIAN_POINT('Ctrl Pts',(2.18183534213973,-55.0534032173182,
-136.548300970225));
#159844=CARTESIAN_POINT('Ctrl Pts',(1.23668893165476,-55.0504165218146,
-136.482360813851));
#159845=CARTESIAN_POINT('Ctrl Pts',(6.82752391167578,-55.1067946098897,
-137.742761979991));
#159846=CARTESIAN_POINT('Ctrl Pts',(6.82865514233252,-55.0906927749922,
-137.709063966307));
#159847=CARTESIAN_POINT('Ctrl Pts',(6.82989569318454,-55.0733143121305,
-137.671794693994));
#159848=CARTESIAN_POINT('Ctrl Pts',(6.83125496840252,-55.0548926081662,
-137.630841859));
#159849=CARTESIAN_POINT('Ctrl Pts',(6.83251854070202,-55.0377679269163,
-137.59277240316));
#159850=CARTESIAN_POINT('Ctrl Pts',(6.83388482437207,-55.0197420755336,
-137.551519359742));
#159851=CARTESIAN_POINT('Ctrl Pts',(6.83535746783391,-55.0010426501733,
-137.506989171318));
#159852=CARTESIAN_POINT('Ctrl Pts',(6.83688588027598,-54.9816350779259,
-137.460772625494));
#159853=CARTESIAN_POINT('Ctrl Pts',(6.83852910258862,-54.9615015335891,
-137.411025472467));
#159854=CARTESIAN_POINT('Ctrl Pts',(6.84028407605309,-54.9409428817604,
-137.357646873862));
#159855=CARTESIAN_POINT('Ctrl Pts',(6.84116156278532,-54.930663555846,-137.330957574559));
#159856=CARTESIAN_POINT('Ctrl Pts',(6.84206685481821,-54.9202787058626,
-137.303360523525));
#159857=CARTESIAN_POINT('Ctrl Pts',(6.84299862087351,-54.9098305132466,
-137.274844194797));
#159858=CARTESIAN_POINT('Ctrl Pts',(6.84346450390116,-54.9046064169385,
-137.260586030434));
#159859=CARTESIAN_POINT('Ctrl Pts',(6.84393700981204,-54.8993665212808,
-137.24609803364));
#159860=CARTESIAN_POINT('Ctrl Pts',(6.84441587811191,-54.8941164051088,
-137.231378905632));
#159861=CARTESIAN_POINT('Ctrl Pts',(6.84478230404662,-54.8900990610369,
-137.220115954545));
#159862=CARTESIAN_POINT('Ctrl Pts',(6.84512750680533,-54.8863462003223,
-137.20948827454));
#159863=CARTESIAN_POINT('Ctrl Pts',(6.84550863637637,-54.8822386442122,
-137.197726631341));
#159864=CARTESIAN_POINT('Ctrl Pts',(6.8456255907356,-54.8809781894236,-137.194117424529));
#159865=CARTESIAN_POINT('Ctrl Pts',(6.84574593077812,-54.8796846645726,
-137.190401311301));
#159866=CARTESIAN_POINT('Ctrl Pts',(6.84587131312705,-54.8783411245515,
-137.186526810165));
#159867=CARTESIAN_POINT('Ctrl Pts',(6.84770105936456,-54.8587343990471,
-137.129984928968));
#159868=CARTESIAN_POINT('Ctrl Pts',(6.84942928243091,-54.8412633928784,
-137.076574520802));
#159869=CARTESIAN_POINT('Ctrl Pts',(6.85104244637681,-54.8256167780335,
-137.026448311966));
#159870=CARTESIAN_POINT('Ctrl Pts',(6.8526724164755,-54.8098071547105,-136.975799881735));
#159871=CARTESIAN_POINT('Ctrl Pts',(6.85418514107506,-54.7958596699486,
-136.928503953666));
#159872=CARTESIAN_POINT('Ctrl Pts',(6.85557654565148,-54.7834863408097,
-136.884677100533));
#159873=CARTESIAN_POINT('Ctrl Pts',(6.85698425116315,-54.7709680525119,
-136.840336795952));
#159874=CARTESIAN_POINT('Ctrl Pts',(6.85826798681468,-54.7600606486674,
-136.799546849772));
#159875=CARTESIAN_POINT('Ctrl Pts',(6.85943030320443,-54.7505060449436,
-136.762393576608));
#159876=CARTESIAN_POINT('Ctrl Pts',(6.85996390280677,-54.7461196895653,
-136.745337143471));
#159877=CARTESIAN_POINT('Ctrl Pts',(6.8604719860349,-54.7420190332804,-136.729046736211));
#159878=CARTESIAN_POINT('Ctrl Pts',(6.86095509270203,-54.7381821800109,
-136.713528729206));
#159879=CARTESIAN_POINT('Ctrl Pts',(6.86155592605446,-54.7334103365039,
-136.694229189775));
#159880=CARTESIAN_POINT('Ctrl Pts',(6.86211812692543,-54.7290463835956,
-136.676124419269));
#159881=CARTESIAN_POINT('Ctrl Pts',(6.8626429567941,-54.7250525423937,-136.659224428366));
#159882=CARTESIAN_POINT('Ctrl Pts',(6.86290537172844,-54.7230556217927,
-136.650774432914));
#159883=CARTESIAN_POINT('Ctrl Pts',(6.8631584500198,-54.7211513090831,-136.642625613791));
#159884=CARTESIAN_POINT('Ctrl Pts',(6.86340235796966,-54.7193353377099,
-136.634778996657));
#159885=CARTESIAN_POINT('Ctrl Pts',(6.86352431194459,-54.7184273520232,
-136.63085568809));
#159886=CARTESIAN_POINT('Ctrl Pts',(6.86364397372556,-54.7175414566762,
-136.627007928831));
#159887=CARTESIAN_POINT('Ctrl Pts',(6.8637613648426,-54.7166771482468,-136.623235838989));
#159888=CARTESIAN_POINT('Ctrl Pts',(6.86382006040112,-54.716244994032,-136.621349794069));
#159889=CARTESIAN_POINT('Ctrl Pts',(6.86387818831689,-54.7158182368597,
-136.619482666432));
#159890=CARTESIAN_POINT('Ctrl Pts',(6.86393575129393,-54.7153968156136,
-136.617634470333));
#159891=CARTESIAN_POINT('Ctrl Pts',(6.86399331427096,-54.7149753943675,
-136.615786274235));
#159892=CARTESIAN_POINT('Ctrl Pts',(6.86399608221759,-54.7149540623116,
-136.615696574571));
#159893=CARTESIAN_POINT('Ctrl Pts',(6.86410674816117,-54.7141484997746,
-136.612146690543));
#159894=CARTESIAN_POINT('Ctrl Pts',(6.86687027771176,-54.6940321405412,
-136.523499640744));
#159895=CARTESIAN_POINT('Ctrl Pts',(6.86957825832433,-54.6766746954665,
-136.436668295782));
#159896=CARTESIAN_POINT('Ctrl Pts',(6.87220179170381,-54.6617598759321,
-136.351863423873));
#159897=CARTESIAN_POINT('Ctrl Pts',(6.87491477571019,-54.6463365284835,
-136.264167089247));
#159898=CARTESIAN_POINT('Ctrl Pts',(6.8775375463631,-54.6335245857754,-136.178637752116));
#159899=CARTESIAN_POINT('Ctrl Pts',(6.88005612234316,-54.622974273047,-136.095454821509));
#159900=CARTESIAN_POINT('Ctrl Pts',(6.88262252285252,-54.6122236234042,
-136.010692353681));
#159901=CARTESIAN_POINT('Ctrl Pts',(6.88508090180449,-54.6038207305193,
-135.928365983663));
#159902=CARTESIAN_POINT('Ctrl Pts',(6.88743275526135,-54.5974048404534,
-135.848613127078));
#159903=CARTESIAN_POINT('Ctrl Pts',(6.88986235560334,-54.5907768557662,
-135.766223823837));
#159904=CARTESIAN_POINT('Ctrl Pts',(6.8921784369626,-54.5862688512884,-135.686580732264));
#159905=CARTESIAN_POINT('Ctrl Pts',(6.89439732976196,-54.5835019137301,
-135.609783871025));
#159906=CARTESIAN_POINT('Ctrl Pts',(6.89633252386602,-54.5810887456623,
-135.542805947115));
#159907=CARTESIAN_POINT('Ctrl Pts',(6.89819411437535,-54.5800000650814,
-135.477991939119));
#159908=CARTESIAN_POINT('Ctrl Pts',(6.9,-54.5800000200014,-135.415380765739));
#159909=CARTESIAN_POINT('Origin',(1.23493664937611,-61.9785327152568,-133.830076534122));
#159910=CARTESIAN_POINT('Ctrl Pts',(14.935633130959,-55.3065630024253,-142.47652148601));
#159911=CARTESIAN_POINT('Ctrl Pts',(15.630331507009,-54.5800000199999,-141.502754952306));
#159912=CARTESIAN_POINT('Ctrl Pts',(16.443141398898,-54.58000002,-140.363430177307));
#159913=CARTESIAN_POINT('Ctrl Pts',(13.9222087476243,-55.2748272571858,
-141.68934947009));
#159914=CARTESIAN_POINT('Ctrl Pts',(14.5800220275964,-54.580000020014,-140.713030388695));
#159915=CARTESIAN_POINT('Ctrl Pts',(15.3397373006696,-54.58000002,-139.576246587186));
#159916=CARTESIAN_POINT('Ctrl Pts',(12.8784929287096,-55.2441433795399,
-140.946005990295));
#159917=CARTESIAN_POINT('Ctrl Pts',(13.4942101985199,-54.5800000200048,
-139.965671699013));
#159918=CARTESIAN_POINT('Ctrl Pts',(14.2001096642283,-54.58000002,-138.832914681508));
#159919=CARTESIAN_POINT('Ctrl Pts',(10.7090288904129,-55.1865297732718,
-139.576073691957));
#159920=CARTESIAN_POINT('Ctrl Pts',(11.2325518044464,-54.5800000199952,
-138.58879503276));
#159921=CARTESIAN_POINT('Ctrl Pts',(11.8242610588971,-54.58000002,-137.462982383337));
#159922=CARTESIAN_POINT('Ctrl Pts',(9.6010395318864,-55.1600903081647,-138.961065386249));
#159923=CARTESIAN_POINT('Ctrl Pts',(10.0748797157148,-54.5800000199999,
-137.970225859417));
#159924=CARTESIAN_POINT('Ctrl Pts',(10.6074840054802,-54.58000002,-136.847973525117));
#159925=CARTESIAN_POINT('Ctrl Pts',(8.46374531288877,-55.1370659744517,
-138.432713944563));
#159926=CARTESIAN_POINT('Ctrl Pts',(8.88330739463766,-54.58000002,-137.438496970103));
#159927=CARTESIAN_POINT('Ctrl Pts',(9.35547519799418,-54.58000002,-136.31962263586));
#159928=CARTESIAN_POINT('',(14.8995695360959,-55.3054344939376,-142.448537924459));
#159929=CARTESIAN_POINT('',(9.30242220787652,-55.1547652726017,-138.840493482365));
#159930=CARTESIAN_POINT('Ctrl Pts',(14.8995696008972,-55.3054345059085,
-142.448537780858));
#159931=CARTESIAN_POINT('Ctrl Pts',(14.4360425314271,-55.2909407491857,
-142.089227172811));
#159932=CARTESIAN_POINT('Ctrl Pts',(13.9756272852217,-55.276965801663,-141.746453688849));
#159933=CARTESIAN_POINT('Ctrl Pts',(13.5167726538588,-55.2635139066454,
-141.419418449115));
#159934=CARTESIAN_POINT('Ctrl Pts',(13.0608088615625,-55.2501467601756,
-141.094443570512));
#159935=CARTESIAN_POINT('Ctrl Pts',(12.6063898761816,-55.2372957621152,
-140.785004198599));
#159936=CARTESIAN_POINT('Ctrl Pts',(12.1520037917279,-55.2249575381717,
-140.490317118194));
#159937=CARTESIAN_POINT('Ctrl Pts',(12.0325966013581,-55.2217152015208,
-140.412876902674));
#159938=CARTESIAN_POINT('Ctrl Pts',(11.913191572675,-55.2185082497222,-140.336455667304));
#159939=CARTESIAN_POINT('Ctrl Pts',(11.7937609095613,-55.2153365764059,
-140.261039841126));
#159940=CARTESIAN_POINT('Ctrl Pts',(11.4455508439728,-55.206089298155,-140.041158705954));
#159941=CARTESIAN_POINT('Ctrl Pts',(11.0989538321641,-55.1971924514801,
-139.831013919457));
#159942=CARTESIAN_POINT('Ctrl Pts',(10.75329986993,-55.1886468974311,-139.63028506502));
#159943=CARTESIAN_POINT('Ctrl Pts',(10.4339817724706,-55.1807524412442,
-139.444850026204));
#159944=CARTESIAN_POINT('Ctrl Pts',(10.1154686315248,-55.1731577288529,
-139.267450490947));
#159945=CARTESIAN_POINT('Ctrl Pts',(9.79721921732249,-55.1658637037984,
-139.097876598179));
#159946=CARTESIAN_POINT('Ctrl Pts',(9.63224811328577,-55.1620826964738,
-139.00997449669));
#159947=CARTESIAN_POINT('Ctrl Pts',(9.46734764252996,-55.1583824957503,
-138.924175954812));
#159948=CARTESIAN_POINT('Ctrl Pts',(9.302440717147,-55.1547633327525,-138.840457107207));
#159949=CARTESIAN_POINT('Ctrl Pts',(14.8995694581843,-55.3054344861034,
-142.448537924463));
#159950=CARTESIAN_POINT('Ctrl Pts',(14.9033493580002,-55.2678130034392,
-142.375124451206));
#159951=CARTESIAN_POINT('Ctrl Pts',(14.9073778485915,-55.2293881917473,
-142.29668067779));
#159952=CARTESIAN_POINT('Ctrl Pts',(14.911659466542,-55.1907336547858,-142.21302758756));
#159953=CARTESIAN_POINT('Ctrl Pts',(14.9132571196824,-55.1763100086129,
-142.18181307383));
#159954=CARTESIAN_POINT('Ctrl Pts',(14.9148900157128,-55.1618548868074,
-142.149873089003));
#159955=CARTESIAN_POINT('Ctrl Pts',(14.9165583830287,-55.1473998475109,
-142.117197815172));
#159956=CARTESIAN_POINT('Ctrl Pts',(14.9196281312329,-55.1208029881141,
-142.057076244693));
#159957=CARTESIAN_POINT('Ctrl Pts',(14.9228177984541,-55.0942074117109,
-141.994468404112));
#159958=CARTESIAN_POINT('Ctrl Pts',(14.9261276135912,-55.0678250719188,
-141.929332565682));
#159959=CARTESIAN_POINT('Ctrl Pts',(14.9277825211597,-55.0546339020227,
-141.896764646467));
#159960=CARTESIAN_POINT('Ctrl Pts',(14.9294674513146,-55.0414962585256,
-141.863564944585));
#159961=CARTESIAN_POINT('Ctrl Pts',(14.9311823387923,-55.0284397939552,
-141.829729698383));
#159962=CARTESIAN_POINT('Ctrl Pts',(14.9320397825312,-55.02191156167,-141.812812075282));
#159963=CARTESIAN_POINT('Ctrl Pts',(14.9329047154423,-55.0154036283467,
-141.795735565119));
#159964=CARTESIAN_POINT('Ctrl Pts',(14.9337771219422,-55.0089195179454,
-141.778499819894));
#159965=CARTESIAN_POINT('Ctrl Pts',(14.9342133251921,-55.0056774627447,
-141.769881947281));
#159966=CARTESIAN_POINT('Ctrl Pts',(14.9346513968287,-55.0024413634032,
-141.761224265859));
#159967=CARTESIAN_POINT('Ctrl Pts',(14.9350913346392,-54.9992116625344,
-141.752526735865));
#159968=CARTESIAN_POINT('Ctrl Pts',(14.9353113035444,-54.9975968120999,
-141.748177970869));
#159969=CARTESIAN_POINT('Ctrl Pts',(14.9355317389924,-54.9959835612893,
-141.743819243727));
#159970=CARTESIAN_POINT('Ctrl Pts',(14.9357526406798,-54.9943719656216,
-141.739450549905));
#159971=CARTESIAN_POINT('Ctrl Pts',(14.9358630915235,-54.9935661677878,
-141.737266202994));
#159972=CARTESIAN_POINT('Ctrl Pts',(14.935973658927,-54.9927607837399,-141.735079364413));
#159973=CARTESIAN_POINT('Ctrl Pts',(14.9360843428507,-54.9919558204301,
-141.732890033624));
#159974=CARTESIAN_POINT('Ctrl Pts',(14.9361950267743,-54.9911508571203,
-141.730700702836));
#159975=CARTESIAN_POINT('Ctrl Pts',(14.9363961066168,-54.9896918156194,
-141.726722844862));
#159976=CARTESIAN_POINT('Ctrl Pts',(14.9364167441416,-54.9895421996708,
-141.726314564106));
#159977=CARTESIAN_POINT('Ctrl Pts',(14.9368011783469,-54.9867551654281,
-141.718709141974));
#159978=CARTESIAN_POINT('Ctrl Pts',(14.9373927756583,-54.98247714105,-141.707003732738));
#159979=CARTESIAN_POINT('Ctrl Pts',(14.938192167618,-54.9767793478659,-141.691174512061));
#159980=CARTESIAN_POINT('Ctrl Pts',(14.9389948449638,-54.9710581375703,
-141.67528023556));
#159981=CARTESIAN_POINT('Ctrl Pts',(14.9400070303623,-54.963905484254,-141.655228174497));
#159982=CARTESIAN_POINT('Ctrl Pts',(14.9412297078366,-54.9554440189646,
-141.630979039362));
#159983=CARTESIAN_POINT('Ctrl Pts',(14.9424598255056,-54.9469310642593,
-141.606582344228));
#159984=CARTESIAN_POINT('Ctrl Pts',(14.9439030078284,-54.9370933577308,
-141.577937327112));
#159985=CARTESIAN_POINT('Ctrl Pts',(14.9455605682887,-54.926106419147,-141.544988792767));
#159986=CARTESIAN_POINT('Ctrl Pts',(14.9471371826498,-54.9156560219706,
-141.513649282887));
#159987=CARTESIAN_POINT('Ctrl Pts',(14.9489078803818,-54.9041655803484,
-141.478413650684));
#159988=CARTESIAN_POINT('Ctrl Pts',(14.9508734591455,-54.8918308314158,
-141.439232919092));
#159989=CARTESIAN_POINT('Ctrl Pts',(14.952969209833,-54.8786792045088,-141.397457414244));
#159990=CARTESIAN_POINT('Ctrl Pts',(14.9552864041832,-54.8645681869741,
-141.351199207159));
#159991=CARTESIAN_POINT('Ctrl Pts',(14.9578257449883,-54.8497843490626,
-141.300393708248));
#159992=CARTESIAN_POINT('Ctrl Pts',(14.96045217177,-54.8344935036002,-141.247845849083));
#159993=CARTESIAN_POINT('Ctrl Pts',(14.9633163444726,-54.8184826601245,
-141.190431529181));
#159994=CARTESIAN_POINT('Ctrl Pts',(14.966417593519,-54.8021261312926,-141.128095288101));
#159995=CARTESIAN_POINT('Ctrl Pts',(14.9684798402318,-54.7912494821385,
-141.086643374264));
#159996=CARTESIAN_POINT('Ctrl Pts',(14.9706469074253,-54.7802210749185,
-141.043015008737));
#159997=CARTESIAN_POINT('Ctrl Pts',(14.9729182170701,-54.7691629909176,
-140.997198199071));
#159998=CARTESIAN_POINT('Ctrl Pts',(14.9732348851946,-54.7676212624576,
-140.990810376424));
#159999=CARTESIAN_POINT('Ctrl Pts',(14.973638654121,-54.7656694673371,-140.982663044327));
#160000=CARTESIAN_POINT('Ctrl Pts',(14.9738959858372,-54.7644321620716,
-140.977469374413));
#160001=CARTESIAN_POINT('Ctrl Pts',(14.973919883941,-54.764317254939,-140.976987044195));
#160002=CARTESIAN_POINT('Ctrl Pts',(14.9739425188767,-54.7642084743528,
-140.976530198892));
#160003=CARTESIAN_POINT('Ctrl Pts',(14.9739637034869,-54.7641067028186,
-140.976102619019));
#160004=CARTESIAN_POINT('Ctrl Pts',(14.973980599117,-54.7640255356802,-140.975761605838));
#160005=CARTESIAN_POINT('Ctrl Pts',(14.9739974936203,-54.7639444036372,
-140.97542062491));
#160006=CARTESIAN_POINT('Ctrl Pts',(14.9740143869953,-54.7638633066688,
-140.975079676237));
#160007=CARTESIAN_POINT('Ctrl Pts',(14.9784467764848,-54.7425855364503,
-140.885623465218));
#160008=CARTESIAN_POINT('Ctrl Pts',(14.9828067301753,-54.723752431795,-140.798271020784));
#160009=CARTESIAN_POINT('Ctrl Pts',(14.987060775946,-54.707055598208,-140.713150818449));
#160010=CARTESIAN_POINT('Ctrl Pts',(14.9904460357961,-54.6937686888951,
-140.645414357927));
#160011=CARTESIAN_POINT('Ctrl Pts',(14.9937642982209,-54.6818350048517,
-140.579090323978));
#160012=CARTESIAN_POINT('Ctrl Pts',(14.9970000845746,-54.6711088502559,
-140.514222173991));
#160013=CARTESIAN_POINT('Ctrl Pts',(15.0014481308539,-54.6563642327732,
-140.42505172154));
#160014=CARTESIAN_POINT('Ctrl Pts',(15.0057417382206,-54.6439011362337,
-140.338634645609));
#160015=CARTESIAN_POINT('Ctrl Pts',(15.009844873679,-54.6333747825093,-140.255118196318));
#160016=CARTESIAN_POINT('Ctrl Pts',(15.0124918200861,-54.6265841965165,
-140.201241455562));
#160017=CARTESIAN_POINT('Ctrl Pts',(15.0150595760332,-54.6205999746682,
-140.148570745906));
#160018=CARTESIAN_POINT('Ctrl Pts',(15.0175392245295,-54.6153339077643,
-140.097135088049));
#160019=CARTESIAN_POINT('Ctrl Pts',(15.0215328220096,-54.6068526445736,
-140.0142953977));
#160020=CARTESIAN_POINT('Ctrl Pts',(15.0253095877784,-54.6002281891966,
-139.934627798416));
#160021=CARTESIAN_POINT('Ctrl Pts',(15.0289022436262,-54.5951143157021,
-139.858202621515));
#160022=CARTESIAN_POINT('Ctrl Pts',(15.0325973374102,-54.5898546295637,
-139.779598322056));
#160023=CARTESIAN_POINT('Ctrl Pts',(15.0360977006467,-54.586192768118,-139.704423490692));
#160024=CARTESIAN_POINT('Ctrl Pts',(15.0394393505371,-54.5837870670199,
-139.632711391223));
#160025=CARTESIAN_POINT('Ctrl Pts',(15.0429021798406,-54.5812941271455,
-139.55839877093));
#160026=CARTESIAN_POINT('Ctrl Pts',(15.0461945921169,-54.5801499181639,
-139.487804108145));
#160027=CARTESIAN_POINT('Ctrl Pts',(15.0493567599704,-54.5800138479308,
-139.420926064183));
#160028=CARTESIAN_POINT('Ctrl Pts',(15.0495717712766,-54.5800045958481,
-139.416378697866));
#160029=CARTESIAN_POINT('Ctrl Pts',(15.0497861804124,-54.58000002,-139.411848502024));
#160030=CARTESIAN_POINT('Ctrl Pts',(15.05,-54.58000002,-139.407335470919));
#160031=CARTESIAN_POINT('Ctrl Pts',(9.4,-54.58000002,-136.338455187671));
#160032=CARTESIAN_POINT('Ctrl Pts',(9.39704729586323,-54.58000002,-136.419371231505));
#160033=CARTESIAN_POINT('Ctrl Pts',(9.39392227292272,-54.5816877330307,
-136.504488584693));
#160034=CARTESIAN_POINT('Ctrl Pts',(9.39062236601488,-54.5856390342835,
-136.59370256742));
#160035=CARTESIAN_POINT('Ctrl Pts',(9.38788200014251,-54.5889203423347,
-136.66778918878));
#160036=CARTESIAN_POINT('Ctrl Pts',(9.38502102565691,-54.5937636778588,
-136.744700772334));
#160037=CARTESIAN_POINT('Ctrl Pts',(9.38203789209161,-54.6005250600446,
-136.824372403604));
#160038=CARTESIAN_POINT('Ctrl Pts',(9.38011505691329,-54.6048832368531,
-136.875726260872));
#160039=CARTESIAN_POINT('Ctrl Pts',(9.3781413302498,-54.6100392192402,-136.928230353818));
#160040=CARTESIAN_POINT('Ctrl Pts',(9.37611681763369,-54.6160916434082,
-136.981852222139));
#160041=CARTESIAN_POINT('Ctrl Pts',(9.37274205280644,-54.6261807424036,
-137.071237288815));
#160042=CARTESIAN_POINT('Ctrl Pts',(9.36922644791226,-54.6387598086005,
-137.163720894536));
#160043=CARTESIAN_POINT('Ctrl Pts',(9.36557170761357,-54.6542903138158,
-137.259119078051));
#160044=CARTESIAN_POINT('Ctrl Pts',(9.36208319537106,-54.6691144471737,
-137.350178278955));
#160045=CARTESIAN_POINT('Ctrl Pts',(9.35846800862529,-54.6866285757306,
-137.443890153689));
#160046=CARTESIAN_POINT('Ctrl Pts',(9.35473005845707,-54.7072218231019,
-137.540033202452));
#160047=CARTESIAN_POINT('Ctrl Pts',(9.35379931983142,-54.7123494812818,
-137.563972539534));
#160048=CARTESIAN_POINT('Ctrl Pts',(9.35286098194924,-54.717667930619,-137.588062319807));
#160049=CARTESIAN_POINT('Ctrl Pts',(9.35191512681452,-54.7231829278603,
-137.612298620553));
#160050=CARTESIAN_POINT('Ctrl Pts',(9.35183953638586,-54.7236236729493,
-137.614235526423));
#160051=CARTESIAN_POINT('Ctrl Pts',(9.35169854945555,-54.7244483876958,
-137.617847328509));
#160052=CARTESIAN_POINT('Ctrl Pts',(9.35168821144854,-54.7245089317618,
-137.618112143096));
#160053=CARTESIAN_POINT('Ctrl Pts',(9.35168605247973,-54.724521575664,-137.618167446447));
#160054=CARTESIAN_POINT('Ctrl Pts',(9.35168387518485,-54.7245343276891,
-137.618223219001));
#160055=CARTESIAN_POINT('Ctrl Pts',(9.35168167956414,-54.7245471878765,
-137.618279460739));
#160056=CARTESIAN_POINT('Ctrl Pts',(9.35147996024536,-54.7257286980637,
-137.62344658501));
#160057=CARTESIAN_POINT('Ctrl Pts',(9.35112356583562,-54.7278191281679,
-137.63257494496));
#160058=CARTESIAN_POINT('Ctrl Pts',(9.35061244390952,-54.7308764847684,
-137.645648506862));
#160059=CARTESIAN_POINT('Ctrl Pts',(9.35010078023794,-54.7339370819051,
-137.658735925619));
#160060=CARTESIAN_POINT('Ctrl Pts',(9.3494340527294,-54.7379666976379,-137.675777088558));
#160061=CARTESIAN_POINT('Ctrl Pts',(9.34861195666339,-54.7430751320782,
-137.696747673966));
#160062=CARTESIAN_POINT('Ctrl Pts',(9.34779010329173,-54.7481820584367,
-137.717712068561));
#160063=CARTESIAN_POINT('Ctrl Pts',(9.3468129601163,-54.7543672342593,-137.74260384324));
#160064=CARTESIAN_POINT('Ctrl Pts',(9.34568012941133,-54.761791078744,-137.771387080926));
#160065=CARTESIAN_POINT('Ctrl Pts',(9.34531457307779,-54.764186700048,-137.780675225032));
#160066=CARTESIAN_POINT('Ctrl Pts',(9.34493280503381,-54.7667116947109,
-137.790368480995));
#160067=CARTESIAN_POINT('Ctrl Pts',(9.34453481372685,-54.7693725613995,
-137.800465300292));
#160068=CARTESIAN_POINT('Ctrl Pts',(9.34330447756737,-54.777598269965,-137.83167824806));
#160069=CARTESIAN_POINT('Ctrl Pts',(9.34191917788062,-54.7871182467248,
-137.866746870592));
#160070=CARTESIAN_POINT('Ctrl Pts',(9.34037911805495,-54.7981536480039,
-137.905603545057));
#160071=CARTESIAN_POINT('Ctrl Pts',(9.33886990694295,-54.80896800077,-137.943681887146));
#160072=CARTESIAN_POINT('Ctrl Pts',(9.33721203400933,-54.8212380911684,
-137.985398920108));
#160073=CARTESIAN_POINT('Ctrl Pts',(9.33540626469946,-54.8352146572672,
-138.030666056994));
#160074=CARTESIAN_POINT('Ctrl Pts',(9.3336674674978,-54.8486728625257,-138.074254332924));
#160075=CARTESIAN_POINT('Ctrl Pts',(9.33179153704424,-54.8637135838245,
-138.121134219645));
#160076=CARTESIAN_POINT('Ctrl Pts',(9.32978002863578,-54.8805951415112,
-138.171196804022));
#160077=CARTESIAN_POINT('Ctrl Pts',(9.32933487316683,-54.8843311028907,
-138.18227586943));
#160078=CARTESIAN_POINT('Ctrl Pts',(9.32888308122865,-54.8881573501098,
-138.193510690821));
#160079=CARTESIAN_POINT('Ctrl Pts',(9.3284245409003,-54.8920769088252,-138.204899835357));
#160080=CARTESIAN_POINT('Ctrl Pts',(9.32819527073613,-54.8940366881829,
-138.210594407626));
#160081=CARTESIAN_POINT('Ctrl Pts',(9.32796379497366,-54.8960198682933,
-138.216327536038));
#160082=CARTESIAN_POINT('Ctrl Pts',(9.32773086568275,-54.8980267301276,
-138.222099070016));
#160083=CARTESIAN_POINT('Ctrl Pts',(9.32751634870292,-54.8998749559901,
-138.2274143828));
#160084=CARTESIAN_POINT('Ctrl Pts',(9.32723514384213,-54.9023128701556,
-138.234385797297));
#160085=CARTESIAN_POINT('Ctrl Pts',(9.32706811894936,-54.903767122238,-138.238527565011));
#160086=CARTESIAN_POINT('Ctrl Pts',(9.32705378295467,-54.9038919428547,
-138.238883059087));
#160087=CARTESIAN_POINT('Ctrl Pts',(9.32704028811105,-54.9040094863335,
-138.239217715686));
#160088=CARTESIAN_POINT('Ctrl Pts',(9.3270277487768,-54.904118743943,-138.239528702318));
#160089=CARTESIAN_POINT('Ctrl Pts',(9.32430541485895,-54.9278389582856,
-138.307045002644));
#160090=CARTESIAN_POINT('Ctrl Pts',(9.3217228284678,-54.9516402280944,-138.370752091378));
#160091=CARTESIAN_POINT('Ctrl Pts',(9.31928109292825,-54.9751497452016,
-138.430727718388));
#160092=CARTESIAN_POINT('Ctrl Pts',(9.31678872725691,-54.9991467393225,
-138.491946958333));
#160093=CARTESIAN_POINT('Ctrl Pts',(9.31444308648543,-55.0228397485265,
-138.549279020443));
#160094=CARTESIAN_POINT('Ctrl Pts',(9.31224377986652,-55.0458832512665,
-138.602828549886));
#160095=CARTESIAN_POINT('Ctrl Pts',(9.3099917528066,-55.0694791388429,-138.65766173609));
#160096=CARTESIAN_POINT('Ctrl Pts',(9.30789313238485,-55.0923939685203,
-138.708529504678));
#160097=CARTESIAN_POINT('Ctrl Pts',(9.30594629905539,-55.1143100558499,
-138.755557219429));
#160098=CARTESIAN_POINT('Ctrl Pts',(9.30471092027362,-55.1282170857209,
-138.785399034894));
#160099=CARTESIAN_POINT('Ctrl Pts',(9.30353663826253,-55.1417230294578,
-138.813694821712));
#160100=CARTESIAN_POINT('Ctrl Pts',(9.30242287129985,-55.1547575084923,
-138.840477529059));
#160101=CARTESIAN_POINT('Origin',(-3.3975957231091E-14,-70.08000002,-174.34995));
#160102=CARTESIAN_POINT('',(16.05,-70.08000002,-177.34995));
#160103=CARTESIAN_POINT('Origin',(16.05,-70.08000002,-174.34995));
#160104=CARTESIAN_POINT('',(16.55,-70.08000002,-177.34995));
#160105=CARTESIAN_POINT('',(-41.5,-70.08000002,-177.34995));
#160106=CARTESIAN_POINT('Origin',(16.55,-70.08000002,-174.34995));
#160107=CARTESIAN_POINT('Ctrl Pts',(23.0246263600192,-55.5929437980769,
-150.090116786386));
#160108=CARTESIAN_POINT('Ctrl Pts',(23.9800829025888,-54.5800000200001,
-149.152655882413));
#160109=CARTESIAN_POINT('Ctrl Pts',(25.1782808829885,-54.58000002,-147.977025477683));
#160110=CARTESIAN_POINT('Ctrl Pts',(21.9091489271198,-55.5502169050949,
-148.872607854072));
#160111=CARTESIAN_POINT('Ctrl Pts',(22.8379194752343,-54.5800000199763,
-147.932452641776));
#160112=CARTESIAN_POINT('Ctrl Pts',(23.9836910796608,-54.58000002,-146.759504150767));
#160113=CARTESIAN_POINT('Ctrl Pts',(20.7612402155903,-55.5070450251362,
-147.681892304448));
#160114=CARTESIAN_POINT('Ctrl Pts',(21.6573291961429,-54.58000002,-146.736008441848));
#160115=CARTESIAN_POINT('Ctrl Pts',(22.7503247929853,-54.58000002,-145.568800995698));
#160116=CARTESIAN_POINT('Ctrl Pts',(18.3837542309683,-55.4210082419989,
-145.38143269084));
#160117=CARTESIAN_POINT('Ctrl Pts',(19.2052975266984,-54.58000002,-144.424597244368));
#160118=CARTESIAN_POINT('Ctrl Pts',(20.1860325764608,-54.58000002,-143.268341382183));
#160119=CARTESIAN_POINT('Ctrl Pts',(17.165895474142,-55.3785603713206,-144.282911778325));
#160120=CARTESIAN_POINT('Ctrl Pts',(17.9461389525456,-54.58000002,-143.320329501862));
#160121=CARTESIAN_POINT('Ctrl Pts',(18.8677311043704,-54.58000002,-142.169807438416));
#160122=CARTESIAN_POINT('Ctrl Pts',(15.9085533562516,-55.3376384323294,
-143.252961163042));
#160123=CARTESIAN_POINT('Ctrl Pts',(16.6396978513013,-54.5800000199999,
-142.283025361002));
#160124=CARTESIAN_POINT('Ctrl Pts',(17.5014165897211,-54.58000002,-141.139869854338));
#160125=CARTESIAN_POINT('',(22.984916421119,-55.5914230669928,-150.046801054874));
#160126=CARTESIAN_POINT('',(17.3782102443508,-55.3867109640869,-144.502505142991));
#160127=CARTESIAN_POINT('Ctrl Pts',(22.9849164538399,-55.5914231005407,
-150.046800950003));
#160128=CARTESIAN_POINT('Ctrl Pts',(22.6020780769818,-55.5767655125104,
-149.629451903776));
#160129=CARTESIAN_POINT('Ctrl Pts',(22.2213190936165,-55.5622829699053,
-149.221717836613));
#160130=CARTESIAN_POINT('Ctrl Pts',(21.8422215127712,-55.5479851256212,
-148.82334844634));
#160131=CARTESIAN_POINT('Ctrl Pts',(21.4142808369546,-55.5318451409448,
-148.3736529729));
#160132=CARTESIAN_POINT('Ctrl Pts',(20.9884579263804,-55.5159405513025,
-147.935890439072));
#160133=CARTESIAN_POINT('Ctrl Pts',(20.5641624498949,-55.5002788324557,
-147.509629730204));
#160134=CARTESIAN_POINT('Ctrl Pts',(20.2327692252654,-55.4880463487279,
-147.176701573593));
#160135=CARTESIAN_POINT('Ctrl Pts',(19.9023081409924,-55.4759618754942,
-146.850788120774));
#160136=CARTESIAN_POINT('Ctrl Pts',(19.5724972232793,-55.4640266335675,
-146.531662497644));
#160137=CARTESIAN_POINT('Ctrl Pts',(19.0486801775887,-55.4450706717427,
-146.024816204406));
#160138=CARTESIAN_POINT('Ctrl Pts',(18.5287744522527,-55.4265728425626,
-145.537272372091));
#160139=CARTESIAN_POINT('Ctrl Pts',(18.0112485729538,-55.4085493182614,
-145.068100484788));
#160140=CARTESIAN_POINT('Ctrl Pts',(17.7998985115879,-55.4011887724037,
-144.876497492283));
#160141=CARTESIAN_POINT('Ctrl Pts',(17.5889457822771,-55.3939071830409,
-144.687958082283));
#160142=CARTESIAN_POINT('Ctrl Pts',(17.3782871134249,-55.3867051178887,
-144.502418094197));
#160143=CARTESIAN_POINT('Ctrl Pts',(22.9849163130661,-55.5914230820925,
-150.046801040559));
#160144=CARTESIAN_POINT('Ctrl Pts',(22.9923323585403,-55.5151362910079,
-149.910354009793));
#160145=CARTESIAN_POINT('Ctrl Pts',(23.0003039790552,-55.4387315810897,
-149.763483417317));
#160146=CARTESIAN_POINT('Ctrl Pts',(23.0088478791706,-55.3639556534274,
-149.605771335223));
#160147=CARTESIAN_POINT('Ctrl Pts',(23.0145515654438,-55.3140371821896,
-149.500486836855));
#160148=CARTESIAN_POINT('Ctrl Pts',(23.0205099502732,-55.2648492749479,
-149.390375691817));
#160149=CARTESIAN_POINT('Ctrl Pts',(23.0267233715385,-55.2169338992284,
-149.275390145685));
#160150=CARTESIAN_POINT('Ctrl Pts',(23.0294188144066,-55.1961477409682,
-149.225508292028));
#160151=CARTESIAN_POINT('Ctrl Pts',(23.0321622052024,-55.1756010871455,
-149.174709924356));
#160152=CARTESIAN_POINT('Ctrl Pts',(23.0349533325796,-55.1553378636498,
-149.122995219546));
#160153=CARTESIAN_POINT('Ctrl Pts',(23.0350402445946,-55.1547068936707,
-149.121384892037));
#160154=CARTESIAN_POINT('Ctrl Pts',(23.0351272028841,-55.1540761984596,
-149.11977367623));
#160155=CARTESIAN_POINT('Ctrl Pts',(23.0352142074399,-55.1534457793315,
-149.118161572165));
#160156=CARTESIAN_POINT('Ctrl Pts',(23.0352372417001,-55.1532788772866,
-149.117734771243));
#160157=CARTESIAN_POINT('Ctrl Pts',(23.0352602792032,-55.1531119945928,
-149.117307908062));
#160158=CARTESIAN_POINT('Ctrl Pts',(23.035283319949,-55.1529451312743,-149.116880982623));
#160159=CARTESIAN_POINT('Ctrl Pts',(23.0353061707342,-55.1527796436693,
-149.116457576993));
#160160=CARTESIAN_POINT('Ctrl Pts',(23.0353294471293,-55.1526111157677,
-149.116026283041));
#160161=CARTESIAN_POINT('Ctrl Pts',(23.0353532502873,-55.1524388205629,
-149.115585226208));
#160162=CARTESIAN_POINT('Ctrl Pts',(23.035511384165,-55.1512941947592,-149.112655109648));
#160163=CARTESIAN_POINT('Ctrl Pts',(23.0356895098257,-55.1500072136442,
-149.109354439163));
#160164=CARTESIAN_POINT('Ctrl Pts',(23.0358496447262,-55.1488523761523,
-149.106387027815));
#160165=CARTESIAN_POINT('Ctrl Pts',(23.0359290866495,-55.1482794684903,
-149.104914913591));
#160166=CARTESIAN_POINT('Ctrl Pts',(23.0360041000042,-55.1477390217724,
-149.103524837171));
#160167=CARTESIAN_POINT('Ctrl Pts',(23.0360700429472,-55.1472642440113,
-149.102302828729));
#160168=CARTESIAN_POINT('Ctrl Pts',(23.0361056558454,-55.1470078373164,
-149.101642875439));
#160169=CARTESIAN_POINT('Ctrl Pts',(23.0361386232162,-55.1467705806098,
-149.101031941976));
#160170=CARTESIAN_POINT('Ctrl Pts',(23.0361682136977,-55.14655769005,-149.100483583949));
#160171=CARTESIAN_POINT('Ctrl Pts',(23.0361856980364,-55.146431897888,-149.100159571734));
#160172=CARTESIAN_POINT('Ctrl Pts',(23.0362016408016,-55.1463172195784,
-149.099864126125));
#160173=CARTESIAN_POINT('Ctrl Pts',(23.0362178547074,-55.1462006107733,
-149.099563654823));
#160174=CARTESIAN_POINT('Ctrl Pts',(23.0396466113122,-55.1215413326975,
-149.036022952368));
#160175=CARTESIAN_POINT('Ctrl Pts',(23.043400856158,-55.0954814004763,-148.966402766032));
#160176=CARTESIAN_POINT('Ctrl Pts',(23.047485051108,-55.06851563719,-148.890588284903));
#160177=CARTESIAN_POINT('Ctrl Pts',(23.0510706678576,-55.0448417201287,
-148.824028858447));
#160178=CARTESIAN_POINT('Ctrl Pts',(23.0549106126203,-55.0204708888616,
-148.752694757299));
#160179=CARTESIAN_POINT('Ctrl Pts',(23.0590081665062,-54.9957694317052,
-148.676498447966));
#160180=CARTESIAN_POINT('Ctrl Pts',(23.0640392087417,-54.9654405873036,
-148.582943399974));
#160181=CARTESIAN_POINT('Ctrl Pts',(23.0694582576189,-54.9346164108002,
-148.482065220825));
#160182=CARTESIAN_POINT('Ctrl Pts',(23.0752666835093,-54.9040407392492,
-148.373778900728));
#160183=CARTESIAN_POINT('Ctrl Pts',(23.0796325654284,-54.8810586483851,
-148.292385887212));
#160184=CARTESIAN_POINT('Ctrl Pts',(23.0842183659314,-54.8582185778991,
-148.206808519094));
#160185=CARTESIAN_POINT('Ctrl Pts',(23.0890230063924,-54.8358481589629,
-148.117037145628));
#160186=CARTESIAN_POINT('Ctrl Pts',(23.0891989614022,-54.8350289119632,
-148.113749548352));
#160187=CARTESIAN_POINT('Ctrl Pts',(23.0893167643732,-54.8344810902222,
-148.111548434336));
#160188=CARTESIAN_POINT('Ctrl Pts',(23.0895517726634,-54.8333923203654,
-148.107157489765));
#160189=CARTESIAN_POINT('Ctrl Pts',(23.0896456095871,-54.8329575833015,
-148.105404220845));
#160190=CARTESIAN_POINT('Ctrl Pts',(23.0897393535851,-54.8325239285302,
-148.103653010558));
#160191=CARTESIAN_POINT('Ctrl Pts',(23.0898330043309,-54.8320913515626,
-148.101903859584));
#160192=CARTESIAN_POINT('Ctrl Pts',(23.0938754387013,-54.8134191670809,
-148.026401759117));
#160193=CARTESIAN_POINT('Ctrl Pts',(23.0977452975731,-54.7967897346283,
-147.954711586754));
#160194=CARTESIAN_POINT('Ctrl Pts',(23.101415260951,-54.7818805610517,-147.88691339402));
#160195=CARTESIAN_POINT('Ctrl Pts',(23.1044740759873,-54.7694541688457,
-147.830405437396));
#160196=CARTESIAN_POINT('Ctrl Pts',(23.107394083234,-54.7582234867518,-147.776600243719));
#160197=CARTESIAN_POINT('Ctrl Pts',(23.1101606721181,-54.7480218486682,
-147.72552530494));
#160198=CARTESIAN_POINT('Ctrl Pts',(23.1136624974754,-54.735109068192,-147.660876915449));
#160199=CARTESIAN_POINT('Ctrl Pts',(23.1169202344087,-54.7238435469161,
-147.600604046303));
#160200=CARTESIAN_POINT('Ctrl Pts',(23.1199182264117,-54.7139339125423,
-147.544776848901));
#160201=CARTESIAN_POINT('Ctrl Pts',(23.1221963802289,-54.7064036485017,
-147.502354139724));
#160202=CARTESIAN_POINT('Ctrl Pts',(23.1243245925392,-54.6996572049997,
-147.462497765974));
#160203=CARTESIAN_POINT('Ctrl Pts',(23.1262966067565,-54.6935835813359,
-147.42522765844));
#160204=CARTESIAN_POINT('Ctrl Pts',(23.1289486271487,-54.6854156007658,
-147.375105765641));
#160205=CARTESIAN_POINT('Ctrl Pts',(23.1313298271167,-54.6784587434828,
-147.329648473762));
#160206=CARTESIAN_POINT('Ctrl Pts',(23.1334524318317,-54.6724823078343,
-147.28888161716));
#160207=CARTESIAN_POINT('Ctrl Pts',(23.1349852367621,-54.6681665207434,
-147.259442485911));
#160208=CARTESIAN_POINT('Ctrl Pts',(23.1363832071279,-54.6643630279866,
-147.232448787815));
#160209=CARTESIAN_POINT('Ctrl Pts',(23.1376511232448,-54.6610006647087,
-147.207904179543));
#160210=CARTESIAN_POINT('Ctrl Pts',(23.1391629766815,-54.6569914085686,
-147.178637377213));
#160211=CARTESIAN_POINT('Ctrl Pts',(23.1404905826859,-54.653608787909,-147.152853815656));
#160212=CARTESIAN_POINT('Ctrl Pts',(23.1416434646309,-54.6507567724492,
-147.130558272819));
#160213=CARTESIAN_POINT('Ctrl Pts',(23.1422199056034,-54.6493307647194,
-147.1194105014));
#160214=CARTESIAN_POINT('Ctrl Pts',(23.1427526592662,-54.6480378218892,
-147.109134681098));
#160215=CARTESIAN_POINT('Ctrl Pts',(23.1432428112175,-54.6468684071695,
-147.099731151217));
#160216=CARTESIAN_POINT('Ctrl Pts',(23.1434878871932,-54.6462836998097,
-147.095029386276));
#160217=CARTESIAN_POINT('Ctrl Pts',(23.1437223155898,-54.6457298994562,
-147.090545691006));
#160218=CARTESIAN_POINT('Ctrl Pts',(23.1439462156013,-54.6452059677569,
-147.086280097254));
#160219=CARTESIAN_POINT('Ctrl Pts',(23.144058165607,-54.6449440019072,-147.084147300378));
#160220=CARTESIAN_POINT('Ctrl Pts',(23.1441674836954,-54.6446895047668,
-147.082069028698));
#160221=CARTESIAN_POINT('Ctrl Pts',(23.1442741846894,-54.6444423559743,
-147.080045285498));
#160222=CARTESIAN_POINT('Ctrl Pts',(23.1443275351864,-54.644318781578,-147.079033413898));
#160223=CARTESIAN_POINT('Ctrl Pts',(23.1443802314206,-54.6441970443651,
-147.078035174407));
#160224=CARTESIAN_POINT('Ctrl Pts',(23.1444322751837,-54.6440771298857,
-147.0770505674));
#160225=CARTESIAN_POINT('Ctrl Pts',(23.1444452861244,-54.6440471512658,
-147.076804415648));
#160226=CARTESIAN_POINT('Ctrl Pts',(23.144451223023,-54.6440334560348,-147.076691896758));
#160227=CARTESIAN_POINT('Ctrl Pts',(23.1444553594622,-54.6440239044945,
-147.076613426546));
#160228=CARTESIAN_POINT('Ctrl Pts',(23.1444615641209,-54.644009577184,-147.076495721228));
#160229=CARTESIAN_POINT('Ctrl Pts',(23.1444637176774,-54.6440045725571,
-147.076454625506));
#160230=CARTESIAN_POINT('Ctrl Pts',(23.1444796267811,-54.6439679929986,
-147.076154034201));
#160231=CARTESIAN_POINT('Ctrl Pts',(23.1444955358848,-54.6439314134401,
-147.075853442895));
#160232=CARTESIAN_POINT('Ctrl Pts',(23.144525196082,-54.6438632191539,-147.075293360595));
#160233=CARTESIAN_POINT('Ctrl Pts',(23.1445864508551,-54.6437228405878,
-147.074137644174));
#160234=CARTESIAN_POINT('Ctrl Pts',(23.1503046784119,-54.630618284894,-146.966249733404));
#160235=CARTESIAN_POINT('Ctrl Pts',(23.1558442763692,-54.61994345285,-146.86156040566));
#160236=CARTESIAN_POINT('Ctrl Pts',(23.1612011702211,-54.6113286071025,
-146.760176180277));
#160237=CARTESIAN_POINT('Ctrl Pts',(23.1666962989783,-54.6024914548433,
-146.656175730048));
#160238=CARTESIAN_POINT('Ctrl Pts',(23.1719991942556,-54.5958218840169,
-146.555652779676));
#160239=CARTESIAN_POINT('Ctrl Pts',(23.1771079416158,-54.5909508424003,
-146.458674807921));
#160240=CARTESIAN_POINT('Ctrl Pts',(23.1824197384654,-54.5858861990172,
-146.357842402532));
#160241=CARTESIAN_POINT('Ctrl Pts',(23.1875216668299,-54.5827657185001,
-146.260842041119));
#160242=CARTESIAN_POINT('Ctrl Pts',(23.1924139148337,-54.5812088322433,
-146.167704256954));
#160243=CARTESIAN_POINT('Ctrl Pts',(23.1950011320887,-54.580385488254,-146.118449255553));
#160244=CARTESIAN_POINT('Ctrl Pts',(23.1975297444135,-54.58000002,-146.07027379222));
#160245=CARTESIAN_POINT('Ctrl Pts',(23.2,-54.58000002,-146.023178055809));
#160246=CARTESIAN_POINT('Ctrl Pts',(17.55,-54.58000002,-141.176536909659));
#160247=CARTESIAN_POINT('Ctrl Pts',(17.5450917051411,-54.58000002,-141.274872500695));
#160248=CARTESIAN_POINT('Ctrl Pts',(17.5399505125397,-54.5819438994493,
-141.377555492718));
#160249=CARTESIAN_POINT('Ctrl Pts',(17.5345757892522,-54.586403208251,-141.484515818682));
#160250=CARTESIAN_POINT('Ctrl Pts',(17.5299889335016,-54.5902088378856,
-141.575797092152));
#160251=CARTESIAN_POINT('Ctrl Pts',(17.5252317046863,-54.5958480133051,
-141.670199207096));
#160252=CARTESIAN_POINT('Ctrl Pts',(17.5203055297054,-54.6037022322593,
-141.767641241343));
#160253=CARTESIAN_POINT('Ctrl Pts',(17.5179769395429,-54.607414901229,-141.813701838711));
#160254=CARTESIAN_POINT('Ctrl Pts',(17.5156106073861,-54.6116228337644,
-141.860441523156));
#160255=CARTESIAN_POINT('Ctrl Pts',(17.5132068481431,-54.6163676372864,
-141.907848522614));
#160256=CARTESIAN_POINT('Ctrl Pts',(17.5121552034742,-54.6184434888273,
-141.928589084877));
#160257=CARTESIAN_POINT('Ctrl Pts',(17.5110963946809,-54.6206221127213,
-141.949457382844));
#160258=CARTESIAN_POINT('Ctrl Pts',(17.510030454982,-54.6229070275371,-141.970452299473));
#160259=CARTESIAN_POINT('Ctrl Pts',(17.5095307957482,-54.623978081357,-141.980293666643));
#160260=CARTESIAN_POINT('Ctrl Pts',(17.509029569696,-54.6250724904199,-141.990162854726));
#160261=CARTESIAN_POINT('Ctrl Pts',(17.5085267804883,-54.6261906184793,
-142.000059744165));
#160262=CARTESIAN_POINT('Ctrl Pts',(17.5082832419657,-54.626732211758,-142.004853549987));
#160263=CARTESIAN_POINT('Ctrl Pts',(17.5080393366981,-54.627279369982,-142.009653855059));
#160264=CARTESIAN_POINT('Ctrl Pts',(17.5077950651136,-54.6278321345572,
-142.01446064557));
#160265=CARTESIAN_POINT('Ctrl Pts',(17.5076748376931,-54.6281041983715,
-142.016826487775));
#160266=CARTESIAN_POINT('Ctrl Pts',(17.5075545215335,-54.6283776203157,
-142.019193901055));
#160267=CARTESIAN_POINT('Ctrl Pts',(17.5074341166875,-54.6286524053284,
-142.021562883736));
#160268=CARTESIAN_POINT('Ctrl Pts',(17.5074008878149,-54.6287282394536,
-142.022216666587));
#160269=CARTESIAN_POINT('Ctrl Pts',(17.5073676521877,-54.628804177394,-142.022870568969));
#160270=CARTESIAN_POINT('Ctrl Pts',(17.507334409807,-54.6288802192535,-142.023524590846));
#160271=CARTESIAN_POINT('Ctrl Pts',(17.5073152865459,-54.6289239636637,
-142.023900828374));
#160272=CARTESIAN_POINT('Ctrl Pts',(17.5072956614674,-54.6289688853366,
-142.024286934388));
#160273=CARTESIAN_POINT('Ctrl Pts',(17.5072756270475,-54.6290147768759,
-142.024681088858));
#160274=CARTESIAN_POINT('Ctrl Pts',(17.5071508485213,-54.6293005989114,
-142.027135964734));
#160275=CARTESIAN_POINT('Ctrl Pts',(17.5070105236846,-54.6296234749094,
-142.029896478475));
#160276=CARTESIAN_POINT('Ctrl Pts',(17.5068832231264,-54.6299177400483,
-142.032400569581));
#160277=CARTESIAN_POINT('Ctrl Pts',(17.5068200701151,-54.6300637231445,
-142.033642833528));
#160278=CARTESIAN_POINT('Ctrl Pts',(17.5067601224481,-54.6302026255319,
-142.034821996459));
#160279=CARTESIAN_POINT('Ctrl Pts',(17.5067068681503,-54.6303262282003,
-142.035869470081));
#160280=CARTESIAN_POINT('Ctrl Pts',(17.506674018948,-54.6304024708555,-142.036515590195));
#160281=CARTESIAN_POINT('Ctrl Pts',(17.5066437164855,-54.6304728896107,
-142.037111604628));
#160282=CARTESIAN_POINT('Ctrl Pts',(17.506616779378,-54.6305355398635,-142.037641418545));
#160283=CARTESIAN_POINT('Ctrl Pts',(17.5066046036626,-54.6305638581099,
-142.037880897245));
#160284=CARTESIAN_POINT('Ctrl Pts',(17.5065931155187,-54.6305905890773,
-142.038106850617));
#160285=CARTESIAN_POINT('Ctrl Pts',(17.506582390544,-54.6306155528778,-142.038317792377));
#160286=CARTESIAN_POINT('Ctrl Pts',(17.506573757314,-54.630635647865,-142.038487593124));
#160287=CARTESIAN_POINT('Ctrl Pts',(17.5065651450398,-54.6306557000247,
-142.038656980808));
#160288=CARTESIAN_POINT('Ctrl Pts',(17.506556518266,-54.6306757918954,-142.038826652775));
#160289=CARTESIAN_POINT('Ctrl Pts',(17.5040536558753,-54.6365049916146,
-142.088053118458));
#160290=CARTESIAN_POINT('Ctrl Pts',(17.5013190433547,-54.6433710812195,
-142.141762487752));
#160291=CARTESIAN_POINT('Ctrl Pts',(17.4983522495595,-54.6515789268995,
-142.199919204864));
#160292=CARTESIAN_POINT('Ctrl Pts',(17.4954972359002,-54.6594775248973,
-142.255884746523));
#160293=CARTESIAN_POINT('Ctrl Pts',(17.4924272058954,-54.6686189847917,
-142.315968772406));
#160294=CARTESIAN_POINT('Ctrl Pts',(17.4891419225996,-54.679319857396,-142.380131530805));
#160295=CARTESIAN_POINT('Ctrl Pts',(17.4857310844324,-54.690429689156,-142.446746420771));
#160296=CARTESIAN_POINT('Ctrl Pts',(17.4820881710593,-54.703220657768,-142.517758749746));
#160297=CARTESIAN_POINT('Ctrl Pts',(17.4782149173148,-54.7180889605125,
-142.593080227175));
#160298=CARTESIAN_POINT('Ctrl Pts',(17.4745803202652,-54.7320411291163,
-142.663760651876));
#160299=CARTESIAN_POINT('Ctrl Pts',(17.4707427448971,-54.7478238397983,
-142.738238326382));
#160300=CARTESIAN_POINT('Ctrl Pts',(17.4667050220054,-54.7657948260213,
-142.816410456738));
#160301=CARTESIAN_POINT('Ctrl Pts',(17.4659350887227,-54.7692216239439,
-142.831316711218));
#160302=CARTESIAN_POINT('Ctrl Pts',(17.4652069807158,-54.7725054352608,
-142.845407203427));
#160303=CARTESIAN_POINT('Ctrl Pts',(17.464419503232,-54.7761059998999,-142.860639856961));
#160304=CARTESIAN_POINT('Ctrl Pts',(17.4640753193298,-54.7776797037997,
-142.867297614473));
#160305=CARTESIAN_POINT('Ctrl Pts',(17.4637197951665,-54.7793145283239,
-142.874173452564));
#160306=CARTESIAN_POINT('Ctrl Pts',(17.4633444876872,-54.7810519867353,
-142.881430292926));
#160307=CARTESIAN_POINT('Ctrl Pts',(17.4633288972216,-54.7811241616509,
-142.881731745805));
#160308=CARTESIAN_POINT('Ctrl Pts',(17.4633132725516,-54.7811965147846,
-142.882033857305));
#160309=CARTESIAN_POINT('Ctrl Pts',(17.4632976130715,-54.7812690492069,
-142.882336639101));
#160310=CARTESIAN_POINT('Ctrl Pts',(17.4594620331563,-54.7990353844282,
-142.956498984717));
#160311=CARTESIAN_POINT('Ctrl Pts',(17.4558121806766,-54.8170427731732,
-143.026475741498));
#160312=CARTESIAN_POINT('Ctrl Pts',(17.4523678570115,-54.8349227405346,
-143.092287995376));
#160313=CARTESIAN_POINT('Ctrl Pts',(17.4488287514492,-54.8532947340214,
-143.159911289936));
#160314=CARTESIAN_POINT('Ctrl Pts',(17.4455065947382,-54.8715319753916,
-143.223138340297));
#160315=CARTESIAN_POINT('Ctrl Pts',(17.4424195593159,-54.889281955583,-143.282020423993));
#160316=CARTESIAN_POINT('Ctrl Pts',(17.4406460230073,-54.8994795173338,
-143.315848838337));
#160317=CARTESIAN_POINT('Ctrl Pts',(17.4389500348636,-54.9095171355183,
-143.348243606101));
#160318=CARTESIAN_POINT('Ctrl Pts',(17.4373346637261,-54.9193351262199,
-143.379217340403));
#160319=CARTESIAN_POINT('Ctrl Pts',(17.4344710960841,-54.9367394736354,
-143.434124464369));
#160320=CARTESIAN_POINT('Ctrl Pts',(17.4318523790683,-54.9534516177662,
-143.484562021165));
#160321=CARTESIAN_POINT('Ctrl Pts',(17.4294659557099,-54.9691829188542,
-143.530596689604));
#160322=CARTESIAN_POINT('Ctrl Pts',(17.4288674276149,-54.9731284156327,
-143.542142437474));
#160323=CARTESIAN_POINT('Ctrl Pts',(17.4282835109883,-54.9770124679958,
-143.553411265062));
#160324=CARTESIAN_POINT('Ctrl Pts',(17.4277140070979,-54.9808310311818,
-143.564404279982));
#160325=CARTESIAN_POINT('Ctrl Pts',(17.4262939054524,-54.9903529114631,
-143.591816206117));
#160326=CARTESIAN_POINT('Ctrl Pts',(17.4249630047959,-54.9994670858898,
-143.617512975608));
#160327=CARTESIAN_POINT('Ctrl Pts',(17.423716451303,-55.0081165229018,-143.641510951399));
#160328=CARTESIAN_POINT('Ctrl Pts',(17.4230931745566,-55.0124412414077,
-143.653509939294));
#160329=CARTESIAN_POINT('Ctrl Pts',(17.422491013171,-55.0166498780522,-143.665084192978));
#160330=CARTESIAN_POINT('Ctrl Pts',(17.4219092597331,-55.0207360609758,
-143.676235714181));
#160331=CARTESIAN_POINT('Ctrl Pts',(17.4216183830142,-55.0227791524376,
-143.681811474783));
#160332=CARTESIAN_POINT('Ctrl Pts',(17.4213326100765,-55.0247916370273,
-143.687281550016));
#160333=CARTESIAN_POINT('Ctrl Pts',(17.4210518583609,-55.0267727596454,
-143.692646178384));
#160334=CARTESIAN_POINT('Ctrl Pts',(17.4209114825031,-55.0277633209545,
-143.695328492568));
#160335=CARTESIAN_POINT('Ctrl Pts',(17.4207723620668,-55.0287460421781,
-143.697984444891));
#160336=CARTESIAN_POINT('Ctrl Pts',(17.420634486589,-55.0297208317899,-143.700614064785));
#160337=CARTESIAN_POINT('Ctrl Pts',(17.4205655488501,-55.0302082265958,
-143.701928874731));
#160338=CARTESIAN_POINT('Ctrl Pts',(17.4204969223581,-55.0306936385243,
-143.703237101561));
#160339=CARTESIAN_POINT('Ctrl Pts',(17.4204286057972,-55.0311770563127,
-143.704538748928));
#160340=CARTESIAN_POINT('Ctrl Pts',(17.4203602892364,-55.0316604741012,
-143.705840396294));
#160341=CARTESIAN_POINT('Ctrl Pts',(17.4203512686763,-55.0317241749196,
-143.706012785973));
#160342=CARTESIAN_POINT('Ctrl Pts',(17.4202245846065,-55.0326213161048,
-143.708423956259));
#160343=CARTESIAN_POINT('Ctrl Pts',(17.4153263458864,-55.0673092740967,
-143.801651839429));
#160344=CARTESIAN_POINT('Ctrl Pts',(17.4106301495559,-55.1027402694995,
-143.89080847027));
#160345=CARTESIAN_POINT('Ctrl Pts',(17.4061366729319,-55.1384916270083,
-143.975935221091));
#160346=CARTESIAN_POINT('Ctrl Pts',(17.4015130535561,-55.1752784366707,
-144.063527463676));
#160347=CARTESIAN_POINT('Ctrl Pts',(17.3971040350605,-55.2124042647293,
-144.146853581447));
#160348=CARTESIAN_POINT('Ctrl Pts',(17.392907680499,-55.2494458827254,-144.226000408684));
#160349=CARTESIAN_POINT('Ctrl Pts',(17.3885528009809,-55.2878868154835,
-144.308137151852));
#160350=CARTESIAN_POINT('Ctrl Pts',(17.3844269236483,-55.3262368051947,
-144.385773482634));
#160351=CARTESIAN_POINT('Ctrl Pts',(17.3805255402537,-55.364065723145,-144.459041732615));
#160352=CARTESIAN_POINT('Ctrl Pts',(17.3797455324459,-55.3716288996847,
-144.473690333193));
#160353=CARTESIAN_POINT('Ctrl Pts',(17.3789744919001,-55.3791713871413,
-144.488164422799));
#160354=CARTESIAN_POINT('Ctrl Pts',(17.3782123737203,-55.3866899569193,
-144.502465186451));
#160355=CARTESIAN_POINT('Ctrl Pts',(41.5,-55.58000002,-171.14995));
#160356=CARTESIAN_POINT('Ctrl Pts',(41.5,-54.58000002,-171.14995));
#160357=CARTESIAN_POINT('Ctrl Pts',(42.5,-54.58000002,-171.14995));
#160358=CARTESIAN_POINT('Ctrl Pts',(41.5,-55.58000002,-171.64995));
#160359=CARTESIAN_POINT('Ctrl Pts',(41.5,-54.58000002,-171.64995));
#160360=CARTESIAN_POINT('Ctrl Pts',(42.5,-54.58000002,-171.64995));
#160361=CARTESIAN_POINT('Ctrl Pts',(42.,-55.58000002,-171.64995));
#160362=CARTESIAN_POINT('Ctrl Pts',(42.,-55.08000002,-171.64995));
#160363=CARTESIAN_POINT('Ctrl Pts',(42.5,-55.08000002,-171.64995));
#160364=CARTESIAN_POINT('',(41.5,-55.58000002,-171.14995));
#160365=CARTESIAN_POINT('',(42.,-55.58000002,-171.64995));
#160366=CARTESIAN_POINT('Origin',(42.,-55.58000002,-171.14995));
#160367=CARTESIAN_POINT('',(42.5,-55.08000002,-171.64995));
#160368=CARTESIAN_POINT('Origin',(42.5,-55.58000002,-171.64995));
#160369=CARTESIAN_POINT('',(42.5,-54.58000002,-171.14995));
#160370=CARTESIAN_POINT('Origin',(42.5,-55.08000002,-171.14995));
#160371=CARTESIAN_POINT('Origin',(42.5,-55.58000002,-171.14995));
#160372=CARTESIAN_POINT('Ctrl Pts',(26.0394480946395,-65.5149709682656,
-172.038055421481));
#160373=CARTESIAN_POINT('Ctrl Pts',(26.1751497442534,-65.4958993451584,
-171.625426858395));
#160374=CARTESIAN_POINT('Ctrl Pts',(26.2234488624093,-65.1680142434972,
-171.34400271074));
#160375=CARTESIAN_POINT('Ctrl Pts',(26.3688360080808,-65.4686785159697,
-172.14852124047));
#160376=CARTESIAN_POINT('Ctrl Pts',(26.5059850091802,-65.4494034808673,
-171.691392643103));
#160377=CARTESIAN_POINT('Ctrl Pts',(26.5325022452051,-65.072358231615,-171.399245459895));
#160378=CARTESIAN_POINT('Ctrl Pts',(26.7013989289162,-65.4219398454845,
-172.23811459301));
#160379=CARTESIAN_POINT('Ctrl Pts',(26.8344935945357,-65.4032346100804,
-171.736704292719));
#160380=CARTESIAN_POINT('Ctrl Pts',(26.843027692162,-64.9750314285332,-171.444032296926));
#160381=CARTESIAN_POINT('Ctrl Pts',(27.3705571684413,-65.3278957879536,
-172.38942269823));
#160382=CARTESIAN_POINT('Ctrl Pts',(27.4914924972326,-65.3108994359038,
-171.799283317704));
#160383=CARTESIAN_POINT('Ctrl Pts',(27.4650077428683,-64.7776672125821,
-171.519686348695));
#160384=CARTESIAN_POINT('Ctrl Pts',(27.7072474293082,-65.2805770576552,
-172.450796940493));
#160385=CARTESIAN_POINT('Ctrl Pts',(27.8213068579945,-65.2645470503453,
-171.81528847728));
#160386=CARTESIAN_POINT('Ctrl Pts',(27.7764978537267,-64.6776202239548,
-171.550373470332));
#160387=CARTESIAN_POINT('Ctrl Pts',(28.7226827355371,-65.1378669321315,
-172.598633897542));
#160388=CARTESIAN_POINT('Ctrl Pts',(28.8291547927028,-65.1229032603379,
-171.822805263071));
#160389=CARTESIAN_POINT('Ctrl Pts',(28.7113572324553,-64.3737932440126,
-171.624291948599));
#160390=CARTESIAN_POINT('Ctrl Pts',(29.4067311934443,-65.0417301908804,
-172.64994999751));
#160391=CARTESIAN_POINT('Ctrl Pts',(29.4938163229,-65.0294911740669,-171.766054775631));
#160392=CARTESIAN_POINT('Ctrl Pts',(29.3350621276793,-64.1663451413114,
-171.64995));
#160393=CARTESIAN_POINT('Ctrl Pts',(30.098151667932,-64.9445573802656,-172.64995));
#160394=CARTESIAN_POINT('Ctrl Pts',(30.098151667932,-64.9445573802655,-171.64995));
#160395=CARTESIAN_POINT('Ctrl Pts',(29.958978566972,-63.954289311524,-171.64995));
#160396=CARTESIAN_POINT('',(30.098151667932,-64.9445573802656,-172.64995));
#160397=CARTESIAN_POINT('Origin',(29.958978566972,-63.954289311524,-172.64995));
#160398=CARTESIAN_POINT('',(26.0394480946395,-65.5149709682656,-172.038055421481));
#160399=CARTESIAN_POINT('Origin',(25.9002749936795,-64.5247028995241,-172.038055421481));
#160400=CARTESIAN_POINT('Ctrl Pts',(30.098151667932,-64.9445573802656,-172.64995));
#160401=CARTESIAN_POINT('Ctrl Pts',(29.5972390119403,-65.0149560630516,
-172.649949998196));
#160402=CARTESIAN_POINT('Ctrl Pts',(29.1003075630642,-65.0847952236665,
-172.623020954985));
#160403=CARTESIAN_POINT('Ctrl Pts',(28.6071269715803,-65.1541072356527,
-172.570721117633));
#160404=CARTESIAN_POINT('Ctrl Pts',(28.4194541761964,-65.1804829269669,
-172.550819165198));
#160405=CARTESIAN_POINT('Ctrl Pts',(28.2323246108958,-65.2067822722717,
-172.527242787954));
#160406=CARTESIAN_POINT('Ctrl Pts',(28.0457258647366,-65.2330070158113,
-172.500075926044));
#160407=CARTESIAN_POINT('Ctrl Pts',(27.7072474293089,-65.2805770576551,
-172.450796940499));
#160408=CARTESIAN_POINT('Ctrl Pts',(27.3705571686055,-65.3278957879305,
-172.389422697018));
#160409=CARTESIAN_POINT('Ctrl Pts',(27.0359780488069,-65.3749178167011,
-172.313768645042));
#160410=CARTESIAN_POINT('Ctrl Pts',(26.7013989290084,-65.4219398454716,
-172.238114593065));
#160411=CARTESIAN_POINT('Ctrl Pts',(26.3688785032062,-65.4686725436693,
-172.14853549193));
#160412=CARTESIAN_POINT('Ctrl Pts',(26.0394480946395,-65.5149709682656,
-172.038055421481));
#160413=CARTESIAN_POINT('Origin',(45.4220505312374,-61.7810962706031,-172.64995));
#160414=CARTESIAN_POINT('',(31.28041344952,-64.7784013226445,-172.64995));
#160415=CARTESIAN_POINT('',(27.530675086669,-65.3053926820751,-172.64995));
#160416=CARTESIAN_POINT('Ctrl Pts',(31.2804134495199,-64.7784013226445,
-172.64995));
#160417=CARTESIAN_POINT('Ctrl Pts',(31.2804134495199,-64.7784013226445,
-172.608983203817));
#160418=CARTESIAN_POINT('Ctrl Pts',(31.2806213080456,-64.7758267410213,
-172.567620053161));
#160419=CARTESIAN_POINT('Ctrl Pts',(31.2810194383274,-64.7705524414083,
-172.52618728165));
#160420=CARTESIAN_POINT('Ctrl Pts',(31.28141235728,-64.76534717978,-172.485296844715));
#160421=CARTESIAN_POINT('Ctrl Pts',(31.2819905477625,-64.7575120457041,
-172.444338940269));
#160422=CARTESIAN_POINT('Ctrl Pts',(31.2827427524648,-64.7469669392553,
-172.403658150027));
#160423=CARTESIAN_POINT('Ctrl Pts',(31.2834809680707,-64.7366179449949,
-172.363733919128));
#160424=CARTESIAN_POINT('Ctrl Pts',(31.2843867483343,-64.7236585728548,
-172.324077002608));
#160425=CARTESIAN_POINT('Ctrl Pts',(31.2854555737588,-64.7080566649442,
-172.285037095554));
#160426=CARTESIAN_POINT('Ctrl Pts',(31.2865128315013,-64.6926236133354,
-172.246419709538));
#160427=CARTESIAN_POINT('Ctrl Pts',(31.2877295873979,-64.6746046531694,
-172.208406475053));
#160428=CARTESIAN_POINT('Ctrl Pts',(31.2891080729451,-64.6540156623694,
-172.171353409327));
#160429=CARTESIAN_POINT('Ctrl Pts',(31.2904653774001,-64.633743031297,-172.134869681744));
#160430=CARTESIAN_POINT('Ctrl Pts',(31.2919794574909,-64.610978585132,-172.099317309204));
#160431=CARTESIAN_POINT('Ctrl Pts',(31.2936593097591,-64.585786337593,-172.065046652145));
#160432=CARTESIAN_POINT('Ctrl Pts',(31.2944218099435,-64.5743513478863,
-172.049490889995));
#160433=CARTESIAN_POINT('Ctrl Pts',(31.2952185612475,-64.5624168365768,
-172.034199306284));
#160434=CARTESIAN_POINT('Ctrl Pts',(31.2960508993985,-64.54999230786,-172.019204984951));
#160435=CARTESIAN_POINT('Ctrl Pts',(31.2967847052814,-64.539038596013,-172.005985692778));
#160436=CARTESIAN_POINT('Ctrl Pts',(31.2975461754486,-64.527704046776,-171.992997455514));
#160437=CARTESIAN_POINT('Ctrl Pts',(31.2983364317961,-64.515996642854,-171.980262947379));
#160438=CARTESIAN_POINT('Ctrl Pts',(31.2986919487447,-64.5107297689691,
-171.9745340045));
#160439=CARTESIAN_POINT('Ctrl Pts',(31.2990750220731,-64.5051055721233,
-171.968556625651));
#160440=CARTESIAN_POINT('Ctrl Pts',(31.2994555591239,-64.4994990189348,
-171.962743472258));
#160441=CARTESIAN_POINT('Ctrl Pts',(31.2998484999594,-64.4937097174994,
-171.956740836387));
#160442=CARTESIAN_POINT('Ctrl Pts',(31.3002387617528,-64.4879394084972,
-171.950913444372));
#160443=CARTESIAN_POINT('Ctrl Pts',(31.3005989639997,-64.4826418592774,
-171.945675867995));
#160444=CARTESIAN_POINT('Ctrl Pts',(31.3006653264322,-64.4816658568904,
-171.9447109148));
#160445=CARTESIAN_POINT('Ctrl Pts',(31.3007306824748,-64.4807060005262,
-171.943765878233));
#160446=CARTESIAN_POINT('Ctrl Pts',(31.3007948782761,-64.4797652514731,
-171.942843218813));
#160447=CARTESIAN_POINT('Ctrl Pts',(31.3023230365058,-64.4573710546937,
-171.920879639337));
#160448=CARTESIAN_POINT('Ctrl Pts',(31.3039802192176,-64.4332657575141,
-171.899286273904));
#160449=CARTESIAN_POINT('Ctrl Pts',(31.3057568294339,-64.4073810738904,
-171.87835788998));
#160450=CARTESIAN_POINT('Ctrl Pts',(31.3074846180388,-64.3822077066572,
-171.858004622318));
#160451=CARTESIAN_POINT('Ctrl Pts',(31.3093252995898,-64.3553509713006,
-171.838280617927));
#160452=CARTESIAN_POINT('Ctrl Pts',(31.3112753249902,-64.3267856146847,
-171.819487496162));
#160453=CARTESIAN_POINT('Ctrl Pts',(31.3132253503906,-64.2982202580688,
-171.800694374398));
#160454=CARTESIAN_POINT('Ctrl Pts',(31.3152846337614,-64.2679456691333,
-171.782832445245));
#160455=CARTESIAN_POINT('Ctrl Pts',(31.3174561053801,-64.2359826978855,
-171.766229742061));
#160456=CARTESIAN_POINT('Ctrl Pts',(31.3185520676279,-64.2198506842245,
-171.757850200856));
#160457=CARTESIAN_POINT('Ctrl Pts',(31.319676718292,-64.2032893725833,-171.749791815626));
#160458=CARTESIAN_POINT('Ctrl Pts',(31.3208311719887,-64.1863066938707,
-171.742098872734));
#160459=CARTESIAN_POINT('Ctrl Pts',(31.3214083988371,-64.1778153545143,
-171.738252401289));
#160460=CARTESIAN_POINT('Ctrl Pts',(31.321993076794,-64.1692186758832,-171.734497284808));
#160461=CARTESIAN_POINT('Ctrl Pts',(31.3225854050853,-64.1605180755428,
-171.730839196989));
#160462=CARTESIAN_POINT('Ctrl Pts',(31.322881569231,-64.1561677753726,-171.729010153079));
#160463=CARTESIAN_POINT('Ctrl Pts',(31.3231796460049,-64.1517914950928,
-171.727205365633));
#160464=CARTESIAN_POINT('Ctrl Pts',(31.3234796624372,-64.1473894270328,
-171.725425545576));
#160465=CARTESIAN_POINT('Ctrl Pts',(31.3236618137701,-64.1447167648781,
-171.724344949446));
#160466=CARTESIAN_POINT('Ctrl Pts',(31.3238943343951,-64.141314308081,-171.72298693083));
#160467=CARTESIAN_POINT('Ctrl Pts',(31.3240866295113,-64.1384929063,-171.721876575885));
#160468=CARTESIAN_POINT('Ctrl Pts',(31.324211058373,-64.1366672550884,-171.72115809585));
#160469=CARTESIAN_POINT('Ctrl Pts',(31.3243187213849,-64.1350854387713,
-171.720541970086));
#160470=CARTESIAN_POINT('Ctrl Pts',(31.3243855589116,-64.1341060601822,
-171.720161698938));
#160471=CARTESIAN_POINT('Ctrl Pts',(31.3254476052599,-64.1185437629861,
-171.714119201495));
#160472=CARTESIAN_POINT('Ctrl Pts',(31.3266376535648,-64.1013293404877,
-171.707866938349));
#160473=CARTESIAN_POINT('Ctrl Pts',(31.3279469264486,-64.0824003384,-171.701654178638));
#160474=CARTESIAN_POINT('Ctrl Pts',(31.3292273680979,-64.0638881680553,
-171.695578228857));
#160475=CARTESIAN_POINT('Ctrl Pts',(31.3306217347893,-64.0437353416621,
-171.689540171929));
#160476=CARTESIAN_POINT('Ctrl Pts',(31.332124061834,-64.0218994182539,-171.68382031885));
#160477=CARTESIAN_POINT('Ctrl Pts',(31.3335678730231,-64.0009140072203,
-171.678323254875));
#160478=CARTESIAN_POINT('Ctrl Pts',(31.3351113079963,-63.9783734175572,
-171.673120412634));
#160479=CARTESIAN_POINT('Ctrl Pts',(31.3367525763832,-63.9542649101158,
-171.668501297287));
#160480=CARTESIAN_POINT('Ctrl Pts',(31.3383524464309,-63.9307645007625,
-171.66399869165));
#160481=CARTESIAN_POINT('Ctrl Pts',(31.3400451860075,-63.9057736267565,
-171.660051059673));
#160482=CARTESIAN_POINT('Ctrl Pts',(31.3418338549193,-63.8793140597499,
-171.656961460455));
#160483=CARTESIAN_POINT('Ctrl Pts',(31.343555301263,-63.8538489082178,-171.65398797596));
#160484=CARTESIAN_POINT('Ctrl Pts',(31.3453655360519,-63.8270229147674,
-171.651809705469));
#160485=CARTESIAN_POINT('Ctrl Pts',(31.3472728234533,-63.7988948820044,
-171.650723766091));
#160486=CARTESIAN_POINT('Ctrl Pts',(31.3481603393926,-63.7858060955955,
-171.65021844712));
#160487=CARTESIAN_POINT('Ctrl Pts',(31.349068956197,-63.7724359890296,-171.64995));
#160488=CARTESIAN_POINT('Ctrl Pts',(31.35,-63.7587939982373,-171.64995));
#160489=CARTESIAN_POINT('Ctrl Pts',(31.85,-65.2735353570153,-176.84995));
#160490=CARTESIAN_POINT('Ctrl Pts',(31.8499999999999,-64.6983511534047,
-176.84995));
#160491=CARTESIAN_POINT('Ctrl Pts',(31.28041344952,-64.7784013226445,-176.84995));
#160492=CARTESIAN_POINT('Ctrl Pts',(31.85,-65.2735353570043,-176.981217345763));
#160493=CARTESIAN_POINT('Ctrl Pts',(31.8499999999783,-64.6983511534012,
-176.958917254529));
#160494=CARTESIAN_POINT('Ctrl Pts',(31.2804134495858,-64.7784013226352,
-177.112484691526));
#160495=CARTESIAN_POINT('Ctrl Pts',(31.9038865634697,-65.2583888317962,
-177.110943344657));
#160496=CARTESIAN_POINT('Ctrl Pts',(31.883334205664,-64.6936663363131,-177.069891898462));
#160497=CARTESIAN_POINT('Ctrl Pts',(31.3881865764622,-64.7632547974255,
-177.371936689315));
#160498=CARTESIAN_POINT('Ctrl Pts',(32.0890066553437,-65.2063549673329,
-177.296063436531));
#160499=CARTESIAN_POINT('Ctrl Pts',(32.0302774403978,-64.6730148114567,
-177.257255781815));
#160500=CARTESIAN_POINT('Ctrl Pts',(31.7584267602047,-64.711220932962,-177.742176873059));
#160501=CARTESIAN_POINT('Ctrl Pts',(32.2187326542366,-65.1698913669989,
-177.34995));
#160502=CARTESIAN_POINT('Ctrl Pts',(32.1431106784802,-64.6571571339907,
-177.331204220089));
#160503=CARTESIAN_POINT('Ctrl Pts',(32.0178787579952,-64.6747573326273,
-177.849949999941));
#160504=CARTESIAN_POINT('Ctrl Pts',(32.35,-65.1329945223129,-177.34995));
#160505=CARTESIAN_POINT('Ctrl Pts',(32.28041344952,-64.637860487942,-177.34995));
#160506=CARTESIAN_POINT('Ctrl Pts',(32.28041344952,-64.6378604879421,-177.84995));
#160507=CARTESIAN_POINT('',(32.28041344952,-64.6378604879421,-177.84995));
#160508=CARTESIAN_POINT('Origin',(32.35,-65.1329945223129,-177.84995));
#160509=CARTESIAN_POINT('',(31.85,-65.2735353570153,-176.84995));
#160510=CARTESIAN_POINT('Ctrl Pts',(31.85,-65.2735353570153,-176.84995));
#160511=CARTESIAN_POINT('Ctrl Pts',(31.85,-65.2735353570131,-176.875860144879));
#160512=CARTESIAN_POINT('Ctrl Pts',(31.85210178423,-65.272936510976,-176.90206911043));
#160513=CARTESIAN_POINT('Ctrl Pts',(31.8563470810216,-65.2717334581292,
-176.928255280411));
#160514=CARTESIAN_POINT('Ctrl Pts',(31.8606310064401,-65.2705194585142,
-176.954679722494));
#160515=CARTESIAN_POINT('Ctrl Pts',(31.8670976465416,-65.2686902017598,
-176.981080902282));
#160516=CARTESIAN_POINT('Ctrl Pts',(31.8757612620159,-65.2662482275523,
-177.007084282781));
#160517=CARTESIAN_POINT('Ctrl Pts',(31.8790093277216,-65.2653327099256,
-177.016833179033));
#160518=CARTESIAN_POINT('Ctrl Pts',(31.8825659056061,-65.2643311515803,
-177.026525725721));
#160519=CARTESIAN_POINT('Ctrl Pts',(31.8864307190677,-65.2632439750754,
-177.036140639745));
#160520=CARTESIAN_POINT('Ctrl Pts',(31.8965777998919,-65.2603895894823,
-177.061384629059));
#160521=CARTESIAN_POINT('Ctrl Pts',(31.9088564664222,-65.2569417248404,
-177.086112146697));
#160522=CARTESIAN_POINT('Ctrl Pts',(31.9232664008841,-65.2528998905346,
-177.109925913984));
#160523=CARTESIAN_POINT('Ctrl Pts',(31.9261741041008,-65.2520843105163,
-177.114731166078));
#160524=CARTESIAN_POINT('Ctrl Pts',(31.9291685418052,-65.2512445582216,
-177.11949905002));
#160525=CARTESIAN_POINT('Ctrl Pts',(31.9322496425496,-65.2503806488339,
-177.124226050868));
#160526=CARTESIAN_POINT('Ctrl Pts',(31.9414248200636,-65.2478080221507,
-177.138302536998));
#160527=CARTESIAN_POINT('Ctrl Pts',(31.9513686606954,-65.2450209957176,
-177.15201654548));
#160528=CARTESIAN_POINT('Ctrl Pts',(31.9620727243129,-65.2420195372944,
-177.165265493157));
#160529=CARTESIAN_POINT('Ctrl Pts',(31.9674247561217,-65.2405188080827,
-177.171889966996));
#160530=CARTESIAN_POINT('Ctrl Pts',(31.9729667901391,-65.2389644717009,
-177.178398084194));
#160531=CARTESIAN_POINT('Ctrl Pts',(31.9786966345161,-65.2373565305258,
-177.184775824989));
#160532=CARTESIAN_POINT('Ctrl Pts',(31.9815615567046,-65.2365525599382,
-177.187964695387));
#160533=CARTESIAN_POINT('Ctrl Pts',(31.9844734220996,-65.2357351882425,
-177.19112096562));
#160534=CARTESIAN_POINT('Ctrl Pts',(31.9874318783457,-65.2349044161532,
-177.194242832635));
#160535=CARTESIAN_POINT('Ctrl Pts',(31.9891481151571,-65.2344224750587,
-177.196053866042));
#160536=CARTESIAN_POINT('Ctrl Pts',(31.9912379161451,-65.2338354383028,
-177.198223860057));
#160537=CARTESIAN_POINT('Ctrl Pts',(31.9930815352964,-65.2333174589098,
-177.200104597085));
#160538=CARTESIAN_POINT('Ctrl Pts',(31.9944159546055,-65.2329425432427,
-177.201465882471));
#160539=CARTESIAN_POINT('Ctrl Pts',(31.9956200660744,-65.2326041814675,
-177.202676847247));
#160540=CARTESIAN_POINT('Ctrl Pts',(31.9964466064336,-65.2323718572572,
-177.20350338762));
#160541=CARTESIAN_POINT('Ctrl Pts',(32.0062413953876,-65.2296187350626,
-177.213298176739));
#160542=CARTESIAN_POINT('Ctrl Pts',(32.0171766858621,-65.2264997668672,
-177.223386446864));
#160543=CARTESIAN_POINT('Ctrl Pts',(32.0293814740844,-65.2230056156829,
-177.233531412475));
#160544=CARTESIAN_POINT('Ctrl Pts',(32.0410442961724,-65.2196666258643,
-177.243225880487));
#160545=CARTESIAN_POINT('Ctrl Pts',(32.0538670706311,-65.2159848445911,
-177.25297216405));
#160546=CARTESIAN_POINT('Ctrl Pts',(32.0679403417523,-65.2119582399725,
-177.262523160562));
#160547=CARTESIAN_POINT('Ctrl Pts',(32.0811785164908,-65.2081705707742,
-177.271507408763));
#160548=CARTESIAN_POINT('Ctrl Pts',(32.0955236210271,-65.2040776753833,
-177.280318781026));
#160549=CARTESIAN_POINT('Ctrl Pts',(32.111023322083,-65.1996854519068,-177.288715370369));
#160550=CARTESIAN_POINT('Ctrl Pts',(32.1172493121663,-65.1979211636983,
-177.292088150386));
#160551=CARTESIAN_POINT('Ctrl Pts',(32.1236612363228,-65.1961086768998,
-177.29539358477));
#160552=CARTESIAN_POINT('Ctrl Pts',(32.1302605707122,-65.1942488102442,
-177.298614236713));
#160553=CARTESIAN_POINT('Ctrl Pts',(32.1454165064926,-65.1899774674195,
-177.30601073932));
#160554=CARTESIAN_POINT('Ctrl Pts',(32.1615733881405,-65.185464996466,-177.312967023304));
#160555=CARTESIAN_POINT('Ctrl Pts',(32.1787235893757,-65.1806932862225,
-177.31924572228));
#160556=CARTESIAN_POINT('Ctrl Pts',(32.195408897906,-65.1760509233407,-177.325354223758));
#160557=CARTESIAN_POINT('Ctrl Pts',(32.2130347093888,-65.1711630872873,
-177.330821391552));
#160558=CARTESIAN_POINT('Ctrl Pts',(32.2315578626383,-65.166023463016,-177.335399595608));
#160559=CARTESIAN_POINT('Ctrl Pts',(32.2496915443714,-65.1609919055103,
-177.339881537432));
#160560=CARTESIAN_POINT('Ctrl Pts',(32.2686855091775,-65.1557189448577,
-177.343511544964));
#160561=CARTESIAN_POINT('Ctrl Pts',(32.2884598244632,-65.1502101232398,
-177.346028622917));
#160562=CARTESIAN_POINT('Ctrl Pts',(32.3082341397488,-65.1447013016219,
-177.34854570087));
#160563=CARTESIAN_POINT('Ctrl Pts',(32.3287891950344,-65.1389564907821,
-177.34995));
#160564=CARTESIAN_POINT('Ctrl Pts',(32.35,-65.1329945223129,-177.34995));
#160565=CARTESIAN_POINT('',(31.28041344952,-64.7784013226445,-176.84995));
#160566=CARTESIAN_POINT('Origin',(31.35,-65.2735353570153,-176.84995));
#160567=CARTESIAN_POINT('Ctrl Pts',(32.28041344952,-64.6378604879421,-177.84995));
#160568=CARTESIAN_POINT('Ctrl Pts',(32.0178787579952,-64.6747573326273,
-177.849949999941));
#160569=CARTESIAN_POINT('Ctrl Pts',(31.7584267602047,-64.711220932962,-177.742176873059));
#160570=CARTESIAN_POINT('Ctrl Pts',(31.5733066683334,-64.7372378651937,
-177.557056781187));
#160571=CARTESIAN_POINT('Ctrl Pts',(31.3881865764622,-64.7632547974255,
-177.371936689315));
#160572=CARTESIAN_POINT('Ctrl Pts',(31.2804134495858,-64.7784013226352,
-177.112484691526));
#160573=CARTESIAN_POINT('Ctrl Pts',(31.28041344952,-64.7784013226445,-176.84995));
#160574=CARTESIAN_POINT('Origin',(45.6308101826775,-63.2664983737155,-177.84995));
#160575=CARTESIAN_POINT('',(32.7804134495199,-64.5675900705909,-177.84995));
#160576=CARTESIAN_POINT('',(45.5612236321975,-62.7713643393447,-177.84995));
#160577=CARTESIAN_POINT('Origin',(32.85,-65.0627241049617,-177.84995));
#160578=CARTESIAN_POINT('Ctrl Pts',(32.85,-65.0627241049617,-177.34995));
#160579=CARTESIAN_POINT('Ctrl Pts',(32.7804134495199,-64.5675900705908,
-177.34995));
#160580=CARTESIAN_POINT('Ctrl Pts',(32.7804134495199,-64.5675900705909,
-177.84995));
#160581=CARTESIAN_POINT('Ctrl Pts',(32.9812673457631,-65.0258272602758,
-177.34995));
#160582=CARTESIAN_POINT('Ctrl Pts',(32.9116024612643,-64.5491526573769,
-177.367861075732));
#160583=CARTESIAN_POINT('Ctrl Pts',(33.0429481410447,-64.5306932259057,
-177.849949999941));
#160584=CARTESIAN_POINT('Ctrl Pts',(33.1109933446567,-64.9893636599417,
-177.29606343653));
#160585=CARTESIAN_POINT('Ctrl Pts',(33.0606847809584,-64.52820050373,-177.329589659683));
#160586=CARTESIAN_POINT('Ctrl Pts',(33.3024001388352,-64.494229625571,-177.742176873059));
#160587=CARTESIAN_POINT('Ctrl Pts',(33.2961134365298,-64.9373297954784,
-177.110943344657));
#160588=CARTESIAN_POINT('Ctrl Pts',(33.280492098389,-64.4973085998594,-177.142957948483));
#160589=CARTESIAN_POINT('Ctrl Pts',(33.6726403225778,-64.4421957611075,
-177.371936689315));
#160590=CARTESIAN_POINT('Ctrl Pts',(33.35,-64.9221832702703,-176.981217345763));
#160591=CARTESIAN_POINT('Ctrl Pts',(33.3499999999424,-64.4875399013621,
-176.997671841189));
#160592=CARTESIAN_POINT('Ctrl Pts',(33.7804134494542,-64.4270492358978,
-177.112484691526));
#160593=CARTESIAN_POINT('Ctrl Pts',(33.35,-64.9221832702593,-176.84995));
#160594=CARTESIAN_POINT('Ctrl Pts',(33.35,-64.4875399013512,-176.84995));
#160595=CARTESIAN_POINT('Ctrl Pts',(33.7804134495199,-64.4270492358885,
-176.84995));
#160596=CARTESIAN_POINT('',(33.7804134495199,-64.4270492358885,-176.84995));
#160597=CARTESIAN_POINT('Ctrl Pts',(33.7804134495199,-64.4270492358885,
-176.84995));
#160598=CARTESIAN_POINT('Ctrl Pts',(33.7804134494542,-64.4270492358978,
-177.112484691526));
#160599=CARTESIAN_POINT('Ctrl Pts',(33.6726403225778,-64.4421957611075,
-177.371936689315));
#160600=CARTESIAN_POINT('Ctrl Pts',(33.4875202307065,-64.4682126933392,
-177.557056781187));
#160601=CARTESIAN_POINT('Ctrl Pts',(33.3024001388352,-64.494229625571,-177.742176873059));
#160602=CARTESIAN_POINT('Ctrl Pts',(33.0429481410447,-64.5306932259057,
-177.849949999941));
#160603=CARTESIAN_POINT('Ctrl Pts',(32.7804134495199,-64.5675900705909,
-177.84995));
#160604=CARTESIAN_POINT('',(33.35,-64.9221832702593,-176.84995));
#160605=CARTESIAN_POINT('Origin',(33.85,-64.9221832702593,-176.84995));
#160606=CARTESIAN_POINT('Ctrl Pts',(32.85,-65.0627241049617,-177.34995));
#160607=CARTESIAN_POINT('Ctrl Pts',(32.8709105170141,-65.0568465419312,
-177.34995));
#160608=CARTESIAN_POINT('Ctrl Pts',(32.8911797466383,-65.0511492330308,
-177.348585219097));
#160609=CARTESIAN_POINT('Ctrl Pts',(32.9106899838339,-65.0456652629893,
-177.346136042571));
#160610=CARTESIAN_POINT('Ctrl Pts',(32.9306295626821,-65.0400606128794,
-177.343632969545));
#160611=CARTESIAN_POINT('Ctrl Pts',(32.9497766651579,-65.0346787133512,
-177.33999719389));
#160612=CARTESIAN_POINT('Ctrl Pts',(32.9680516974346,-65.0295419367704,
-177.335495637057));
#160613=CARTESIAN_POINT('Ctrl Pts',(32.9869112963546,-65.0242408492217,
-177.330850088141));
#160614=CARTESIAN_POINT('Ctrl Pts',(33.004842416708,-65.0192007399784,-177.32528246904));
#160615=CARTESIAN_POINT('Ctrl Pts',(33.0218018468558,-65.0144337550403,
-177.319052501424));
#160616=CARTESIAN_POINT('Ctrl Pts',(33.0374915731195,-65.0100236605896,
-177.313288953611));
#160617=CARTESIAN_POINT('Ctrl Pts',(33.0523504278524,-65.0058471088959,
-177.306958054963));
#160618=CARTESIAN_POINT('Ctrl Pts',(33.0663727601658,-65.0019056883203,
-177.300241547042));
#160619=CARTESIAN_POINT('Ctrl Pts',(33.0846217845958,-64.9967762220685,
-177.291500510645));
#160620=CARTESIAN_POINT('Ctrl Pts',(33.1014605911939,-64.9920431421992,
-177.282104513304));
#160621=CARTESIAN_POINT('Ctrl Pts',(33.1169358413832,-64.9876933330415,
-177.272394746015));
#160622=CARTESIAN_POINT('Ctrl Pts',(33.1322211818847,-64.983396904016,-177.26280413537));
#160623=CARTESIAN_POINT('Ctrl Pts',(33.1461768441267,-64.9794742231754,
-177.252906955711));
#160624=CARTESIAN_POINT('Ctrl Pts',(33.1588862630228,-64.9759018384949,
-177.242983686098));
#160625=CARTESIAN_POINT('Ctrl Pts',(33.1717549881601,-64.9722846757503,
-177.232936033239));
#160626=CARTESIAN_POINT('Ctrl Pts',(33.1833462719647,-64.9690265783479,
-177.222861820351));
#160627=CARTESIAN_POINT('Ctrl Pts',(33.1937756504663,-64.9660950712279,
-177.21300750887));
#160628=CARTESIAN_POINT('Ctrl Pts',(33.1950359580597,-64.9657408218656,
-177.211816693561));
#160629=CARTESIAN_POINT('Ctrl Pts',(33.1962793259514,-64.9653913339429,
-177.210629037074));
#160630=CARTESIAN_POINT('Ctrl Pts',(33.1975059843104,-64.9650465427636,
-177.209444926089));
#160631=CARTESIAN_POINT('Ctrl Pts',(33.1987673970184,-64.9646919827738,
-177.20822726623));
#160632=CARTESIAN_POINT('Ctrl Pts',(33.1996021366106,-64.9644573527714,
-177.207413007319));
#160633=CARTESIAN_POINT('Ctrl Pts',(33.2007626710069,-64.9641311320666,
-177.206271333214));
#160634=CARTESIAN_POINT('Ctrl Pts',(33.2014998739257,-64.9639239078288,
-177.205546110864));
#160635=CARTESIAN_POINT('Ctrl Pts',(33.2023682910512,-64.9636797953249,
-177.204688490104));
#160636=CARTESIAN_POINT('Ctrl Pts',(33.2035533858467,-64.9633466601626,
-177.20350339534));
#160637=CARTESIAN_POINT('Ctrl Pts',(33.224102627464,-64.9575701813806,-177.182954154274));
#160638=CARTESIAN_POINT('Ctrl Pts',(33.2425303081954,-64.9523902391111,
-177.160790380395));
#160639=CARTESIAN_POINT('Ctrl Pts',(33.258793554525,-64.9478188139827,-177.137499857771));
#160640=CARTESIAN_POINT('Ctrl Pts',(33.2750773096424,-64.9432416240528,
-177.114179964603));
#160641=CARTESIAN_POINT('Ctrl Pts',(33.2891911870376,-64.9392744816987,
-177.089730493789));
#160642=CARTESIAN_POINT('Ctrl Pts',(33.3011153275693,-64.9359229034905,
-177.06459461214));
#160643=CARTESIAN_POINT('Ctrl Pts',(33.3130600466424,-64.9325655411681,
-177.039415351282));
#160644=CARTESIAN_POINT('Ctrl Pts',(33.3228074903105,-64.9298258622901,
-177.013547308706));
#160645=CARTESIAN_POINT('Ctrl Pts',(33.3303606028096,-64.9277029771689,
-176.987389234916));
#160646=CARTESIAN_POINT('Ctrl Pts',(33.3379480469477,-64.9255704427639,
-176.961112263183));
#160647=CARTESIAN_POINT('Ctrl Pts',(33.3433211912071,-64.9240603151624,
-176.934542621745));
#160648=CARTESIAN_POINT('Ctrl Pts',(33.3465057497558,-64.9231653054218,
-176.908037356488));
#160649=CARTESIAN_POINT('Ctrl Pts',(33.3488411540378,-64.9225089477042,
-176.888599651378));
#160650=CARTESIAN_POINT('Ctrl Pts',(33.35,-64.9221832702593,-176.869195583396));
#160651=CARTESIAN_POINT('Ctrl Pts',(33.35,-64.9221832702593,-176.84995));
#160652=CARTESIAN_POINT('Origin',(45.4220505312374,-61.7810962706031,-172.64995));
#160653=CARTESIAN_POINT('',(39.43041344952,-63.6329935198201,-172.64995));
#160654=CARTESIAN_POINT('',(33.7804134495199,-64.4270492358885,-172.64995));
#160655=CARTESIAN_POINT('',(33.35,-64.4875399013512,-172.64995));
#160656=CARTESIAN_POINT('Ctrl Pts',(39.4304134495199,-63.6329935198201,
-172.64995));
#160657=CARTESIAN_POINT('Ctrl Pts',(39.4304134495199,-63.6329935198201,
-172.608983203963));
#160658=CARTESIAN_POINT('Ctrl Pts',(39.4306213080459,-63.6304189382149,
-172.567620053442));
#160659=CARTESIAN_POINT('Ctrl Pts',(39.431019438328,-63.6251446386348,-172.526187282055));
#160660=CARTESIAN_POINT('Ctrl Pts',(39.4314123572806,-63.6199393770401,
-172.485296845251));
#160661=CARTESIAN_POINT('Ctrl Pts',(39.4319905477632,-63.6121042430135,
-172.444338940925));
#160662=CARTESIAN_POINT('Ctrl Pts',(39.4327427524647,-63.6015591366258,
-172.403658150787));
#160663=CARTESIAN_POINT('Ctrl Pts',(39.4334809680696,-63.5912101424279,
-172.36373392));
#160664=CARTESIAN_POINT('Ctrl Pts',(39.4343867483315,-63.578250770363,-172.324077003577));
#160665=CARTESIAN_POINT('Ctrl Pts',(39.435455573753,-63.5626488625364,-172.285037096605));
#160666=CARTESIAN_POINT('Ctrl Pts',(39.4365128314928,-63.5472158110073,
-172.246419710661));
#160667=CARTESIAN_POINT('Ctrl Pts',(39.4377295873855,-63.5291968509287,
-172.208406476233));
#160668=CARTESIAN_POINT('Ctrl Pts',(39.439108072927,-63.5086078602195,-172.171353410548));
#160669=CARTESIAN_POINT('Ctrl Pts',(39.4404653773755,-63.4883352292506,
-172.13486968303));
#160670=CARTESIAN_POINT('Ctrl Pts',(39.4419794574579,-63.465570783196,-172.09931731054));
#160671=CARTESIAN_POINT('Ctrl Pts',(39.4436593097151,-63.4403785357705,
-172.065046653512));
#160672=CARTESIAN_POINT('Ctrl Pts',(39.4444218099166,-63.4289435457853,
-172.049490890928));
#160673=CARTESIAN_POINT('Ctrl Pts',(39.445218561239,-63.4170090341692,-172.034199306794));
#160674=CARTESIAN_POINT('Ctrl Pts',(39.4460508994101,-63.404584505118,-172.019204985054));
#160675=CARTESIAN_POINT('Ctrl Pts',(39.4467847052916,-63.3936307932609,
-172.005985692865));
#160676=CARTESIAN_POINT('Ctrl Pts',(39.4475461754571,-63.3822962440122,
-171.992997455584));
#160677=CARTESIAN_POINT('Ctrl Pts',(39.4483364318027,-63.3705888400765,
-171.980262947432));
#160678=CARTESIAN_POINT('Ctrl Pts',(39.4486919487457,-63.3653219662557,
-171.974534004621));
#160679=CARTESIAN_POINT('Ctrl Pts',(39.4490750220687,-63.3596977694689,
-171.968556625832));
#160680=CARTESIAN_POINT('Ctrl Pts',(39.4494555591141,-63.3540912163381,
-171.962743472495));
#160681=CARTESIAN_POINT('Ctrl Pts',(39.4498484999446,-63.348301914955,-171.956740836674));
#160682=CARTESIAN_POINT('Ctrl Pts',(39.4502387617329,-63.3425316060038,
-171.950913444705));
#160683=CARTESIAN_POINT('Ctrl Pts',(39.4505989639742,-63.3372340568394,
-171.945675868377));
#160684=CARTESIAN_POINT('Ctrl Pts',(39.4506653264156,-63.3362580543183,
-171.944710915048));
#160685=CARTESIAN_POINT('Ctrl Pts',(39.4507306824667,-63.3352981978247,
-171.943765878353));
#160686=CARTESIAN_POINT('Ctrl Pts',(39.4507948782762,-63.3343574486486,
-171.942843218813));
#160687=CARTESIAN_POINT('Ctrl Pts',(39.4523230364769,-63.3119632521963,
-171.920879639657));
#160688=CARTESIAN_POINT('Ctrl Pts',(39.4539802191624,-63.2878579553574,
-171.899286274498));
#160689=CARTESIAN_POINT('Ctrl Pts',(39.4557568293543,-63.2619732720811,
-171.878357890799));
#160690=CARTESIAN_POINT('Ctrl Pts',(39.4574846179602,-63.2367999048249,
-171.858004623066));
#160691=CARTESIAN_POINT('Ctrl Pts',(39.4593252995171,-63.2099431694035,
-171.838280618575));
#160692=CARTESIAN_POINT('Ctrl Pts',(39.4612753249272,-63.1813778126731,
-171.819487496696));
#160693=CARTESIAN_POINT('Ctrl Pts',(39.4632253503372,-63.1528124559428,
-171.800694374818));
#160694=CARTESIAN_POINT('Ctrl Pts',(39.4652846337216,-63.1225378668433,
-171.782832445536));
#160695=CARTESIAN_POINT('Ctrl Pts',(39.4674561053568,-63.0905748953762,
-171.766229742224));
#160696=CARTESIAN_POINT('Ctrl Pts',(39.4685520676076,-63.0744428816831,
-171.757850200996));
#160697=CARTESIAN_POINT('Ctrl Pts',(39.4696767182751,-63.05788157,-171.749791815739));
#160698=CARTESIAN_POINT('Ctrl Pts',(39.4708311719758,-63.0408988912349,
-171.74209887282));
#160699=CARTESIAN_POINT('Ctrl Pts',(39.4714083988261,-63.0324075518524,
-171.73825240136));
#160700=CARTESIAN_POINT('Ctrl Pts',(39.4719930767851,-63.0238108731925,
-171.734497284865));
#160701=CARTESIAN_POINT('Ctrl Pts',(39.4725854050786,-63.0151102728207,
-171.730839197032));
#160702=CARTESIAN_POINT('Ctrl Pts',(39.4728815692253,-63.0107599726348,
-171.729010153115));
#160703=CARTESIAN_POINT('Ctrl Pts',(39.4731796460004,-63.0063836923387,
-171.727205365662));
#160704=CARTESIAN_POINT('Ctrl Pts',(39.4734796624338,-63.0019816242616,
-171.725425545597));
#160705=CARTESIAN_POINT('Ctrl Pts',(39.4736618137668,-62.999308962104,-171.724344949466));
#160706=CARTESIAN_POINT('Ctrl Pts',(39.4738943343923,-62.9959065053002,
-171.722986930847));
#160707=CARTESIAN_POINT('Ctrl Pts',(39.474086629509,-62.9930851035116,-171.721876575899));
#160708=CARTESIAN_POINT('Ctrl Pts',(39.4742110583718,-62.991259452282,-171.721158095857));
#160709=CARTESIAN_POINT('Ctrl Pts',(39.4743187213847,-62.98967763595,-171.720541970087));
#160710=CARTESIAN_POINT('Ctrl Pts',(39.4743855589116,-62.9886982573578,
-171.720161698938));
#160711=CARTESIAN_POINT('Ctrl Pts',(39.4754476052573,-62.9731359601951,
-171.714119201508));
#160712=CARTESIAN_POINT('Ctrl Pts',(39.4766376535597,-62.9559215377298,
-171.707866938373));
#160713=CARTESIAN_POINT('Ctrl Pts',(39.4779469264412,-62.9369925356752,
-171.70165417867));
#160714=CARTESIAN_POINT('Ctrl Pts',(39.4792273680883,-62.9184803653616,
-171.695578228898));
#160715=CARTESIAN_POINT('Ctrl Pts',(39.4806217347776,-62.8983275389991,
-171.689540171976));
#160716=CARTESIAN_POINT('Ctrl Pts',(39.4821240618203,-62.8764916156212,
-171.6838203189));
#160717=CARTESIAN_POINT('Ctrl Pts',(39.4835678730075,-62.8555062046158,
-171.678323254929));
#160718=CARTESIAN_POINT('Ctrl Pts',(39.485111307979,-62.8329656149803,-171.673120412688));
#160719=CARTESIAN_POINT('Ctrl Pts',(39.4867525763642,-62.8088571075656,
-171.66850129734));
#160720=CARTESIAN_POINT('Ctrl Pts',(39.4883524464103,-62.7853566982382,
-171.663998691701));
#160721=CARTESIAN_POINT('Ctrl Pts',(39.4900451859854,-62.7603658242571,
-171.66005105972));
#160722=CARTESIAN_POINT('Ctrl Pts',(39.4918338548956,-62.7339062572745,
-171.656961460496));
#160723=CARTESIAN_POINT('Ctrl Pts',(39.4935553012377,-62.7084411057663,
-171.653987975995));
#160724=CARTESIAN_POINT('Ctrl Pts',(39.4953655360251,-62.6816151123391,
-171.651809705496));
#160725=CARTESIAN_POINT('Ctrl Pts',(39.497272823425,-62.653487079598,-171.650723766108));
#160726=CARTESIAN_POINT('Ctrl Pts',(39.4981603393732,-62.6403982930561,
-171.650218447126));
#160727=CARTESIAN_POINT('Ctrl Pts',(39.499068956187,-62.6270281863508,-171.64995));
#160728=CARTESIAN_POINT('Ctrl Pts',(39.5,-62.6133861954129,-171.64995));
#160729=CARTESIAN_POINT('Ctrl Pts',(33.85,-63.4074419114814,-171.64995));
#160730=CARTESIAN_POINT('Ctrl Pts',(33.8480582289195,-63.4358934441742,
-171.64995));
#160731=CARTESIAN_POINT('Ctrl Pts',(33.8461974246871,-63.4631586213041,
-171.651129585063));
#160732=CARTESIAN_POINT('Ctrl Pts',(33.8444225652799,-63.4891645037474,
-171.653192621539));
#160733=CARTESIAN_POINT('Ctrl Pts',(33.8425545166564,-63.5165358283173,
-171.655363978005));
#160734=CARTESIAN_POINT('Ctrl Pts',(33.8407816512719,-63.5425124936179,
-171.658513818808));
#160735=CARTESIAN_POINT('Ctrl Pts',(33.8391066446573,-63.5670552968023,
-171.66233503357));
#160736=CARTESIAN_POINT('Ctrl Pts',(33.837607521914,-63.589020985843,-171.665755002128));
#160737=CARTESIAN_POINT('Ctrl Pts',(33.8361867195622,-63.6098390961603,
-171.669713339737));
#160738=CARTESIAN_POINT('Ctrl Pts',(33.8348444729116,-63.6295061799083,
-171.674015027606));
#160739=CARTESIAN_POINT('Ctrl Pts',(33.8332381237839,-63.6530429887437,
-171.679163122074));
#160740=CARTESIAN_POINT('Ctrl Pts',(33.8317442597807,-63.6749316248201,
-171.6848021004));
#160741=CARTESIAN_POINT('Ctrl Pts',(33.8303611921804,-63.6951968318997,
-171.690639736311));
#160742=CARTESIAN_POINT('Ctrl Pts',(33.8289186268559,-63.7163338211679,
-171.696728499535));
#160743=CARTESIAN_POINT('Ctrl Pts',(33.8275965325062,-63.7357056261111,
-171.703033282501));
#160744=CARTESIAN_POINT('Ctrl Pts',(33.8263912815561,-63.753365399271,-171.709272496442));
#160745=CARTESIAN_POINT('Ctrl Pts',(33.825874494011,-63.7609375574312,-171.711947746816));
#160746=CARTESIAN_POINT('Ctrl Pts',(33.825379175863,-63.7681951382168,-171.714611542066));
#160747=CARTESIAN_POINT('Ctrl Pts',(33.8249049735087,-63.7751433227486,
-171.717244495107));
#160748=CARTESIAN_POINT('Ctrl Pts',(33.8247845954601,-63.7769071454876,
-171.717912880126));
#160749=CARTESIAN_POINT('Ctrl Pts',(33.8247281084716,-63.7777337764561,
-171.718228248952));
#160750=CARTESIAN_POINT('Ctrl Pts',(33.8246071368902,-63.7795056823664,
-171.71890895899));
#160751=CARTESIAN_POINT('Ctrl Pts',(33.8245512101083,-63.780324858194,-171.719223660355));
#160752=CARTESIAN_POINT('Ctrl Pts',(33.8244815093962,-63.7813459451167,
-171.71961677203));
#160753=CARTESIAN_POINT('Ctrl Pts',(33.8243854515167,-63.7827534613978,
-171.720163005656));
#160754=CARTESIAN_POINT('Ctrl Pts',(33.8240448575363,-63.7877441146917,
-171.72209979508));
#160755=CARTESIAN_POINT('Ctrl Pts',(33.8237064547845,-63.7927026508811,
-171.724069245188));
#160756=CARTESIAN_POINT('Ctrl Pts',(33.8233702655348,-63.7976287443672,
-171.72607046184));
#160757=CARTESIAN_POINT('Ctrl Pts',(33.8210922898814,-63.8310073281163,
-171.739630451674));
#160758=CARTESIAN_POINT('Ctrl Pts',(33.8189167622032,-63.8628843636977,
-171.754642782109));
#160759=CARTESIAN_POINT('Ctrl Pts',(33.816846962281,-63.8932120250278,-171.77077929301));
#160760=CARTESIAN_POINT('Ctrl Pts',(33.8148622623441,-63.9222927621974,
-171.786252350007));
#160761=CARTESIAN_POINT('Ctrl Pts',(33.8129747403056,-63.9499494177769,
-171.802759466717));
#160762=CARTESIAN_POINT('Ctrl Pts',(33.8111851663565,-63.9761709030137,
-171.820043746716));
#160763=CARTESIAN_POINT('Ctrl Pts',(33.8091798424695,-64.0055536344305,
-171.839411808912));
#160764=CARTESIAN_POINT('Ctrl Pts',(33.8072974703405,-64.0331348321881,
-171.859755775727));
#160765=CARTESIAN_POINT('Ctrl Pts',(33.8055364549802,-64.0589378666435,
-171.880757614385));
#160766=CARTESIAN_POINT('Ctrl Pts',(33.8047081977239,-64.0710737917499,
-171.890635396065));
#160767=CARTESIAN_POINT('Ctrl Pts',(33.803906752079,-64.0828168634207,-171.900659292116));
#160768=CARTESIAN_POINT('Ctrl Pts',(33.8031317849169,-64.0941719627785,
-171.910799109343));
#160769=CARTESIAN_POINT('Ctrl Pts',(33.8027566361001,-64.0996687790261,
-171.915707627562));
#160770=CARTESIAN_POINT('Ctrl Pts',(33.8024097468116,-64.1047515263583,
-171.920348851345));
#160771=CARTESIAN_POINT('Ctrl Pts',(33.8020599418533,-64.1098768430549,
-171.925124127276));
#160772=CARTESIAN_POINT('Ctrl Pts',(33.8017205761744,-64.1148492041924,
-171.929756893964));
#160773=CARTESIAN_POINT('Ctrl Pts',(33.8013784560457,-64.1198617813615,
-171.9345159123));
#160774=CARTESIAN_POINT('Ctrl Pts',(33.8010073810434,-64.1252983348553,
-171.939801580717));
#160775=CARTESIAN_POINT('Ctrl Pts',(33.800937583903,-64.1263209202765,-171.940795785495));
#160776=CARTESIAN_POINT('Ctrl Pts',(33.8008667695503,-64.127358400323,-171.941808724667));
#160777=CARTESIAN_POINT('Ctrl Pts',(33.8007947743349,-64.1284131719497,
-171.94284321151));
#160778=CARTESIAN_POINT('Ctrl Pts',(33.7984463931901,-64.1628183166118,
-171.976586695486));
#160779=CARTESIAN_POINT('Ctrl Pts',(33.7962900974017,-64.1944120724635,
-172.012463058108));
#160780=CARTESIAN_POINT('Ctrl Pts',(33.7943343814619,-64.2230682849126,
-172.049959758061));
#160781=CARTESIAN_POINT('Ctrl Pts',(33.7923469358344,-64.2521894179834,
-172.088064807393));
#160782=CARTESIAN_POINT('Ctrl Pts',(33.7905666289932,-64.278276951698,-172.127843232782));
#160783=CARTESIAN_POINT('Ctrl Pts',(33.789000571919,-64.3012249965493,-172.168804472182));
#160784=CARTESIAN_POINT('Ctrl Pts',(33.7877708916472,-64.3192439809744,
-172.200967557951));
#160785=CARTESIAN_POINT('Ctrl Pts',(33.7866732704194,-64.3353278524982,
-172.233860874847));
#160786=CARTESIAN_POINT('Ctrl Pts',(33.785710408276,-64.3494362499387,-172.267266567535));
#160787=CARTESIAN_POINT('Ctrl Pts',(33.7856150487614,-64.350833511157,-172.270574985735));
#160788=CARTESIAN_POINT('Ctrl Pts',(33.7855210125593,-64.3522113735592,
-172.27388835426));
#160789=CARTESIAN_POINT('Ctrl Pts',(33.7854282968075,-64.3535698783134,
-172.277206441635));
#160790=CARTESIAN_POINT('Ctrl Pts',(33.7842160400822,-64.371332302627,-172.320590372142));
#160791=CARTESIAN_POINT('Ctrl Pts',(33.7832297201077,-64.3857842198915,
-172.364775502606));
#160792=CARTESIAN_POINT('Ctrl Pts',(33.7824628528102,-64.3970206371015,
-172.409267414372));
#160793=CARTESIAN_POINT('Ctrl Pts',(33.7816869655113,-64.4083892186358,
-172.454282646281));
#160794=CARTESIAN_POINT('Ctrl Pts',(33.7811357225718,-64.4164662297078,
-172.499611949937));
#160795=CARTESIAN_POINT('Ctrl Pts',(33.7808018218098,-64.4213586645272,
-172.544796240172));
#160796=CARTESIAN_POINT('Ctrl Pts',(33.7805416776482,-64.4251703909416,
-172.579999601885));
#160797=CARTESIAN_POINT('Ctrl Pts',(33.7804134495199,-64.4270492358885,
-172.615116019715));
#160798=CARTESIAN_POINT('Ctrl Pts',(33.7804134495199,-64.4270492358885,
-172.64995));
#160799=CARTESIAN_POINT('Ctrl Pts',(40.,-64.1281275541908,-176.84995));
#160800=CARTESIAN_POINT('Ctrl Pts',(40.,-63.5529433505803,-176.84995));
#160801=CARTESIAN_POINT('Ctrl Pts',(39.43041344952,-63.63299351982,-176.84995));
#160802=CARTESIAN_POINT('Ctrl Pts',(40.,-64.1281275541799,-176.981217345763));
#160803=CARTESIAN_POINT('Ctrl Pts',(39.9999999999783,-63.5529433505767,
-176.958917254529));
#160804=CARTESIAN_POINT('Ctrl Pts',(39.4304134495858,-63.6329935198108,
-177.112484691526));
#160805=CARTESIAN_POINT('Ctrl Pts',(40.0538865634702,-64.1129810289718,
-177.110943344657));
#160806=CARTESIAN_POINT('Ctrl Pts',(40.033334205665,-63.5482585334886,-177.069891898461));
#160807=CARTESIAN_POINT('Ctrl Pts',(39.5381865764622,-63.6178469946011,
-177.371936689315));
#160808=CARTESIAN_POINT('Ctrl Pts',(40.2390066553433,-64.0609471645084,
-177.29606343653));
#160809=CARTESIAN_POINT('Ctrl Pts',(40.1802774403969,-63.5276070086322,
-177.257255781815));
#160810=CARTESIAN_POINT('Ctrl Pts',(39.9084267602046,-63.5658131301376,
-177.742176873059));
#160811=CARTESIAN_POINT('Ctrl Pts',(40.3687326542369,-64.0244835641743,
-177.34995));
#160812=CARTESIAN_POINT('Ctrl Pts',(40.2931106784809,-63.5117493311662,
-177.331204220089));
#160813=CARTESIAN_POINT('Ctrl Pts',(40.1678787579952,-63.5293495298029,
-177.849949999941));
#160814=CARTESIAN_POINT('Ctrl Pts',(40.5,-63.9875867194884,-177.34995));
#160815=CARTESIAN_POINT('Ctrl Pts',(40.4304134495199,-63.4924526851176,
-177.34995));
#160816=CARTESIAN_POINT('Ctrl Pts',(40.4304134495199,-63.4924526851176,
-177.84995));
#160817=CARTESIAN_POINT('',(40.,-64.1281275541909,-176.84995));
#160818=CARTESIAN_POINT('',(39.43041344952,-63.63299351982,-176.84995));
#160819=CARTESIAN_POINT('Origin',(39.5,-64.1281275541909,-176.84995));
#160820=CARTESIAN_POINT('',(40.4304134495199,-63.4924526851176,-177.84995));
#160821=CARTESIAN_POINT('Ctrl Pts',(40.4304134495199,-63.4924526851176,
-177.84995));
#160822=CARTESIAN_POINT('Ctrl Pts',(40.1678787579952,-63.5293495298029,
-177.849949999941));
#160823=CARTESIAN_POINT('Ctrl Pts',(39.9084267602046,-63.5658131301376,
-177.742176873059));
#160824=CARTESIAN_POINT('Ctrl Pts',(39.7233066683334,-63.5918300623693,
-177.557056781187));
#160825=CARTESIAN_POINT('Ctrl Pts',(39.5381865764622,-63.6178469946011,
-177.371936689315));
#160826=CARTESIAN_POINT('Ctrl Pts',(39.4304134495858,-63.6329935198108,
-177.112484691526));
#160827=CARTESIAN_POINT('Ctrl Pts',(39.43041344952,-63.63299351982,-176.84995));
#160828=CARTESIAN_POINT('Origin',(40.5,-63.9875867194884,-177.84995));
#160829=CARTESIAN_POINT('Ctrl Pts',(40.,-64.1281275541908,-176.84995));
#160830=CARTESIAN_POINT('Ctrl Pts',(40.,-64.1281275541887,-176.875860144686));
#160831=CARTESIAN_POINT('Ctrl Pts',(40.0021017841988,-64.1275287081581,
-176.902069110053));
#160832=CARTESIAN_POINT('Ctrl Pts',(40.0063470809329,-64.1263256553243,
-176.928255279864));
#160833=CARTESIAN_POINT('Ctrl Pts',(40.0106310062881,-64.125111655724,-176.954679721742));
#160834=CARTESIAN_POINT('Ctrl Pts',(40.017097646294,-64.1232823989925,-176.981080901339));
#160835=CARTESIAN_POINT('Ctrl Pts',(40.0257612616457,-64.120840424816,-177.007084281669));
#160836=CARTESIAN_POINT('Ctrl Pts',(40.0290093274313,-64.1199249071655,
-177.016833178237));
#160837=CARTESIAN_POINT('Ctrl Pts',(40.032565905416,-64.1189233487908,-177.026525725238));
#160838=CARTESIAN_POINT('Ctrl Pts',(40.0364307189981,-64.117836172251,-177.036140639572));
#160839=CARTESIAN_POINT('Ctrl Pts',(40.0465777997294,-64.1149817866814,
-177.061384628681));
#160840=CARTESIAN_POINT('Ctrl Pts',(40.0588564661358,-64.1115339220729,
-177.086112146133));
#160841=CARTESIAN_POINT('Ctrl Pts',(40.0732664004475,-64.1074920878103,
-177.109925913263));
#160842=CARTESIAN_POINT('Ctrl Pts',(40.0761741037768,-64.1066765077606,
-177.114731165561));
#160843=CARTESIAN_POINT('Ctrl Pts',(40.0791685416013,-64.1058367554325,
-177.119499049704));
#160844=CARTESIAN_POINT('Ctrl Pts',(40.0822496424732,-64.1049728460094,
-177.124226050751));
#160845=CARTESIAN_POINT('Ctrl Pts',(40.0914248199918,-64.1024002193263,
-177.138302536896));
#160846=CARTESIAN_POINT('Ctrl Pts',(40.1013686606316,-64.0996131928932,
-177.152016545396));
#160847=CARTESIAN_POINT('Ctrl Pts',(40.1120727242617,-64.09661173447,-177.165265493094));
#160848=CARTESIAN_POINT('Ctrl Pts',(40.1174247560767,-64.0951110052584,
-177.171889966943));
#160849=CARTESIAN_POINT('Ctrl Pts',(40.1229667901013,-64.0935566688765,
-177.178398084151));
#160850=CARTESIAN_POINT('Ctrl Pts',(40.1286966344869,-64.0919487277014,
-177.184775824956));
#160851=CARTESIAN_POINT('Ctrl Pts',(40.1315615566797,-64.0911447571138,
-177.187964695359));
#160852=CARTESIAN_POINT('Ctrl Pts',(40.1344734220793,-64.0903273854181,
-177.191120965598));
#160853=CARTESIAN_POINT('Ctrl Pts',(40.1374318783303,-64.0894966133288,
-177.194242832619));
#160854=CARTESIAN_POINT('Ctrl Pts',(40.1391481151386,-64.0890146722359,
-177.196053866022));
#160855=CARTESIAN_POINT('Ctrl Pts',(40.1412379161258,-64.0884276354813,
-177.198223860036));
#160856=CARTESIAN_POINT('Ctrl Pts',(40.1430815352768,-64.0879096560891,
-177.200104597065));
#160857=CARTESIAN_POINT('Ctrl Pts',(40.1444159545965,-64.0875347404196,
-177.201465882462));
#160858=CARTESIAN_POINT('Ctrl Pts',(40.1456200660741,-64.0871963786422,
-177.202676847247));
#160859=CARTESIAN_POINT('Ctrl Pts',(40.1464466064337,-64.0869640544319,
-177.20350338762));
#160860=CARTESIAN_POINT('Ctrl Pts',(40.1562413953246,-64.0842109322552,
-177.213298176676));
#160861=CARTESIAN_POINT('Ctrl Pts',(40.1671766857346,-64.0810919640796,
-177.223386446747));
#160862=CARTESIAN_POINT('Ctrl Pts',(40.1793814738916,-64.0775978129156,
-177.233531412315));
#160863=CARTESIAN_POINT('Ctrl Pts',(40.1910442959181,-64.0742588231162,
-177.243225880286));
#160864=CARTESIAN_POINT('Ctrl Pts',(40.2038670703147,-64.0705770418626,
-177.252972163816));
#160865=CARTESIAN_POINT('Ctrl Pts',(40.2179403413746,-64.0665504372626,
-177.262523160305));
#160866=CARTESIAN_POINT('Ctrl Pts',(40.231178516052,-64.062762768083,-177.271507408483));
#160867=CARTESIAN_POINT('Ctrl Pts',(40.2455236205272,-64.0586698727101,
-177.28031878073));
#160868=CARTESIAN_POINT('Ctrl Pts',(40.2610233215231,-64.0542776492498,
-177.288715370066));
#160869=CARTESIAN_POINT('Ctrl Pts',(40.2672493116986,-64.0525133610149,
-177.292088150142));
#160870=CARTESIAN_POINT('Ctrl Pts',(40.2736612359544,-64.050700874188,-177.295393584586));
#160871=CARTESIAN_POINT('Ctrl Pts',(40.2802605704505,-64.0488410075018,
-177.298614236585));
#160872=CARTESIAN_POINT('Ctrl Pts',(40.2954165061835,-64.0445696646893,
-177.306010739179));
#160873=CARTESIAN_POINT('Ctrl Pts',(40.3115733877844,-64.0400571937476,
-177.312967023157));
#160874=CARTESIAN_POINT('Ctrl Pts',(40.3287235889739,-64.0352854835157,
-177.319245722133));
#160875=CARTESIAN_POINT('Ctrl Pts',(40.3454088974569,-64.030643120646,-177.325354223609));
#160876=CARTESIAN_POINT('Ctrl Pts',(40.3630347088931,-64.0257552846044,
-177.330821391408));
#160877=CARTESIAN_POINT('Ctrl Pts',(40.3815578620981,-64.0206156603447,
-177.335399595475));
#160878=CARTESIAN_POINT('Ctrl Pts',(40.3996915438975,-64.0155841028197,
-177.339881537336));
#160879=CARTESIAN_POINT('Ctrl Pts',(40.4186855087824,-64.0103111421447,
-177.343511544901));
#160880=CARTESIAN_POINT('Ctrl Pts',(40.4384598241584,-64.0048023205012,
-177.346028622878));
#160881=CARTESIAN_POINT('Ctrl Pts',(40.4582341395344,-63.9992934988578,
-177.348545700855));
#160882=CARTESIAN_POINT('Ctrl Pts',(40.4787891949221,-63.9935486879891,
-177.34995));
#160883=CARTESIAN_POINT('Ctrl Pts',(40.5,-63.9875867194884,-177.34995));
#160884=CARTESIAN_POINT('Origin',(45.6308101826775,-63.2664983737155,-177.84995));
#160885=CARTESIAN_POINT('',(40.9304134495199,-63.4221822677665,-177.84995));
#160886=CARTESIAN_POINT('',(45.5612236321975,-62.7713643393447,-177.84995));
#160887=CARTESIAN_POINT('Origin',(41.,-63.9173163021373,-177.84995));
#160888=CARTESIAN_POINT('Ctrl Pts',(41.,-63.9173163021373,-177.34995));
#160889=CARTESIAN_POINT('Ctrl Pts',(40.9304134495199,-63.4221822677665,
-177.34995));
#160890=CARTESIAN_POINT('Ctrl Pts',(40.9304134495199,-63.4221822677665,
-177.84995));
#160891=CARTESIAN_POINT('Ctrl Pts',(41.1312673457634,-63.8804194574513,
-177.34995));
#160892=CARTESIAN_POINT('Ctrl Pts',(41.0616024612649,-63.4037448545523,
-177.367861075732));
#160893=CARTESIAN_POINT('Ctrl Pts',(41.1929481410454,-63.3852854230811,
-177.849949999941));
#160894=CARTESIAN_POINT('Ctrl Pts',(41.2609933446562,-63.8439558571173,
-177.296063436531));
#160895=CARTESIAN_POINT('Ctrl Pts',(41.2106847809575,-63.3827927009057,
-177.329589659683));
#160896=CARTESIAN_POINT('Ctrl Pts',(41.4524001388343,-63.3488218227467,
-177.742176873059));
#160897=CARTESIAN_POINT('Ctrl Pts',(41.4461134365302,-63.7919219926539,
-177.110943344657));
#160898=CARTESIAN_POINT('Ctrl Pts',(41.4304920983899,-63.3519007970349,
-177.142957948483));
#160899=CARTESIAN_POINT('Ctrl Pts',(41.8226403225787,-63.2967879582829,
-177.371936689315));
#160900=CARTESIAN_POINT('Ctrl Pts',(41.5,-63.7767754674458,-176.981217345763));
#160901=CARTESIAN_POINT('Ctrl Pts',(41.4999999999415,-63.342132098545,-176.997671841189));
#160902=CARTESIAN_POINT('Ctrl Pts',(41.9304134494542,-63.2816414330733,
-177.112484691526));
#160903=CARTESIAN_POINT('Ctrl Pts',(41.5,-63.7767754674349,-176.84995));
#160904=CARTESIAN_POINT('Ctrl Pts',(41.5,-63.3421320985267,-176.84995));
#160905=CARTESIAN_POINT('Ctrl Pts',(41.9304134495199,-63.2816414330641,
-176.84995));
#160906=CARTESIAN_POINT('',(41.9304134495199,-63.2816414330641,-176.84995));
#160907=CARTESIAN_POINT('Ctrl Pts',(41.9304134495199,-63.2816414330641,
-176.84995));
#160908=CARTESIAN_POINT('Ctrl Pts',(41.9304134494542,-63.2816414330733,
-177.112484691526));
#160909=CARTESIAN_POINT('Ctrl Pts',(41.8226403225787,-63.2967879582829,
-177.371936689315));
#160910=CARTESIAN_POINT('Ctrl Pts',(41.6375202307065,-63.3228048905148,
-177.557056781187));
#160911=CARTESIAN_POINT('Ctrl Pts',(41.4524001388343,-63.3488218227467,
-177.742176873059));
#160912=CARTESIAN_POINT('Ctrl Pts',(41.1929481410454,-63.3852854230811,
-177.849949999941));
#160913=CARTESIAN_POINT('Ctrl Pts',(40.9304134495199,-63.4221822677665,
-177.84995));
#160914=CARTESIAN_POINT('',(41.5,-63.7767754674349,-176.84995));
#160915=CARTESIAN_POINT('Origin',(42.,-63.7767754674349,-176.84995));
#160916=CARTESIAN_POINT('Ctrl Pts',(41.,-63.9173163021373,-177.34995));
#160917=CARTESIAN_POINT('Ctrl Pts',(41.0209105170156,-63.9114387391064,
-177.34995));
#160918=CARTESIAN_POINT('Ctrl Pts',(41.0411797466411,-63.9057414302056,
-177.348585219097));
#160919=CARTESIAN_POINT('Ctrl Pts',(41.0606899838377,-63.9002574601638,
-177.346136042571));
#160920=CARTESIAN_POINT('Ctrl Pts',(41.0806295626856,-63.894652810054,-177.343632969544));
#160921=CARTESIAN_POINT('Ctrl Pts',(41.0997766651611,-63.8892709105259,
-177.33999719389));
#160922=CARTESIAN_POINT('Ctrl Pts',(41.1180516974373,-63.8841341339452,
-177.335495637057));
#160923=CARTESIAN_POINT('Ctrl Pts',(41.1369112963569,-63.8788330463966,
-177.33085008814));
#160924=CARTESIAN_POINT('Ctrl Pts',(41.1548424167097,-63.8737929371535,
-177.32528246904));
#160925=CARTESIAN_POINT('Ctrl Pts',(41.1718018468568,-63.8690259522156,
-177.319052501424));
#160926=CARTESIAN_POINT('Ctrl Pts',(41.1874915731201,-63.864615857765,-177.313288953611));
#160927=CARTESIAN_POINT('Ctrl Pts',(41.2023504278525,-63.8604393060714,
-177.306958054963));
#160928=CARTESIAN_POINT('Ctrl Pts',(41.2163727601653,-63.8564978854959,
-177.300241547043));
#160929=CARTESIAN_POINT('Ctrl Pts',(41.2346217845916,-63.8513684192452,
-177.291500510647));
#160930=CARTESIAN_POINT('Ctrl Pts',(41.2514605911863,-63.8466353393768,
-177.282104513309));
#160931=CARTESIAN_POINT('Ctrl Pts',(41.2669358413727,-63.84228553022,-177.272394746022));
#160932=CARTESIAN_POINT('Ctrl Pts',(41.2822211818629,-63.8379891011976,
-177.262804135385));
#160933=CARTESIAN_POINT('Ctrl Pts',(41.2961768440954,-63.8340664203597,
-177.252906955733));
#160934=CARTESIAN_POINT('Ctrl Pts',(41.3088862629837,-63.8304940356814,
-177.242983686129));
#160935=CARTESIAN_POINT('Ctrl Pts',(41.321754987491,-63.8268768731138,-177.232936033763));
#160936=CARTESIAN_POINT('Ctrl Pts',(41.3333462707914,-63.8236187758533,
-177.222861821372));
#160937=CARTESIAN_POINT('Ctrl Pts',(41.3437756488962,-63.8206872688448,
-177.213007510354));
#160938=CARTESIAN_POINT('Ctrl Pts',(41.3450359570273,-63.8203330193313,
-177.211816694547));
#160939=CARTESIAN_POINT('Ctrl Pts',(41.3462793254426,-63.8199835312615,
-177.210629037565));
#160940=CARTESIAN_POINT('Ctrl Pts',(41.3475059843113,-63.8196387399389,
-177.209444926088));
#160941=CARTESIAN_POINT('Ctrl Pts',(41.348767397019,-63.8192841799492,-177.208227266229));
#160942=CARTESIAN_POINT('Ctrl Pts',(41.3496021366109,-63.8190495499469,
-177.207413007319));
#160943=CARTESIAN_POINT('Ctrl Pts',(41.3507626710068,-63.8187233292422,
-177.206271333214));
#160944=CARTESIAN_POINT('Ctrl Pts',(41.3514998739256,-63.8185161050044,
-177.205546110864));
#160945=CARTESIAN_POINT('Ctrl Pts',(41.3523682910511,-63.8182719925005,
-177.204688490104));
#160946=CARTESIAN_POINT('Ctrl Pts',(41.3535533858468,-63.8179388573381,
-177.20350339534));
#160947=CARTESIAN_POINT('Ctrl Pts',(41.3741026274597,-63.8121623785577,
-177.182954154279));
#160948=CARTESIAN_POINT('Ctrl Pts',(41.3925303081874,-63.8069824362895,
-177.160790380405));
#160949=CARTESIAN_POINT('Ctrl Pts',(41.4087935545141,-63.802411011162,-177.137499857787));
#160950=CARTESIAN_POINT('Ctrl Pts',(41.4250773096292,-63.7978338212329,
-177.114179964625));
#160951=CARTESIAN_POINT('Ctrl Pts',(41.4391911870226,-63.7938666788792,
-177.089730493817));
#160952=CARTESIAN_POINT('Ctrl Pts',(41.4511153275536,-63.7905151006712,
-177.064594612174));
#160953=CARTESIAN_POINT('Ctrl Pts',(41.463060046626,-63.7871577383489,-177.039415351322));
#160954=CARTESIAN_POINT('Ctrl Pts',(41.4728074902942,-63.7844180594708,
-177.013547308752));
#160955=CARTESIAN_POINT('Ctrl Pts',(41.4803606027944,-63.7822951743491,
-176.98738923497));
#160956=CARTESIAN_POINT('Ctrl Pts',(41.4879480469337,-63.7801626399437,
-176.961112263243));
#160957=CARTESIAN_POINT('Ctrl Pts',(41.4933211911952,-63.7786525123415,
-176.934542621811));
#160958=CARTESIAN_POINT('Ctrl Pts',(41.4965057497471,-63.7777575025999,
-176.908037356561));
#160959=CARTESIAN_POINT('Ctrl Pts',(41.498841154035,-63.7771011448806,-176.888599651426));
#160960=CARTESIAN_POINT('Ctrl Pts',(41.5,-63.7767754674349,-176.86919558342));
#160961=CARTESIAN_POINT('Ctrl Pts',(41.5,-63.7767754674349,-176.84995));
#160962=CARTESIAN_POINT('Origin',(45.4220505312374,-61.7810962706031,-172.64995));
#160963=CARTESIAN_POINT('',(42.,-62.2620341086569,-171.64995));
#160964=CARTESIAN_POINT('',(44.489435756687,-61.9121667294742,-171.64995));
#160965=CARTESIAN_POINT('',(44.489435756687,-61.9121667294742,-171.64995));
#160966=CARTESIAN_POINT('',(41.9304134495199,-63.2816414330641,-172.64995));
#160967=CARTESIAN_POINT('Ctrl Pts',(42.,-62.2620341086569,-171.64995));
#160968=CARTESIAN_POINT('Ctrl Pts',(41.9980582289126,-62.2904856414507,
-171.64995));
#160969=CARTESIAN_POINT('Ctrl Pts',(41.9961974246729,-62.3177508186883,
-171.651129585072));
#160970=CARTESIAN_POINT('Ctrl Pts',(41.9944225652579,-62.3437567012451,
-171.653192621565));
#160971=CARTESIAN_POINT('Ctrl Pts',(41.992554516627,-62.3711280259236,-171.655363978048));
#160972=CARTESIAN_POINT('Ctrl Pts',(41.9907816512346,-62.3971046913403,
-171.658513818877));
#160973=CARTESIAN_POINT('Ctrl Pts',(41.9891066446116,-62.4216474946475,
-171.662335033674));
#160974=CARTESIAN_POINT('Ctrl Pts',(41.9876075219068,-62.4436131831248,
-171.665755002159));
#160975=CARTESIAN_POINT('Ctrl Pts',(41.9861867195882,-62.4644312929545,
-171.66971333967));
#160976=CARTESIAN_POINT('Ctrl Pts',(41.9848444729658,-62.48409837629,-171.674015027433));
#160977=CARTESIAN_POINT('Ctrl Pts',(41.9832381238233,-62.5076351853414,
-171.679163121929));
#160978=CARTESIAN_POINT('Ctrl Pts',(41.9817442598049,-62.529523821642,-171.684802100301));
#160979=CARTESIAN_POINT('Ctrl Pts',(41.9803611921887,-62.5497890289526,
-171.690639736275));
#160980=CARTESIAN_POINT('Ctrl Pts',(41.9789186268577,-62.5709260183172,
-171.696728499524));
#160981=CARTESIAN_POINT('Ctrl Pts',(41.9775965324992,-62.5902978233885,
-171.703033282531));
#160982=CARTESIAN_POINT('Ctrl Pts',(41.9763912815383,-62.6079575967058,
-171.709272496533));
#160983=CARTESIAN_POINT('Ctrl Pts',(41.9758744940028,-62.6155297547265,
-171.711947746861));
#160984=CARTESIAN_POINT('Ctrl Pts',(41.9753791758627,-62.6227873353951,
-171.714611542068));
#160985=CARTESIAN_POINT('Ctrl Pts',(41.9749049735149,-62.6297355198322,
-171.717244495073));
#160986=CARTESIAN_POINT('Ctrl Pts',(41.9747845954644,-62.6314993425993,
-171.717912880101));
#160987=CARTESIAN_POINT('Ctrl Pts',(41.9747281084734,-62.6323259736101,
-171.718228248943));
#160988=CARTESIAN_POINT('Ctrl Pts',(41.9746071368898,-62.6340978795566,
-171.718908958995));
#160989=CARTESIAN_POINT('Ctrl Pts',(41.9745512101076,-62.6349170553895,
-171.719223660362));
#160990=CARTESIAN_POINT('Ctrl Pts',(41.9744815093958,-62.6359381423105,
-171.719616772037));
#160991=CARTESIAN_POINT('Ctrl Pts',(41.9743854515175,-62.6373456585733,
-171.720163005656));
#160992=CARTESIAN_POINT('Ctrl Pts',(41.974044857537,-62.6423363118667,-171.72209979508));
#160993=CARTESIAN_POINT('Ctrl Pts',(41.9737064547852,-62.6472948480561,
-171.724069245188));
#160994=CARTESIAN_POINT('Ctrl Pts',(41.9733702655354,-62.6522209415428,
-171.72607046184));
#160995=CARTESIAN_POINT('Ctrl Pts',(41.9710922898651,-62.6855995255356,
-171.739630451773));
#160996=CARTESIAN_POINT('Ctrl Pts',(41.96891676217,-62.7174765613617,-171.754642782338));
#160997=CARTESIAN_POINT('Ctrl Pts',(41.9668469622313,-62.7478042229328,
-171.770779293398));
#160998=CARTESIAN_POINT('Ctrl Pts',(41.9648622623225,-62.7768849596891,
-171.786252350205));
#160999=CARTESIAN_POINT('Ctrl Pts',(41.9629747403081,-62.8045416149154,
-171.802759466707));
#161000=CARTESIAN_POINT('Ctrl Pts',(41.9611851663792,-62.8307630998555,
-171.820043746496));
#161001=CARTESIAN_POINT('Ctrl Pts',(41.9591798424644,-62.8601458316816,
-171.839411808946));
#161002=CARTESIAN_POINT('Ctrl Pts',(41.9572974703087,-62.8877270298286,
-171.85975577606));
#161003=CARTESIAN_POINT('Ctrl Pts',(41.9555364549236,-62.9135300646481,
-171.88075761506));
#161004=CARTESIAN_POINT('Ctrl Pts',(41.954708197691,-62.9256659894071,-171.890635396478));
#161005=CARTESIAN_POINT('Ctrl Pts',(41.9539067520679,-62.9374090607585,
-171.900659292264));
#161006=CARTESIAN_POINT('Ctrl Pts',(41.9531317849258,-62.9487641598237,
-171.910799109226));
#161007=CARTESIAN_POINT('Ctrl Pts',(41.9527566361052,-62.9542609761269,
-171.915707627493));
#161008=CARTESIAN_POINT('Ctrl Pts',(41.9524097468125,-62.9593437235203,
-171.920348851332));
#161009=CARTESIAN_POINT('Ctrl Pts',(41.95205994185,-62.9644690402784,-171.92512412732));
#161010=CARTESIAN_POINT('Ctrl Pts',(41.9517205761669,-62.9694414014787,
-171.929756894068));
#161011=CARTESIAN_POINT('Ctrl Pts',(41.9513784560339,-62.9744539787111,
-171.934515912466));
#161012=CARTESIAN_POINT('Ctrl Pts',(41.9510073810277,-62.9798905322648,
-171.939801580944));
#161013=CARTESIAN_POINT('Ctrl Pts',(41.9509375838925,-62.9809131176108,
-171.94079578565));
#161014=CARTESIAN_POINT('Ctrl Pts',(41.9508667695452,-62.9819505975796,
-171.941808724746));
#161015=CARTESIAN_POINT('Ctrl Pts',(41.9507947743353,-62.9830053691253,
-171.94284321151));
#161016=CARTESIAN_POINT('Ctrl Pts',(41.9484463931933,-63.0174105137634,
-171.976586695463));
#161017=CARTESIAN_POINT('Ctrl Pts',(41.9462900974066,-63.0490042695942,
-172.012463058058));
#161018=CARTESIAN_POINT('Ctrl Pts',(41.9443343814679,-63.077660482026,-172.04995975798));
#161019=CARTESIAN_POINT('Ctrl Pts',(41.9423469358413,-63.1067816150827,
-172.088064807285));
#161020=CARTESIAN_POINT('Ctrl Pts',(41.9405666290003,-63.1328691487862,
-172.127843232645));
#161021=CARTESIAN_POINT('Ctrl Pts',(41.9390005719262,-63.1558171936301,
-172.168804472013));
#161022=CARTESIAN_POINT('Ctrl Pts',(41.9377708916514,-63.1738361780941,
-172.200967557837));
#161023=CARTESIAN_POINT('Ctrl Pts',(41.9366732704211,-63.1899200496495,
-172.23386087479));
#161024=CARTESIAN_POINT('Ctrl Pts',(41.935710408276,-63.2040284471142,-172.267266567535));
#161025=CARTESIAN_POINT('Ctrl Pts',(41.9356150487611,-63.2054257083375,
-172.270574985747));
#161026=CARTESIAN_POINT('Ctrl Pts',(41.9355210125586,-63.2068035707444,
-172.273888354284));
#161027=CARTESIAN_POINT('Ctrl Pts',(41.9354282968065,-63.2081620755033,
-172.27720644167));
#161028=CARTESIAN_POINT('Ctrl Pts',(41.9342160400824,-63.2259244997996,
-172.320590372139));
#161029=CARTESIAN_POINT('Ctrl Pts',(41.9332297201087,-63.240376417052,-172.364775502563));
#161030=CARTESIAN_POINT('Ctrl Pts',(41.9324628528116,-63.2516128342556,
-172.409267414287));
#161031=CARTESIAN_POINT('Ctrl Pts',(41.9316869655132,-63.262981415784,-172.454282646156));
#161032=CARTESIAN_POINT('Ctrl Pts',(41.9311357225737,-63.2710584268555,
-172.49961194977));
#161033=CARTESIAN_POINT('Ctrl Pts',(41.9308018218113,-63.27595086168,-172.544796239962));
#161034=CARTESIAN_POINT('Ctrl Pts',(41.9305416776487,-63.2797625881098,
-172.579999601747));
#161035=CARTESIAN_POINT('Ctrl Pts',(41.9304134495199,-63.2816414330641,
-172.615116019647));
#161036=CARTESIAN_POINT('Ctrl Pts',(41.9304134495199,-63.2816414330641,
-172.64995));
#161037=CARTESIAN_POINT('',(44.628608857647,-62.9024347982158,-172.64995));
#161038=CARTESIAN_POINT('',(41.5,-63.3421320985267,-172.64995));
#161039=CARTESIAN_POINT('Origin',(44.489435756687,-61.9121667294742,-172.64995));
#161040=CARTESIAN_POINT('Origin',(44.2110895547669,-59.9316305919911,-172.64995));
#161041=CARTESIAN_POINT('',(46.2674193015002,-62.1160087581289,-172.64995));
#161042=CARTESIAN_POINT('Origin',(44.2110895547669,-59.9316305919911,-172.64995));
#161043=CARTESIAN_POINT('',(45.5819760525891,-61.3878827027496,-171.64995));
#161044=CARTESIAN_POINT('Origin',(45.5819760525891,-61.3878827027496,-172.64995));
#161045=CARTESIAN_POINT('Origin',(44.2110895547669,-59.9316305919911,-171.64995));
#161046=CARTESIAN_POINT('Origin',(0.,-12.9675000200281,-172.64995));
#161047=CARTESIAN_POINT('',(49.148508738101,-59.2349193215281,-172.64995));
#161048=CARTESIAN_POINT('Origin',(0.,-12.9675000200281,-172.64995));
#161049=CARTESIAN_POINT('',(48.4203826827217,-58.549476072617,-171.64995));
#161050=CARTESIAN_POINT('Origin',(48.4203826827217,-58.549476072617,-172.64995));
#161051=CARTESIAN_POINT('Origin',(0.,-12.9675000200281,-171.64995));
#161052=CARTESIAN_POINT('Origin',(46.9641305719631,-57.1785895747948,-172.64995));
#161053=CARTESIAN_POINT('',(49.9349347781878,-57.596108877675,-172.64995));
#161054=CARTESIAN_POINT('Origin',(46.9641305719631,-57.1785895747948,-172.64995));
#161055=CARTESIAN_POINT('',(48.9446667094463,-57.4569357767149,-171.64995));
#161056=CARTESIAN_POINT('Origin',(48.9446667094463,-57.4569357767149,-172.64995));
#161057=CARTESIAN_POINT('Origin',(46.9641305719631,-57.1785895747948,-171.64995));
#161058=CARTESIAN_POINT('Ctrl Pts',(51.9388724063314,-46.43000002,-176.84995));
#161059=CARTESIAN_POINT('Ctrl Pts',(51.5042290374232,-46.43000002,-176.84995));
#161060=CARTESIAN_POINT('Ctrl Pts',(51.4437383719606,-46.86041346952,-176.84995));
#161061=CARTESIAN_POINT('Ctrl Pts',(51.9388724063423,-46.43000002,-176.981217345763));
#161062=CARTESIAN_POINT('Ctrl Pts',(51.5042290374242,-46.4300000199415,
-176.997671841189));
#161063=CARTESIAN_POINT('Ctrl Pts',(51.4437383719698,-46.8604134694541,
-177.112484691526));
#161064=CARTESIAN_POINT('Ctrl Pts',(51.9540189315504,-46.3761134565303,
-177.110943344657));
#161065=CARTESIAN_POINT('Ctrl Pts',(51.5139977359314,-46.3604921183892,
-177.142957948483));
#161066=CARTESIAN_POINT('Ctrl Pts',(51.4588848971795,-46.7526403425778,
-177.371936689315));
#161067=CARTESIAN_POINT('Ctrl Pts',(52.0060527960138,-46.1909933646562,
-177.296063436531));
#161068=CARTESIAN_POINT('Ctrl Pts',(51.5448896398021,-46.1406848009587,
-177.329589659683));
#161069=CARTESIAN_POINT('Ctrl Pts',(51.5109187616431,-46.3824001588352,
-177.742176873059));
#161070=CARTESIAN_POINT('Ctrl Pts',(52.0425163963479,-46.0612673657634,
-177.34995));
#161071=CARTESIAN_POINT('Ctrl Pts',(51.5658417934483,-45.9916024812643,
-177.367861075732));
#161072=CARTESIAN_POINT('Ctrl Pts',(51.5473823619777,-46.1229481610447,
-177.849949999941));
#161073=CARTESIAN_POINT('Ctrl Pts',(52.0794132410337,-45.93000002,-177.34995));
#161074=CARTESIAN_POINT('Ctrl Pts',(51.584279206663,-45.8604134695199,-177.34995));
#161075=CARTESIAN_POINT('Ctrl Pts',(51.584279206663,-45.86041346952,-177.84995));
#161076=CARTESIAN_POINT('',(51.584279206663,-45.86041346952,-177.84995));
#161077=CARTESIAN_POINT('Origin',(52.0794132410337,-45.93000002,-177.84995));
#161078=CARTESIAN_POINT('',(51.9388724063314,-46.43000002,-176.84995));
#161079=CARTESIAN_POINT('Ctrl Pts',(51.9388724063314,-46.43000002,-176.84995));
#161080=CARTESIAN_POINT('Ctrl Pts',(51.9388724063314,-46.43000002,-176.875800002306));
#161081=CARTESIAN_POINT('Ctrl Pts',(51.939460433088,-46.4279080061138,-176.901947474014));
#161082=CARTESIAN_POINT('Ctrl Pts',(51.9406481740044,-46.4236823982402,
-176.928073316625));
#161083=CARTESIAN_POINT('Ctrl Pts',(51.9418458934022,-46.4194212900745,
-176.954418648378));
#161084=CARTESIAN_POINT('Ctrl Pts',(51.9436534585173,-46.4129905430327,
-176.980741922985));
#161085=CARTESIAN_POINT('Ctrl Pts',(51.9460748639913,-46.4043759454358,
-177.006671795364));
#161086=CARTESIAN_POINT('Ctrl Pts',(51.9469983122141,-46.4010906076739,
-177.016560636708));
#161087=CARTESIAN_POINT('Ctrl Pts',(51.9480109554861,-46.3974879420354,
-177.026391811965));
#161088=CARTESIAN_POINT('Ctrl Pts',(51.9491127083337,-46.3935682526079,
-177.036143091591));
#161089=CARTESIAN_POINT('Ctrl Pts',(51.9519697581159,-46.3834037698484,
-177.06142997094));
#161090=CARTESIAN_POINT('Ctrl Pts',(51.9554279693915,-46.3711005439436,
-177.086198360269));
#161091=CARTESIAN_POINT('Ctrl Pts',(51.9594871634071,-46.3566592108427,
-177.110048753582));
#161092=CARTESIAN_POINT('Ctrl Pts',(51.9627845431406,-46.3449281728812,
-177.129422994686));
#161093=CARTESIAN_POINT('Ctrl Pts',(51.966478933354,-46.3317846967454,-177.148192204337));
#161094=CARTESIAN_POINT('Ctrl Pts',(51.9705652450017,-46.3172468876564,
-177.166105767697));
#161095=CARTESIAN_POINT('Ctrl Pts',(51.9727647076396,-46.3094218927259,
-177.175747766819));
#161096=CARTESIAN_POINT('Ctrl Pts',(51.9750776449811,-46.3011931905608,
-177.185141381874));
#161097=CARTESIAN_POINT('Ctrl Pts',(51.9775020131174,-46.2925680527438,
-177.194242926223));
#161098=CARTESIAN_POINT('Ctrl Pts',(51.977984409055,-46.2908518400194,-177.19605393337));
#161099=CARTESIAN_POINT('Ctrl Pts',(51.978571809157,-46.2887620555822,-177.198223909681));
#161100=CARTESIAN_POINT('Ctrl Pts',(51.9790900053177,-46.2869184469911,
-177.200104635539));
#161101=CARTESIAN_POINT('Ctrl Pts',(51.9794650751736,-46.2855840449618,
-177.201465903008));
#161102=CARTESIAN_POINT('Ctrl Pts',(51.9798035148913,-46.2843799457124,
-177.202676855488));
#161103=CARTESIAN_POINT('Ctrl Pts',(51.9800358214742,-46.2835534076204,
-177.203503393566));
#161104=CARTESIAN_POINT('Ctrl Pts',(51.982778794659,-46.2737940121103,-177.213262788912));
#161105=CARTESIAN_POINT('Ctrl Pts',(51.9858410519141,-46.2628991858342,
-177.223316643279));
#161106=CARTESIAN_POINT('Ctrl Pts',(51.9892581813619,-46.2507420960314,
-177.23342869837));
#161107=CARTESIAN_POINT('Ctrl Pts',(51.9925283434545,-46.2391078706274,
-177.243105843981));
#161108=CARTESIAN_POINT('Ctrl Pts',(51.9961237076887,-46.22631691666,-177.252836300724));
#161109=CARTESIAN_POINT('Ctrl Pts',(52.0000690386848,-46.2122809307154,
-177.262372868916));
#161110=CARTESIAN_POINT('Ctrl Pts',(52.0037880358436,-46.1990501544125,
-177.271362347883));
#161111=CARTESIAN_POINT('Ctrl Pts',(52.0078181206063,-46.1847126616024,
-177.280179445043));
#161112=CARTESIAN_POINT('Ctrl Pts',(52.0121719933272,-46.1692230962462,
-177.288581471766));
#161113=CARTESIAN_POINT('Ctrl Pts',(52.0139487850297,-46.1629018891359,
-177.29201029303));
#161114=CARTESIAN_POINT('Ctrl Pts',(52.0157793940052,-46.1563891942317,
-177.295369566868));
#161115=CARTESIAN_POINT('Ctrl Pts',(52.0176641944465,-46.1496836682356,
-177.298640995833));
#161116=CARTESIAN_POINT('Ctrl Pts',(52.0219346251205,-46.1344908216757,
-177.306053138942));
#161117=CARTESIAN_POINT('Ctrl Pts',(52.0264864211104,-46.1182969659914,
-177.313020714078));
#161118=CARTESIAN_POINT('Ctrl Pts',(52.0313178036988,-46.1011084292979,
-177.319306663921));
#161119=CARTESIAN_POINT('Ctrl Pts',(52.0360111994689,-46.084410806219,-177.325413083744));
#161120=CARTESIAN_POINT('Ctrl Pts',(52.0409685266907,-46.06677419821,-177.330876292405));
#161121=CARTESIAN_POINT('Ctrl Pts',(52.0461782020365,-46.0482398151008,
-177.335449266094));
#161122=CARTESIAN_POINT('Ctrl Pts',(52.0512666586451,-46.0301366900576,
-177.339915835822));
#161123=CARTESIAN_POINT('Ctrl Pts',(52.0565959389366,-46.0111767902437,
-177.343533167656));
#161124=CARTESIAN_POINT('Ctrl Pts',(52.0621443742083,-45.9914372060744,
-177.34604166628));
#161125=CARTESIAN_POINT('Ctrl Pts',(52.06769280948,-45.9716976219051,-177.348550164905));
#161126=CARTESIAN_POINT('Ctrl Pts',(52.0734605256988,-45.9511779052299,
-177.34995));
#161127=CARTESIAN_POINT('Ctrl Pts',(52.0794132410337,-45.93000002,-177.34995));
#161128=CARTESIAN_POINT('',(51.4437383719606,-46.86041346952,-176.84995));
#161129=CARTESIAN_POINT('Origin',(51.9388724063314,-46.93000002,-176.84995));
#161130=CARTESIAN_POINT('Ctrl Pts',(51.584279206663,-45.86041346952,-177.84995));
#161131=CARTESIAN_POINT('Ctrl Pts',(51.5473823619777,-46.1229481610447,
-177.849949999941));
#161132=CARTESIAN_POINT('Ctrl Pts',(51.5109187616431,-46.3824001588352,
-177.742176873059));
#161133=CARTESIAN_POINT('Ctrl Pts',(51.4849018294113,-46.5675202507065,
-177.557056781187));
#161134=CARTESIAN_POINT('Ctrl Pts',(51.4588848971795,-46.7526403425778,
-177.371936689315));
#161135=CARTESIAN_POINT('Ctrl Pts',(51.4437383719698,-46.8604134694541,
-177.112484691526));
#161136=CARTESIAN_POINT('Ctrl Pts',(51.4437383719606,-46.86041346952,-176.84995));
#161137=CARTESIAN_POINT('Origin',(53.1076143453209,-38.6139690140329,-177.84995));
#161138=CARTESIAN_POINT('',(51.6545496240141,-45.3604134695199,-177.84995));
#161139=CARTESIAN_POINT('',(52.6124803109501,-38.5443824635529,-177.84995));
#161140=CARTESIAN_POINT('Origin',(52.1496836583849,-45.43000002,-177.84995));
#161141=CARTESIAN_POINT('Ctrl Pts',(52.1497209086987,-45.4300399704538,
-177.349950000614));
#161142=CARTESIAN_POINT('Ctrl Pts',(51.6545448046101,-45.3604477613618,
-177.349907583593));
#161143=CARTESIAN_POINT('Ctrl Pts',(51.6545402370025,-45.3604802615783,
-177.849949997675));
#161144=CARTESIAN_POINT('Ctrl Pts',(52.1866217328369,-45.2987616698911,
-177.349960874823));
#161145=CARTESIAN_POINT('Ctrl Pts',(51.6738419432767,-45.2231414851577,
-177.331166751555));
#161146=CARTESIAN_POINT('Ctrl Pts',(51.6914402841046,-45.097922783674,-177.849968278574));
#161147=CARTESIAN_POINT('Ctrl Pts',(52.2230902788089,-45.1690198513555,
-177.296074808573));
#161148=CARTESIAN_POINT('Ctrl Pts',(51.6896993598511,-45.1103101034141,
-177.25721607327));
#161149=CARTESIAN_POINT('Ctrl Pts',(51.7279078626935,-44.8384424791336,
-177.742192571987));
#161150=CARTESIAN_POINT('Ctrl Pts',(52.2751299595662,-44.9838805435436,
-177.110939115585));
#161151=CARTESIAN_POINT('Ctrl Pts',(51.7103493697401,-44.9633776482459,
-177.069853325702));
#161152=CARTESIAN_POINT('Ctrl Pts',(51.7799461398382,-44.4681708975332,
-177.371920990387));
#161153=CARTESIAN_POINT('Ctrl Pts',(52.2902773198134,-44.9299908778567,
-176.981197291835));
#161154=CARTESIAN_POINT('Ctrl Pts',(51.7150329623736,-44.9300521550416,
-176.95888267251));
#161155=CARTESIAN_POINT('Ctrl Pts',(51.7950930276016,-44.3603951909531,
-177.112440685846));
#161156=CARTESIAN_POINT('Ctrl Pts',(52.2902747589836,-44.9300000186359,
-176.849916603474));
#161157=CARTESIAN_POINT('Ctrl Pts',(51.7150321621775,-44.9300578487394,
-176.849922286133));
#161158=CARTESIAN_POINT('Ctrl Pts',(51.7950904583897,-44.3604134718452,
-176.849883207942));
#161159=CARTESIAN_POINT('',(51.7950904587165,-44.36041346952,-176.84995));
#161160=CARTESIAN_POINT('Ctrl Pts',(51.7950904587165,-44.36041346952,-176.84995));
#161161=CARTESIAN_POINT('Ctrl Pts',(51.7950904587073,-44.3604134695857,
-177.112484691526));
#161162=CARTESIAN_POINT('Ctrl Pts',(51.7799439334977,-44.4681865964612,
-177.371936689315));
#161163=CARTESIAN_POINT('Ctrl Pts',(51.7539270012658,-44.6533066883334,
-177.557056781187));
#161164=CARTESIAN_POINT('Ctrl Pts',(51.7279100690339,-44.8384267802056,
-177.742176873059));
#161165=CARTESIAN_POINT('Ctrl Pts',(51.6914464686995,-45.0978787779945,
-177.849949999941));
#161166=CARTESIAN_POINT('Ctrl Pts',(51.6545496240141,-45.3604134695199,
-177.84995));
#161167=CARTESIAN_POINT('',(52.2902244930873,-44.93000002,-176.84995));
#161168=CARTESIAN_POINT('Origin',(52.2902244930873,-44.43000002,-176.84995));
#161169=CARTESIAN_POINT('Ctrl Pts',(52.1496836583849,-45.43000002,-177.34995));
#161170=CARTESIAN_POINT('Ctrl Pts',(52.1557508202169,-45.4084149701999,
-177.34995));
#161171=CARTESIAN_POINT('Ctrl Pts',(52.1615771773264,-45.3874879725988,
-177.348552025671));
#161172=CARTESIAN_POINT('Ctrl Pts',(52.1671627297135,-45.367368300209,-177.346011757925));
#161173=CARTESIAN_POINT('Ctrl Pts',(52.172739418816,-45.3472805541836,-177.343475521136));
#161174=CARTESIAN_POINT('Ctrl Pts',(52.1780760668187,-45.3279969954851,
-177.339801327605));
#161175=CARTESIAN_POINT('Ctrl Pts',(52.1831726737217,-45.309608680057,-177.335239527258));
#161176=CARTESIAN_POINT('Ctrl Pts',(52.1884924652697,-45.2904151250394,
-177.33047796189));
#161177=CARTESIAN_POINT('Ctrl Pts',(52.1935507322084,-45.2721966220856,
-177.324750042966));
#161178=CARTESIAN_POINT('Ctrl Pts',(52.1983474745379,-45.2550003525823,
-177.318324974143));
#161179=CARTESIAN_POINT('Ctrl Pts',(52.2027636467357,-45.2391684228957,
-177.31240966572));
#161180=CARTESIAN_POINT('Ctrl Pts',(52.206958146453,-45.2242018844323,-177.305903491103));
#161181=CARTESIAN_POINT('Ctrl Pts',(52.2109309736898,-45.2101026376804,
-177.298999152375));
#161182=CARTESIAN_POINT('Ctrl Pts',(52.2155599839996,-45.1936746495792,
-177.290954439316));
#161183=CARTESIAN_POINT('Ctrl Pts',(52.2198880482107,-45.1784243291713,
-177.282370206816));
#161184=CARTESIAN_POINT('Ctrl Pts',(52.223915166323,-45.1643108658193,-177.273517318558));
#161185=CARTESIAN_POINT('Ctrl Pts',(52.2270926918441,-45.1531748899825,
-177.266532105414));
#161186=CARTESIAN_POINT('Ctrl Pts',(52.2300828568474,-45.1427456090391,
-177.259378907546));
#161187=CARTESIAN_POINT('Ctrl Pts',(52.232885661333,-45.13298799345,-177.252173639391));
#161188=CARTESIAN_POINT('Ctrl Pts',(52.2360631664952,-45.1219259040088,
-177.244005115015));
#161189=CARTESIAN_POINT('Ctrl Pts',(52.238999866935,-45.111726951001,-177.235770093483));
#161190=CARTESIAN_POINT('Ctrl Pts',(52.2416957626522,-45.1023265017848,
-177.227613958382));
#161191=CARTESIAN_POINT('Ctrl Pts',(52.2430437105108,-45.0976262771767,
-177.223535890831));
#161192=CARTESIAN_POINT('Ctrl Pts',(52.2443314571889,-45.0931254933336,
-177.219477157756));
#161193=CARTESIAN_POINT('Ctrl Pts',(52.2455590026863,-45.0888152125502,
-177.215453662315));
#161194=CARTESIAN_POINT('Ctrl Pts',(52.246172775435,-45.0866600721585,-177.213441914594));
#161195=CARTESIAN_POINT('Ctrl Pts',(52.2467714978885,-45.0845525658363,
-177.211438967526));
#161196=CARTESIAN_POINT('Ctrl Pts',(52.2473551700469,-45.0824915202267,
-177.209446651703));
#161197=CARTESIAN_POINT('Ctrl Pts',(52.2477174877031,-45.0812121149925,
-177.208209910855));
#161198=CARTESIAN_POINT('Ctrl Pts',(52.2479568632044,-45.0803718707492,
-177.20738941522));
#161199=CARTESIAN_POINT('Ctrl Pts',(52.2482914474766,-45.0791841923715,
-177.206219918861));
#161200=CARTESIAN_POINT('Ctrl Pts',(52.2484958585334,-45.0784585916408,
-177.20550542626));
#161201=CARTESIAN_POINT('Ctrl Pts',(52.2487358060927,-45.0776035977889,
-177.204660358975));
#161202=CARTESIAN_POINT('Ctrl Pts',(52.2490610356366,-45.0764466294067,
-177.203503390593));
#161203=CARTESIAN_POINT('Ctrl Pts',(52.2541090747794,-45.0584887845861,
-177.185545545773));
#161204=CARTESIAN_POINT('Ctrl Pts',(52.2586928180255,-45.0420748638293,
-177.166390617213));
#161205=CARTESIAN_POINT('Ctrl Pts',(52.2628122653748,-45.027308366338,-177.146327178728));
#161206=CARTESIAN_POINT('Ctrl Pts',(52.2669899506247,-45.0123331103072,
-177.125980097212));
#161207=CARTESIAN_POINT('Ctrl Pts',(52.2706901193928,-44.9990520483592,
-177.104699239602));
#161208=CARTESIAN_POINT('Ctrl Pts',(52.2739127716791,-44.9875196153263,
-177.082782754311));
#161209=CARTESIAN_POINT('Ctrl Pts',(52.2772061377067,-44.9757341293998,
-177.060385361824));
#161210=CARTESIAN_POINT('Ctrl Pts',(52.2800008013202,-44.9657746706807,
-177.037324735901));
#161211=CARTESIAN_POINT('Ctrl Pts',(52.2822967625197,-44.9576461996328,
-177.013906910146));
#161212=CARTESIAN_POINT('Ctrl Pts',(52.2846217509038,-44.9494149626367,
-176.990193019478));
#161213=CARTESIAN_POINT('Ctrl Pts',(52.2864353472564,-44.9430609412307,
-176.966113358338));
#161214=CARTESIAN_POINT('Ctrl Pts',(52.2877375515776,-44.9385396784594,
-176.941964850393));
#161215=CARTESIAN_POINT('Ctrl Pts',(52.2890642583169,-44.9339333431161,
-176.917361961496));
#161216=CARTESIAN_POINT('Ctrl Pts',(52.2898601471524,-44.9312289800572,
-176.892688085414));
#161217=CARTESIAN_POINT('Ctrl Pts',(52.2901252180841,-44.9303342185764,
-176.868228043869));
#161218=CARTESIAN_POINT('Ctrl Pts',(52.2901914014196,-44.9301108130943,
-176.862120821454));
#161219=CARTESIAN_POINT('Ctrl Pts',(52.2902244930873,-44.93000002,-176.856026770997));
#161220=CARTESIAN_POINT('Ctrl Pts',(52.2902244930873,-44.93000002,-176.84995));
#161221=CARTESIAN_POINT('Origin',(51.6222122422086,-38.4052093625928,-172.64995));
#161222=CARTESIAN_POINT('',(51.7950904587165,-44.36041346952,-172.64995));
#161223=CARTESIAN_POINT('Ctrl Pts',(50.7754831343094,-44.43000002,-171.64995));
#161224=CARTESIAN_POINT('Ctrl Pts',(50.8046140710912,-44.4280118806895,
-171.64995));
#161225=CARTESIAN_POINT('Ctrl Pts',(50.8325027036972,-44.4261255344678,
-171.651172745859));
#161226=CARTESIAN_POINT('Ctrl Pts',(50.859069989913,-44.4243298726759,-171.653316375858));
#161227=CARTESIAN_POINT('Ctrl Pts',(50.8868184408941,-44.4224543768949,
-171.655555310293));
#161228=CARTESIAN_POINT('Ctrl Pts',(50.9131258825754,-44.4206778703683,
-171.658798248564));
#161229=CARTESIAN_POINT('Ctrl Pts',(50.9379516616092,-44.4189946396407,
-171.662728774772));
#161230=CARTESIAN_POINT('Ctrl Pts',(50.9633985651933,-44.417269295595,-171.666757640143));
#161231=CARTESIAN_POINT('Ctrl Pts',(50.9872894292095,-44.4156420502453,
-171.671508529141));
#161232=CARTESIAN_POINT('Ctrl Pts',(51.0096221990147,-44.4141126148304,
-171.676676564296));
#161233=CARTESIAN_POINT('Ctrl Pts',(51.0326894620957,-44.4125328784436,
-171.682014568832));
#161234=CARTESIAN_POINT('Ctrl Pts',(51.0540951810777,-44.4110575929876,
-171.687797262872));
#161235=CARTESIAN_POINT('Ctrl Pts',(51.0738701191736,-44.40969108195,-171.693732405553));
#161236=CARTESIAN_POINT('Ctrl Pts',(51.0768409738807,-44.4094857864528,
-171.694624061774));
#161237=CARTESIAN_POINT('Ctrl Pts',(51.0797750688298,-44.4092829526126,
-171.69551924183));
#161238=CARTESIAN_POINT('Ctrl Pts',(51.0826725543606,-44.4090826015581,
-171.696417042979));
#161239=CARTESIAN_POINT('Ctrl Pts',(51.0954249653932,-44.4082008166554,
-171.700368444688));
#161240=CARTESIAN_POINT('Ctrl Pts',(51.1074680002581,-44.407367092164,-171.70436993824));
#161241=CARTESIAN_POINT('Ctrl Pts',(51.1188164928691,-44.4065835128548,
-171.708349867282));
#161242=CARTESIAN_POINT('Ctrl Pts',(51.1244907391747,-44.4061917232002,
-171.710339831803));
#161243=CARTESIAN_POINT('Ctrl Pts',(51.1299913124772,-44.4058124645793,
-171.712324508957));
#161244=CARTESIAN_POINT('Ctrl Pts',(51.1353203844627,-44.4054460422028,
-171.714295777063));
#161245=CARTESIAN_POINT('Ctrl Pts',(51.1379849204555,-44.4052628310145,
-171.715281411117));
#161246=CARTESIAN_POINT('Ctrl Pts',(51.1406065787668,-44.4050828285567,
-171.716263699775));
#161247=CARTESIAN_POINT('Ctrl Pts',(51.143185625721,-44.4049060722589,-171.717241672115));
#161248=CARTESIAN_POINT('Ctrl Pts',(51.1449546614015,-44.4047848304966,
-171.717912488892));
#161249=CARTESIAN_POINT('Ctrl Pts',(51.1457809331891,-44.4047277477496,
-171.718227889236));
#161250=CARTESIAN_POINT('Ctrl Pts',(51.1475638474567,-44.4046060349278,
-171.718913272981));
#161251=CARTESIAN_POINT('Ctrl Pts',(51.1483802134989,-44.404550304702,-171.719227098512));
#161252=CARTESIAN_POINT('Ctrl Pts',(51.1493970225313,-44.4044810069703,
-171.719618819405));
#161253=CARTESIAN_POINT('Ctrl Pts',(51.1507951962543,-44.4043855789116,
-171.720161698938));
#161254=CARTESIAN_POINT('Ctrl Pts',(51.1845048073339,-44.4020848328094,
-171.733250385712));
#161255=CARTESIAN_POINT('Ctrl Pts',(51.2167470072588,-44.3998963013987,
-171.747810336066));
#161256=CARTESIAN_POINT('Ctrl Pts',(51.2474534328981,-44.3978103768682,
-171.763538020509));
#161257=CARTESIAN_POINT('Ctrl Pts',(51.278964188969,-44.3956698132013,-171.779677679156));
#161258=CARTESIAN_POINT('Ctrl Pts',(51.3088579736835,-44.3936373462816,
-171.797046561303));
#161259=CARTESIAN_POINT('Ctrl Pts',(51.337111582541,-44.3917097149291,-171.815335003271));
#161260=CARTESIAN_POINT('Ctrl Pts',(51.3395010289291,-44.3915466925062,
-171.81688168185));
#161261=CARTESIAN_POINT('Ctrl Pts',(51.3418787717478,-44.3913844237635,
-171.818434950475));
#161262=CARTESIAN_POINT('Ctrl Pts',(51.3442448118475,-44.3912229088206,
-171.819994629286));
#161263=CARTESIAN_POINT('Ctrl Pts',(51.3730476143694,-44.3892567194037,
-171.838981256258));
#161264=CARTESIAN_POINT('Ctrl Pts',(51.4001125383987,-44.3874017274751,
-171.858915412102));
#161265=CARTESIAN_POINT('Ctrl Pts',(51.4254654811503,-44.3856615726511,
-171.879488097268));
#161266=CARTESIAN_POINT('Ctrl Pts',(51.4381419525261,-44.3847914952391,
-171.889774439851));
#161267=CARTESIAN_POINT('Ctrl Pts',(51.4503911131589,-44.3839502233142,
-171.900220871966));
#161268=CARTESIAN_POINT('Ctrl Pts',(51.4622199181929,-44.3831387343582,
-171.91079164189));
#161269=CARTESIAN_POINT('Ctrl Pts',(51.4677366951224,-44.3827602681024,
-171.915721690148));
#161270=CARTESIAN_POINT('Ctrl Pts',(51.472836767171,-44.3824082123661,-171.920381836519));
#161271=CARTESIAN_POINT('Ctrl Pts',(51.4779815600685,-44.3820555671411,
-171.925178375141));
#161272=CARTESIAN_POINT('Ctrl Pts',(51.4829853346238,-44.3817125878921,
-171.929843441042));
#161273=CARTESIAN_POINT('Ctrl Pts',(51.4880315628651,-44.3813690722246,
-171.934637611724));
#161274=CARTESIAN_POINT('Ctrl Pts',(51.4935119510881,-44.3809955693083,
-171.93996907612));
#161275=CARTESIAN_POINT('Ctrl Pts',(51.4944786714865,-44.3809296847627,
-171.940909526902));
#161276=CARTESIAN_POINT('Ctrl Pts',(51.4954588090377,-44.3808628542106,
-171.941866786846));
#161277=CARTESIAN_POINT('Ctrl Pts',(51.4964543875452,-44.3807948982762,
-171.942843218813));
#161278=CARTESIAN_POINT('Ctrl Pts',(51.527246566966,-44.378693093839,-171.97304321622));
#161279=CARTESIAN_POINT('Ctrl Pts',(51.5558098726652,-44.3767752596171,
-172.004935794556));
#161280=CARTESIAN_POINT('Ctrl Pts',(51.5820175750055,-44.3750235849214,
-172.038177891501));
#161281=CARTESIAN_POINT('Ctrl Pts',(51.608536381873,-44.3732511165704,-172.071814596365));
#161282=CARTESIAN_POINT('Ctrl Pts',(51.6326434300992,-44.3716487903803,
-172.106832536843));
#161283=CARTESIAN_POINT('Ctrl Pts',(51.6542606346252,-44.3702056322116,
-172.142877708409));
#161284=CARTESIAN_POINT('Ctrl Pts',(51.6761396036481,-44.3687449987228,
-172.179359353905));
#161285=CARTESIAN_POINT('Ctrl Pts',(51.695468239182,-44.3674474359092,-172.216892769522));
#161286=CARTESIAN_POINT('Ctrl Pts',(51.7122176676771,-44.3663088858582,
-172.255120022089));
#161287=CARTESIAN_POINT('Ctrl Pts',(51.7292787416113,-44.3651491515662,
-172.294058543635));
#161288=CARTESIAN_POINT('Ctrl Pts',(51.743663933231,-44.3641544300339,-172.333716479681));
#161289=CARTESIAN_POINT('Ctrl Pts',(51.7553936826929,-44.3633275939378,
-172.373732379002));
#161290=CARTESIAN_POINT('Ctrl Pts',(51.7672496456042,-44.3624918609906,
-172.414178853989));
#161291=CARTESIAN_POINT('Ctrl Pts',(51.7763930408945,-44.361827691907,-172.454990623027));
#161292=CARTESIAN_POINT('Ctrl Pts',(51.7828924549402,-44.3613447258736,
-172.495818301195));
#161293=CARTESIAN_POINT('Ctrl Pts',(51.7894949535036,-44.3608540997158,
-172.537293530278));
#161294=CARTESIAN_POINT('Ctrl Pts',(51.7933692868094,-44.3605505195348,
-172.578784792061));
#161295=CARTESIAN_POINT('Ctrl Pts',(51.7946309645435,-44.3604502191584,
-172.619956446103));
#161296=CARTESIAN_POINT('Ctrl Pts',(51.7949379634072,-44.3604258134796,
-172.629974575665));
#161297=CARTESIAN_POINT('Ctrl Pts',(51.7950904587166,-44.36041346952,-172.639973936947));
#161298=CARTESIAN_POINT('Ctrl Pts',(51.7950904587166,-44.36041346952,-172.64995));
#161299=CARTESIAN_POINT('',(51.9770573602378,-43.0656516879596,-172.64995));
#161300=CARTESIAN_POINT('',(51.7150402894768,-44.93000002,-172.64995));
#161301=CARTESIAN_POINT('Origin',(50.9867892914962,-42.9264785869994,-172.64995));
#161302=CARTESIAN_POINT('Ctrl Pts',(51.9770573602378,-43.0656516879596,
-172.64995));
#161303=CARTESIAN_POINT('Ctrl Pts',(51.9770573602378,-43.0656516879595,
-171.64995));
#161304=CARTESIAN_POINT('Ctrl Pts',(50.9867892914962,-42.9264785869994,
-171.64995));
#161305=CARTESIAN_POINT('Ctrl Pts',(52.0666747393887,-42.4279909017497,
-172.649949997757));
#161306=CARTESIAN_POINT('Ctrl Pts',(52.0557320324863,-42.5058523071511,
-171.757498535929));
#161307=CARTESIAN_POINT('Ctrl Pts',(51.1823572933545,-42.3510730842576,
-171.64995));
#161308=CARTESIAN_POINT('Ctrl Pts',(52.1554800333146,-41.7961084021622,
-172.606056153133));
#161309=CARTESIAN_POINT('Ctrl Pts',(52.1416679592955,-41.8943864154851,
-171.81403941883));
#161310=CARTESIAN_POINT('Ctrl Pts',(51.3741578990751,-41.7754043578546,
-171.628003076365));
#161311=CARTESIAN_POINT('Ctrl Pts',(52.3315472405273,-40.5433251268562,
-172.43788181511));
#161312=CARTESIAN_POINT('Ctrl Pts',(52.3125022740342,-40.6788371047634,
-171.821280489149));
#161313=CARTESIAN_POINT('Ctrl Pts',(51.7497860966445,-40.6237611991777,
-171.543915907757));
#161314=CARTESIAN_POINT('Ctrl Pts',(52.4188787332529,-39.9219292677054,
-172.315208572937));
#161315=CARTESIAN_POINT('Ctrl Pts',(52.3988291636532,-40.0645893682337,
-171.781794156641));
#161316=CARTESIAN_POINT('Ctrl Pts',(51.9336694513069,-40.0475756797307,
-171.482621144039));
#161317=CARTESIAN_POINT('Ctrl Pts',(52.5050296388285,-39.3089337226171,
-172.133326251627));
#161318=CARTESIAN_POINT('Ctrl Pts',(52.4864722882118,-39.4409761333229,
-171.679515584751));
#161319=CARTESIAN_POINT('Ctrl Pts',(52.1126146143194,-39.473850183348,-171.391638125813));
#161320=CARTESIAN_POINT('',(52.5050296388285,-39.3089337226171,-172.133326251627));
#161321=CARTESIAN_POINT('Ctrl Pts',(52.5050296388285,-39.3089337226171,
-172.133326251627));
#161322=CARTESIAN_POINT('Ctrl Pts',(52.4540911811658,-39.6713796819752,
-172.240867836497));
#161323=CARTESIAN_POINT('Ctrl Pts',(52.4027597205579,-40.0366220025906,
-172.327673864957));
#161324=CARTESIAN_POINT('Ctrl Pts',(52.3511170282711,-40.4040788516705,
-172.398058085082));
#161325=CARTESIAN_POINT('Ctrl Pts',(52.3153892921751,-40.6582949033369,
-172.446751689745));
#161326=CARTESIAN_POINT('Ctrl Pts',(52.2795125603003,-40.9135711150572,
-172.487583846606));
#161327=CARTESIAN_POINT('Ctrl Pts',(52.2435136369167,-41.1697167645394,
-172.521968983892));
#161328=CARTESIAN_POINT('Ctrl Pts',(52.1712955694614,-41.6835750151203,
-172.590949606937));
#161329=CARTESIAN_POINT('Ctrl Pts',(52.0985648108855,-42.2010812525765,
-172.632879273599));
#161330=CARTESIAN_POINT('Ctrl Pts',(52.0252827479162,-42.7225102246227,
-172.645720761145));
#161331=CARTESIAN_POINT('Ctrl Pts',(52.0092341999946,-42.8367015765921,
-172.648533007689));
#161332=CARTESIAN_POINT('Ctrl Pts',(51.9931592080447,-42.9510810876001,
-172.649949999597));
#161333=CARTESIAN_POINT('Ctrl Pts',(51.9770573602378,-43.0656516879596,
-172.64995));
#161334=CARTESIAN_POINT('Origin',(51.5147615700869,-39.1697606216571,-172.133326251627));
#161335=CARTESIAN_POINT('Origin',(51.6222122422086,-38.4052093625928,-172.64995));
#161336=CARTESIAN_POINT('',(50.2983305691361,-55.0104134695199,-172.64995));
#161337=CARTESIAN_POINT('',(49.9349347781878,-57.596108877675,-172.64995));
#161338=CARTESIAN_POINT('',(49.2787232447289,-55.08000002,-171.64995));
#161339=CARTESIAN_POINT('Ctrl Pts',(50.2983305691361,-55.0104134695199,
-172.64995));
#161340=CARTESIAN_POINT('Ctrl Pts',(50.2983305691361,-55.0104134695199,
-172.605172304705));
#161341=CARTESIAN_POINT('Ctrl Pts',(50.2952256853384,-55.0106253728164,
-172.559925284473));
#161342=CARTESIAN_POINT('Ctrl Pts',(50.2889016465528,-55.0110569782332,
-172.514629908981));
#161343=CARTESIAN_POINT('Ctrl Pts',(50.2826524098944,-55.0114834785258,
-172.469870297193));
#161344=CARTESIAN_POINT('Ctrl Pts',(50.2732597042546,-55.0121245154913,
-172.425063433793));
#161345=CARTESIAN_POINT('Ctrl Pts',(50.260621229954,-55.0129870709171,-172.380665523989));
#161346=CARTESIAN_POINT('Ctrl Pts',(50.2507110648879,-55.0136634236512,
-172.34585193777));
#161347=CARTESIAN_POINT('Ctrl Pts',(50.2388053749292,-55.0144759677311,
-172.311290758928));
#161348=CARTESIAN_POINT('Ctrl Pts',(50.2248584410366,-55.0154278234074,
-172.277224099798));
#161349=CARTESIAN_POINT('Ctrl Pts',(50.2234976012156,-55.0155206985238,
-172.273900124315));
#161350=CARTESIAN_POINT('Ctrl Pts',(50.2221173289147,-55.0156148998755,
-172.270580868756));
#161351=CARTESIAN_POINT('Ctrl Pts',(50.2207175829473,-55.0157104302734,
-172.267266567635));
#161352=CARTESIAN_POINT('Ctrl Pts',(50.2026895854313,-55.0169408119401,
-172.224580098969));
#161353=CARTESIAN_POINT('Ctrl Pts',(50.1814340508794,-55.0183914677883,
-172.182726614308));
#161354=CARTESIAN_POINT('Ctrl Pts',(50.1570394248576,-55.0200563615513,
-172.142169045314));
#161355=CARTESIAN_POINT('Ctrl Pts',(50.1336253811801,-55.0216543321555,
-172.103241754893));
#161356=CARTESIAN_POINT('Ctrl Pts',(50.1073206492679,-55.0234495875555,
-172.065509332316));
#161357=CARTESIAN_POINT('Ctrl Pts',(50.0782208862319,-55.0254355993083,
-172.029413465929));
#161358=CARTESIAN_POINT('Ctrl Pts',(50.0647174562256,-55.0263571865618,
-172.012663569901));
#161359=CARTESIAN_POINT('Ctrl Pts',(50.0506123834973,-55.0273198349579,
-171.996266629338));
#161360=CARTESIAN_POINT('Ctrl Pts',(50.0359174318355,-55.0283227416369,
-171.980270642));
#161361=CARTESIAN_POINT('Ctrl Pts',(50.0306737152842,-55.0286806168088,
-171.974562666534));
#161362=CARTESIAN_POINT('Ctrl Pts',(50.0250757653012,-55.0290626678437,
-171.968608245928));
#161363=CARTESIAN_POINT('Ctrl Pts',(50.0194929266255,-55.0294436801627,
-171.962815606048));
#161364=CARTESIAN_POINT('Ctrl Pts',(50.0137424541554,-55.0298361329952,
-171.956849032751));
#161365=CARTESIAN_POINT('Ctrl Pts',(50.008008174688,-55.0302274728359,-171.951054248133));
#161366=CARTESIAN_POINT('Ctrl Pts',(50.002735256722,-55.0305873095219,-171.945838282879));
#161367=CARTESIAN_POINT('Ctrl Pts',(50.0017027010506,-55.0306577736204,
-171.944816879826));
#161368=CARTESIAN_POINT('Ctrl Pts',(50.0006879511706,-55.0307270218896,
-171.943817557218));
#161369=CARTESIAN_POINT('Ctrl Pts',(49.9996945037156,-55.0307948156288,
-171.942843213006));
#161370=CARTESIAN_POINT('Ctrl Pts',(49.9775385427164,-55.0323067581414,
-171.921113294381));
#161371=CARTESIAN_POINT('Ctrl Pts',(49.9536976238303,-55.0339338834397,
-171.899758993455));
#161372=CARTESIAN_POINT('Ctrl Pts',(49.9281170980912,-55.0356797757925,
-171.879051282674));
#161373=CARTESIAN_POINT('Ctrl Pts',(49.9029338030088,-55.0373985568197,
-171.858665134382));
#161374=CARTESIAN_POINT('Ctrl Pts',(49.8760642222839,-55.0392324645958,
-171.838905512263));
#161375=CARTESIAN_POINT('Ctrl Pts',(49.8474888776852,-55.0411826856386,
-171.820067900575));
#161376=CARTESIAN_POINT('Ctrl Pts',(49.8203035381361,-55.0430380410853,
-171.802146616433));
#161377=CARTESIAN_POINT('Ctrl Pts',(49.7915729570549,-55.0449988567668,
-171.785058883054));
#161378=CARTESIAN_POINT('Ctrl Pts',(49.7613085510039,-55.0470643535212,
-171.769091901678));
#161379=CARTESIAN_POINT('Ctrl Pts',(49.731938617721,-55.0490688039563,-171.753596828788));
#161380=CARTESIAN_POINT('Ctrl Pts',(49.7011235740018,-55.0511718808408,
-171.739157140893));
#161381=CARTESIAN_POINT('Ctrl Pts',(49.6689100752976,-55.0533704000159,
-171.726070467489));
#161382=CARTESIAN_POINT('Ctrl Pts',(49.6683799863872,-55.0534065777265,
-171.725855119864));
#161383=CARTESIAN_POINT('Ctrl Pts',(49.6678495213746,-55.0534427811054,
-171.725640139907));
#161384=CARTESIAN_POINT('Ctrl Pts',(49.6673186805243,-55.0534790101347,
-171.725425528679));
#161385=CARTESIAN_POINT('Ctrl Pts',(49.6646555879062,-55.0536607618979,
-171.724348879102));
#161386=CARTESIAN_POINT('Ctrl Pts',(49.6612679260877,-55.0538919407015,
-171.722996951244));
#161387=CARTESIAN_POINT('Ctrl Pts',(49.6584523482381,-55.0540840712475,
-171.721889199757));
#161388=CARTESIAN_POINT('Ctrl Pts',(49.6566137537786,-55.0542095340037,
-171.721165829331));
#161389=CARTESIAN_POINT('Ctrl Pts',(49.6550196708291,-55.0543183073482,
-171.720545222463));
#161390=CARTESIAN_POINT('Ctrl Pts',(49.6540347939841,-55.0543855068274,
-171.720163007342));
#161391=CARTESIAN_POINT('Ctrl Pts',(49.6382987468942,-55.0554591986035,
-171.714056096449));
#161392=CARTESIAN_POINT('Ctrl Pts',(49.620874316751,-55.0566482285285,-171.707738814429));
#161393=CARTESIAN_POINT('Ctrl Pts',(49.6016963861777,-55.0579570088307,
-171.701466818893));
#161394=CARTESIAN_POINT('Ctrl Pts',(49.5821836919874,-55.0592886347693,
-171.695085341476));
#161395=CARTESIAN_POINT('Ctrl Pts',(49.5608547090479,-55.0607442990113,
-171.68875040177));
#161396=CARTESIAN_POINT('Ctrl Pts',(49.5376610747394,-55.0623272682998,
-171.682785652347));
#161397=CARTESIAN_POINT('Ctrl Pts',(49.5167527758563,-55.0637542630763,
-171.677408626822));
#161398=CARTESIAN_POINT('Ctrl Pts',(49.4943288267278,-55.0652847355981,
-171.672333011424));
#161399=CARTESIAN_POINT('Ctrl Pts',(49.4703789307845,-55.0669193633298,
-171.667836203527));
#161400=CARTESIAN_POINT('Ctrl Pts',(49.4472084654267,-55.0685007933835,
-171.663485740716));
#161401=CARTESIAN_POINT('Ctrl Pts',(49.4226092365823,-55.0701797452918,
-171.659677091764));
#161402=CARTESIAN_POINT('Ctrl Pts',(49.3966032219418,-55.0719546957534,
-171.656697423783));
#161403=CARTESIAN_POINT('Ctrl Pts',(49.3718021780105,-55.0736474051124,
-171.653855816658));
#161404=CARTESIAN_POINT('Ctrl Pts',(49.3457213525921,-55.0754274463003,
-171.651768285729));
#161405=CARTESIAN_POINT('Ctrl Pts',(49.3184147391538,-55.0772911135977,
-171.650715593428));
#161406=CARTESIAN_POINT('Ctrl Pts',(49.3054566987733,-55.0781754955497,
-171.650216050364));
#161407=CARTESIAN_POINT('Ctrl Pts',(49.2922231788487,-55.0790786713351,
-171.64995));
#161408=CARTESIAN_POINT('Ctrl Pts',(49.2787232447289,-55.08000002,-171.64995));
#161409=CARTESIAN_POINT('',(49.3685531658572,-54.4408269190399,-171.64995));
#161410=CARTESIAN_POINT('Ctrl Pts',(50.7934646035069,-54.58000002,-176.84995));
#161411=CARTESIAN_POINT('Ctrl Pts',(50.3588212345988,-54.58000002,-176.84995));
#161412=CARTESIAN_POINT('Ctrl Pts',(50.2983305691361,-55.0104134695199,
-176.84995));
#161413=CARTESIAN_POINT('Ctrl Pts',(50.7934646035178,-54.58000002,-176.981217345763));
#161414=CARTESIAN_POINT('Ctrl Pts',(50.358821234607,-54.5800000199424,-176.997671841189));
#161415=CARTESIAN_POINT('Ctrl Pts',(50.2983305691453,-55.0104134694541,
-177.112484691526));
#161416=CARTESIAN_POINT('Ctrl Pts',(50.8086111287259,-54.5261134565302,
-177.110943344657));
#161417=CARTESIAN_POINT('Ctrl Pts',(50.3685899331079,-54.5104921183889,
-177.142957948483));
#161418=CARTESIAN_POINT('Ctrl Pts',(50.313477094355,-54.9026403425777,-177.371936689315));
#161419=CARTESIAN_POINT('Ctrl Pts',(50.8606449931892,-54.3409933646562,
-177.296063436531));
#161420=CARTESIAN_POINT('Ctrl Pts',(50.3994818369767,-54.2906848009584,
-177.329589659683));
#161421=CARTESIAN_POINT('Ctrl Pts',(50.3655109588186,-54.5324001588352,
-177.742176873059));
#161422=CARTESIAN_POINT('Ctrl Pts',(50.8971085935234,-54.2112673657634,
-177.34995));
#161423=CARTESIAN_POINT('Ctrl Pts',(50.420433990624,-54.1416024812641,-177.367861075731));
#161424=CARTESIAN_POINT('Ctrl Pts',(50.4019745591532,-54.2729481610447,
-177.849949999941));
#161425=CARTESIAN_POINT('Ctrl Pts',(50.9340054382093,-54.08000002,-177.34995));
#161426=CARTESIAN_POINT('Ctrl Pts',(50.4388714038384,-54.0104134695199,
-177.34995));
#161427=CARTESIAN_POINT('Ctrl Pts',(50.4388714038385,-54.0104134695199,
-177.84995));
#161428=CARTESIAN_POINT('',(50.7934646035069,-54.58000002,-176.84995));
#161429=CARTESIAN_POINT('',(50.2983305691361,-55.0104134695199,-176.84995));
#161430=CARTESIAN_POINT('Origin',(50.7934646035069,-55.08000002,-176.84995));
#161431=CARTESIAN_POINT('',(50.4388714038385,-54.0104134695199,-177.84995));
#161432=CARTESIAN_POINT('Ctrl Pts',(50.4388714038385,-54.0104134695199,
-177.84995));
#161433=CARTESIAN_POINT('Ctrl Pts',(50.4019745591532,-54.2729481610447,
-177.849949999941));
#161434=CARTESIAN_POINT('Ctrl Pts',(50.3655109588186,-54.5324001588352,
-177.742176873059));
#161435=CARTESIAN_POINT('Ctrl Pts',(50.3394940265868,-54.7175202507064,
-177.557056781187));
#161436=CARTESIAN_POINT('Ctrl Pts',(50.313477094355,-54.9026403425777,-177.371936689315));
#161437=CARTESIAN_POINT('Ctrl Pts',(50.2983305691453,-55.0104134694541,
-177.112484691526));
#161438=CARTESIAN_POINT('Ctrl Pts',(50.2983305691361,-55.0104134695199,
-176.84995));
#161439=CARTESIAN_POINT('Origin',(50.9340054382093,-54.0800000199999,-177.84995));
#161440=CARTESIAN_POINT('Ctrl Pts',(50.7934646035069,-54.58000002,-176.84995));
#161441=CARTESIAN_POINT('Ctrl Pts',(50.7934646035069,-54.58000002,-176.875800002307));
#161442=CARTESIAN_POINT('Ctrl Pts',(50.7940526302635,-54.5779080061136,
-176.901947474016));
#161443=CARTESIAN_POINT('Ctrl Pts',(50.79524037118,-54.5736823982397,-176.928073316629));
#161444=CARTESIAN_POINT('Ctrl Pts',(50.7964380905779,-54.5694212900735,
-176.954418648383));
#161445=CARTESIAN_POINT('Ctrl Pts',(50.7982456556932,-54.5629905430313,
-176.980741922991));
#161446=CARTESIAN_POINT('Ctrl Pts',(50.8006670611674,-54.5543759454336,
-177.00667179537));
#161447=CARTESIAN_POINT('Ctrl Pts',(50.8015905093901,-54.5510906076722,
-177.016560636713));
#161448=CARTESIAN_POINT('Ctrl Pts',(50.8026031526618,-54.5474879420343,
-177.026391811967));
#161449=CARTESIAN_POINT('Ctrl Pts',(50.8037049055093,-54.5435682526075,
-177.036143091591));
#161450=CARTESIAN_POINT('Ctrl Pts',(50.8065619552914,-54.5334037698481,
-177.06142997094));
#161451=CARTESIAN_POINT('Ctrl Pts',(50.810020166567,-54.5211005439435,-177.086198360269));
#161452=CARTESIAN_POINT('Ctrl Pts',(50.8140793605825,-54.506659210843,-177.110048753582));
#161453=CARTESIAN_POINT('Ctrl Pts',(50.8173767403582,-54.4949281727313,
-177.129422994933));
#161454=CARTESIAN_POINT('Ctrl Pts',(50.8210711306239,-54.4817846964092,
-177.148192204817));
#161455=CARTESIAN_POINT('Ctrl Pts',(50.825157442334,-54.4672468870987,-177.166105768384));
#161456=CARTESIAN_POINT('Ctrl Pts',(50.827356904925,-54.4594218923349,-177.175747767266));
#161457=CARTESIAN_POINT('Ctrl Pts',(50.8296698422141,-54.4511931903559,
-177.18514138209));
#161458=CARTESIAN_POINT('Ctrl Pts',(50.8320942102929,-54.4425680527437,
-177.194242926223));
#161459=CARTESIAN_POINT('Ctrl Pts',(50.8325766062305,-54.4408518400193,
-177.19605393337));
#161460=CARTESIAN_POINT('Ctrl Pts',(50.8331640063325,-54.4387620555821,
-177.198223909681));
#161461=CARTESIAN_POINT('Ctrl Pts',(50.8336822024932,-54.436918446991,-177.200104635539));
#161462=CARTESIAN_POINT('Ctrl Pts',(50.834057272349,-54.4355840449617,-177.201465903008));
#161463=CARTESIAN_POINT('Ctrl Pts',(50.8343957120667,-54.4343799457124,
-177.202676855488));
#161464=CARTESIAN_POINT('Ctrl Pts',(50.8346280186497,-54.4335534076203,
-177.203503393566));
#161465=CARTESIAN_POINT('Ctrl Pts',(50.8373709918346,-54.4237940121101,
-177.213262788913));
#161466=CARTESIAN_POINT('Ctrl Pts',(50.8404332490898,-54.4128991858337,
-177.22331664328));
#161467=CARTESIAN_POINT('Ctrl Pts',(50.8438503785376,-54.4007420960308,
-177.233428698371));
#161468=CARTESIAN_POINT('Ctrl Pts',(50.8471205406303,-54.3891078706266,
-177.243105843982));
#161469=CARTESIAN_POINT('Ctrl Pts',(50.8507159048646,-54.3763169166589,
-177.252836300725));
#161470=CARTESIAN_POINT('Ctrl Pts',(50.8546612358606,-54.3622809307141,
-177.262372868916));
#161471=CARTESIAN_POINT('Ctrl Pts',(50.8583802330195,-54.349050154411,-177.271362347884));
#161472=CARTESIAN_POINT('Ctrl Pts',(50.8624103177822,-54.3347126616006,
-177.280179445045));
#161473=CARTESIAN_POINT('Ctrl Pts',(50.8667641905032,-54.3192230962442,
-177.288581471767));
#161474=CARTESIAN_POINT('Ctrl Pts',(50.8685409822056,-54.3129018891342,
-177.29201029303));
#161475=CARTESIAN_POINT('Ctrl Pts',(50.8703715911811,-54.3063891942303,
-177.295369566868));
#161476=CARTESIAN_POINT('Ctrl Pts',(50.8722563916222,-54.2996836682345,
-177.298640995834));
#161477=CARTESIAN_POINT('Ctrl Pts',(50.8765268222964,-54.2844908216743,
-177.306053138943));
#161478=CARTESIAN_POINT('Ctrl Pts',(50.8810786182863,-54.2682969659899,
-177.313020714078));
#161479=CARTESIAN_POINT('Ctrl Pts',(50.8859100008748,-54.2511084292962,
-177.319306663922));
#161480=CARTESIAN_POINT('Ctrl Pts',(50.8906033966449,-54.2344108062172,
-177.325413083744));
#161481=CARTESIAN_POINT('Ctrl Pts',(50.8955607238668,-54.2167741982081,
-177.330876292405));
#161482=CARTESIAN_POINT('Ctrl Pts',(50.9007703992126,-54.1982398150987,
-177.335449266095));
#161483=CARTESIAN_POINT('Ctrl Pts',(50.9058588558212,-54.1801366900557,
-177.339915835823));
#161484=CARTESIAN_POINT('Ctrl Pts',(50.9111881361125,-54.1611767902422,
-177.343533167656));
#161485=CARTESIAN_POINT('Ctrl Pts',(50.9167365713841,-54.1414372060732,
-177.34604166628));
#161486=CARTESIAN_POINT('Ctrl Pts',(50.9222850066558,-54.1216976219043,
-177.348550164905));
#161487=CARTESIAN_POINT('Ctrl Pts',(50.9280527228745,-54.1011779052295,
-177.34995));
#161488=CARTESIAN_POINT('Ctrl Pts',(50.9340054382093,-54.08000002,-177.34995));
#161489=CARTESIAN_POINT('Origin',(53.1076143453209,-38.6139690140329,-177.84995));
#161490=CARTESIAN_POINT('',(50.5091418211897,-53.5104134695199,-177.84995));
#161491=CARTESIAN_POINT('',(52.6124803109501,-38.5443824635529,-177.84995));
#161492=CARTESIAN_POINT('Origin',(51.0042758555605,-53.58000002,-177.84995));
#161493=CARTESIAN_POINT('Ctrl Pts',(51.0043131058742,-53.5800399704537,
-177.349950000614));
#161494=CARTESIAN_POINT('Ctrl Pts',(50.5091370017856,-53.5104477613619,
-177.349907583593));
#161495=CARTESIAN_POINT('Ctrl Pts',(50.5091324341781,-53.5104802615782,
-177.849949997675));
#161496=CARTESIAN_POINT('Ctrl Pts',(51.0412139300136,-53.4487616698901,
-177.349960874823));
#161497=CARTESIAN_POINT('Ctrl Pts',(50.5284341404524,-53.3731414851579,
-177.331166751555));
#161498=CARTESIAN_POINT('Ctrl Pts',(50.5460324812801,-53.247922783674,-177.849968278574));
#161499=CARTESIAN_POINT('Ctrl Pts',(51.0776824759844,-53.3190198513573,
-177.296074808575));
#161500=CARTESIAN_POINT('Ctrl Pts',(50.5442915570248,-53.2603101034141,
-177.25721607327));
#161501=CARTESIAN_POINT('Ctrl Pts',(50.582500059869,-52.9884424791336,-177.742192571987));
#161502=CARTESIAN_POINT('Ctrl Pts',(51.1297221567416,-53.1338805435418,
-177.110939115584));
#161503=CARTESIAN_POINT('Ctrl Pts',(50.5649415669174,-53.1133776482461,
-177.069853325703));
#161504=CARTESIAN_POINT('Ctrl Pts',(50.6345383370137,-52.6181708975332,
-177.371920990387));
#161505=CARTESIAN_POINT('Ctrl Pts',(51.1448695169889,-53.0799908778568,
-176.981197291836));
#161506=CARTESIAN_POINT('Ctrl Pts',(50.5696251595464,-53.0800521550443,
-176.95888267251));
#161507=CARTESIAN_POINT('Ctrl Pts',(50.6496852247771,-52.5103951909531,
-177.112440685846));
#161508=CARTESIAN_POINT('Ctrl Pts',(51.144866956159,-53.080000018636,-176.849916603474));
#161509=CARTESIAN_POINT('Ctrl Pts',(50.5696243593531,-53.0800578487393,
-176.849922286134));
#161510=CARTESIAN_POINT('Ctrl Pts',(50.6496826555653,-52.5104134718451,
-176.849883207942));
#161511=CARTESIAN_POINT('',(50.6496826558921,-52.51041346952,-176.84995));
#161512=CARTESIAN_POINT('Ctrl Pts',(50.6496826558921,-52.51041346952,-176.84995));
#161513=CARTESIAN_POINT('Ctrl Pts',(50.6496826558828,-52.5104134695858,
-177.112484691526));
#161514=CARTESIAN_POINT('Ctrl Pts',(50.6345361306733,-52.6181865964613,
-177.371936689314));
#161515=CARTESIAN_POINT('Ctrl Pts',(50.6085191984413,-52.8033066883334,
-177.557056781187));
#161516=CARTESIAN_POINT('Ctrl Pts',(50.5825022662094,-52.9884267802056,
-177.742176873059));
#161517=CARTESIAN_POINT('Ctrl Pts',(50.546038665875,-53.2478787779945,-177.849949999941));
#161518=CARTESIAN_POINT('Ctrl Pts',(50.5091418211897,-53.5104134695199,
-177.84995));
#161519=CARTESIAN_POINT('',(51.1448166902628,-53.08000002,-176.84995));
#161520=CARTESIAN_POINT('Origin',(51.1448166902628,-52.58000002,-176.84995));
#161521=CARTESIAN_POINT('Ctrl Pts',(51.0042758555605,-53.58000002,-177.34995));
#161522=CARTESIAN_POINT('Ctrl Pts',(51.0103430173925,-53.5584149702,-177.34995));
#161523=CARTESIAN_POINT('Ctrl Pts',(51.016169374502,-53.5374879725988,-177.348552025671));
#161524=CARTESIAN_POINT('Ctrl Pts',(51.021754926889,-53.517368300209,-177.346011757925));
#161525=CARTESIAN_POINT('Ctrl Pts',(51.0273316159915,-53.4972805541836,
-177.343475521136));
#161526=CARTESIAN_POINT('Ctrl Pts',(51.0326682639943,-53.4779969954851,
-177.339801327605));
#161527=CARTESIAN_POINT('Ctrl Pts',(51.0377648708973,-53.459608680057,-177.335239527258));
#161528=CARTESIAN_POINT('Ctrl Pts',(51.0430846624452,-53.4404151250393,
-177.33047796189));
#161529=CARTESIAN_POINT('Ctrl Pts',(51.048142929384,-53.4221966220856,-177.324750042966));
#161530=CARTESIAN_POINT('Ctrl Pts',(51.0529396717135,-53.4050003525822,
-177.318324974143));
#161531=CARTESIAN_POINT('Ctrl Pts',(51.0573558439112,-53.3891684228957,
-177.31240966572));
#161532=CARTESIAN_POINT('Ctrl Pts',(51.0615503436285,-53.3742018844323,
-177.305903491103));
#161533=CARTESIAN_POINT('Ctrl Pts',(51.0655231708653,-53.3601026376805,
-177.298999152375));
#161534=CARTESIAN_POINT('Ctrl Pts',(51.070152181175,-53.3436746495795,-177.290954439316));
#161535=CARTESIAN_POINT('Ctrl Pts',(51.0744802453861,-53.3284243291718,
-177.282370206816));
#161536=CARTESIAN_POINT('Ctrl Pts',(51.0785073634984,-53.31431086582,-177.273517318559));
#161537=CARTESIAN_POINT('Ctrl Pts',(51.0816848890195,-53.3031748899829,
-177.266532105414));
#161538=CARTESIAN_POINT('Ctrl Pts',(51.0846750540229,-53.2927456090393,
-177.259378907547));
#161539=CARTESIAN_POINT('Ctrl Pts',(51.0874778585085,-53.28298799345,-177.252173639391));
#161540=CARTESIAN_POINT('Ctrl Pts',(51.0906553636708,-53.2719259040087,
-177.244005115015));
#161541=CARTESIAN_POINT('Ctrl Pts',(51.0935920641105,-53.261726951001,-177.235770093483));
#161542=CARTESIAN_POINT('Ctrl Pts',(51.0962879598278,-53.2523265017848,
-177.227613958382));
#161543=CARTESIAN_POINT('Ctrl Pts',(51.0976359076864,-53.2476262771767,
-177.223535890831));
#161544=CARTESIAN_POINT('Ctrl Pts',(51.0989236543645,-53.2431254933336,
-177.219477157756));
#161545=CARTESIAN_POINT('Ctrl Pts',(51.1001511998619,-53.2388152125502,
-177.215453662315));
#161546=CARTESIAN_POINT('Ctrl Pts',(51.1007649726106,-53.2366600721585,
-177.213441914594));
#161547=CARTESIAN_POINT('Ctrl Pts',(51.1013636950641,-53.2345525658363,
-177.211438967526));
#161548=CARTESIAN_POINT('Ctrl Pts',(51.1019473672225,-53.2324915202267,
-177.209446651703));
#161549=CARTESIAN_POINT('Ctrl Pts',(51.1023096848787,-53.2312121149924,
-177.208209910855));
#161550=CARTESIAN_POINT('Ctrl Pts',(51.10254906038,-53.2303718707492,-177.20738941522));
#161551=CARTESIAN_POINT('Ctrl Pts',(51.1028836446522,-53.2291841923715,
-177.206219918861));
#161552=CARTESIAN_POINT('Ctrl Pts',(51.103088055709,-53.2284585916408,-177.20550542626));
#161553=CARTESIAN_POINT('Ctrl Pts',(51.1033280032683,-53.227603597789,-177.204660358976));
#161554=CARTESIAN_POINT('Ctrl Pts',(51.1036532328122,-53.2264466294068,
-177.203503390593));
#161555=CARTESIAN_POINT('Ctrl Pts',(51.108701271955,-53.2084887845862,-177.185545545773));
#161556=CARTESIAN_POINT('Ctrl Pts',(51.1132850152011,-53.1920748638293,
-177.166390617213));
#161557=CARTESIAN_POINT('Ctrl Pts',(51.1174044625504,-53.177308366338,-177.146327178728));
#161558=CARTESIAN_POINT('Ctrl Pts',(51.1215821478003,-53.1623331103072,
-177.125980097212));
#161559=CARTESIAN_POINT('Ctrl Pts',(51.1252823165684,-53.1490520483592,
-177.104699239602));
#161560=CARTESIAN_POINT('Ctrl Pts',(51.1285049688547,-53.1375196153263,
-177.08278275431));
#161561=CARTESIAN_POINT('Ctrl Pts',(51.1317983348823,-53.1257341293998,
-177.060385361824));
#161562=CARTESIAN_POINT('Ctrl Pts',(51.1345929984958,-53.1157746706807,
-177.037324735901));
#161563=CARTESIAN_POINT('Ctrl Pts',(51.1368889596953,-53.1076461996327,
-177.013906910145));
#161564=CARTESIAN_POINT('Ctrl Pts',(51.1392139480793,-53.0994149626366,
-176.990193019477));
#161565=CARTESIAN_POINT('Ctrl Pts',(51.1410275444319,-53.0930609412306,
-176.966113358338));
#161566=CARTESIAN_POINT('Ctrl Pts',(51.1423297487532,-53.0885396784593,
-176.941964850392));
#161567=CARTESIAN_POINT('Ctrl Pts',(51.1436564554925,-53.0839333431161,
-176.917361961496));
#161568=CARTESIAN_POINT('Ctrl Pts',(51.144452344328,-53.0812289800571,-176.892688085413));
#161569=CARTESIAN_POINT('Ctrl Pts',(51.1447174152596,-53.0803342185763,
-176.868228043868));
#161570=CARTESIAN_POINT('Ctrl Pts',(51.1447835985951,-53.0801108130943,
-176.862120821453));
#161571=CARTESIAN_POINT('Ctrl Pts',(51.1448166902628,-53.08000002,-176.856026770997));
#161572=CARTESIAN_POINT('Ctrl Pts',(51.1448166902628,-53.08000002,-176.84995));
#161573=CARTESIAN_POINT('Origin',(51.6222122422086,-38.4052093625928,-172.64995));
#161574=CARTESIAN_POINT('',(51.4437383719606,-46.86041346952,-172.64995));
#161575=CARTESIAN_POINT('',(50.6496826558921,-52.51041346952,-172.64995));
#161576=CARTESIAN_POINT('',(50.5696324866523,-53.08000002,-172.64995));
#161577=CARTESIAN_POINT('Ctrl Pts',(51.4437383719606,-46.86041346952,-172.64995));
#161578=CARTESIAN_POINT('Ctrl Pts',(51.4437383719606,-46.86041346952,-172.605172304724));
#161579=CARTESIAN_POINT('Ctrl Pts',(51.4406334881656,-46.8606253728163,
-172.559925284512));
#161580=CARTESIAN_POINT('Ctrl Pts',(51.4343094493851,-46.8610569782327,
-172.514629909038));
#161581=CARTESIAN_POINT('Ctrl Pts',(51.428060212732,-46.861483478525,-172.469870297268));
#161582=CARTESIAN_POINT('Ctrl Pts',(51.4186675071001,-46.8621245154899,
-172.425063433886));
#161583=CARTESIAN_POINT('Ctrl Pts',(51.4060290328097,-46.862987070915,-172.380665524099));
#161584=CARTESIAN_POINT('Ctrl Pts',(51.396118867739,-46.8636634236495,-172.345851937849));
#161585=CARTESIAN_POINT('Ctrl Pts',(51.384213177772,-46.86447596773,-172.311290758975));
#161586=CARTESIAN_POINT('Ctrl Pts',(51.3702662438672,-46.8654278234071,
-172.277224099813));
#161587=CARTESIAN_POINT('Ctrl Pts',(51.3689054040442,-46.8655206985236,
-172.273900124325));
#161588=CARTESIAN_POINT('Ctrl Pts',(51.3675251317413,-46.8656148998754,
-172.270580868761));
#161589=CARTESIAN_POINT('Ctrl Pts',(51.3661253857718,-46.8657104302735,
-172.267266567635));
#161590=CARTESIAN_POINT('Ctrl Pts',(51.3480973882623,-46.8669408119397,
-172.224580098984));
#161591=CARTESIAN_POINT('Ctrl Pts',(51.3268418537189,-46.8683914677873,
-172.182726614337));
#161592=CARTESIAN_POINT('Ctrl Pts',(51.3024472277073,-46.8700563615496,
-172.142169045356));
#161593=CARTESIAN_POINT('Ctrl Pts',(51.2790331840628,-46.8716543321515,
-172.103241754985));
#161594=CARTESIAN_POINT('Ctrl Pts',(51.2527284521908,-46.8734495875488,
-172.065509332455));
#161595=CARTESIAN_POINT('Ctrl Pts',(51.2236286892016,-46.8754355992983,
-172.029413466109));
#161596=CARTESIAN_POINT('Ctrl Pts',(51.2101252591521,-46.8763571865548,
-172.01266357002));
#161597=CARTESIAN_POINT('Ctrl Pts',(51.1960201863762,-46.8773198349542,
-171.996266629397));
#161598=CARTESIAN_POINT('Ctrl Pts',(51.1813252346626,-46.8783227416367,
-171.980270642003));
#161599=CARTESIAN_POINT('Ctrl Pts',(51.1760815181382,-46.8786806168068,
-171.974562666566));
#161600=CARTESIAN_POINT('Ctrl Pts',(51.1704835681801,-46.87906266784,-171.968608245986));
#161601=CARTESIAN_POINT('Ctrl Pts',(51.1649007295291,-46.8794436801573,
-171.96281560613));
#161602=CARTESIAN_POINT('Ctrl Pts',(51.1591502570813,-46.8798361329882,
-171.956849032855));
#161603=CARTESIAN_POINT('Ctrl Pts',(51.1534159776358,-46.8802274728275,
-171.951054248257));
#161604=CARTESIAN_POINT('Ctrl Pts',(51.1481430596939,-46.8805873095117,
-171.945838283025));
#161605=CARTESIAN_POINT('Ctrl Pts',(51.1471105039711,-46.8806577736137,
-171.944816879921));
#161606=CARTESIAN_POINT('Ctrl Pts',(51.1460957540418,-46.8807270218863,
-171.943817557264));
#161607=CARTESIAN_POINT('Ctrl Pts',(51.1451023065401,-46.8807948156287,
-171.942843213006));
#161608=CARTESIAN_POINT('Ctrl Pts',(51.1229463457133,-46.8823067581293,
-171.92111329455));
#161609=CARTESIAN_POINT('Ctrl Pts',(51.0991054270076,-46.8839338834152,
-171.89975899377));
#161610=CARTESIAN_POINT('Ctrl Pts',(51.0735249014539,-46.8856797757556,
-171.879051283109));
#161611=CARTESIAN_POINT('Ctrl Pts',(51.0483416062908,-46.8873985567883,
-171.858665134724));
#161612=CARTESIAN_POINT('Ctrl Pts',(51.0214720254546,-46.8892324645722,
-171.8389055125));
#161613=CARTESIAN_POINT('Ctrl Pts',(50.9928966807099,-46.8911826856249,
-171.820067900707));
#161614=CARTESIAN_POINT('Ctrl Pts',(50.9657113411477,-46.8930380410725,
-171.802146616547));
#161615=CARTESIAN_POINT('Ctrl Pts',(50.9369807600363,-46.8949988567561,
-171.785058883141));
#161616=CARTESIAN_POINT('Ctrl Pts',(50.9067163539354,-46.8970643535139,
-171.769091901735));
#161617=CARTESIAN_POINT('Ctrl Pts',(50.877346420633,-46.8990688039503,-171.75359682883));
#161618=CARTESIAN_POINT('Ctrl Pts',(50.8465313768786,-46.9011718808373,
-171.739157140914));
#161619=CARTESIAN_POINT('Ctrl Pts',(50.8143178781222,-46.9033704000159,
-171.726070467489));
#161620=CARTESIAN_POINT('Ctrl Pts',(50.8137877892207,-46.9034065777259,
-171.725855119867));
#161621=CARTESIAN_POINT('Ctrl Pts',(50.8132573242171,-46.9034427811042,
-171.725640139914));
#161622=CARTESIAN_POINT('Ctrl Pts',(50.8127264833758,-46.9034790101329,
-171.72542552869));
#161623=CARTESIAN_POINT('Ctrl Pts',(50.8100633907649,-46.9036607618955,
-171.724348879115));
#161624=CARTESIAN_POINT('Ctrl Pts',(50.8066757289513,-46.903891940699,-171.722996951259));
#161625=CARTESIAN_POINT('Ctrl Pts',(50.8038601511023,-46.9040840712449,
-171.721889199772));
#161626=CARTESIAN_POINT('Ctrl Pts',(50.8020215566215,-46.9042095340026,
-171.721165829338));
#161627=CARTESIAN_POINT('Ctrl Pts',(50.8004274736547,-46.9043183073482,
-171.720545222463));
#161628=CARTESIAN_POINT('Ctrl Pts',(50.7994425968086,-46.9043855068274,
-171.720163007342));
#161629=CARTESIAN_POINT('Ctrl Pts',(50.7837065498889,-46.9054591985905,
-171.714056096515));
#161630=CARTESIAN_POINT('Ctrl Pts',(50.7662821199151,-46.906648228503,-171.707738814551));
#161631=CARTESIAN_POINT('Ctrl Pts',(50.7471041895102,-46.9079570087933,
-171.701466819059));
#161632=CARTESIAN_POINT('Ctrl Pts',(50.7275914953754,-46.9092886347276,
-171.695085341649));
#161633=CARTESIAN_POINT('Ctrl Pts',(50.7062625124688,-46.9107442989673,
-171.688750401938));
#161634=CARTESIAN_POINT('Ctrl Pts',(50.6830688781689,-46.9123272682553,
-171.682785652503));
#161635=CARTESIAN_POINT('Ctrl Pts',(50.6621605794063,-46.9137542630237,
-171.677408626996));
#161636=CARTESIAN_POINT('Ctrl Pts',(50.6397366303949,-46.9152847355379,
-171.672333011606));
#161637=CARTESIAN_POINT('Ctrl Pts',(50.6157867345646,-46.9169193632623,
-171.667836203706));
#161638=CARTESIAN_POINT('Ctrl Pts',(50.5926162693159,-46.9185007933089,
-171.663485740894));
#161639=CARTESIAN_POINT('Ctrl Pts',(50.5680170405766,-46.9201797452105,
-171.65967709193));
#161640=CARTESIAN_POINT('Ctrl Pts',(50.5420110260361,-46.9219546956657,
-171.656697423928));
#161641=CARTESIAN_POINT('Ctrl Pts',(50.5172099822075,-46.9236474050181,
-171.653855816784));
#161642=CARTESIAN_POINT('Ctrl Pts',(50.4911291568878,-46.9254274461996,
-171.651768285827));
#161643=CARTESIAN_POINT('Ctrl Pts',(50.4638225435433,-46.9272911134907,
-171.650715593488));
#161644=CARTESIAN_POINT('Ctrl Pts',(50.4508645026649,-46.9281754954768,
-171.650216050385));
#161645=CARTESIAN_POINT('Ctrl Pts',(50.4376309822184,-46.9290786712979,
-171.64995));
#161646=CARTESIAN_POINT('Ctrl Pts',(50.4241310475534,-46.93000002,-171.64995));
#161647=CARTESIAN_POINT('Ctrl Pts',(49.6300753314849,-52.58000002,-171.64995));
#161648=CARTESIAN_POINT('Ctrl Pts',(49.6592062683373,-52.5780118806847,
-171.64995));
#161649=CARTESIAN_POINT('Ctrl Pts',(49.6870949010184,-52.576125534458,-171.651172745865));
#161650=CARTESIAN_POINT('Ctrl Pts',(49.7136621873133,-52.5743298726611,
-171.653316375876));
#161651=CARTESIAN_POINT('Ctrl Pts',(49.7414106383736,-52.572454376875,-171.655555310323));
#161652=CARTESIAN_POINT('Ctrl Pts',(49.7677180801388,-52.5706778703431,
-171.658798248614));
#161653=CARTESIAN_POINT('Ctrl Pts',(49.7925438592604,-52.5689946396099,
-171.662728774848));
#161654=CARTESIAN_POINT('Ctrl Pts',(49.8179907629401,-52.567269295558,-171.666757640246));
#161655=CARTESIAN_POINT('Ctrl Pts',(49.8418816270552,-52.565642050202,-171.671508529278));
#161656=CARTESIAN_POINT('Ctrl Pts',(49.8642143969623,-52.5641126147803,
-171.676676564475));
#161657=CARTESIAN_POINT('Ctrl Pts',(49.887281660145,-52.5625328783868,-171.682014569053));
#161658=CARTESIAN_POINT('Ctrl Pts',(49.9086873792323,-52.5610575929236,
-171.687797263142));
#161659=CARTESIAN_POINT('Ctrl Pts',(49.9284623174369,-52.5596910818783,
-171.693732405879));
#161660=CARTESIAN_POINT('Ctrl Pts',(49.9314331716388,-52.559485786416,-171.694624061952));
#161661=CARTESIAN_POINT('Ctrl Pts',(49.9343672660957,-52.5592829526098,
-171.69551924186));
#161662=CARTESIAN_POINT('Ctrl Pts',(49.9372647511473,-52.5590826015885,
-171.696417042859));
#161663=CARTESIAN_POINT('Ctrl Pts',(49.9500171622246,-52.5582008166826,
-171.700368444576));
#161664=CARTESIAN_POINT('Ctrl Pts',(49.9620601971446,-52.5573670921872,
-171.704369938142));
#161665=CARTESIAN_POINT('Ctrl Pts',(49.9734086898205,-52.5565835128729,
-171.708349867204));
#161666=CARTESIAN_POINT('Ctrl Pts',(49.9790829361585,-52.5561917232158,
-171.710339831735));
#161667=CARTESIAN_POINT('Ctrl Pts',(49.9845835094961,-52.5558124645922,
-171.7123245089));
#161668=CARTESIAN_POINT('Ctrl Pts',(49.9899125815189,-52.5554460422126,
-171.714295777019));
#161669=CARTESIAN_POINT('Ctrl Pts',(49.9925771175304,-52.5552628310228,
-171.715281411079));
#161670=CARTESIAN_POINT('Ctrl Pts',(49.995198775861,-52.5550828285634,-171.716263699745));
#161671=CARTESIAN_POINT('Ctrl Pts',(49.9977778228351,-52.554906072264,-171.717241672092));
#161672=CARTESIAN_POINT('Ctrl Pts',(49.9995468585359,-52.5547848305001,
-171.717912488876));
#161673=CARTESIAN_POINT('Ctrl Pts',(50.0003731303544,-52.5547277477509,
-171.718227889232));
#161674=CARTESIAN_POINT('Ctrl Pts',(50.0021560446491,-52.5546060349271,
-171.718913272988));
#161675=CARTESIAN_POINT('Ctrl Pts',(50.0029724106939,-52.554550304701,-171.719227098519));
#161676=CARTESIAN_POINT('Ctrl Pts',(50.0039892197234,-52.5544810069693,
-171.719618819411));
#161677=CARTESIAN_POINT('Ctrl Pts',(50.0053873934298,-52.5543855789116,
-171.720161698938));
#161678=CARTESIAN_POINT('Ctrl Pts',(50.0390970047312,-52.5520848327899,
-171.733250385798));
#161679=CARTESIAN_POINT('Ctrl Pts',(50.0713392048815,-52.5498963013618,
-171.747810336266));
#161680=CARTESIAN_POINT('Ctrl Pts',(50.1020456307454,-52.5478103768153,
-171.763538020853));
#161681=CARTESIAN_POINT('Ctrl Pts',(50.1335563870302,-52.5456698131331,
-171.779677679638));
#161682=CARTESIAN_POINT('Ctrl Pts',(50.1634501719592,-52.5436373461994,
-171.797046561953));
#161683=CARTESIAN_POINT('Ctrl Pts',(50.1917037810275,-52.5417097148338,
-171.815335004119));
#161684=CARTESIAN_POINT('Ctrl Pts',(50.1940932268591,-52.541546692449,-171.816881682343));
#161685=CARTESIAN_POINT('Ctrl Pts',(50.1964709691268,-52.541384423744,-171.81843495061));
#161686=CARTESIAN_POINT('Ctrl Pts',(50.1988370086813,-52.5412229088385,
-171.81999462906));
#161687=CARTESIAN_POINT('Ctrl Pts',(50.2276398112107,-52.5392567194225,
-171.83898125602));
#161688=CARTESIAN_POINT('Ctrl Pts',(50.2547047352767,-52.5374017274936,
-171.858915411873));
#161689=CARTESIAN_POINT('Ctrl Pts',(50.2800576780874,-52.535661572667,-171.879488097075));
#161690=CARTESIAN_POINT('Ctrl Pts',(50.2927341494928,-52.5347914952537,
-171.889774439675));
#161691=CARTESIAN_POINT('Ctrl Pts',(50.3049833101608,-52.5339502233269,
-171.900220871814));
#161692=CARTESIAN_POINT('Ctrl Pts',(50.3168121152348,-52.5331387343682,
-171.910791641771));
#161693=CARTESIAN_POINT('Ctrl Pts',(50.3223288922278,-52.5327602681082,
-171.915721690083));
#161694=CARTESIAN_POINT('Ctrl Pts',(50.3274289643461,-52.5324082123672,
-171.920381836518));
#161695=CARTESIAN_POINT('Ctrl Pts',(50.3325737573137,-52.5320555671373,
-171.925178375207));
#161696=CARTESIAN_POINT('Ctrl Pts',(50.3375775319413,-52.5317125878833,
-171.929843441175));
#161697=CARTESIAN_POINT('Ctrl Pts',(50.3426237602553,-52.5313690722106,
-171.934637611929));
#161698=CARTESIAN_POINT('Ctrl Pts',(50.348104148547,-52.5309955692892,-171.939969076396));
#161699=CARTESIAN_POINT('Ctrl Pts',(50.3490708688542,-52.5309296847497,
-171.940909527089));
#161700=CARTESIAN_POINT('Ctrl Pts',(50.3500510063111,-52.530862854204,-171.941866786942));
#161701=CARTESIAN_POINT('Ctrl Pts',(50.3510465847208,-52.5307948982762,
-171.942843218813));
#161702=CARTESIAN_POINT('Ctrl Pts',(50.3818387641553,-52.5286930938358,
-171.973043216233));
#161703=CARTESIAN_POINT('Ctrl Pts',(50.4104020698678,-52.5267752596114,
-172.004935794585));
#161704=CARTESIAN_POINT('Ctrl Pts',(50.43660977222,-52.5250235849138,-172.03817789155));
#161705=CARTESIAN_POINT('Ctrl Pts',(50.4631285790983,-52.5232511165611,
-172.071814596431));
#161706=CARTESIAN_POINT('Ctrl Pts',(50.4872356273342,-52.5216487903698,
-172.10683253693));
#161707=CARTESIAN_POINT('Ctrl Pts',(50.508852831868,-52.5202056322005,-172.14287770852));
#161708=CARTESIAN_POINT('Ctrl Pts',(50.5307318008976,-52.518744998711,-172.179359354038));
#161709=CARTESIAN_POINT('Ctrl Pts',(50.5500604364366,-52.5174474358973,
-172.216892769679));
#161710=CARTESIAN_POINT('Ctrl Pts',(50.5668098649344,-52.5163088858466,
-172.255120022273));
#161711=CARTESIAN_POINT('Ctrl Pts',(50.583870938874,-52.5151491515546,-172.294058543854));
#161712=CARTESIAN_POINT('Ctrl Pts',(50.5982561304957,-52.5141544300228,
-172.333716479937));
#161713=CARTESIAN_POINT('Ctrl Pts',(50.6099858799555,-52.5133275939276,
-172.373732379297));
#161714=CARTESIAN_POINT('Ctrl Pts',(50.6218418428613,-52.5124918609815,
-172.414178854313));
#161715=CARTESIAN_POINT('Ctrl Pts',(50.6309852381434,-52.5118276918993,
-172.454990623381));
#161716=CARTESIAN_POINT('Ctrl Pts',(50.6374846521774,-52.5113447258674,
-172.495818301581));
#161717=CARTESIAN_POINT('Ctrl Pts',(50.6440871507285,-52.5108540997111,
-172.537293530694));
#161718=CARTESIAN_POINT('Ctrl Pts',(50.6479614840189,-52.5105505195319,
-172.578784792508));
#161719=CARTESIAN_POINT('Ctrl Pts',(50.6492231617337,-52.5104502191572,
-172.619956446583));
#161720=CARTESIAN_POINT('Ctrl Pts',(50.6495301605875,-52.5104258134792,
-172.629974575984));
#161721=CARTESIAN_POINT('Ctrl Pts',(50.6496826558921,-52.51041346952,-172.639973937106));
#161722=CARTESIAN_POINT('Ctrl Pts',(50.6496826558921,-52.51041346952,-172.64995));
#161723=CARTESIAN_POINT('Ctrl Pts',(52.5050296388285,-39.3089337226171,
-172.133326251627));
#161724=CARTESIAN_POINT('Ctrl Pts',(52.4864722882118,-39.4409761333229,
-171.679515584751));
#161725=CARTESIAN_POINT('Ctrl Pts',(52.1126146143194,-39.4738501833479,
-171.391638125813));
#161726=CARTESIAN_POINT('Ctrl Pts',(52.541270746464,-39.0510648426419,-172.04151129494));
#161727=CARTESIAN_POINT('Ctrl Pts',(52.5176461244299,-39.1701487854048,
-171.633412526629));
#161728=CARTESIAN_POINT('Ctrl Pts',(52.2029436074416,-39.18424163534,-171.345711176575));
#161729=CARTESIAN_POINT('Ctrl Pts',(52.5971684400779,-38.7973422647502,
-171.953442620307));
#161730=CARTESIAN_POINT('Ctrl Pts',(52.5724535929286,-38.8910154875477,
-171.580271166833));
#161731=CARTESIAN_POINT('Ctrl Pts',(52.3057718899875,-38.8932964873464,
-171.301698499895));
#161732=CARTESIAN_POINT('Ctrl Pts',(52.6743159902015,-38.5446760769969,
-171.890184412595));
#161733=CARTESIAN_POINT('Ctrl Pts',(52.6539547691069,-38.61136117722,-171.540761416572));
#161734=CARTESIAN_POINT('Ctrl Pts',(52.4226914394942,-38.5972250898729,
-171.270067206297));
#161735=CARTESIAN_POINT('',(52.6451353368861,-38.6439093768522,-171.916253407912));
#161736=CARTESIAN_POINT('Ctrl Pts',(52.6451215732066,-38.6439145871468,
-171.916241762849));
#161737=CARTESIAN_POINT('Ctrl Pts',(52.6327200436122,-38.6877262200968,
-171.928258148288));
#161738=CARTESIAN_POINT('Ctrl Pts',(52.6204218089369,-38.7334430503703,
-171.941450676397));
#161739=CARTESIAN_POINT('Ctrl Pts',(52.6083879533182,-38.7810797529306,
-171.955850381936));
#161740=CARTESIAN_POINT('Ctrl Pts',(52.5975991294693,-38.8237879263498,
-171.96876028309));
#161741=CARTESIAN_POINT('Ctrl Pts',(52.5870229477254,-38.8680394620078,
-171.982640380926));
#161742=CARTESIAN_POINT('Ctrl Pts',(52.5767804085671,-38.9138488166889,
-171.997474376372));
#161743=CARTESIAN_POINT('Ctrl Pts',(52.574859932475,-38.9224380706917,-172.000255750518));
#161744=CARTESIAN_POINT('Ctrl Pts',(52.5729511953933,-38.9310821107148,
-172.003070546334));
#161745=CARTESIAN_POINT('Ctrl Pts',(52.5710550072722,-38.9397810591365,
-172.005918494111));
#161746=CARTESIAN_POINT('Ctrl Pts',(52.5701661690904,-38.9438586912092,
-172.007253469632));
#161747=CARTESIAN_POINT('Ctrl Pts',(52.5692800882732,-38.9479483883608,
-172.008595728785));
#161748=CARTESIAN_POINT('Ctrl Pts',(52.5683968484763,-38.9520501640132,
-172.009945239696));
#161749=CARTESIAN_POINT('Ctrl Pts',(52.5682526090381,-38.9527200136028,
-172.010165624574));
#161750=CARTESIAN_POINT('Ctrl Pts',(52.5681091671282,-38.9533868184525,
-172.010385093187));
#161751=CARTESIAN_POINT('Ctrl Pts',(52.5679617607653,-38.9540727644232,
-172.010610953635));
#161752=CARTESIAN_POINT('Ctrl Pts',(52.567091942239,-38.9581204086464,-172.011943715654));
#161753=CARTESIAN_POINT('Ctrl Pts',(52.5661205622637,-38.9626690977524,
-172.013445117389));
#161754=CARTESIAN_POINT('Ctrl Pts',(52.5652406411583,-38.9668167293616,
-172.014817530366));
#161755=CARTESIAN_POINT('Ctrl Pts',(52.5648144293729,-38.9688257384223,
-172.015482292902));
#161756=CARTESIAN_POINT('Ctrl Pts',(52.5644095232376,-38.970740631272,-172.016116692328));
#161757=CARTESIAN_POINT('Ctrl Pts',(52.5640471013215,-38.9724587861977,
-172.016686420464));
#161758=CARTESIAN_POINT('Ctrl Pts',(52.5638603874838,-38.9733439514863,
-172.016979935072));
#161759=CARTESIAN_POINT('Ctrl Pts',(52.5636849424823,-38.9741768987548,
-172.01725628059));
#161760=CARTESIAN_POINT('Ctrl Pts',(52.563523628473,-38.9749435910523,-172.017510745119));
#161761=CARTESIAN_POINT('Ctrl Pts',(52.5634372349735,-38.9753542015808,
-172.017647026409));
#161762=CARTESIAN_POINT('Ctrl Pts',(52.5633560421201,-38.9757403405034,
-172.017775215173));
#161763=CARTESIAN_POINT('Ctrl Pts',(52.5632737953258,-38.9761317175597,
-172.017905169922));
#161764=CARTESIAN_POINT('Ctrl Pts',(52.5564953797729,-39.0083872765447,
-172.028615463309));
#161765=CARTESIAN_POINT('Ctrl Pts',(52.5494159142318,-39.0436596555478,
-172.040521990413));
#161766=CARTESIAN_POINT('Ctrl Pts',(52.5422310058208,-39.0819615094717,
-172.053670741783));
#161767=CARTESIAN_POINT('Ctrl Pts',(52.5357568450765,-39.1164744559038,
-172.065518788423));
#161768=CARTESIAN_POINT('Ctrl Pts',(52.5291975175797,-39.1534471810898,
-172.078375959746));
#161769=CARTESIAN_POINT('Ctrl Pts',(52.5227135897134,-39.192898939103,-172.092240973108));
#161770=CARTESIAN_POINT('Ctrl Pts',(52.5167076842734,-39.2294421476268,
-172.105083799384));
#161771=CARTESIAN_POINT('Ctrl Pts',(52.5107667105805,-39.2681123359778,
-172.118791679458));
#161772=CARTESIAN_POINT('Ctrl Pts',(52.5050296388285,-39.3089337226171,
-172.133326251627));
#161773=CARTESIAN_POINT('Ctrl Pts',(52.6451353368861,-38.6439093768522,
-171.916253407912));
#161774=CARTESIAN_POINT('Ctrl Pts',(52.6464058796499,-38.6394159797481,
-171.881371542694));
#161775=CARTESIAN_POINT('Ctrl Pts',(52.6459390342692,-38.6353252452434,
-171.84657946844));
#161776=CARTESIAN_POINT('Ctrl Pts',(52.6436236858027,-38.6316512514798,
-171.812021915484));
#161777=CARTESIAN_POINT('Ctrl Pts',(52.6416753037096,-38.6285595597699,
-171.782941490513));
#161778=CARTESIAN_POINT('Ctrl Pts',(52.6384182215079,-38.6257624918022,
-171.754024489139));
#161779=CARTESIAN_POINT('Ctrl Pts',(52.633815177568,-38.6232615998417,-171.725358956929));
#161780=CARTESIAN_POINT('Ctrl Pts',(52.6300898783601,-38.6212375976898,
-171.702159594543));
#161781=CARTESIAN_POINT('Ctrl Pts',(52.6254838305633,-38.6194078000763,
-171.67912846901));
#161782=CARTESIAN_POINT('Ctrl Pts',(52.6199955276943,-38.6177699986579,
-171.656318341932));
#161783=CARTESIAN_POINT('Ctrl Pts',(52.6170443172279,-38.6168893080686,
-171.644052713124));
#161784=CARTESIAN_POINT('Ctrl Pts',(52.6137814340186,-38.6160491681525,
-171.631632234766));
#161785=CARTESIAN_POINT('Ctrl Pts',(52.6102740456651,-38.6152700458307,
-171.619352410973));
#161786=CARTESIAN_POINT('Ctrl Pts',(52.6067346866106,-38.6144838216188,
-171.606960653589));
#161787=CARTESIAN_POINT('Ctrl Pts',(52.6029463207216,-38.6137596916157,
-171.594712118775));
#161788=CARTESIAN_POINT('Ctrl Pts',(52.5990294893407,-38.6131080795974,
-171.582899413039));
#161789=CARTESIAN_POINT('Ctrl Pts',(52.5979152610766,-38.6129227143219,
-171.5795390308));
#161790=CARTESIAN_POINT('Ctrl Pts',(52.5967909510326,-38.6127431551648,
-171.576213850961));
#161791=CARTESIAN_POINT('Ctrl Pts',(52.5956600639907,-38.6125694994672,
-171.572930455134));
#161792=CARTESIAN_POINT('Ctrl Pts',(52.5951960360173,-38.6124982446924,
-171.571583205183));
#161793=CARTESIAN_POINT('Ctrl Pts',(52.5947281719133,-38.612427569521,-171.57023506049));
#161794=CARTESIAN_POINT('Ctrl Pts',(52.5942564505892,-38.6123574779562,
-171.568886040307));
#161795=CARTESIAN_POINT('Ctrl Pts',(52.5844642885233,-38.610902491872,-171.540882590844));
#161796=CARTESIAN_POINT('Ctrl Pts',(52.5731590893685,-38.6097161264722,
-171.512940465127));
#161797=CARTESIAN_POINT('Ctrl Pts',(52.560232179002,-38.6088174063243,-171.485293111838));
#161798=CARTESIAN_POINT('Ctrl Pts',(52.5474861932036,-38.607931264631,-171.458032709902));
#161799=CARTESIAN_POINT('Ctrl Pts',(52.5331634401878,-38.6073246921442,
-171.431059045936));
#161800=CARTESIAN_POINT('Ctrl Pts',(52.5172023231265,-38.607001419367,-171.404574211142));
#161801=CARTESIAN_POINT('Ctrl Pts',(52.5014583125321,-38.606682543814,-171.378449628634));
#161802=CARTESIAN_POINT('Ctrl Pts',(52.4841201593532,-38.6066392012133,
-171.352800783014));
#161803=CARTESIAN_POINT('Ctrl Pts',(52.4651717697575,-38.606862192425,-171.327798354999));
#161804=CARTESIAN_POINT('Ctrl Pts',(52.4505678703726,-38.6070340561712,
-171.308528488224));
#161805=CARTESIAN_POINT('Ctrl Pts',(52.435008333388,-38.6073638509613,-171.28964214896));
#161806=CARTESIAN_POINT('Ctrl Pts',(52.418503743379,-38.6078427661477,-171.27120723903));
#161807=CARTESIAN_POINT('Ctrl Pts',(52.9938276306004,-37.7501447842495,
-177.831926349313));
#161808=CARTESIAN_POINT('Ctrl Pts',(53.0290644361633,-37.6768546791036,
-177.379478122309));
#161809=CARTESIAN_POINT('Ctrl Pts',(53.4403098198818,-37.8775685921338,
-177.340139197757));
#161810=CARTESIAN_POINT('Ctrl Pts',(52.8644526083797,-38.0038787899799,
-177.788318381118));
#161811=CARTESIAN_POINT('Ctrl Pts',(52.9387831734984,-37.8445082365119,
-177.396106921235));
#161812=CARTESIAN_POINT('Ctrl Pts',(53.3237240701773,-37.9919010307737,
-177.318314744026));
#161813=CARTESIAN_POINT('Ctrl Pts',(52.7697107392458,-38.2534999676582,
-177.654124612897));
#161814=CARTESIAN_POINT('Ctrl Pts',(52.8575871067054,-38.0208239861393,
-177.3297491457));
#161815=CARTESIAN_POINT('Ctrl Pts',(53.2386901038944,-38.1039031063401,
-177.251398738488));
#161816=CARTESIAN_POINT('Ctrl Pts',(52.6567775733111,-38.592091397267,-177.247773453598));
#161817=CARTESIAN_POINT('Ctrl Pts',(52.7597859066203,-38.2459774998252,
-177.093855210388));
#161818=CARTESIAN_POINT('Ctrl Pts',(53.1371100205879,-38.2560577153129,
-177.048553549081));
#161819=CARTESIAN_POINT('Ctrl Pts',(52.6371617173208,-38.6755874697231,
-176.979974147571));
#161820=CARTESIAN_POINT('Ctrl Pts',(52.7392639513461,-38.2994134985588,
-176.927419692177));
#161821=CARTESIAN_POINT('Ctrl Pts',(53.1194519999705,-38.2935777262418,
-176.914856994736));
#161822=CARTESIAN_POINT('Ctrl Pts',(52.6472666300096,-38.6354176228512,
-176.719388397061));
#161823=CARTESIAN_POINT('Ctrl Pts',(52.7494003756538,-38.2736022260138,
-176.771349933471));
#161824=CARTESIAN_POINT('Ctrl Pts',(53.1285467956633,-38.2755266296908,
-176.784773168118));
#161825=CARTESIAN_POINT('',(53.1262583325313,-38.28000002,-176.84995));
#161826=CARTESIAN_POINT('',(52.6451348158641,-38.6439112191758,-176.84995));
#161827=CARTESIAN_POINT('Origin',(53.1262583325313,-38.78000002,-176.84995));
#161828=CARTESIAN_POINT('',(52.9322463618642,-37.8758780299853,-177.801086692062));
#161829=CARTESIAN_POINT('Ctrl Pts',(52.9322463618642,-37.8758780299853,
-177.801086692062));
#161830=CARTESIAN_POINT('Ctrl Pts',(52.8821502360452,-37.9823362053254,
-177.769982861881));
#161831=CARTESIAN_POINT('Ctrl Pts',(52.8404306738594,-38.0806649492,-177.726394810699));
#161832=CARTESIAN_POINT('Ctrl Pts',(52.7876627669651,-38.2144165753642,
-177.642286402424));
#161833=CARTESIAN_POINT('Ctrl Pts',(52.7717128843553,-38.2567167732527,
-177.611129211082));
#161834=CARTESIAN_POINT('Ctrl Pts',(52.7499450355462,-38.3166003893438,
-177.559711841195));
#161835=CARTESIAN_POINT('Ctrl Pts',(52.743048896851,-38.3359674737686,-177.541792454086));
#161836=CARTESIAN_POINT('Ctrl Pts',(52.7299298022954,-38.3734935229716,
-177.504393152244));
#161837=CARTESIAN_POINT('Ctrl Pts',(52.7239522510328,-38.3909236892047,
-177.485754776825));
#161838=CARTESIAN_POINT('Ctrl Pts',(52.6931841096669,-38.4822980769602,
-177.380246187521));
#161839=CARTESIAN_POINT('Ctrl Pts',(52.6758770663329,-38.5389294441427,
-177.287304310837));
#161840=CARTESIAN_POINT('Ctrl Pts',(52.6511315042833,-38.6222038742842,
-177.073724745201));
#161841=CARTESIAN_POINT('Ctrl Pts',(52.6452799403198,-38.6433981513254,
-176.963536569195));
#161842=CARTESIAN_POINT('Ctrl Pts',(52.6451348158641,-38.6439112191758,
-176.84995));
#161843=CARTESIAN_POINT('',(53.3846587239314,-37.9343850848642,-177.325518346031));
#161844=CARTESIAN_POINT('Origin',(53.3846587239314,-38.0887701497285,-177.801086692062));
#161845=CARTESIAN_POINT('Ctrl Pts',(53.1262583325313,-38.28000002,-176.84995));
#161846=CARTESIAN_POINT('Ctrl Pts',(53.1262583325313,-38.28000002,-176.881246264157));
#161847=CARTESIAN_POINT('Ctrl Pts',(53.1278631222718,-38.2769604420907,
-176.912161979889));
#161848=CARTESIAN_POINT('Ctrl Pts',(53.1310877945824,-38.2712384373324,
-176.942246935877));
#161849=CARTESIAN_POINT('Ctrl Pts',(53.1344117918852,-38.2653401858042,
-176.97325855595));
#161850=CARTESIAN_POINT('Ctrl Pts',(53.1394569106395,-38.2565916101631,
-177.003387789554));
#161851=CARTESIAN_POINT('Ctrl Pts',(53.1462419631605,-38.2453451529124,
-177.032183119753));
#161852=CARTESIAN_POINT('Ctrl Pts',(53.1533750701167,-38.2335217834987,
-177.062455570778));
#161853=CARTESIAN_POINT('Ctrl Pts',(53.1624310737952,-38.2189376813828,
-177.09125406242));
#161854=CARTESIAN_POINT('Ctrl Pts',(53.1734359847931,-38.201960916429,-177.118094373856));
#161855=CARTESIAN_POINT('Ctrl Pts',(53.1779314035387,-38.1950260427687,
-177.129058427921));
#161856=CARTESIAN_POINT('Ctrl Pts',(53.1827520853554,-38.1876914539528,
-177.139696152833));
#161857=CARTESIAN_POINT('Ctrl Pts',(53.1879000622338,-38.1799804108256,
-177.149976143786));
#161858=CARTESIAN_POINT('Ctrl Pts',(53.188619169172,-38.1789032761096,-177.151412127861));
#161859=CARTESIAN_POINT('Ctrl Pts',(53.1893448856165,-38.1778193219541,
-177.152840685413));
#161860=CARTESIAN_POINT('Ctrl Pts',(53.1900771912037,-38.1767286560635,
-177.154261804692));
#161861=CARTESIAN_POINT('Ctrl Pts',(53.2032198647385,-38.1571544974243,
-177.179766603611));
#161862=CARTESIAN_POINT('Ctrl Pts',(53.2185121297572,-38.1353791413438,
-177.202931559866));
#161863=CARTESIAN_POINT('Ctrl Pts',(53.235872888282,-38.1119750815074,-177.223655356482));
#161864=CARTESIAN_POINT('Ctrl Pts',(53.2503574923944,-38.0924483689579,
-177.24094584464));
#161865=CARTESIAN_POINT('Ctrl Pts',(53.2662825550407,-38.0717865852687,
-177.256537463912));
#161866=CARTESIAN_POINT('Ctrl Pts',(53.2836107583403,-38.0503026809971,
-177.270367729685));
#161867=CARTESIAN_POINT('Ctrl Pts',(53.3088054318523,-38.0190657463577,
-177.290476509845));
#161868=CARTESIAN_POINT('Ctrl Pts',(53.3369667492511,-37.9860904738857,
-177.306863401143));
#161869=CARTESIAN_POINT('Ctrl Pts',(53.3679987952442,-37.9523040600082,
-177.319310738459));
#161870=CARTESIAN_POINT('Ctrl Pts',(53.3734631729281,-37.9463546705915,
-177.321502567908));
#161871=CARTESIAN_POINT('Ctrl Pts',(53.3790166292581,-37.9403800305232,
-177.323572190274));
#161872=CARTESIAN_POINT('Ctrl Pts',(53.3846587239314,-37.9343850848643,
-177.325518346031));
#161873=CARTESIAN_POINT('Ctrl Pts',(53.0752347700893,-37.5697245962714,
-177.84995));
#161874=CARTESIAN_POINT('Ctrl Pts',(53.0752347700892,-37.5697245962714,
-177.34995));
#161875=CARTESIAN_POINT('Ctrl Pts',(53.5288692553037,-37.78000002,-177.34995));
#161876=CARTESIAN_POINT('Ctrl Pts',(53.0269261151962,-37.673942537699,-177.849949988053));
#161877=CARTESIAN_POINT('Ctrl Pts',(53.0475810937503,-37.6293828354337,
-177.371580332169));
#161878=CARTESIAN_POINT('Ctrl Pts',(53.4801386760123,-37.8325641065285,
-177.34995));
#161879=CARTESIAN_POINT('Ctrl Pts',(52.9791793012708,-37.7761418725299,
-177.833741031442));
#161880=CARTESIAN_POINT('Ctrl Pts',(53.0170937964823,-37.6950135347464,
-177.382936820891));
#161881=CARTESIAN_POINT('Ctrl Pts',(53.4320050770023,-37.884077740683,-177.341849758034));
#161882=CARTESIAN_POINT('Ctrl Pts',(52.9322463618642,-37.8758780299853,
-177.801086692062));
#161883=CARTESIAN_POINT('Ctrl Pts',(52.9848137611505,-37.764168205744,-177.380776321343));
#161884=CARTESIAN_POINT('Ctrl Pts',(53.3846587239314,-37.9343850848642,
-177.325518346031));
#161885=CARTESIAN_POINT('',(53.0752347700893,-37.5697245962714,-177.84995));
#161886=CARTESIAN_POINT('Origin',(53.46537255433,-36.3098838506748,-168.829790838513));
#161887=CARTESIAN_POINT('Origin',(53.5288692553037,-37.78000002,-177.84995));
#161888=CARTESIAN_POINT('Origin',(54.0849713004979,-36.8984163346077,-171.288907793803));
#161889=CARTESIAN_POINT('Origin',(0.,-12.9675000200281,-177.84995));
#161890=CARTESIAN_POINT('',(53.3022372549338,-37.073961884407,-177.84995));
#161891=CARTESIAN_POINT('Origin',(0.,-12.9675000200281,-177.84995));
#161892=CARTESIAN_POINT('Origin',(53.7578119323263,-37.28000002,-177.84995));
#161893=CARTESIAN_POINT('Ctrl Pts',(53.7396474992599,-36.0824364606782,
-176.84995));
#161894=CARTESIAN_POINT('Ctrl Pts',(53.4396057593646,-36.78000002,-176.84995));
#161895=CARTESIAN_POINT('Ctrl Pts',(54.1989607257493,-36.78000002,-176.84995));
#161896=CARTESIAN_POINT('Ctrl Pts',(53.7396474882981,-36.0824364861631,
-176.986685785392));
#161897=CARTESIAN_POINT('Ctrl Pts',(53.4396057606977,-36.7800000160094,
-176.873130497251));
#161898=CARTESIAN_POINT('Ctrl Pts',(54.1989607146972,-36.78000002,-176.918317891383));
#161899=CARTESIAN_POINT('Ctrl Pts',(53.7273175494953,-36.1111537311933,
-177.124284716345));
#161900=CARTESIAN_POINT('Ctrl Pts',(53.4415801188845,-36.7743609339043,
-176.898046003587));
#161901=CARTESIAN_POINT('Ctrl Pts',(54.1865253922149,-36.7944813746413,
-176.987117359946));
#161902=CARTESIAN_POINT('Ctrl Pts',(53.6813602693863,-36.2175520155611,
-177.371624356797));
#161903=CARTESIAN_POINT('Ctrl Pts',(53.4422054158915,-36.7696056006871,
-176.971124353297));
#161904=CARTESIAN_POINT('Ctrl Pts',(54.1401753140075,-36.8481352183371,
-177.110787176626));
#161905=CARTESIAN_POINT('Ctrl Pts',(53.64758418971,-36.2955323627627,-177.48288953791));
#161906=CARTESIAN_POINT('Ctrl Pts',(53.4404233153528,-36.7716343519663,
-177.018743720143));
#161907=CARTESIAN_POINT('Ctrl Pts',(54.1061105508192,-36.8874586360784,
-177.16641977034));
#161908=CARTESIAN_POINT('Ctrl Pts',(53.565994475128,-36.4822744877163,-177.662885027711));
#161909=CARTESIAN_POINT('Ctrl Pts',(53.4231809570326,-36.8072884980391,
-177.124958325117));
#161910=CARTESIAN_POINT('Ctrl Pts',(54.0238234872226,-36.9816277442484,
-177.25641751247));
#161911=CARTESIAN_POINT('Ctrl Pts',(53.5177345753394,-36.5920295740937,
-177.73300576859));
#161912=CARTESIAN_POINT('Ctrl Pts',(53.408253154931,-36.8396793680934,-177.182243847129));
#161913=CARTESIAN_POINT('Ctrl Pts',(53.9751511105352,-37.0369743252984,
-177.291477883886));
#161914=CARTESIAN_POINT('Ctrl Pts',(53.4140738058199,-36.825476258465,-177.826284139284));
#161915=CARTESIAN_POINT('Ctrl Pts',(53.3641465670514,-36.936877735883,-177.281217994791));
#161916=CARTESIAN_POINT('Ctrl Pts',(53.8706043508049,-37.1546953024018,
-177.33811707005));
#161917=CARTESIAN_POINT('Ctrl Pts',(53.3581698892714,-36.9502882170505,
-177.849949987733));
#161918=CARTESIAN_POINT('Ctrl Pts',(53.3356547273387,-37.0000719000691,
-177.323538819178));
#161919=CARTESIAN_POINT('Ctrl Pts',(53.8142255012181,-37.2176314844153,
-177.34995));
#161920=CARTESIAN_POINT('Ctrl Pts',(53.3022372549337,-37.073961884407,-177.84995));
#161921=CARTESIAN_POINT('Ctrl Pts',(53.3022372549337,-37.073961884407,-177.34995));
#161922=CARTESIAN_POINT('Ctrl Pts',(53.7578119323263,-37.28000002,-177.34995));
#161923=CARTESIAN_POINT('',(53.7396474992599,-36.0824364606782,-176.84995));
#161924=CARTESIAN_POINT('',(54.1989607257493,-36.78000002,-176.84995));
#161925=CARTESIAN_POINT('Origin',(54.1989607257493,-36.28000002,-176.84995));
#161926=CARTESIAN_POINT('Ctrl Pts',(53.7578119323263,-37.28000002,-177.34995));
#161927=CARTESIAN_POINT('Ctrl Pts',(53.7742161642685,-37.2618641718634,
-177.34995));
#161928=CARTESIAN_POINT('Ctrl Pts',(53.7896996386724,-37.2446503004515,
-177.348965174158));
#161929=CARTESIAN_POINT('Ctrl Pts',(53.8042623555378,-37.2284354820834,
-177.347283990825));
#161930=CARTESIAN_POINT('Ctrl Pts',(53.8188250724033,-37.2122206637153,
-177.345602807491));
#161931=CARTESIAN_POINT('Ctrl Pts',(53.8324670317305,-37.1970039098326,
-177.343225742402));
#161932=CARTESIAN_POINT('Ctrl Pts',(53.8451882335193,-37.1828122174664,
-177.340413587883));
#161933=CARTESIAN_POINT('Ctrl Pts',(53.857909435308,-37.1686205251002,-177.337601433363));
#161934=CARTESIAN_POINT('Ctrl Pts',(53.8697098795585,-37.1554529856455,
-177.334354420005));
#161935=CARTESIAN_POINT('Ctrl Pts',(53.8805895662706,-37.1433007895161,
-177.330900434437));
#161936=CARTESIAN_POINT('Ctrl Pts',(53.8860294096267,-37.1372246914513,
-177.329173441653));
#161937=CARTESIAN_POINT('Ctrl Pts',(53.8912390635981,-37.1314019563217,
-177.327394169022));
#161938=CARTESIAN_POINT('Ctrl Pts',(53.896218528185,-37.1258291482413,-177.325587826819));
#161939=CARTESIAN_POINT('Ctrl Pts',(53.8987082604785,-37.123042744201,-177.324684655718));
#161940=CARTESIAN_POINT('Ctrl Pts',(53.9011404454257,-37.1203188302431,
-177.323774692228));
#161941=CARTESIAN_POINT('Ctrl Pts',(53.9035150830269,-37.1176568289441,
-177.322860867202));
#161942=CARTESIAN_POINT('Ctrl Pts',(53.9050269887681,-37.1159619618851,
-177.322279044821));
#161943=CARTESIAN_POINT('Ctrl Pts',(53.9060312701474,-37.1148383391854,
-177.321886952289));
#161944=CARTESIAN_POINT('Ctrl Pts',(53.9074529654649,-37.1132418564841,
-177.32132216178));
#161945=CARTESIAN_POINT('Ctrl Pts',(53.9082642209632,-37.1123308628601,
-177.320999877954));
#161946=CARTESIAN_POINT('Ctrl Pts',(53.9092113920242,-37.11126605107,-177.32062090017));
#161947=CARTESIAN_POINT('Ctrl Pts',(53.9104663537919,-37.1098560275704,
-177.320110634082));
#161948=CARTESIAN_POINT('Ctrl Pts',(53.9286403697806,-37.0894364496314,
-177.312721098969));
#161949=CARTESIAN_POINT('Ctrl Pts',(53.945830114481,-37.0700140267857,-177.30418716129));
#161950=CARTESIAN_POINT('Ctrl Pts',(53.9620355878932,-37.0516626268298,
-177.294766855436));
#161951=CARTESIAN_POINT('Ctrl Pts',(53.9704708009668,-37.0421104240097,
-177.289863432681));
#161952=CARTESIAN_POINT('Ctrl Pts',(53.9786393383145,-37.0328475167389,
-177.284719695117));
#161953=CARTESIAN_POINT('Ctrl Pts',(53.9865411999362,-37.0238789920465,
-177.279370561967));
#161954=CARTESIAN_POINT('Ctrl Pts',(53.9980825382031,-37.0107797020075,
-177.271557699875));
#161955=CARTESIAN_POINT('Ctrl Pts',(54.0090549750916,-36.9983089772956,
-177.263307000333));
#161956=CARTESIAN_POINT('Ctrl Pts',(54.0194585106015,-36.9864704300919,
-177.254722009715));
#161957=CARTESIAN_POINT('Ctrl Pts',(54.0246602783564,-36.9805511564901,
-177.250429514406));
#161958=CARTESIAN_POINT('Ctrl Pts',(54.0297198207667,-36.9747897105812,
-177.24605334149));
#161959=CARTESIAN_POINT('Ctrl Pts',(54.0346371378324,-36.9691853307801,
-177.241605753137));
#161960=CARTESIAN_POINT('Ctrl Pts',(54.0370957963652,-36.9663831408796,
-177.23938195896));
#161961=CARTESIAN_POINT('Ctrl Pts',(54.0395188985619,-36.9636202164527,
-177.237140312228));
#161962=CARTESIAN_POINT('Ctrl Pts',(54.0419064444224,-36.9608963777589,
-177.234882286914));
#161963=CARTESIAN_POINT('Ctrl Pts',(54.043405607905,-36.9591860527052,-177.233464450653));
#161964=CARTESIAN_POINT('Ctrl Pts',(54.0445719721906,-36.9578593946011,
-177.232350366739));
#161965=CARTESIAN_POINT('Ctrl Pts',(54.0460060332577,-36.9562209688304,
-177.230958039316));
#161966=CARTESIAN_POINT('Ctrl Pts',(54.0468558368952,-36.9552500616551,
-177.230132966427));
#161967=CARTESIAN_POINT('Ctrl Pts',(54.0477996442507,-36.954170063335,-177.229209704986));
#161968=CARTESIAN_POINT('Ctrl Pts',(54.0489624129955,-36.9528419344281,
-177.228060548709));
#161969=CARTESIAN_POINT('Ctrl Pts',(54.0658572581406,-36.933544432399,-177.211363490556));
#161970=CARTESIAN_POINT('Ctrl Pts',(54.0813249082697,-36.9157048558455,
-177.193340117963));
#161971=CARTESIAN_POINT('Ctrl Pts',(54.0953653633829,-36.899453296305,-177.174271123402));
#161972=CARTESIAN_POINT('Ctrl Pts',(54.1095973246742,-36.8829800720087,
-177.154942035402));
#161973=CARTESIAN_POINT('Ctrl Pts',(54.1223628927005,-36.8681384062243,
-177.134539220605));
#161974=CARTESIAN_POINT('Ctrl Pts',(54.133662067462,-36.8550100974057,-177.113357603712));
#161975=CARTESIAN_POINT('Ctrl Pts',(54.1452128022232,-36.8415895055282,
-177.091704408349));
#161976=CARTESIAN_POINT('Ctrl Pts',(54.1552311225709,-36.8299592999462,
-177.069237960316));
#161977=CARTESIAN_POINT('Ctrl Pts',(54.1637170285051,-36.8201524333186,
-177.046266573481));
#161978=CARTESIAN_POINT('Ctrl Pts',(54.1723062109049,-36.8102262136684,
-177.023015616773));
#161979=CARTESIAN_POINT('Ctrl Pts',(54.1793254518669,-36.8021676798368,
-176.999247911822));
#161980=CARTESIAN_POINT('Ctrl Pts',(54.1847747513913,-36.7959591590977,
-176.975267376995));
#161981=CARTESIAN_POINT('Ctrl Pts',(54.1903346383764,-36.7896246433495,
-176.95080018394));
#161982=CARTESIAN_POINT('Ctrl Pts',(54.1942602169326,-36.785215650759,-176.926111964466));
#161983=CARTESIAN_POINT('Ctrl Pts',(54.1965514870599,-36.7826646057738,
-176.901500807525));
#161984=CARTESIAN_POINT('Ctrl Pts',(54.1981576461862,-36.7808763468795,
-176.884248614578));
#161985=CARTESIAN_POINT('Ctrl Pts',(54.1989607257493,-36.78000002,-176.867033759598));
#161986=CARTESIAN_POINT('Ctrl Pts',(54.1989607257493,-36.78000002,-176.84995));
#161987=CARTESIAN_POINT('Ctrl Pts',(53.7396474992599,-36.0824364606782,
-176.84995));
#161988=CARTESIAN_POINT('Ctrl Pts',(53.7396474962954,-36.0824364675704,
-176.886929243848));
#161989=CARTESIAN_POINT('Ctrl Pts',(53.7387474700292,-36.084532659728,-176.923734373979));
#161990=CARTESIAN_POINT('Ctrl Pts',(53.7370043459075,-36.0885863209691,
-176.960178957691));
#161991=CARTESIAN_POINT('Ctrl Pts',(53.7352184275947,-36.0927395007422,
-176.997518266259));
#161992=CARTESIAN_POINT('Ctrl Pts',(53.7325474396826,-36.0989476220766,
-177.034480202452));
#161993=CARTESIAN_POINT('Ctrl Pts',(53.7290307937802,-36.1071124473777,
-177.070872685113));
#161994=CARTESIAN_POINT('Ctrl Pts',(53.7254987744607,-36.11531296614,-177.107424261645));
#161995=CARTESIAN_POINT('Ctrl Pts',(53.721113562465,-36.1254876499988,-177.143402563609));
#161996=CARTESIAN_POINT('Ctrl Pts',(53.7158949175063,-36.1375837241688,
-177.178604159827));
#161997=CARTESIAN_POINT('Ctrl Pts',(53.712488356777,-36.1454796457293,-177.201582610408));
#161998=CARTESIAN_POINT('Ctrl Pts',(53.7087262603451,-36.1541952209923,
-177.224229886336));
#161999=CARTESIAN_POINT('Ctrl Pts',(53.7046098856868,-36.1637255131277,
-177.246483747673));
#162000=CARTESIAN_POINT('Ctrl Pts',(53.7045192628111,-36.1639353245641,
-177.246973671229));
#162001=CARTESIAN_POINT('Ctrl Pts',(53.7044284725267,-36.1641455209115,
-177.247463380496));
#162002=CARTESIAN_POINT('Ctrl Pts',(53.7043375149313,-36.1643561019227,
-177.247952874551));
#162003=CARTESIAN_POINT('Ctrl Pts',(53.6892733519024,-36.1992319874284,
-177.329021620976));
#162004=CARTESIAN_POINT('Ctrl Pts',(53.6695548792007,-36.2447904442859,
-177.40484536344));
#162005=CARTESIAN_POINT('Ctrl Pts',(53.6462229782969,-36.2984391069866,
-177.472877385971));
#162006=CARTESIAN_POINT('Ctrl Pts',(53.6342065867359,-36.3260692319555,
-177.507915226427));
#162007=CARTESIAN_POINT('Ctrl Pts',(53.6212319843108,-36.3558446669907,
-177.540885760619));
#162008=CARTESIAN_POINT('Ctrl Pts',(53.6074429005481,-36.3874074842064,
-177.571437587764));
#162009=CARTESIAN_POINT('Ctrl Pts',(53.6072249340652,-36.3879064032337,
-177.571920525892));
#162010=CARTESIAN_POINT('Ctrl Pts',(53.6070067635404,-36.3884057700779,
-177.572402861668));
#162011=CARTESIAN_POINT('Ctrl Pts',(53.6067883895477,-36.3889055833105,
-177.572884593669));
#162012=CARTESIAN_POINT('Ctrl Pts',(53.5821747509553,-36.4452411483475,
-177.627182164609));
#162013=CARTESIAN_POINT('Ctrl Pts',(53.5548118941676,-36.5076136010272,
-177.674313675416));
#162014=CARTESIAN_POINT('Ctrl Pts',(53.5255575781486,-36.573947440762,-177.713411209492));
#162015=CARTESIAN_POINT('Ctrl Pts',(53.5065780536929,-36.6169833036638,
-177.738776786444));
#162016=CARTESIAN_POINT('Ctrl Pts',(53.4868028977424,-36.6616853915005,
-177.760761117544));
#162017=CARTESIAN_POINT('Ctrl Pts',(53.4664703600909,-36.7074778455205,
-177.779132991661));
#162018=CARTESIAN_POINT('Ctrl Pts',(53.4662816165212,-36.7079029292647,
-177.779303534716));
#162019=CARTESIAN_POINT('Ctrl Pts',(53.4660928305315,-36.7083280943329,
-177.779473761639));
#162020=CARTESIAN_POINT('Ctrl Pts',(53.4659040022552,-36.7087533403953,
-177.77964367236));
#162021=CARTESIAN_POINT('Ctrl Pts',(53.4491838139251,-36.7464076281518,
-177.794688766856));
#162022=CARTESIAN_POINT('Ctrl Pts',(53.4320805422693,-36.7848119006859,
-177.807311664152));
#162023=CARTESIAN_POINT('Ctrl Pts',(53.4146874063871,-36.8237527438973,
-177.817537516946));
#162024=CARTESIAN_POINT('Ctrl Pts',(53.3964494296166,-36.8645850698631,
-177.828260072497));
#162025=CARTESIAN_POINT('Ctrl Pts',(53.3778922436239,-36.9060085268254,
-177.836347616446));
#162026=CARTESIAN_POINT('Ctrl Pts',(53.3591168326373,-36.9477888085124,
-177.841770056554));
#162027=CARTESIAN_POINT('Ctrl Pts',(53.341462719104,-36.9870739052212,-177.846868659901));
#162028=CARTESIAN_POINT('Ctrl Pts',(53.3236152017301,-37.0266755174965,
-177.84961057998));
#162029=CARTESIAN_POINT('Ctrl Pts',(53.3056598276503,-37.0663926738597,
-177.849920463284));
#162030=CARTESIAN_POINT('Ctrl Pts',(53.3045193956943,-37.0689153010195,
-177.84994014546));
#162031=CARTESIAN_POINT('Ctrl Pts',(53.3033785305219,-37.0714383891502,
-177.84994999975));
#162032=CARTESIAN_POINT('Ctrl Pts',(53.3022372549337,-37.073961884407,-177.84995));
#162033=CARTESIAN_POINT('Origin',(0.,-12.9675000200281,-171.871644662643));
#162034=CARTESIAN_POINT('',(55.8171229357418,-30.4803178166104,-171.871644662643));
#162035=CARTESIAN_POINT('',(53.7396474992599,-36.0824364606782,-171.871644662643));
#162036=CARTESIAN_POINT('Origin',(0.,-12.9675000200281,-171.871644662643));
#162037=CARTESIAN_POINT('Origin',(54.4948546080238,-30.6573850072952,-171.918810387206));
#162038=CARTESIAN_POINT('Origin',(52.5054720186909,-36.2860506553486,-171.88554415973));
#162039=CARTESIAN_POINT('Ctrl Pts',(56.1493945347971,-29.3837986277054,
-177.844785936526));
#162040=CARTESIAN_POINT('Ctrl Pts',(56.1342142259205,-29.434121619597,-177.331871678519));
#162041=CARTESIAN_POINT('Ctrl Pts',(56.6292894962144,-29.5770787035811,
-177.347150262834));
#162042=CARTESIAN_POINT('Ctrl Pts',(56.1018775093323,-29.5463985702924,
-177.862162411574));
#162043=CARTESIAN_POINT('Ctrl Pts',(56.1107577442959,-29.5139684054722,
-177.363880182749));
#162044=CARTESIAN_POINT('Ctrl Pts',(56.5813906191514,-29.6590318360781,
-177.355839748236));
#162045=CARTESIAN_POINT('Ctrl Pts',(56.0531240578036,-29.7103292972412,
-177.838935726109));
#162046=CARTESIAN_POINT('Ctrl Pts',(56.0827340742419,-29.6092564207282,
-177.376045780878));
#162047=CARTESIAN_POINT('Ctrl Pts',(56.5322373018424,-29.741669930829,-177.344237126135));
#162048=CARTESIAN_POINT('Ctrl Pts',(55.9715766151803,-29.9806728083875,
-177.728264152115));
#162049=CARTESIAN_POINT('Ctrl Pts',(56.0322849866008,-29.7793916826648,
-177.345524396139));
#162050=CARTESIAN_POINT('Ctrl Pts',(56.4500227583409,-29.8779487295679,
-177.288930648015));
#162051=CARTESIAN_POINT('Ctrl Pts',(55.9382308891443,-30.08981673834,-177.656430226304));
#162052=CARTESIAN_POINT('Ctrl Pts',(56.0104065995869,-29.8527129786242,
-177.315401802148));
#162053=CARTESIAN_POINT('Ctrl Pts',(56.4164036466448,-29.9329688836733,
-177.253030654974));
#162054=CARTESIAN_POINT('Ctrl Pts',(55.8448807512244,-30.3929945255238,
-177.357276649046));
#162055=CARTESIAN_POINT('Ctrl Pts',(55.9486579283204,-30.0584540429376,
-177.165590247966));
#162056=CARTESIAN_POINT('Ctrl Pts',(56.3222892817487,-30.0858012522341,
-177.10352016636));
#162057=CARTESIAN_POINT('Ctrl Pts',(55.8076346494222,-30.5102974021064,
-177.049065942077));
#162058=CARTESIAN_POINT('Ctrl Pts',(55.9196838433792,-30.1531627459377,
-176.973586313919));
#162059=CARTESIAN_POINT('Ctrl Pts',(56.2847345577538,-30.1449403478704,
-176.949470753));
#162060=CARTESIAN_POINT('Ctrl Pts',(55.8190628544783,-30.4741856133569,
-176.737644210045));
#162061=CARTESIAN_POINT('Ctrl Pts',(55.928299612176,-30.1249513476889,-176.780220154851));
#162062=CARTESIAN_POINT('Ctrl Pts',(56.2962571325131,-30.1267348532474,
-176.793818000512));
#162063=CARTESIAN_POINT('',(56.1185967245324,-29.4887923928816,-177.84995));
#162064=CARTESIAN_POINT('Origin',(56.5982428503831,-29.63000002,-177.84995));
#162065=CARTESIAN_POINT('',(56.294192362543,-30.13000002,-176.84995));
#162066=CARTESIAN_POINT('Ctrl Pts',(56.294192362543,-30.1300000200003,-176.84995));
#162067=CARTESIAN_POINT('Ctrl Pts',(56.294192362543,-30.1300000200003,-176.872532726662));
#162068=CARTESIAN_POINT('Ctrl Pts',(56.2951871195896,-30.128424325105,-176.895415122225));
#162069=CARTESIAN_POINT('Ctrl Pts',(56.2972200545588,-30.1251924179988,
-176.918380988318));
#162070=CARTESIAN_POINT('Ctrl Pts',(56.2992533574375,-30.1219599259996,
-176.941351010649));
#162071=CARTESIAN_POINT('Ctrl Pts',(56.3023252550559,-30.1170705541272,
-176.96440447796));
#162072=CARTESIAN_POINT('Ctrl Pts',(56.3064575683391,-30.1104754876797,
-176.987289624132));
#162073=CARTESIAN_POINT('Ctrl Pts',(56.3098470935837,-30.1050658919688,
-177.006061139107));
#162074=CARTESIAN_POINT('Ctrl Pts',(56.3139496794318,-30.0985092698674,
-177.024718724667));
#162075=CARTESIAN_POINT('Ctrl Pts',(56.3187663016207,-30.0907949872297,
-177.043106194985));
#162076=CARTESIAN_POINT('Ctrl Pts',(56.3247125232521,-30.0812715426887,
-177.065805914718));
#162077=CARTESIAN_POINT('Ctrl Pts',(56.3317495940632,-30.0699796808652,
-177.088105999951));
#162078=CARTESIAN_POINT('Ctrl Pts',(56.339872577453,-30.0569073841108,-177.109701679162));
#162079=CARTESIAN_POINT('Ctrl Pts',(56.3471147754336,-30.0452525331019,
-177.128955711438));
#162080=CARTESIAN_POINT('Ctrl Pts',(56.3552202898462,-30.0321821766178,
-177.147649859116));
#162081=CARTESIAN_POINT('Ctrl Pts',(56.3641742816089,-30.017703673564,-177.165535027629));
#162082=CARTESIAN_POINT('Ctrl Pts',(56.3713982853061,-30.006022541577,-177.179964628067));
#162083=CARTESIAN_POINT('Ctrl Pts',(56.379174697935,-29.9934245779848,-177.193867303819));
#162084=CARTESIAN_POINT('Ctrl Pts',(56.3874868256334,-29.9799269208526,
-177.207093049855));
#162085=CARTESIAN_POINT('Ctrl Pts',(56.3875437244285,-29.9798345256854,
-177.207183583716));
#162086=CARTESIAN_POINT('Ctrl Pts',(56.387601036394,-29.9797414581918,-177.207274703301));
#162087=CARTESIAN_POINT('Ctrl Pts',(56.3876587294906,-29.9796477703371,
-177.207366354808));
#162088=CARTESIAN_POINT('Ctrl Pts',(56.3889136919176,-29.9776098360883,
-177.209359993644));
#162089=CARTESIAN_POINT('Ctrl Pts',(56.3903497458509,-29.9752768610671,
-177.211601751091));
#162090=CARTESIAN_POINT('Ctrl Pts',(56.3916257120584,-29.9732030439594,
-177.21355908278));
#162091=CARTESIAN_POINT('Ctrl Pts',(56.3923646670942,-29.9720020265766,
-177.214692639532));
#162092=CARTESIAN_POINT('Ctrl Pts',(56.3930494838134,-29.9708886927357,
-177.215731700275));
#162093=CARTESIAN_POINT('Ctrl Pts',(56.3936111551582,-29.9699753935331,
-177.216578542608));
#162094=CARTESIAN_POINT('Ctrl Pts',(56.4016177287422,-29.9569563970344,
-177.228650202519));
#162095=CARTESIAN_POINT('Ctrl Pts',(56.4103290610794,-29.9427602351245,
-177.240522400568));
#162096=CARTESIAN_POINT('Ctrl Pts',(56.4197694089464,-29.927327989156,-177.251935492811));
#162097=CARTESIAN_POINT('Ctrl Pts',(56.4251958207122,-29.9184573710099,
-177.258495858902));
#162098=CARTESIAN_POINT('Ctrl Pts',(56.4308627050949,-29.9091789043299,
-177.264903978388));
#162099=CARTESIAN_POINT('Ctrl Pts',(56.4367709939623,-29.8994866145252,
-177.271105875826));
#162100=CARTESIAN_POINT('Ctrl Pts',(56.4448644739841,-29.8862096140839,
-177.279601556072));
#162101=CARTESIAN_POINT('Ctrl Pts',(56.4533986337169,-29.8721528086074,
-177.287712267273));
#162102=CARTESIAN_POINT('Ctrl Pts',(56.4623751203678,-29.8573176056849,
-177.295286194668));
#162103=CARTESIAN_POINT('Ctrl Pts',(56.4668633636933,-29.8499000042236,
-177.299073158366));
#162104=CARTESIAN_POINT('Ctrl Pts',(56.4714629450669,-29.8422883156734,
-177.302725612065));
#162105=CARTESIAN_POINT('Ctrl Pts',(56.4761738644651,-29.8344848904029,
-177.306223351956));
#162106=CARTESIAN_POINT('Ctrl Pts',(56.4785293241642,-29.8305831777676,
-177.307972221902));
#162107=CARTESIAN_POINT('Ctrl Pts',(56.4809126183669,-29.8266335308248,
-177.309682411394));
#162108=CARTESIAN_POINT('Ctrl Pts',(56.4833237470588,-29.822636425974,-177.311351308538));
#162109=CARTESIAN_POINT('Ctrl Pts',(56.48425029345,-29.8211004220737,-177.311992630849));
#162110=CARTESIAN_POINT('Ctrl Pts',(56.4851808230756,-29.8195576151434,
-177.312627772066));
#162111=CARTESIAN_POINT('Ctrl Pts',(56.4861156809213,-29.8180074786435,
-177.313256809317));
#162112=CARTESIAN_POINT('Ctrl Pts',(56.4863972017675,-29.8175406742613,
-177.313446236083));
#162113=CARTESIAN_POINT('Ctrl Pts',(56.4866790769756,-29.8170732678944,
-177.313635087301));
#162114=CARTESIAN_POINT('Ctrl Pts',(56.4869613159624,-29.8166052453073,
-177.313823365211));
#162115=CARTESIAN_POINT('Ctrl Pts',(56.4878096716068,-29.8151984601995,
-177.314389292088));
#162116=CARTESIAN_POINT('Ctrl Pts',(56.4890156263261,-29.8131986777992,
-177.315181623139));
#162117=CARTESIAN_POINT('Ctrl Pts',(56.4898401272641,-29.8118311447542,
-177.315715538206));
#162118=CARTESIAN_POINT('Ctrl Pts',(56.4902008176112,-29.8112328968372,
-177.315949107389));
#162119=CARTESIAN_POINT('Ctrl Pts',(56.490488387549,-29.8107558902657,-177.316133993143));
#162120=CARTESIAN_POINT('Ctrl Pts',(56.4906406366203,-29.8105033735255,
-177.316231754416));
#162121=CARTESIAN_POINT('Ctrl Pts',(56.4936938884552,-29.805439321616,-177.318192290436));
#162122=CARTESIAN_POINT('Ctrl Pts',(56.4974503833496,-29.7992068257096,
-177.320515037228));
#162123=CARTESIAN_POINT('Ctrl Pts',(56.501924074846,-29.7917729201856,-177.323057554814));
#162124=CARTESIAN_POINT('Ctrl Pts',(56.5063933256274,-29.7843463937703,
-177.325597548624));
#162125=CARTESIAN_POINT('Ctrl Pts',(56.5115787181557,-29.7757202500415,
-177.328356894483));
#162126=CARTESIAN_POINT('Ctrl Pts',(56.517493697644,-29.7658589234036,-177.331141834804));
#162127=CARTESIAN_POINT('Ctrl Pts',(56.5232708007539,-29.7562274612994,
-177.33386185901));
#162128=CARTESIAN_POINT('Ctrl Pts',(56.5297442839822,-29.7454170581434,
-177.336606151603));
#162129=CARTESIAN_POINT('Ctrl Pts',(56.5369204854749,-29.733401340339,-177.339146059258));
#162130=CARTESIAN_POINT('Ctrl Pts',(56.5439111552341,-29.7216962739225,
-177.341620300771));
#162131=CARTESIAN_POINT('Ctrl Pts',(56.5515690870145,-29.7088467394085,
-177.34390045058));
#162132=CARTESIAN_POINT('Ctrl Pts',(56.5598882273037,-29.6948446285046,
-177.345731013883));
#162133=CARTESIAN_POINT('Ctrl Pts',(56.5678117360862,-29.6815084128786,
-177.347474521494));
#162134=CARTESIAN_POINT('Ctrl Pts',(56.5763353622145,-29.6671261312445,
-177.348809934402));
#162135=CARTESIAN_POINT('Ctrl Pts',(56.5854379174801,-29.6517140428296,
-177.34947899318));
#162136=CARTESIAN_POINT('Ctrl Pts',(56.5895873306717,-29.6446884196817,
-177.349783984607));
#162137=CARTESIAN_POINT('Ctrl Pts',(56.5938567934851,-29.6374491756204,
-177.34995));
#162138=CARTESIAN_POINT('Ctrl Pts',(56.598242850383,-29.6300000200001,-177.34995));
#162139=CARTESIAN_POINT('',(55.8171229357418,-30.4803178166104,-176.84995));
#162140=CARTESIAN_POINT('Origin',(56.294192362543,-30.63000002,-176.84995));
#162141=CARTESIAN_POINT('Ctrl Pts',(56.1185967245324,-29.4887923928816,
-177.84995));
#162142=CARTESIAN_POINT('Ctrl Pts',(56.0804686085136,-29.6183038329331,
-177.84995));
#162143=CARTESIAN_POINT('Ctrl Pts',(56.0435105516164,-29.7422083237505,
-177.825637538525));
#162144=CARTESIAN_POINT('Ctrl Pts',(55.9706438254141,-29.983755289409,-177.726373245353));
#162145=CARTESIAN_POINT('Ctrl Pts',(55.9379975051363,-30.0905814889907,
-177.655514525474));
#162146=CARTESIAN_POINT('Ctrl Pts',(55.880677894362,-30.276726517591,-177.471099911401));
#162147=CARTESIAN_POINT('Ctrl Pts',(55.8583243128169,-30.3485429953493,
-177.364626418289));
#162148=CARTESIAN_POINT('Ctrl Pts',(55.8254079947302,-30.4539768569356,
-177.113213750895));
#162149=CARTESIAN_POINT('Ctrl Pts',(55.8171229357418,-30.4803178166104,
-176.983557056031));
#162150=CARTESIAN_POINT('Ctrl Pts',(55.8171229357418,-30.4803178166104,
-176.84995));
#162151=CARTESIAN_POINT('Origin',(0.,-12.9675000200281,-177.84995));
#162152=CARTESIAN_POINT('',(56.262175563026,-28.9930296810172,-177.84995));
#162153=CARTESIAN_POINT('Origin',(56.7430488584365,-29.13000002,-177.84995));
#162154=CARTESIAN_POINT('Origin',(0.,-12.9675000200281,-177.84995));
#162155=CARTESIAN_POINT('Ctrl Pts',(56.7430488584365,-29.13000002,-177.34995));
#162156=CARTESIAN_POINT('Ctrl Pts',(56.262175563026,-28.9930296810172,-177.34995));
#162157=CARTESIAN_POINT('Ctrl Pts',(56.262175563026,-28.9930296810172,-177.84995));
#162158=CARTESIAN_POINT('Ctrl Pts',(56.799051006553,-29.0316942919675,-177.34995));
#162159=CARTESIAN_POINT('Ctrl Pts',(56.2928119947094,-28.8854717787751,
-177.322103214377));
#162160=CARTESIAN_POINT('Ctrl Pts',(56.3176963010821,-28.7981083537361,
-177.849949971516));
#162161=CARTESIAN_POINT('Ctrl Pts',(56.8539225877547,-28.933239542368,-177.320220947896));
#162162=CARTESIAN_POINT('Ctrl Pts',(56.3169386704035,-28.8006430758332,
-177.261063208671));
#162163=CARTESIAN_POINT('Ctrl Pts',(56.3721096851181,-28.6028436438479,
-177.790491903933));
#162164=CARTESIAN_POINT('Ctrl Pts',(56.9443314005494,-28.7684056938368,
-177.209281314082));
#162165=CARTESIAN_POINT('Ctrl Pts',(56.3506671101773,-28.684579593959,-177.121256964593));
#162166=CARTESIAN_POINT('Ctrl Pts',(56.4617523202342,-28.2759697513382,
-177.568612620023));
#162167=CARTESIAN_POINT('Ctrl Pts',(56.9801582405499,-28.7016493747432,
-177.12717563931));
#162168=CARTESIAN_POINT('Ctrl Pts',(56.3596918685657,-28.6555519736166,
-177.043271150691));
#162169=CARTESIAN_POINT('Ctrl Pts',(56.4972682976465,-28.1436156829388,
-177.404470992826));
#162170=CARTESIAN_POINT('Ctrl Pts',(57.,-28.664523125878,-177.032518510534));
#162171=CARTESIAN_POINT('Ctrl Pts',(56.364125065416,-28.6418687251214,-176.974758823107));
#162172=CARTESIAN_POINT('Ctrl Pts',(56.5169491525423,-28.0699653316567,
-177.215087021068));
#162173=CARTESIAN_POINT('',(56.5169491525423,-28.0699653316567,-177.215087021068));
#162174=CARTESIAN_POINT('Origin',(57.,-28.199046231756,-177.215087021068));
#162175=CARTESIAN_POINT('Ctrl Pts',(56.5169491525423,-28.0699653316567,
-177.215087021068));
#162176=CARTESIAN_POINT('Ctrl Pts',(56.5114199834419,-28.0906567725875,
-177.26829284014));
#162177=CARTESIAN_POINT('Ctrl Pts',(56.5046490590763,-28.1159513561152,
-177.319440198101));
#162178=CARTESIAN_POINT('Ctrl Pts',(56.4967764105797,-28.145254791308,-177.367985903784));
#162179=CARTESIAN_POINT('Ctrl Pts',(56.488835970741,-28.1748105582542,-177.416949636328));
#162180=CARTESIAN_POINT('Ctrl Pts',(56.4797745088228,-28.2084455503732,
-177.46326787819));
#162181=CARTESIAN_POINT('Ctrl Pts',(56.4697238291809,-28.2455931588451,
-177.506354841674));
#162182=CARTESIAN_POINT('Ctrl Pts',(56.4600615204675,-28.281305336907,-177.547776870584));
#162183=CARTESIAN_POINT('Ctrl Pts',(56.4494846922707,-28.3202650328622,
-177.586213261633));
#162184=CARTESIAN_POINT('Ctrl Pts',(56.4381034255685,-28.3619923283887,
-177.621103904538));
#162185=CARTESIAN_POINT('Ctrl Pts',(56.4313704755802,-28.3866774360556,
-177.641744573093));
#162186=CARTESIAN_POINT('Ctrl Pts',(56.4243558827027,-28.4123314859347,
-177.661143532174));
#162187=CARTESIAN_POINT('Ctrl Pts',(56.4170817736066,-28.438856914084,-177.679176296163));
#162188=CARTESIAN_POINT('Ctrl Pts',(56.4170314275401,-28.4390405037103,
-177.679301105775));
#162189=CARTESIAN_POINT('Ctrl Pts',(56.4169810706746,-28.4392241291221,
-177.679425845849));
#162190=CARTESIAN_POINT('Ctrl Pts',(56.4169307030184,-28.4394077902846,
-177.679550516358));
#162191=CARTESIAN_POINT('Ctrl Pts',(56.4068381994777,-28.4762092036084,
-177.70453157867));
#162192=CARTESIAN_POINT('Ctrl Pts',(56.3962987764838,-28.5144807857784,
-177.726809957994));
#162193=CARTESIAN_POINT('Ctrl Pts',(56.3853954829433,-28.5539082918042,
-177.746384040078));
#162194=CARTESIAN_POINT('Ctrl Pts',(56.3741127545824,-28.5947078757818,
-177.766639300587));
#162195=CARTESIAN_POINT('Ctrl Pts',(56.3624401562768,-28.6367461405691,
-177.783999255699));
#162196=CARTESIAN_POINT('Ctrl Pts',(56.3504605117084,-28.6797057531804,
-177.798417329991));
#162197=CARTESIAN_POINT('Ctrl Pts',(56.3384882188013,-28.7226390023617,
-177.812826556209));
#162198=CARTESIAN_POINT('Ctrl Pts',(56.3262089639832,-28.7664935773127,
-177.824297783191));
#162199=CARTESIAN_POINT('Ctrl Pts',(56.3137004593873,-28.8109674781278,
-177.832735185289));
#162200=CARTESIAN_POINT('Ctrl Pts',(56.301553921008,-28.8541544105859,-177.840928429144));
#162201=CARTESIAN_POINT('Ctrl Pts',(56.2891909417748,-28.897926340654,-177.846260934398));
#162202=CARTESIAN_POINT('Ctrl Pts',(56.2766821207918,-28.942005178833,-177.848596484849));
#162203=CARTESIAN_POINT('Ctrl Pts',(56.2718668221819,-28.9589734261602,
-177.849495560218));
#162204=CARTESIAN_POINT('Ctrl Pts',(56.2670299262029,-28.9759870597071,
-177.84994999751));
#162205=CARTESIAN_POINT('Ctrl Pts',(56.262175563026,-28.9930296810172,-177.84995));
#162206=CARTESIAN_POINT('Ctrl Pts',(56.5350158381137,-28.0021946997704,
-176.811903784796));
#162207=CARTESIAN_POINT('Ctrl Pts',(56.3679651457268,-28.6303533640722,
-176.837499657378));
#162208=CARTESIAN_POINT('Ctrl Pts',(57.0184194087067,-28.6303484782574,
-176.830899202224));
#162209=CARTESIAN_POINT('Ctrl Pts',(56.5364806901874,-27.9966690056784,
-176.964298400169));
#162210=CARTESIAN_POINT('Ctrl Pts',(56.3684339309491,-28.6288435574528,
-176.887126065441));
#162211=CARTESIAN_POINT('Ctrl Pts',(57.019316568372,-28.6275595516668,-176.907060450972));
#162212=CARTESIAN_POINT('Ctrl Pts',(56.5291525614316,-28.0243358857953,
-177.110977601639));
#162213=CARTESIAN_POINT('Ctrl Pts',(56.367312788345,-28.6317888732642,-176.934996710032));
#162214=CARTESIAN_POINT('Ctrl Pts',(57.0114138500124,-28.6415256904292,
-176.980508103715));
#162215=CARTESIAN_POINT('Ctrl Pts',(56.5131231233502,-28.0842779073417,
-177.250001316319));
#162216=CARTESIAN_POINT('Ctrl Pts',(56.3631318544866,-28.6450072835911,
-176.98772630256));
#162217=CARTESIAN_POINT('Ctrl Pts',(56.9964657809338,-28.6717398279222,
-177.049971678832));
#162218=CARTESIAN_POINT('',(56.5351989170821,-28.0015042572884,-176.849882244789));
#162219=CARTESIAN_POINT('',(57.0184057454332,-28.63000002,-176.849882244789));
#162220=CARTESIAN_POINT('Origin',(57.0184057454332,-28.13000002,-176.849882244789));
#162221=CARTESIAN_POINT('Ctrl Pts',(57.,-28.6645231258781,-177.032518510534));
#162222=CARTESIAN_POINT('Ctrl Pts',(57.0039800912305,-28.6565690730968,
-177.012238847993));
#162223=CARTESIAN_POINT('Ctrl Pts',(57.0072713934122,-28.6501272490681,
-176.991904897329));
#162224=CARTESIAN_POINT('Ctrl Pts',(57.0099157186547,-28.6450662877334,
-176.971747813479));
#162225=CARTESIAN_POINT('Ctrl Pts',(57.0126656382054,-28.6398032299614,
-176.950785808475));
#162226=CARTESIAN_POINT('Ctrl Pts',(57.0147161314663,-28.636032896984,-176.930015335143));
#162227=CARTESIAN_POINT('Ctrl Pts',(57.0161153714143,-28.6335822714496,
-176.909643884951));
#162228=CARTESIAN_POINT('Ctrl Pts',(57.0175146113622,-28.6311316459152,
-176.889272434758));
#162229=CARTESIAN_POINT('Ctrl Pts',(57.018262799339,-28.63000002,-176.869299784457));
#162230=CARTESIAN_POINT('Ctrl Pts',(57.0184057454332,-28.63000002,-176.849882244789));
#162231=CARTESIAN_POINT('Origin',(55.1126545812022,-33.3251112519863,-176.014041861122));
#162232=CARTESIAN_POINT('Origin',(0.,-12.9675000200281,-171.871644662643));
#162233=CARTESIAN_POINT('',(57.7346476057222,-22.3993856132206,-171.871644662643));
#162234=CARTESIAN_POINT('',(56.5351989170821,-28.0015042572884,-171.871644662643));
#162235=CARTESIAN_POINT('Origin',(0.,-12.9675000200281,-171.871644662643));
#162236=CARTESIAN_POINT('Origin',(56.3007888374198,-22.509667514428,-171.959861518035));
#162237=CARTESIAN_POINT('Origin',(55.1752186158567,-28.1616465678281,-171.933521226257));
#162238=CARTESIAN_POINT('Ctrl Pts',(57.8819282087167,-21.4487963148736,
-177.697497252237));
#162239=CARTESIAN_POINT('Ctrl Pts',(57.8810878095005,-21.4545317502846,
-177.368333266163));
#162240=CARTESIAN_POINT('Ctrl Pts',(58.1799818947148,-21.5006430233977,
-177.238261718413));
#162241=CARTESIAN_POINT('Ctrl Pts',(57.8629489711247,-21.5783230793646,
-177.699822299871));
#162242=CARTESIAN_POINT('Ctrl Pts',(57.868876514339,-21.5377805372773,-177.374493960823));
#162243=CARTESIAN_POINT('Ctrl Pts',(58.1643305096628,-21.5659716479372,
-177.242027715059));
#162244=CARTESIAN_POINT('Ctrl Pts',(57.8432533717849,-21.7094932883126,
-177.67338127456));
#162245=CARTESIAN_POINT('Ctrl Pts',(57.8561193903755,-21.6237742374893,
-177.3594824509));
#162246=CARTESIAN_POINT('Ctrl Pts',(58.1516959167317,-21.6321056009482,
-177.229926261063));
#162247=CARTESIAN_POINT('Ctrl Pts',(57.8068932864249,-21.9467814783138,
-177.56730490578));
#162248=CARTESIAN_POINT('Ctrl Pts',(57.833274341657,-21.7763737806991,-177.289541220421));
#162249=CARTESIAN_POINT('Ctrl Pts',(58.135834617463,-21.751763745641,-177.175847704912));
#162250=CARTESIAN_POINT('Ctrl Pts',(57.7900355525622,-22.0542721190802,
-177.487158575097));
#162251=CARTESIAN_POINT('Ctrl Pts',(57.822969521998,-21.8444848229842,-177.233860492204));
#162252=CARTESIAN_POINT('Ctrl Pts',(58.1325374345936,-21.8059684297317,
-177.133613057603));
#162253=CARTESIAN_POINT('Ctrl Pts',(57.7626304144021,-22.2268825024457,
-177.290851905635));
#162254=CARTESIAN_POINT('Ctrl Pts',(57.8075855468967,-21.9461185785114,
-177.096669117024));
#162255=CARTESIAN_POINT('Ctrl Pts',(58.1379476084663,-21.8930112710375,
-177.027055273752));
#162256=CARTESIAN_POINT('Ctrl Pts',(57.7519076537925,-22.2932204551335,
-177.173672169064));
#162257=CARTESIAN_POINT('Ctrl Pts',(57.8023886323833,-21.9804905067127,
-177.013273949454));
#162258=CARTESIAN_POINT('Ctrl Pts',(58.1467121091855,-21.9264637442851,
-176.962169933093));
#162259=CARTESIAN_POINT('Ctrl Pts',(57.7379487783882,-22.3792570371924,
-176.923566462093));
#162260=CARTESIAN_POINT('Ctrl Pts',(57.7982009932088,-22.0095200736329,
-176.838338250264));
#162261=CARTESIAN_POINT('Ctrl Pts',(58.1775901524469,-21.9698497118448,
-176.818815489061));
#162262=CARTESIAN_POINT('Ctrl Pts',(57.7346476044917,-22.3993856207533,
-176.79021969384));
#162263=CARTESIAN_POINT('Ctrl Pts',(57.7993206334297,-22.0035077749888,
-176.744992431703));
#162264=CARTESIAN_POINT('Ctrl Pts',(58.1997838724148,-21.98000002,-176.740111438881));
#162265=CARTESIAN_POINT('Ctrl Pts',(57.7346476057222,-22.3993856132206,
-176.657965001855));
#162266=CARTESIAN_POINT('Ctrl Pts',(57.8031610044997,-21.98000002,-176.657965001855));
#162267=CARTESIAN_POINT('Ctrl Pts',(58.2281061322669,-21.98000002,-176.657965001855));
#162268=CARTESIAN_POINT('',(57.8819282087167,-21.4487963148736,-177.697497252237));
#162269=CARTESIAN_POINT('Origin',(58.376645543834,-21.5212860267954,-177.697497252237));
#162270=CARTESIAN_POINT('',(58.2281061322626,-21.9800000072249,-176.657965001847));
#162271=CARTESIAN_POINT('Ctrl Pts',(58.2281061322669,-21.98000002,-176.657965001855));
#162272=CARTESIAN_POINT('Ctrl Pts',(58.2156432050873,-21.98000002,-176.694112706195));
#162273=CARTESIAN_POINT('Ctrl Pts',(58.2044053428825,-21.9780314444789,
-176.729472360225));
#162274=CARTESIAN_POINT('Ctrl Pts',(58.1944420590819,-21.9740340480493,
-176.763689754096));
#162275=CARTESIAN_POINT('Ctrl Pts',(58.1894604171816,-21.9720353498345,
-176.780798451031));
#162276=CARTESIAN_POINT('Ctrl Pts',(58.1847976426165,-21.9695299941169,
-176.797620591924));
#162277=CARTESIAN_POINT('Ctrl Pts',(58.1804606715693,-21.9665165584178,
-176.814106030133));
#162278=CARTESIAN_POINT('Ctrl Pts',(58.1787278993621,-21.9653125850524,
-176.820692541512));
#162279=CARTESIAN_POINT('Ctrl Pts',(58.1771363661171,-21.9640945924079,
-176.826879459107));
#162280=CARTESIAN_POINT('Ctrl Pts',(58.1755739593543,-21.9627918105726,
-176.833082972166));
#162281=CARTESIAN_POINT('Ctrl Pts',(58.17407480742,-21.9615417725191,-176.839035332859));
#162282=CARTESIAN_POINT('Ctrl Pts',(58.1726025352164,-21.9602135784298,
-176.845003047828));
#162283=CARTESIAN_POINT('Ctrl Pts',(58.1710791571693,-21.9587089640121,
-176.851334149985));
#162284=CARTESIAN_POINT('Ctrl Pts',(58.1702164342252,-21.9578568673295,
-176.854919594256));
#162285=CARTESIAN_POINT('Ctrl Pts',(58.1693376867143,-21.9569475664076,
-176.858621235351));
#162286=CARTESIAN_POINT('Ctrl Pts',(58.1684321549172,-21.9559574019423,
-176.862498842424));
#162287=CARTESIAN_POINT('Ctrl Pts',(58.1662308623925,-21.9535503725674,
-176.871925068526));
#162288=CARTESIAN_POINT('Ctrl Pts',(58.1641348742942,-21.9509516579958,
-176.881260355963));
#162289=CARTESIAN_POINT('Ctrl Pts',(58.1621473919756,-21.9481572100565,
-176.890493088755));
#162290=CARTESIAN_POINT('Ctrl Pts',(58.1566032426735,-21.9403620027998,
-176.916248109862));
#162291=CARTESIAN_POINT('Ctrl Pts',(58.1518943927396,-21.9310133708706,
-176.941234732476));
#162292=CARTESIAN_POINT('Ctrl Pts',(58.1480208458896,-21.9201857317733,
-176.965150077762));
#162293=CARTESIAN_POINT('Ctrl Pts',(58.1463352305236,-21.9154739687441,
-176.975557096202));
#162294=CARTESIAN_POINT('Ctrl Pts',(58.1448350754385,-21.9105702566688,
-176.985577584898));
#162295=CARTESIAN_POINT('Ctrl Pts',(58.1434852751035,-21.9054093827837,
-176.995378681003));
#162296=CARTESIAN_POINT('Ctrl Pts',(58.1421472864369,-21.9002936700451,
-177.005094010869));
#162297=CARTESIAN_POINT('Ctrl Pts',(58.1409571143495,-21.8949250790412,
-177.014594131085));
#162298=CARTESIAN_POINT('Ctrl Pts',(58.1399011290586,-21.8892047551052,
-177.024011615046));
#162299=CARTESIAN_POINT('Ctrl Pts',(58.1388806139833,-21.883676575061,-177.033112768667));
#162300=CARTESIAN_POINT('Ctrl Pts',(58.1379854764992,-21.8778197504792,
-177.042137097446));
#162301=CARTESIAN_POINT('Ctrl Pts',(58.1372216369892,-21.8715145130864,
-177.051170949139));
#162302=CARTESIAN_POINT('Ctrl Pts',(58.1370840173307,-21.8703785092458,
-177.052798562753));
#162303=CARTESIAN_POINT('Ctrl Pts',(58.1369507081154,-21.8692278697024,
-177.054426386573));
#162304=CARTESIAN_POINT('Ctrl Pts',(58.1368218087854,-21.8680617875073,
-177.056054789025));
#162305=CARTESIAN_POINT('Ctrl Pts',(58.1361650523263,-21.8621204687019,
-177.064351681087));
#162306=CARTESIAN_POINT('Ctrl Pts',(58.1356363393907,-21.8559283084116,
-177.07245496925));
#162307=CARTESIAN_POINT('Ctrl Pts',(58.1352380015467,-21.8494904929985,
-177.08033537195));
#162308=CARTESIAN_POINT('Ctrl Pts',(58.1344071771017,-21.83606296032,-177.096771749506));
#162309=CARTESIAN_POINT('Ctrl Pts',(58.1341394415401,-21.8215054517519,
-177.112290333485));
#162310=CARTESIAN_POINT('Ctrl Pts',(58.1344181335807,-21.8059909922371,
-177.126663547938));
#162311=CARTESIAN_POINT('Ctrl Pts',(58.1344801685191,-21.8025375798625,
-177.129862926982));
#162312=CARTESIAN_POINT('Ctrl Pts',(58.1345691972595,-21.7990369110223,
-177.133005658565));
#162313=CARTESIAN_POINT('Ctrl Pts',(58.1346849015299,-21.7954911519696,
-177.136089423575));
#162314=CARTESIAN_POINT('Ctrl Pts',(58.1349931881012,-21.7860437055044,
-177.144305916688));
#162315=CARTESIAN_POINT('Ctrl Pts',(58.1354941233143,-21.7761663325933,
-177.152194777092));
#162316=CARTESIAN_POINT('Ctrl Pts',(58.1361828836554,-21.7659911953573,
-177.159618268632));
#162317=CARTESIAN_POINT('Ctrl Pts',(58.1368690686029,-21.7558541047117,
-177.167014002458));
#162318=CARTESIAN_POINT('Ctrl Pts',(58.1377415390541,-21.7454219712837,
-177.173947428276));
#162319=CARTESIAN_POINT('Ctrl Pts',(58.1387787204352,-21.7348510683059,
-177.180324083576));
#162320=CARTESIAN_POINT('Ctrl Pts',(58.1396881507361,-21.7255821982215,
-177.185915317331));
#162321=CARTESIAN_POINT('Ctrl Pts',(58.1407238858634,-21.7162072526313,
-177.19107901569));
#162322=CARTESIAN_POINT('Ctrl Pts',(58.1418621794207,-21.7068430038689,
-177.195781098596));
#162323=CARTESIAN_POINT('Ctrl Pts',(58.142458961938,-21.701933532219,-177.198246298241));
#162324=CARTESIAN_POINT('Ctrl Pts',(58.1430910223037,-21.6969631041976,
-177.200617659317));
#162325=CARTESIAN_POINT('Ctrl Pts',(58.1437581575669,-21.6919348657256,
-177.202889874908));
#162326=CARTESIAN_POINT('Ctrl Pts',(58.1462286069172,-21.6733149408743,
-177.211304050922));
#162327=CARTESIAN_POINT('Ctrl Pts',(58.1491881991552,-21.6538329623342,
-177.218381304938));
#162328=CARTESIAN_POINT('Ctrl Pts',(58.1526065770555,-21.633732508915,-177.223966894812));
#162329=CARTESIAN_POINT('Ctrl Pts',(58.1562202733795,-21.6124835608022,
-177.229871632727));
#162330=CARTESIAN_POINT('Ctrl Pts',(58.1603466629203,-21.5905439782932,
-177.234108763021));
#162331=CARTESIAN_POINT('Ctrl Pts',(58.1649305053795,-21.5682460893206,
-177.236532779346));
#162332=CARTESIAN_POINT('Ctrl Pts',(58.1695143478386,-21.5459482003481,
-177.23895679567));
#162333=CARTESIAN_POINT('Ctrl Pts',(58.1745553917398,-21.5232931578517,
-177.239567429792));
#162334=CARTESIAN_POINT('Ctrl Pts',(58.1799818945846,-21.5006430239411,
-177.238261718445));
#162335=CARTESIAN_POINT('',(57.7346476057222,-22.3993856132206,-176.657965001855));
#162336=CARTESIAN_POINT('Origin',(58.2281061322669,-22.48000002,-176.657965001855));
#162337=CARTESIAN_POINT('Ctrl Pts',(57.8819282087167,-21.4487963148736,
-177.697497252237));
#162338=CARTESIAN_POINT('Ctrl Pts',(57.8765896421257,-21.4852301944857,
-177.698151252249));
#162339=CARTESIAN_POINT('Ctrl Pts',(57.8712308062151,-21.5215461998528,
-177.696528688191));
#162340=CARTESIAN_POINT('Ctrl Pts',(57.8658871784514,-21.5575327106497,
-177.692745867402));
#162341=CARTESIAN_POINT('Ctrl Pts',(57.8604287549616,-21.5942923100331,
-177.688881781285));
#162342=CARTESIAN_POINT('Ctrl Pts',(57.8549860188209,-21.6307092686159,
-177.682763561799));
#162343=CARTESIAN_POINT('Ctrl Pts',(57.849594035819,-21.6665701891048,-177.674461317079));
#162344=CARTESIAN_POINT('Ctrl Pts',(57.8442188129476,-21.7023196415671,
-177.66618487858));
#162345=CARTESIAN_POINT('Ctrl Pts',(57.8388938392211,-21.737517702457,-177.655737740554));
#162346=CARTESIAN_POINT('Ctrl Pts',(57.8336539589831,-21.7719470718026,
-177.643138949619));
#162347=CARTESIAN_POINT('Ctrl Pts',(57.8307658910941,-21.7909235276622,
-177.63619486657));
#162348=CARTESIAN_POINT('Ctrl Pts',(57.8279036918339,-21.8096662565538,
-177.62859626689));
#162349=CARTESIAN_POINT('Ctrl Pts',(57.8250735265724,-21.8281360946975,
-177.620340114691));
#162350=CARTESIAN_POINT('Ctrl Pts',(57.825000507433,-21.8286126222366,-177.62012710341));
#162351=CARTESIAN_POINT('Ctrl Pts',(57.8249275065196,-21.8290889901148,
-177.619913645942));
#162352=CARTESIAN_POINT('Ctrl Pts',(57.8248545239147,-21.8295651979082,
-177.619699742645));
#162353=CARTESIAN_POINT('Ctrl Pts',(57.8134041423538,-21.904278356602,-177.58614004201));
#162354=CARTESIAN_POINT('Ctrl Pts',(57.8024908179688,-21.9744875656816,
-177.541849255809));
#162355=CARTESIAN_POINT('Ctrl Pts',(57.7925715206938,-22.0376966071709,
-177.489169880472));
#162356=CARTESIAN_POINT('Ctrl Pts',(57.7867917707715,-22.0745270844222,
-177.458474801268));
#162357=CARTESIAN_POINT('Ctrl Pts',(57.7813493744923,-22.1089817246111,
-177.424931754292));
#162358=CARTESIAN_POINT('Ctrl Pts',(57.776333363324,-22.1405749184086,-177.389003065334));
#162359=CARTESIAN_POINT('Ctrl Pts',(57.7762581999322,-22.1410483327462,
-177.388464684929));
#162360=CARTESIAN_POINT('Ctrl Pts',(57.7761831269836,-22.141521141353,-177.387925738145));
#162361=CARTESIAN_POINT('Ctrl Pts',(57.7761081445995,-22.1419933437069,
-177.387386226876));
#162362=CARTESIAN_POINT('Ctrl Pts',(57.7675362470193,-22.1959749590559,
-177.325709935871));
#162363=CARTESIAN_POINT('Ctrl Pts',(57.7601479409397,-22.2420339156115,
-177.256653403133));
#162364=CARTESIAN_POINT('Ctrl Pts',(57.754120051989,-22.2794160573152,-177.182965839566));
#162365=CARTESIAN_POINT('Ctrl Pts',(57.7505729125365,-22.3014137534806,
-177.139604048062));
#162366=CARTESIAN_POINT('Ctrl Pts',(57.7474968850881,-22.3204065587762,
-177.094637483872));
#162367=CARTESIAN_POINT('Ctrl Pts',(57.7449284196372,-22.3362374915981,
-177.048618868861));
#162368=CARTESIAN_POINT('Ctrl Pts',(57.7449026192307,-22.3363965143726,
-177.048156608808));
#162369=CARTESIAN_POINT('Ctrl Pts',(57.7448768691533,-22.3365552239542,
-177.047694236815));
#162370=CARTESIAN_POINT('Ctrl Pts',(57.7448511693847,-22.3367136204909,
-177.04723175335));
#162371=CARTESIAN_POINT('Ctrl Pts',(57.7426315058001,-22.3503941726404,
-177.007287514071));
#162372=CARTESIAN_POINT('Ctrl Pts',(57.740792620676,-22.3617057222206,-176.966623027288));
#162373=CARTESIAN_POINT('Ctrl Pts',(57.7393137106679,-22.3707907309251,
-176.925440939058));
#162374=CARTESIAN_POINT('Ctrl Pts',(57.7377438892451,-22.3804342124164,
-176.881727309435));
#162375=CARTESIAN_POINT('Ctrl Pts',(57.7365796223128,-22.3875691725098,
-176.837429305389));
#162376=CARTESIAN_POINT('Ctrl Pts',(57.7358055387825,-22.3923071177908,
-176.792774052489));
#162377=CARTESIAN_POINT('Ctrl Pts',(57.7350314552522,-22.3970450630717,
-176.748118799589));
#162378=CARTESIAN_POINT('Ctrl Pts',(57.7346476057222,-22.3993856132206,
-176.703104836952));
#162379=CARTESIAN_POINT('Ctrl Pts',(57.7346476057222,-22.3993856132206,
-176.657965001855));
#162380=CARTESIAN_POINT('Ctrl Pts',(58.1799818947148,-21.5006430233976,
-177.238261718413));
#162381=CARTESIAN_POINT('Ctrl Pts',(57.8810878095005,-21.4545317502846,
-177.368333266163));
#162382=CARTESIAN_POINT('Ctrl Pts',(57.8819282087167,-21.4487963148739,
-177.697497252237));
#162383=CARTESIAN_POINT('Ctrl Pts',(58.2008748005355,-21.3341357689658,
-177.236799145875));
#162384=CARTESIAN_POINT('Ctrl Pts',(57.9052384907138,-21.2898253143233,
-177.368094235677));
#162385=CARTESIAN_POINT('Ctrl Pts',(57.906096697535,-21.2838546967462,-177.694536471641));
#162386=CARTESIAN_POINT('Ctrl Pts',(58.2211580737071,-21.1675764425398,
-177.235439894836));
#162387=CARTESIAN_POINT('Ctrl Pts',(57.9287492734302,-21.1245836426315,
-177.367866070024));
#162388=CARTESIAN_POINT('Ctrl Pts',(57.9295599753438,-21.1188110827801,
-177.691677811931));
#162389=CARTESIAN_POINT('Ctrl Pts',(58.2408316684984,-21.0009616906551,
-177.234173073119));
#162390=CARTESIAN_POINT('Ctrl Pts',(57.9515978527783,-20.958891271667,-177.367648026607));
#162391=CARTESIAN_POINT('Ctrl Pts',(57.952317989407,-20.9536655363853,-177.688917160843));
#162392=CARTESIAN_POINT('',(57.9523179894071,-20.9536655363849,-177.688917160843));
#162393=CARTESIAN_POINT('Origin',(1.12335876888057,-12.987558319356,-185.751570788792));
#162394=CARTESIAN_POINT('Origin',(58.4476369465814,-21.0219233613115,-177.688917160843));
#162395=CARTESIAN_POINT('Ctrl Pts',(58.0841784519436,-19.9304621405658,
-176.259519378371));
#162396=CARTESIAN_POINT('Ctrl Pts',(58.0105886540739,-20.5442112516041,
-176.323704335026));
#162397=CARTESIAN_POINT('Ctrl Pts',(58.6287087693006,-20.4848108664684,
-176.310034217439));
#162398=CARTESIAN_POINT('Ctrl Pts',(58.0887038582403,-19.8911762730753,
-176.615064002266));
#162399=CARTESIAN_POINT('Ctrl Pts',(58.0268439039754,-20.4108954967624,
-176.520977425154));
#162400=CARTESIAN_POINT('Ctrl Pts',(58.5368873558551,-20.4653641571308,
-176.572149418256));
#162401=CARTESIAN_POINT('Ctrl Pts',(58.0801409030891,-19.9672777568629,
-176.996564457697));
#162402=CARTESIAN_POINT('Ctrl Pts',(58.0299460242795,-20.3808131077243,
-176.814822746134));
#162403=CARTESIAN_POINT('Ctrl Pts',(58.4542388827497,-20.504002186848,-176.810590092819));
#162404=CARTESIAN_POINT('Ctrl Pts',(58.0411746905458,-20.2805473548039,
-177.404658872083));
#162405=CARTESIAN_POINT('Ctrl Pts',(58.0083595382399,-20.5404571645344,
-177.132443882723));
#162406=CARTESIAN_POINT('Ctrl Pts',(58.3544824851918,-20.6619976365417,
-177.058899043469));
#162407=CARTESIAN_POINT('Ctrl Pts',(58.0268899075637,-20.3936565135702,
-177.503861519498));
#162408=CARTESIAN_POINT('Ctrl Pts',(57.9996775864985,-20.6054116810074,
-177.21060993225));
#162409=CARTESIAN_POINT('Ctrl Pts',(58.3280900169859,-20.7190107839085,
-177.1181514199));
#162410=CARTESIAN_POINT('Ctrl Pts',(57.9855747517757,-20.7107497140498,
-177.674988342283));
#162411=CARTESIAN_POINT('Ctrl Pts',(57.9736028397066,-20.7986778387088,
-177.34726402373));
#162412=CARTESIAN_POINT('Ctrl Pts',(58.2701722703655,-20.8787887637927,
-177.221713795304));
#162413=CARTESIAN_POINT('Ctrl Pts',(57.9575440958208,-20.9188769733095,
-177.71328609301));
#162414=CARTESIAN_POINT('Ctrl Pts',(57.9549784509418,-20.9354291942737,
-177.38433863335));
#162415=CARTESIAN_POINT('Ctrl Pts',(58.243188774626,-20.9835514316547,-177.246401767638));
#162416=CARTESIAN_POINT('Ctrl Pts',(57.9264125504997,-21.1393961655747,
-177.673640454257));
#162417=CARTESIAN_POINT('Ctrl Pts',(57.9348086722084,-21.0798758079841,
-177.36100914447));
#162418=CARTESIAN_POINT('Ctrl Pts',(58.2231123045576,-21.0947564262227,
-177.22865633177));
#162419=CARTESIAN_POINT('',(58.0853233553176,-19.9205720538986,-176.438901946458));
#162420=CARTESIAN_POINT('Ctrl Pts',(58.0853233553176,-19.9205720538985,
-176.438901946458));
#162421=CARTESIAN_POINT('Ctrl Pts',(58.0853233553176,-19.9205720538985,
-176.480417501913));
#162422=CARTESIAN_POINT('Ctrl Pts',(58.0851376391211,-19.9221605933746,
-176.521365344842));
#162423=CARTESIAN_POINT('Ctrl Pts',(58.0847722160181,-19.9252576141166,
-176.561736215164));
#162424=CARTESIAN_POINT('Ctrl Pts',(58.0844515754477,-19.9279750955489,
-176.597159642919));
#162425=CARTESIAN_POINT('Ctrl Pts',(58.08399251563,-19.9318546494952,-176.632139799579));
#162426=CARTESIAN_POINT('Ctrl Pts',(58.0833958455804,-19.9368720425748,
-176.666683991487));
#162427=CARTESIAN_POINT('Ctrl Pts',(58.0826836629924,-19.9428607795499,
-176.707915777809));
#162428=CARTESIAN_POINT('Ctrl Pts',(58.0817755947734,-19.9504692662353,
-176.7485257386));
#162429=CARTESIAN_POINT('Ctrl Pts',(58.0806675194151,-19.9597044874771,
-176.788520564059));
#162430=CARTESIAN_POINT('Ctrl Pts',(58.0804191620121,-19.9617744148938,
-176.797484765736));
#162431=CARTESIAN_POINT('Ctrl Pts',(58.0801607337195,-19.9639262624655,
-176.806418007041));
#162432=CARTESIAN_POINT('Ctrl Pts',(58.0798921481857,-19.9661604475892,
-176.815320243471));
#162433=CARTESIAN_POINT('Ctrl Pts',(58.0797944403183,-19.9669732146084,
-176.818558759425));
#162434=CARTESIAN_POINT('Ctrl Pts',(58.0796953880843,-19.9677968794911,
-176.821793172049));
#162435=CARTESIAN_POINT('Ctrl Pts',(58.079594986812,-19.9686314666135,-176.825023478714));
#162436=CARTESIAN_POINT('Ctrl Pts',(58.0795419300216,-19.9690725020011,
-176.826730525844));
#162437=CARTESIAN_POINT('Ctrl Pts',(58.0794884363611,-19.9695170872346,
-176.828438329814));
#162438=CARTESIAN_POINT('Ctrl Pts',(58.0794346961384,-19.96996363886,-176.8301408435));
#162439=CARTESIAN_POINT('Ctrl Pts',(58.0791314907293,-19.9724831086644,
-176.839746523066));
#162440=CARTESIAN_POINT('Ctrl Pts',(58.0788279335445,-19.9750029926094,
-176.848964250386));
#162441=CARTESIAN_POINT('Ctrl Pts',(58.0785049287239,-19.9776815321688,
-176.858384082359));
#162442=CARTESIAN_POINT('Ctrl Pts',(58.0782649644311,-19.979671452474,-176.865382192523));
#162443=CARTESIAN_POINT('Ctrl Pts',(58.0780141570239,-19.9817498314461,
-176.872491632651));
#162444=CARTESIAN_POINT('Ctrl Pts',(58.077742468928,-19.9839993345726,-176.879948694056));
#162445=CARTESIAN_POINT('Ctrl Pts',(58.0776814788505,-19.9845043157327,
-176.881622697295));
#162446=CARTESIAN_POINT('Ctrl Pts',(58.0776192226438,-19.9850196879432,
-176.883319688304));
#162447=CARTESIAN_POINT('Ctrl Pts',(58.0775567873286,-19.98553644744,-176.885009630243));
#162448=CARTESIAN_POINT('Ctrl Pts',(58.0760209778769,-19.9982479091728,
-176.926579514123));
#162449=CARTESIAN_POINT('Ctrl Pts',(58.0742695942654,-20.01268646212,-176.966883058534));
#162450=CARTESIAN_POINT('Ctrl Pts',(58.0723050521356,-20.0288060439935,
-177.005937009045));
#162451=CARTESIAN_POINT('Ctrl Pts',(58.0703050747586,-20.0452163813369,
-177.045695391583));
#162452=CARTESIAN_POINT('Ctrl Pts',(58.0680841820432,-20.0633690707768,
-177.084159548166));
#162453=CARTESIAN_POINT('Ctrl Pts',(58.0656387397512,-20.0832683280962,
-177.121336601679));
#162454=CARTESIAN_POINT('Ctrl Pts',(58.0640588170965,-20.0961246067136,
-177.145355516077));
#162455=CARTESIAN_POINT('Ctrl Pts',(58.062385084809,-20.1097106147667,-177.16883614858));
#162456=CARTESIAN_POINT('Ctrl Pts',(58.0606154075581,-20.1240370308985,
-177.19177397913));
#162457=CARTESIAN_POINT('Ctrl Pts',(58.0596819789832,-20.1315935987333,
-177.203872697396));
#162458=CARTESIAN_POINT('Ctrl Pts',(58.0587426302185,-20.1391881554284,
-177.215558619911));
#162459=CARTESIAN_POINT('Ctrl Pts',(58.0577743364992,-20.1470064780078,
-177.227139348827));
#162460=CARTESIAN_POINT('Ctrl Pts',(58.056830585,-20.1546266386137,-177.23842655441));
#162461=CARTESIAN_POINT('Ctrl Pts',(58.0558593277325,-20.1624594678433,
-177.249613960001));
#162462=CARTESIAN_POINT('Ctrl Pts',(58.0548338958529,-20.1707182132201,
-177.260961622157));
#162463=CARTESIAN_POINT('Ctrl Pts',(58.0541858470239,-20.1759375460464,
-177.268133077734));
#162464=CARTESIAN_POINT('Ctrl Pts',(58.0535160584687,-20.181327777909,-177.275368058178));
#162465=CARTESIAN_POINT('Ctrl Pts',(58.0528166218735,-20.1869517239637,
-177.282726277947));
#162466=CARTESIAN_POINT('Ctrl Pts',(58.0527562346118,-20.1874372786291,
-177.283361564613));
#162467=CARTESIAN_POINT('Ctrl Pts',(58.052695768784,-20.1879234298963,-177.283996259984));
#162468=CARTESIAN_POINT('Ctrl Pts',(58.0526352243748,-20.1884101777465,
-177.28463036415));
#162469=CARTESIAN_POINT('Ctrl Pts',(58.0495306484098,-20.2133694712422,
-177.317145745527));
#162470=CARTESIAN_POINT('Ctrl Pts',(58.0462539781284,-20.2395848887864,
-177.347770869852));
#162471=CARTESIAN_POINT('Ctrl Pts',(58.0428045171782,-20.2670162191791,
-177.376559123591));
#162472=CARTESIAN_POINT('Ctrl Pts',(58.0397672394745,-20.2911697229848,
-177.401907409157));
#162473=CARTESIAN_POINT('Ctrl Pts',(58.0365959190527,-20.3162667107182,
-177.425831470904));
#162474=CARTESIAN_POINT('Ctrl Pts',(58.0332867315621,-20.3423070408666,
-177.448348708029));
#162475=CARTESIAN_POINT('Ctrl Pts',(58.029716355988,-20.3704026863883,-177.472643189274));
#162476=CARTESIAN_POINT('Ctrl Pts',(58.0259860234872,-20.3995923819501,
-177.495296637396));
#162477=CARTESIAN_POINT('Ctrl Pts',(58.0220887490277,-20.4298923026491,
-177.516296202654));
#162478=CARTESIAN_POINT('Ctrl Pts',(58.0205742820626,-20.4416667438437,
-177.524456558871));
#162479=CARTESIAN_POINT('Ctrl Pts',(58.0190626232285,-20.4533913856618,
-177.532220439175));
#162480=CARTESIAN_POINT('Ctrl Pts',(58.0175217099449,-20.4653139806825,
-177.539766005896));
#162481=CARTESIAN_POINT('Ctrl Pts',(58.0160111045326,-20.4770020729061,
-177.547163160588));
#162482=CARTESIAN_POINT('Ctrl Pts',(58.0144723753573,-20.4888805286016,
-177.554350567559));
#162483=CARTESIAN_POINT('Ctrl Pts',(58.0128709932783,-20.5012113818323,
-177.561456314767));
#162484=CARTESIAN_POINT('Ctrl Pts',(58.0119022679131,-20.5086706949185,
-177.565754800212));
#162485=CARTESIAN_POINT('Ctrl Pts',(58.0109105339349,-20.516296094051,-177.570022646716));
#162486=CARTESIAN_POINT('Ctrl Pts',(58.0098873447433,-20.5241507522577,
-177.574280477352));
#162487=CARTESIAN_POINT('Ctrl Pts',(58.0098166280059,-20.5246936194092,
-177.574574753224));
#162488=CARTESIAN_POINT('Ctrl Pts',(58.0097458731121,-20.525236720801,-177.574868509872));
#162489=CARTESIAN_POINT('Ctrl Pts',(58.0096750800606,-20.5257800563078,
-177.575161747436));
#162490=CARTESIAN_POINT('Ctrl Pts',(58.0048770914619,-20.5626045399239,
-177.595035879935));
#162491=CARTESIAN_POINT('Ctrl Pts',(57.9999760159288,-20.5999426940359,
-177.612257905606));
#162492=CARTESIAN_POINT('Ctrl Pts',(57.9949733613778,-20.6377651830716,
-177.626891543277));
#162493=CARTESIAN_POINT('Ctrl Pts',(57.9900036151859,-20.6753388689884,
-177.641428918254));
#162494=CARTESIAN_POINT('Ctrl Pts',(57.9849335849506,-20.7133909289184,
-177.653412127068));
#162495=CARTESIAN_POINT('Ctrl Pts',(57.9797608952366,-20.7519186238698,
-177.662859907759));
#162496=CARTESIAN_POINT('Ctrl Pts',(57.9746750259199,-20.7897996552932,
-177.672149113294));
#162497=CARTESIAN_POINT('Ctrl Pts',(57.9694898790257,-20.8281408458448,
-177.678987476667));
#162498=CARTESIAN_POINT('Ctrl Pts',(57.9642000006941,-20.8669592766756,
-177.683347065177));
#162499=CARTESIAN_POINT('Ctrl Pts',(57.9602974573845,-20.8955971012205,
-177.686563298501));
#162500=CARTESIAN_POINT('Ctrl Pts',(57.9563378466394,-20.9244950860455,
-177.688429530829));
#162501=CARTESIAN_POINT('Ctrl Pts',(57.9523179894072,-20.9536655363841,
-177.688917160843));
#162502=CARTESIAN_POINT('',(58.5817791104913,-20.48000002,-176.438901946458));
#162503=CARTESIAN_POINT('Origin',(58.5817791104913,-19.98000002,-176.438901946458));
#162504=CARTESIAN_POINT('Ctrl Pts',(58.2408316684982,-21.000961690655,-177.234173073119));
#162505=CARTESIAN_POINT('Ctrl Pts',(58.2576191604414,-20.9259549021678,
-177.229990785726));
#162506=CARTESIAN_POINT('Ctrl Pts',(58.2811129081519,-20.8454420300561,
-177.203239464309));
#162507=CARTESIAN_POINT('Ctrl Pts',(58.3217884188213,-20.7363693827747,
-177.127664840087));
#162508=CARTESIAN_POINT('Ctrl Pts',(58.3362806968749,-20.7020244820194,
-177.096770053335));
#162509=CARTESIAN_POINT('Ctrl Pts',(58.3592272802903,-20.6555911910452,
-177.043321716498));
#162510=CARTESIAN_POINT('Ctrl Pts',(58.3670808352308,-20.6409521412524,
-177.024331107606));
#162511=CARTESIAN_POINT('Ctrl Pts',(58.379170673949,-20.6204149031061,-176.994325460603));
#162512=CARTESIAN_POINT('Ctrl Pts',(58.3852932151404,-20.6105004973145,
-176.978943105286));
#162513=CARTESIAN_POINT('Ctrl Pts',(58.3915345498872,-20.6011376986809,
-176.963039016323));
#162514=CARTESIAN_POINT('Ctrl Pts',(58.3957222043316,-20.5950199469896,
-176.952325670182));
#162515=CARTESIAN_POINT('Ctrl Pts',(58.3983722576607,-20.591272141354,-176.945514912726));
#162516=CARTESIAN_POINT('Ctrl Pts',(58.450443842201,-20.5192322826388,-176.81134072458));
#162517=CARTESIAN_POINT('Ctrl Pts',(58.5136487505111,-20.4800032267732,
-176.633649218076));
#162518=CARTESIAN_POINT('Ctrl Pts',(58.5817791104913,-20.48000002,-176.438901946458));
#162519=CARTESIAN_POINT('Origin',(0.,-12.9675000200281,-171.871644662643));
#162520=CARTESIAN_POINT('',(58.4843989875811,-14.3184534098307,-171.871644662643));
#162521=CARTESIAN_POINT('',(58.0853233553176,-19.9205720538986,-171.871644662643));
#162522=CARTESIAN_POINT('Origin',(0.,-12.9675000200281,-171.871644662643));
#162523=CARTESIAN_POINT('Origin',(56.9993922208425,-14.3352334529356,-171.97869344348));
#162524=CARTESIAN_POINT('Origin',(56.6288585600676,-20.00413998012,-171.968919992346));
#162525=CARTESIAN_POINT('Ctrl Pts',(58.4988784725361,-13.3298521511415,
-177.625121132168));
#162526=CARTESIAN_POINT('Ctrl Pts',(58.4984400659509,-13.3300368724616,
-177.363350721044));
#162527=CARTESIAN_POINT('Ctrl Pts',(58.7133155825256,-13.3314748983277,
-177.213850156091));
#162528=CARTESIAN_POINT('Ctrl Pts',(58.4979162725433,-13.485191578753,-177.625232807249));
#162529=CARTESIAN_POINT('Ctrl Pts',(58.4977839239423,-13.43598157919,-177.363622380296));
#162530=CARTESIAN_POINT('Ctrl Pts',(58.712578798724,-13.4097305125617,-177.214081551648));
#162531=CARTESIAN_POINT('Ctrl Pts',(58.4962858223951,-13.6398775654542,
-177.579193599722));
#162532=CARTESIAN_POINT('Ctrl Pts',(58.4968545902725,-13.5420809464769,
-177.326105364235));
#162533=CARTESIAN_POINT('Ctrl Pts',(58.7189266696638,-13.4876555148705,
-177.186196932532));
#162534=CARTESIAN_POINT('Ctrl Pts',(58.4926514029654,-13.9041359548645,
-177.416655260997));
#162535=CARTESIAN_POINT('Ctrl Pts',(58.4950669867845,-13.7147773263519,
-177.195381605071));
#162536=CARTESIAN_POINT('Ctrl Pts',(58.7446596953841,-13.6207725574733,
-177.084964984215));
#162537=CARTESIAN_POINT('Ctrl Pts',(58.4906746501567,-14.0153382250041,
-177.30007538425));
#162538=CARTESIAN_POINT('Ctrl Pts',(58.4942174562181,-13.7830844191732,
-177.100284844236));
#162539=CARTESIAN_POINT('Ctrl Pts',(58.7642460079756,-13.6767862384015,
-177.011404867089));
#162540=CARTESIAN_POINT('Ctrl Pts',(58.4858641857367,-14.264167834758,-176.902914238843));
#162541=CARTESIAN_POINT('Ctrl Pts',(58.4926218253665,-13.9162949426866,
-176.774744028082));
#162542=CARTESIAN_POINT('Ctrl Pts',(58.8384701265889,-13.8021130095289,
-176.749843894667));
#162543=CARTESIAN_POINT('Ctrl Pts',(58.4843734141373,-14.3196187432775,
-176.581150226222));
#162544=CARTESIAN_POINT('Ctrl Pts',(58.4931402301446,-13.8979533027039,
-176.507351292119));
#162545=CARTESIAN_POINT('Ctrl Pts',(58.9093648689647,-13.8300000199992,
-176.524836788664));
#162546=CARTESIAN_POINT('Ctrl Pts',(58.4843714753642,-14.3197132046691,
-176.2719717603));
#162547=CARTESIAN_POINT('Ctrl Pts',(58.4944487865147,-13.8300000200033,
-176.271971760298));
#162548=CARTESIAN_POINT('Ctrl Pts',(58.9842656455913,-13.83000002,-176.271971760298));
#162549=CARTESIAN_POINT('',(58.4988777713114,-13.3298527448197,-177.624285947696));
#162550=CARTESIAN_POINT('Origin',(58.9988681796133,-13.3329497766555,-177.624285947696));
#162551=CARTESIAN_POINT('',(58.984265645584,-13.8300000195596,-176.2719717603));
#162552=CARTESIAN_POINT('Ctrl Pts',(58.984265645584,-13.83000002,-176.2719717603));
#162553=CARTESIAN_POINT('Ctrl Pts',(58.9679069037307,-13.83000002,-176.327198874233));
#162554=CARTESIAN_POINT('Ctrl Pts',(58.9517045549244,-13.8286735475642,
-176.380696852843));
#162555=CARTESIAN_POINT('Ctrl Pts',(58.9359530227723,-13.8258115631793,
-176.43234588609));
#162556=CARTESIAN_POINT('Ctrl Pts',(58.9219297356961,-13.8232635933533,
-176.478328030139));
#162557=CARTESIAN_POINT('Ctrl Pts',(58.9082644377509,-13.8194986722545,
-176.522845347178));
#162558=CARTESIAN_POINT('Ctrl Pts',(58.8951729075458,-13.814331864178,-176.565820637321));
#162559=CARTESIAN_POINT('Ctrl Pts',(58.893559493195,-13.8136951011589,-176.571116958589));
#162560=CARTESIAN_POINT('Ctrl Pts',(58.8919547470568,-13.8130370072512,
-176.576389834502));
#162561=CARTESIAN_POINT('Ctrl Pts',(58.8903590337597,-13.8123572066797,
-176.581639097253));
#162562=CARTESIAN_POINT('Ctrl Pts',(58.8830872267535,-13.8092592951893,
-176.605560453127));
#162563=CARTESIAN_POINT('Ctrl Pts',(58.8759903846586,-13.8057120618013,
-176.628995175177));
#162564=CARTESIAN_POINT('Ctrl Pts',(58.8690798010049,-13.8016888293515,
-176.651917956065));
#162565=CARTESIAN_POINT('Ctrl Pts',(58.8621692173512,-13.7976655969018,
-176.674840736953));
#162566=CARTESIAN_POINT('Ctrl Pts',(58.8554448348755,-13.7931663671043,
-176.697251516217));
#162567=CARTESIAN_POINT('Ctrl Pts',(58.8489181184766,-13.7881680806183,
-176.719125005848));
#162568=CARTESIAN_POINT('Ctrl Pts',(58.8423914020777,-13.7831697941324,
-176.740998495479));
#162569=CARTESIAN_POINT('Ctrl Pts',(58.8360616849599,-13.777673013475,-176.762332133587));
#162570=CARTESIAN_POINT('Ctrl Pts',(58.8299384580245,-13.7716665856965,
-176.78308775253));
#162571=CARTESIAN_POINT('Ctrl Pts',(58.8268768445568,-13.7686633718073,
-176.793465562002));
#162572=CARTESIAN_POINT('Ctrl Pts',(58.823866884387,-13.7655328586488,-176.803698896827));
#162573=CARTESIAN_POINT('Ctrl Pts',(58.8209097885442,-13.7622749477684,
-176.813782297736));
#162574=CARTESIAN_POINT('Ctrl Pts',(58.8194312406228,-13.7606459923282,
-176.818823998191));
#162575=CARTESIAN_POINT('Ctrl Pts',(58.8179659123987,-13.7589851974192,
-176.82382821912));
#162576=CARTESIAN_POINT('Ctrl Pts',(58.8165139718298,-13.7572926247388,
-176.828794281536));
#162577=CARTESIAN_POINT('Ctrl Pts',(58.8156352418151,-13.7562682615877,
-176.831799795807));
#162578=CARTESIAN_POINT('Ctrl Pts',(58.8149249638452,-13.7554264249111,
-176.834231835516));
#162579=CARTESIAN_POINT('Ctrl Pts',(58.814085451631,-13.75441677938,-176.837108091733));
#162580=CARTESIAN_POINT('Ctrl Pts',(58.8135378235159,-13.7537581704047,
-176.838984322649));
#162581=CARTESIAN_POINT('Ctrl Pts',(58.8129353571127,-13.7530277220208,
-176.841049175964));
#162582=CARTESIAN_POINT('Ctrl Pts',(58.8121984954057,-13.7521196840738,
-176.843577321287));
#162583=CARTESIAN_POINT('Ctrl Pts',(58.8047326216658,-13.7429194547781,
-176.86919245856));
#162584=CARTESIAN_POINT('Ctrl Pts',(58.7976492777345,-13.7328159590292,
-176.893793723174));
#162585=CARTESIAN_POINT('Ctrl Pts',(58.7909628880544,-13.7218493579643,
-176.917269265914));
#162586=CARTESIAN_POINT('Ctrl Pts',(58.7903000239319,-13.7207621694008,
-176.919596545026));
#162587=CARTESIAN_POINT('Ctrl Pts',(58.7896415247005,-13.7196663449181,
-176.921912715834));
#162588=CARTESIAN_POINT('Ctrl Pts',(58.7889873808467,-13.7185618287773,
-176.924217876282));
#162589=CARTESIAN_POINT('Ctrl Pts',(58.7863423110571,-13.7140956517135,
-176.933538930398));
#162590=CARTESIAN_POINT('Ctrl Pts',(58.7837661701099,-13.7094837714519,
-176.942668924438));
#162591=CARTESIAN_POINT('Ctrl Pts',(58.7812577939148,-13.7047306884386,
-176.951606378371));
#162592=CARTESIAN_POINT('Ctrl Pts',(58.778129079127,-13.6988021354804,-176.962754125802));
#162593=CARTESIAN_POINT('Ctrl Pts',(58.7751063849037,-13.6926551088693,
-176.973599905223));
#162594=CARTESIAN_POINT('Ctrl Pts',(58.772182362733,-13.686303335553,-176.984136237167));
#162595=CARTESIAN_POINT('Ctrl Pts',(58.7663343183917,-13.6735997889203,
-177.005208901055));
#162596=CARTESIAN_POINT('Ctrl Pts',(58.7609024431394,-13.6600739570901,
-177.025031703479));
#162597=CARTESIAN_POINT('Ctrl Pts',(58.7559183857717,-13.6458151546945,
-177.04349077111));
#162598=CARTESIAN_POINT('Ctrl Pts',(58.7534263570878,-13.6386857534967,
-177.052720304925));
#162599=CARTESIAN_POINT('Ctrl Pts',(58.7510460967611,-13.6313732492002,
-177.06160869806));
#162600=CARTESIAN_POINT('Ctrl Pts',(58.7487798730375,-13.6238905734078,
-177.070141215375));
#162601=CARTESIAN_POINT('Ctrl Pts',(58.7476467611757,-13.6201492355116,
-177.074407474033));
#162602=CARTESIAN_POINT('Ctrl Pts',(58.7465421602532,-13.6163653600285,
-177.07858476562));
#162603=CARTESIAN_POINT('Ctrl Pts',(58.7454662933704,-13.6125407267456,
-177.082671233078));
#162604=CARTESIAN_POINT('Ctrl Pts',(58.7448786850993,-13.6104518194775,
-177.084903146818));
#162605=CARTESIAN_POINT('Ctrl Pts',(58.744372827281,-13.6086170289023,-177.086828912308));
#162606=CARTESIAN_POINT('Ctrl Pts',(58.7438276832832,-13.6066025097304,
-177.088909271721));
#162607=CARTESIAN_POINT('Ctrl Pts',(58.7433747093129,-13.6049285946708,
-177.090637895106));
#162608=CARTESIAN_POINT('Ctrl Pts',(58.7428946837808,-13.6031304142461,
-177.092473045025));
#162609=CARTESIAN_POINT('Ctrl Pts',(58.7423251299313,-13.6009463862979,
-177.094656337774));
#162610=CARTESIAN_POINT('Ctrl Pts',(58.7384401112559,-13.586048779385,-177.109548929774));
#162611=CARTESIAN_POINT('Ctrl Pts',(58.7349185884774,-13.5704346140225,
-177.123253023635));
#162612=CARTESIAN_POINT('Ctrl Pts',(58.7317901864608,-13.5542149695198,
-177.135582555746));
#162613=CARTESIAN_POINT('Ctrl Pts',(58.7308762483141,-13.5494765274145,
-177.139184531984));
#162614=CARTESIAN_POINT('Ctrl Pts',(58.7299947746698,-13.5446823603777,
-177.142670531144));
#162615=CARTESIAN_POINT('Ctrl Pts',(58.729145971874,-13.5398381541873,-177.146037999423));
#162616=CARTESIAN_POINT('Ctrl Pts',(58.7252281330667,-13.5174786390013,
-177.161581301084));
#162617=CARTESIAN_POINT('Ctrl Pts',(58.7220323680021,-13.4940622836547,
-177.174572918194));
#162618=CARTESIAN_POINT('Ctrl Pts',(58.7195645574954,-13.4700429785437,
-177.184872363911));
#162619=CARTESIAN_POINT('Ctrl Pts',(58.7175984325081,-13.4509066000294,
-177.193078017272));
#162620=CARTESIAN_POINT('Ctrl Pts',(58.716094193839,-13.4313878853066,-177.199575495156));
#162621=CARTESIAN_POINT('Ctrl Pts',(58.7150495463886,-13.4117105994086,
-177.204316500607));
#162622=CARTESIAN_POINT('Ctrl Pts',(58.7137256604449,-13.3867734953148,
-177.210324796013));
#162623=CARTESIAN_POINT('Ctrl Pts',(58.7131400085458,-13.3615857919425,
-177.213511143853));
#162624=CARTESIAN_POINT('Ctrl Pts',(58.7132776892154,-13.3365560747486,
-177.213825716594));
#162625=CARTESIAN_POINT('Ctrl Pts',(58.7132870100049,-13.3348615977753,
-177.21384701273));
#162626=CARTESIAN_POINT('Ctrl Pts',(58.7132996430622,-13.3331678319628,
-177.213855162194));
#162627=CARTESIAN_POINT('Ctrl Pts',(58.7133155825256,-13.3314748983292,
-177.213850156091));
#162628=CARTESIAN_POINT('',(58.4843989875811,-14.3184534098307,-176.2719717603));
#162629=CARTESIAN_POINT('Origin',(58.9842656455946,-14.33000002,-176.2719717603));
#162630=CARTESIAN_POINT('Ctrl Pts',(58.4988777713114,-13.3298527448197,
-177.624285947696));
#162631=CARTESIAN_POINT('Ctrl Pts',(58.4983908181541,-13.4084673412756,
-177.624342719651));
#162632=CARTESIAN_POINT('Ctrl Pts',(58.4974447796673,-13.5228546462299,
-177.608365198208));
#162633=CARTESIAN_POINT('Ctrl Pts',(58.4960362646421,-13.6501200351752,
-177.561615067615));
#162634=CARTESIAN_POINT('Ctrl Pts',(58.4953746377398,-13.7033366219318,
-177.535555792594));
#162635=CARTESIAN_POINT('Ctrl Pts',(58.4949214728157,-13.7385197366069,
-177.516844385966));
#162636=CARTESIAN_POINT('Ctrl Pts',(58.4946730914668,-13.7571080789305,
-177.506112042692));
#162637=CARTESIAN_POINT('Ctrl Pts',(58.4935605637375,-13.8378723566693,
-177.456177551313));
#162638=CARTESIAN_POINT('Ctrl Pts',(58.4921730279003,-13.9270164501794,
-177.384838642241));
#162639=CARTESIAN_POINT('Ctrl Pts',(58.4905865207784,-14.017416254816,-177.281629256011));
#162640=CARTESIAN_POINT('Ctrl Pts',(58.4898144182803,-14.0592159333627,
-177.22502939815));
#162641=CARTESIAN_POINT('Ctrl Pts',(58.4894893930172,-14.0764014812318,
-177.199701923765));
#162642=CARTESIAN_POINT('Ctrl Pts',(58.4892741579113,-14.0876966042115,
-177.182579075853));
#162643=CARTESIAN_POINT('Ctrl Pts',(58.489149697308,-14.0941715098239,-177.172441758713));
#162644=CARTESIAN_POINT('Ctrl Pts',(58.4862281559377,-14.2452242270742,
-176.930144926363));
#162645=CARTESIAN_POINT('Ctrl Pts',(58.4843989875812,-14.3184534098306,
-176.632435702977));
#162646=CARTESIAN_POINT('Ctrl Pts',(58.4843989875811,-14.3184534098307,
-176.2719717603));
#162647=CARTESIAN_POINT('Ctrl Pts',(58.7133155825256,-13.3314748983275,
-177.213850156091));
#162648=CARTESIAN_POINT('Ctrl Pts',(58.4988766126948,-13.3300397939931,
-177.363046991769));
#162649=CARTESIAN_POINT('Ctrl Pts',(58.4988777713114,-13.3298527448209,
-177.624285947696));
#162650=CARTESIAN_POINT('Ctrl Pts',(58.7142076600563,-13.1641303210821,
-177.213830854253));
#162651=CARTESIAN_POINT('Ctrl Pts',(58.4999095201947,-13.1633713364571,
-177.363039299942));
#162652=CARTESIAN_POINT('Ctrl Pts',(58.4999097084608,-13.1632549492482,
-177.624165638205));
#162653=CARTESIAN_POINT('Ctrl Pts',(58.7144845107404,-12.9967863561848,
-177.213824921703));
#162654=CARTESIAN_POINT('Ctrl Pts',(58.5002301876544,-12.9966649765953,
-177.363036914652));
#162655=CARTESIAN_POINT('Ctrl Pts',(58.500229964035,-12.996655767065,-177.624128301462));
#162656=CARTESIAN_POINT('Ctrl Pts',(58.7141461350386,-12.8294402383605,
-177.213832217124));
#162657=CARTESIAN_POINT('Ctrl Pts',(58.4998383709332,-12.8299842764725,
-177.363039831106));
#162658=CARTESIAN_POINT('Ctrl Pts',(58.4998385375645,-12.8300551987823,
-177.624173936067));
#162659=CARTESIAN_POINT('',(58.4998385375645,-12.8300551987823,-177.624173936067));
#162660=CARTESIAN_POINT('Origin',(0.784740066134875,-12.9675005363404,-184.352939507241));
#162661=CARTESIAN_POINT('Origin',(58.9998371575436,-12.8288804567203,-177.624173936068));
#162662=CARTESIAN_POINT('Ctrl Pts',(58.48912660861,-11.8396398505087,-176.26629097911));
#162663=CARTESIAN_POINT('Ctrl Pts',(58.4985823439911,-12.33000002,-176.26629097911));
#162664=CARTESIAN_POINT('Ctrl Pts',(58.9890336736409,-12.33000002,-176.26629097911));
#162665=CARTESIAN_POINT('Ctrl Pts',(58.4891266082067,-11.8396398295935,
-176.423373313634));
#162666=CARTESIAN_POINT('Ctrl Pts',(58.4978924302213,-12.2942221356202,
-176.390394119799));
#162667=CARTESIAN_POINT('Ctrl Pts',(58.9511729872871,-12.33000002,-176.394565470062));
#162668=CARTESIAN_POINT('Ctrl Pts',(58.4893923301638,-11.8529830432079,
-176.578231191384));
#162669=CARTESIAN_POINT('Ctrl Pts',(58.4973632374244,-12.2720420811237,
-176.51680491203));
#162670=CARTESIAN_POINT('Ctrl Pts',(58.9148079297158,-12.3367286443605,
-176.512401023853));
#162671=CARTESIAN_POINT('Ctrl Pts',(58.4906521273108,-11.9211841187055,
-176.880933630382));
#162672=CARTESIAN_POINT('Ctrl Pts',(58.4968786243544,-12.2700692006727,
-176.761217862814));
#162673=CARTESIAN_POINT('Ctrl Pts',(58.8482938287677,-12.3711206280572,
-176.731313674606));
#162674=CARTESIAN_POINT('Ctrl Pts',(58.4916809553489,-11.9775042760042,
-177.031063990607));
#162675=CARTESIAN_POINT('Ctrl Pts',(58.4969059340918,-12.2890138650664,
-176.883349034336));
#162676=CARTESIAN_POINT('Ctrl Pts',(58.817725908538,-12.3995214017445,-176.833790628028));
#162677=CARTESIAN_POINT('Ctrl Pts',(58.4936040475389,-12.1014782716709,
-177.230049861356));
#162678=CARTESIAN_POINT('Ctrl Pts',(58.4973396692349,-12.3546251483512,
-177.045101981496));
#162679=CARTESIAN_POINT('Ctrl Pts',(58.7801197877863,-12.4620381958002,
-176.965157505607));
#162680=CARTESIAN_POINT('Ctrl Pts',(58.494315776837,-12.1502025268642,-177.293200512009));
#162681=CARTESIAN_POINT('Ctrl Pts',(58.4975444264886,-12.3825831770725,
-177.096147908481));
#162682=CARTESIAN_POINT('Ctrl Pts',(58.7686983660461,-12.486608549538,-177.006030037118));
#162683=CARTESIAN_POINT('Ctrl Pts',(58.4957333150688,-12.2588835334819,
-177.404811094274));
#162684=CARTESIAN_POINT('Ctrl Pts',(58.4980148214299,-12.4487602363349,
-177.186076538859));
#162685=CARTESIAN_POINT('Ctrl Pts',(58.7491768361659,-12.5414135007217,
-177.077379300711));
#162686=CARTESIAN_POINT('Ctrl Pts',(58.4964422014533,-12.3189060674576,
-177.453832155185));
#162687=CARTESIAN_POINT('Ctrl Pts',(58.4982801309887,-12.4869468894055,
-177.22572537075));
#162688=CARTESIAN_POINT('Ctrl Pts',(58.7409598721377,-12.5716812769085,
-177.108237839695));
#162689=CARTESIAN_POINT('Ctrl Pts',(58.4984277184057,-12.5184434004461,
-177.577650852379));
#162690=CARTESIAN_POINT('Ctrl Pts',(58.4990784570061,-12.6167275534409,
-177.325053017822));
#162691=CARTESIAN_POINT('Ctrl Pts',(58.7207402303504,-12.6723026604245,
-177.185595547246));
#162692=CARTESIAN_POINT('Ctrl Pts',(58.4994668010734,-12.6718351617763,
-177.624217264241));
#162693=CARTESIAN_POINT('Ctrl Pts',(58.4995844948381,-12.722010160726,-177.363144865678));
#162694=CARTESIAN_POINT('Ctrl Pts',(58.7138612409819,-12.7496539972653,
-177.213921724966));
#162695=CARTESIAN_POINT('Ctrl Pts',(58.4998385375645,-12.8300551987826,
-177.624173936067));
#162696=CARTESIAN_POINT('Ctrl Pts',(58.4998383709333,-12.8299842764724,
-177.363039831107));
#162697=CARTESIAN_POINT('Ctrl Pts',(58.7141461350374,-12.8294402383603,
-177.213832217126));
#162698=CARTESIAN_POINT('',(58.48912660861,-11.8396398505087,-176.26629097911));
#162699=CARTESIAN_POINT('Ctrl Pts',(58.48912660861,-11.8396398505087,-176.26629097911));
#162700=CARTESIAN_POINT('Ctrl Pts',(58.48912660861,-11.8396398505087,-176.409811534268));
#162701=CARTESIAN_POINT('Ctrl Pts',(58.4893483896326,-11.850776103237,-176.551488494012));
#162702=CARTESIAN_POINT('Ctrl Pts',(58.4898674690038,-11.8787272918346,
-176.690381503724));
#162703=CARTESIAN_POINT('Ctrl Pts',(58.4899146582257,-11.8812683191145,
-176.703008191331));
#162704=CARTESIAN_POINT('Ctrl Pts',(58.4899643050978,-11.8839483504648,
-176.715611866645));
#162705=CARTESIAN_POINT('Ctrl Pts',(58.4900164667572,-11.8867716762097,
-176.728191820333));
#162706=CARTESIAN_POINT('Ctrl Pts',(58.4900183886416,-11.8868757010012,
-176.72865532585));
#162707=CARTESIAN_POINT('Ctrl Pts',(58.4900203139396,-11.8869799203049,
-176.72911879896));
#162708=CARTESIAN_POINT('Ctrl Pts',(58.4900222426542,-11.8870843343361,
-176.729582239632));
#162709=CARTESIAN_POINT('Ctrl Pts',(58.4904143757935,-11.9083130858161,
-176.82380584864));
#162710=CARTESIAN_POINT('Ctrl Pts',(58.4909611779827,-11.9381550632001,
-176.917576442103));
#162711=CARTESIAN_POINT('Ctrl Pts',(58.491628008076,-11.9776372784523,-177.007000513355));
#162712=CARTESIAN_POINT('Ctrl Pts',(58.4920261001825,-12.0012078377276,
-177.060385951801));
#162713=CARTESIAN_POINT('Ctrl Pts',(58.4924669768134,-12.0282147910086,
-177.112221932541));
#162714=CARTESIAN_POINT('Ctrl Pts',(58.4929432955759,-12.0588830464209,
-177.16167335862));
#162715=CARTESIAN_POINT('Ctrl Pts',(58.4929498715258,-12.0593064454722,
-177.16235607391));
#162716=CARTESIAN_POINT('Ctrl Pts',(58.4929564542504,-12.0597305436947,
-177.163038337515));
#162717=CARTESIAN_POINT('Ctrl Pts',(58.4929630437302,-12.0601553416844,
-177.163720147168));
#162718=CARTESIAN_POINT('Ctrl Pts',(58.4935968230333,-12.1010126145907,
-177.229296924179));
#162719=CARTESIAN_POINT('Ctrl Pts',(58.4943004033954,-12.1491458631888,
-177.291840545738));
#162720=CARTESIAN_POINT('Ctrl Pts',(58.4950024041184,-12.2028473374637,
-177.347256942163));
#162721=CARTESIAN_POINT('Ctrl Pts',(58.4950097920195,-12.203412495261,-177.347840147912));
#162722=CARTESIAN_POINT('Ctrl Pts',(58.4950171797681,-12.2039782717463,
-177.348422567924));
#162723=CARTESIAN_POINT('Ctrl Pts',(58.4950245672806,-12.2045446649403,
-177.349004197405));
#162724=CARTESIAN_POINT('Ctrl Pts',(58.4957264419677,-12.2583566950054,
-177.404263800622));
#162725=CARTESIAN_POINT('Ctrl Pts',(58.4964292592559,-12.3178002283294,
-177.452938198817));
#162726=CARTESIAN_POINT('Ctrl Pts',(58.4970868450185,-12.3836929510146,
-177.494029767074));
#162727=CARTESIAN_POINT('Ctrl Pts',(58.497092582954,-12.3842679150954,-177.494388322234));
#162728=CARTESIAN_POINT('Ctrl Pts',(58.4970983175096,-12.3848433769923,
-177.494746304328));
#162729=CARTESIAN_POINT('Ctrl Pts',(58.4971040486531,-12.3854193371859,
-177.495103712595));
#162730=CARTESIAN_POINT('Ctrl Pts',(58.4975789393159,-12.4331442135456,
-177.524719067147));
#162731=CARTESIAN_POINT('Ctrl Pts',(58.4980179792089,-12.4835732800606,
-177.549749276722));
#162732=CARTESIAN_POINT('Ctrl Pts',(58.4984026087055,-12.5359391558249,
-177.569640300795));
#162733=CARTESIAN_POINT('Ctrl Pts',(58.4987756724465,-12.5867303969686,
-177.588933204532));
#162734=CARTESIAN_POINT('Ctrl Pts',(58.4990975247222,-12.6393425576463,
-177.603390836161));
#162735=CARTESIAN_POINT('Ctrl Pts',(58.4993516232989,-12.6930550659192,
-177.612550490846));
#162736=CARTESIAN_POINT('Ctrl Pts',(58.499564677447,-12.7380914169331,-177.620230590637));
#162737=CARTESIAN_POINT('Ctrl Pts',(58.4997300980036,-12.7839007002384,
-177.624186575364));
#162738=CARTESIAN_POINT('Ctrl Pts',(58.4998385375645,-12.8300551987823,
-177.624173936067));
#162739=CARTESIAN_POINT('',(58.9890336736409,-12.3300000204739,-176.26629097911));
#162740=CARTESIAN_POINT('Origin',(58.9890336736409,-11.83000002,-176.26629097911));
#162741=CARTESIAN_POINT('Ctrl Pts',(58.7141461350374,-12.8294402383603,
-177.213832217126));
#162742=CARTESIAN_POINT('Ctrl Pts',(58.7140819296199,-12.811459412521,-177.21385238952));
#162743=CARTESIAN_POINT('Ctrl Pts',(58.7143816551427,-12.7933544705259,
-177.212425421223));
#162744=CARTESIAN_POINT('Ctrl Pts',(58.7150632987668,-12.7752997321945,
-177.209516903944));
#162745=CARTESIAN_POINT('Ctrl Pts',(58.7152846118919,-12.7694377972727,
-177.208572579042));
#162746=CARTESIAN_POINT('Ctrl Pts',(58.7155460928643,-12.7635812153741,
-177.207472475417));
#162747=CARTESIAN_POINT('Ctrl Pts',(58.7158480917974,-12.7577360874582,
-177.206216550884));
#162748=CARTESIAN_POINT('Ctrl Pts',(58.716816069541,-12.7390010751397,-177.202191016809));
#162749=CARTESIAN_POINT('Ctrl Pts',(58.7182010244667,-12.7203874846099,
-177.196561750169));
#162750=CARTESIAN_POINT('Ctrl Pts',(58.7200061839669,-12.7020882148015,
-177.189361547879));
#162751=CARTESIAN_POINT('Ctrl Pts',(58.7216704793852,-12.6852169129054,
-177.182723207234));
#162752=CARTESIAN_POINT('Ctrl Pts',(58.723691597054,-12.6686147413198,-177.174751108997));
#162753=CARTESIAN_POINT('Ctrl Pts',(58.7260634953738,-12.6524255210882,
-177.165504848793));
#162754=CARTESIAN_POINT('Ctrl Pts',(58.727449441156,-12.6429658485087,-177.160102081219));
#162755=CARTESIAN_POINT('Ctrl Pts',(58.7289550679102,-12.6336465746835,
-177.154264608281));
#162756=CARTESIAN_POINT('Ctrl Pts',(58.7305781768371,-12.6244942829079,
-177.148008033313));
#162757=CARTESIAN_POINT('Ctrl Pts',(58.7317328456457,-12.6179834038989,
-177.143557147828));
#162758=CARTESIAN_POINT('Ctrl Pts',(58.732946110831,-12.6115611006134,-177.138897443365));
#162759=CARTESIAN_POINT('Ctrl Pts',(58.7342199915419,-12.6052217380805,
-177.134023742212));
#162760=CARTESIAN_POINT('Ctrl Pts',(58.735402267938,-12.5993382368829,-177.129500507198));
#162761=CARTESIAN_POINT('Ctrl Pts',(58.7366319475121,-12.5935452263529,
-177.124813678365));
#162762=CARTESIAN_POINT('Ctrl Pts',(58.7379129452138,-12.5878291335991,
-177.119951431684));
#162763=CARTESIAN_POINT('Ctrl Pts',(58.7387647963682,-12.5840279868799,
-177.116718084393));
#162764=CARTESIAN_POINT('Ctrl Pts',(58.7396386693894,-12.5802640997989,
-177.113409732084));
#162765=CARTESIAN_POINT('Ctrl Pts',(58.7405344197273,-12.5765391217875,
-177.110027828988));
#162766=CARTESIAN_POINT('Ctrl Pts',(58.7407707132952,-12.5755564949246,
-177.10913570323));
#162767=CARTESIAN_POINT('Ctrl Pts',(58.7410085288087,-12.5745765746215,
-177.108238460817));
#162768=CARTESIAN_POINT('Ctrl Pts',(58.74124786267,-12.5735993889851,-177.107336131755));
#162769=CARTESIAN_POINT('Ctrl Pts',(58.7413598187595,-12.5731422790637,
-177.106914038398));
#162770=CARTESIAN_POINT('Ctrl Pts',(58.7414736198389,-12.5726795881164,
-177.106485128439));
#162771=CARTESIAN_POINT('Ctrl Pts',(58.74158951008,-12.5722104964838,-177.106048495697));
#162772=CARTESIAN_POINT('Ctrl Pts',(58.7422420312352,-12.5695692713822,
-177.103590030701));
#162773=CARTESIAN_POINT('Ctrl Pts',(58.7429540566299,-12.5667591487054,
-177.100912580599));
#162774=CARTESIAN_POINT('Ctrl Pts',(58.7436251133995,-12.5641756692348,
-177.098394190095));
#162775=CARTESIAN_POINT('Ctrl Pts',(58.7439823525257,-12.5628003460278,
-177.097053517199));
#162776=CARTESIAN_POINT('Ctrl Pts',(58.7443277438613,-12.5614887596861,
-177.095758708694));
#162777=CARTESIAN_POINT('Ctrl Pts',(58.7446447061254,-12.5602976725631,
-177.09457147636));
#162778=CARTESIAN_POINT('Ctrl Pts',(58.7447641846295,-12.5598486938555,
-177.094123950709));
#162779=CARTESIAN_POINT('Ctrl Pts',(58.744879615129,-12.5594168198056,-177.093691738289));
#162780=CARTESIAN_POINT('Ctrl Pts',(58.7449900830053,-12.5590050376963,
-177.093278230413));
#162781=CARTESIAN_POINT('Ctrl Pts',(58.7450575067238,-12.55875370779,-177.093025847191));
#162782=CARTESIAN_POINT('Ctrl Pts',(58.7451231516292,-12.5585095853754,
-177.092780168902));
#162783=CARTESIAN_POINT('Ctrl Pts',(58.7451895613975,-12.5582631790804,
-177.092531673465));
#162784=CARTESIAN_POINT('Ctrl Pts',(58.7493441098919,-12.5428481742039,
-177.076985973327));
#162785=CARTESIAN_POINT('Ctrl Pts',(58.7539230266605,-12.5280889949087,
-177.060032443229));
#162786=CARTESIAN_POINT('Ctrl Pts',(58.758937601106,-12.5140110251299,-177.041704668915));
#162787=CARTESIAN_POINT('Ctrl Pts',(58.7637684671953,-12.5004488001493,
-177.024048330497));
#162788=CARTESIAN_POINT('Ctrl Pts',(58.7690325800979,-12.4875098220423,
-177.005022325128));
#162789=CARTESIAN_POINT('Ctrl Pts',(58.7746562065322,-12.4753590626234,
-176.984935558188));
#162790=CARTESIAN_POINT('Ctrl Pts',(58.7760519396443,-12.4723433542623,
-176.979950204687));
#162791=CARTESIAN_POINT('Ctrl Pts',(58.7774703718805,-12.469374709313,-176.974897500936));
#162792=CARTESIAN_POINT('Ctrl Pts',(58.7789129322744,-12.4664507071385,
-176.969773145284));
#162793=CARTESIAN_POINT('Ctrl Pts',(58.7832826727381,-12.4575934484255,
-176.954250672645));
#162794=CARTESIAN_POINT('Ctrl Pts',(58.7878685478042,-12.4491565790701,
-176.93808929468));
#162795=CARTESIAN_POINT('Ctrl Pts',(58.7926551613702,-12.4411992644483,
-176.921368546414));
#162796=CARTESIAN_POINT('Ctrl Pts',(58.7932827345557,-12.4401559804613,
-176.919176288128));
#162797=CARTESIAN_POINT('Ctrl Pts',(58.7939144101258,-12.4391199222591,
-176.91697239607));
#162798=CARTESIAN_POINT('Ctrl Pts',(58.7945501814039,-12.4380910843739,
-176.914756880988));
#162799=CARTESIAN_POINT('Ctrl Pts',(58.7979343273103,-12.4326146848608,
-176.902963919341));
#162800=CARTESIAN_POINT('Ctrl Pts',(58.80142242488,-12.4273626370271,-176.89088421705));
#162801=CARTESIAN_POINT('Ctrl Pts',(58.8049977587502,-12.4223299660034,
-176.878537167771));
#162802=CARTESIAN_POINT('Ctrl Pts',(58.8067854256853,-12.4198136304916,
-176.872363643132));
#162803=CARTESIAN_POINT('Ctrl Pts',(58.8085966099864,-12.4173527374792,
-176.866122892953));
#162804=CARTESIAN_POINT('Ctrl Pts',(58.8104321298967,-12.4149474978988,
-176.859816564017));
#162805=CARTESIAN_POINT('Ctrl Pts',(58.8115041159289,-12.4135427824174,
-176.856133522228));
#162806=CARTESIAN_POINT('Ctrl Pts',(58.8127336302357,-12.4119666704472,
-176.851916809599));
#162807=CARTESIAN_POINT('Ctrl Pts',(58.8138602537382,-12.4105555372891,
-176.848059758556));
#162808=CARTESIAN_POINT('Ctrl Pts',(58.8146627037572,-12.409550442129,-176.845312531398));
#162809=CARTESIAN_POINT('Ctrl Pts',(58.8154125443209,-12.408627963248,-176.842748880392));
#162810=CARTESIAN_POINT('Ctrl Pts',(58.8160115760595,-12.4078985515024,
-176.840702677788));
#162811=CARTESIAN_POINT('Ctrl Pts',(58.8244081864246,-12.397674408391,-176.812021115717));
#162812=CARTESIAN_POINT('Ctrl Pts',(58.8333248152985,-12.3884835890777,
-176.78188929717));
#162813=CARTESIAN_POINT('Ctrl Pts',(58.8426847877196,-12.3803541547745,
-176.750536379343));
#162814=CARTESIAN_POINT('Ctrl Pts',(58.8525227202813,-12.371809596859,-176.717582447717));
#162815=CARTESIAN_POINT('Ctrl Pts',(58.8628503464016,-12.3644376787052,
-176.68327982788));
#162816=CARTESIAN_POINT('Ctrl Pts',(58.8735611615879,-12.3582406628378,
-176.647940399611));
#162817=CARTESIAN_POINT('Ctrl Pts',(58.8761776845034,-12.3567268066333,
-176.639307403683));
#162818=CARTESIAN_POINT('Ctrl Pts',(58.8788170008591,-12.3552829261018,
-176.630612725113));
#162819=CARTESIAN_POINT('Ctrl Pts',(58.8814774221998,-12.3539087910943,
-176.62186125809));
#162820=CARTESIAN_POINT('Ctrl Pts',(58.8939117687074,-12.3474863231306,
-176.580958423731));
#162821=CARTESIAN_POINT('Ctrl Pts',(58.9068669263435,-12.3424881234721,
-176.538617876985));
#162822=CARTESIAN_POINT('Ctrl Pts',(58.9202241992701,-12.3387709208172,
-176.494828120573));
#162823=CARTESIAN_POINT('Ctrl Pts',(58.9340586940389,-12.3349209118397,
-176.449473866052));
#162824=CARTESIAN_POINT('Ctrl Pts',(58.9483242256657,-12.3324443653281,
-176.402564210775));
#162825=CARTESIAN_POINT('Ctrl Pts',(58.962873779728,-12.331138362007,-176.354117959566));
#162826=CARTESIAN_POINT('Ctrl Pts',(58.9715048174126,-12.3303636190952,
-176.325378836835));
#162827=CARTESIAN_POINT('Ctrl Pts',(58.9802355398853,-12.33000002,-176.296099633879));
#162828=CARTESIAN_POINT('Ctrl Pts',(58.9890336736409,-12.33000002,-176.26629097911));
#162829=CARTESIAN_POINT('Origin',(0.,-12.9675000200281,-171.871644662643));
#162830=CARTESIAN_POINT('',(58.1115942404669,-6.23752120644091,-171.871644662643));
#162831=CARTESIAN_POINT('',(58.48912660861,-11.8396398505087,-171.871644662643));
#162832=CARTESIAN_POINT('Origin',(0.,-12.9675000200281,-171.871644662643));
#162833=CARTESIAN_POINT('Origin',(56.6526047464346,-6.15642511055022,-171.969110145006));
#162834=CARTESIAN_POINT('Origin',(57.0042957475178,-11.8256297436875,-171.97932653822));
#162835=CARTESIAN_POINT('Ctrl Pts',(57.9826110754301,-5.20432973493148,
-177.68524973918));
#162836=CARTESIAN_POINT('Ctrl Pts',(57.9819403936437,-5.19932045653773,
-177.367360689002));
#162837=CARTESIAN_POINT('Ctrl Pts',(58.267019098174,-5.15898893607643,-177.232518219478));
#162838=CARTESIAN_POINT('Ctrl Pts',(58.0025119651788,-5.35296817875971,
-177.682845100084));
#162839=CARTESIAN_POINT('Ctrl Pts',(57.9949888374176,-5.2966803543509,-177.360992500472));
#162840=CARTESIAN_POINT('Ctrl Pts',(58.2832677496941,-5.23392550092992,
-177.228417054074));
#162841=CARTESIAN_POINT('Ctrl Pts',(58.0218092186127,-5.50176990585681,
-177.64204201157));
#162842=CARTESIAN_POINT('Ctrl Pts',(58.0077051406755,-5.39303977887496,
-177.325226539032));
#162843=CARTESIAN_POINT('Ctrl Pts',(58.3041451880796,-5.30898013469752,
-177.202784454736));
#162844=CARTESIAN_POINT('Ctrl Pts',(58.0549536715593,-5.76404075854571,
-177.499799765465));
#162845=CARTESIAN_POINT('Ctrl Pts',(58.0288513197851,-5.5545561633354,-177.210890020253));
#162846=CARTESIAN_POINT('Ctrl Pts',(58.3514580290103,-5.44123637401812,
-177.116293661504));
#162847=CARTESIAN_POINT('Ctrl Pts',(58.0690822624578,-5.87947228735883,
-177.397969070777));
#162848=CARTESIAN_POINT('Ctrl Pts',(58.0375028694103,-5.62129124259478,
-177.130382190313));
#162849=CARTESIAN_POINT('Ctrl Pts',(58.3782554149277,-5.49944543725108,
-177.055134470277));
#162850=CARTESIAN_POINT('Ctrl Pts',(58.0910734645313,-6.0620213485957,-177.158256835825));
#162851=CARTESIAN_POINT('Ctrl Pts',(58.049471160706,-5.71257363005819,-176.947755762969));
#162852=CARTESIAN_POINT('Ctrl Pts',(58.4364471667621,-5.59150009130694,
-176.908395287787));
#162853=CARTESIAN_POINT('Ctrl Pts',(58.0990088104622,-6.12958052854701,
-177.021022282342));
#162854=CARTESIAN_POINT('Ctrl Pts',(58.0527451569459,-5.73669128650856,
-176.84391309495));
#162855=CARTESIAN_POINT('Ctrl Pts',(58.4678181796127,-5.62556839623242,
-176.823203787185));
#162856=CARTESIAN_POINT('Ctrl Pts',(58.1093120435936,-6.21769842661734,
-176.729452616794));
#162857=CARTESIAN_POINT('Ctrl Pts',(58.0539894201321,-5.74161490543249,
-176.632064657874));
#162858=CARTESIAN_POINT('Ctrl Pts',(58.5354785511785,-5.67000391722627,
-176.63504101192));
#162859=CARTESIAN_POINT('Ctrl Pts',(58.1115942412421,-6.23752121313465,
-176.57952555449));
#162860=CARTESIAN_POINT('Ctrl Pts',(58.0517037498764,-5.72038259956876,
-176.525060913865));
#162861=CARTESIAN_POINT('Ctrl Pts',(58.5707923905479,-5.68000002000002,
-176.534945859098));
#162862=CARTESIAN_POINT('Ctrl Pts',(58.1115942404669,-6.2375212064409,-176.427328712824));
#162863=CARTESIAN_POINT('Ctrl Pts',(58.0470269915055,-5.68000001999982,
-176.427328712824));
#162864=CARTESIAN_POINT('Ctrl Pts',(58.6082745331206,-5.68000001999999,
-176.427328712824));
#162865=CARTESIAN_POINT('',(57.9826110754301,-5.20432973493148,-177.68524973918));
#162866=CARTESIAN_POINT('Origin',(58.4781889478697,-5.13797785215286,-177.68524973918));
#162867=CARTESIAN_POINT('',(58.6082745331212,-5.68000001999999,-176.427328712824));
#162868=CARTESIAN_POINT('Ctrl Pts',(58.6082745331206,-5.68000001999999,
-176.427328712824));
#162869=CARTESIAN_POINT('Ctrl Pts',(58.5970324095344,-5.68000002,-176.459606623727));
#162870=CARTESIAN_POINT('Ctrl Pts',(58.5859083959314,-5.67909758005478,
-176.491428394012));
#162871=CARTESIAN_POINT('Ctrl Pts',(58.5749508380644,-5.67721411211561,
-176.522640354069));
#162872=CARTESIAN_POINT('Ctrl Pts',(58.5641075990386,-5.67535029416368,
-176.553526683621));
#162873=CARTESIAN_POINT('Ctrl Pts',(58.5534272139788,-5.67252542423281,
-176.583816198249));
#162874=CARTESIAN_POINT('Ctrl Pts',(58.5429485109152,-5.66870453919802,
-176.613388490099));
#162875=CARTESIAN_POINT('Ctrl Pts',(58.5357937630411,-5.66609567921663,
-176.633580138909));
#162876=CARTESIAN_POINT('Ctrl Pts',(58.5287328734313,-5.66302333872094,
-176.65343800953));
#162877=CARTESIAN_POINT('Ctrl Pts',(58.5217765613204,-5.65948888494477,
-176.672930259477));
#162878=CARTESIAN_POINT('Ctrl Pts',(58.5172529280574,-5.65719045836277,
-176.685605911291));
#162879=CARTESIAN_POINT('Ctrl Pts',(58.5127742345477,-5.65469728174271,
-176.698124986584));
#162880=CARTESIAN_POINT('Ctrl Pts',(58.5083407613764,-5.65201071061408,
-176.710486547715));
#162881=CARTESIAN_POINT('Ctrl Pts',(58.5060990024534,-5.65065226215459,
-176.716737096415));
#162882=CARTESIAN_POINT('Ctrl Pts',(58.5038683421279,-5.64924411240428,
-176.72294866782));
#162883=CARTESIAN_POINT('Ctrl Pts',(58.5016483653956,-5.64778615672935,
-176.729122399553));
#162884=CARTESIAN_POINT('Ctrl Pts',(58.4898362654193,-5.64002863479541,
-176.761971724228));
#162885=CARTESIAN_POINT('Ctrl Pts',(58.4784451172372,-5.63090809605689,
-176.793399371308));
#162886=CARTESIAN_POINT('Ctrl Pts',(58.4674297681207,-5.62048392576165,
-176.823405937733));
#162887=CARTESIAN_POINT('Ctrl Pts',(58.4631068061411,-5.61639297127818,
-176.835181982634));
#162888=CARTESIAN_POINT('Ctrl Pts',(58.4588444780111,-5.61210324517753,
-176.846731684525));
#162889=CARTESIAN_POINT('Ctrl Pts',(58.454647608505,-5.60762712545288,-176.858035618715));
#162890=CARTESIAN_POINT('Ctrl Pts',(58.4481504254091,-5.60069763446731,
-176.875535264589));
#162891=CARTESIAN_POINT('Ctrl Pts',(58.4418083102892,-5.59331915800136,
-176.892450478896));
#162892=CARTESIAN_POINT('Ctrl Pts',(58.4356299325352,-5.58553811454111,
-176.908739450309));
#162893=CARTESIAN_POINT('Ctrl Pts',(58.4339980164171,-5.58348288083035,
-176.913041912226));
#162894=CARTESIAN_POINT('Ctrl Pts',(58.432377517179,-5.58139962042743,-176.917300718298));
#162895=CARTESIAN_POINT('Ctrl Pts',(58.4307664293617,-5.57928998993657,
-176.921515480085));
#162896=CARTESIAN_POINT('Ctrl Pts',(58.4297367314208,-5.57794165736942,
-176.924209269639));
#162897=CARTESIAN_POINT('Ctrl Pts',(58.428884895563,-5.57681225945347,-176.926433647857));
#162898=CARTESIAN_POINT('Ctrl Pts',(58.4278796327049,-5.57546258463045,
-176.929055357636));
#162899=CARTESIAN_POINT('Ctrl Pts',(58.4273120394084,-5.57470052883984,
-176.930535632058));
#162900=CARTESIAN_POINT('Ctrl Pts',(58.4266956310907,-5.57386775174087,
-176.932142116037));
#162901=CARTESIAN_POINT('Ctrl Pts',(58.4259718144521,-5.5728798358495,-176.934025799901));
#162902=CARTESIAN_POINT('Ctrl Pts',(58.4196479910485,-5.56424863659143,
-176.950483122753));
#162903=CARTESIAN_POINT('Ctrl Pts',(58.4134394553127,-5.55510712130321,
-176.9664084859));
#162904=CARTESIAN_POINT('Ctrl Pts',(58.4073502234499,-5.54547311803255,
-176.98176505197));
#162905=CARTESIAN_POINT('Ctrl Pts',(58.3979885804448,-5.53066170973654,
-177.005374382763));
#162906=CARTESIAN_POINT('Ctrl Pts',(58.3889117915324,-5.51466287933301,
-177.027596666233));
#162907=CARTESIAN_POINT('Ctrl Pts',(58.3801633276821,-5.49770409370011,
-177.048237284276));
#162908=CARTESIAN_POINT('Ctrl Pts',(58.372943899417,-5.48370932405424,-177.06527038447));
#162909=CARTESIAN_POINT('Ctrl Pts',(58.3659447782497,-5.46905542971186,
-177.081234299931));
#162910=CARTESIAN_POINT('Ctrl Pts',(58.3591786862378,-5.45387223042539,
-177.096045819018));
#162911=CARTESIAN_POINT('Ctrl Pts',(58.3557956402319,-5.44628063078215,
-177.103451578561));
#162912=CARTESIAN_POINT('Ctrl Pts',(58.3524730577879,-5.43855609988564,
-177.110568847175));
#162913=CARTESIAN_POINT('Ctrl Pts',(58.3492141964119,-5.43071541842866,
-177.117387967907));
#162914=CARTESIAN_POINT('Ctrl Pts',(58.3477437626597,-5.42717761754519,
-177.120464829463));
#162915=CARTESIAN_POINT('Ctrl Pts',(58.3464013095158,-5.42389707592293,
-177.123242460199));
#162916=CARTESIAN_POINT('Ctrl Pts',(58.3450298856348,-5.42049936370148,
-177.126050672046));
#162917=CARTESIAN_POINT('Ctrl Pts',(58.3437250496098,-5.41726662335737,
-177.128722534506));
#162918=CARTESIAN_POINT('Ctrl Pts',(58.342393972099,-5.41392771186506,-177.13142219143));
#162919=CARTESIAN_POINT('Ctrl Pts',(58.3409084629875,-5.41013924246599,
-177.134394284005));
#162920=CARTESIAN_POINT('Ctrl Pts',(58.3404950069453,-5.4090848123374,-177.13522149511));
#162921=CARTESIAN_POINT('Ctrl Pts',(58.3400696340722,-5.40799542616371,
-177.136069548477));
#162922=CARTESIAN_POINT('Ctrl Pts',(58.3396296994008,-5.40686335247274,
-177.136943044253));
#162923=CARTESIAN_POINT('Ctrl Pts',(58.3355952543372,-5.39648160852046,
-177.144953485235));
#162924=CARTESIAN_POINT('Ctrl Pts',(58.3316482276062,-5.38588752655005,
-177.152494532144));
#162925=CARTESIAN_POINT('Ctrl Pts',(58.3277942727314,-5.37511057187182,
-177.159541643791));
#162926=CARTESIAN_POINT('Ctrl Pts',(58.3203781128629,-5.35437249335602,
-177.173102390681));
#162927=CARTESIAN_POINT('Ctrl Pts',(58.3132716974141,-5.33285868715332,
-177.184860820779));
#162928=CARTESIAN_POINT('Ctrl Pts',(58.3065400889278,-5.31093152612779,
-177.194732398229));
#162929=CARTESIAN_POINT('Ctrl Pts',(58.3000030628719,-5.28963818691342,
-177.20431862998));
#162930=CARTESIAN_POINT('Ctrl Pts',(58.2938195924287,-5.26795588312359,
-177.212125463235));
#162931=CARTESIAN_POINT('Ctrl Pts',(58.2880381913187,-5.24620561892136,
-177.218121248799));
#162932=CARTESIAN_POINT('Ctrl Pts',(58.2824668436432,-5.22524559874663,
-177.223899191781));
#162933=CARTESIAN_POINT('Ctrl Pts',(58.2772689190291,-5.20422301863945,
-177.227995395089));
#162934=CARTESIAN_POINT('Ctrl Pts',(58.2724764146032,-5.18340504051878,
-177.230424191671));
#162935=CARTESIAN_POINT('Ctrl Pts',(58.2705944502693,-5.17523004706118,
-177.231377953658));
#162936=CARTESIAN_POINT('Ctrl Pts',(58.2687748732832,-5.16708633698723,
-177.232075061476));
#162937=CARTESIAN_POINT('Ctrl Pts',(58.267019098174,-5.15898893607643,-177.232518219478));
#162938=CARTESIAN_POINT('',(58.1115942404669,-6.2375212064409,-176.427328712824));
#162939=CARTESIAN_POINT('Origin',(58.6082745331205,-6.18000001999999,-176.427328712824));
#162940=CARTESIAN_POINT('Ctrl Pts',(57.9826110754301,-5.20432973493148,
-177.68524973918));
#162941=CARTESIAN_POINT('Ctrl Pts',(57.9864133803307,-5.23272890152749,
-177.684790303892));
#162942=CARTESIAN_POINT('Ctrl Pts',(57.9901585317883,-5.26087114190313,
-177.682937908873));
#162943=CARTESIAN_POINT('Ctrl Pts',(57.9938499513603,-5.28876235919758,
-177.679797008529));
#162944=CARTESIAN_POINT('Ctrl Pts',(57.9976152499095,-5.31721178304886,
-177.676593247137));
#162945=CARTESIAN_POINT('Ctrl Pts',(58.0013246616446,-5.34540021247657,
-177.672048874718));
#162946=CARTESIAN_POINT('Ctrl Pts',(58.0049820412409,-5.37334248086366,
-177.666219172833));
#162947=CARTESIAN_POINT('Ctrl Pts',(58.0071009194111,-5.38953064535426,
-177.662841774414));
#162948=CARTESIAN_POINT('Ctrl Pts',(58.0092023028964,-5.40563608053747,
-177.659031970271));
#162949=CARTESIAN_POINT('Ctrl Pts',(58.0112866328472,-5.42166024630227,
-177.654792733909));
#162950=CARTESIAN_POINT('Ctrl Pts',(58.0127082279006,-5.43258935797033,
-177.651901407879));
#162951=CARTESIAN_POINT('Ctrl Pts',(58.0141227858999,-5.44348757569641,
-177.648808284626));
#162952=CARTESIAN_POINT('Ctrl Pts',(58.0155294925108,-5.45434822190824,
-177.645514358109));
#162953=CARTESIAN_POINT('Ctrl Pts',(58.0189462259726,-5.48072752022124,
-177.637513777986));
#162954=CARTESIAN_POINT('Ctrl Pts',(58.0223147701654,-5.50687103546922,
-177.628330087141));
#162955=CARTESIAN_POINT('Ctrl Pts',(58.0256102732283,-5.5325791664003,-177.618027059099));
#162956=CARTESIAN_POINT('Ctrl Pts',(58.0292381208969,-5.56087990867951,
-177.606684992183));
#162957=CARTESIAN_POINT('Ctrl Pts',(58.0327774052014,-5.58865274716744,
-177.593984257917));
#162958=CARTESIAN_POINT('Ctrl Pts',(58.0361953413919,-5.61562914495522,
-177.580061370296));
#162959=CARTESIAN_POINT('Ctrl Pts',(58.0369297082257,-5.62142520746961,
-177.57706994321));
#162960=CARTESIAN_POINT('Ctrl Pts',(58.0376584880585,-5.62718459988006,
-177.57402226185));
#162961=CARTESIAN_POINT('Ctrl Pts',(58.0383813818279,-5.63290483163267,
-177.570919942798));
#162962=CARTESIAN_POINT('Ctrl Pts',(58.0384493306635,-5.63344250826458,
-177.570628338448));
#162963=CARTESIAN_POINT('Ctrl Pts',(58.0385172322329,-5.63397987194777,
-177.570336244847));
#162964=CARTESIAN_POINT('Ctrl Pts',(58.0385850863885,-5.63451692127423,
-177.570043663697));
#162965=CARTESIAN_POINT('Ctrl Pts',(58.0490694432024,-5.71749808456103,
-177.524836039378));
#162966=CARTESIAN_POINT('Ctrl Pts',(58.058560690856,-5.79407235500778,-177.467381876558));
#162967=CARTESIAN_POINT('Ctrl Pts',(58.0668921625494,-5.86215495272362,
-177.400951487669));
#162968=CARTESIAN_POINT('Ctrl Pts',(58.0716810779975,-5.90128871155427,
-177.362767415601));
#162969=CARTESIAN_POINT('Ctrl Pts',(58.076086829394,-5.93761722714732,-177.32161665146));
#162970=CARTESIAN_POINT('Ctrl Pts',(58.0800778613687,-5.97074680033053,
-177.278112939551));
#162971=CARTESIAN_POINT('Ctrl Pts',(58.0801358840197,-5.97122844660027,
-177.27748047138));
#162972=CARTESIAN_POINT('Ctrl Pts',(58.0801938210413,-5.97170942905892,
-177.276847523818));
#162973=CARTESIAN_POINT('Ctrl Pts',(58.0802516724784,-5.97218974777174,
-177.276214098177));
#162974=CARTESIAN_POINT('Ctrl Pts',(58.0863462475121,-6.02279071087329,
-177.209483515684));
#162975=CARTESIAN_POINT('Ctrl Pts',(58.091488245137,-6.06600199005368,-177.137485615194));
#162976=CARTESIAN_POINT('Ctrl Pts',(58.0957336562474,-6.10193041986059,
-177.061710183542));
#162977=CARTESIAN_POINT('Ctrl Pts',(58.0990967930802,-6.13039226312736,
-177.001682276096));
#162978=CARTESIAN_POINT('Ctrl Pts',(58.1018971540569,-6.15428295037301,
-176.939282520674));
#162979=CARTESIAN_POINT('Ctrl Pts',(58.1041602520257,-6.17363798086329,
-176.875236987128));
#162980=CARTESIAN_POINT('Ctrl Pts',(58.1041777800786,-6.17378788864584,
-176.874740944307));
#162981=CARTESIAN_POINT('Ctrl Pts',(58.1041952749008,-6.17393751574848,
-176.874244853752));
#162982=CARTESIAN_POINT('Ctrl Pts',(58.104212736516,-6.17408686234949,-176.873748715522));
#162983=CARTESIAN_POINT('Ctrl Pts',(58.1067717090136,-6.19597337403404,
-176.801040431038));
#162984=CARTESIAN_POINT('Ctrl Pts',(58.1086155525892,-6.21181886439977,
-176.72738700765));
#162985=CARTESIAN_POINT('Ctrl Pts',(58.1098212142836,-6.22220604020925,
-176.652935850911));
#162986=CARTESIAN_POINT('Ctrl Pts',(58.1110268759779,-6.23259321601873,
-176.578484694172));
#162987=CARTESIAN_POINT('Ctrl Pts',(58.1115942404669,-6.23752120644093,
-176.50323543809));
#162988=CARTESIAN_POINT('Ctrl Pts',(58.1115942404669,-6.2375212064409,-176.427328712824));
#162989=CARTESIAN_POINT('Ctrl Pts',(58.2670190981741,-5.15898893607704,
-177.232518219478));
#162990=CARTESIAN_POINT('Ctrl Pts',(57.9819403936438,-5.19932045653815,
-177.367360689003));
#162991=CARTESIAN_POINT('Ctrl Pts',(57.9826110754301,-5.20432973493151,
-177.68524973918));
#162992=CARTESIAN_POINT('Ctrl Pts',(58.2478951756903,-4.99233199195458,
-177.233703806904));
#162993=CARTESIAN_POINT('Ctrl Pts',(57.9597329881765,-5.03356356782781,
-177.367569378206));
#162994=CARTESIAN_POINT('Ctrl Pts',(57.9604889110946,-5.0391007365056,-177.687922734557));
#162995=CARTESIAN_POINT('Ctrl Pts',(58.2281612527228,-4.82572915883349,
-177.234977247299));
#162996=CARTESIAN_POINT('Ctrl Pts',(57.936860143276,-4.86824210971035,-177.367787815378));
#162997=CARTESIAN_POINT('Ctrl Pts',(57.9376611104107,-4.87397087657654,
-177.690692163097));
#162998=CARTESIAN_POINT('Ctrl Pts',(58.207817372083,-4.65917712520044,-177.236349008084));
#162999=CARTESIAN_POINT('Ctrl Pts',(57.9133432880526,-4.70343927025946,
-177.368016692624));
#163000=CARTESIAN_POINT('Ctrl Pts',(57.9141277227909,-4.70894021166782,
-177.693561815623));
#163001=CARTESIAN_POINT('',(57.914127722791,-4.70894021166827,-177.693561815623));
#163002=CARTESIAN_POINT('Origin',(1.08576145822724,-12.9503575433999,-185.613344152246));
#163003=CARTESIAN_POINT('Origin',(58.4091202674301,-4.63835423039998,-177.693561815623));
#163004=CARTESIAN_POINT('Ctrl Pts',(57.7719896917998,-3.76686746433079,
-176.487816214668));
#163005=CARTESIAN_POINT('Ctrl Pts',(57.8426304086464,-4.22014242411439,
-176.540115608276));
#163006=CARTESIAN_POINT('Ctrl Pts',(58.3023950569127,-4.18492067076111,
-176.54510707307));
#163007=CARTESIAN_POINT('Ctrl Pts',(57.7656488319951,-3.72809386701247,
-176.804681178765));
#163008=CARTESIAN_POINT('Ctrl Pts',(57.8281144931389,-4.12556715300443,
-176.735939864345));
#163009=CARTESIAN_POINT('Ctrl Pts',(58.2201998825318,-4.16532008285243,
-176.752600827192));
#163010=CARTESIAN_POINT('Ctrl Pts',(57.7783333144461,-3.80457033547739,
-177.140063733512));
#163011=CARTESIAN_POINT('Ctrl Pts',(57.8296205489137,-4.13610505104128,
-176.987574312776));
#163012=CARTESIAN_POINT('Ctrl Pts',(58.1755280883538,-4.20378312244756,
-176.943056377667));
#163013=CARTESIAN_POINT('Ctrl Pts',(57.8431686999111,-4.22319358998163,
-177.622644986573));
#163014=CARTESIAN_POINT('Ctrl Pts',(57.8659572284752,-4.38142129799194,
-177.327226280779));
#163015=CARTESIAN_POINT('Ctrl Pts',(58.1582320325074,-4.41455172597864,
-177.206615941663));
#163016=CARTESIAN_POINT('Ctrl Pts',(57.8918930477109,-4.54705885986191,
-177.742945331961));
#163017=CARTESIAN_POINT('Ctrl Pts',(57.8985608374326,-4.60362668953059,
-177.410684031821));
#163018=CARTESIAN_POINT('Ctrl Pts',(58.1843609366024,-4.57776276467961,
-177.265681912745));
#163019=CARTESIAN_POINT('Ctrl Pts',(57.9368177485324,-4.86994787109087,
-177.677206679151));
#163020=CARTESIAN_POINT('Ctrl Pts',(57.9271674646007,-4.80719227924389,
-177.349355107446));
#163021=CARTESIAN_POINT('Ctrl Pts',(58.228168972613,-4.74018086702697,-177.223609336047));
#163022=CARTESIAN_POINT('',(57.7706512256236,-3.75870764711888,-176.647241333324));
#163023=CARTESIAN_POINT('Ctrl Pts',(57.7706512256236,-3.75870764711887,
-176.647241333324));
#163024=CARTESIAN_POINT('Ctrl Pts',(57.7706512256236,-3.75870764711892,
-176.716132142105));
#163025=CARTESIAN_POINT('Ctrl Pts',(57.7714731229875,-3.76385932402702,
-176.783073604645));
#163026=CARTESIAN_POINT('Ctrl Pts',(57.7731127828381,-3.77416333624056,
-176.848065720941));
#163027=CARTESIAN_POINT('Ctrl Pts',(57.7739326127634,-3.77931534234734,
-176.880561779089));
#163028=CARTESIAN_POINT('Ctrl Pts',(57.7749567540909,-3.78575545282719,
-176.912570500677));
#163029=CARTESIAN_POINT('Ctrl Pts',(57.7761839145684,-3.79348387278035,
-176.944091885703));
#163030=CARTESIAN_POINT('Ctrl Pts',(57.777411075046,-3.80121229273351,-176.97561327073));
#163031=CARTESIAN_POINT('Ctrl Pts',(57.778746960844,-3.80963337741544,-177.004881728095));
#163032=CARTESIAN_POINT('Ctrl Pts',(57.7804726441157,-3.8205343470524,-177.037194031102));
#163033=CARTESIAN_POINT('Ctrl Pts',(57.7839240106591,-3.84233628632631,
-177.101818637114));
#163034=CARTESIAN_POINT('Ctrl Pts',(57.7881819478627,-3.86930866299404,
-177.16259800506));
#163035=CARTESIAN_POINT('Ctrl Pts',(57.7932247359729,-3.90145487248269,
-177.219532134939));
#163036=CARTESIAN_POINT('Ctrl Pts',(57.795746130028,-3.91752797722698,-177.247999199879));
#163037=CARTESIAN_POINT('Ctrl Pts',(57.7984636067391,-3.93489456053134,
-177.275504955302));
#163038=CARTESIAN_POINT('Ctrl Pts',(57.8013736694665,-3.95355516093848,
-177.302049401209));
#163039=CARTESIAN_POINT('Ctrl Pts',(57.8042837321939,-3.97221576134561,
-177.328593847115));
#163040=CARTESIAN_POINT('Ctrl Pts',(57.8072614019285,-3.99136347062015,
-177.353242005971));
#163041=CARTESIAN_POINT('Ctrl Pts',(57.8106775980806,-4.01341962890035,
-177.378798810378));
#163042=CARTESIAN_POINT('Ctrl Pts',(57.820877452893,-4.07927346227552,-177.455104643772));
#163043=CARTESIAN_POINT('Ctrl Pts',(57.8322332475662,-4.15330818745427,
-177.51785062654));
#163044=CARTESIAN_POINT('Ctrl Pts',(57.8448789412148,-4.23709451534444,
-177.567745265917));
#163045=CARTESIAN_POINT('Ctrl Pts',(57.8491747318432,-4.26555705224762,
-177.584694666258));
#163046=CARTESIAN_POINT('Ctrl Pts',(57.8536189541738,-4.29514496864859,
-177.600161038337));
#163047=CARTESIAN_POINT('Ctrl Pts',(57.8582154512499,-4.32592002579372,
-177.614172156613));
#163048=CARTESIAN_POINT('Ctrl Pts',(57.8763428437788,-4.44728887075097,
-177.669428373808));
#163049=CARTESIAN_POINT('Ctrl Pts',(57.8950217283446,-4.57495716519149,
-177.695891593478));
#163050=CARTESIAN_POINT('Ctrl Pts',(57.914127722791,-4.70894021166828,-177.693561815623));
#163051=CARTESIAN_POINT('',(58.2644174754116,-4.18000003136422,-176.647241333317));
#163052=CARTESIAN_POINT('Origin',(58.2644174754153,-3.68000001999999,-176.647241333324));
#163053=CARTESIAN_POINT('Ctrl Pts',(58.2078173718681,-4.65917712427737,
-177.236349008137));
#163054=CARTESIAN_POINT('Ctrl Pts',(58.1948301492149,-4.60331060815716,
-177.23952272256));
#163055=CARTESIAN_POINT('Ctrl Pts',(58.1843326939393,-4.54860640735877,
-177.231092666144));
#163056=CARTESIAN_POINT('Ctrl Pts',(58.1770121417029,-4.49749087444241,
-177.212340891078));
#163057=CARTESIAN_POINT('Ctrl Pts',(58.1744085339799,-4.47931126285495,
-177.205671685695));
#163058=CARTESIAN_POINT('Ctrl Pts',(58.1722067390647,-4.46158638555533,
-177.197697525224));
#163059=CARTESIAN_POINT('Ctrl Pts',(58.1704367005146,-4.44441968451078,
-177.188473620115));
#163060=CARTESIAN_POINT('Ctrl Pts',(58.1685748231361,-4.4263622855139,-177.178771130719));
#163061=CARTESIAN_POINT('Ctrl Pts',(58.1671922722601,-4.40892606256636,
-177.167682895421));
#163062=CARTESIAN_POINT('Ctrl Pts',(58.1663236940235,-4.39229679467997,
-177.155335364104));
#163063=CARTESIAN_POINT('Ctrl Pts',(58.1655193809276,-4.3768979078848,-177.143901412938));
#163064=CARTESIAN_POINT('Ctrl Pts',(58.1651557313076,-4.3621915965796,-177.131388762485));
#163065=CARTESIAN_POINT('Ctrl Pts',(58.1652462837178,-4.3483007781872,-177.117926071166));
#163066=CARTESIAN_POINT('Ctrl Pts',(58.1652984126327,-4.34030415736272,
-177.110175913132));
#163067=CARTESIAN_POINT('Ctrl Pts',(58.1655008078473,-4.33257711780437,
-177.102111193057));
#163068=CARTESIAN_POINT('Ctrl Pts',(58.1658539559977,-4.32513860657448,
-177.093759366692));
#163069=CARTESIAN_POINT('Ctrl Pts',(58.1661142565689,-4.31965578379691,
-177.08760335208));
#163070=CARTESIAN_POINT('Ctrl Pts',(58.1664559934947,-4.31433507611524,
-177.081298147169));
#163071=CARTESIAN_POINT('Ctrl Pts',(58.1668800604306,-4.30916742421314,
-177.074836159665));
#163072=CARTESIAN_POINT('Ctrl Pts',(58.16695135481,-4.3082986355757,-177.073749766575));
#163073=CARTESIAN_POINT('Ctrl Pts',(58.167025065974,-4.3074347774271,-177.072659864222));
#163074=CARTESIAN_POINT('Ctrl Pts',(58.1671011947531,-4.30657576506413,
-177.071566398619));
#163075=CARTESIAN_POINT('Ctrl Pts',(58.1673524923837,-4.30374020439798,
-177.067956918493));
#163076=CARTESIAN_POINT('Ctrl Pts',(58.1676478381592,-4.3007629757407,-177.06405441704));
#163077=CARTESIAN_POINT('Ctrl Pts',(58.1679620654409,-4.29793615717124,
-177.060231622647));
#163078=CARTESIAN_POINT('Ctrl Pts',(58.1682762927225,-4.29510933860178,
-177.056408828254));
#163079=CARTESIAN_POINT('Ctrl Pts',(58.1686091516182,-4.29243243934732,
-177.052666252106));
#163080=CARTESIAN_POINT('Ctrl Pts',(58.1689138852836,-4.29015774532314,
-177.049410570726));
#163081=CARTESIAN_POINT('Ctrl Pts',(58.1694279402103,-4.28632056616321,
-177.04391856494));
#163082=CARTESIAN_POINT('Ctrl Pts',(58.1700074737126,-4.28257531700519,
-177.038318568171));
#163083=CARTESIAN_POINT('Ctrl Pts',(58.1706463882517,-4.27892301202666,
-177.032614290244));
#163084=CARTESIAN_POINT('Ctrl Pts',(58.1727964644394,-4.26663226970529,
-177.013418245402));
#163085=CARTESIAN_POINT('Ctrl Pts',(58.175618532156,-4.25539973890795,-176.993043260651));
#163086=CARTESIAN_POINT('Ctrl Pts',(58.1791407681495,-4.24530419939267,
-176.971613968747));
#163087=CARTESIAN_POINT('Ctrl Pts',(58.1827233690694,-4.2350356400965,-176.949817416491));
#163088=CARTESIAN_POINT('Ctrl Pts',(58.1870304587187,-4.22594345645078,
-176.92693044205));
#163089=CARTESIAN_POINT('Ctrl Pts',(58.1920726605442,-4.21807418246598,
-176.903119223703));
#163090=CARTESIAN_POINT('Ctrl Pts',(58.1972784148855,-4.20994965500221,
-176.878535647406));
#163091=CARTESIAN_POINT('Ctrl Pts',(58.2032679068386,-4.20312878672857,
-176.852967296043));
#163092=CARTESIAN_POINT('Ctrl Pts',(58.2100304868865,-4.19762260354405,
-176.826628541868));
#163093=CARTESIAN_POINT('Ctrl Pts',(58.2169370087538,-4.19199922100361,
-176.79972916613));
#163094=CARTESIAN_POINT('Ctrl Pts',(58.2246499872768,-4.18774708342058,
-176.772026842204));
#163095=CARTESIAN_POINT('Ctrl Pts',(58.2331330995294,-4.18483579450576,
-176.743774442892));
#163096=CARTESIAN_POINT('Ctrl Pts',(58.241867148002,-4.18183838768823,-176.714686318427));
#163097=CARTESIAN_POINT('Ctrl Pts',(58.2514176874185,-4.18026231439924,
-176.685015815368));
#163098=CARTESIAN_POINT('Ctrl Pts',(58.2617170359672,-4.18003022393884,
-176.655054447656));
#163099=CARTESIAN_POINT('Ctrl Pts',(58.2626115695454,-4.18001006609011,
-176.652452200598));
#163100=CARTESIAN_POINT('Ctrl Pts',(58.2635117341523,-4.18000001999999,
-176.649847764673));
#163101=CARTESIAN_POINT('Ctrl Pts',(58.2644174754153,-4.18000001999999,
-176.647241333323));
#163102=CARTESIAN_POINT('Origin',(0.,-12.9675000200281,-171.871644662643));
#163103=CARTESIAN_POINT('',(56.5940537057312,1.84341099694893,-171.871644662643));
#163104=CARTESIAN_POINT('',(57.7706512256236,-3.75870764711888,-171.871644662643));
#163105=CARTESIAN_POINT('Origin',(0.,-12.9675000200281,-171.871644662643));
#163106=CARTESIAN_POINT('Origin',(55.2297899960015,2.001980827273,-171.934292975586));
#163107=CARTESIAN_POINT('Origin',(56.3352965291918,-3.65078706877886,-171.961175715908));
#163108=CARTESIAN_POINT('Ctrl Pts',(56.5169491525423,2.13496529160038,-177.558207897086));
#163109=CARTESIAN_POINT('Ctrl Pts',(56.409292540301,2.53784145482491,-177.125154911669));
#163110=CARTESIAN_POINT('Ctrl Pts',(57.,2.61702308584989,-177.204078948543));
#163111=CARTESIAN_POINT('Ctrl Pts',(56.5659347005564,1.95164994081541,-177.37392715461));
#163112=CARTESIAN_POINT('Ctrl Pts',(56.4267635932219,2.4778594556634,-177.032282865396));
#163113=CARTESIAN_POINT('Ctrl Pts',(57.043897408659,2.52469464001198,-177.112050866152));
#163114=CARTESIAN_POINT('Ctrl Pts',(56.5940537017931,1.84341101199667,-177.116606872607));
#163115=CARTESIAN_POINT('Ctrl Pts',(56.4314543935154,2.46472012384626,-176.935564924353));
#163116=CARTESIAN_POINT('Ctrl Pts',(57.0736014896981,2.46999998000001,-176.982739539051));
#163117=CARTESIAN_POINT('Ctrl Pts',(56.5940537057312,1.84341099694892,-176.848740272858));
#163118=CARTESIAN_POINT('Ctrl Pts',(56.430072632376,2.46999998,-176.848740272858));
#163119=CARTESIAN_POINT('Ctrl Pts',(57.077763566464,2.46999998000001,-176.848740272858));
#163120=CARTESIAN_POINT('',(56.5169491525423,2.13496529160038,-177.558207897086));
#163121=CARTESIAN_POINT('Origin',(57.,2.26404619169977,-177.558207897086));
#163122=CARTESIAN_POINT('',(57.077763566464,2.46999998000001,-176.848740272858));
#163123=CARTESIAN_POINT('Ctrl Pts',(57.077763566464,2.46999998000001,-176.848740272858));
#163124=CARTESIAN_POINT('Ctrl Pts',(57.0760574119627,2.46999998000001,-176.903670626367));
#163125=CARTESIAN_POINT('Ctrl Pts',(57.069539132854,2.47909807637283,-176.964460625587));
#163126=CARTESIAN_POINT('Ctrl Pts',(57.0443985826942,2.52546697496909,-177.087725761396));
#163127=CARTESIAN_POINT('Ctrl Pts',(57.0257001863846,2.56296846543371,-177.150200178938));
#163128=CARTESIAN_POINT('Ctrl Pts',(57.,2.61702308584989,-177.204078948543));
#163129=CARTESIAN_POINT('',(56.5940537057312,1.84341099694892,-176.848740272858));
#163130=CARTESIAN_POINT('Origin',(57.077763566464,1.96999998000001,-176.848740272858));
#163131=CARTESIAN_POINT('Ctrl Pts',(56.5169491525423,2.13496529160038,-177.558207897086));
#163132=CARTESIAN_POINT('Ctrl Pts',(56.5229386918135,2.11255103806931,-177.535675603609));
#163133=CARTESIAN_POINT('Ctrl Pts',(56.528571815665,2.09142571598422,-177.512223964754));
#163134=CARTESIAN_POINT('Ctrl Pts',(56.5338654144839,2.07153817047639,-177.487923467016));
#163135=CARTESIAN_POINT('Ctrl Pts',(56.5392385869434,2.0513516743957,-177.463257682989));
#163136=CARTESIAN_POINT('Ctrl Pts',(56.5442620552539,2.03244001840271,-177.437717820727));
#163137=CARTESIAN_POINT('Ctrl Pts',(56.5489480395883,2.01476843117717,-177.41132463543));
#163138=CARTESIAN_POINT('Ctrl Pts',(56.5536246352264,1.99713225020854,-177.38498433072));
#163139=CARTESIAN_POINT('Ctrl Pts',(56.5579650856442,1.98073116282666,-177.357794129274));
#163140=CARTESIAN_POINT('Ctrl Pts',(56.561970784984,1.96557003493501,-177.329742709106));
#163141=CARTESIAN_POINT('Ctrl Pts',(56.565631524691,1.95171454100795,-177.304106998851));
#163142=CARTESIAN_POINT('Ctrl Pts',(56.5690127023447,1.93889452819214,-177.277750345696));
#163143=CARTESIAN_POINT('Ctrl Pts',(56.5721056483258,1.92715023624348,-177.250654113369));
#163144=CARTESIAN_POINT('Ctrl Pts',(56.572670163045,1.92500670521764,-177.245708594735));
#163145=CARTESIAN_POINT('Ctrl Pts',(56.5732250495913,1.92289910945411,-177.240738434495));
#163146=CARTESIAN_POINT('Ctrl Pts',(56.5737702212793,1.9208278227753,-177.235743502986));
#163147=CARTESIAN_POINT('Ctrl Pts',(56.5742136264815,1.91914318047097,-177.231680968807));
#163148=CARTESIAN_POINT('Ctrl Pts',(56.5746500692504,1.91748459286997,-177.227606869171));
#163149=CARTESIAN_POINT('Ctrl Pts',(56.5750788200599,1.91585486103934,-177.223528406682));
#163150=CARTESIAN_POINT('Ctrl Pts',(56.5782241786983,1.90389898602246,-177.193608399685));
#163151=CARTESIAN_POINT('Ctrl Pts',(56.5809693098902,1.89344399206872,-177.163338973001));
#163152=CARTESIAN_POINT('Ctrl Pts',(56.5833278536963,1.88444881109869,-177.132732821239));
#163153=CARTESIAN_POINT('Ctrl Pts',(56.5857124029625,1.87535444866779,-177.101789204022));
#163154=CARTESIAN_POINT('Ctrl Pts',(56.5877019367001,1.86775166258739,-177.070499522563));
#163155=CARTESIAN_POINT('Ctrl Pts',(56.5892981114555,1.86164434117929,-177.038856203194));
#163156=CARTESIAN_POINT('Ctrl Pts',(56.5899925100869,1.85898741679645,-177.025090118004));
#163157=CARTESIAN_POINT('Ctrl Pts',(56.5906123032695,1.85661411889969,-177.011256862245));
#163158=CARTESIAN_POINT('Ctrl Pts',(56.5911568728243,1.85452762189294,-176.997354903683));
#163159=CARTESIAN_POINT('Ctrl Pts',(56.592110679146,1.85087315017689,-176.97300580843));
#163160=CARTESIAN_POINT('Ctrl Pts',(56.5928339105565,1.84809776611721,-176.948446283833));
#163161=CARTESIAN_POINT('Ctrl Pts',(56.593315736919,1.8462472490988,-176.923675152294));
#163162=CARTESIAN_POINT('Ctrl Pts',(56.5935566501002,1.8453219905896,-176.911289586525));
#163163=CARTESIAN_POINT('Ctrl Pts',(56.5937366253393,1.84463019464051,-176.898851402341));
#163164=CARTESIAN_POINT('Ctrl Pts',(56.5938590328877,1.84415954091471,-176.886362089455));
#163165=CARTESIAN_POINT('Ctrl Pts',(56.5939814404361,1.84368888718891,-176.87387277657));
#163166=CARTESIAN_POINT('Ctrl Pts',(56.5940462830325,1.84343935986365,-176.861332171026));
#163167=CARTESIAN_POINT('Ctrl Pts',(56.5940537057312,1.84341099694892,-176.848740272859));
#163168=CARTESIAN_POINT('Ctrl Pts',(56.3252430313217,2.83493642067777,-177.84995));
#163169=CARTESIAN_POINT('Ctrl Pts',(56.3252430313216,2.83493642067775,-177.34995));
#163170=CARTESIAN_POINT('Ctrl Pts',(56.8066553649227,2.96999998000003,-177.34995));
#163171=CARTESIAN_POINT('Ctrl Pts',(56.3976379760506,2.57689628418379,-177.849949962148));
#163172=CARTESIAN_POINT('Ctrl Pts',(56.3657038976309,2.69072016585579,-177.313059794074));
#163173=CARTESIAN_POINT('Ctrl Pts',(56.8796685247676,2.83987814625872,-177.34995));
#163174=CARTESIAN_POINT('Ctrl Pts',(56.4669147992933,2.32220551629932,-177.746434148089));
#163175=CARTESIAN_POINT('Ctrl Pts',(56.393446522619,2.59195606221812,-177.219869815671));
#163176=CARTESIAN_POINT('Ctrl Pts',(56.9495585329053,2.71140496526165,-177.298153784266));
#163177=CARTESIAN_POINT('Ctrl Pts',(56.5169491525424,2.13496529160036,-177.558207897086));
#163178=CARTESIAN_POINT('Ctrl Pts',(56.409292540301,2.5378414548249,-177.125154911669));
#163179=CARTESIAN_POINT('Ctrl Pts',(57.,2.61702308584988,-177.204078948543));
#163180=CARTESIAN_POINT('',(56.3252430313217,2.83493642067774,-177.84995));
#163181=CARTESIAN_POINT('Origin',(56.8066553649227,2.96999998000001,-177.84995));
#163182=CARTESIAN_POINT('Ctrl Pts',(56.3252430313217,2.83493642067774,-177.84995));
#163183=CARTESIAN_POINT('Ctrl Pts',(56.3337905757477,2.80447007335715,-177.849949995531));
#163184=CARTESIAN_POINT('Ctrl Pts',(56.3422168470079,2.77432812514565,-177.848511343748));
#163185=CARTESIAN_POINT('Ctrl Pts',(56.3505347180946,2.74447917084385,-177.845717295416));
#163186=CARTESIAN_POINT('Ctrl Pts',(56.3586925281077,2.71520460097504,-177.84297701305));
#163187=CARTESIAN_POINT('Ctrl Pts',(56.3667461939752,2.68621137428779,-177.838933157927));
#163188=CARTESIAN_POINT('Ctrl Pts',(56.3747119330389,2.65745132354449,-177.833612584578));
#163189=CARTESIAN_POINT('Ctrl Pts',(56.3826465426729,2.62880366462976,-177.828312803577));
#163190=CARTESIAN_POINT('Ctrl Pts',(56.3904942639185,2.60038604323579,-177.821746106604));
#163191=CARTESIAN_POINT('Ctrl Pts',(56.3982693165815,2.5721540750335,-177.813887718037));
#163192=CARTESIAN_POINT('Ctrl Pts',(56.4059472278018,2.54427483680477,-177.806127512112));
#163193=CARTESIAN_POINT('Ctrl Pts',(56.4135548018023,2.51657466550273,-177.797106929139));
#163194=CARTESIAN_POINT('Ctrl Pts',(56.4210985479533,2.48903439318015,-177.786757501498));
#163195=CARTESIAN_POINT('Ctrl Pts',(56.4239423298017,2.47865247881527,-177.782856055998));
#163196=CARTESIAN_POINT('Ctrl Pts',(56.426776958486,2.4682935670556,-177.778765345278));
#163197=CARTESIAN_POINT('Ctrl Pts',(56.4296024917091,2.45795762024076,-177.774480127077));
#163198=CARTESIAN_POINT('Ctrl Pts',(56.4379967235467,2.42725108558959,-177.761749391951));
#163199=CARTESIAN_POINT('Ctrl Pts',(56.4461165623565,2.39745763002353,-177.747600314328));
#163200=CARTESIAN_POINT('Ctrl Pts',(56.4539709812586,2.36855912289836,-177.73209578844));
#163201=CARTESIAN_POINT('Ctrl Pts',(56.4618532758604,2.33955805362101,-177.716536236265));
#163202=CARTESIAN_POINT('Ctrl Pts',(56.4694684313471,2.31145762034201,-177.699611308859));
#163203=CARTESIAN_POINT('Ctrl Pts',(56.4768213142896,2.28425147073979,-177.681333396443));
#163204=CARTESIAN_POINT('Ctrl Pts',(56.4840747389559,2.25741332328893,-177.663302718978));
#163205=CARTESIAN_POINT('Ctrl Pts',(56.4910730820105,2.23144484455675,-177.643955073003));
#163206=CARTESIAN_POINT('Ctrl Pts',(56.4978146447403,2.20636084783545,-177.623257500239));
#163207=CARTESIAN_POINT('Ctrl Pts',(56.5044442829978,2.18169329952633,-177.602903551794));
#163208=CARTESIAN_POINT('Ctrl Pts',(56.5108257274528,2.15788057710433,-177.581243854425));
#163209=CARTESIAN_POINT('Ctrl Pts',(56.5169491525424,2.13496529160041,-177.558207897086));
#163210=CARTESIAN_POINT('Origin',(0.,-12.9675000200281,-177.84995));
#163211=CARTESIAN_POINT('',(56.1837939657261,3.33069913254215,-177.84995));
#163212=CARTESIAN_POINT('Origin',(56.6639973329545,3.46999998000001,-177.84995));
#163213=CARTESIAN_POINT('Origin',(0.,-12.9675000200281,-177.84995));
#163214=CARTESIAN_POINT('Ctrl Pts',(55.8907344288187,4.30901060783351,-176.690850240902));
#163215=CARTESIAN_POINT('Ctrl Pts',(55.9989092657488,3.95901908419397,-176.752404542197));
#163216=CARTESIAN_POINT('Ctrl Pts',(56.3697825056489,3.96335046636153,-176.770466133952));
#163217=CARTESIAN_POINT('Ctrl Pts',(55.8810800353191,4.34006612171963,-176.874277739409));
#163218=CARTESIAN_POINT('Ctrl Pts',(55.9918208819094,3.98257552011186,-176.864245565378));
#163219=CARTESIAN_POINT('Ctrl Pts',(56.360041241732,3.97898206969736,-176.862106001368));
#163220=CARTESIAN_POINT('Ctrl Pts',(55.8887283478319,4.31560402300748,-177.06862236504));
#163221=CARTESIAN_POINT('Ctrl Pts',(55.9976409365186,3.96330447540303,-176.985952090623));
#163222=CARTESIAN_POINT('Ctrl Pts',(56.3677577343663,3.96667187476728,-176.959188328205));
#163223=CARTESIAN_POINT('Ctrl Pts',(55.9266115295683,4.19254080857125,-177.361891255001));
#163224=CARTESIAN_POINT('Ctrl Pts',(56.0241238299815,3.87468354526111,-177.158432257995));
#163225=CARTESIAN_POINT('Ctrl Pts',(56.4059865293426,3.90470993307104,-177.105730604552));
#163226=CARTESIAN_POINT('Ctrl Pts',(55.9498205047936,4.11690393979646,-177.473010794577));
#163227=CARTESIAN_POINT('Ctrl Pts',(56.0403831092186,3.82012609038464,-177.220853928335));
#163228=CARTESIAN_POINT('Ctrl Pts',(56.4294064346049,3.866625884224,-177.161267442876));
#163229=CARTESIAN_POINT('Ctrl Pts',(56.0057627129126,3.93261288273155,-177.655191732052));
#163230=CARTESIAN_POINT('Ctrl Pts',(56.0777953809631,3.69371421455791,-177.313208384807));
#163231=CARTESIAN_POINT('Ctrl Pts',(56.4858608229818,3.7738058294262,-177.252357953738));
#163232=CARTESIAN_POINT('Ctrl Pts',(56.0389442880078,3.82243329271981,-177.727752411286));
#163233=CARTESIAN_POINT('Ctrl Pts',(56.0994690237907,3.6200556053818,-177.343574237135));
#163234=CARTESIAN_POINT('Ctrl Pts',(56.51934628745,3.71830354331151,-177.288661380879));
#163235=CARTESIAN_POINT('Ctrl Pts',(56.1230975683705,3.53939517412226,-177.843941866969));
#163236=CARTESIAN_POINT('Ctrl Pts',(56.1514384840657,3.44234559640889,-177.375806045407));
#163237=CARTESIAN_POINT('Ctrl Pts',(56.6042740428564,3.57567859252058,-177.346848135714));
#163238=CARTESIAN_POINT('Ctrl Pts',(56.1775019211747,3.35356550968309,-177.866562127611));
#163239=CARTESIAN_POINT('Ctrl Pts',(56.1824782924758,3.33526976742397,-177.359497704487));
#163240=CARTESIAN_POINT('Ctrl Pts',(56.6591858730236,3.48199543258953,-177.358249465165));
#163241=CARTESIAN_POINT('Ctrl Pts',(56.2275049818161,3.17916207692579,-177.837621610915));
#163242=CARTESIAN_POINT('Ctrl Pts',(56.2060958053042,3.25377207835719,-177.320175302413));
#163243=CARTESIAN_POINT('Ctrl Pts',(56.7096544558747,3.39403127791385,-177.343857300475));
#163244=CARTESIAN_POINT('',(55.8866301012659,4.32222455627096,-176.84995));
#163245=CARTESIAN_POINT('',(56.3642936064049,3.96999998000001,-176.84995));
#163246=CARTESIAN_POINT('Origin',(56.3642936064049,4.46999998000001,-176.84995));
#163247=CARTESIAN_POINT('Ctrl Pts',(56.6639973329545,3.46999998000001,-177.34995));
#163248=CARTESIAN_POINT('Ctrl Pts',(56.6132926555039,3.55739556046625,-177.34995));
#163249=CARTESIAN_POINT('Ctrl Pts',(56.5711004619007,3.63103186791303,-177.32741150463));
#163250=CARTESIAN_POINT('Ctrl Pts',(56.5205808972673,3.71540754291555,-177.2866997194));
#163251=CARTESIAN_POINT('Ctrl Pts',(56.5058691633514,3.73942485859416,-177.271891810804));
#163252=CARTESIAN_POINT('Ctrl Pts',(56.4869937439203,3.76997568356519,-177.250163369964));
#163253=CARTESIAN_POINT('Ctrl Pts',(56.4812339676837,3.77925206162339,-177.242992983045));
#163254=CARTESIAN_POINT('Ctrl Pts',(56.4733923486896,3.79192114453357,-177.232568181681));
#163255=CARTESIAN_POINT('Ctrl Pts',(56.4696710505327,3.79794447782133,-177.227437770765));
#163256=CARTESIAN_POINT('Ctrl Pts',(56.4656786808617,3.80445324466831,-177.221637219552));
#163257=CARTESIAN_POINT('Ctrl Pts',(56.4640424820409,3.80713442288003,-177.21919490467));
#163258=CARTESIAN_POINT('Ctrl Pts',(56.4629683087721,3.80889811921587,-177.217576826329));
#163259=CARTESIAN_POINT('Ctrl Pts',(56.4629360063793,3.80894940169979,-177.217534734494));
#163260=CARTESIAN_POINT('Ctrl Pts',(56.3968354290769,3.91795014829009,-177.116097367134));
#163261=CARTESIAN_POINT('Ctrl Pts',(56.3642936064049,3.96999998000001,-176.977117050922));
#163262=CARTESIAN_POINT('Ctrl Pts',(56.3642936064049,3.96999998000001,-176.84995));
#163263=CARTESIAN_POINT('Ctrl Pts',(55.8866301012659,4.32222455627096,-176.84995));
#163264=CARTESIAN_POINT('Ctrl Pts',(55.8866301033422,4.3222245495596,-176.887711783017));
#163265=CARTESIAN_POINT('Ctrl Pts',(55.8873019941254,4.32005750494367,-176.925285001291));
#163266=CARTESIAN_POINT('Ctrl Pts',(55.8886053322676,4.31584578460431,-176.962497615251));
#163267=CARTESIAN_POINT('Ctrl Pts',(55.8899346297675,4.31155017693619,-177.000451414885));
#163268=CARTESIAN_POINT('Ctrl Pts',(55.8919208352951,4.30512748218138,-177.038031169975));
#163269=CARTESIAN_POINT('Ctrl Pts',(55.8945372498695,4.2966554166734,-177.075061157623));
#163270=CARTESIAN_POINT('Ctrl Pts',(55.8971529093906,4.28818579606139,-177.112080459038));
#163271=CARTESIAN_POINT('Ctrl Pts',(55.9003985106906,4.27766770883152,-177.148551411106));
#163272=CARTESIAN_POINT('Ctrl Pts',(55.9042621819464,4.26513074059417,-177.184288779349));
#163273=CARTESIAN_POINT('Ctrl Pts',(55.9062291959159,4.25874810862931,-177.202482848646));
#163274=CARTESIAN_POINT('Ctrl Pts',(55.9083566338582,4.25184146461301,-177.22048652526));
#163275=CARTESIAN_POINT('Ctrl Pts',(55.9106442880651,4.24441025685161,-177.238272995257));
#163276=CARTESIAN_POINT('Ctrl Pts',(55.9107052688196,4.24421216718633,-177.238747119518));
#163277=CARTESIAN_POINT('Ctrl Pts',(55.9107663607186,4.2440137135512,-177.239221068301));
#163278=CARTESIAN_POINT('Ctrl Pts',(55.9108275637053,4.24381489610749,-177.239694840879));
#163279=CARTESIAN_POINT('Ctrl Pts',(55.9214558682229,4.20928892853583,-177.321968590921));
#163280=CARTESIAN_POINT('Ctrl Pts',(55.9354579988728,4.16369334127204,-177.399293819936));
#163281=CARTESIAN_POINT('Ctrl Pts',(55.9520401750176,4.10936168614259,-177.468909678493));
#163282=CARTESIAN_POINT('Ctrl Pts',(55.9599200188449,4.08354330419055,-177.501991108129));
#163283=CARTESIAN_POINT('Ctrl Pts',(55.9683824151874,4.05575233687934,-177.533330971157));
#163284=CARTESIAN_POINT('Ctrl Pts',(55.977341715845,4.02624042822255,-177.562628970791));
#163285=CARTESIAN_POINT('Ctrl Pts',(55.9774917411594,4.02574624530113,-177.563119571762));
#163286=CARTESIAN_POINT('Ctrl Pts',(55.9776419059241,4.025251579432,-177.563609601226));
#163287=CARTESIAN_POINT('Ctrl Pts',(55.9777922097306,4.02475643181778,-177.564099057738));
#163288=CARTESIAN_POINT('Ctrl Pts',(55.9952457911942,3.96725889118211,-177.620935736125));
#163289=CARTESIAN_POINT('Ctrl Pts',(56.01475026219,3.90266672703547,-177.67062951941));
#163290=CARTESIAN_POINT('Ctrl Pts',(56.0354959803716,3.83347839359387,-177.711737746814));
#163291=CARTESIAN_POINT('Ctrl Pts',(56.0478214929256,3.79237199925456,-177.736161098587));
#163292=CARTESIAN_POINT('Ctrl Pts',(56.0605847921289,3.74964437877247,-177.757554032042));
#163293=CARTESIAN_POINT('Ctrl Pts',(56.0736137591996,3.70582717944107,-177.775616713982));
#163294=CARTESIAN_POINT('Ctrl Pts',(56.0737452759341,3.7053848807584,-177.775799041938));
#163295=CARTESIAN_POINT('Ctrl Pts',(56.0738768160358,3.70494248350759,-177.775981025699));
#163296=CARTESIAN_POINT('Ctrl Pts',(56.0740083793673,3.7044999881052,-177.776162665075));
#163297=CARTESIAN_POINT('Ctrl Pts',(56.0854652800848,3.66596625811822,-177.791980326975));
#163298=CARTESIAN_POINT('Ctrl Pts',(56.0971863579253,3.62638912180278,-177.805308764985));
#163299=CARTESIAN_POINT('Ctrl Pts',(56.1090759206044,3.58608423515434,-177.816113161796));
#163300=CARTESIAN_POINT('Ctrl Pts',(56.1213067753347,3.54462238943049,-177.827227700776));
#163301=CARTESIAN_POINT('Ctrl Pts',(56.1337163559748,3.502389009303,-177.835671763787));
#163302=CARTESIAN_POINT('Ctrl Pts',(56.1462034955942,3.45971409454014,-177.841352247251));
#163303=CARTESIAN_POINT('Ctrl Pts',(56.1579134207248,3.41969531745755,-177.846679170638));
#163304=CARTESIAN_POINT('Ctrl Pts',(56.1696918925472,3.37928709608564,-177.849575574952));
#163305=CARTESIAN_POINT('Ctrl Pts',(56.1814524996762,3.33876843673258,-177.849916077404));
#163306=CARTESIAN_POINT('Ctrl Pts',(56.182233078045,3.33607912072376,-177.84993867733));
#163307=CARTESIAN_POINT('Ctrl Pts',(56.1830135754985,3.33338932446759,-177.849949999684));
#163308=CARTESIAN_POINT('Ctrl Pts',(56.1837939657261,3.33069913254215,-177.84995));
#163309=CARTESIAN_POINT('Origin',(0.,-12.9675000200281,-171.871644662643));
#163310=CARTESIAN_POINT('',(53.8350584096845,9.92434320033876,-171.871644662643));
#163311=CARTESIAN_POINT('',(55.8866301012659,4.32222455627096,-171.871644662643));
#163312=CARTESIAN_POINT('Origin',(0.,-12.9675000200281,-171.871644662643));
#163313=CARTESIAN_POINT('Origin',(52.5977860076314,10.1271303560196,-171.886170842901));
#163314=CARTESIAN_POINT('Origin',(54.5615907362999,4.49781486075725,-171.920628921479));
#163315=CARTESIAN_POINT('Ctrl Pts',(53.4025720561297,10.9158686240697,-177.84995));
#163316=CARTESIAN_POINT('Ctrl Pts',(53.4025720561301,10.9158686240688,-177.34995));
#163317=CARTESIAN_POINT('Ctrl Pts',(53.8590042959257,11.1199999800011,-177.34995));
#163318=CARTESIAN_POINT('Ctrl Pts',(53.4583000366404,10.7912623535259,-177.849949984912));
#163319=CARTESIAN_POINT('Ctrl Pts',(53.4357429270681,10.8416994438452,-177.323612898224));
#163320=CARTESIAN_POINT('Ctrl Pts',(53.9152095126149,11.0571633006792,-177.34995));
#163321=CARTESIAN_POINT('Ctrl Pts',(53.5126282698489,10.6685980808388,-177.826730821509));
#163322=CARTESIAN_POINT('Ctrl Pts',(53.4634087021834,10.7796461652398,-177.282275394088));
#163323=CARTESIAN_POINT('Ctrl Pts',(53.9700011606116,10.9953079956486,-177.338340413074));
#163324=CARTESIAN_POINT('Ctrl Pts',(53.6159658107279,10.4332420187126,-177.732767091856));
#163325=CARTESIAN_POINT('Ctrl Pts',(53.5073796187504,10.6816635307577,-177.18321412648));
#163326=CARTESIAN_POINT('Ctrl Pts',(54.0742219292009,10.8766241714759,-177.291358543608));
#163327=CARTESIAN_POINT('Ctrl Pts',(53.6629085389549,10.3252623899094,-177.663867719202));
#163328=CARTESIAN_POINT('Ctrl Pts',(53.5219518286219,10.649686808137,-177.127170956772));
#163329=CARTESIAN_POINT('Ctrl Pts',(54.1215658763003,10.8221729031368,-177.256908861057));
#163330=CARTESIAN_POINT('Ctrl Pts',(53.7443081182388,10.1368259480206,-177.482357798918));
#163331=CARTESIAN_POINT('Ctrl Pts',(53.5394251697822,10.6131024574854,-177.020421798311));
#163332=CARTESIAN_POINT('Ctrl Pts',(54.2036611796727,10.7271494012897,-177.166153898004));
#163333=CARTESIAN_POINT('Ctrl Pts',(53.7772720937282,10.0598397490546,-177.372348961349));
#163334=CARTESIAN_POINT('Ctrl Pts',(53.5413185515592,10.6107526879388,-176.973405437982));
#163335=CARTESIAN_POINT('Ctrl Pts',(54.2369068974943,10.6883272976786,-177.111149481396));
#163336=CARTESIAN_POINT('Ctrl Pts',(53.8228725022638,9.95305333910152,-177.124428650036));
#163337=CARTESIAN_POINT('Ctrl Pts',(53.5410688387025,10.6146700040362,-176.899444869037));
#163338=CARTESIAN_POINT('Ctrl Pts',(54.282897054019,10.6344777440414,-176.987189324297));
#163339=CARTESIAN_POINT('Ctrl Pts',(53.8350584050868,9.92434321115133,-176.989642564215));
#163340=CARTESIAN_POINT('Ctrl Pts',(53.5392499462662,10.6199999783344,-176.8744703999));
#163341=CARTESIAN_POINT('Ctrl Pts',(54.2951871094022,10.61999998,-176.919796282647));
#163342=CARTESIAN_POINT('Ctrl Pts',(53.8350584096845,9.92434320033874,-176.84995));
#163343=CARTESIAN_POINT('Ctrl Pts',(53.5392499457278,10.61999998,-176.84995));
#163344=CARTESIAN_POINT('Ctrl Pts',(54.2951871140408,10.61999998,-176.84995));
#163345=CARTESIAN_POINT('',(54.2951871140408,10.61999998,-176.84995));
#163346=CARTESIAN_POINT('',(53.8350584096845,9.92434320033876,-176.84995));
#163347=CARTESIAN_POINT('Origin',(54.2951871140408,10.11999998,-176.84995));
#163348=CARTESIAN_POINT('',(53.4025720561307,10.9158686240676,-177.84995));
#163349=CARTESIAN_POINT('Ctrl Pts',(53.4025720561307,10.9158686240675,-177.84995));
#163350=CARTESIAN_POINT('Ctrl Pts',(53.4256992941538,10.8641567398107,-177.849949993739));
#163351=CARTESIAN_POINT('Ctrl Pts',(53.4485179803107,10.8129304526924,-177.845955353724));
#163352=CARTESIAN_POINT('Ctrl Pts',(53.4709798749291,10.7623159210356,-177.837971298851));
#163353=CARTESIAN_POINT('Ctrl Pts',(53.4932283385006,10.7121823244322,-177.8300631078));
#163354=CARTESIAN_POINT('Ctrl Pts',(53.5151269426183,10.6626484619091,-177.818240932981));
#163355=CARTESIAN_POINT('Ctrl Pts',(53.5366259143439,10.613840772558,-177.80245915115));
#163356=CARTESIAN_POINT('Ctrl Pts',(53.5459258227761,10.5927278073638,-177.795632353674));
#163357=CARTESIAN_POINT('Ctrl Pts',(53.5551508985508,10.5717508130024,-177.788063986787));
#163358=CARTESIAN_POINT('Ctrl Pts',(53.5642968110718,10.5509205718341,-177.77974738364));
#163359=CARTESIAN_POINT('Ctrl Pts',(53.5644850520156,10.5504918443291,-177.779576211522));
#163360=CARTESIAN_POINT('Ctrl Pts',(53.5646732319863,10.5500632415521,-177.779404746864));
#163361=CARTESIAN_POINT('Ctrl Pts',(53.5648613509312,10.5496347636521,-177.779232989633));
#163362=CARTESIAN_POINT('Ctrl Pts',(53.5997722939237,10.4701182239948,-177.747358438588));
#163363=CARTESIAN_POINT('Ctrl Pts',(53.6324973478409,10.3950941639631,-177.705483670659));
#163364=CARTESIAN_POINT('Ctrl Pts',(53.662565751538,10.3258245179345,-177.653697116807));
#163365=CARTESIAN_POINT('Ctrl Pts',(53.6768635990437,10.292886060487,-177.629072056652));
#163366=CARTESIAN_POINT('Ctrl Pts',(53.6905609342839,10.2612483121622,-177.602206386713));
#163367=CARTESIAN_POINT('Ctrl Pts',(53.7036082895117,10.2310442594454,-177.573112646646));
#163368=CARTESIAN_POINT('Ctrl Pts',(53.7038266840866,10.2305386856232,-177.572625657913));
#163369=CARTESIAN_POINT('Ctrl Pts',(53.7040448535835,10.2300336133805,-177.572138119876));
#163370=CARTESIAN_POINT('Ctrl Pts',(53.7042627976345,10.2295290436849,-177.571650033405));
#163371=CARTESIAN_POINT('Ctrl Pts',(53.7326736221979,10.1637541760665,-177.508023891492));
#163372=CARTESIAN_POINT('Ctrl Pts',(53.7572655280445,10.1064913273751,-177.435049789256));
#163373=CARTESIAN_POINT('Ctrl Pts',(53.7772301637647,10.0598657379883,-177.354607724291));
#163374=CARTESIAN_POINT('Ctrl Pts',(53.7856960958606,10.0400943242139,-177.320496555463));
#163375=CARTESIAN_POINT('Ctrl Pts',(53.7933301997489,10.0222350963587,-177.28504246553));
#163376=CARTESIAN_POINT('Ctrl Pts',(53.8000719149495,10.0064474410942,-177.248388344963));
#163377=CARTESIAN_POINT('Ctrl Pts',(53.8001626051628,10.0062350640088,-177.247895270142));
#163378=CARTESIAN_POINT('Ctrl Pts',(53.8002531267728,10.006023079014,-177.247402027608));
#163379=CARTESIAN_POINT('Ctrl Pts',(53.800343479687,10.005811486348,-177.246908617746));
#163380=CARTESIAN_POINT('Ctrl Pts',(53.8073717082883,9.98935245300704,-177.208528037134));
#163381=CARTESIAN_POINT('Ctrl Pts',(53.8133972227366,9.97522506645289,-177.169027476767));
#163382=CARTESIAN_POINT('Ctrl Pts',(53.8183528652338,9.96359686430571,-177.128668162154));
#163383=CARTESIAN_POINT('Ctrl Pts',(53.8232487909443,9.95210878503228,-177.088795187826));
#163384=CARTESIAN_POINT('Ctrl Pts',(53.8271003741327,9.94306028562344,-177.048084581928));
#163385=CARTESIAN_POINT('Ctrl Pts',(53.829861825915,9.93656859429008,-177.006803377711));
#163386=CARTESIAN_POINT('Ctrl Pts',(53.8325710248907,9.93019974018788,-176.966303305646));
#163387=CARTESIAN_POINT('Ctrl Pts',(53.8342309082794,9.92629199069111,-176.925254528035));
#163388=CARTESIAN_POINT('Ctrl Pts',(53.8348176649726,9.92491022336675,-176.883916088102));
#163389=CARTESIAN_POINT('Ctrl Pts',(53.8349780875801,9.92453244034421,-176.872613924192));
#163390=CARTESIAN_POINT('Ctrl Pts',(53.8350584093113,9.92434320121651,-176.861290124361));
#163391=CARTESIAN_POINT('Ctrl Pts',(53.8350584096845,9.92434320033876,-176.84995));
#163392=CARTESIAN_POINT('Origin',(53.8590042959267,11.11999998,-177.84995));
#163393=CARTESIAN_POINT('Ctrl Pts',(54.2951871140408,10.61999998,-176.84995));
#163394=CARTESIAN_POINT('Ctrl Pts',(54.295187112658,10.61999998,-176.870771477027));
#163395=CARTESIAN_POINT('Ctrl Pts',(54.2940343032734,10.6212900755915,-176.891794363281));
#163396=CARTESIAN_POINT('Ctrl Pts',(54.2916911849701,10.6239505106872,-176.912836670541));
#163397=CARTESIAN_POINT('Ctrl Pts',(54.2893026016019,10.6266625679541,-176.934287275524));
#163398=CARTESIAN_POINT('Ctrl Pts',(54.2856770724215,10.630798428608,-176.955757775013));
#163399=CARTESIAN_POINT('Ctrl Pts',(54.280809897557,10.6364012547725,-176.977053069232));
#163400=CARTESIAN_POINT('Ctrl Pts',(54.2757855218655,10.6421850419525,-176.999036162422));
#163401=CARTESIAN_POINT('Ctrl Pts',(54.2694380093634,10.649531872693,-177.020832355256));
#163402=CARTESIAN_POINT('Ctrl Pts',(54.2617991887197,10.6584484085697,-177.042228441581));
#163403=CARTESIAN_POINT('Ctrl Pts',(54.2609825719224,10.6594016176199,-177.044515758473));
#163404=CARTESIAN_POINT('Ctrl Pts',(54.260151231088,10.660372730439,-177.046798505411));
#163405=CARTESIAN_POINT('Ctrl Pts',(54.2593052287969,10.6613617303426,-177.049076423852));
#163406=CARTESIAN_POINT('Ctrl Pts',(54.2589052193173,10.6618293524056,-177.050153476455));
#163407=CARTESIAN_POINT('Ctrl Pts',(54.2585020693351,10.66230080757,-177.051228977642));
#163408=CARTESIAN_POINT('Ctrl Pts',(54.2580957907476,10.6627760870642,-177.052302900297));
#163409=CARTESIAN_POINT('Ctrl Pts',(54.2504067447387,10.67177101323,-177.072627477953));
#163410=CARTESIAN_POINT('Ctrl Pts',(54.2415263947062,10.6822029113807,-177.092532024772));
#163411=CARTESIAN_POINT('Ctrl Pts',(54.2314451843677,10.6940494493327,-177.111801613672));
#163412=CARTESIAN_POINT('Ctrl Pts',(54.2253160858662,10.7012518184505,-177.123516993521));
#163413=CARTESIAN_POINT('Ctrl Pts',(54.2187437276912,10.7089763005547,-177.134997409078));
#163414=CARTESIAN_POINT('Ctrl Pts',(54.2117316348916,10.7172105764342,-177.146192801267));
#163415=CARTESIAN_POINT('Ctrl Pts',(54.2024588038328,10.7280996292896,-177.160997651028));
#163416=CARTESIAN_POINT('Ctrl Pts',(54.192413237421,10.7398811588086,-177.175304855698));
#163417=CARTESIAN_POINT('Ctrl Pts',(54.1815949348861,10.752515497233,-177.188999491326));
#163418=CARTESIAN_POINT('Ctrl Pts',(54.1761857836187,10.7588326664453,-177.19584680914));
#163419=CARTESIAN_POINT('Ctrl Pts',(54.1705834483029,10.765362824047,-177.202540970492));
#163420=CARTESIAN_POINT('Ctrl Pts',(54.1647879289713,10.7720997079721,-177.209067514237));
#163421=CARTESIAN_POINT('Ctrl Pts',(54.1640579820703,10.7729482199452,-177.209889533819));
#163422=CARTESIAN_POINT('Ctrl Pts',(54.1633248766812,10.7738001056606,-177.210708987479));
#163423=CARTESIAN_POINT('Ctrl Pts',(54.1625884803548,10.7746554933064,-177.211525975779));
#163424=CARTESIAN_POINT('Ctrl Pts',(54.1604015139413,10.7771958428235,-177.213952286052));
#163425=CARTESIAN_POINT('Ctrl Pts',(54.158189835222,10.779762066631,-177.216353164041));
#163426=CARTESIAN_POINT('Ctrl Pts',(54.1559497621978,10.7823577707401,-177.218731355435));
#163427=CARTESIAN_POINT('Ctrl Pts',(54.1544525864815,10.7840926361293,-177.220320843977));
#163428=CARTESIAN_POINT('Ctrl Pts',(54.1529433368185,10.7858400389663,-177.221899598547));
#163429=CARTESIAN_POINT('Ctrl Pts',(54.1514220132121,10.7875999079006,-177.223467359814));
#163430=CARTESIAN_POINT('Ctrl Pts',(54.1502918620496,10.7889072680923,-177.22463200829));
#163431=CARTESIAN_POINT('Ctrl Pts',(54.1487914911753,10.7906414389948,-177.226158503531));
#163432=CARTESIAN_POINT('Ctrl Pts',(54.1477305915031,10.7918671107764,-177.22722583738));
#163433=CARTESIAN_POINT('Ctrl Pts',(54.147363388662,10.7922913451995,-177.227595267244));
#163434=CARTESIAN_POINT('Ctrl Pts',(54.147049085478,10.7926543863909,-177.227910135178));
#163435=CARTESIAN_POINT('Ctrl Pts',(54.146821820558,10.7929168335172,-177.228137406876));
#163436=CARTESIAN_POINT('Ctrl Pts',(54.1342953618731,10.8073824760096,-177.240664239137));
#163437=CARTESIAN_POINT('Ctrl Pts',(54.1198488297753,10.8238052428689,-177.25344441977));
#163438=CARTESIAN_POINT('Ctrl Pts',(54.1034633204787,10.842370556489,-177.265842564197));
#163439=CARTESIAN_POINT('Ctrl Pts',(54.088970645158,10.8587912278061,-177.276808490156));
#163440=CARTESIAN_POINT('Ctrl Pts',(54.0729605932981,10.8768889662157,-177.287474913187));
#163441=CARTESIAN_POINT('Ctrl Pts',(54.0554395607018,10.8967687287218,-177.297375727477));
#163442=CARTESIAN_POINT('Ctrl Pts',(54.0480420828295,10.905162075543,-177.301555906597));
#163443=CARTESIAN_POINT('Ctrl Pts',(54.0403755551798,10.913872699112,-177.305599307741));
#163444=CARTESIAN_POINT('Ctrl Pts',(54.0324419334657,10.9229063569136,-177.309469503735));
#163445=CARTESIAN_POINT('Ctrl Pts',(54.0287742229151,10.9270826137637,-177.311258693993));
#163446=CARTESIAN_POINT('Ctrl Pts',(54.0250526063655,10.9313257163362,-177.313010020251));
#163447=CARTESIAN_POINT('Ctrl Pts',(54.0212673431407,10.9356453298748,-177.314723399853));
#163448=CARTESIAN_POINT('Ctrl Pts',(54.0188642208532,10.938387691225,-177.315811160589));
#163449=CARTESIAN_POINT('Ctrl Pts',(54.0164398861093,10.9411558257346,-177.316881633396));
#163450=CARTESIAN_POINT('Ctrl Pts',(54.0139919510376,10.9439520922684,-177.317934517196));
#163451=CARTESIAN_POINT('Ctrl Pts',(53.9984512906739,10.9617041270301,-177.324618726156));
#163452=CARTESIAN_POINT('Ctrl Pts',(53.9819783775985,10.9805730655438,-177.330584054845));
#163453=CARTESIAN_POINT('Ctrl Pts',(53.9645670843843,11.0004694748766,-177.33549234988));
#163454=CARTESIAN_POINT('Ctrl Pts',(53.9572593724224,11.0088202175061,-177.337552415488));
#163455=CARTESIAN_POINT('Ctrl Pts',(53.9497866998397,11.01735154001,-177.339426565227));
#163456=CARTESIAN_POINT('Ctrl Pts',(53.9421501581125,11.0260550554856,-177.341091294699));
#163457=CARTESIAN_POINT('Ctrl Pts',(53.9232699100964,11.0475732422071,-177.345207098219));
#163458=CARTESIAN_POINT('Ctrl Pts',(53.903385736146,11.0701430681308,-177.348040800477));
#163459=CARTESIAN_POINT('Ctrl Pts',(53.8824911975385,11.0936551403296,-177.349265802689));
#163460=CARTESIAN_POINT('Ctrl Pts',(53.8747985514822,11.102311471674,-177.349716806112));
#163461=CARTESIAN_POINT('Ctrl Pts',(53.8669692913113,11.1110952218607,-177.34995));
#163462=CARTESIAN_POINT('Ctrl Pts',(53.8590042959267,11.11999998,-177.34995));
#163463=CARTESIAN_POINT('Origin',(0.,-12.9675000200281,-177.84995));
#163464=CARTESIAN_POINT('',(53.1780777607544,11.411631335932,-177.84995));
#163465=CARTESIAN_POINT('Origin',(0.,-12.9675000200281,-177.84995));
#163466=CARTESIAN_POINT('Origin',(53.6325912458891,11.61999998,-177.84995));
#163467=CARTESIAN_POINT('Ctrl Pts',(52.9099958749003,11.9881018181948,-177.663675223808));
#163468=CARTESIAN_POINT('Ctrl Pts',(52.9997517486903,11.797676512519,-177.337555142414));
#163469=CARTESIAN_POINT('Ctrl Pts',(53.3622278820666,11.9106883715865,-177.256778275814));
#163470=CARTESIAN_POINT('Ctrl Pts',(52.9976548387626,11.8022980130591,-177.797387815582));
#163471=CARTESIAN_POINT('Ctrl Pts',(53.0664188011436,11.6545589022485,-177.39893190434));
#163472=CARTESIAN_POINT('Ctrl Pts',(53.4506644997516,11.8169620310944,-177.323650098968));
#163473=CARTESIAN_POINT('Ctrl Pts',(53.1011582398324,11.5800093343372,-177.861139569353));
#163474=CARTESIAN_POINT('Ctrl Pts',(53.1375549029137,11.499963173746,-177.390455278679));
#163475=CARTESIAN_POINT('Ctrl Pts',(53.5550086872502,11.7049144813144,-177.355501814437));
#163476=CARTESIAN_POINT('Ctrl Pts',(53.2037302934161,11.3555915204785,-177.848448015576));
#163477=CARTESIAN_POINT('Ctrl Pts',(53.1927421255947,11.3794221790895,-177.337053842004));
#163478=CARTESIAN_POINT('Ctrl Pts',(53.6584638339975,11.5917397245118,-177.349157933747));
#163479=CARTESIAN_POINT('',(52.9322463618642,11.9408779899289,-177.695579616717));
#163480=CARTESIAN_POINT('Ctrl Pts',(52.9322463618642,11.940877989929,-177.695579616717));
#163481=CARTESIAN_POINT('Ctrl Pts',(52.9695658609497,11.861571143096,-177.746066773083));
#163482=CARTESIAN_POINT('Ctrl Pts',(53.009594439893,11.7760355127808,-177.784659368904));
#163483=CARTESIAN_POINT('Ctrl Pts',(53.0510018552188,11.6869357301078,-177.810630175633));
#163484=CARTESIAN_POINT('Ctrl Pts',(53.0924092705445,11.5978359474347,-177.836600982362));
#163485=CARTESIAN_POINT('Ctrl Pts',(53.1351948005685,11.5051717233266,-177.84995));
#163486=CARTESIAN_POINT('Ctrl Pts',(53.1780777607544,11.411631335932,-177.84995));
#163487=CARTESIAN_POINT('',(53.3846587239314,11.8868850448361,-177.272764808359));
#163488=CARTESIAN_POINT('Origin',(53.3846587239314,12.1537701096722,-177.695579616717));
#163489=CARTESIAN_POINT('Ctrl Pts',(53.6325912458891,11.61999998,-177.34995));
#163490=CARTESIAN_POINT('Ctrl Pts',(53.6193902496202,11.6343976136465,-177.34995));
#163491=CARTESIAN_POINT('Ctrl Pts',(53.6071216945481,11.647745990074,-177.349336222758));
#163492=CARTESIAN_POINT('Ctrl Pts',(53.5958029190205,11.6600403513377,-177.348353185436));
#163493=CARTESIAN_POINT('Ctrl Pts',(53.5831048880715,11.6738328485423,-177.347250359578));
#163494=CARTESIAN_POINT('Ctrl Pts',(53.5715986168778,11.6863027073468,-177.345682762576));
#163495=CARTESIAN_POINT('Ctrl Pts',(53.5613057001372,11.6974417930555,-177.343941078924));
#163496=CARTESIAN_POINT('Ctrl Pts',(53.5514335858369,11.7081254826343,-177.342270600037));
#163497=CARTESIAN_POINT('Ctrl Pts',(53.5426828084495,11.7175793620638,-177.34044118093));
#163498=CARTESIAN_POINT('Ctrl Pts',(53.535036882964,11.7258313494675,-177.338656510057));
#163499=CARTESIAN_POINT('Ctrl Pts',(53.5312693392627,11.7298975312822,-177.337777110235));
#163500=CARTESIAN_POINT('Ctrl Pts',(53.5277703317232,11.7336715434635,-177.33690786316));
#163501=CARTESIAN_POINT('Ctrl Pts',(53.5245383140635,11.7371559990051,-177.336068813023));
#163502=CARTESIAN_POINT('Ctrl Pts',(53.5207506930954,11.7412394534479,-177.335085525112));
#163503=CARTESIAN_POINT('Ctrl Pts',(53.5173269143261,11.7449241460667,-177.334144097169));
#163504=CARTESIAN_POINT('Ctrl Pts',(53.5142595429646,11.7482126391687,-177.333272132227));
#163505=CARTESIAN_POINT('Ctrl Pts',(53.5127258572839,11.7498568857197,-177.332836149756));
#163506=CARTESIAN_POINT('Ctrl Pts',(53.5112838669721,11.7514031852974,-177.332417154949));
#163507=CARTESIAN_POINT('Ctrl Pts',(53.5099335719791,11.752852238671,-177.332017926533));
#163508=CARTESIAN_POINT('Ctrl Pts',(53.5092584244826,11.7535767653578,-177.331818312325));
#163509=CARTESIAN_POINT('Ctrl Pts',(53.5086062008165,11.7542769791225,-177.331623634357));
#163510=CARTESIAN_POINT('Ctrl Pts',(53.507976900977,11.7549529596041,-177.331434207795));
#163511=CARTESIAN_POINT('Ctrl Pts',(53.5076622510572,11.7552909498449,-177.331339494514));
#163512=CARTESIAN_POINT('Ctrl Pts',(53.5075769762504,11.7553821019031,-177.331313791835));
#163513=CARTESIAN_POINT('Ctrl Pts',(53.507385610281,11.7555876789724,-177.331255890439));
#163514=CARTESIAN_POINT('Ctrl Pts',(53.5071942443116,11.7557932560417,-177.331197989043));
#163515=CARTESIAN_POINT('Ctrl Pts',(53.5068967871326,11.7561133566317,-177.331108233285));
#163516=CARTESIAN_POINT('Ctrl Pts',(53.5061577729354,11.7569082763594,-177.330881975835));
#163517=CARTESIAN_POINT('Ctrl Pts',(53.4886819350222,11.7757061402844,-177.325531552884));
#163518=CARTESIAN_POINT('Ctrl Pts',(53.4721182870987,11.7934851338263,-177.31927585382));
#163519=CARTESIAN_POINT('Ctrl Pts',(53.4564928503932,11.8102233474837,-177.312383460726));
#163520=CARTESIAN_POINT('Ctrl Pts',(53.4400282994755,11.8278604334882,-177.305120933657));
#163521=CARTESIAN_POINT('Ctrl Pts',(53.4246052146097,11.8443421754681,-177.297151753489));
#163522=CARTESIAN_POINT('Ctrl Pts',(53.4102166329,11.8596818104284,-177.28876587707));
#163523=CARTESIAN_POINT('Ctrl Pts',(53.4013036283722,11.8691839447327,-177.283571247327));
#163524=CARTESIAN_POINT('Ctrl Pts',(53.3927868566238,11.8782485868146,-177.278216229675));
#163525=CARTESIAN_POINT('Ctrl Pts',(53.3846587239315,11.8868850448361,-177.272764808359));
#163526=CARTESIAN_POINT('Ctrl Pts',(52.1126146143195,13.5388501432916,-171.391638125813));
#163527=CARTESIAN_POINT('Ctrl Pts',(52.4864722882118,13.5059760932666,-171.679515584751));
#163528=CARTESIAN_POINT('Ctrl Pts',(52.5050296388285,13.3739336825608,-172.133326251627));
#163529=CARTESIAN_POINT('Ctrl Pts',(52.2275734081837,13.1702746923549,-171.333188379966));
#163530=CARTESIAN_POINT('Ctrl Pts',(52.5259488232545,13.163017811976,-171.621133646225));
#163531=CARTESIAN_POINT('Ctrl Pts',(52.5511257748791,13.045942631788,-172.016544094259));
#163532=CARTESIAN_POINT('Ctrl Pts',(52.3625569744519,12.7995634785289,-171.277518845311));
#163533=CARTESIAN_POINT('Ctrl Pts',(52.6036316644729,12.8055197818762,-171.550813695775));
#163534=CARTESIAN_POINT('Ctrl Pts',(52.6287970696452,12.7242148673197,-171.90506362857));
#163535=CARTESIAN_POINT('Ctrl Pts',(52.521634376552,12.4186874453849,-171.247275980756));
#163536=CARTESIAN_POINT('Ctrl Pts',(52.7259743335333,12.4493753091149,-171.512222020089));
#163537=CARTESIAN_POINT('Ctrl Pts',(52.7423614633688,12.4030287528935,-171.844601961512));
#163538=CARTESIAN_POINT('',(52.7229719177955,12.458911061641,-171.855631342512));
#163539=CARTESIAN_POINT('Ctrl Pts',(52.5103993792154,12.4456688476555,-171.249463186897));
#163540=CARTESIAN_POINT('Ctrl Pts',(52.5297066417322,12.4444102902161,-171.271932598649));
#163541=CARTESIAN_POINT('Ctrl Pts',(52.5475880394989,12.4433468997068,-171.294915021113));
#163542=CARTESIAN_POINT('Ctrl Pts',(52.5640300074807,12.442495320782,-171.318251747026));
#163543=CARTESIAN_POINT('Ctrl Pts',(52.5803556661806,12.4416497658643,-171.341423390643));
#163544=CARTESIAN_POINT('Ctrl Pts',(52.5952623602387,12.441013117922,-171.364944185641));
#163545=CARTESIAN_POINT('Ctrl Pts',(52.6087807058339,12.4405907657944,-171.388635430273));
#163546=CARTESIAN_POINT('Ctrl Pts',(52.623312668846,12.4401367453337,-171.414103065219));
#163547=CARTESIAN_POINT('Ctrl Pts',(52.6362425608597,12.4399303027981,-171.439769352997));
#163548=CARTESIAN_POINT('Ctrl Pts',(52.647675798678,12.4399636610286,-171.465430214553));
#163549=CARTESIAN_POINT('Ctrl Pts',(52.6522530291883,12.4399770158029,-171.475703391785));
#163550=CARTESIAN_POINT('Ctrl Pts',(52.6565910749825,12.4400286515715,-171.485976052153));
#163551=CARTESIAN_POINT('Ctrl Pts',(52.6606989661368,12.4401175158482,-171.49623639269));
#163552=CARTESIAN_POINT('Ctrl Pts',(52.6630824957991,12.44016907774,-171.502189770006));
#163553=CARTESIAN_POINT('Ctrl Pts',(52.6652494160276,12.4402293235166,-171.507780348161));
#163554=CARTESIAN_POINT('Ctrl Pts',(52.6674149000463,12.4403025724068,-171.513538486835));
#163555=CARTESIAN_POINT('Ctrl Pts',(52.6695392899826,12.4403744312632,-171.519187354131));
#163556=CARTESIAN_POINT('Ctrl Pts',(52.6716624958677,12.4404587371184,-171.524997386882));
#163557=CARTESIAN_POINT('Ctrl Pts',(52.6739462816228,12.4405683544587,-171.531492117076));
#163558=CARTESIAN_POINT('Ctrl Pts',(52.6740124707888,12.4405715314118,-171.531680348732));
#163559=CARTESIAN_POINT('Ctrl Pts',(52.6740787844409,12.4405747302306,-171.53186913741));
#163560=CARTESIAN_POINT('Ctrl Pts',(52.6741452257962,12.4405779513586,-171.532058495837));
#163561=CARTESIAN_POINT('Ctrl Pts',(52.6846243513975,12.4410859874213,-171.561924092684));
#163562=CARTESIAN_POINT('Ctrl Pts',(52.6933788831336,12.4419134247877,-171.592007876766));
#163563=CARTESIAN_POINT('Ctrl Pts',(52.7004429961507,12.4430787347014,-171.622183769804));
#163564=CARTESIAN_POINT('Ctrl Pts',(52.7075705499667,12.4442545099334,-171.652630663993));
#163565=CARTESIAN_POINT('Ctrl Pts',(52.712977310938,12.4457744135457,-171.683171329686));
#163566=CARTESIAN_POINT('Ctrl Pts',(52.7167490255101,12.4476434139055,-171.713665889365));
#163567=CARTESIAN_POINT('Ctrl Pts',(52.7205968921899,12.4495501499725,-171.74477614383));
#163568=CARTESIAN_POINT('Ctrl Pts',(52.722743139262,12.4518203906959,-171.77583841498));
#163569=CARTESIAN_POINT('Ctrl Pts',(52.7233295870902,12.4544423301942,-171.806693370106));
#163570=CARTESIAN_POINT('Ctrl Pts',(52.7236409084908,12.4558342116845,-171.823073016147));
#163571=CARTESIAN_POINT('Ctrl Pts',(52.7235135000264,12.4573249035982,-171.839394056547));
#163572=CARTESIAN_POINT('Ctrl Pts',(52.7229739807576,12.4589105225087,-171.855631463706));
#163573=CARTESIAN_POINT('',(52.5050296388285,13.3739336825608,-172.133326251627));
#163574=CARTESIAN_POINT('Ctrl Pts',(52.5050296388285,13.3739336825608,-172.133326251627));
#163575=CARTESIAN_POINT('Ctrl Pts',(52.5113922936146,13.3286610413417,-172.117206797456));
#163576=CARTESIAN_POINT('Ctrl Pts',(52.5180677265498,13.2855571710499,-172.101923158766));
#163577=CARTESIAN_POINT('Ctrl Pts',(52.5249057325846,13.2445934907971,-172.087543541658));
#163578=CARTESIAN_POINT('Ctrl Pts',(52.5320889680496,13.2015616830932,-172.072437942883));
#163579=CARTESIAN_POINT('Ctrl Pts',(52.5394513985051,13.1608916606645,-172.058329381205));
#163580=CARTESIAN_POINT('Ctrl Pts',(52.5468293681514,13.1225611963807,-172.045238297065));
#163581=CARTESIAN_POINT('Ctrl Pts',(52.5548629048856,13.0808248911878,-172.030984008911));
#163582=CARTESIAN_POINT('Ctrl Pts',(52.5629143627139,13.0418628361347,-172.017935616994));
#163583=CARTESIAN_POINT('Ctrl Pts',(52.570789876164,13.0056574082241,-172.006060015165));
#163584=CARTESIAN_POINT('Ctrl Pts',(52.5742287729683,12.9898480605375,-172.000874452415));
#163585=CARTESIAN_POINT('Ctrl Pts',(52.5776343821988,12.9745644067251,-171.995911826329));
#163586=CARTESIAN_POINT('Ctrl Pts',(52.5809918470595,12.9598053140195,-171.991166699342));
#163587=CARTESIAN_POINT('Ctrl Pts',(52.5827654361525,12.9520087868984,-171.988660074309));
#163588=CARTESIAN_POINT('Ctrl Pts',(52.5845256033797,12.9443586463142,-171.986214119865));
#163589=CARTESIAN_POINT('Ctrl Pts',(52.5862702312371,12.9368548371707,-171.983827461247));
#163590=CARTESIAN_POINT('Ctrl Pts',(52.5871425451659,12.9331029325989,-171.982634131938));
#163591=CARTESIAN_POINT('Ctrl Pts',(52.588010880141,12.9293880210105,-171.981453986818));
#163592=CARTESIAN_POINT('Ctrl Pts',(52.5888751232003,12.9257094662639,-171.980289358009));
#163593=CARTESIAN_POINT('Ctrl Pts',(52.5896959593966,12.9222156680164,-171.979183223026));
#163594=CARTESIAN_POINT('Ctrl Pts',(52.5901687724434,12.9202071686556,-171.978548012444));
#163595=CARTESIAN_POINT('Ctrl Pts',(52.5912744272476,12.9155453298856,-171.977081560367));
#163596=CARTESIAN_POINT('Ctrl Pts',(52.5913328956812,12.9152988059168,-171.977004012514));
#163597=CARTESIAN_POINT('Ctrl Pts',(52.5913931436171,12.9150448631177,-171.976924147958));
#163598=CARTESIAN_POINT('Ctrl Pts',(52.5914553200437,12.9147828898895,-171.976841777287));
#163599=CARTESIAN_POINT('Ctrl Pts',(52.6038700340288,12.8624749192527,-171.960394895763));
#163600=CARTESIAN_POINT('Ctrl Pts',(52.6168327657393,12.8116557021248,-171.945092080409));
#163601=CARTESIAN_POINT('Ctrl Pts',(52.6302178818164,12.7623034905211,-171.9309914502));
#163602=CARTESIAN_POINT('Ctrl Pts',(52.6439822275001,12.7115530228484,-171.916491318305));
#163603=CARTESIAN_POINT('Ctrl Pts',(52.6581931596669,12.6623538907316,-171.903262171156));
#163604=CARTESIAN_POINT('Ctrl Pts',(52.6727149251186,12.6146907174398,-171.891312060373));
#163605=CARTESIAN_POINT('Ctrl Pts',(52.6878982669679,12.5648561256253,-171.878817531538));
#163606=CARTESIAN_POINT('Ctrl Pts',(52.7034213118224,12.5167006425706,-171.867720993698));
#163607=CARTESIAN_POINT('Ctrl Pts',(52.7191311438969,12.4702153439479,-171.857976087372));
#163608=CARTESIAN_POINT('Ctrl Pts',(52.7204083062534,12.4664362282162,-171.857183855637));
#163609=CARTESIAN_POINT('Ctrl Pts',(52.7216867047946,12.4626681555264,-171.856400529307));
#163610=CARTESIAN_POINT('Ctrl Pts',(52.7229662582911,12.4589111234036,-171.855626069084));
#163611=CARTESIAN_POINT('Origin',(51.5147615700869,13.2347605816008,-172.133326251627));
#163612=CARTESIAN_POINT('Ctrl Pts',(52.7228616924159,12.4592197450689,-176.820632909447));
#163613=CARTESIAN_POINT('Ctrl Pts',(52.8378230805615,12.1196543833272,-176.831752638987));
#163614=CARTESIAN_POINT('Ctrl Pts',(53.1964757989599,12.1197761140302,-176.835304824703));
#163615=CARTESIAN_POINT('Ctrl Pts',(52.7208610202525,12.4653983050582,-177.002115882214));
#163616=CARTESIAN_POINT('Ctrl Pts',(52.8359625560594,12.1237916221297,-176.944353244896));
#163617=CARTESIAN_POINT('Ctrl Pts',(53.1946754990687,12.1225542377913,-176.925963491801));
#163618=CARTESIAN_POINT('Ctrl Pts',(52.7374134643798,12.4138498331152,-177.18556360953));
#163619=CARTESIAN_POINT('Ctrl Pts',(52.8514409345781,12.0892511690341,-177.059386795892));
#163620=CARTESIAN_POINT('Ctrl Pts',(53.2095700879098,12.099376493835,-177.017605185139));
#163621=CARTESIAN_POINT('Ctrl Pts',(52.8100292410526,12.2198706620515,-177.495904173093));
#163622=CARTESIAN_POINT('Ctrl Pts',(52.9147988673353,11.9568596714106,-177.246828041132));
#163623=CARTESIAN_POINT('Ctrl Pts',(53.2749021302737,12.0121566707775,-177.172631305935));
#163624=CARTESIAN_POINT('Ctrl Pts',(52.867357957607,12.0764932764824,-177.624786878572));
#163625=CARTESIAN_POINT('Ctrl Pts',(52.9645940841351,11.8559530379094,-177.320932244844));
#163626=CARTESIAN_POINT('Ctrl Pts',(53.3264267869461,11.9477421916568,-177.236975784533));
#163627=CARTESIAN_POINT('Ctrl Pts',(52.9443095206334,11.9154395316641,-177.710596296728));
#163628=CARTESIAN_POINT('Ctrl Pts',(53.0251950686999,11.7443762835566,-177.357540682165));
#163629=CARTESIAN_POINT('Ctrl Pts',(53.3957081880351,11.8752586579091,-177.279873126825));
#163630=CARTESIAN_POINT('',(52.7229737572976,12.4589111791821,-176.84995));
#163631=CARTESIAN_POINT('',(53.1963133798215,12.11999998,-176.84995));
#163632=CARTESIAN_POINT('Origin',(53.1963133798215,12.61999998,-176.84995));
#163633=CARTESIAN_POINT('Ctrl Pts',(53.3846587239314,11.8868850448361,-177.272764808359));
#163634=CARTESIAN_POINT('Ctrl Pts',(53.3218769425614,11.9535931363301,-177.230657973471));
#163635=CARTESIAN_POINT('Ctrl Pts',(53.2747906065339,12.0124550402845,-177.170935103968));
#163636=CARTESIAN_POINT('Ctrl Pts',(53.2120088251639,12.0957858369083,-177.025107728));
#163637=CARTESIAN_POINT('Ctrl Pts',(53.1963133798215,12.11999998,-176.939021563529));
#163638=CARTESIAN_POINT('Ctrl Pts',(53.1963133798215,12.11999998,-176.84995));
#163639=CARTESIAN_POINT('Ctrl Pts',(52.7229737572976,12.4589111791821,-176.84995));
#163640=CARTESIAN_POINT('Ctrl Pts',(52.7230767593181,12.458608520417,-176.940255331482));
#163641=CARTESIAN_POINT('Ctrl Pts',(52.7273331507401,12.4459433761744,-177.027109684591));
#163642=CARTESIAN_POINT('Ctrl Pts',(52.7403923566312,12.4085558894172,-177.152214746696));
#163643=CARTESIAN_POINT('Ctrl Pts',(52.7458669121792,12.3930315358947,-177.193053689472));
#163644=CARTESIAN_POINT('Ctrl Pts',(52.7558971321586,12.365201810831,-177.253017986745));
#163645=CARTESIAN_POINT('Ctrl Pts',(52.7595441580411,12.3551682611144,-177.272790399688));
#163646=CARTESIAN_POINT('Ctrl Pts',(52.7674747337066,12.3335983394208,-177.311903853277));
#163647=CARTESIAN_POINT('Ctrl Pts',(52.7720465255225,12.3212955152219,-177.332438473495));
#163648=CARTESIAN_POINT('Ctrl Pts',(52.8110199539533,12.2176628634023,-177.493824447827));
#163649=CARTESIAN_POINT('Ctrl Pts',(52.8604414114892,12.0934691109458,-177.608894237259));
#163650=CARTESIAN_POINT('Ctrl Pts',(52.9322463618642,11.9408779899289,-177.695579616717));
#163651=CARTESIAN_POINT('Ctrl Pts',(52.5050296388285,13.3739336825608,-172.133326251627));
#163652=CARTESIAN_POINT('Ctrl Pts',(52.4864722882118,13.5059760932665,-171.679515584751));
#163653=CARTESIAN_POINT('Ctrl Pts',(52.1126146143195,13.5388501432916,-171.391638125813));
#163654=CARTESIAN_POINT('Ctrl Pts',(52.4188787332531,13.9869292276479,-172.315208572937));
#163655=CARTESIAN_POINT('Ctrl Pts',(52.3988291636435,14.129589328176,-171.781794156641));
#163656=CARTESIAN_POINT('Ctrl Pts',(51.9336694513028,14.1125756396742,-171.482621144035));
#163657=CARTESIAN_POINT('Ctrl Pts',(52.3315472405275,14.6083250867988,-172.437881815118));
#163658=CARTESIAN_POINT('Ctrl Pts',(52.3125022740344,14.7438370647052,-171.821280489149));
#163659=CARTESIAN_POINT('Ctrl Pts',(51.7497860966453,14.6887611591208,-171.543915907757));
#163660=CARTESIAN_POINT('Ctrl Pts',(52.1554800333145,15.861108362107,-172.606056153125));
#163661=CARTESIAN_POINT('Ctrl Pts',(52.1416679592957,15.9593863754288,-171.81403941883));
#163662=CARTESIAN_POINT('Ctrl Pts',(51.3741578990745,15.8404043177988,-171.628003076365));
#163663=CARTESIAN_POINT('Ctrl Pts',(52.0666747393889,16.4929908616926,-172.649949997757));
#163664=CARTESIAN_POINT('Ctrl Pts',(52.0557320324868,16.5708522670934,-171.757498535929));
#163665=CARTESIAN_POINT('Ctrl Pts',(51.1823572933404,16.4160730441958,-171.64995));
#163666=CARTESIAN_POINT('Ctrl Pts',(51.9770573602378,17.1306516479033,-172.64995));
#163667=CARTESIAN_POINT('Ctrl Pts',(51.9770573602378,17.1306516479032,-171.64995));
#163668=CARTESIAN_POINT('Ctrl Pts',(50.9867892914963,16.9914785469432,-171.64995));
#163669=CARTESIAN_POINT('',(51.9770573602378,17.1306516479033,-172.64995));
#163670=CARTESIAN_POINT('Origin',(50.9867892914963,16.9914785469432,-172.64995));
#163671=CARTESIAN_POINT('Ctrl Pts',(51.9770573602378,17.1306516479033,-172.64995));
#163672=CARTESIAN_POINT('Ctrl Pts',(52.0505828082768,16.6074909011026,-172.64994999816));
#163673=CARTESIAN_POINT('Ctrl Pts',(52.1235483666999,16.0883139759218,-172.620408747532));
#163674=CARTESIAN_POINT('Ctrl Pts',(52.1959928599553,15.5728446220586,-172.563374785654));
#163675=CARTESIAN_POINT('Ctrl Pts',(52.2118579788213,15.4599584356373,-172.550884525264));
#163676=CARTESIAN_POINT('Ctrl Pts',(52.2276981039083,15.3472500891946,-172.537075526609));
#163677=CARTESIAN_POINT('Ctrl Pts',(52.2435136369168,15.2347167244825,-172.521968983896));
#163678=CARTESIAN_POINT('Ctrl Pts',(52.2955483171871,14.8644707359736,-172.472266952379));
#163679=CARTESIAN_POINT('Ctrl Pts',(52.3473277334916,14.4960410449573,-172.409096799907));
#163680=CARTESIAN_POINT('Ctrl Pts',(52.39877081545,14.1300044971647,-172.328180486669));
#163681=CARTESIAN_POINT('Ctrl Pts',(52.4343604559388,13.8767710467997,-172.272200510582));
#163682=CARTESIAN_POINT('Ctrl Pts',(52.4697891103105,13.6246830721786,-172.207726272012));
#163683=CARTESIAN_POINT('Ctrl Pts',(52.5050296388285,13.3739336825608,-172.133326251627));
#163684=CARTESIAN_POINT('Origin',(51.6222122422086,12.4702093225365,-172.64995));
#163685=CARTESIAN_POINT('',(51.8267121465167,18.20041342952,-172.64995));
#163686=CARTESIAN_POINT('',(52.3378926620474,14.5631750666398,-172.64995));
#163687=CARTESIAN_POINT('Ctrl Pts',(51.8267121465167,18.20041342952,-172.64995));
#163688=CARTESIAN_POINT('Ctrl Pts',(51.8267121465167,18.20041342952,-172.608983203783));
#163689=CARTESIAN_POINT('Ctrl Pts',(51.8241375648893,18.2006212880455,-172.567620053095));
#163690=CARTESIAN_POINT('Ctrl Pts',(51.8188632652687,18.2010194183273,-172.526187281556));
#163691=CARTESIAN_POINT('Ctrl Pts',(51.8136580036326,18.2014123372798,-172.48529684459));
#163692=CARTESIAN_POINT('Ctrl Pts',(51.8058228695452,18.2019905277624,-172.444338940117));
#163693=CARTESIAN_POINT('Ctrl Pts',(51.7952777630821,18.2027427324649,-172.403658149851));
#163694=CARTESIAN_POINT('Ctrl Pts',(51.7849287688052,18.2034809480711,-172.363733918918));
#163695=CARTESIAN_POINT('Ctrl Pts',(51.7719693966446,18.2043867283353,-172.324077002367));
#163696=CARTESIAN_POINT('Ctrl Pts',(51.7563674887103,18.2054555537608,-172.285037095287));
#163697=CARTESIAN_POINT('Ctrl Pts',(51.7409344370744,18.2065128115045,-172.246419709235));
#163698=CARTESIAN_POINT('Ctrl Pts',(51.7229154768771,18.2077295674027,-172.20840647472));
#163699=CARTESIAN_POINT('Ctrl Pts',(51.7023264860424,18.2091080529521,-172.171353408967));
#163700=CARTESIAN_POINT('Ctrl Pts',(51.68205385491,18.2104653574111,-172.134869681311));
#163701=CARTESIAN_POINT('Ctrl Pts',(51.6592894086755,18.2119794375068,-172.099317308706));
#163702=CARTESIAN_POINT('Ctrl Pts',(51.6340971610588,18.2136592897809,-172.065046651591));
#163703=CARTESIAN_POINT('Ctrl Pts',(51.6226621714695,18.2144217899579,-172.049490889624));
#163704=CARTESIAN_POINT('Ctrl Pts',(51.6107276602892,18.2152185412537,-172.034199306089));
#163705=CARTESIAN_POINT('Ctrl Pts',(51.598303131713,18.2160508793958,-172.019204984927));
#163706=CARTESIAN_POINT('Ctrl Pts',(51.5873494198683,18.2167846852791,-172.005985692758));
#163707=CARTESIAN_POINT('Ctrl Pts',(51.5760148706341,18.2175461554467,-171.992997455498));
#163708=CARTESIAN_POINT('Ctrl Pts',(51.5643074667153,18.2183364117946,-171.980262947367));
#163709=CARTESIAN_POINT('Ctrl Pts',(51.5590405928199,18.2186919287442,-171.974534004477));
#163710=CARTESIAN_POINT('Ctrl Pts',(51.5534163959643,18.2190750020736,-171.968556625618));
#163711=CARTESIAN_POINT('Ctrl Pts',(51.5478098427664,18.2194555391254,-171.962743472216));
#163712=CARTESIAN_POINT('Ctrl Pts',(51.5420205413225,18.2198484799619,-171.956740836337));
#163713=CARTESIAN_POINT('Ctrl Pts',(51.536250232312,18.2202387417562,-171.950913444314));
#163714=CARTESIAN_POINT('Ctrl Pts',(51.5309526830832,18.220598944004,-171.945675867929));
#163715=CARTESIAN_POINT('Ctrl Pts',(51.5299766807193,18.2206653064351,-171.944710914757));
#163716=CARTESIAN_POINT('Ctrl Pts',(51.5290168243772,18.2207306624763,-171.943765878212));
#163717=CARTESIAN_POINT('Ctrl Pts',(51.5280760753453,18.2207948582762,-171.942843218813));
#163718=CARTESIAN_POINT('Ctrl Pts',(51.5058324918989,18.2223127387999,-171.921027356531));
#163719=CARTESIAN_POINT('Ctrl Pts',(51.4819007881196,18.2239579199193,-171.899576783543));
#163720=CARTESIAN_POINT('Ctrl Pts',(51.4562139231078,18.2257209796507,-171.878780245327));
#163721=CARTESIAN_POINT('Ctrl Pts',(51.4311267483435,18.2274428786671,-171.858469226895));
#163722=CARTESIAN_POINT('Ctrl Pts',(51.4043649569905,18.2292771530807,-171.838782360866));
#163723=CARTESIAN_POINT('Ctrl Pts',(51.3759031475289,18.2312202329405,-171.820018775919));
#163724=CARTESIAN_POINT('Ctrl Pts',(51.3471011588778,18.2331865367396,-171.801030926204));
#163725=CARTESIAN_POINT('Ctrl Pts',(51.3165575490232,18.2352641608903,-171.782988824438));
#163726=CARTESIAN_POINT('Ctrl Pts',(51.2842935217107,18.2374560853849,-171.766229742036));
#163727=CARTESIAN_POINT('Ctrl Pts',(51.2681615080545,18.2385520476321,-171.757850200836));
#163728=CARTESIAN_POINT('Ctrl Pts',(51.2516001964196,18.2396766982955,-171.749791815609));
#163729=CARTESIAN_POINT('Ctrl Pts',(51.2346175177148,18.2408311519914,-171.742098872722));
#163730=CARTESIAN_POINT('Ctrl Pts',(51.2261261783623,18.2414083788394,-171.738252401278));
#163731=CARTESIAN_POINT('Ctrl Pts',(51.2175294997355,18.2419930567959,-171.734497284799));
#163732=CARTESIAN_POINT('Ctrl Pts',(51.2088288993997,18.2425853850868,-171.730839196982));
#163733=CARTESIAN_POINT('Ctrl Pts',(51.2044785992318,18.2428815492322,-171.729010153074));
#163734=CARTESIAN_POINT('Ctrl Pts',(51.2001023189545,18.2431796260059,-171.727205365629));
#163735=CARTESIAN_POINT('Ctrl Pts',(51.195700250897,18.243479642438,-171.725425545573));
#163736=CARTESIAN_POINT('Ctrl Pts',(51.1930275887413,18.2436617937708,-171.724344949442));
#163737=CARTESIAN_POINT('Ctrl Pts',(51.1896251319421,18.243894314396,-171.722986930825));
#163738=CARTESIAN_POINT('Ctrl Pts',(51.1868037301612,18.2440866095122,-171.721876575881));
#163739=CARTESIAN_POINT('Ctrl Pts',(51.1849780789541,18.2442110383735,-171.721158095848));
#163740=CARTESIAN_POINT('Ctrl Pts',(51.1833962626412,18.2443187013851,-171.720541970085));
#163741=CARTESIAN_POINT('Ctrl Pts',(51.1824168840543,18.2443855389116,-171.720161698938));
#163742=CARTESIAN_POINT('Ctrl Pts',(51.1668545868817,18.2454475852581,-171.714119201504));
#163743=CARTESIAN_POINT('Ctrl Pts',(51.1496401644066,18.2466376335613,-171.707866938366));
#163744=CARTESIAN_POINT('Ctrl Pts',(51.1307111623421,18.2479469064434,-171.701654178661));
#163745=CARTESIAN_POINT('Ctrl Pts',(51.1121989920192,18.2492273480912,-171.695578228886));
#163746=CARTESIAN_POINT('Ctrl Pts',(51.0920461656476,18.2506217147811,-171.689540171962));
#163747=CARTESIAN_POINT('Ctrl Pts',(51.0702102422606,18.2521240418244,-171.683820318885));
#163748=CARTESIAN_POINT('Ctrl Pts',(51.0492248312468,18.2535678530122,-171.678323254913));
#163749=CARTESIAN_POINT('Ctrl Pts',(51.026684241603,18.2551112879842,-171.673120412672));
#163750=CARTESIAN_POINT('Ctrl Pts',(51.0025757341803,18.2567525563699,-171.668501297324));
#163751=CARTESIAN_POINT('Ctrl Pts',(50.9790753248452,18.2583524264164,-171.663998691686));
#163752=CARTESIAN_POINT('Ctrl Pts',(50.9540844508566,18.260045165992,-171.660051059706));
#163753=CARTESIAN_POINT('Ctrl Pts',(50.9276248838668,18.2618338349027,-171.656961460484));
#163754=CARTESIAN_POINT('Ctrl Pts',(50.9021597323515,18.2635552812453,-171.653987975984));
#163755=CARTESIAN_POINT('Ctrl Pts',(50.8753337389174,18.2653655160331,-171.651809705488));
#163756=CARTESIAN_POINT('Ctrl Pts',(50.8472057061698,18.2672728034334,-171.650723766103));
#163757=CARTESIAN_POINT('Ctrl Pts',(50.8341169196676,18.268160319379,-171.650218447125));
#163758=CARTESIAN_POINT('Ctrl Pts',(50.820746813004,18.26906893619,-171.64995));
#163759=CARTESIAN_POINT('Ctrl Pts',(50.8071048221096,18.26999998,-171.64995));
#163760=CARTESIAN_POINT('Ctrl Pts',(52.3218461808875,18.76999998,-176.84995));
#163761=CARTESIAN_POINT('Ctrl Pts',(51.746661977277,18.76999998,-176.84995));
#163762=CARTESIAN_POINT('Ctrl Pts',(51.8267121465167,18.20041342952,-176.84995));
#163763=CARTESIAN_POINT('Ctrl Pts',(52.3218461808802,18.76999998,-176.981217345763));
#163764=CARTESIAN_POINT('Ctrl Pts',(51.7466619772798,18.7699999799806,-176.958917254526));
#163765=CARTESIAN_POINT('Ctrl Pts',(51.8267121465076,18.2004134295853,-177.112484691526));
#163766=CARTESIAN_POINT('Ctrl Pts',(52.3066996556685,18.8238865434699,-177.110943344657));
#163767=CARTESIAN_POINT('Ctrl Pts',(51.7419771601862,18.8033341856637,-177.069891898465));
#163768=CARTESIAN_POINT('Ctrl Pts',(51.8115656212979,18.3081865564618,-177.371936689315));
#163769=CARTESIAN_POINT('Ctrl Pts',(52.2546657912052,19.0090066353435,-177.29606343653));
#163770=CARTESIAN_POINT('Ctrl Pts',(51.721325635328,18.9502774203983,-177.257255781811));
#163771=CARTESIAN_POINT('Ctrl Pts',(51.7595317568342,18.6784267402051,-177.742176873059));
#163772=CARTESIAN_POINT('Ctrl Pts',(52.2182021908711,19.1387326342368,-177.34995));
#163773=CARTESIAN_POINT('Ctrl Pts',(51.7054679578625,19.0631106584802,-177.331204220089));
#163774=CARTESIAN_POINT('Ctrl Pts',(51.7230681564996,18.9378787379949,-177.849949999941));
#163775=CARTESIAN_POINT('Ctrl Pts',(52.1813053461851,19.26999998,-177.34995));
#163776=CARTESIAN_POINT('Ctrl Pts',(51.6861713118143,19.2004134295199,-177.34995));
#163777=CARTESIAN_POINT('Ctrl Pts',(51.6861713118143,19.20041342952,-177.84995));
#163778=CARTESIAN_POINT('',(51.6861713118143,19.20041342952,-177.84995));
#163779=CARTESIAN_POINT('Origin',(52.1813053461851,19.26999998,-177.84995));
#163780=CARTESIAN_POINT('',(52.3218461808875,18.76999998,-176.84995));
#163781=CARTESIAN_POINT('Ctrl Pts',(52.3218461808875,18.76999998,-176.84995));
#163782=CARTESIAN_POINT('Ctrl Pts',(52.3218461808861,18.76999998,-176.875860144688));
#163783=CARTESIAN_POINT('Ctrl Pts',(52.3212473348555,18.7721017641991,-176.902069110057));
#163784=CARTESIAN_POINT('Ctrl Pts',(52.3200442820214,18.7763470609339,-176.92825527987));
#163785=CARTESIAN_POINT('Ctrl Pts',(52.3188302824207,18.7806309862899,-176.954679721752));
#163786=CARTESIAN_POINT('Ctrl Pts',(52.3170010256884,18.7870976262972,-176.981080901352));
#163787=CARTESIAN_POINT('Ctrl Pts',(52.3145590515113,18.7957612416509,-177.007084281685));
#163788=CARTESIAN_POINT('Ctrl Pts',(52.313643533861,18.7990093074351,-177.016833178247));
#163789=CARTESIAN_POINT('Ctrl Pts',(52.3126419754868,18.802565885418,-177.026525725243));
#163790=CARTESIAN_POINT('Ctrl Pts',(52.3115547989476,18.8064306989981,-177.036140639572));
#163791=CARTESIAN_POINT('Ctrl Pts',(52.3087004133778,18.8165777797304,-177.061384628684));
#163792=CARTESIAN_POINT('Ctrl Pts',(52.3052525487689,18.8288564461382,-177.086112146138));
#163793=CARTESIAN_POINT('Ctrl Pts',(52.3012107145058,18.8432663804517,-177.10992591327));
#163794=CARTESIAN_POINT('Ctrl Pts',(52.3003951344565,18.8461740837797,-177.114731165565));
#163795=CARTESIAN_POINT('Ctrl Pts',(52.2995553821288,18.8491685216028,-177.119499049706));
#163796=CARTESIAN_POINT('Ctrl Pts',(52.2986914727062,18.8522496224732,-177.124226050751));
#163797=CARTESIAN_POINT('Ctrl Pts',(52.296118846023,18.8614247999918,-177.138302536896));
#163798=CARTESIAN_POINT('Ctrl Pts',(52.2933318195899,18.8713686406316,-177.152016545396));
#163799=CARTESIAN_POINT('Ctrl Pts',(52.2903303611667,18.8820727042616,-177.165265493094));
#163800=CARTESIAN_POINT('Ctrl Pts',(52.2888296319551,18.8874247360766,-177.171889966943));
#163801=CARTESIAN_POINT('Ctrl Pts',(52.2872752955732,18.8929667701014,-177.178398084151));
#163802=CARTESIAN_POINT('Ctrl Pts',(52.2856673543981,18.898696614487,-177.184775824956));
#163803=CARTESIAN_POINT('Ctrl Pts',(52.2848633838106,18.9015615366797,-177.187964695359));
#163804=CARTESIAN_POINT('Ctrl Pts',(52.2840460121149,18.9044734020793,-177.191120965597));
#163805=CARTESIAN_POINT('Ctrl Pts',(52.2832152400256,18.9074318583303,-177.194242832619));
#163806=CARTESIAN_POINT('Ctrl Pts',(52.2827332989327,18.9091480951386,-177.196053866022));
#163807=CARTESIAN_POINT('Ctrl Pts',(52.2821462621781,18.9112378961258,-177.198223860036));
#163808=CARTESIAN_POINT('Ctrl Pts',(52.2816282827859,18.9130815152767,-177.200104597065));
#163809=CARTESIAN_POINT('Ctrl Pts',(52.2812533671164,18.9144159345966,-177.201465882462));
#163810=CARTESIAN_POINT('Ctrl Pts',(52.280915005339,18.9156200460742,-177.202676847247));
#163811=CARTESIAN_POINT('Ctrl Pts',(52.2806826811287,18.9164465864338,-177.20350338762));
#163812=CARTESIAN_POINT('Ctrl Pts',(52.277929558952,18.9262413753247,-177.213298176676));
#163813=CARTESIAN_POINT('Ctrl Pts',(52.2748105907763,18.9371766657348,-177.223386446747));
#163814=CARTESIAN_POINT('Ctrl Pts',(52.2713164396122,18.9493814538919,-177.233531412315));
#163815=CARTESIAN_POINT('Ctrl Pts',(52.2679774498128,18.9610442759185,-177.243225880286));
#163816=CARTESIAN_POINT('Ctrl Pts',(52.2642956685592,18.9738670503152,-177.252972163816));
#163817=CARTESIAN_POINT('Ctrl Pts',(52.2602690639592,18.9879403213751,-177.262523160306));
#163818=CARTESIAN_POINT('Ctrl Pts',(52.2564813947795,19.0011784960526,-177.271507408483));
#163819=CARTESIAN_POINT('Ctrl Pts',(52.2523884994066,19.0155236005279,-177.28031878073));
#163820=CARTESIAN_POINT('Ctrl Pts',(52.2479962759463,19.031023301524,-177.288715370066));
#163821=CARTESIAN_POINT('Ctrl Pts',(52.2462319877114,19.0372492916992,-177.292088150143));
#163822=CARTESIAN_POINT('Ctrl Pts',(52.2444195008846,19.0436612159548,-177.295393584586));
#163823=CARTESIAN_POINT('Ctrl Pts',(52.2425596341985,19.0502605504507,-177.298614236585));
#163824=CARTESIAN_POINT('Ctrl Pts',(52.2382882913859,19.0654164861837,-177.306010739179));
#163825=CARTESIAN_POINT('Ctrl Pts',(52.2337758204442,19.0815733677847,-177.312967023157));
#163826=CARTESIAN_POINT('Ctrl Pts',(52.2290041102122,19.0987235689744,-177.319245722133));
#163827=CARTESIAN_POINT('Ctrl Pts',(52.2243617473424,19.1154088774575,-177.325354223609));
#163828=CARTESIAN_POINT('Ctrl Pts',(52.2194739113008,19.1330346888939,-177.330821391408));
#163829=CARTESIAN_POINT('Ctrl Pts',(52.214334287041,19.1515578420991,-177.335399595475));
#163830=CARTESIAN_POINT('Ctrl Pts',(52.2093027295161,19.1696915238984,-177.339881537337));
#163831=CARTESIAN_POINT('Ctrl Pts',(52.2040297688411,19.1886854887831,-177.343511544901));
#163832=CARTESIAN_POINT('Ctrl Pts',(52.1985209471977,19.2084598041589,-177.346028622878));
#163833=CARTESIAN_POINT('Ctrl Pts',(52.1930121255543,19.2282341195348,-177.348545700856));
#163834=CARTESIAN_POINT('Ctrl Pts',(52.1872673146857,19.2487891749223,-177.34995));
#163835=CARTESIAN_POINT('Ctrl Pts',(52.1813053461851,19.26999998,-177.34995));
#163836=CARTESIAN_POINT('',(51.8267121465167,18.20041342952,-176.84995));
#163837=CARTESIAN_POINT('Origin',(52.3218461808875,18.26999998,-176.84995));
#163838=CARTESIAN_POINT('Ctrl Pts',(51.6861713118143,19.20041342952,-177.84995));
#163839=CARTESIAN_POINT('Ctrl Pts',(51.7230681564996,18.9378787379949,-177.849949999941));
#163840=CARTESIAN_POINT('Ctrl Pts',(51.7595317568342,18.6784267402051,-177.742176873059));
#163841=CARTESIAN_POINT('Ctrl Pts',(51.7855486890661,18.4933066483335,-177.557056781187));
#163842=CARTESIAN_POINT('Ctrl Pts',(51.8115656212979,18.3081865564618,-177.371936689315));
#163843=CARTESIAN_POINT('Ctrl Pts',(51.8267121465076,18.2004134295853,-177.112484691526));
#163844=CARTESIAN_POINT('Ctrl Pts',(51.8267121465167,18.20041342952,-176.84995));
#163845=CARTESIAN_POINT('Origin',(53.107614345321,12.6789689739766,-177.84995));
#163846=CARTESIAN_POINT('',(51.6159008944631,19.70041342952,-177.84995));
#163847=CARTESIAN_POINT('',(52.6124803109502,12.6093824234965,-177.84995));
#163848=CARTESIAN_POINT('Origin',(52.1110349288339,19.76999998,-177.84995));
#163849=CARTESIAN_POINT('Ctrl Pts',(52.1110349288339,19.76999998,-177.34995));
#163850=CARTESIAN_POINT('Ctrl Pts',(51.6159008944631,19.70041342952,-177.34995));
#163851=CARTESIAN_POINT('Ctrl Pts',(51.6159008944631,19.70041342952,-177.84995));
#163852=CARTESIAN_POINT('Ctrl Pts',(52.0741380841476,19.9012673257632,-177.34995));
#163853=CARTESIAN_POINT('Ctrl Pts',(51.5974634812487,19.8316024412644,-177.367861075732));
#163854=CARTESIAN_POINT('Ctrl Pts',(51.5790040497779,19.9629481210451,-177.849949999941));
#163855=CARTESIAN_POINT('Ctrl Pts',(52.0376744838139,20.0309933246565,-177.29606343653));
#163856=CARTESIAN_POINT('Ctrl Pts',(51.5765113276013,19.980684760958,-177.329589659683));
#163857=CARTESIAN_POINT('Ctrl Pts',(51.5425404494433,20.2224001188348,-177.742176873059));
#163858=CARTESIAN_POINT('Ctrl Pts',(51.9856406193506,20.2161134165301,-177.110943344657));
#163859=CARTESIAN_POINT('Ctrl Pts',(51.5456194237325,20.2004920783894,-177.142957948484));
#163860=CARTESIAN_POINT('Ctrl Pts',(51.4905065849796,20.5926403025782,-177.371936689315));
#163861=CARTESIAN_POINT('Ctrl Pts',(51.9704940941388,20.26999998,-176.981217345763));
#163862=CARTESIAN_POINT('Ctrl Pts',(51.5358507252279,20.2699999799402,-176.997671841189));
#163863=CARTESIAN_POINT('Ctrl Pts',(51.4753600597699,20.7004134294547,-177.112484691526));
#163864=CARTESIAN_POINT('Ctrl Pts',(51.9704940941315,20.26999998,-176.84995));
#163865=CARTESIAN_POINT('Ctrl Pts',(51.5358507252234,20.26999998,-176.84995));
#163866=CARTESIAN_POINT('Ctrl Pts',(51.4753600597607,20.70041342952,-176.84995));
#163867=CARTESIAN_POINT('',(51.4753600597607,20.70041342952,-176.84995));
#163868=CARTESIAN_POINT('Ctrl Pts',(51.4753600597607,20.70041342952,-176.84995));
#163869=CARTESIAN_POINT('Ctrl Pts',(51.4753600597699,20.7004134294547,-177.112484691526));
#163870=CARTESIAN_POINT('Ctrl Pts',(51.4905065849796,20.5926403025782,-177.371936689315));
#163871=CARTESIAN_POINT('Ctrl Pts',(51.5165235172115,20.4075202107065,-177.557056781187));
#163872=CARTESIAN_POINT('Ctrl Pts',(51.5425404494433,20.2224001188348,-177.742176873059));
#163873=CARTESIAN_POINT('Ctrl Pts',(51.5790040497779,19.9629481210451,-177.849949999941));
#163874=CARTESIAN_POINT('Ctrl Pts',(51.6159008944631,19.70041342952,-177.84995));
#163875=CARTESIAN_POINT('',(51.9704940941315,20.26999998,-176.84995));
#163876=CARTESIAN_POINT('Origin',(51.9704940941315,20.76999998,-176.84995));
#163877=CARTESIAN_POINT('Ctrl Pts',(52.1110349288339,19.76999998,-177.34995));
#163878=CARTESIAN_POINT('Ctrl Pts',(52.1051573658154,19.790910496971,-177.34995));
#163879=CARTESIAN_POINT('Ctrl Pts',(52.0994600569256,19.8111797265574,-177.348585219103));
#163880=CARTESIAN_POINT('Ctrl Pts',(52.0939760868931,19.8306899637212,-177.346136042585));
#163881=CARTESIAN_POINT('Ctrl Pts',(52.0883714367758,19.8506295425955,-177.34363296956));
#163882=CARTESIAN_POINT('Ctrl Pts',(52.0829895372398,19.8697766450989,-177.339997193904));
#163883=CARTESIAN_POINT('Ctrl Pts',(52.077852760651,19.8880516774042,-177.335495637065));
#163884=CARTESIAN_POINT('Ctrl Pts',(52.0725516730947,19.9069112763512,-177.330850088143));
#163885=CARTESIAN_POINT('Ctrl Pts',(52.0675115638435,19.9248423967328,-177.325282469033));
#163886=CARTESIAN_POINT('Ctrl Pts',(52.0627445788973,19.9418018269093,-177.319052501404));
#163887=CARTESIAN_POINT('Ctrl Pts',(52.0583344844422,19.9574915531887,-177.313288953584));
#163888=CARTESIAN_POINT('Ctrl Pts',(52.0541579327436,19.972350407939,-177.306958054925));
#163889=CARTESIAN_POINT('Ctrl Pts',(52.0502165121628,19.986372740271,-177.300241546992));
#163890=CARTESIAN_POINT('Ctrl Pts',(52.0450870458873,20.0046217647853,-177.291500510549));
#163891=CARTESIAN_POINT('Ctrl Pts',(52.0403539659962,20.0214605714607,-177.282104513154));
#163892=CARTESIAN_POINT('Ctrl Pts',(52.036004156819,20.0369358217199,-177.272394745804));
#163893=CARTESIAN_POINT('Ctrl Pts',(52.0317077277822,20.0522211622615,-177.262804135117));
#163894=CARTESIAN_POINT('Ctrl Pts',(52.027785046931,20.0661768245414,-177.25290695541));
#163895=CARTESIAN_POINT('Ctrl Pts',(52.0242126622406,20.0788862434728,-177.242983685746));
#163896=CARTESIAN_POINT('Ctrl Pts',(52.0205954994723,20.0917549686943,-177.232936032798));
#163897=CARTESIAN_POINT('Ctrl Pts',(52.0173374020497,20.103346252571,-177.222861819816));
#163898=CARTESIAN_POINT('Ctrl Pts',(52.0144058949125,20.1137756311337,-177.213007508239));
#163899=CARTESIAN_POINT('Ctrl Pts',(52.0140516456167,20.1150359384904,-177.211816693149));
#163900=CARTESIAN_POINT('Ctrl Pts',(52.0137021577588,20.1162793061519,-177.21062903688));
#163901=CARTESIAN_POINT('Ctrl Pts',(52.0133573666424,20.1175059642869,-177.209444926111));
#163902=CARTESIAN_POINT('Ctrl Pts',(52.0130028066504,20.1187673770028,-177.208227266245));
#163903=CARTESIAN_POINT('Ctrl Pts',(52.012768176645,20.1196021166056,-177.207413007324));
#163904=CARTESIAN_POINT('Ctrl Pts',(52.0124419559371,20.120762651012,-177.206271333209));
#163905=CARTESIAN_POINT('Ctrl Pts',(52.0122347316986,20.1214998539325,-177.205546110857));
#163906=CARTESIAN_POINT('Ctrl Pts',(52.0119906191944,20.1223682710577,-177.204688490097));
#163907=CARTESIAN_POINT('Ctrl Pts',(52.0116574840334,20.1235533658466,-177.20350339534));
#163908=CARTESIAN_POINT('Ctrl Pts',(52.0058810051988,20.1441026076184,-177.18295415412));
#163909=CARTESIAN_POINT('Ctrl Pts',(52.0007010628878,20.1625302884788,-177.160790380055));
#163910=CARTESIAN_POINT('Ctrl Pts',(51.9961296377291,20.1787935349074,-177.137499857223));
#163911=CARTESIAN_POINT('Ctrl Pts',(51.9915524477765,20.1950772900965,-177.114179963887));
#163912=CARTESIAN_POINT('Ctrl Pts',(51.9875853054089,20.2091911675404,-177.089730492885));
#163913=CARTESIAN_POINT('Ctrl Pts',(51.9842337271962,20.2211153080935,-177.064594611035));
#163914=CARTESIAN_POINT('Ctrl Pts',(51.9808763648716,20.23306002718,-177.039415349994));
#163915=CARTESIAN_POINT('Ctrl Pts',(51.9781366859997,20.2428074708371,-177.013547307222));
#163916=CARTESIAN_POINT('Ctrl Pts',(51.9760138008928,20.2503605832966,-176.98738923323));
#163917=CARTESIAN_POINT('Ctrl Pts',(51.9738812665038,20.2579480273889,-176.961112261315));
#163918=CARTESIAN_POINT('Ctrl Pts',(51.9723711389257,20.2633211715772,-176.934542619689));
#163919=CARTESIAN_POINT('Ctrl Pts',(51.9714761292155,20.2665057300255,-176.908037354243));
#163920=CARTESIAN_POINT('Ctrl Pts',(51.9708197715504,20.2688411341264,-176.88859964989));
#163921=CARTESIAN_POINT('Ctrl Pts',(51.9704940941315,20.26999998,-176.869195582661));
#163922=CARTESIAN_POINT('Ctrl Pts',(51.9704940941315,20.26999998,-176.84995));
#163923=CARTESIAN_POINT('Origin',(51.6222122422086,12.4702093225365,-172.64995));
#163924=CARTESIAN_POINT('',(50.6813043436922,26.35041342952,-172.64995));
#163925=CARTESIAN_POINT('',(51.4753600597607,20.70041342952,-172.64995));
#163926=CARTESIAN_POINT('',(51.5358507252234,20.26999998,-172.64995));
#163927=CARTESIAN_POINT('Ctrl Pts',(50.6813043436922,26.35041342952,-172.64995));
#163928=CARTESIAN_POINT('Ctrl Pts',(50.6813043436922,26.35041342952,-172.608927207252));
#163929=CARTESIAN_POINT('Ctrl Pts',(50.6787227100171,26.3506218554067,-172.567506968074));
#163930=CARTESIAN_POINT('Ctrl Pts',(50.6734338193897,26.35102105198,-172.5260173808));
#163931=CARTESIAN_POINT('Ctrl Pts',(50.6682470560006,26.3514125401611,-172.485328947731));
#163932=CARTESIAN_POINT('Ctrl Pts',(50.660456259095,26.3519874576975,-172.444574188382));
#163933=CARTESIAN_POINT('Ctrl Pts',(50.649982463067,26.3527347066972,-172.404092569325));
#163934=CARTESIAN_POINT('Ctrl Pts',(50.6396244504326,26.3534736951746,-172.364058457478));
#163935=CARTESIAN_POINT('Ctrl Pts',(50.626642107556,26.3543811808045,-172.324291861792));
#163936=CARTESIAN_POINT('Ctrl Pts',(50.6110029101186,26.355452592592,-172.285145271694));
#163937=CARTESIAN_POINT('Ctrl Pts',(50.5956188188146,26.3565065275415,-172.246637239636));
#163938=CARTESIAN_POINT('Ctrl Pts',(50.5776636255519,26.357719053777,-172.20872959003));
#163939=CARTESIAN_POINT('Ctrl Pts',(50.5571529561684,26.3590923673666,-172.171775260274));
#163940=CARTESIAN_POINT('Ctrl Pts',(50.5438380830478,26.3599838787969,-172.147785686714));
#163941=CARTESIAN_POINT('Ctrl Pts',(50.5294472385948,26.3609432834134,-172.124198204066));
#163942=CARTESIAN_POINT('Ctrl Pts',(50.513996097651,26.3619727841711,-172.10111200409));
#163943=CARTESIAN_POINT('Ctrl Pts',(50.4951854859102,26.3632261245628,-172.073006277406));
#163944=CARTESIAN_POINT('Ctrl Pts',(50.4748027525668,26.3645832676277,-172.045643569251));
#163945=CARTESIAN_POINT('Ctrl Pts',(50.4528953288796,26.3660508793946,-172.019204984916));
#163946=CARTESIAN_POINT('Ctrl Pts',(50.4419416170359,26.366784685278,-172.005985692749));
#163947=CARTESIAN_POINT('Ctrl Pts',(50.430607067803,26.3675461554458,-171.99299745549));
#163948=CARTESIAN_POINT('Ctrl Pts',(50.4188996638857,26.3683364117939,-171.980262947361));
#163949=CARTESIAN_POINT('Ctrl Pts',(50.4136327899799,26.3686919287444,-171.97453400446));
#163950=CARTESIAN_POINT('Ctrl Pts',(50.4080085931148,26.3690750020745,-171.968556625591));
#163951=CARTESIAN_POINT('Ctrl Pts',(50.4024020399075,26.3694555391271,-171.96274347218));
#163952=CARTESIAN_POINT('Ctrl Pts',(50.396612738455,26.3698484799643,-171.956740836293));
#163953=CARTESIAN_POINT('Ctrl Pts',(50.3908424294362,26.3702387417594,-171.950913444262));
#163954=CARTESIAN_POINT('Ctrl Pts',(50.3855448801983,26.370598944008,-171.945675867869));
#163955=CARTESIAN_POINT('Ctrl Pts',(50.3845688778554,26.3706653064377,-171.944710914718));
#163956=CARTESIAN_POINT('Ctrl Pts',(50.3836090215335,26.3707306624775,-171.943765878193));
#163957=CARTESIAN_POINT('Ctrl Pts',(50.3826682725208,26.3707948582762,-171.942843218813));
#163958=CARTESIAN_POINT('Ctrl Pts',(50.3602740756354,26.3723230165153,-171.920879639234));
#163959=CARTESIAN_POINT('Ctrl Pts',(50.3361687783455,26.3739801992357,-171.899286273711));
#163960=CARTESIAN_POINT('Ctrl Pts',(50.3102840946091,26.37575680946,-171.878357889714));
#163961=CARTESIAN_POINT('Ctrl Pts',(50.2851107273834,26.3774845980647,-171.858004622076));
#163962=CARTESIAN_POINT('Ctrl Pts',(50.2582539920478,26.3793252796138,-171.838280617717));
#163963=CARTESIAN_POINT('Ctrl Pts',(50.229688635469,26.3812753050111,-171.819487495989));
#163964=CARTESIAN_POINT('Ctrl Pts',(50.2011232788901,26.3832253304083,-171.800694374262));
#163965=CARTESIAN_POINT('Ctrl Pts',(50.1708486900078,26.3852846137747,-171.782832445151));
#163966=CARTESIAN_POINT('Ctrl Pts',(50.138885718831,26.3874560853879,-171.766229742008));
#163967=CARTESIAN_POINT('Ctrl Pts',(50.1227537051804,26.3885520476348,-171.757850200811));
#163968=CARTESIAN_POINT('Ctrl Pts',(50.1061923935528,26.3896766982976,-171.749791815589));
#163969=CARTESIAN_POINT('Ctrl Pts',(50.0892097148571,26.3908311519931,-171.742098872707));
#163970=CARTESIAN_POINT('Ctrl Pts',(50.0807183755093,26.3914083788408,-171.738252401266));
#163971=CARTESIAN_POINT('Ctrl Pts',(50.0721216968875,26.391993056797,-171.734497284789));
#163972=CARTESIAN_POINT('Ctrl Pts',(50.0634210965573,26.3925853850876,-171.730839196975));
#163973=CARTESIAN_POINT('Ctrl Pts',(50.0590707963921,26.3928815492329,-171.729010153068));
#163974=CARTESIAN_POINT('Ctrl Pts',(50.0546945161177,26.3931796260065,-171.727205365624));
#163975=CARTESIAN_POINT('Ctrl Pts',(50.0502924480632,26.3934796424384,-171.725425545569));
#163976=CARTESIAN_POINT('Ctrl Pts',(50.0476197859243,26.3936617937702,-171.724344949445));
#163977=CARTESIAN_POINT('Ctrl Pts',(50.0442173291523,26.3938943143935,-171.722986930839));
#163978=CARTESIAN_POINT('Ctrl Pts',(50.0413959273829,26.3940866095089,-171.721876575899));
#163979=CARTESIAN_POINT('Ctrl Pts',(50.0395702761572,26.3942110383716,-171.721158095858));
#163980=CARTESIAN_POINT('Ctrl Pts',(50.0379884598262,26.3943187013844,-171.720541970088));
#163981=CARTESIAN_POINT('Ctrl Pts',(50.0370090812298,26.3943855389116,-171.720161698938));
#163982=CARTESIAN_POINT('Ctrl Pts',(50.0214467840286,26.3954475852603,-171.714119201493));
#163983=CARTESIAN_POINT('Ctrl Pts',(50.004232361525,26.3966376335655,-171.707866938345));
#163984=CARTESIAN_POINT('Ctrl Pts',(49.9853033594322,26.3979469064497,-171.701654178633));
#163985=CARTESIAN_POINT('Ctrl Pts',(49.9667911890826,26.3992273480994,-171.695578228851));
#163986=CARTESIAN_POINT('Ctrl Pts',(49.9466383626846,26.4006217147911,-171.689540171922));
#163987=CARTESIAN_POINT('Ctrl Pts',(49.9248024392717,26.4021240418361,-171.683820318842));
#163988=CARTESIAN_POINT('Ctrl Pts',(49.9038170282338,26.4035678530255,-171.678323254867));
#163989=CARTESIAN_POINT('Ctrl Pts',(49.8812764385664,26.405111287999,-171.673120412625));
#163990=CARTESIAN_POINT('Ctrl Pts',(49.8571679311208,26.4067525563862,-171.668501297279));
#163991=CARTESIAN_POINT('Ctrl Pts',(49.8336675217635,26.4083524264341,-171.663998691642));
#163992=CARTESIAN_POINT('Ctrl Pts',(49.8086766477535,26.410045166011,-171.660051059665));
#163993=CARTESIAN_POINT('Ctrl Pts',(49.7822170807432,26.411833834923,-171.656961460449));
#163994=CARTESIAN_POINT('Ctrl Pts',(49.7567519292073,26.4135552812669,-171.653987975954));
#163995=CARTESIAN_POINT('Ctrl Pts',(49.7299259357533,26.4153655160561,-171.651809705465));
#163996=CARTESIAN_POINT('Ctrl Pts',(49.701797902987,26.4172728034577,-171.650723766089));
#163997=CARTESIAN_POINT('Ctrl Pts',(49.6887091165988,26.4181603193956,-171.65021844712));
#163998=CARTESIAN_POINT('Ctrl Pts',(49.6753390100547,26.4190689361985,-171.64995));
#163999=CARTESIAN_POINT('Ctrl Pts',(49.6616970192851,26.41999998,-171.64995));
#164000=CARTESIAN_POINT('Ctrl Pts',(50.4557527353536,20.76999998,-171.64995));
#164001=CARTESIAN_POINT('Ctrl Pts',(50.4842042680624,20.7680582089184,-171.64995));
#164002=CARTESIAN_POINT('Ctrl Pts',(50.5114694452097,20.7661974046848,-171.651129585064));
#164003=CARTESIAN_POINT('Ctrl Pts',(50.5374753276717,20.7644225452763,-171.653192621543));
#164004=CARTESIAN_POINT('Ctrl Pts',(50.5648466522595,20.7625544966515,-171.655363978012));
#164005=CARTESIAN_POINT('Ctrl Pts',(50.5908233175796,20.7607816312657,-171.658513818819));
#164006=CARTESIAN_POINT('Ctrl Pts',(50.6153661207849,20.7591066246496,-171.662335033587));
#164007=CARTESIAN_POINT('Ctrl Pts',(50.6373318097271,20.757607501913,-171.665755002132));
#164008=CARTESIAN_POINT('Ctrl Pts',(50.6581499199593,20.756186699567,-171.669713339724));
#164009=CARTESIAN_POINT('Ctrl Pts',(50.6778170036355,20.7548444529213,-171.674015027575));
#164010=CARTESIAN_POINT('Ctrl Pts',(50.7013538125097,20.753238103791,-171.679163122048));
#164011=CARTESIAN_POINT('Ctrl Pts',(50.7232424486265,20.7517442397851,-171.684802100382));
#164012=CARTESIAN_POINT('Ctrl Pts',(50.7435076557478,20.7503611721819,-171.690639736304));
#164013=CARTESIAN_POINT('Ctrl Pts',(50.7646446447714,20.7489186068742,-171.696728499457));
#164014=CARTESIAN_POINT('Ctrl Pts',(50.7840164495197,20.7475965125377,-171.703033282349));
#164015=CARTESIAN_POINT('Ctrl Pts',(50.8016762225318,20.7463912615977,-171.709272496226));
#164016=CARTESIAN_POINT('Ctrl Pts',(50.8092483809043,20.7458744740382,-171.71194774667));
#164017=CARTESIAN_POINT('Ctrl Pts',(50.8165059618879,20.7453791558767,-171.71461154199));
#164018=CARTESIAN_POINT('Ctrl Pts',(50.823454146604,20.7449049535098,-171.717244495101));
#164019=CARTESIAN_POINT('Ctrl Pts',(50.8252179693497,20.7447845754607,-171.717912880122));
#164020=CARTESIAN_POINT('Ctrl Pts',(50.8260446003286,20.7447280884717,-171.718228248952));
#164021=CARTESIAN_POINT('Ctrl Pts',(50.8278165062487,20.7446071168896,-171.718908958993));
#164022=CARTESIAN_POINT('Ctrl Pts',(50.8286356820764,20.7445511901077,-171.719223660358));
#164023=CARTESIAN_POINT('Ctrl Pts',(50.8296567689968,20.7444814893959,-171.719616772033));
#164024=CARTESIAN_POINT('Ctrl Pts',(50.83106428527,20.7443854315169,-171.720163005656));
#164025=CARTESIAN_POINT('Ctrl Pts',(50.8360549385636,20.7440448375364,-171.72209979508));
#164026=CARTESIAN_POINT('Ctrl Pts',(50.841013474753,20.7437064347847,-171.724069245188));
#164027=CARTESIAN_POINT('Ctrl Pts',(50.8459395682395,20.743370245535,-171.72607046184));
#164028=CARTESIAN_POINT('Ctrl Pts',(50.8793181521241,20.7410922698724,-171.739630451729));
#164029=CARTESIAN_POINT('Ctrl Pts',(50.911195187842,20.7389167421848,-171.754642782237));
#164030=CARTESIAN_POINT('Ctrl Pts',(50.9415228493068,20.7368469422535,-171.770779293227));
#164031=CARTESIAN_POINT('Ctrl Pts',(50.9706035862437,20.7348622423324,-171.786252350117));
#164032=CARTESIAN_POINT('Ctrl Pts',(50.9982602416247,20.7329747203074,-171.802759466709));
#164033=CARTESIAN_POINT('Ctrl Pts',(51.0244817266949,20.7311851463697,-171.82004374659));
#164034=CARTESIAN_POINT('Ctrl Pts',(51.0538644581718,20.7291798224786,-171.839411808817));
#164035=CARTESIAN_POINT('Ctrl Pts',(51.0814456559995,20.7272974503447,-171.859755775677));
#164036=CARTESIAN_POINT('Ctrl Pts',(51.1072486905314,20.7255364349792,-171.880757614398));
#164037=CARTESIAN_POINT('Ctrl Pts',(51.1193846156018,20.7247081777253,-171.890635396049));
#164038=CARTESIAN_POINT('Ctrl Pts',(51.1311276872427,20.7239067320825,-171.900659292073));
#164039=CARTESIAN_POINT('Ctrl Pts',(51.1424827865761,20.723131764922,-171.910799109276));
#164040=CARTESIAN_POINT('Ctrl Pts',(51.1479796028623,20.7227566161026,-171.915707627529));
#164041=CARTESIAN_POINT('Ctrl Pts',(51.1530623502369,20.7224097268112,-171.92034885135));
#164042=CARTESIAN_POINT('Ctrl Pts',(51.1581876669761,20.7220599218499,-171.925124127321));
#164043=CARTESIAN_POINT('Ctrl Pts',(51.1631600281573,20.7217205561679,-171.929756894051));
#164044=CARTESIAN_POINT('Ctrl Pts',(51.1681726053704,20.7213784360359,-171.934515912431));
#164045=CARTESIAN_POINT('Ctrl Pts',(51.1736091589058,20.7210073610304,-171.93980158089));
#164046=CARTESIAN_POINT('Ctrl Pts',(51.1746317442697,20.7209375638938,-171.940795785613));
#164047=CARTESIAN_POINT('Ctrl Pts',(51.175669224257,20.7208667495451,-171.941808724727));
#164048=CARTESIAN_POINT('Ctrl Pts',(51.176723995822,20.7207947543338,-171.94284321151));
#164049=CARTESIAN_POINT('Ctrl Pts',(51.2111291405428,20.7184463731819,-171.976586695543));
#164050=CARTESIAN_POINT('Ctrl Pts',(51.2427228964462,20.7162900773892,-172.012463058233));
#164051=CARTESIAN_POINT('Ctrl Pts',(51.2713791089379,20.7143343614467,-172.04995975826));
#164052=CARTESIAN_POINT('Ctrl Pts',(51.3005002420468,20.712346915817,-172.088064807662));
#164053=CARTESIAN_POINT('Ctrl Pts',(51.3265877757913,20.7105666089751,-172.127843233128));
#164054=CARTESIAN_POINT('Ctrl Pts',(51.3495358206626,20.7090005519007,-172.168804472612));
#164055=CARTESIAN_POINT('Ctrl Pts',(51.3675548049889,20.7077708716366,-172.200967558242));
#164056=CARTESIAN_POINT('Ctrl Pts',(51.3836386764324,20.706673250415,-172.233860874994));
#164057=CARTESIAN_POINT('Ctrl Pts',(51.3977470738109,20.705710388276,-172.267266567535));
#164058=CARTESIAN_POINT('Ctrl Pts',(51.399144335016,20.7056150287623,-172.270574985704));
#164059=CARTESIAN_POINT('Ctrl Pts',(51.4005221974052,20.7055209925611,-172.273888354197));
#164060=CARTESIAN_POINT('Ctrl Pts',(51.4018807021469,20.7054282768102,-172.27720644154));
#164061=CARTESIAN_POINT('Ctrl Pts',(51.419643126508,20.7042160200817,-172.320590372151));
#164062=CARTESIAN_POINT('Ctrl Pts',(51.4340950438057,20.7032297001049,-172.364775502726));
#164063=CARTESIAN_POINT('Ctrl Pts',(51.4453314610336,20.7024628328062,-172.40926741461));
#164064=CARTESIAN_POINT('Ctrl Pts',(51.456700042584,20.7016869455063,-172.454282646629));
#164065=CARTESIAN_POINT('Ctrl Pts',(51.4647770536576,20.7011357025666,-172.499611950402));
#164066=CARTESIAN_POINT('Ctrl Pts',(51.4696694884625,20.7008018018056,-172.544796240755));
#164067=CARTESIAN_POINT('Ctrl Pts',(51.4734812148342,20.7005416576469,-172.57999960227));
#164068=CARTESIAN_POINT('Ctrl Pts',(51.4753600597607,20.70041342952,-172.615116019904));
#164069=CARTESIAN_POINT('Ctrl Pts',(51.4753600597607,20.70041342952,-172.64995));
#164070=CARTESIAN_POINT('Ctrl Pts',(51.176438378063,26.91999998,-176.84995));
#164071=CARTESIAN_POINT('Ctrl Pts',(50.6012541744525,26.9199999800001,-176.84995));
#164072=CARTESIAN_POINT('Ctrl Pts',(50.6813043436922,26.35041342952,-176.84995));
#164073=CARTESIAN_POINT('Ctrl Pts',(51.1764383780557,26.91999998,-176.981217345763));
#164074=CARTESIAN_POINT('Ctrl Pts',(50.6012541744552,26.9199999799806,-176.958917254526));
#164075=CARTESIAN_POINT('Ctrl Pts',(50.681304343683,26.3504134295853,-177.112484691526));
#164076=CARTESIAN_POINT('Ctrl Pts',(51.161291852844,26.9738865434699,-177.110943344657));
#164077=CARTESIAN_POINT('Ctrl Pts',(50.5965693573617,26.9533341856637,-177.069891898465));
#164078=CARTESIAN_POINT('Ctrl Pts',(50.6661578184733,26.4581865564618,-177.371936689315));
#164079=CARTESIAN_POINT('Ctrl Pts',(51.1092579883806,27.1590066353435,-177.29606343653));
#164080=CARTESIAN_POINT('Ctrl Pts',(50.5759178325036,27.1002774203984,-177.257255781812));
#164081=CARTESIAN_POINT('Ctrl Pts',(50.6141239540097,26.8284267402052,-177.742176873059));
#164082=CARTESIAN_POINT('Ctrl Pts',(51.0727943880466,27.2887326342368,-177.34995));
#164083=CARTESIAN_POINT('Ctrl Pts',(50.5600601550379,27.2131106584802,-177.331204220089));
#164084=CARTESIAN_POINT('Ctrl Pts',(50.5776603536751,27.0878787379949,-177.849949999941));
#164085=CARTESIAN_POINT('Ctrl Pts',(51.0358975433606,27.41999998,-177.34995));
#164086=CARTESIAN_POINT('Ctrl Pts',(50.5407635089898,27.35041342952,-177.34995));
#164087=CARTESIAN_POINT('Ctrl Pts',(50.5407635089898,27.3504134295199,-177.84995));
#164088=CARTESIAN_POINT('',(51.176438378063,26.91999998,-176.84995));
#164089=CARTESIAN_POINT('',(50.6813043436922,26.35041342952,-176.84995));
#164090=CARTESIAN_POINT('Origin',(51.176438378063,26.41999998,-176.84995));
#164091=CARTESIAN_POINT('',(50.5407635089898,27.3504134295199,-177.84995));
#164092=CARTESIAN_POINT('Ctrl Pts',(50.5407635089898,27.3504134295199,-177.84995));
#164093=CARTESIAN_POINT('Ctrl Pts',(50.5776603536751,27.0878787379949,-177.849949999941));
#164094=CARTESIAN_POINT('Ctrl Pts',(50.6141239540097,26.8284267402052,-177.742176873059));
#164095=CARTESIAN_POINT('Ctrl Pts',(50.6401408862415,26.6433066483335,-177.557056781187));
#164096=CARTESIAN_POINT('Ctrl Pts',(50.6661578184733,26.4581865564618,-177.371936689315));
#164097=CARTESIAN_POINT('Ctrl Pts',(50.681304343683,26.3504134295853,-177.112484691526));
#164098=CARTESIAN_POINT('Ctrl Pts',(50.6813043436922,26.35041342952,-176.84995));
#164099=CARTESIAN_POINT('Origin',(51.0358975433606,27.41999998,-177.84995));
#164100=CARTESIAN_POINT('Ctrl Pts',(51.176438378063,26.91999998,-176.84995));
#164101=CARTESIAN_POINT('Ctrl Pts',(51.1764383780616,26.91999998,-176.875860144656));
#164102=CARTESIAN_POINT('Ctrl Pts',(51.1758395320321,26.9221017641939,-176.902069109994));
#164103=CARTESIAN_POINT('Ctrl Pts',(51.1746364792001,26.9263470609191,-176.928255279779));
#164104=CARTESIAN_POINT('Ctrl Pts',(51.1734224796019,26.9306309862647,-176.954679721627));
#164105=CARTESIAN_POINT('Ctrl Pts',(51.1715932228734,26.9370976262562,-176.981080901196));
#164106=CARTESIAN_POINT('Ctrl Pts',(51.1691512487013,26.9457612415897,-177.007084281502));
#164107=CARTESIAN_POINT('Ctrl Pts',(51.1682357310471,26.9490093073872,-177.016833178116));
#164108=CARTESIAN_POINT('Ctrl Pts',(51.167234172668,26.9525658853867,-177.026525725163));
#164109=CARTESIAN_POINT('Ctrl Pts',(51.1661469961231,26.9564306989867,-177.036140639544));
#164110=CARTESIAN_POINT('Ctrl Pts',(51.1632926105572,26.9665777797031,-177.06138462862));
#164111=CARTESIAN_POINT('Ctrl Pts',(51.1598447459541,26.9788564460896,-177.086112146043));
#164112=CARTESIAN_POINT('Ctrl Pts',(51.1558029116984,26.9932663803772,-177.109925913147));
#164113=CARTESIAN_POINT('Ctrl Pts',(51.1549873316437,26.9961740837246,-177.114731165477));
#164114=CARTESIAN_POINT('Ctrl Pts',(51.1541475793103,26.9991685215683,-177.119499049653));
#164115=CARTESIAN_POINT('Ctrl Pts',(51.1532836698816,27.0022496224607,-177.124226050732));
#164116=CARTESIAN_POINT('Ctrl Pts',(51.1507110431984,27.0114247999801,-177.138302536879));
#164117=CARTESIAN_POINT('Ctrl Pts',(51.1479240167653,27.0213686406213,-177.152016545382));
#164118=CARTESIAN_POINT('Ctrl Pts',(51.1449225583421,27.0320727042533,-177.165265493083));
#164119=CARTESIAN_POINT('Ctrl Pts',(51.1434218291305,27.0374247360693,-177.171889966934));
#164120=CARTESIAN_POINT('Ctrl Pts',(51.1418674927487,27.0429667700952,-177.178398084144));
#164121=CARTESIAN_POINT('Ctrl Pts',(51.1402595515736,27.0486966144822,-177.184775824951));
#164122=CARTESIAN_POINT('Ctrl Pts',(51.139455580986,27.0515615366757,-177.187964695355));
#164123=CARTESIAN_POINT('Ctrl Pts',(51.1386382092902,27.0544734020759,-177.191120965594));
#164124=CARTESIAN_POINT('Ctrl Pts',(51.137807437201,27.0574318583278,-177.194242832616));
#164125=CARTESIAN_POINT('Ctrl Pts',(51.1373254961083,27.0591480951356,-177.196053866019));
#164126=CARTESIAN_POINT('Ctrl Pts',(51.136738459354,27.0612378961227,-177.198223860033));
#164127=CARTESIAN_POINT('Ctrl Pts',(51.1362204799618,27.0630815152736,-177.200104597062));
#164128=CARTESIAN_POINT('Ctrl Pts',(51.135845564292,27.0644159345951,-177.20146588246));
#164129=CARTESIAN_POINT('Ctrl Pts',(51.1355072025142,27.0656200460742,-177.202676847247));
#164130=CARTESIAN_POINT('Ctrl Pts',(51.135274878304,27.0664465864337,-177.20350338762));
#164131=CARTESIAN_POINT('Ctrl Pts',(51.1325217561302,27.0762413753144,-177.213298176666));
#164132=CARTESIAN_POINT('Ctrl Pts',(51.1294027879578,27.087176665714,-177.223386446728));
#164133=CARTESIAN_POINT('Ctrl Pts',(51.125908636797,27.0993814538605,-177.233531412289));
#164134=CARTESIAN_POINT('Ctrl Pts',(51.1225696470007,27.111044275877,-177.243225880253));
#164135=CARTESIAN_POINT('Ctrl Pts',(51.1188878657503,27.1238670502636,-177.252972163778));
#164136=CARTESIAN_POINT('Ctrl Pts',(51.1148612611533,27.1379403213136,-177.262523160264));
#164137=CARTESIAN_POINT('Ctrl Pts',(51.1110735919767,27.1511784959811,-177.271507408437));
#164138=CARTESIAN_POINT('Ctrl Pts',(51.1069806966066,27.1655236004465,-177.280318780682));
#164139=CARTESIAN_POINT('Ctrl Pts',(51.102588473149,27.1810233014328,-177.288715370017));
#164140=CARTESIAN_POINT('Ctrl Pts',(51.1008241849099,27.187249291623,-177.292088150103));
#164141=CARTESIAN_POINT('Ctrl Pts',(51.0990116980784,27.1936612158948,-177.295393584556));
#164142=CARTESIAN_POINT('Ctrl Pts',(51.0971518313873,27.2002605504079,-177.298614236564));
#164143=CARTESIAN_POINT('Ctrl Pts',(51.0928804885768,27.2154164861333,-177.306010739157));
#164144=CARTESIAN_POINT('Ctrl Pts',(51.0883680176369,27.2315733677267,-177.312967023133));
#164145=CARTESIAN_POINT('Ctrl Pts',(51.0835963074068,27.248723568909,-177.319245722109));
#164146=CARTESIAN_POINT('Ctrl Pts',(51.078953944539,27.2654088773845,-177.325354223585));
#164147=CARTESIAN_POINT('Ctrl Pts',(51.0740661084993,27.2830346888134,-177.330821391385));
#164148=CARTESIAN_POINT('Ctrl Pts',(51.0689264842414,27.3015578420114,-177.335399595453));
#164149=CARTESIAN_POINT('Ctrl Pts',(51.0638949267134,27.3196915238215,-177.339881537321));
#164150=CARTESIAN_POINT('Ctrl Pts',(51.0586219660347,27.3386854887189,-177.343511544891));
#164151=CARTESIAN_POINT('Ctrl Pts',(51.0531131443872,27.3584598041094,-177.346028622872));
#164152=CARTESIAN_POINT('Ctrl Pts',(51.0476043227396,27.3782341195,-177.348545700853));
#164153=CARTESIAN_POINT('Ctrl Pts',(51.0418595118664,27.3987891749041,-177.34995));
#164154=CARTESIAN_POINT('Ctrl Pts',(51.0358975433606,27.41999998,-177.34995));
#164155=CARTESIAN_POINT('Origin',(53.107614345321,12.6789689739766,-177.84995));
#164156=CARTESIAN_POINT('',(50.4704930916386,27.85041342952,-177.84995));
#164157=CARTESIAN_POINT('',(52.6124803109502,12.6093824234965,-177.84995));
#164158=CARTESIAN_POINT('Origin',(50.9656271260094,27.91999998,-177.84995));
#164159=CARTESIAN_POINT('Ctrl Pts',(50.9656271260094,27.91999998,-177.34995));
#164160=CARTESIAN_POINT('Ctrl Pts',(50.4704930916386,27.85041342952,-177.34995));
#164161=CARTESIAN_POINT('Ctrl Pts',(50.4704930916386,27.85041342952,-177.84995));
#164162=CARTESIAN_POINT('Ctrl Pts',(50.9287302813235,28.0512673257631,-177.34995));
#164163=CARTESIAN_POINT('Ctrl Pts',(50.4520556784241,27.9816024412645,-177.367861075731));
#164164=CARTESIAN_POINT('Ctrl Pts',(50.4335962469534,28.1129481210447,-177.849949999941));
#164165=CARTESIAN_POINT('Ctrl Pts',(50.8922666809894,28.1809933246567,-177.29606343653));
#164166=CARTESIAN_POINT('Ctrl Pts',(50.4311035247778,28.1306847609584,-177.32958965968));
#164167=CARTESIAN_POINT('Ctrl Pts',(50.3971326466187,28.3724001188352,-177.742176873059));
#164168=CARTESIAN_POINT('Ctrl Pts',(50.840232816526,28.3661134165298,-177.110943344657));
#164169=CARTESIAN_POINT('Ctrl Pts',(50.4002116209072,28.3504920783889,-177.142957948487));
#164170=CARTESIAN_POINT('Ctrl Pts',(50.3450987821552,28.7426403025778,-177.371936689315));
#164171=CARTESIAN_POINT('Ctrl Pts',(50.8250862913143,28.41999998,-176.981217345763));
#164172=CARTESIAN_POINT('Ctrl Pts',(50.3904429224034,28.4199999799438,-176.997671841187));
#164173=CARTESIAN_POINT('Ctrl Pts',(50.3299522569454,28.8504134294547,-177.112484691526));
#164174=CARTESIAN_POINT('Ctrl Pts',(50.825086291307,28.41999998,-176.84995));
#164175=CARTESIAN_POINT('Ctrl Pts',(50.3904429223989,28.41999998,-176.84995));
#164176=CARTESIAN_POINT('Ctrl Pts',(50.3299522569362,28.85041342952,-176.84995));
#164177=CARTESIAN_POINT('',(50.3299522569362,28.85041342952,-176.84995));
#164178=CARTESIAN_POINT('Ctrl Pts',(50.3299522569362,28.85041342952,-176.84995));
#164179=CARTESIAN_POINT('Ctrl Pts',(50.3299522569454,28.8504134294547,-177.112484691526));
#164180=CARTESIAN_POINT('Ctrl Pts',(50.3450987821552,28.7426403025778,-177.371936689315));
#164181=CARTESIAN_POINT('Ctrl Pts',(50.3711157143869,28.5575202107065,-177.557056781187));
#164182=CARTESIAN_POINT('Ctrl Pts',(50.3971326466187,28.3724001188352,-177.742176873059));
#164183=CARTESIAN_POINT('Ctrl Pts',(50.4335962469534,28.1129481210447,-177.849949999941));
#164184=CARTESIAN_POINT('Ctrl Pts',(50.4704930916386,27.85041342952,-177.84995));
#164185=CARTESIAN_POINT('',(50.825086291307,28.41999998,-176.84995));
#164186=CARTESIAN_POINT('Origin',(50.825086291307,28.91999998,-176.84995));
#164187=CARTESIAN_POINT('Ctrl Pts',(50.9656271260094,27.91999998,-177.34995));
#164188=CARTESIAN_POINT('Ctrl Pts',(50.9597495629756,27.9409104970259,-177.34995));
#164189=CARTESIAN_POINT('Ctrl Pts',(50.9540522540723,27.9611797266605,-177.348585219096));
#164190=CARTESIAN_POINT('Ctrl Pts',(50.9485682840283,27.9806899638649,-177.346136042567));
#164191=CARTESIAN_POINT('Ctrl Pts',(50.9429636339204,28.0006295427059,-177.343632969541));
#164192=CARTESIAN_POINT('Ctrl Pts',(50.9375817343943,28.0197766451743,-177.339997193887));
#164193=CARTESIAN_POINT('Ctrl Pts',(50.9324449578157,28.0380516774433,-177.335495637055));
#164194=CARTESIAN_POINT('Ctrl Pts',(50.927143870269,28.056911276356,-177.33085008814));
#164195=CARTESIAN_POINT('Ctrl Pts',(50.9221037610279,28.0748423967018,-177.325282469042));
#164196=CARTESIAN_POINT('Ctrl Pts',(50.917336776092,28.0918018268417,-177.319052501429));
#164197=CARTESIAN_POINT('Ctrl Pts',(50.9129266816434,28.107491553098,-177.31328895362));
#164198=CARTESIAN_POINT('Ctrl Pts',(50.9087501299518,28.1223504078232,-177.306958054975));
#164199=CARTESIAN_POINT('Ctrl Pts',(50.9048087093783,28.1363727401291,-177.30024154706));
#164200=CARTESIAN_POINT('Ctrl Pts',(50.8996792431315,28.1546217645412,-177.291500510673));
#164201=CARTESIAN_POINT('Ctrl Pts',(50.8949461632669,28.1714605711226,-177.282104513345));
#164202=CARTESIAN_POINT('Ctrl Pts',(50.8905963541135,28.1869358212966,-177.27239474607));
#164203=CARTESIAN_POINT('Ctrl Pts',(50.8862999250947,28.2022211617742,-177.262804135444));
#164204=CARTESIAN_POINT('Ctrl Pts',(50.88237724426,28.216176823995,-177.252906955805));
#164205=CARTESIAN_POINT('Ctrl Pts',(50.8788048595848,28.2288862428727,-177.242983686215));
#164206=CARTESIAN_POINT('Ctrl Pts',(50.8751876970077,28.2417549674139,-177.232936033829));
#164207=CARTESIAN_POINT('Ctrl Pts',(50.8719295997398,28.2533462507402,-177.222861821418));
#164208=CARTESIAN_POINT('Ctrl Pts',(50.8689980927258,28.2637756288644,-177.213007510384));
#164209=CARTESIAN_POINT('Ctrl Pts',(50.8686438432088,28.2650359370083,-177.211816694565));
#164210=CARTESIAN_POINT('Ctrl Pts',(50.8682943551355,28.266279305436,-177.210629037571));
#164211=CARTESIAN_POINT('Ctrl Pts',(50.8679495638095,28.2675059643168,-177.209444926082));
#164212=CARTESIAN_POINT('Ctrl Pts',(50.8675950038203,28.2687673770226,-177.208227266226));
#164213=CARTESIAN_POINT('Ctrl Pts',(50.8673603738187,28.2696021166119,-177.207413007318));
#164214=CARTESIAN_POINT('Ctrl Pts',(50.8670341531148,28.2707626510054,-177.206271333216));
#164215=CARTESIAN_POINT('Ctrl Pts',(50.8668269288771,28.2714998539238,-177.205546110866));
#164216=CARTESIAN_POINT('Ctrl Pts',(50.8665828163733,28.2723682710494,-177.204688490105));
#164217=CARTESIAN_POINT('Ctrl Pts',(50.8662496812106,28.2735533658467,-177.20350339534));
#164218=CARTESIAN_POINT('Ctrl Pts',(50.8604732024432,28.2941026074213,-177.182954154317));
#164219=CARTESIAN_POINT('Ctrl Pts',(50.8552932601851,28.312530288117,-177.160790380489));
#164220=CARTESIAN_POINT('Ctrl Pts',(50.8507218350651,28.3287935344193,-177.137499857922));
#164221=CARTESIAN_POINT('Ctrl Pts',(50.8461446451417,28.3450772895161,-177.114179964803));
#164222=CARTESIAN_POINT('Ctrl Pts',(50.8421775027915,28.3591911668972,-177.089730494042));
#164223=CARTESIAN_POINT('Ctrl Pts',(50.8388259245845,28.3711153074227,-177.064594612449));
#164224=CARTESIAN_POINT('Ctrl Pts',(50.8354685622628,28.3830600264916,-177.039415351644));
#164225=CARTESIAN_POINT('Ctrl Pts',(50.8327288833832,28.3928074701625,-177.013547309123));
#164226=CARTESIAN_POINT('Ctrl Pts',(50.8306059982581,28.4003605826727,-176.987389235391));
#164227=CARTESIAN_POINT('Ctrl Pts',(50.8284734638487,28.4079480268235,-176.961112263709));
#164228=CARTESIAN_POINT('Ctrl Pts',(50.8269633362407,28.4133211711029,-176.934542622323));
#164229=CARTESIAN_POINT('Ctrl Pts',(50.8260683264915,28.4165057296799,-176.90803735712));
#164230=CARTESIAN_POINT('Ctrl Pts',(50.8254119687592,28.4188411340129,-176.888599651797));
#164231=CARTESIAN_POINT('Ctrl Pts',(50.825086291307,28.41999998,-176.869195583603));
#164232=CARTESIAN_POINT('Ctrl Pts',(50.825086291307,28.41999998,-176.84995));
#164233=CARTESIAN_POINT('Origin',(51.6222122422086,12.4702093225365,-172.64995));
#164234=CARTESIAN_POINT('',(49.3103449325291,28.91999998,-171.64995));
#164235=CARTESIAN_POINT('',(48.9446667094463,31.5219357366587,-171.64995));
#164236=CARTESIAN_POINT('',(48.9446667094463,31.5219357366587,-171.64995));
#164237=CARTESIAN_POINT('',(50.3299522569362,28.85041342952,-172.64995));
#164238=CARTESIAN_POINT('Ctrl Pts',(49.3103449325291,28.91999998,-171.64995));
#164239=CARTESIAN_POINT('Ctrl Pts',(49.3387697982907,28.9180600288945,-171.64995));
#164240=CARTESIAN_POINT('Ctrl Pts',(49.3660105379016,28.9162008924831,-171.651127379994));
#164241=CARTESIAN_POINT('Ctrl Pts',(49.39199439745,28.9144275361028,-171.653186822974));
#164242=CARTESIAN_POINT('Ctrl Pts',(49.4189288617229,28.9125893024879,-171.655321609504));
#164243=CARTESIAN_POINT('Ctrl Pts',(49.4445132303009,28.91084321072,-171.658404102285));
#164244=CARTESIAN_POINT('Ctrl Pts',(49.4687098143076,28.9091918330042,-171.662141420469));
#164245=CARTESIAN_POINT('Ctrl Pts',(49.4943977208127,28.9074386749403,-171.666109083014));
#164246=CARTESIAN_POINT('Ctrl Pts',(49.5185218170459,28.9057922443977,-171.670814501406));
#164247=CARTESIAN_POINT('Ctrl Pts',(49.5410788798076,28.9042527613546,-171.675950032829));
#164248=CARTESIAN_POINT('Ctrl Pts',(49.5642968214887,28.9026681743944,-171.681236025528));
#164249=CARTESIAN_POINT('Ctrl Pts',(49.58585545163,28.9011968327624,-171.686977732447));
#164250=CARTESIAN_POINT('Ctrl Pts',(49.6057833608668,28.8998367851943,-171.692885218569));
#164251=CARTESIAN_POINT('Ctrl Pts',(49.6265086028921,28.8984223209531,-171.699029068292));
#164252=CARTESIAN_POINT('Ctrl Pts',(49.6454709588003,28.8971281708376,-171.705352160828));
#164253=CARTESIAN_POINT('Ctrl Pts',(49.6627257368561,28.8959505601483,-171.71157813447));
#164254=CARTESIAN_POINT('Ctrl Pts',(49.6679908341232,28.8955912257771,-171.713477918791));
#164255=CARTESIAN_POINT('Ctrl Pts',(49.6730970826779,28.8952427325736,-171.715369016405));
#164256=CARTESIAN_POINT('Ctrl Pts',(49.6780463437716,28.8949049535104,-171.717244495098));
#164257=CARTESIAN_POINT('Ctrl Pts',(49.6798101665193,28.8947845754611,-171.717912880119));
#164258=CARTESIAN_POINT('Ctrl Pts',(49.6806367975012,28.8947280884719,-171.718228248951));
#164259=CARTESIAN_POINT('Ctrl Pts',(49.6824087034236,28.8946071168897,-171.718908958993));
#164260=CARTESIAN_POINT('Ctrl Pts',(49.6832278792519,28.8945511901078,-171.719223660358));
#164261=CARTESIAN_POINT('Ctrl Pts',(49.6842489661727,28.8944814893959,-171.719616772033));
#164262=CARTESIAN_POINT('Ctrl Pts',(49.6856564824454,28.894385431517,-171.720163005656));
#164263=CARTESIAN_POINT('Ctrl Pts',(49.6906471357391,28.8940448375365,-171.72209979508));
#164264=CARTESIAN_POINT('Ctrl Pts',(49.6956056719285,28.8937064347848,-171.724069245188));
#164265=CARTESIAN_POINT('Ctrl Pts',(49.700531765415,28.8933702455351,-171.72607046184));
#164266=CARTESIAN_POINT('Ctrl Pts',(49.7339103492972,28.8910922698726,-171.739630451728));
#164267=CARTESIAN_POINT('Ctrl Pts',(49.7657873850126,28.8889167421851,-171.754642782234));
#164268=CARTESIAN_POINT('Ctrl Pts',(49.7961150464751,28.886846942254,-171.770779293223));
#164269=CARTESIAN_POINT('Ctrl Pts',(49.8251957834159,28.8848622423326,-171.786252350114));
#164270=CARTESIAN_POINT('Ctrl Pts',(49.8528524388002,28.8829747203074,-171.802759466709));
#164271=CARTESIAN_POINT('Ctrl Pts',(49.8790739238732,28.8811851463695,-171.820043746592));
#164272=CARTESIAN_POINT('Ctrl Pts',(49.9084566554647,28.8791798224706,-171.839411808894));
#164273=CARTESIAN_POINT('Ctrl Pts',(49.9360378533926,28.8772974503299,-171.859755775837));
#164274=CARTESIAN_POINT('Ctrl Pts',(49.9618408880107,28.8755364349585,-171.880757614645));
#164275=CARTESIAN_POINT('Ctrl Pts',(49.9739768129737,28.8747081777119,-171.890635396217));
#164276=CARTESIAN_POINT('Ctrl Pts',(49.9857198845137,28.873906732076,-171.900659292158));
#164277=CARTESIAN_POINT('Ctrl Pts',(49.9970749837527,28.8731317649219,-171.910799109277));
#164278=CARTESIAN_POINT('Ctrl Pts',(50.0025718000368,28.8727566161027,-171.915707627528));
#164279=CARTESIAN_POINT('Ctrl Pts',(50.0076545474091,28.8724097268114,-171.920348851347));
#164280=CARTESIAN_POINT('Ctrl Pts',(50.012779864146,28.8720599218503,-171.925124127316));
#164281=CARTESIAN_POINT('Ctrl Pts',(50.0177522253248,28.8717205561685,-171.929756894044));
#164282=CARTESIAN_POINT('Ctrl Pts',(50.0227648025355,28.8713784360368,-171.934515912421));
#164283=CARTESIAN_POINT('Ctrl Pts',(50.0282013560687,28.8710073610315,-171.939801580878));
#164284=CARTESIAN_POINT('Ctrl Pts',(50.0292239414366,28.8709375638947,-171.940795785605));
#164285=CARTESIAN_POINT('Ctrl Pts',(50.0302614214281,28.8708667495457,-171.941808724723));
#164286=CARTESIAN_POINT('Ctrl Pts',(50.0313161929975,28.8707947543342,-171.94284321151));
#164287=CARTESIAN_POINT('Ctrl Pts',(50.0657213376989,28.8684463731845,-171.976586695524));
#164288=CARTESIAN_POINT('Ctrl Pts',(50.0973150935852,28.8662900773931,-172.012463058192));
#164289=CARTESIAN_POINT('Ctrl Pts',(50.1259713060629,28.8643343614516,-172.049959758195));
#164290=CARTESIAN_POINT('Ctrl Pts',(50.1550924391609,28.8623469158224,-172.088064807575));
#164291=CARTESIAN_POINT('Ctrl Pts',(50.1811799728969,28.8605666089807,-172.127843233018));
#164292=CARTESIAN_POINT('Ctrl Pts',(50.2041280177626,28.8590005519064,-172.168804472477));
#164293=CARTESIAN_POINT('Ctrl Pts',(50.2221470021198,28.8577708716399,-172.200967558151));
#164294=CARTESIAN_POINT('Ctrl Pts',(50.2382308735885,28.8566732504164,-172.233860874948));
#164295=CARTESIAN_POINT('Ctrl Pts',(50.2523392709864,28.855710388276,-172.267266567535));
#164296=CARTESIAN_POINT('Ctrl Pts',(50.2537365321953,28.8556150287621,-172.270574985713));
#164297=CARTESIAN_POINT('Ctrl Pts',(50.2551143945883,28.8555209925606,-172.273888354216));
#164298=CARTESIAN_POINT('Ctrl Pts',(50.2564728993336,28.8554282768094,-172.277206441568));
#164299=CARTESIAN_POINT('Ctrl Pts',(50.2742353236811,28.8542160200819,-172.320590372148));
#164300=CARTESIAN_POINT('Ctrl Pts',(50.2886872409692,28.8532297001058,-172.364775502692));
#164301=CARTESIAN_POINT('Ctrl Pts',(50.2999236581919,28.8524628328074,-172.409267414542));
#164302=CARTESIAN_POINT('Ctrl Pts',(50.3112922397379,28.8516869455078,-172.45428264653));
#164303=CARTESIAN_POINT('Ctrl Pts',(50.3193692508111,28.8511357025681,-172.49961195027));
#164304=CARTESIAN_POINT('Ctrl Pts',(50.3242616856201,28.8508018018068,-172.54479624059));
#164305=CARTESIAN_POINT('Ctrl Pts',(50.3280734120039,28.8505416576473,-172.579999602161));
#164306=CARTESIAN_POINT('Ctrl Pts',(50.3299522569362,28.85041342952,-172.615116019851));
#164307=CARTESIAN_POINT('Ctrl Pts',(50.3299522569362,28.85041342952,-172.64995));
#164308=CARTESIAN_POINT('',(49.9349347781878,31.6611088376188,-172.64995));
#164309=CARTESIAN_POINT('',(50.3904429223989,28.41999998,-172.64995));
#164310=CARTESIAN_POINT('Origin',(48.9446667094463,31.5219357366587,-172.64995));
#164311=CARTESIAN_POINT('Origin',(46.9641305719631,31.2435895347386,-172.64995));
#164312=CARTESIAN_POINT('',(49.1485087381009,33.2999192814719,-172.64995));
#164313=CARTESIAN_POINT('Origin',(46.9641305719631,31.2435895347386,-172.64995));
#164314=CARTESIAN_POINT('',(48.4203826827217,32.6144760325608,-171.64995));
#164315=CARTESIAN_POINT('Origin',(48.4203826827217,32.6144760325608,-172.64995));
#164316=CARTESIAN_POINT('Origin',(46.9641305719631,31.2435895347386,-171.64995));
#164317=CARTESIAN_POINT('Origin',(0.,-12.9675000200281,-172.64995));
#164318=CARTESIAN_POINT('',(46.2674193015002,36.1810087180727,-172.64995));
#164319=CARTESIAN_POINT('Origin',(0.,-12.9675000200281,-172.64995));
#164320=CARTESIAN_POINT('',(45.5819760525891,35.4528826626933,-171.64995));
#164321=CARTESIAN_POINT('Origin',(45.5819760525891,35.4528826626933,-172.64995));
#164322=CARTESIAN_POINT('Origin',(0.,-12.9675000200281,-171.64995));
#164323=CARTESIAN_POINT('Origin',(44.2110895547669,33.9966305519348,-172.64995));
#164324=CARTESIAN_POINT('',(44.628608857647,36.9674347581595,-172.64995));
#164325=CARTESIAN_POINT('Origin',(44.2110895547669,33.9966305519348,-172.64995));
#164326=CARTESIAN_POINT('',(44.489435756687,35.9771666894179,-171.64995));
#164327=CARTESIAN_POINT('Origin',(44.489435756687,35.9771666894179,-172.64995));
#164328=CARTESIAN_POINT('Origin',(44.2110895547669,33.9966305519348,-171.64995));
#164329=CARTESIAN_POINT('Origin',(45.4220505312374,35.8460962305468,-172.64995));
#164330=CARTESIAN_POINT('',(41.93041344952,37.3466413930079,-172.64995));
#164331=CARTESIAN_POINT('',(44.628608857647,36.9674347581595,-172.64995));
#164332=CARTESIAN_POINT('',(42.,36.3270340686007,-171.64995));
#164333=CARTESIAN_POINT('Ctrl Pts',(41.93041344952,37.3466413930079,-172.64995));
#164334=CARTESIAN_POINT('Ctrl Pts',(41.93041344952,37.3466413930079,-172.605172304593));
#164335=CARTESIAN_POINT('Ctrl Pts',(41.9306253528176,37.3435365091946,-172.559925284252));
#164336=CARTESIAN_POINT('Ctrl Pts',(41.9310569582364,37.337212470379,-172.514629908656));
#164337=CARTESIAN_POINT('Ctrl Pts',(41.9314834585311,37.3309632336908,-172.469870296763));
#164338=CARTESIAN_POINT('Ctrl Pts',(41.9321244954995,37.321570528007,-172.425063433264));
#164339=CARTESIAN_POINT('Ctrl Pts',(41.9329870509292,37.3089320536492,-172.380665523369));
#164340=CARTESIAN_POINT('Ctrl Pts',(41.9336634036616,37.2990218886089,-172.345851937327));
#164341=CARTESIAN_POINT('Ctrl Pts',(41.9344759477384,37.2871161986963,-172.311290758663));
#164342=CARTESIAN_POINT('Ctrl Pts',(41.93542780341,37.2731692648717,-172.277224099708));
#164343=CARTESIAN_POINT('Ctrl Pts',(41.9355206785256,37.2718084250625,-172.273900124256));
#164344=CARTESIAN_POINT('Ctrl Pts',(41.9356148798764,37.2704281527738,-172.270580868726));
#164345=CARTESIAN_POINT('Ctrl Pts',(41.9357104102735,37.269028406819,-172.267266567635));
#164346=CARTESIAN_POINT('Ctrl Pts',(41.9369407919429,37.2510004092627,-172.224580098873));
#164347=CARTESIAN_POINT('Ctrl Pts',(41.9383914477948,37.2297448746573,-172.182726614124));
#164348=CARTESIAN_POINT('Ctrl Pts',(41.9400563415622,37.2053502485713,-172.142169045052));
#164349=CARTESIAN_POINT('Ctrl Pts',(41.9416543121738,37.1819362047876,-172.103241754481));
#164350=CARTESIAN_POINT('Ctrl Pts',(41.9434495675826,37.1556314727481,-172.065509331767));
#164351=CARTESIAN_POINT('Ctrl Pts',(41.9454355793453,37.1265317095662,-172.029413465262));
#164352=CARTESIAN_POINT('Ctrl Pts',(41.946357166588,37.113028279718,-172.01266356946));
#164353=CARTESIAN_POINT('Ctrl Pts',(41.9473198149722,37.0989232071639,-171.996266629114));
#164354=CARTESIAN_POINT('Ctrl Pts',(41.9483227216382,37.0842282556921,-171.980270641983));
#164355=CARTESIAN_POINT('Ctrl Pts',(41.9486805968113,37.0789845391231,-171.974562666498));
#164356=CARTESIAN_POINT('Ctrl Pts',(41.9490626478473,37.073386589124,-171.968608245876));
#164357=CARTESIAN_POINT('Ctrl Pts',(41.9494436601674,37.0678037504325,-171.96281560598));
#164358=CARTESIAN_POINT('Ctrl Pts',(41.9498361130009,37.0620532779482,-171.95684903267));
#164359=CARTESIAN_POINT('Ctrl Pts',(41.9502274528427,37.0563189984669,-171.951054248039));
#164360=CARTESIAN_POINT('Ctrl Pts',(41.95058728953,37.0510460804859,-171.945838282772));
#164361=CARTESIAN_POINT('Ctrl Pts',(41.950657753626,37.050013524852,-171.944816879757));
#164362=CARTESIAN_POINT('Ctrl Pts',(41.9507270018928,37.0489987750081,-171.943817557184));
#164363=CARTESIAN_POINT('Ctrl Pts',(41.9507947956297,37.0480053275874,-171.942843213006));
#164364=CARTESIAN_POINT('Ctrl Pts',(41.9523067381499,37.025849366502,-171.921113294297));
#164365=CARTESIAN_POINT('Ctrl Pts',(41.953933863454,37.002008447526,-171.899758993298));
#164366=CARTESIAN_POINT('Ctrl Pts',(41.9556797558124,36.9764279216952,-171.879051282457));
#164367=CARTESIAN_POINT('Ctrl Pts',(41.9573985368362,36.9512446266509,-171.85866513421));
#164368=CARTESIAN_POINT('Ctrl Pts',(41.9592324446076,36.9243750459795,-171.838905512141));
#164369=CARTESIAN_POINT('Ctrl Pts',(41.9611826656455,36.8957997014518,-171.820067900506));
#164370=CARTESIAN_POINT('Ctrl Pts',(41.9630380210983,36.8686143618144,-171.80214661631));
#164371=CARTESIAN_POINT('Ctrl Pts',(41.964998836786,36.8398837806431,-171.785058882888));
#164372=CARTESIAN_POINT('Ctrl Pts',(41.9670643335467,36.8096193745015,-171.769091901481));
#164373=CARTESIAN_POINT('Ctrl Pts',(41.9690687839745,36.7802494413244,-171.753596828662));
#164374=CARTESIAN_POINT('Ctrl Pts',(41.9711718608506,36.7494343977296,-171.739157140834));
#164375=CARTESIAN_POINT('Ctrl Pts',(41.9733703800159,36.7172208991694,-171.726070467489));
#164376=CARTESIAN_POINT('Ctrl Pts',(41.9734065577268,36.7166908102542,-171.725855119862));
#164377=CARTESIAN_POINT('Ctrl Pts',(41.9734427611061,36.716160345237,-171.725640139903));
#164378=CARTESIAN_POINT('Ctrl Pts',(41.9734789901357,36.7156295043819,-171.725425528673));
#164379=CARTESIAN_POINT('Ctrl Pts',(41.973660741901,36.7129664117315,-171.724348879083));
#164380=CARTESIAN_POINT('Ctrl Pts',(41.9738919207081,36.709578749863,-171.722996951206));
#164381=CARTESIAN_POINT('Ctrl Pts',(41.9740840512554,36.7067631719946,-171.721889199711));
#164382=CARTESIAN_POINT('Ctrl Pts',(41.9742095140083,36.7049245775841,-171.721165829305));
#164383=CARTESIAN_POINT('Ctrl Pts',(41.9743182873496,36.7033304946806,-171.720545222455));
#164384=CARTESIAN_POINT('Ctrl Pts',(41.9743854868274,36.7023456178558,-171.720163007342));
#164385=CARTESIAN_POINT('Ctrl Pts',(41.9754591786029,36.686609570775,-171.714056096453));
#164386=CARTESIAN_POINT('Ctrl Pts',(41.9766482085272,36.6691851406408,-171.707738814436));
#164387=CARTESIAN_POINT('Ctrl Pts',(41.9779569888288,36.6500072100763,-171.701466818902));
#164388=CARTESIAN_POINT('Ctrl Pts',(41.9792886147671,36.6304945158891,-171.695085341485));
#164389=CARTESIAN_POINT('Ctrl Pts',(41.980744279009,36.6091655329514,-171.688750401779));
#164390=CARTESIAN_POINT('Ctrl Pts',(41.9823272482974,36.5859718986434,-171.682785652356));
#164391=CARTESIAN_POINT('Ctrl Pts',(41.9837542430735,36.5650635997658,-171.677408626831));
#164392=CARTESIAN_POINT('Ctrl Pts',(41.9852847155951,36.5426396506425,-171.672333011434));
#164393=CARTESIAN_POINT('Ctrl Pts',(41.9869193433264,36.518689754704,-171.667836203536));
#164394=CARTESIAN_POINT('Ctrl Pts',(41.9885007733798,36.4955192893508,-171.663485740725));
#164395=CARTESIAN_POINT('Ctrl Pts',(41.9901797252878,36.4709200605105,-171.659677091772));
#164396=CARTESIAN_POINT('Ctrl Pts',(41.9919546757492,36.4449140458738,-171.65669742379));
#164397=CARTESIAN_POINT('Ctrl Pts',(41.993647385108,36.4201130019462,-171.653855816664));
#164398=CARTESIAN_POINT('Ctrl Pts',(41.9954274262957,36.3940321765311,-171.651768285733));
#164399=CARTESIAN_POINT('Ctrl Pts',(41.9972910935929,36.3667255630958,-171.650715593431));
#164400=CARTESIAN_POINT('Ctrl Pts',(41.9981754755464,36.3537675226929,-171.650216050365));
#164401=CARTESIAN_POINT('Ctrl Pts',(41.9990786513334,36.340534002745,-171.64995));
#164402=CARTESIAN_POINT('Ctrl Pts',(42.,36.3270340686007,-171.64995));
#164403=CARTESIAN_POINT('',(41.3608268990399,36.416863989729,-171.64995));
#164404=CARTESIAN_POINT('Origin',(42.,28.91999998,-171.14995));
#164405=CARTESIAN_POINT('',(42.,28.41999998,-171.14995));
#164406=CARTESIAN_POINT('',(41.5,28.91999998,-171.14995));
#164407=CARTESIAN_POINT('Origin',(42.,28.91999998,-171.14995));
#164408=CARTESIAN_POINT('',(42.,28.91999998,-171.64995));
#164409=CARTESIAN_POINT('Origin',(42.,28.91999998,-171.14995));
#164410=CARTESIAN_POINT('Origin',(42.,28.91999998,-171.14995));
#164411=CARTESIAN_POINT('Ctrl Pts',(36.7529144574179,29.9771506489281,-64.6451542155005));
#164412=CARTESIAN_POINT('Ctrl Pts',(37.9544308619569,28.41999998,-65.5068366539031));
#164413=CARTESIAN_POINT('Ctrl Pts',(39.6993756576748,28.41999998,-66.758245524204));
#164414=CARTESIAN_POINT('Ctrl Pts',(35.4221830133223,29.9261764058054,-66.5837572422386));
#164415=CARTESIAN_POINT('Ctrl Pts',(36.6139893647491,28.4199999799959,-67.4471428080874));
#164416=CARTESIAN_POINT('Ctrl Pts',(38.3090750828473,28.41999998,-68.6968587227942));
#164417=CARTESIAN_POINT('Ctrl Pts',(34.0676680572731,29.8734031042169,-68.5045591474479));
#164418=CARTESIAN_POINT('Ctrl Pts',(35.2435893151229,28.41999998,-69.3754183593105));
#164419=CARTESIAN_POINT('Ctrl Pts',(36.8898270007225,28.4199999800001,-70.617650456175));
#164420=CARTESIAN_POINT('Ctrl Pts',(31.2955902801573,29.7642394885798,-72.2991303428252));
#164421=CARTESIAN_POINT('Ctrl Pts',(32.4319411374915,28.41999998,-73.1856180617498));
#164422=CARTESIAN_POINT('Ctrl Pts',(33.9748337796689,28.4199999800001,-74.4122216515051));
#164423=CARTESIAN_POINT('Ctrl Pts',(29.8799523105758,29.7079117212239,-74.1702869851635));
#164424=CARTESIAN_POINT('Ctrl Pts',(30.9935194672858,28.4199999800042,-75.0646492888564));
#164425=CARTESIAN_POINT('Ctrl Pts',(32.4811021033977,28.41999998,-76.2833884926716));
#164426=CARTESIAN_POINT('Ctrl Pts',(28.4305705461597,29.6502955521147,-75.9979827843214));
#164427=CARTESIAN_POINT('Ctrl Pts',(29.5115669185301,28.41999998,-76.9063064032585));
#164428=CARTESIAN_POINT('Ctrl Pts',(30.9453615210646,28.41999998,-78.1110740930249));
#164429=CARTESIAN_POINT('',(31.,28.41999998,-78.0460091084363));
#164430=CARTESIAN_POINT('',(37.,28.41999998,-70.4461836365688));
#164431=CARTESIAN_POINT('Ctrl Pts',(31.,28.41999998,-78.0460091084363));
#164432=CARTESIAN_POINT('Ctrl Pts',(31.6054626504307,28.4199999800001,-77.3245680023315));
#164433=CARTESIAN_POINT('Ctrl Pts',(32.203700232555,28.4199999800031,-76.5972335154402));
#164434=CARTESIAN_POINT('Ctrl Pts',(32.7954596657013,28.4199999800058,-75.8646586780434));
#164435=CARTESIAN_POINT('Ctrl Pts',(33.4345463105989,28.4199999800088,-75.0734946192315));
#164436=CARTESIAN_POINT('Ctrl Pts',(34.0660773010416,28.4199999800106,-74.2762178948239));
#164437=CARTESIAN_POINT('Ctrl Pts',(34.6909510193213,28.4199999800288,-73.4736062556159));
#164438=CARTESIAN_POINT('Ctrl Pts',(34.939102988304,28.4199999800361,-73.15487040104));
#164439=CARTESIAN_POINT('Ctrl Pts',(35.1862046047012,28.4199999800463,-72.8352927773716));
#164440=CARTESIAN_POINT('Ctrl Pts',(35.4323104279066,28.4199999800634,-72.5149207187905));
#164441=CARTESIAN_POINT('Ctrl Pts',(35.9594751118247,28.4199999801002,-71.8286759449022));
#164442=CARTESIAN_POINT('Ctrl Pts',(36.4818085017622,28.4199999801598,-71.1391285306312));
#164443=CARTESIAN_POINT('Ctrl Pts',(37.,28.4199999803545,-70.4461836365688));
#164444=CARTESIAN_POINT('Ctrl Pts',(31.,28.41999998,-78.0460091084363));
#164445=CARTESIAN_POINT('Ctrl Pts',(30.9953507488642,28.41999998,-77.9571322255713));
#164446=CARTESIAN_POINT('Ctrl Pts',(30.9904343156938,28.4210644426645,-77.8631868791632));
#164447=CARTESIAN_POINT('Ctrl Pts',(30.9852500369792,28.4236029528388,-77.7641731707001));
#164448=CARTESIAN_POINT('Ctrl Pts',(30.9804902860296,28.4259335906918,-77.6732674499945));
#164449=CARTESIAN_POINT('Ctrl Pts',(30.9755047623887,28.4295072224175,-77.5780895208821));
#164450=CARTESIAN_POINT('Ctrl Pts',(30.9702932674828,28.4346829171186,-77.4786459095534));
#164451=CARTESIAN_POINT('Ctrl Pts',(30.9647250948557,28.4402128393543,-77.372396320033));
#164452=CARTESIAN_POINT('Ctrl Pts',(30.9588989638651,28.4475712846398,-77.2612772547267));
#164453=CARTESIAN_POINT('Ctrl Pts',(30.9528170728823,28.4572452512149,-77.1453434183624));
#164454=CARTESIAN_POINT('Ctrl Pts',(30.9494041569204,28.4626738975081,-77.0802859482809));
#164455=CARTESIAN_POINT('Ctrl Pts',(30.9459106839778,28.4688326969503,-77.0137119621315));
#164456=CARTESIAN_POINT('Ctrl Pts',(30.942337363506,28.4758143402156,-76.9456372159907));
#164457=CARTESIAN_POINT('Ctrl Pts',(30.9405507032701,28.4793051618483,-76.9115998429203));
#164458=CARTESIAN_POINT('Ctrl Pts',(30.9387440785685,28.483001778153,-76.8771872300242));
#164459=CARTESIAN_POINT('Ctrl Pts',(30.9369176023688,28.4869161892589,-76.8424018044853));
#164460=CARTESIAN_POINT('Ctrl Pts',(30.9360043642689,28.4888733948118,-76.8250090917158));
#164461=CARTESIAN_POINT('Ctrl Pts',(30.9350861633931,28.4908850535414,-76.8075231775984));
#164462=CARTESIAN_POINT('Ctrl Pts',(30.9341630151144,28.4929526905484,-76.7899443889576));
#164463=CARTESIAN_POINT('Ctrl Pts',(30.9337014409751,28.493986509052,-76.7811549946371));
#164464=CARTESIAN_POINT('Ctrl Pts',(30.9332386299823,28.4950343224187,-76.772342381627));
#164465=CARTESIAN_POINT('Ctrl Pts',(30.9327745841645,28.4960963227561,-76.7635065927854));
#164466=CARTESIAN_POINT('Ctrl Pts',(30.9327340001398,28.4961892020499,-76.7627338417804));
#164467=CARTESIAN_POINT('Ctrl Pts',(30.9326934066704,28.4962821898565,-76.7619609135104));
#164468=CARTESIAN_POINT('Ctrl Pts',(30.9326528037575,28.4963752863047,-76.7611878080044));
#164469=CARTESIAN_POINT('Ctrl Pts',(30.9326153917186,28.4964610665529,-76.7604754587855));
#164470=CARTESIAN_POINT('Ctrl Pts',(30.9325775167222,28.4965479821107,-76.7597542967421));
#164471=CARTESIAN_POINT('Ctrl Pts',(30.932539159609,28.4966360826217,-76.759023957238));
#164472=CARTESIAN_POINT('Ctrl Pts',(30.9321431556995,28.4975456439494,-76.7514838356034));
#164473=CARTESIAN_POINT('Ctrl Pts',(30.9317015992017,28.4985703405887,-76.7430766793829));
#164474=CARTESIAN_POINT('Ctrl Pts',(30.9313787443117,28.4993250778052,-76.7369297425032));
#164475=CARTESIAN_POINT('Ctrl Pts',(30.9243094913047,28.5158508561152,-76.6023359873139));
#164476=CARTESIAN_POINT('Ctrl Pts',(30.9170546130173,28.5350544953412,-76.4677566994279));
#164477=CARTESIAN_POINT('Ctrl Pts',(30.9097979232358,28.5569559412352,-76.333337137572));
#164478=CARTESIAN_POINT('Ctrl Pts',(30.9054759833442,28.5700000061663,-76.2532795239633));
#164479=CARTESIAN_POINT('Ctrl Pts',(30.9011530346219,28.5840000959786,-76.1732784199905));
#164480=CARTESIAN_POINT('Ctrl Pts',(30.8968642854843,28.5989526153992,-76.0933627491102));
#164481=CARTESIAN_POINT('Ctrl Pts',(30.8939918578668,28.6089671973573,-76.0398385226402));
#164482=CARTESIAN_POINT('Ctrl Pts',(30.8911353205105,28.6194087482988,-75.9863527556447));
#164483=CARTESIAN_POINT('Ctrl Pts',(30.8883057354998,28.630274392489,-75.9329141284561));
#164484=CARTESIAN_POINT('Ctrl Pts',(30.8854761504891,28.6411400366793,-75.8794755012675));
#164485=CARTESIAN_POINT('Ctrl Pts',(30.8826735236571,28.6524297677877,-75.8260840188183));
#164486=CARTESIAN_POINT('Ctrl Pts',(30.879908391992,28.6641395635773,-75.7727479419548));
#164487=CARTESIAN_POINT('Ctrl Pts',(30.8771432603269,28.6758493593668,-75.7194118650914));
#164488=CARTESIAN_POINT('Ctrl Pts',(30.8744156231211,28.687979218675,-75.6661311939467));
#164489=CARTESIAN_POINT('Ctrl Pts',(30.8717358482434,28.700523890345,-75.6129139541153));
#164490=CARTESIAN_POINT('Ctrl Pts',(30.8703959608046,28.70679622618,-75.5863053341995));
#164491=CARTESIAN_POINT('Ctrl Pts',(30.8690680299892,28.7131722483955,-75.5597125647804));
#164492=CARTESIAN_POINT('Ctrl Pts',(30.8677533039181,28.7196512016491,-75.5331366064521));
#164493=CARTESIAN_POINT('Ctrl Pts',(30.8670959408825,28.7228906782759,-75.519848627288));
#164494=CARTESIAN_POINT('Ctrl Pts',(30.8664418784498,28.7261558866934,-75.5065648504057));
#164495=CARTESIAN_POINT('Ctrl Pts',(30.8657912703874,28.7294467262534,-75.4932853935933));
#164496=CARTESIAN_POINT('Ctrl Pts',(30.8654659663562,28.7310921460333,-75.4866456651871));
#164497=CARTESIAN_POINT('Ctrl Pts',(30.8651415258812,28.7327439735401,-75.4800070167672));
#164498=CARTESIAN_POINT('Ctrl Pts',(30.8648179680418,28.7344021958109,-75.4733694629099));
#164499=CARTESIAN_POINT('Ctrl Pts',(30.8645513322407,28.7357686946863,-75.4678996232866));
#164500=CARTESIAN_POINT('Ctrl Pts',(30.8643311330534,28.7369019898584,-75.4633764419093));
#164501=CARTESIAN_POINT('Ctrl Pts',(30.8640263227981,28.738394063327,-75.4574625920758));
#164502=CARTESIAN_POINT('Ctrl Pts',(30.8639612511876,28.7387125946821,-75.4562000894974));
#164503=CARTESIAN_POINT('Ctrl Pts',(30.8638923228878,28.7390475481913,-75.4548741968345));
#164504=CARTESIAN_POINT('Ctrl Pts',(30.8638182635132,28.7394047935033,-75.4534621817682));
#164505=CARTESIAN_POINT('Ctrl Pts',(30.858008398083,28.7674302420227,-75.3426913634633));
#164506=CARTESIAN_POINT('Ctrl Pts',(30.8523016334403,28.7968590694777,-75.234384024023));
#164507=CARTESIAN_POINT('Ctrl Pts',(30.8467210193799,28.8275021583711,-75.1285627604439));
#164508=CARTESIAN_POINT('Ctrl Pts',(30.8458318845886,28.832384387487,-75.1117027220868));
#164509=CARTESIAN_POINT('Ctrl Pts',(30.8449459413324,28.8372974903014,-75.0949056976548));
#164510=CARTESIAN_POINT('Ctrl Pts',(30.8440632708079,28.8422407586805,-75.0781716749711));
#164511=CARTESIAN_POINT('Ctrl Pts',(30.8392462368768,28.8692178592538,-74.9868484090043));
#164512=CARTESIAN_POINT('Ctrl Pts',(30.8345268703748,28.8970918830449,-74.8974052661039));
#164513=CARTESIAN_POINT('Ctrl Pts',(30.8299062263507,28.9257497007075,-74.8098577609863));
#164514=CARTESIAN_POINT('Ctrl Pts',(30.8239245086087,28.9628490694253,-74.6965219441801));
#164515=CARTESIAN_POINT('Ctrl Pts',(30.8181056496567,29.0012784332636,-74.586316278858));
#164516=CARTESIAN_POINT('Ctrl Pts',(30.8124473228795,29.0407768010215,-74.4793548016011));
#164517=CARTESIAN_POINT('Ctrl Pts',(30.8074704278574,29.07551838411,-74.385274684869));
#164518=CARTESIAN_POINT('Ctrl Pts',(30.8026176973093,29.1110871607376,-74.2937033724066));
#164519=CARTESIAN_POINT('Ctrl Pts',(30.7978867098362,29.1473126769893,-74.2046860321974));
#164520=CARTESIAN_POINT('Ctrl Pts',(30.7955318228038,29.1653442188076,-74.1603769357753));
#164521=CARTESIAN_POINT('Ctrl Pts',(30.7932062256382,29.1835361617856,-74.1166837486454));
#164522=CARTESIAN_POINT('Ctrl Pts',(30.7909090745396,29.2018763553954,-74.073600366696));
#164523=CARTESIAN_POINT('Ctrl Pts',(30.784538562423,29.2527378009856,-73.9541205436641));
#164524=CARTESIAN_POINT('Ctrl Pts',(30.7784374998368,29.3046763395262,-73.8394377704279));
#164525=CARTESIAN_POINT('Ctrl Pts',(30.7726131471017,29.3573237688943,-73.7294995389662));
#164526=CARTESIAN_POINT('Ctrl Pts',(30.7685560771346,29.3939963940342,-73.6529198540828));
#164527=CARTESIAN_POINT('Ctrl Pts',(30.7646331869072,29.4310117754566,-73.5786417333732));
#164528=CARTESIAN_POINT('Ctrl Pts',(30.7608459868074,29.4682320688712,-73.5066413939787));
#164529=CARTESIAN_POINT('Ctrl Pts',(30.7545181321184,29.5304217081824,-73.3863394101293));
#164530=CARTESIAN_POINT('Ctrl Pts',(30.7485612047523,29.5931874761478,-73.2724011812726));
#164531=CARTESIAN_POINT('Ctrl Pts',(30.7429002557377,29.6558866113949,-73.1647049054821));
#164532=CARTESIAN_POINT('Ctrl Pts',(30.7403095914777,29.6845801057894,-73.1154190186269));
#164533=CARTESIAN_POINT('Ctrl Pts',(30.7377811237821,29.7132588940408,-73.0674402016844));
#164534=CARTESIAN_POINT('Ctrl Pts',(30.7353086514483,29.741858118838,-73.0207560182717));
#164535=CARTESIAN_POINT('Ctrl Pts',(36.7055659821298,29.9753365605362,-64.7141088904942));
#164536=CARTESIAN_POINT('Ctrl Pts',(36.7103806723968,29.9138048831183,-64.8077062813706));
#164537=CARTESIAN_POINT('Ctrl Pts',(36.7154239961427,29.8523768893488,-64.9057516538932));
#164538=CARTESIAN_POINT('Ctrl Pts',(36.720700743777,29.7914623159788,-65.0083394071988));
#164539=CARTESIAN_POINT('Ctrl Pts',(36.72586695935,29.731823720507,-65.1087782542803));
#164540=CARTESIAN_POINT('Ctrl Pts',(36.7312569354101,29.6726779118629,-65.2135714316818));
#164541=CARTESIAN_POINT('Ctrl Pts',(36.7368742111855,29.6143645132415,-65.3227893322482));
#164542=CARTESIAN_POINT('Ctrl Pts',(36.7419663316423,29.5615027948742,-65.4217965250528));
#164543=CARTESIAN_POINT('Ctrl Pts',(36.7472447702708,29.5093303810589,-65.5244308868896));
#164544=CARTESIAN_POINT('Ctrl Pts',(36.7527092637514,29.4580763652213,-65.630689057867));
#164545=CARTESIAN_POINT('Ctrl Pts',(36.7579504941924,29.408916436862,-65.7326058342887));
#164546=CARTESIAN_POINT('Ctrl Pts',(36.7633629109637,29.360601408339,-65.8378568245558));
#164547=CARTESIAN_POINT('Ctrl Pts',(36.7689447807834,29.3132934632658,-65.9464101551646));
#164548=CARTESIAN_POINT('Ctrl Pts',(36.7701147474361,29.3033776608683,-65.9691630643058));
#164549=CARTESIAN_POINT('Ctrl Pts',(36.7712921542238,29.2935059409922,-65.9920609696869));
#164550=CARTESIAN_POINT('Ctrl Pts',(36.7724769784619,29.2836795313646,-66.015103448616));
#164551=CARTESIAN_POINT('Ctrl Pts',(36.7728652777524,29.2804591483213,-66.0226550988353));
#164552=CARTESIAN_POINT('Ctrl Pts',(36.7733444989399,29.2765012562496,-66.0319750492162));
#164553=CARTESIAN_POINT('Ctrl Pts',(36.773659114264,29.2739116254867,-66.0380915384093));
#164554=CARTESIAN_POINT('Ctrl Pts',(36.7736772492176,29.2737623548375,-66.0384441030783));
#164555=CARTESIAN_POINT('Ctrl Pts',(36.7736948370056,29.2736176171791,-66.0387860190953));
#164556=CARTESIAN_POINT('Ctrl Pts',(36.7737118286106,29.2734778116659,-66.0391163327188));
#164557=CARTESIAN_POINT('Ctrl Pts',(36.7739318943408,29.2716671291314,-66.0433943693668));
#164558=CARTESIAN_POINT('Ctrl Pts',(36.7741524800775,29.2698557797349,-66.0476826125677));
#164559=CARTESIAN_POINT('Ctrl Pts',(36.7743735861458,29.2680437946507,-66.0519810661563));
#164560=CARTESIAN_POINT('Ctrl Pts',(36.7830263907577,29.1971332447106,-66.2201975214263));
#164561=CARTESIAN_POINT('Ctrl Pts',(36.7924804704293,29.125303390636,-66.4041364543566));
#164562=CARTESIAN_POINT('Ctrl Pts',(36.8027632687972,29.0549146566565,-66.6041834017324));
#164563=CARTESIAN_POINT('Ctrl Pts',(36.8041298320501,29.0455601352671,-66.630769239299));
#164564=CARTESIAN_POINT('Ctrl Pts',(36.8055110279142,29.0362310691301,-66.6576394973203));
#164565=CARTESIAN_POINT('Ctrl Pts',(36.8069069162596,29.026932976743,-66.6847949968068));
#164566=CARTESIAN_POINT('Ctrl Pts',(36.8132112795187,28.98493925123,-66.8074395720736));
#164567=CARTESIAN_POINT('Ctrl Pts',(36.819813780274,28.9435824406279,-66.9358954277359));
#164568=CARTESIAN_POINT('Ctrl Pts',(36.8267147784773,28.9033780952543,-67.0701745666682));
#164569=CARTESIAN_POINT('Ctrl Pts',(36.8330290005385,28.8665922336971,-67.1930362565894));
#164570=CARTESIAN_POINT('Ctrl Pts',(36.839593079154,28.830771907803,-67.320772322381));
#164571=CARTESIAN_POINT('Ctrl Pts',(36.8464052868298,28.7962973206778,-67.4533537498322));
#164572=CARTESIAN_POINT('Ctrl Pts',(36.8465175503647,28.7957291878196,-67.4555386596919));
#164573=CARTESIAN_POINT('Ctrl Pts',(36.8467080818096,28.794766653035,-67.4592468559418));
#164574=CARTESIAN_POINT('Ctrl Pts',(36.8467422843428,28.7945940172133,-67.4599124240971));
#164575=CARTESIAN_POINT('Ctrl Pts',(36.8470175925643,28.7932044107582,-67.4652698162981));
#164576=CARTESIAN_POINT('Ctrl Pts',(36.8473091770429,28.7917368396073,-67.4709441072806));
#164577=CARTESIAN_POINT('Ctrl Pts',(36.8476170703693,28.7901927171027,-67.4769359322928));
#164578=CARTESIAN_POINT('Ctrl Pts',(36.8489153744216,28.7836815642673,-67.5022018605477));
#164579=CARTESIAN_POINT('Ctrl Pts',(36.8505025879075,28.7758079031284,-67.5330928362682));
#164580=CARTESIAN_POINT('Ctrl Pts',(36.8523800154265,28.7667137612429,-67.56963455819));
#164581=CARTESIAN_POINT('Ctrl Pts',(36.8542628670224,28.7575933454673,-67.6062818528199));
#164582=CARTESIAN_POINT('Ctrl Pts',(36.8564376124816,28.7472454102247,-67.6486125967218));
#164583=CARTESIAN_POINT('Ctrl Pts',(36.8589058566037,28.735865441364,-67.6966587851417));
#164584=CARTESIAN_POINT('Ctrl Pts',(36.8613895458258,28.7244142620601,-67.7450056238019));
#164585=CARTESIAN_POINT('Ctrl Pts',(36.8641704189541,28.7119181101614,-67.7991396646537));
#164586=CARTESIAN_POINT('Ctrl Pts',(36.867250395188,28.6986287032735,-67.8590995811083));
#164587=CARTESIAN_POINT('Ctrl Pts',(36.8688433532771,28.6917554462763,-67.8901107405077));
#164588=CARTESIAN_POINT('Ctrl Pts',(36.870516324212,28.6846708525742,-67.9226803849028));
#164589=CARTESIAN_POINT('Ctrl Pts',(36.8722696020682,28.6774151685508,-67.9568144872987));
#164590=CARTESIAN_POINT('Ctrl Pts',(36.8757493427449,28.6630147706079,-68.02456063726));
#164591=CARTESIAN_POINT('Ctrl Pts',(36.8795451946842,28.6479379180227,-68.0984658218493));
#164592=CARTESIAN_POINT('Ctrl Pts',(36.8836579616209,28.6325466976036,-68.178548971691));
#164593=CARTESIAN_POINT('Ctrl Pts',(36.8875264392335,28.618069681877,-68.2538753583012));
#164594=CARTESIAN_POINT('Ctrl Pts',(36.8916753646144,28.6033149445469,-68.3346688134664));
#164595=CARTESIAN_POINT('Ctrl Pts',(36.8961054173322,28.5886254921191,-68.4209460266021));
#164596=CARTESIAN_POINT('Ctrl Pts',(36.9008326532897,28.5729506204786,-68.5130110132352));
#164597=CARTESIAN_POINT('Ctrl Pts',(36.9058797909972,28.5573508491198,-68.6113160918283));
#164598=CARTESIAN_POINT('Ctrl Pts',(36.9112460479487,28.5422930359456,-68.7158512369764));
#164599=CARTESIAN_POINT('Ctrl Pts',(36.9139116353246,28.5348133499989,-68.7677771074236));
#164600=CARTESIAN_POINT('Ctrl Pts',(36.9166559335202,28.5274681519236,-68.8212396433565));
#164601=CARTESIAN_POINT('Ctrl Pts',(36.9194786897652,28.5203187159499,-68.8762346670231));
#164602=CARTESIAN_POINT('Ctrl Pts',(36.9201402732601,28.5186430668936,-68.889124125695));
#164603=CARTESIAN_POINT('Ctrl Pts',(36.9208061659157,28.5169781823619,-68.9020977537259));
#164604=CARTESIAN_POINT('Ctrl Pts',(36.9214763635607,28.5153248700445,-68.9151554800575));
#164605=CARTESIAN_POINT('Ctrl Pts',(36.9215588292865,28.5151214351304,-68.9167621924772));
#164606=CARTESIAN_POINT('Ctrl Pts',(36.9216413601916,28.5149181754348,-68.9183701781779));
#164607=CARTESIAN_POINT('Ctrl Pts',(36.9217239562676,28.5147150924694,-68.9199794370191));
#164608=CARTESIAN_POINT('Ctrl Pts',(36.921774586875,28.5145906045473,-68.9209658973506));
#164609=CARTESIAN_POINT('Ctrl Pts',(36.9218252419709,28.5144661830329,-68.9219528360739));
#164610=CARTESIAN_POINT('Ctrl Pts',(36.9218759215533,28.5143418282747,-68.9229402531568));
#164611=CARTESIAN_POINT('Ctrl Pts',(36.9219012452481,28.5142796903922,-68.9234336480827));
#164612=CARTESIAN_POINT('Ctrl Pts',(36.9219268191552,28.5142169699783,-68.9239319183434));
#164613=CARTESIAN_POINT('Ctrl Pts',(36.9219529250405,28.5141529789799,-68.9244405537663));
#164614=CARTESIAN_POINT('Ctrl Pts',(36.9221227453373,28.5137367138275,-68.9277492566648));
#164615=CARTESIAN_POINT('Ctrl Pts',(36.9223099561208,28.5132794300097,-68.9313968042199));
#164616=CARTESIAN_POINT('Ctrl Pts',(36.9224823318152,28.5128599042257,-68.9347553255715));
#164617=CARTESIAN_POINT('Ctrl Pts',(36.9225681829912,28.51265096072,-68.9364280266354));
#164618=CARTESIAN_POINT('Ctrl Pts',(36.9226503541162,28.5124513467347,-68.9380290303443));
#164619=CARTESIAN_POINT('Ctrl Pts',(36.9227248629765,28.5122706024224,-68.9394807467957));
#164620=CARTESIAN_POINT('Ctrl Pts',(36.9227703374086,28.5121602901063,-68.9403667619736));
#164621=CARTESIAN_POINT('Ctrl Pts',(36.9228129576836,28.5120570042161,-68.941197168337));
#164622=CARTESIAN_POINT('Ctrl Pts',(36.9228518183949,28.5119628977735,-68.9419543246753));
#164623=CARTESIAN_POINT('Ctrl Pts',(36.9228692062893,28.5119207906468,-68.9422931078331));
#164624=CARTESIAN_POINT('Ctrl Pts',(36.9228857465798,28.5118807504019,-68.9426153765461));
#164625=CARTESIAN_POINT('Ctrl Pts',(36.9229025306906,28.5118401334067,-68.9429423959565));
#164626=CARTESIAN_POINT('Ctrl Pts',(36.929440276446,28.4960190040928,-69.0703229754156));
#164627=CARTESIAN_POINT('Ctrl Pts',(36.9357346908991,28.4828904264568,-69.1929838435217));
#164628=CARTESIAN_POINT('Ctrl Pts',(36.9417839751952,28.4719638693738,-69.3108866229627));
#164629=CARTESIAN_POINT('Ctrl Pts',(36.9479506457248,28.4608252826823,-69.4310773033385));
#164630=CARTESIAN_POINT('Ctrl Pts',(36.9538625812405,28.4519750415136,-69.5463234505226));
#164631=CARTESIAN_POINT('Ctrl Pts',(36.9595182310889,28.4449475684845,-69.6565910160207));
#164632=CARTESIAN_POINT('Ctrl Pts',(36.9652344171721,28.4378448756717,-69.7680388496438));
#164633=CARTESIAN_POINT('Ctrl Pts',(36.9706888032379,28.4326042890806,-69.8744009702031));
#164634=CARTESIAN_POINT('Ctrl Pts',(36.9758801287652,28.4287986088424,-69.975648698779));
#164635=CARTESIAN_POINT('Ctrl Pts',(36.9811558032791,28.4249310936702,-70.0785415068729));
#164636=CARTESIAN_POINT('Ctrl Pts',(36.9861598004273,28.4225455482904,-70.1761523856826));
#164637=CARTESIAN_POINT('Ctrl Pts',(36.9908911285026,28.4212473708485,-70.2684576807743));
#164638=CARTESIAN_POINT('Ctrl Pts',(36.9940489481048,28.4203809312129,-70.3300647952238));
#164639=CARTESIAN_POINT('Ctrl Pts',(36.9970853114138,28.41999998,-70.3893086183834));
#164640=CARTESIAN_POINT('Ctrl Pts',(37.,28.41999998,-70.4461836365688));
#164641=CARTESIAN_POINT('Ctrl Pts',(28.2935777143944,29.6448500754942,-76.1704746152117));
#164642=CARTESIAN_POINT('Ctrl Pts',(29.3719438459593,28.4199999800001,-77.079545860612));
#164643=CARTESIAN_POINT('Ctrl Pts',(30.800186642726,28.4199999800001,-78.2835659239152));
#164644=CARTESIAN_POINT('Ctrl Pts',(27.0582328538907,29.5957479131388,-77.7235993982802));
#164645=CARTESIAN_POINT('Ctrl Pts',(28.1162846817441,28.4199999800035,-78.6350614606686));
#164646=CARTESIAN_POINT('Ctrl Pts',(29.4908802242649,28.4199999800001,-79.8367023859018));
#164647=CARTESIAN_POINT('Ctrl Pts',(25.7920491676122,29.54547115812,-79.2528873037006));
#164648=CARTESIAN_POINT('Ctrl Pts',(26.8231903788109,28.41999998,-80.171186708314));
#164649=CARTESIAN_POINT('Ctrl Pts',(28.1443442258615,28.41999998,-81.3659786124399));
#164650=CARTESIAN_POINT('Ctrl Pts',(23.1839068120671,29.4434760286189,-82.2366052581402));
#164651=CARTESIAN_POINT('Ctrl Pts',(24.151734271497,28.41999998,-83.168456079353));
#164652=CARTESIAN_POINT('Ctrl Pts',(25.359343066053,28.41999998,-84.349696566808));
#164653=CARTESIAN_POINT('Ctrl Pts',(21.8495491428221,29.3920399293098,-83.6826429630518));
#164654=CARTESIAN_POINT('Ctrl Pts',(22.7816855628193,28.4199999799965,-84.621550748069));
#164655=CARTESIAN_POINT('Ctrl Pts',(23.928985790681,28.41999998,-85.7957524739721));
#164656=CARTESIAN_POINT('Ctrl Pts',(20.4734286051771,29.3409536236015,-85.0667234623348));
#164657=CARTESIAN_POINT('Ctrl Pts',(21.3602588054756,28.41999998,-86.0160960137185));
#164658=CARTESIAN_POINT('Ctrl Pts',(22.4473146057945,28.41999998,-87.1798147710383));
#164659=CARTESIAN_POINT('',(22.5,28.41999998,-87.1305533863517));
#164660=CARTESIAN_POINT('',(28.5,28.41999998,-80.9397703408579));
#164661=CARTESIAN_POINT('Ctrl Pts',(22.5,28.41999998,-87.1305533863517));
#164662=CARTESIAN_POINT('Ctrl Pts',(22.9996306884473,28.4199999800004,-86.6629501694533));
#164663=CARTESIAN_POINT('Ctrl Pts',(23.492564146587,28.4199999800118,-86.1891300413686));
#164664=CARTESIAN_POINT('Ctrl Pts',(23.9796464830061,28.4199999800316,-85.7094996089096));
#164665=CARTESIAN_POINT('Ctrl Pts',(24.4984981224754,28.4199999800526,-85.1985859140089));
#164666=CARTESIAN_POINT('Ctrl Pts',(25.0107103809196,28.4199999800828,-84.6810791338132));
#164667=CARTESIAN_POINT('Ctrl Pts',(25.5172665601395,28.4199999801285,-84.1574232895664));
#164668=CARTESIAN_POINT('Ctrl Pts',(25.9324040800864,28.419999980166,-83.7282720968575));
#164669=CARTESIAN_POINT('Ctrl Pts',(26.3437419377213,28.4199999802138,-83.294989959686));
#164670=CARTESIAN_POINT('Ctrl Pts',(26.7518048403013,28.4199999802818,-82.85780136844));
#164671=CARTESIAN_POINT('Ctrl Pts',(27.3023421757742,28.4199999803735,-82.2679691621747));
#164672=CARTESIAN_POINT('Ctrl Pts',(27.8456527104564,28.4199999804996,-81.6723376117131));
#164673=CARTESIAN_POINT('Ctrl Pts',(28.38269634666,28.4199999807123,-81.0712589143752));
#164674=CARTESIAN_POINT('Ctrl Pts',(28.4218307391359,28.4199999807278,-81.027458284287));
#164675=CARTESIAN_POINT('Ctrl Pts',(28.4609318358966,28.4199999807438,-80.9836287163286));
#164676=CARTESIAN_POINT('Ctrl Pts',(28.5,28.4199999807603,-80.9397703408579));
#164677=CARTESIAN_POINT('',(22.2890532034791,29.4093902975657,-83.1809305852948));
#164678=CARTESIAN_POINT('Ctrl Pts',(22.5,28.41999998,-87.1305533863517));
#164679=CARTESIAN_POINT('Ctrl Pts',(22.4951047682498,28.41999998,-87.0370152632459));
#164680=CARTESIAN_POINT('Ctrl Pts',(22.489969023803,28.4214973912862,-86.9390314876809));
#164681=CARTESIAN_POINT('Ctrl Pts',(22.4845922316981,28.4249676368345,-86.8366329910864));
#164682=CARTESIAN_POINT('Ctrl Pts',(22.4803327151963,28.4277167794254,-86.7555124869833));
#164683=CARTESIAN_POINT('Ctrl Pts',(22.4759218121537,28.4317051628399,-86.6716193602151));
#164684=CARTESIAN_POINT('Ctrl Pts',(22.471359830805,28.4371915964678,-86.5849805610453));
#164685=CARTESIAN_POINT('Ctrl Pts',(22.4673677205461,28.441992678782,-86.5091644599796));
#164686=CARTESIAN_POINT('Ctrl Pts',(22.4632600604673,28.4479411595211,-86.4312485168285));
#164687=CARTESIAN_POINT('Ctrl Pts',(22.4590378193768,28.4552211396799,-86.3512653363311));
#164688=CARTESIAN_POINT('Ctrl Pts',(22.4569266988316,28.4588611297592,-86.3112737460824));
#164689=CARTESIAN_POINT('Ctrl Pts',(22.4547869543608,28.4628341254629,-86.2707657503527));
#164690=CARTESIAN_POINT('Ctrl Pts',(22.4526187803266,28.4671639280558,-86.2297467972352));
#164691=CARTESIAN_POINT('Ctrl Pts',(22.4515346933096,28.4693288293523,-86.2092373206764));
#164692=CARTESIAN_POINT('Ctrl Pts',(22.4504435002051,28.4715829389777,-86.1886001291912));
#164693=CARTESIAN_POINT('Ctrl Pts',(22.4493452313998,28.4739292712921,-86.1678360170587));
#164694=CARTESIAN_POINT('Ctrl Pts',(22.4487960969971,28.4751024374493,-86.1574539609925));
#164695=CARTESIAN_POINT('Ctrl Pts',(22.4482451937128,28.4762986596964,-86.147040175564));
#164696=CARTESIAN_POINT('Ctrl Pts',(22.4476925255692,28.4775183173404,-86.1365947641351));
#164697=CARTESIAN_POINT('Ctrl Pts',(22.4474161914973,28.4781281461624,-86.1313720584206));
#164698=CARTESIAN_POINT('Ctrl Pts',(22.4471394162153,28.4787438338542,-86.1261414462916));
#164699=CARTESIAN_POINT('Ctrl Pts',(22.4468622002481,28.4793654279613,-86.1209029410792));
#164700=CARTESIAN_POINT('Ctrl Pts',(22.4467928962564,28.479520826488,-86.1195933147761));
#164701=CARTESIAN_POINT('Ctrl Pts',(22.4467235647218,28.4796765941662,-86.1182831951567));
#164702=CARTESIAN_POINT('Ctrl Pts',(22.446654205653,28.4798327317393,-86.1169725824328));
#164703=CARTESIAN_POINT('Ctrl Pts',(22.4466281960021,28.4798912833292,-86.1164811026613));
#164704=CARTESIAN_POINT('Ctrl Pts',(22.4466021824793,28.4799498869356,-86.115989553547));
#164705=CARTESIAN_POINT('Ctrl Pts',(22.4465761650848,28.4800085425977,-86.115497935101));
#164706=CARTESIAN_POINT('Ctrl Pts',(22.446559066732,28.4800470904703,-86.1151748487266));
#164707=CARTESIAN_POINT('Ctrl Pts',(22.4465419667071,28.4800856608257,-86.114851732408));
#164708=CARTESIAN_POINT('Ctrl Pts',(22.4465248650102,28.4801242536749,-86.1145285861484));
#164709=CARTESIAN_POINT('Ctrl Pts',(22.4465111475424,28.4801552094431,-86.1142693868174));
#164710=CARTESIAN_POINT('Ctrl Pts',(22.4464975359983,28.4801859375989,-86.1140121899836));
#164711=CARTESIAN_POINT('Ctrl Pts',(22.4464829918517,28.4802187848952,-86.1137373723805));
#164712=CARTESIAN_POINT('Ctrl Pts',(22.446322533286,28.4805811732965,-86.1107054421114));
#164713=CARTESIAN_POINT('Ctrl Pts',(22.4460801860419,28.4811319103387,-86.1061264923159));
#164714=CARTESIAN_POINT('Ctrl Pts',(22.4460292308326,28.4812479771557,-86.1051637598205));
#164715=CARTESIAN_POINT('Ctrl Pts',(22.4449780310017,28.4836424216106,-86.0853027043907));
#164716=CARTESIAN_POINT('Ctrl Pts',(22.4436696588496,28.4866890992066,-86.0605885877759));
#164717=CARTESIAN_POINT('Ctrl Pts',(22.442103617021,28.490518899134,-86.0310232998984));
#164718=CARTESIAN_POINT('Ctrl Pts',(22.44054125975,28.4943396883708,-86.0015275727468));
#164719=CARTESIAN_POINT('Ctrl Pts',(22.4387224427457,28.4989399023362,-85.9672034699557));
#164720=CARTESIAN_POINT('Ctrl Pts',(22.4366469102226,28.5045005891629,-85.928061544957));
#164721=CARTESIAN_POINT('Ctrl Pts',(22.4345758991035,28.5100491624183,-85.889004887933));
#164722=CARTESIAN_POINT('Ctrl Pts',(22.4322492882742,28.5165540132362,-85.8451513709574));
#164723=CARTESIAN_POINT('Ctrl Pts',(22.4296670800832,28.5242461697488,-85.7965202067969));
#164724=CARTESIAN_POINT('Ctrl Pts',(22.4270880170419,28.5319289571546,-85.7479482757746));
#164725=CARTESIAN_POINT('Ctrl Pts',(22.4242538570598,28.540796561228,-85.6946080669459));
#164726=CARTESIAN_POINT('Ctrl Pts',(22.4211653956423,28.5511287615564,-85.6365371663577));
#164727=CARTESIAN_POINT('Ctrl Pts',(22.4181315437853,28.5612782699737,-85.5794930638834));
#164728=CARTESIAN_POINT('Ctrl Pts',(22.4148523490072,28.5728410679315,-85.517884975594));
#164729=CARTESIAN_POINT('Ctrl Pts',(22.4113291382384,28.5861288281457,-85.4517621039892));
#164730=CARTESIAN_POINT('Ctrl Pts',(22.4077443244978,28.5996489234573,-85.3844830808907));
#164731=CARTESIAN_POINT('Ctrl Pts',(22.4039069812495,28.6149545647562,-85.3125318340768));
#164732=CARTESIAN_POINT('Ctrl Pts',(22.3998201352734,28.6324173313141,-85.2359930321443));
#164733=CARTESIAN_POINT('Ctrl Pts',(22.3979169863125,28.6405493348751,-85.2003506951866));
#164734=CARTESIAN_POINT('Ctrl Pts',(22.3959597547803,28.6491497204908,-85.1637139891818));
#164735=CARTESIAN_POINT('Ctrl Pts',(22.393948882839,28.6582589314929,-85.1260941361953));
#164736=CARTESIAN_POINT('Ctrl Pts',(22.3935500158385,28.6600657912909,-85.1186320409653));
#164737=CARTESIAN_POINT('Ctrl Pts',(22.3930644920505,28.6622797595882,-85.1095498956867));
#164738=CARTESIAN_POINT('Ctrl Pts',(22.392720765649,28.6638553527948,-85.1031208045394));
#164739=CARTESIAN_POINT('Ctrl Pts',(22.3926828656075,28.6640290812243,-85.1024119185758));
#164740=CARTESIAN_POINT('Ctrl Pts',(22.3926466889428,28.6641950072837,-85.1017352740096));
#164741=CARTESIAN_POINT('Ctrl Pts',(22.3926125418634,28.6643516992126,-85.101096595959));
#164742=CARTESIAN_POINT('Ctrl Pts',(22.3877821780164,28.6865169631871,-85.0107507327198));
#164743=CARTESIAN_POINT('Ctrl Pts',(22.3831370999249,28.7092875749723,-84.9245013585229));
#164744=CARTESIAN_POINT('Ctrl Pts',(22.3787041414205,28.7322906723717,-84.8423472438193));
#164745=CARTESIAN_POINT('Ctrl Pts',(22.3740953037289,28.7562064257484,-84.7569336357291));
#164746=CARTESIAN_POINT('Ctrl Pts',(22.3697157117241,28.7803731382638,-84.6759461611083));
#164747=CARTESIAN_POINT('Ctrl Pts',(22.365590291958,28.8044073200015,-84.5993406230004));
#164748=CARTESIAN_POINT('Ctrl Pts',(22.3646452728677,28.8099128835203,-84.5817924218366));
#164749=CARTESIAN_POINT('Ctrl Pts',(22.3637135718636,28.8154116467859,-84.5644740070615));
#164750=CARTESIAN_POINT('Ctrl Pts',(22.3627954557692,28.820899277231,-84.5473845938951));
#164751=CARTESIAN_POINT('Ctrl Pts',(22.3586289219162,28.8458028794692,-84.4698305471638));
#164752=CARTESIAN_POINT('Ctrl Pts',(22.3547334364831,28.8704744451308,-84.397000610347));
#164753=CARTESIAN_POINT('Ctrl Pts',(22.3510910329502,28.8945421918395,-84.3288273774177));
#164754=CARTESIAN_POINT('Ctrl Pts',(22.3508951884565,28.8958362647298,-84.3251618438866));
#164755=CARTESIAN_POINT('Ctrl Pts',(22.3507000755983,28.8971286029019,-84.3215097668994));
#164756=CARTESIAN_POINT('Ctrl Pts',(22.3505056915785,28.8984191522915,-84.3178711340653));
#164757=CARTESIAN_POINT('Ctrl Pts',(22.3486008790756,28.9110655345192,-84.2822153567841));
#164758=CARTESIAN_POINT('Ctrl Pts',(22.3467655974202,28.9235399337527,-84.2478508654111));
#164759=CARTESIAN_POINT('Ctrl Pts',(22.3449949120567,28.9357938806202,-84.2147662769381));
#164760=CARTESIAN_POINT('Ctrl Pts',(22.344109569375,28.941920854054,-84.1982239827016));
#164761=CARTESIAN_POINT('Ctrl Pts',(22.3432403894245,28.9479927535013,-84.1820016780921));
#164762=CARTESIAN_POINT('Ctrl Pts',(22.3423866078272,28.9540039023431,-84.1660978565589));
#164763=CARTESIAN_POINT('Ctrl Pts',(22.3419597170285,28.957009476764,-84.1581459457924));
#164764=CARTESIAN_POINT('Ctrl Pts',(22.3415366767081,28.9599998661409,-84.1502736567013));
#164765=CARTESIAN_POINT('Ctrl Pts',(22.3411173918452,28.9629743794316,-84.14248080323));
#164766=CARTESIAN_POINT('Ctrl Pts',(22.3409077494137,28.964461636077,-84.1385843764944));
#164767=CARTESIAN_POINT('Ctrl Pts',(22.3406990459045,28.9659449238627,-84.1347078087226));
#164768=CARTESIAN_POINT('Ctrl Pts',(22.3404912690254,28.9674241578559,-84.1308510764665));
#164769=CARTESIAN_POINT('Ctrl Pts',(22.3402834921463,28.968903391849,-84.1269943442105));
#164770=CARTESIAN_POINT('Ctrl Pts',(22.3401740841416,28.9696825228617,-84.124963567216));
#164771=CARTESIAN_POINT('Ctrl Pts',(22.3398707060041,28.9718496143136,-84.1193403628843));
#164772=CARTESIAN_POINT('Ctrl Pts',(22.3341418138434,29.0127722507775,-84.0131536366896));
#164773=CARTESIAN_POINT('Ctrl Pts',(22.3286290027088,29.0547685352277,-83.9110986363527));
#164774=CARTESIAN_POINT('Ctrl Pts',(22.3233329971592,29.09743018428,-83.8131653118839));
#164775=CARTESIAN_POINT('Ctrl Pts',(22.3178665094664,29.1414651418176,-83.7120794448276));
#164776=CARTESIAN_POINT('Ctrl Pts',(22.3126309837291,29.186208771893,-83.6153844056887));
#164777=CARTESIAN_POINT('Ctrl Pts',(22.3076242361681,29.2312362706003,-83.5230179678608));
#164778=CARTESIAN_POINT('Ctrl Pts',(22.302380749841,29.2783928469877,-83.426284080656));
#164779=CARTESIAN_POINT('Ctrl Pts',(22.2973881622895,29.3258604388178,-83.334297338755));
#164780=CARTESIAN_POINT('Ctrl Pts',(22.2926411499906,29.3731816212461,-83.2469383796063));
#164781=CARTESIAN_POINT('Ctrl Pts',(22.2914299907881,29.3852552123732,-83.2246494954339));
#164782=CARTESIAN_POINT('Ctrl Pts',(22.2902348052996,29.3973194356256,-83.2026616552453));
#164783=CARTESIAN_POINT('Ctrl Pts',(22.2890554809091,29.4093670318967,-83.1809724699472));
#164784=CARTESIAN_POINT('',(28.2496026321977,29.6431021634044,-76.2257352260018));
#164785=CARTESIAN_POINT('Ctrl Pts',(28.2496026843433,29.6431021904052,-76.2257353081032));
#164786=CARTESIAN_POINT('Ctrl Pts',(27.8439324295553,29.6269781482949,-76.7352715965501));
#164787=CARTESIAN_POINT('Ctrl Pts',(27.4405910184951,29.6109534525765,-77.2351086235097));
#164788=CARTESIAN_POINT('Ctrl Pts',(27.0393215418638,29.5950412497677,-77.7253786106869));
#164789=CARTESIAN_POINT('Ctrl Pts',(26.6071317885992,29.577902914045,-78.2534269102236));
#164790=CARTESIAN_POINT('Ctrl Pts',(26.1773458282904,29.5608950892855,-78.7703771082137));
#164791=CARTESIAN_POINT('Ctrl Pts',(25.7496553125592,29.544029978792,-79.2764572215566));
#164792=CARTESIAN_POINT('Ctrl Pts',(25.3271476948443,29.5273692453994,-79.7764044852826));
#164793=CARTESIAN_POINT('Ctrl Pts',(24.906685430099,29.5108477454557,-80.2657444716429));
#164794=CARTESIAN_POINT('Ctrl Pts',(24.4879779898396,29.4944735933695,-80.7447462809204));
#164795=CARTESIAN_POINT('Ctrl Pts',(24.0419205535757,29.4770298806519,-81.2550365181317));
#164796=CARTESIAN_POINT('Ctrl Pts',(23.5987412348824,29.4597865708662,-81.7526119366807));
#164797=CARTESIAN_POINT('Ctrl Pts',(23.1578556033775,29.4427591879028,-82.2378302632723));
#164798=CARTESIAN_POINT('Ctrl Pts',(22.8673437674819,29.4315393704905,-82.5575541480974));
#164799=CARTESIAN_POINT('Ctrl Pts',(22.5778286446949,29.4204131853293,-82.8719138375261));
#164800=CARTESIAN_POINT('Ctrl Pts',(22.2891503923498,29.4093838642276,-83.1810211213626));
#164801=CARTESIAN_POINT('Ctrl Pts',(28.2496025526968,29.6431021742755,-76.2257352367271));
#164802=CARTESIAN_POINT('Ctrl Pts',(28.255183736006,29.5810914147569,-76.3299584484354));
#164803=CARTESIAN_POINT('Ctrl Pts',(28.2610740674642,29.5190700705727,-76.4400011095444));
#164804=CARTESIAN_POINT('Ctrl Pts',(28.2672804894903,29.4576860819767,-76.5560107358913));
#164805=CARTESIAN_POINT('Ctrl Pts',(28.2704089728608,29.4267441339864,-76.6144879366551));
#164806=CARTESIAN_POINT('Ctrl Pts',(28.2736177556735,29.3959634873014,-76.6744810429466));
#164807=CARTESIAN_POINT('Ctrl Pts',(28.2769076118698,29.3654221838543,-76.7360071763375));
#164808=CARTESIAN_POINT('Ctrl Pts',(28.2821860203022,29.3164202019934,-76.8347227559663));
#164809=CARTESIAN_POINT('Ctrl Pts',(28.2876727741999,29.2680404155082,-76.9373783773371));
#164810=CARTESIAN_POINT('Ctrl Pts',(28.2933680075836,29.2205986057973,-77.0439895897435));
#164811=CARTESIAN_POINT('Ctrl Pts',(28.2979333863715,29.1825685871616,-77.1294506296846));
#164812=CARTESIAN_POINT('Ctrl Pts',(28.3026326762123,29.1451412031537,-77.2174524831978));
#164813=CARTESIAN_POINT('Ctrl Pts',(28.3074648801551,29.108462887641,-77.3079840345561));
#164814=CARTESIAN_POINT('Ctrl Pts',(28.3078152123237,29.1058037296322,-77.3145475229955));
#164815=CARTESIAN_POINT('Ctrl Pts',(28.3082600170683,29.1024416508876,-77.3228812792815));
#164816=CARTESIAN_POINT('Ctrl Pts',(28.3085180026056,29.1004972415241,-77.3277143555029));
#164817=CARTESIAN_POINT('Ctrl Pts',(28.3086435314212,29.0995511442857,-77.33006600025));
#164818=CARTESIAN_POINT('Ctrl Pts',(28.3087692964991,29.0986044393851,-77.3324221074881));
#164819=CARTESIAN_POINT('Ctrl Pts',(28.3088952979202,29.0976571367595,-77.3347826788554));
#164820=CARTESIAN_POINT('Ctrl Pts',(28.3142335624862,29.0575230494133,-77.4347923007826));
#164821=CARTESIAN_POINT('Ctrl Pts',(28.3199963653331,29.0163232038439,-77.5428200375934));
#164822=CARTESIAN_POINT('Ctrl Pts',(28.3261919085518,28.9749251754602,-77.6590324417008));
#164823=CARTESIAN_POINT('Ctrl Pts',(28.3294675063405,28.9530379437128,-77.7204742040247));
#164824=CARTESIAN_POINT('Ctrl Pts',(28.3328640791694,28.931096280647,-77.7842041423692));
#164825=CARTESIAN_POINT('Ctrl Pts',(28.3363829000878,28.9092337070165,-77.8502488180608));
#164826=CARTESIAN_POINT('Ctrl Pts',(28.3420752382563,28.8738669846907,-77.9570881932308));
#164827=CARTESIAN_POINT('Ctrl Pts',(28.3480866891023,28.8387109592594,-78.0699758528063));
#164828=CARTESIAN_POINT('Ctrl Pts',(28.3544180938211,28.804361897349,-78.1889520040999));
#164829=CARTESIAN_POINT('Ctrl Pts',(28.3593985277568,28.7773421061341,-78.282541481911));
#164830=CARTESIAN_POINT('Ctrl Pts',(28.3645768739889,28.7508225548804,-78.3798971860222));
#164831=CARTESIAN_POINT('Ctrl Pts',(28.3699520794374,28.7250966301013,-78.4810129983013));
#164832=CARTESIAN_POINT('Ctrl Pts',(28.3701458646069,28.7241691673761,-78.4846583928838));
#164833=CARTESIAN_POINT('Ctrl Pts',(28.3704257902458,28.7228336879588,-78.4899243609925));
#164834=CARTESIAN_POINT('Ctrl Pts',(28.3705342074466,28.722317348061,-78.4919638340097));
#164835=CARTESIAN_POINT('Ctrl Pts',(28.3706986208292,28.7215343248089,-78.4950566703395));
#164836=CARTESIAN_POINT('Ctrl Pts',(28.3708651149875,28.7207430073931,-78.4981887192797));
#164837=CARTESIAN_POINT('Ctrl Pts',(28.3710336910261,28.7199435124741,-78.5013600047023));
#164838=CARTESIAN_POINT('Ctrl Pts',(28.373006883928,28.7105853752683,-78.538480095648));
#164839=CARTESIAN_POINT('Ctrl Pts',(28.3752653039959,28.7001058776199,-78.5809756952539));
#164840=CARTESIAN_POINT('Ctrl Pts',(28.3778104891178,28.688725450316,-78.6288819284805));
#164841=CARTESIAN_POINT('Ctrl Pts',(28.3796362123637,28.6805619927754,-78.663246235763));
#164842=CARTESIAN_POINT('Ctrl Pts',(28.3816094990746,28.6719360567712,-78.7003947879149));
#164843=CARTESIAN_POINT('Ctrl Pts',(28.383730846252,28.6629455066605,-78.7403399456306));
#164844=CARTESIAN_POINT('Ctrl Pts',(28.3869252065252,28.6494073850304,-78.8004900362284));
#164845=CARTESIAN_POINT('Ctrl Pts',(28.3904835574881,28.6349272591564,-78.867509044862));
#164846=CARTESIAN_POINT('Ctrl Pts',(28.3943564253042,28.620103437781,-78.9404874769925));
#164847=CARTESIAN_POINT('Ctrl Pts',(28.3969472734419,28.6101866856927,-78.9893081556088));
#164848=CARTESIAN_POINT('Ctrl Pts',(28.3996788336818,28.6001162870024,-79.040795056823));
#164849=CARTESIAN_POINT('Ctrl Pts',(28.4025356366335,28.5900659246857,-79.0946635154937));
#164850=CARTESIAN_POINT('Ctrl Pts',(28.4063205663074,28.5767503704769,-79.1660329207915));
#164851=CARTESIAN_POINT('Ctrl Pts',(28.4098729825914,28.5650881944288,-79.2328695271597));
#164852=CARTESIAN_POINT('Ctrl Pts',(28.4131801735685,28.5547889850124,-79.2951206573735));
#164853=CARTESIAN_POINT('Ctrl Pts',(28.416100601828,28.545694226821,-79.3500917676345));
#164854=CARTESIAN_POINT('Ctrl Pts',(28.4188298586093,28.537662889555,-79.4014880882629));
#164855=CARTESIAN_POINT('Ctrl Pts',(28.4213603911671,28.5305215651011,-79.4492940109026));
#164856=CARTESIAN_POINT('Ctrl Pts',(28.4240584874455,28.522907365129,-79.5002654878583));
#164857=CARTESIAN_POINT('Ctrl Pts',(28.4265337063652,28.5163045723416,-79.5471525710561));
#164858=CARTESIAN_POINT('Ctrl Pts',(28.42879051022,28.5105339014271,-79.5899402886357));
#164859=CARTESIAN_POINT('Ctrl Pts',(28.4299189121475,28.5076485659698,-79.6113341474255));
#164860=CARTESIAN_POINT('Ctrl Pts',(28.4309928115677,28.5049717606348,-79.6317033009445));
#164861=CARTESIAN_POINT('Ctrl Pts',(28.4320132245346,28.5024840629928,-79.6510465723521));
#164862=CARTESIAN_POINT('Ctrl Pts',(28.4325234310181,28.5012402141718,-79.6607182080559));
#164863=CARTESIAN_POINT('Ctrl Pts',(28.4330202701749,28.5000436735233,-79.6701333769929));
#164864=CARTESIAN_POINT('Ctrl Pts',(28.4335038854641,28.4988921989618,-79.6792919688879));
#164865=CARTESIAN_POINT('Ctrl Pts',(28.4337456931087,28.4983164616811,-79.6838712648354));
#164866=CARTESIAN_POINT('Ctrl Pts',(28.4339841950586,28.4977519928503,-79.688386416761));
#164867=CARTESIAN_POINT('Ctrl Pts',(28.4342194100622,28.4971985238549,-79.69283741224));
#164868=CARTESIAN_POINT('Ctrl Pts',(28.434337017564,28.4969217893572,-79.6950629099794));
#164869=CARTESIAN_POINT('Ctrl Pts',(28.4344538033452,28.4966478049383,-79.6972723686213));
#164870=CARTESIAN_POINT('Ctrl Pts',(28.4345697697949,28.4963765377427,-79.6994657867326));
#164871=CARTESIAN_POINT('Ctrl Pts',(28.4346857362446,28.4961052705471,-79.7016592048439));
#164872=CARTESIAN_POINT('Ctrl Pts',(28.4347179301366,28.496029621214,-79.7022684074304));
#164873=CARTESIAN_POINT('Ctrl Pts',(28.4349152167509,28.495570855037,-79.7059979180573));
#164874=CARTESIAN_POINT('Ctrl Pts',(28.4350220546971,28.4953224163059,-79.7080175850115));
#164875=CARTESIAN_POINT('Ctrl Pts',(28.4351288270614,28.4950747520133,-79.7100360387155));
#164876=CARTESIAN_POINT('Ctrl Pts',(28.4352355337918,28.4948278599047,-79.7120532781116));
#164877=CARTESIAN_POINT('Ctrl Pts',(28.4424961980171,28.4780285381237,-79.8493126418011));
#164878=CARTESIAN_POINT('Ctrl Pts',(28.4494650758024,28.4647367196518,-79.9811770740478));
#164879=CARTESIAN_POINT('Ctrl Pts',(28.456139456048,28.4542917122619,-80.1075719763809));
#164880=CARTESIAN_POINT('Ctrl Pts',(28.4627813333619,28.4438975700234,-80.2333513601604));
#164881=CARTESIAN_POINT('Ctrl Pts',(28.4691315766389,28.4363225305539,-80.3537143519523));
#164882=CARTESIAN_POINT('Ctrl Pts',(28.475187812645,28.4309666690402,-80.4685926700759));
#164883=CARTESIAN_POINT('Ctrl Pts',(28.4812043109995,28.4256459497102,-80.5827172205828));
#164884=CARTESIAN_POINT('Ctrl Pts',(28.4869306496675,28.4225153561887,-80.6914288347818));
#164885=CARTESIAN_POINT('Ctrl Pts',(28.4923647656175,28.4210378446978,-80.7946657755264));
#164886=CARTESIAN_POINT('Ctrl Pts',(28.4949774611128,28.4203274646375,-80.8443015750761));
#164887=CARTESIAN_POINT('Ctrl Pts',(28.4975226090316,28.41999998,-80.8926719059585));
#164888=CARTESIAN_POINT('Ctrl Pts',(28.5,28.41999998,-80.9397703408579));
#164889=CARTESIAN_POINT('Origin',(-3.54807775957937E-14,-73.08000002,3.11172719585489E-30));
#164890=CARTESIAN_POINT('',(24.7,-73.08000002,-58.24995));
#164891=CARTESIAN_POINT('',(24.2,-73.08000002,-58.24995));
#164892=CARTESIAN_POINT('',(-41.5,-73.0800000199999,-58.24995));
#164893=CARTESIAN_POINT('',(24.2,-73.08000002,-174.34995));
#164894=CARTESIAN_POINT('',(24.7,-73.08000002,-58.24995));
#164895=CARTESIAN_POINT('Origin',(0.,-12.9675000200281,-179.64995));
#164896=CARTESIAN_POINT('',(41.0540572871253,28.7076050220164,-61.14995));
#164897=CARTESIAN_POINT('',(41.0540572871253,28.7076050220164,-93.3976987687948));
#164898=CARTESIAN_POINT('',(41.0540572871253,28.7076050220164,-179.64995));
#164899=CARTESIAN_POINT('',(39.3277310924369,30.3404619167909,-92.0491293459315));
#164900=CARTESIAN_POINT('Ctrl Pts',(41.0540572871253,28.7076050220164,-93.3976987687948));
#164901=CARTESIAN_POINT('Ctrl Pts',(41.0005485183022,28.7603163963106,-93.3173972926641));
#164902=CARTESIAN_POINT('Ctrl Pts',(40.944160634441,28.8156580071379,-93.239741406992));
#164903=CARTESIAN_POINT('Ctrl Pts',(40.8848550499675,28.8736049764068,-93.1647596830525));
#164904=CARTESIAN_POINT('Ctrl Pts',(40.825549465494,28.9315519456757,-93.089777959113));
#164905=CARTESIAN_POINT('Ctrl Pts',(40.7633261602461,28.992104346973,-93.0174706190487));
#164906=CARTESIAN_POINT('Ctrl Pts',(40.6981582073462,29.0552176990714,-92.9478087613683));
#164907=CARTESIAN_POINT('Ctrl Pts',(40.6329902544463,29.1183310511698,-92.8781469036879));
#164908=CARTESIAN_POINT('Ctrl Pts',(40.5648738243989,29.1840092134169,-92.8111449499777));
#164909=CARTESIAN_POINT('Ctrl Pts',(40.4937697303936,29.252209946825,-92.7468029017649));
#164910=CARTESIAN_POINT('Ctrl Pts',(40.4582176833909,29.2863103135291,-92.7146318776585));
#164911=CARTESIAN_POINT('Ctrl Pts',(40.4219186395222,29.3210412388419,-92.6831258300065));
#164912=CARTESIAN_POINT('Ctrl Pts',(40.3848672142056,29.3563968380406,-92.6522847588729));
#164913=CARTESIAN_POINT('Ctrl Pts',(40.3663415015473,29.3740746376399,-92.636864223306));
#164914=CARTESIAN_POINT('Ctrl Pts',(40.3476276875811,29.3919085994207,-92.6216099318634));
#164915=CARTESIAN_POINT('Ctrl Pts',(40.3287250640418,29.4098979464083,-92.6065218845213));
#164916=CARTESIAN_POINT('Ctrl Pts',(40.3174895957419,29.4205905752593,-92.5975537496341));
#164917=CARTESIAN_POINT('Ctrl Pts',(40.3057313639822,29.4317717047969,-92.5882858994004));
#164918=CARTESIAN_POINT('Ctrl Pts',(40.2942617097069,29.4426692733808,-92.5793606574514));
#164919=CARTESIAN_POINT('Ctrl Pts',(40.2864347444641,29.4501058436985,-92.573270015411));
#164920=CARTESIAN_POINT('Ctrl Pts',(40.2787427202192,29.4574099458675,-92.5673379096353));
#164921=CARTESIAN_POINT('Ctrl Pts',(40.2714498226746,29.4643315355271,-92.5617569979654));
#164922=CARTESIAN_POINT('Ctrl Pts',(40.2711504835721,29.4646156341893,-92.5615279278215));
#164923=CARTESIAN_POINT('Ctrl Pts',(40.270851117812,29.4648997520497,-92.5612989110134));
#164924=CARTESIAN_POINT('Ctrl Pts',(40.2705517253855,29.4651838891131,-92.5610699475012));
#164925=CARTESIAN_POINT('Ctrl Pts',(40.2116149290431,29.5211175960337,-92.5159974116276));
#164926=CARTESIAN_POINT('Ctrl Pts',(40.1515495404995,29.5778784346942,-92.4730805866532));
#164927=CARTESIAN_POINT('Ctrl Pts',(40.0903677987547,29.6354412520569,-92.4322300633291));
#164928=CARTESIAN_POINT('Ctrl Pts',(40.0278547511154,29.6942566280402,-92.3904906384971));
#164929=CARTESIAN_POINT('Ctrl Pts',(39.9641756860206,29.7539098610732,-92.3509081401424));
#164930=CARTESIAN_POINT('Ctrl Pts',(39.8993230643698,29.8143876478948,-92.3134354060481));
#164931=CARTESIAN_POINT('Ctrl Pts',(39.83468856135,29.8746620299545,-92.2760887038898));
#164932=CARTESIAN_POINT('Ctrl Pts',(39.7688877366747,29.9357560969925,-92.2408374710607));
#164933=CARTESIAN_POINT('Ctrl Pts',(39.7019020445249,29.9976603583428,-92.2076851487087));
#164934=CARTESIAN_POINT('Ctrl Pts',(39.6368741274445,30.0577553584066,-92.1755017614847));
#164935=CARTESIAN_POINT('Ctrl Pts',(39.5707289868318,30.1186144848593,-92.1452964437428));
#164936=CARTESIAN_POINT('Ctrl Pts',(39.5034483725263,30.1802232711375,-92.1171198578927));
#164937=CARTESIAN_POINT('Ctrl Pts',(39.4457147020241,30.2330899312259,-92.0929414561326));
#164938=CARTESIAN_POINT('Ctrl Pts',(39.3871446932213,30.2865087402759,-92.070257565583));
#164939=CARTESIAN_POINT('Ctrl Pts',(39.3277310924369,30.3404619167909,-92.0491293459315));
#164940=CARTESIAN_POINT('',(39.3277310924369,30.3404619167909,-61.14995));
#164941=CARTESIAN_POINT('',(39.3277310924369,30.340461916791,-179.64995));
#164942=CARTESIAN_POINT('Origin',(0.,-12.9675000200281,-61.14995));
#164943=CARTESIAN_POINT('Origin',(0.,-12.9675000200281,-60.64995));
#164944=CARTESIAN_POINT('',(42.,-56.3473237326805,-60.64995));
#164945=CARTESIAN_POINT('',(43.1572831724516,-55.08000002,-60.64995));
#164946=CARTESIAN_POINT('Origin',(44.5079524583206,-57.4754524783489,-60.64995));
#164947=CARTESIAN_POINT('',(42.,-12.9675000200281,-60.64995));
#164948=CARTESIAN_POINT('',(-1.8445455022812E-14,-55.08000002,-60.64995));
#164949=CARTESIAN_POINT('Origin',(57.,-45.43000002,-174.34995));
#164950=CARTESIAN_POINT('',(57.,-44.93000002,-176.84995));
#164951=CARTESIAN_POINT('Origin',(57.,-45.43000002,-176.84995));
#164952=CARTESIAN_POINT('',(59.5,-44.93000002,-174.34995));
#164953=CARTESIAN_POINT('Origin',(57.,-44.93000002,-174.34995));
#164954=CARTESIAN_POINT('Origin',(59.5,-45.43000002,-174.34995));
#164955=CARTESIAN_POINT('Origin',(59.5,-45.43000002,-55.2499500000007));
#164956=CARTESIAN_POINT('',(59.5,-44.93000002,-58.24995));
#164957=CARTESIAN_POINT('',(59.5,-44.93000002,-174.34995));
#164958=CARTESIAN_POINT('Origin',(59.5,-45.43000002,-58.24995));
#164959=CARTESIAN_POINT('Ctrl Pts',(40.7712064624936,-44.93000002,-76.6047958451324));
#164960=CARTESIAN_POINT('Ctrl Pts',(39.9673804148565,-44.93000002,-76.1313366308109));
#164961=CARTESIAN_POINT('Ctrl Pts',(40.4124516249929,-44.1531545436406,
-76.3934867142621));
#164962=CARTESIAN_POINT('Ctrl Pts',(43.7236852143189,-44.93000002,-71.5921585277583));
#164963=CARTESIAN_POINT('Ctrl Pts',(42.8619820924489,-44.9300000200589,
-71.2817568775718));
#164964=CARTESIAN_POINT('Ctrl Pts',(43.3552388512871,-44.1657199195518,
-71.3808409460202));
#164965=CARTESIAN_POINT('Ctrl Pts',(46.5890843541627,-44.93000002,-66.5297716146547));
#164966=CARTESIAN_POINT('Ctrl Pts',(45.7723278216974,-44.9300000200823,
-66.2016926213901));
#164967=CARTESIAN_POINT('Ctrl Pts',(46.2131449010667,-44.1767154324357,
-66.3184583453296));
#164968=CARTESIAN_POINT('Ctrl Pts',(49.4036629110189,-44.93000002,-61.4386408691297));
#164969=CARTESIAN_POINT('Ctrl Pts',(48.6588221091936,-44.93000002,-61.026863396898));
#164970=CARTESIAN_POINT('Ctrl Pts',(49.0214378669496,-44.1865817238571,
-61.2273317382593));
#164971=CARTESIAN_POINT('',(40.7712064624936,-44.93000002,-76.6047958451324));
#164972=CARTESIAN_POINT('Origin',(40.7712064624936,-44.43000002,-76.6047958451324));
#164973=CARTESIAN_POINT('',(49.0214378669496,-44.1865817238571,-61.2273317382593));
#164974=CARTESIAN_POINT('Ctrl Pts',(49.0214378669496,-44.1865817238571,
-61.2273317382593));
#164975=CARTESIAN_POINT('Ctrl Pts',(48.4420648309483,-44.1845462299615,
-62.2776713982629));
#164976=CARTESIAN_POINT('Ctrl Pts',(47.868763221355,-44.1824913928638,-63.3119433794598));
#164977=CARTESIAN_POINT('Ctrl Pts',(47.3014167078854,-44.180417648187,-64.3300966156723));
#164978=CARTESIAN_POINT('Ctrl Pts',(46.7009617895993,-44.1782228868536,
-65.4076657973598));
#164979=CARTESIAN_POINT('Ctrl Pts',(46.1071770969554,-44.1760069450256,
-66.4671799588015));
#164980=CARTESIAN_POINT('Ctrl Pts',(45.5199776965721,-44.1737709346618,
-67.5086101966259));
#164981=CARTESIAN_POINT('Ctrl Pts',(44.9377500540171,-44.1715538563711,
-68.5412227501437));
#164982=CARTESIAN_POINT('Ctrl Pts',(44.3619970347197,-44.1693170524919,
-69.5560565352758));
#164983=CARTESIAN_POINT('Ctrl Pts',(43.7926841712506,-44.1670621447943,
-70.5531122444581));
#164984=CARTESIAN_POINT('Ctrl Pts',(43.2048774090488,-44.1647339873297,
-71.5825569061823));
#164985=CARTESIAN_POINT('Ctrl Pts',(42.623936078368,-44.1623865319684,-72.5930497443139));
#164986=CARTESIAN_POINT('Ctrl Pts',(42.0498710589263,-44.160022100411,-73.5846206914654));
#164987=CARTESIAN_POINT('Ctrl Pts',(41.4976856632468,-44.1577477856019,
-74.5383994051199));
#164988=CARTESIAN_POINT('Ctrl Pts',(40.9518629506906,-44.1554577703291,
-75.4746714241381));
#164989=CARTESIAN_POINT('Ctrl Pts',(40.4124516249929,-44.1531545436406,
-76.3934867142621));
#164990=CARTESIAN_POINT('',(49.4036629110189,-44.93000002,-61.4386408691297));
#164991=CARTESIAN_POINT('Origin',(49.4036629110189,-44.43000002,-61.4386408691297));
#164992=CARTESIAN_POINT('Ctrl Pts',(40.7712064624936,-44.93000002,-76.6047958451324));
#164993=CARTESIAN_POINT('Ctrl Pts',(43.723712605206,-44.93000002,-71.5921120242627));
#164994=CARTESIAN_POINT('Ctrl Pts',(46.5890589653218,-44.93000002,-66.5298175388285));
#164995=CARTESIAN_POINT('Ctrl Pts',(49.4036629110189,-44.93000002,-61.4386408691297));
#164996=CARTESIAN_POINT('Ctrl Pts',(40.4124516249929,-44.1531545436406,
-76.3934867142621));
#164997=CARTESIAN_POINT('Ctrl Pts',(39.9673804148565,-44.93000002,-76.1313366308109));
#164998=CARTESIAN_POINT('Ctrl Pts',(40.7712064624936,-44.93000002,-76.6047958451324));
#164999=CARTESIAN_POINT('Ctrl Pts',(40.1609837329219,-44.174100053011,-76.7929803513312));
#165000=CARTESIAN_POINT('Ctrl Pts',(39.7695444931039,-44.93000002,-76.5732367689873));
#165001=CARTESIAN_POINT('Ctrl Pts',(40.5448762480367,-44.93000002,-76.9890530774658));
#165002=CARTESIAN_POINT('Ctrl Pts',(39.9523146669981,-44.1958519161918,
-77.2080863135005));
#165003=CARTESIAN_POINT('Ctrl Pts',(39.6033636235116,-44.93000002,-77.035174184732));
#165004=CARTESIAN_POINT('Ctrl Pts',(40.3570832012011,-44.93000002,-77.3881516643461));
#165005=CARTESIAN_POINT('Ctrl Pts',(39.5996235521064,-44.2405416721215,
-78.0616481127407));
#165006=CARTESIAN_POINT('Ctrl Pts',(39.3379923637148,-44.93000002,-77.9585218257824));
#165007=CARTESIAN_POINT('Ctrl Pts',(40.039661195993,-44.93000002,-78.208477386432));
#165008=CARTESIAN_POINT('Ctrl Pts',(39.4559266167971,-44.2634896702644,
-78.5002957502421));
#165009=CARTESIAN_POINT('Ctrl Pts',(39.2335339077575,-44.93000002,-78.4222204753855));
#165010=CARTESIAN_POINT('Ctrl Pts',(39.9103339554084,-44.93000002,-78.6298739674098));
#165011=CARTESIAN_POINT('Ctrl Pts',(39.1112085107541,-44.333906530637,-79.8478079198197));
#165012=CARTESIAN_POINT('Ctrl Pts',(39.010584818663,-44.93000002,-79.7803625539821));
#165013=CARTESIAN_POINT('Ctrl Pts',(39.6000876590965,-44.93000002,-79.9237827775448));
#165014=CARTESIAN_POINT('Ctrl Pts',(39.,-44.381938656112,-80.7689356438042));
#165015=CARTESIAN_POINT('Ctrl Pts',(38.9494857171145,-44.9300000199999,
-80.7217336743568));
#165016=CARTESIAN_POINT('Ctrl Pts',(39.5000000012115,-44.93000002,-80.807470573569));
#165017=CARTESIAN_POINT('Ctrl Pts',(39.,-44.43000002,-81.6937887068282));
#165018=CARTESIAN_POINT('Ctrl Pts',(38.9999999999999,-44.9300000199999,
-81.6937887068281));
#165019=CARTESIAN_POINT('Ctrl Pts',(39.5,-44.93000002,-81.6937887068282));
#165020=CARTESIAN_POINT('',(39.5,-44.93000002,-81.6937887068282));
#165021=CARTESIAN_POINT('Origin',(39.5,-44.43000002,-81.6937887068282));
#165022=CARTESIAN_POINT('Ctrl Pts',(39.5,-44.93000002,-81.6937887068282));
#165023=CARTESIAN_POINT('Ctrl Pts',(39.5,-44.93000002,-81.4715915443628));
#165024=CARTESIAN_POINT('Ctrl Pts',(39.5062851881924,-44.93000002,-81.2500804744028));
#165025=CARTESIAN_POINT('Ctrl Pts',(39.5189031887286,-44.93000002,-81.0292580402079));
#165026=CARTESIAN_POINT('Ctrl Pts',(39.5308326200064,-44.93000002,-80.82048597321));
#165027=CARTESIAN_POINT('Ctrl Pts',(39.548422932141,-44.93000002,-80.6123290364182));
#165028=CARTESIAN_POINT('Ctrl Pts',(39.5717668549556,-44.93000002,-80.404790058523));
#165029=CARTESIAN_POINT('Ctrl Pts',(39.5731142710433,-44.93000002,-80.3928108654859));
#165030=CARTESIAN_POINT('Ctrl Pts',(39.5744808704138,-44.93000002,-80.3808337323854));
#165031=CARTESIAN_POINT('Ctrl Pts',(39.5758666762242,-44.93000002,-80.3688586602484));
#165032=CARTESIAN_POINT('Ctrl Pts',(39.5992261762147,-44.93000002,-80.167003757221));
#165033=CARTESIAN_POINT('Ctrl Pts',(39.6280811656786,-44.93000002,-79.9654411052776));
#165034=CARTESIAN_POINT('Ctrl Pts',(39.6625124125991,-44.93000002,-79.7646415180466));
#165035=CARTESIAN_POINT('Ctrl Pts',(39.6964841131886,-44.93000002,-79.5665219590398));
#165036=CARTESIAN_POINT('Ctrl Pts',(39.7358842319638,-44.93000002,-79.3691455608367));
#165037=CARTESIAN_POINT('Ctrl Pts',(39.780739886981,-44.93000002,-79.1729578992698));
#165038=CARTESIAN_POINT('Ctrl Pts',(39.7892690083243,-44.93000002,-79.1356536090772));
#165039=CARTESIAN_POINT('Ctrl Pts',(39.7979952284866,-44.93000002,-79.0983922704899));
#165040=CARTESIAN_POINT('Ctrl Pts',(39.8069185231454,-44.93000002,-79.0611769040833));
#165041=CARTESIAN_POINT('Ctrl Pts',(39.910333955099,-44.93000002,-78.6298739672844));
#165042=CARTESIAN_POINT('Ctrl Pts',(40.0396611959927,-44.93000002,-78.2084773864585));
#165043=CARTESIAN_POINT('Ctrl Pts',(40.1983721980467,-44.93000002,-77.7983145251761));
#165044=CARTESIAN_POINT('Ctrl Pts',(40.3310078543844,-44.93000002,-77.4555391686635));
#165045=CARTESIAN_POINT('Ctrl Pts',(40.483938162075,-44.93000002,-77.1205226744407));
#165046=CARTESIAN_POINT('Ctrl Pts',(40.662722300217,-44.93000002,-76.7953903626101));
#165047=CARTESIAN_POINT('Ctrl Pts',(40.697870150647,-44.93000002,-76.7314713707748));
#165048=CARTESIAN_POINT('Ctrl Pts',(40.734017377992,-44.93000002,-76.6679344511747));
#165049=CARTESIAN_POINT('Ctrl Pts',(40.7712064624936,-44.93000002,-76.6047958451324));
#165050=CARTESIAN_POINT('Origin',(39.5,-44.43000002,-55.2499500000007));
#165051=CARTESIAN_POINT('',(39.5,-44.93000002,-150.364854264666));
#165052=CARTESIAN_POINT('Origin',(39.5,-44.43000002,-150.364854264666));
#165053=CARTESIAN_POINT('',(39.5,-44.93000002,-55.2499500000007));
#165054=CARTESIAN_POINT('Ctrl Pts',(39.0055150586856,-44.4477113456027,
-150.003379856068));
#165055=CARTESIAN_POINT('Ctrl Pts',(39.0227012659498,-44.93000002,-150.00371437679));
#165056=CARTESIAN_POINT('Ctrl Pts',(39.5049987237219,-44.93000002,-150.018486848937));
#165057=CARTESIAN_POINT('Ctrl Pts',(38.9734136439675,-44.3930232755833,
-151.055460419798));
#165058=CARTESIAN_POINT('Ctrl Pts',(38.9344833976404,-44.93000002,-151.111926007989));
#165059=CARTESIAN_POINT('Ctrl Pts',(39.4760001584505,-44.93000002,-151.026575388255));
#165060=CARTESIAN_POINT('Ctrl Pts',(39.0810964939062,-44.3391675960254,
-152.087737194438));
#165061=CARTESIAN_POINT('Ctrl Pts',(38.9915721940229,-44.93000002,-152.165744946158));
#165062=CARTESIAN_POINT('Ctrl Pts',(39.5728295161603,-44.93000002,-152.016813423143));
#165063=CARTESIAN_POINT('Ctrl Pts',(39.4525277093705,-44.2629792367123,
-153.545360859045));
#165064=CARTESIAN_POINT('Ctrl Pts',(39.2290603541538,-44.93000002,-153.623344231399));
#165065=CARTESIAN_POINT('Ctrl Pts',(39.9069198952433,-44.93000002,-153.416428338509));
#165066=CARTESIAN_POINT('Ctrl Pts',(39.5975827673942,-44.2397053437839,
-153.990247284421));
#165067=CARTESIAN_POINT('Ctrl Pts',(39.3342779655495,-44.93000002,-154.093989914495));
#165068=CARTESIAN_POINT('Ctrl Pts',(40.0374208080396,-44.93000002,-153.8438516675));
#165069=CARTESIAN_POINT('Ctrl Pts',(39.9982241297396,-44.1889106964072,
-154.960684718783));
#165070=CARTESIAN_POINT('Ctrl Pts',(39.638422111897,-44.9300000199999,-155.155380476238));
#165071=CARTESIAN_POINT('Ctrl Pts',(40.3978966779789,-44.93000002,-154.776621822351));
#165072=CARTESIAN_POINT('Ctrl Pts',(40.2725981949087,-44.1616758422127,
-155.480642655351));
#165073=CARTESIAN_POINT('Ctrl Pts',(39.8606808421836,-44.9300000200001,
-155.739479736185));
#165074=CARTESIAN_POINT('Ctrl Pts',(40.6447774862557,-44.93000002,-155.276660282544));
#165075=CARTESIAN_POINT('Ctrl Pts',(40.6171580660072,-44.1359519133608,
-155.971665887251));
#165076=CARTESIAN_POINT('Ctrl Pts',(40.1350091672924,-44.93000002,-156.289052674551));
#165077=CARTESIAN_POINT('Ctrl Pts',(40.9548496935007,-44.93000002,-155.74912533543));
#165078=CARTESIAN_POINT('',(40.7712064624936,-44.93000002,-155.453847126373));
#165079=CARTESIAN_POINT('Origin',(40.7712064624936,-44.43000002,-155.453847126373));
#165080=CARTESIAN_POINT('Ctrl Pts',(40.7712064624936,-44.93000002,-155.453847126373));
#165081=CARTESIAN_POINT('Ctrl Pts',(40.5636969173263,-44.93000002,-155.101543121101));
#165082=CARTESIAN_POINT('Ctrl Pts',(40.3878808276675,-44.93000002,-154.735494168673));
#165083=CARTESIAN_POINT('Ctrl Pts',(40.2370488760061,-44.93000002,-154.35860999499));
#165084=CARTESIAN_POINT('Ctrl Pts',(40.2234902738163,-44.93000002,-154.324731081893));
#165085=CARTESIAN_POINT('Ctrl Pts',(40.2101335892401,-44.93000002,-154.290764600318));
#165086=CARTESIAN_POINT('Ctrl Pts',(40.1969739657515,-44.93000002,-154.256712656464));
#165087=CARTESIAN_POINT('Ctrl Pts',(40.0374208080236,-44.93000002,-153.843851667435));
#165088=CARTESIAN_POINT('Ctrl Pts',(39.9069198944888,-44.93000002,-153.416428338648));
#165089=CARTESIAN_POINT('Ctrl Pts',(39.8044156663649,-44.93000002,-152.987004278786));
#165090=CARTESIAN_POINT('Ctrl Pts',(39.6913863431124,-44.93000002,-152.513487119906));
#165091=CARTESIAN_POINT('Ctrl Pts',(39.6104670975054,-44.93000002,-152.035255380817));
#165092=CARTESIAN_POINT('Ctrl Pts',(39.5605987441789,-44.93000002,-151.552464535406));
#165093=CARTESIAN_POINT('Ctrl Pts',(39.5200177005092,-44.93000002,-151.159586987341));
#165094=CARTESIAN_POINT('Ctrl Pts',(39.4999999999997,-44.93000002,-150.763690175803));
#165095=CARTESIAN_POINT('Ctrl Pts',(39.5,-44.93000002,-150.364854264666));
#165096=CARTESIAN_POINT('Ctrl Pts',(49.5369875341119,-44.93000002,-170.861259130871));
#165097=CARTESIAN_POINT('Ctrl Pts',(48.7929216289437,-44.9300000199999,
-171.272289063137));
#165098=CARTESIAN_POINT('Ctrl Pts',(49.1544657093286,-44.1870483688939,
-171.07256826174));
#165099=CARTESIAN_POINT('Ctrl Pts',(46.6796506810215,-44.93000002,-165.688772250388));
#165100=CARTESIAN_POINT('Ctrl Pts',(45.8620651160177,-44.9300000199373,
-166.013584137672));
#165101=CARTESIAN_POINT('Ctrl Pts',(46.303473398785,-44.1770628106394,-165.900085726624));
#165102=CARTESIAN_POINT('Ctrl Pts',(43.7703248719811,-44.93000002,-160.54566797298));
#165103=CARTESIAN_POINT('Ctrl Pts',(42.9064403928045,-44.93000002,-160.851370978315));
#165104=CARTESIAN_POINT('Ctrl Pts',(43.4017256360502,-44.1659184128467,
-160.756986066495));
#165105=CARTESIAN_POINT('Ctrl Pts',(40.7712064624936,-44.93000002,-155.453847126373));
#165106=CARTESIAN_POINT('Ctrl Pts',(39.9673804148566,-44.93000002,-155.927306340695));
#165107=CARTESIAN_POINT('Ctrl Pts',(40.4124516249929,-44.1531545436406,
-155.665156257244));
#165108=CARTESIAN_POINT('',(49.5369875341119,-44.93000002,-170.861259130871));
#165109=CARTESIAN_POINT('Origin',(49.5369875341119,-44.43000002,-170.861259130871));
#165110=CARTESIAN_POINT('Ctrl Pts',(49.5369875341119,-44.93000002,-170.861259130871));
#165111=CARTESIAN_POINT('Ctrl Pts',(46.6796235355215,-44.93000002,-165.688723110732));
#165112=CARTESIAN_POINT('Ctrl Pts',(43.770354187064,-44.93000002,-160.545717743323));
#165113=CARTESIAN_POINT('Ctrl Pts',(40.7712064624936,-44.93000002,-155.453847126373));
#165114=CARTESIAN_POINT('Ctrl Pts',(49.1544657093286,-44.1870483688939,
-171.07256826174));
#165115=CARTESIAN_POINT('Ctrl Pts',(48.7929216289437,-44.9300000199999,
-171.272289063137));
#165116=CARTESIAN_POINT('Ctrl Pts',(49.5369875341119,-44.93000002,-170.861259130871));
#165117=CARTESIAN_POINT('Ctrl Pts',(49.1988333494309,-44.1988790013969,
-171.166486883581));
#165118=CARTESIAN_POINT('Ctrl Pts',(48.8869683938206,-44.93000002,-171.389208114715));
#165119=CARTESIAN_POINT('Ctrl Pts',(49.5629323055535,-44.93000002,-170.908225431312));
#165120=CARTESIAN_POINT('Ctrl Pts',(49.2553422033029,-44.2139336491638,
-171.248946535323));
#165121=CARTESIAN_POINT('Ctrl Pts',(48.9974211832039,-44.93000002,-171.47664075754));
#165122=CARTESIAN_POINT('Ctrl Pts',(49.5959607588443,-44.93000002,-170.94944826591));
#165123=CARTESIAN_POINT('Ctrl Pts',(49.3888358236751,-44.249424483408,-171.394272113556));
#165124=CARTESIAN_POINT('Ctrl Pts',(49.2286028218105,-44.93000002,-171.604363908288));
#165125=CARTESIAN_POINT('Ctrl Pts',(49.673955990897,-44.93000002,-171.02211105853));
#165126=CARTESIAN_POINT('Ctrl Pts',(49.4642369070823,-44.2694386569593,
-171.45497652175));
#165127=CARTESIAN_POINT('Ctrl Pts',(49.3448677594853,-44.9300000199992,
-171.644582495821));
#165128=CARTESIAN_POINT('Ctrl Pts',(49.7179930277929,-44.93000002,-171.052463257479));
#165129=CARTESIAN_POINT('Ctrl Pts',(49.7071198591548,-44.3337582466603,
-171.601144400479));
#165130=CARTESIAN_POINT('Ctrl Pts',(49.6719308335793,-44.9300000200013,
-171.711639121533));
#165131=CARTESIAN_POINT('Ctrl Pts',(49.8597665056525,-44.93000002,-171.125547207032));
#165132=CARTESIAN_POINT('Ctrl Pts',(49.8895242589787,-44.3818638633066,
-171.64995));
#165133=CARTESIAN_POINT('Ctrl Pts',(49.8809090309114,-44.93000002,-171.700346637809));
#165134=CARTESIAN_POINT('Ctrl Pts',(49.9661358829125,-44.93000002,-171.149949988199));
#165135=CARTESIAN_POINT('Ctrl Pts',(50.0729884546894,-44.43000002,-171.64995));
#165136=CARTESIAN_POINT('Ctrl Pts',(50.0729884546893,-44.93000002,-171.64995));
#165137=CARTESIAN_POINT('Ctrl Pts',(50.0729884546894,-44.93000002,-171.14995));
#165138=CARTESIAN_POINT('',(50.0729884546894,-44.93000002,-171.14995));
#165139=CARTESIAN_POINT('Origin',(50.0729884546894,-44.43000002,-171.14995));
#165140=CARTESIAN_POINT('Ctrl Pts',(50.0729884546894,-44.93000002,-171.14995));
#165141=CARTESIAN_POINT('Ctrl Pts',(50.0168171487347,-44.93000002,-171.14995));
#165142=CARTESIAN_POINT('Ctrl Pts',(49.9608486377796,-44.93000002,-171.143210614633));
#165143=CARTESIAN_POINT('Ctrl Pts',(49.9066731284767,-44.93000002,-171.129767219264));
#165144=CARTESIAN_POINT('Ctrl Pts',(49.8576729639836,-44.93000002,-171.117608061132));
#165145=CARTESIAN_POINT('Ctrl Pts',(49.8101382025079,-44.93000002,-171.099963916563));
#165146=CARTESIAN_POINT('Ctrl Pts',(49.7652508518366,-44.93000002,-171.076824577701));
#165147=CARTESIAN_POINT('Ctrl Pts',(49.7179896877752,-44.93000002,-171.052461542819));
#165148=CARTESIAN_POINT('Ctrl Pts',(49.6739559670876,-44.93000002,-171.022111093102));
#165149=CARTESIAN_POINT('Ctrl Pts',(49.6349583346168,-44.93000002,-170.985779705428));
#165150=CARTESIAN_POINT('Ctrl Pts',(49.5959662083459,-44.93000002,-170.949453447498));
#165151=CARTESIAN_POINT('Ctrl Pts',(49.5629377334322,-44.93000002,-170.908235414179));
#165152=CARTESIAN_POINT('Ctrl Pts',(49.5369875341119,-44.93000002,-170.861259130871));
#165153=CARTESIAN_POINT('Origin',(-1.31515029790052E-14,-44.43000002,-171.14995));
#165154=CARTESIAN_POINT('',(50.7754831343094,-44.93000002,-171.14995));
#165155=CARTESIAN_POINT('Origin',(50.7754831343094,-44.43000002,-171.14995));
#165156=CARTESIAN_POINT('',(49.7553180351958,-44.93000002,-171.14995));
#165157=CARTESIAN_POINT('Ctrl Pts',(52.2902244930873,-44.93000002,-172.64995));
#165158=CARTESIAN_POINT('Ctrl Pts',(51.7150402894768,-44.93000002,-172.64995));
#165159=CARTESIAN_POINT('Ctrl Pts',(51.7950904587165,-44.36041346952,-172.64995));
#165160=CARTESIAN_POINT('Ctrl Pts',(52.2902244930723,-44.93000002,-172.453565067926));
#165161=CARTESIAN_POINT('Ctrl Pts',(51.7150402894748,-44.9300000200027,
-172.529650273729));
#165162=CARTESIAN_POINT('Ctrl Pts',(51.7950904587162,-44.3604134695225,
-172.51902671195));
#165163=CARTESIAN_POINT('Ctrl Pts',(52.2507998243741,-44.93000002,-172.257328160063));
#165164=CARTESIAN_POINT('Ctrl Pts',(51.6933705738162,-44.93000002,-172.409726298163));
#165165=CARTESIAN_POINT('Ctrl Pts',(51.7685528054411,-44.3622246214263,
-172.38820210671));
#165166=CARTESIAN_POINT('Ctrl Pts',(52.0990435210912,-44.93000002,-171.894521542842));
#165167=CARTESIAN_POINT('Ctrl Pts',(51.6069372443981,-44.93000002,-172.182182441317));
#165168=CARTESIAN_POINT('Ctrl Pts',(51.6664021396144,-44.3691962391205,
-172.14633102856));
#165169=CARTESIAN_POINT('Ctrl Pts',(51.9867715634496,-44.93000002,-171.728129909852));
#165170=CARTESIAN_POINT('Ctrl Pts',(51.5426661785871,-44.9300000199979,
-172.075215659168));
#165171=CARTESIAN_POINT('Ctrl Pts',(51.5908292969809,-44.3743539633763,
-172.035403273235));
#165172=CARTESIAN_POINT('Ctrl Pts',(51.7063624782404,-44.93000002,-171.450449746589));
#165173=CARTESIAN_POINT('Ctrl Pts',(51.3750094074331,-44.930000020002,-171.888983273332));
#165174=CARTESIAN_POINT('Ctrl Pts',(51.4020794781095,-44.387235833176,-171.850283164392));
#165175=CARTESIAN_POINT('Ctrl Pts',(51.5383356195984,-44.93000002,-171.339270411997));
#165176=CARTESIAN_POINT('Ctrl Pts',(51.2724346946947,-44.9300000200007,
-171.809929875206));
#165177=CARTESIAN_POINT('Ctrl Pts',(51.2889767264242,-44.3949549130127,
-171.776163607997));
#165178=CARTESIAN_POINT('Ctrl Pts',(51.1719634936654,-44.93000002,-171.18899099047));
#165179=CARTESIAN_POINT('Ctrl Pts',(51.0396558988745,-44.9300000199993,
-171.69520402023));
#165180=CARTESIAN_POINT('Ctrl Pts',(51.0423632033321,-44.411785887019,-171.675977326981));
#165181=CARTESIAN_POINT('Ctrl Pts',(50.9737980536844,-44.93000002,-171.149950000016));
#165182=CARTESIAN_POINT('Ctrl Pts',(50.9102650806209,-44.93000002,-171.659148653595));
#165183=CARTESIAN_POINT('Ctrl Pts',(50.9089734778343,-44.4208895200012,
-171.64995));
#165184=CARTESIAN_POINT('Ctrl Pts',(50.7754831343094,-44.93000002,-171.14995));
#165185=CARTESIAN_POINT('Ctrl Pts',(50.7754831343094,-44.9300000199999,
-171.64995));
#165186=CARTESIAN_POINT('Ctrl Pts',(50.7754831343094,-44.43000002,-171.64995));
#165187=CARTESIAN_POINT('',(52.2902244930873,-44.93000002,-172.64995));
#165188=CARTESIAN_POINT('',(51.7902244930873,-44.43000002,-172.64995));
#165189=CARTESIAN_POINT('Origin',(52.2902244930873,-44.43000002,-172.64995));
#165190=CARTESIAN_POINT('Origin',(52.2902244930873,-44.43000002,-172.64995));
#165191=CARTESIAN_POINT('Ctrl Pts',(52.2902244930873,-44.93000002,-172.64995));
#165192=CARTESIAN_POINT('Ctrl Pts',(52.2902244930723,-44.93000002,-172.453565067926));
#165193=CARTESIAN_POINT('Ctrl Pts',(52.2507998243741,-44.93000002,-172.257328160063));
#165194=CARTESIAN_POINT('Ctrl Pts',(52.0990435210912,-44.93000002,-171.894521542842));
#165195=CARTESIAN_POINT('Ctrl Pts',(51.9867715634496,-44.93000002,-171.728129909852));
#165196=CARTESIAN_POINT('Ctrl Pts',(51.7063624782404,-44.93000002,-171.450449746589));
#165197=CARTESIAN_POINT('Ctrl Pts',(51.5383356195984,-44.93000002,-171.339270411997));
#165198=CARTESIAN_POINT('Ctrl Pts',(51.1719634936654,-44.93000002,-171.18899099047));
#165199=CARTESIAN_POINT('Ctrl Pts',(50.9737980536844,-44.93000002,-171.149950000016));
#165200=CARTESIAN_POINT('Ctrl Pts',(50.7754831343094,-44.93000002,-171.14995));
#165201=CARTESIAN_POINT('Origin',(52.2902244930873,-44.43000002,-171.64995));
#165202=CARTESIAN_POINT('',(52.2902244930873,-44.93000002,-55.2499500000007));
#165203=CARTESIAN_POINT('',(51.7950904587165,-44.36041346952,-171.64995));
#165204=CARTESIAN_POINT('Origin',(60.,-45.43000002,-176.84995));
#165205=CARTESIAN_POINT('',(-83.2809572255632,-44.93000002,-176.84995));
#165206=CARTESIAN_POINT('Origin',(-83.2809572255632,-44.43000002,-61.14995));
#165207=CARTESIAN_POINT('',(49.940073970993,-44.93000002,-61.14995));
#165208=CARTESIAN_POINT('',(49.940073970993,-44.43000002,-60.64995));
#165209=CARTESIAN_POINT('Origin',(49.940073970993,-44.43000002,-61.14995));
#165210=CARTESIAN_POINT('',(51.3752989258075,-44.43000002,-60.64995));
#165211=CARTESIAN_POINT('',(-1.31515029790052E-14,-44.43000002,-60.64995));
#165212=CARTESIAN_POINT('',(51.3752989258075,-44.93000002,-61.14995));
#165213=CARTESIAN_POINT('Origin',(51.3752989258075,-44.43000002,-61.14995));
#165214=CARTESIAN_POINT('',(-83.2809572255632,-44.93000002,-61.14995));
#165215=CARTESIAN_POINT('Origin',(57.,-45.43000002,-58.24995));
#165216=CARTESIAN_POINT('',(57.,-44.93000002,-55.74995));
#165217=CARTESIAN_POINT('Origin',(57.,-44.93000002,-58.24995));
#165218=CARTESIAN_POINT('',(57.,-45.43000002,-55.24995));
#165219=CARTESIAN_POINT('Origin',(57.,-45.43000002,-55.74995));
#165220=CARTESIAN_POINT('Origin',(57.,-45.43000002,-58.24995));
#165221=CARTESIAN_POINT('Origin',(57.,-2.42462934179819E-14,-58.24995));
#165222=CARTESIAN_POINT('',(57.,-45.93000002,-55.24995));
#165223=CARTESIAN_POINT('',(57.,28.41999998,-55.24995));
#165224=CARTESIAN_POINT('Origin',(57.,-45.93000002,-58.24995));
#165225=CARTESIAN_POINT('Origin',(57.,-45.93000002,-58.24995));
#165226=CARTESIAN_POINT('',(57.,-46.43000002,-55.74995));
#165227=CARTESIAN_POINT('Origin',(57.,-45.93000002,-55.74995));
#165228=CARTESIAN_POINT('',(59.5,-46.43000002,-58.24995));
#165229=CARTESIAN_POINT('Origin',(57.,-46.43000002,-58.24995));
#165230=CARTESIAN_POINT('Origin',(59.5,-45.93000002,-58.24995));
#165231=CARTESIAN_POINT('Origin',(59.5,-45.93000002,-55.2499500000008));
#165232=CARTESIAN_POINT('',(59.5,-46.43000002,-174.34995));
#165233=CARTESIAN_POINT('',(59.5,-46.43000002,-58.24995));
#165234=CARTESIAN_POINT('Origin',(59.5,-45.93000002,-174.34995));
#165235=CARTESIAN_POINT('Origin',(57.,-45.93000002,-174.34995));
#165236=CARTESIAN_POINT('',(57.,-46.43000002,-176.84995));
#165237=CARTESIAN_POINT('Origin',(57.,-46.43000002,-174.34995));
#165238=CARTESIAN_POINT('Origin',(57.,-45.93000002,-176.84995));
#165239=CARTESIAN_POINT('Origin',(-83.2809572255632,-45.9300000199999,-176.84995));
#165240=CARTESIAN_POINT('',(-83.2809572255632,-46.4300000199999,-176.84995));
#165241=CARTESIAN_POINT('Origin',(51.9388724063314,-46.93000002,-171.64995));
#165242=CARTESIAN_POINT('',(51.9388724063314,-46.43000002,-172.64995));
#165243=CARTESIAN_POINT('',(51.9388724063314,-46.43000002,-55.2499500000008));
#165244=CARTESIAN_POINT('Origin',(51.9388724063314,-46.93000002,-172.64995));
#165245=CARTESIAN_POINT('',(51.4437383719606,-46.86041346952,-171.64995));
#165246=CARTESIAN_POINT('Ctrl Pts',(50.4241310475534,-46.43000002,-171.14995));
#165247=CARTESIAN_POINT('Ctrl Pts',(50.4241310475535,-46.43000002,-171.64995));
#165248=CARTESIAN_POINT('Ctrl Pts',(50.4241310475534,-46.93000002,-171.64995));
#165249=CARTESIAN_POINT('Ctrl Pts',(50.6224459669284,-46.43000002,-171.149950000016));
#165250=CARTESIAN_POINT('Ctrl Pts',(50.5563794763166,-46.43000002,-171.640924254979));
#165251=CARTESIAN_POINT('Ctrl Pts',(50.5576213910783,-46.9208895200013,
-171.64995));
#165252=CARTESIAN_POINT('Ctrl Pts',(50.8206114069094,-46.43000002,-171.18899099047));
#165253=CARTESIAN_POINT('Ctrl Pts',(50.6936490544688,-46.43000002,-171.658003579003));
#165254=CARTESIAN_POINT('Ctrl Pts',(50.6910111165761,-46.911785887019,-171.675977326981));
#165255=CARTESIAN_POINT('Ctrl Pts',(51.1869835328424,-46.43000002,-171.339270411997));
#165256=CARTESIAN_POINT('Ctrl Pts',(50.9520843153697,-46.4300000199999,
-171.746711574348));
#165257=CARTESIAN_POINT('Ctrl Pts',(50.9376246396682,-46.8949549130127,
-171.776163607997));
#165258=CARTESIAN_POINT('Ctrl Pts',(51.3550103914843,-46.43000002,-171.450449746589));
#165259=CARTESIAN_POINT('Ctrl Pts',(51.0736480315269,-46.4300000199987,
-171.817687494207));
#165260=CARTESIAN_POINT('Ctrl Pts',(51.0507273913534,-46.887235833176,-171.850283164392));
#165261=CARTESIAN_POINT('Ctrl Pts',(51.6354194766937,-46.43000002,-171.728129909852));
#165262=CARTESIAN_POINT('Ctrl Pts',(51.2780932509,-46.4300000200014,-172.003556970023));
#165263=CARTESIAN_POINT('Ctrl Pts',(51.239477210225,-46.8743539633763,-172.035403273235));
#165264=CARTESIAN_POINT('Ctrl Pts',(51.7476914343352,-46.43000002,-171.894521542842));
#165265=CARTESIAN_POINT('Ctrl Pts',(51.3616623431659,-46.43000002,-172.118296873734));
#165266=CARTESIAN_POINT('Ctrl Pts',(51.3150500528584,-46.8691962391206,
-172.14633102856));
#165267=CARTESIAN_POINT('Ctrl Pts',(51.8994477376182,-46.43000002,-172.257328160063));
#165268=CARTESIAN_POINT('Ctrl Pts',(51.4744733522994,-46.43000002,-172.371853931892));
#165269=CARTESIAN_POINT('Ctrl Pts',(51.4172007186852,-46.8622246214263,
-172.38820210671));
#165270=CARTESIAN_POINT('Ctrl Pts',(51.9388724063164,-46.43000002,-172.453565067926));
#165271=CARTESIAN_POINT('Ctrl Pts',(51.5042290374097,-46.43000002,-172.511015867073));
#165272=CARTESIAN_POINT('Ctrl Pts',(51.4437383719602,-46.8604134695225,
-172.51902671195));
#165273=CARTESIAN_POINT('Ctrl Pts',(51.9388724063314,-46.43000002,-172.64995));
#165274=CARTESIAN_POINT('Ctrl Pts',(51.5042290374232,-46.43000002,-172.64995));
#165275=CARTESIAN_POINT('Ctrl Pts',(51.4437383719606,-46.86041346952,-172.64995));
#165276=CARTESIAN_POINT('',(50.4241310475534,-46.43000002,-171.14995));
#165277=CARTESIAN_POINT('Ctrl Pts',(50.4241310475534,-46.43000002,-171.14995));
#165278=CARTESIAN_POINT('Ctrl Pts',(50.6224459669284,-46.43000002,-171.149950000016));
#165279=CARTESIAN_POINT('Ctrl Pts',(50.8206114069094,-46.43000002,-171.18899099047));
#165280=CARTESIAN_POINT('Ctrl Pts',(51.1869835328424,-46.43000002,-171.339270411997));
#165281=CARTESIAN_POINT('Ctrl Pts',(51.3550103914843,-46.43000002,-171.450449746589));
#165282=CARTESIAN_POINT('Ctrl Pts',(51.6354194766937,-46.43000002,-171.728129909852));
#165283=CARTESIAN_POINT('Ctrl Pts',(51.7476914343352,-46.43000002,-171.894521542842));
#165284=CARTESIAN_POINT('Ctrl Pts',(51.8994477376182,-46.43000002,-172.257328160063));
#165285=CARTESIAN_POINT('Ctrl Pts',(51.9388724063164,-46.43000002,-172.453565067926));
#165286=CARTESIAN_POINT('Ctrl Pts',(51.9388724063314,-46.43000002,-172.64995));
#165287=CARTESIAN_POINT('Origin',(50.4241310475534,-46.93000002,-171.14995));
#165288=CARTESIAN_POINT('Origin',(-1.41965171211599E-14,-46.93000002,-171.14995));
#165289=CARTESIAN_POINT('',(48.4122058243951,-46.43000002,-171.14995));
#165290=CARTESIAN_POINT('',(50.4944014649046,-46.43000002,-171.14995));
#165291=CARTESIAN_POINT('Origin',(48.4122058243951,-46.93000002,-171.14995));
#165292=CARTESIAN_POINT('Ctrl Pts',(48.5201235179867,-46.9606462876662,
-171.644181328151));
#165293=CARTESIAN_POINT('Ctrl Pts',(48.5228147479093,-46.4300000200001,
-171.676734375474));
#165294=CARTESIAN_POINT('Ctrl Pts',(48.4767984570328,-46.43000002,-171.147074844096));
#165295=CARTESIAN_POINT('Ctrl Pts',(48.3058611060635,-46.9004466821901,
-171.667220120137));
#165296=CARTESIAN_POINT('Ctrl Pts',(48.311325817959,-46.4300000199996,-171.634847520409));
#165297=CARTESIAN_POINT('Ctrl Pts',(48.3485998488332,-46.43000002,-171.158575233343));
#165298=CARTESIAN_POINT('Ctrl Pts',(48.0796981189137,-46.8364853152072,
-171.621252940216));
#165299=CARTESIAN_POINT('Ctrl Pts',(48.1036590804166,-46.4300000200009,
-171.543768248534));
#165300=CARTESIAN_POINT('Ctrl Pts',(48.2130231518178,-46.43000002,-171.135576813935));
#165301=CARTESIAN_POINT('Ctrl Pts',(47.6908242556552,-46.7259662378658,
-171.391170182407));
#165302=CARTESIAN_POINT('Ctrl Pts',(47.7775505894744,-46.4300000199991,
-171.283378605487));
#165303=CARTESIAN_POINT('Ctrl Pts',(47.9796068491616,-46.43000002,-171.020522742606));
#165304=CARTESIAN_POINT('Ctrl Pts',(47.5227534239133,-46.677891632908,-171.205193874949));
#165305=CARTESIAN_POINT('Ctrl Pts',(47.6425982485164,-46.4300000200003,
-171.112712451737));
#165306=CARTESIAN_POINT('Ctrl Pts',(47.8785659772877,-46.43000002,-170.92757795489));
#165307=CARTESIAN_POINT('Ctrl Pts',(47.4395650454936,-46.654055562307,-170.951379521332));
#165308=CARTESIAN_POINT('Ctrl Pts',(47.5779186181849,-46.4300000199999,
-170.897903745869));
#165309=CARTESIAN_POINT('Ctrl Pts',(47.8284835237321,-46.43000002,-170.800621877871));
#165310=CARTESIAN_POINT('',(47.8576079004676,-46.43000002,-170.861259130871));
#165311=CARTESIAN_POINT('Ctrl Pts',(47.8576079004676,-46.43000002,-170.861259130871));
#165312=CARTESIAN_POINT('Ctrl Pts',(47.8760580377294,-46.43000002,-170.89352615778));
#165313=CARTESIAN_POINT('Ctrl Pts',(47.8980723549739,-46.43000002,-170.923203523829));
#165314=CARTESIAN_POINT('Ctrl Pts',(47.9228861329632,-46.43000002,-170.950192158739));
#165315=CARTESIAN_POINT('Ctrl Pts',(47.9503841163783,-46.43000002,-170.980100262029));
#165316=CARTESIAN_POINT('Ctrl Pts',(47.9813190176472,-46.43000002,-171.00670574507));
#165317=CARTESIAN_POINT('Ctrl Pts',(48.0145941519147,-46.43000002,-171.029912775459));
#165318=CARTESIAN_POINT('Ctrl Pts',(48.0405863852467,-46.43000002,-171.048040502427));
#165319=CARTESIAN_POINT('Ctrl Pts',(48.0680050205664,-46.43000002,-171.06409541242));
#165320=CARTESIAN_POINT('Ctrl Pts',(48.0963149978629,-46.43000002,-171.078049783599));
#165321=CARTESIAN_POINT('Ctrl Pts',(48.1225339813698,-46.43000002,-171.090973475624));
#165322=CARTESIAN_POINT('Ctrl Pts',(48.1495923840829,-46.43000002,-171.102104191555));
#165323=CARTESIAN_POINT('Ctrl Pts',(48.177275111639,-46.43000002,-171.111506345608));
#165324=CARTESIAN_POINT('Ctrl Pts',(48.2055749629088,-46.43000002,-171.121118099391));
#165325=CARTESIAN_POINT('Ctrl Pts',(48.2345286556579,-46.43000002,-171.128923533851));
#165326=CARTESIAN_POINT('Ctrl Pts',(48.2639285033283,-46.43000002,-171.134940493274));
#165327=CARTESIAN_POINT('Ctrl Pts',(48.2928212065519,-46.43000002,-171.140853660745));
#165328=CARTESIAN_POINT('Ctrl Pts',(48.3221462163588,-46.43000002,-171.145039422868));
#165329=CARTESIAN_POINT('Ctrl Pts',(48.35170660164,-46.43000002,-171.147466016794));
#165330=CARTESIAN_POINT('Ctrl Pts',(48.3717866301035,-46.43000002,-171.149114374034));
#165331=CARTESIAN_POINT('Ctrl Pts',(48.3919752683815,-46.43000002,-171.14995));
#165332=CARTESIAN_POINT('Ctrl Pts',(48.4122058243951,-46.43000002,-171.14995));
#165333=CARTESIAN_POINT('Origin',(47.8576079004676,-46.93000002,-170.861259130871));
#165334=CARTESIAN_POINT('Ctrl Pts',(40.8634877666247,-46.43000002,-158.96051646616));
#165335=CARTESIAN_POINT('Ctrl Pts',(40.6428186202086,-46.43000002,-159.094316247135));
#165336=CARTESIAN_POINT('Ctrl Pts',(40.5149864073608,-46.6403532458042,
-159.17182559703));
#165337=CARTESIAN_POINT('Ctrl Pts',(43.2493416424527,-46.43000002,-162.895383432653));
#165338=CARTESIAN_POINT('Ctrl Pts',(43.0357695446718,-46.4300000199999,
-163.055969456472));
#165339=CARTESIAN_POINT('Ctrl Pts',(42.8925295367156,-46.6503554345072,
-163.106696326736));
#165340=CARTESIAN_POINT('Ctrl Pts',(45.5734830336511,-46.43000002,-166.866604917879));
#165341=CARTESIAN_POINT('Ctrl Pts',(45.3499681200706,-46.4300000200635,
-167.025403443097));
#165342=CARTESIAN_POINT('Ctrl Pts',(45.2098379840441,-46.6594189992588,
-167.077916061371));
#165343=CARTESIAN_POINT('Ctrl Pts',(47.8576079004676,-46.43000002,-170.861259130871));
#165344=CARTESIAN_POINT('Ctrl Pts',(47.6152001643476,-46.4300000199999,
-170.99986675708));
#165345=CARTESIAN_POINT('Ctrl Pts',(47.4880541505298,-46.6677435098469,
-171.07256826174));
#165346=CARTESIAN_POINT('',(40.8634877666247,-46.43000002,-158.96051646616));
#165347=CARTESIAN_POINT('Ctrl Pts',(40.8634877666247,-46.43000002,-158.96051646616));
#165348=CARTESIAN_POINT('Ctrl Pts',(43.2493545263947,-46.43000002,-162.895404681481));
#165349=CARTESIAN_POINT('Ctrl Pts',(45.5734709768386,-46.43000002,-166.866583832071));
#165350=CARTESIAN_POINT('Ctrl Pts',(47.8576079004676,-46.43000002,-170.861259130871));
#165351=CARTESIAN_POINT('Origin',(40.8634877666247,-46.93000002,-158.96051646616));
#165352=CARTESIAN_POINT('Ctrl Pts',(40.5149864073608,-46.6403532458042,
-159.17182559703));
#165353=CARTESIAN_POINT('Ctrl Pts',(40.6428186202086,-46.43000002,-159.094316247135));
#165354=CARTESIAN_POINT('Ctrl Pts',(40.8634877666247,-46.43000002,-158.96051646616));
#165355=CARTESIAN_POINT('Ctrl Pts',(40.2420911121462,-46.6621010340167,
-158.751563565514));
#165356=CARTESIAN_POINT('Ctrl Pts',(40.3700931620574,-46.4300000200016,
-158.677563865504));
#165357=CARTESIAN_POINT('Ctrl Pts',(40.6178692894368,-46.43000002,-158.555430440935));
#165358=CARTESIAN_POINT('Ctrl Pts',(40.0174528618108,-46.6847857442649,
-158.313094806771));
#165359=CARTESIAN_POINT('Ctrl Pts',(40.1461325131811,-46.43000002,-158.247022454196));
#165360=CARTESIAN_POINT('Ctrl Pts',(40.4157075765897,-46.43000002,-158.132972668916));
#165361=CARTESIAN_POINT('Ctrl Pts',(39.638679212826,-46.73149352613,-157.409902189902));
#165362=CARTESIAN_POINT('Ctrl Pts',(39.7602015168115,-46.43000002,-157.36115128782));
#165363=CARTESIAN_POINT('Ctrl Pts',(40.0748112905834,-46.43000002,-157.263052526127));
#165364=CARTESIAN_POINT('Ctrl Pts',(39.4849903409058,-46.7555303756697,
-156.944912677889));
#165365=CARTESIAN_POINT('Ctrl Pts',(39.6001411399911,-46.43000002,-156.903057342463));
#165366=CARTESIAN_POINT('Ctrl Pts',(39.936491307137,-46.43000002,-156.81535457804));
#165367=CARTESIAN_POINT('Ctrl Pts',(39.1168883482047,-46.8294056411102,
-155.514886495441));
#165368=CARTESIAN_POINT('Ctrl Pts',(39.1919344928279,-46.43000002,-155.466951428797));
#165369=CARTESIAN_POINT('Ctrl Pts',(39.6051995127405,-46.43000002,-155.439088754162));
#165370=CARTESIAN_POINT('Ctrl Pts',(38.9999999999987,-46.8794682890831,
-154.544622066149));
#165371=CARTESIAN_POINT('Ctrl Pts',(39.0480945221819,-46.4300000199999,
-154.497280022653));
#165372=CARTESIAN_POINT('Ctrl Pts',(39.5000000011581,-46.43000002,-154.50605775913));
#165373=CARTESIAN_POINT('Ctrl Pts',(39.,-46.9300000200008,-153.563058845195));
#165374=CARTESIAN_POINT('Ctrl Pts',(38.9999999999992,-46.4300000199999,
-153.563058845195));
#165375=CARTESIAN_POINT('Ctrl Pts',(39.5,-46.43000002,-153.563058845195));
#165376=CARTESIAN_POINT('',(39.5,-46.43000002,-153.563058845195));
#165377=CARTESIAN_POINT('Ctrl Pts',(39.5,-46.43000002,-153.563058845195));
#165378=CARTESIAN_POINT('Ctrl Pts',(39.4999999999995,-46.43000002,-153.949465551025));
#165379=CARTESIAN_POINT('Ctrl Pts',(39.517659421908,-46.43000002,-154.333958533359));
#165380=CARTESIAN_POINT('Ctrl Pts',(39.5536573145516,-46.43000002,-154.716308049405));
#165381=CARTESIAN_POINT('Ctrl Pts',(39.5886363261002,-46.43000002,-155.087835579357));
#165382=CARTESIAN_POINT('Ctrl Pts',(39.64093030875,-46.43000002,-155.457339415578));
#165383=CARTESIAN_POINT('Ctrl Pts',(39.7112111415895,-46.43000002,-155.82460411365));
#165384=CARTESIAN_POINT('Ctrl Pts',(39.7452479661589,-46.43000002,-156.002469451805));
#165385=CARTESIAN_POINT('Ctrl Pts',(39.7835042486626,-46.43000002,-156.179809528774));
#165386=CARTESIAN_POINT('Ctrl Pts',(39.8260607087682,-46.43000002,-156.356599303471));
#165387=CARTESIAN_POINT('Ctrl Pts',(39.9364913068056,-46.43000002,-156.815354578187));
#165388=CARTESIAN_POINT('Ctrl Pts',(40.0748112905465,-46.43000002,-157.263052526106));
#165389=CARTESIAN_POINT('Ctrl Pts',(40.2452594329879,-46.43000002,-157.698012597756));
#165390=CARTESIAN_POINT('Ctrl Pts',(40.3764895639052,-46.43000002,-158.032893731271));
#165391=CARTESIAN_POINT('Ctrl Pts',(40.5265005955851,-46.43000002,-158.360328778652));
#165392=CARTESIAN_POINT('Ctrl Pts',(40.7006921181186,-46.43000002,-158.678176979737));
#165393=CARTESIAN_POINT('Ctrl Pts',(40.7527491045009,-46.43000002,-158.773165640694));
#165394=CARTESIAN_POINT('Ctrl Pts',(40.8069659798326,-46.43000002,-158.86729796943));
#165395=CARTESIAN_POINT('Ctrl Pts',(40.8634877666246,-46.43000002,-158.960516466159));
#165396=CARTESIAN_POINT('Origin',(39.5,-46.9300000199999,-153.563058845195));
#165397=CARTESIAN_POINT('Origin',(39.5,-46.93000002,-55.2499500000008));
#165398=CARTESIAN_POINT('',(39.5,-46.43000002,-78.4955841262963));
#165399=CARTESIAN_POINT('',(39.5,-46.43000002,-55.2499500000008));
#165400=CARTESIAN_POINT('Origin',(39.5,-46.93000002,-78.4955841262963));
#165401=CARTESIAN_POINT('Ctrl Pts',(39.,-46.93000002,-78.4955841262963));
#165402=CARTESIAN_POINT('Ctrl Pts',(38.9999999999999,-46.43000002,-78.4955841262962));
#165403=CARTESIAN_POINT('Ctrl Pts',(39.5,-46.43000002,-78.4955841262963));
#165404=CARTESIAN_POINT('Ctrl Pts',(39.,-46.8794362305035,-77.5133981771651));
#165405=CARTESIAN_POINT('Ctrl Pts',(39.0481232855841,-46.43000002,-77.5608042317299));
#165406=CARTESIAN_POINT('Ctrl Pts',(39.5000000013422,-46.43000002,-77.5519859229414));
#165407=CARTESIAN_POINT('Ctrl Pts',(39.1168166022506,-46.8295915161778,
-76.5473620219989));
#165408=CARTESIAN_POINT('Ctrl Pts',(39.1918385782378,-46.43000002,-76.5948804619986));
#165409=CARTESIAN_POINT('Ctrl Pts',(39.6051349405938,-46.43000002,-76.623019511696));
#165410=CARTESIAN_POINT('Ctrl Pts',(39.4815968642216,-46.7561268840582,
-75.1252733895882));
#165411=CARTESIAN_POINT('Ctrl Pts',(39.5965629951149,-46.4300000199999,
-75.1668461367765));
#165412=CARTESIAN_POINT('Ctrl Pts',(39.9334371785153,-46.43000002,-75.2543998581027));
#165413=CARTESIAN_POINT('Ctrl Pts',(39.6366096849062,-46.7317722003096,
-74.6541303933052));
#165414=CARTESIAN_POINT('Ctrl Pts',(39.7580432024793,-46.43000002,-74.70285740618));
#165415=CARTESIAN_POINT('Ctrl Pts',(40.0729487155202,-46.43000002,-74.8007807728849));
#165416=CARTESIAN_POINT('Ctrl Pts',(40.0169566636517,-46.6848236156742,
-73.7462796297709));
#165417=CARTESIAN_POINT('Ctrl Pts',(40.1456168964303,-46.4300000199999,
-73.8124084195595));
#165418=CARTESIAN_POINT('Ctrl Pts',(40.4152609981819,-46.43000002,-73.9263755541419));
#165419=CARTESIAN_POINT('Ctrl Pts',(40.242297390109,-46.662084595994,-73.3067617342949));
#165420=CARTESIAN_POINT('Ctrl Pts',(40.3703022790479,-46.4300000199999,
-73.3807595522296));
#165421=CARTESIAN_POINT('Ctrl Pts',(40.6180555307315,-46.43000002,-73.5029053716939));
#165422=CARTESIAN_POINT('Ctrl Pts',(40.5149864073608,-46.6403532458042,
-72.8868173744763));
#165423=CARTESIAN_POINT('Ctrl Pts',(40.6428186202086,-46.43000002,-72.9643267243715));
#165424=CARTESIAN_POINT('Ctrl Pts',(40.8634877666247,-46.43000002,-73.0981265053466));
#165425=CARTESIAN_POINT('',(40.8634877666247,-46.43000002,-73.0981265053466));
#165426=CARTESIAN_POINT('Ctrl Pts',(40.8634877666247,-46.43000002,-73.0981265053466));
#165427=CARTESIAN_POINT('Ctrl Pts',(40.6610441993496,-46.43000002,-73.4320063432836));
#165428=CARTESIAN_POINT('Ctrl Pts',(40.4876415800324,-46.43000002,-73.778541855119));
#165429=CARTESIAN_POINT('Ctrl Pts',(40.3370596438484,-46.43000002,-74.1350223226475));
#165430=CARTESIAN_POINT('Ctrl Pts',(40.3050640471142,-46.43000002,-74.2107671667616));
#165431=CARTESIAN_POINT('Ctrl Pts',(40.2740989238689,-46.43000002,-74.2869610781261));
#165432=CARTESIAN_POINT('Ctrl Pts',(40.2441048562922,-46.43000002,-74.3635781632946));
#165433=CARTESIAN_POINT('Ctrl Pts',(40.0729487154701,-46.43000002,-74.8007807729435));
#165434=CARTESIAN_POINT('Ctrl Pts',(39.9334371777349,-46.43000002,-75.2543998579721));
#165435=CARTESIAN_POINT('Ctrl Pts',(39.8240030986842,-46.43000002,-75.7106064091748));
#165436=CARTESIAN_POINT('Ctrl Pts',(39.7066850117826,-46.43000002,-76.1996796511065));
#165437=CARTESIAN_POINT('Ctrl Pts',(39.6220553949041,-46.43000002,-76.69344465813));
#165438=CARTESIAN_POINT('Ctrl Pts',(39.568767518,-46.43000002,-77.1917081792567));
#165439=CARTESIAN_POINT('Ctrl Pts',(39.5226417428821,-46.43000002,-77.6230031089889));
#165440=CARTESIAN_POINT('Ctrl Pts',(39.5,-46.43000002,-78.057668743091));
#165441=CARTESIAN_POINT('Ctrl Pts',(39.5,-46.43000002,-78.4955841262963));
#165442=CARTESIAN_POINT('Origin',(40.8634877666247,-46.93000002,-73.0981265053466));
#165443=CARTESIAN_POINT('Ctrl Pts',(47.7195914591242,-46.43000002,-61.4386408691297));
#165444=CARTESIAN_POINT('Ctrl Pts',(47.4775784747622,-46.43000002,-61.3001247789676));
#165445=CARTESIAN_POINT('Ctrl Pts',(47.3503956976423,-46.6672397853475,
-61.2273317382593));
#165446=CARTESIAN_POINT('Ctrl Pts',(45.4798241095785,-46.43000002,-65.3519247333759));
#165447=CARTESIAN_POINT('Ctrl Pts',(45.2561496318399,-46.43000002,-65.1939977276857));
#165448=CARTESIAN_POINT('Ctrl Pts',(45.1164556950575,-46.6590534862623,
-65.1406137191269));
#165449=CARTESIAN_POINT('Ctrl Pts',(43.2012981267977,-46.43000002,-69.2424952559608));
#165450=CARTESIAN_POINT('Ctrl Pts',(42.9872821964954,-46.43000002,-69.082946811334));
#165451=CARTESIAN_POINT('Ctrl Pts',(42.8446532485491,-46.6501540216799,
-69.0311826437503));
#165452=CARTESIAN_POINT('Ctrl Pts',(40.8634877666247,-46.43000002,-73.0981265053466));
#165453=CARTESIAN_POINT('Ctrl Pts',(40.6428186202086,-46.43000002,-72.9643267243714));
#165454=CARTESIAN_POINT('Ctrl Pts',(40.5149864073608,-46.6403532458042,
-72.8868173744763));
#165455=CARTESIAN_POINT('',(47.7195914591242,-46.43000002,-61.4386408691297));
#165456=CARTESIAN_POINT('Ctrl Pts',(47.7195914591242,-46.43000002,-61.4386408691297));
#165457=CARTESIAN_POINT('Ctrl Pts',(45.4798130845491,-46.43000002,-65.351943995909));
#165458=CARTESIAN_POINT('Ctrl Pts',(43.2013098945494,-46.43000002,-69.2424758480089));
#165459=CARTESIAN_POINT('Ctrl Pts',(40.8634877666247,-46.43000002,-73.0981265053466));
#165460=CARTESIAN_POINT('Origin',(47.7195914591242,-46.93000002,-61.4386408691297));
#165461=CARTESIAN_POINT('Ctrl Pts',(47.3503956976423,-46.6672397853475,
-61.2273317382593));
#165462=CARTESIAN_POINT('Ctrl Pts',(47.4775784747621,-46.4300000199999,
-61.3001247789676));
#165463=CARTESIAN_POINT('Ctrl Pts',(47.7195914591242,-46.43000002,-61.4386408691297));
#165464=CARTESIAN_POINT('Ctrl Pts',(47.4408676817955,-46.6931677917013,
-61.0370194599865));
#165465=CARTESIAN_POINT('Ctrl Pts',(47.5485238823607,-46.43000002,-61.1353180501949));
#165466=CARTESIAN_POINT('Ctrl Pts',(47.7740598678193,-46.43000002,-61.3434749301835));
#165467=CARTESIAN_POINT('Ctrl Pts',(47.5839744124439,-46.7341093359256,
-60.8908220076151));
#165468=CARTESIAN_POINT('Ctrl Pts',(47.6638566779936,-46.43000002,-60.997955986762));
#165469=CARTESIAN_POINT('Ctrl Pts',(47.8601584717208,-46.43000002,-61.2703860128396));
#165470=CARTESIAN_POINT('Ctrl Pts',(47.9099463828816,-46.8268793795224,
-60.6975716107228));
#165471=CARTESIAN_POINT('Ctrl Pts',(47.9370084437089,-46.4300000199999,
-60.7796218648572));
#165472=CARTESIAN_POINT('Ctrl Pts',(48.0559929527306,-46.43000002,-61.1737607963294));
#165473=CARTESIAN_POINT('Ctrl Pts',(48.0917170178641,-46.8783971335546,
-60.64995));
#165474=CARTESIAN_POINT('Ctrl Pts',(48.1007647709628,-46.43000002,-60.6990016989097));
#165475=CARTESIAN_POINT('Ctrl Pts',(48.1650685977726,-46.43000002,-61.1499500105546));
#165476=CARTESIAN_POINT('Ctrl Pts',(48.2747189347426,-46.93000002,-60.64995));
#165477=CARTESIAN_POINT('Ctrl Pts',(48.2747189347426,-46.43000002,-60.64995));
#165478=CARTESIAN_POINT('Ctrl Pts',(48.2747189347426,-46.43000002,-61.14995));
#165479=CARTESIAN_POINT('',(48.2747189347426,-46.43000002,-61.14995));
#165480=CARTESIAN_POINT('Ctrl Pts',(48.2747189347426,-46.43000002,-61.14995));
#165481=CARTESIAN_POINT('Ctrl Pts',(48.2086234136051,-46.43000002,-61.14995));
#165482=CARTESIAN_POINT('Ctrl Pts',(48.1427915915172,-46.43000002,-61.1585974051143));
#165483=CARTESIAN_POINT('Ctrl Pts',(48.0794858636046,-46.43000002,-61.1760262255644));
#165484=CARTESIAN_POINT('Ctrl Pts',(48.0376978539717,-46.43000002,-61.1875309620373));
#165485=CARTESIAN_POINT('Ctrl Pts',(47.9970101587091,-46.43000002,-61.2028630486499));
#165486=CARTESIAN_POINT('Ctrl Pts',(47.9580757097656,-46.43000002,-61.2220733995985));
#165487=CARTESIAN_POINT('Ctrl Pts',(47.9230818282114,-46.43000002,-61.2393394650997));
#165488=CARTESIAN_POINT('Ctrl Pts',(47.8896549296877,-46.43000002,-61.259737076485));
#165489=CARTESIAN_POINT('Ctrl Pts',(47.8586276391544,-46.43000002,-61.2831656716458));
#165490=CARTESIAN_POINT('Ctrl Pts',(47.8304660966178,-46.43000002,-61.3044303508315));
#165491=CARTESIAN_POINT('Ctrl Pts',(47.804280240527,-46.43000002,-61.328192714375));
#165492=CARTESIAN_POINT('Ctrl Pts',(47.7807177502453,-46.43000002,-61.3544087872415));
#165493=CARTESIAN_POINT('Ctrl Pts',(47.7576005025356,-46.43000002,-61.3801294747914));
#165494=CARTESIAN_POINT('Ctrl Pts',(47.7370072711931,-46.43000002,-61.4082122550318));
#165495=CARTESIAN_POINT('Ctrl Pts',(47.7195914591242,-46.43000002,-61.4386408691297));
#165496=CARTESIAN_POINT('',(48.2747189347426,-46.93000002,-60.64995));
#165497=CARTESIAN_POINT('Origin',(48.2747189347426,-46.93000002,-61.14995));
#165498=CARTESIAN_POINT('Ctrl Pts',(47.3503956976423,-46.6672397853475,
-61.2273317382593));
#165499=CARTESIAN_POINT('Ctrl Pts',(47.3649754155722,-46.6714181287613,
-61.1966625829204));
#165500=CARTESIAN_POINT('Ctrl Pts',(47.381438058307,-46.6761016674855,-61.166101816227));
#165501=CARTESIAN_POINT('Ctrl Pts',(47.399867274259,-46.681341395581,-61.135942748396));
#165502=CARTESIAN_POINT('Ctrl Pts',(47.4051456277002,-46.6828421179609,
-61.1273048215368));
#165503=CARTESIAN_POINT('Ctrl Pts',(47.4105849912208,-46.6843883931268,
-61.1186998973957));
#165504=CARTESIAN_POINT('Ctrl Pts',(47.4161865603661,-46.6859812459015,
-61.1101349958363));
#165505=CARTESIAN_POINT('Ctrl Pts',(47.4287662019821,-46.6895583716198,
-61.0909004939857));
#165506=CARTESIAN_POINT('Ctrl Pts',(47.4421651842185,-46.6933699882567,
-61.0718670663287));
#165507=CARTESIAN_POINT('Ctrl Pts',(47.456397415961,-46.6974246653117,-61.0531100816564));
#165508=CARTESIAN_POINT('Ctrl Pts',(47.4706296477036,-46.7014793423668,
-61.0343530969841));
#165509=CARTESIAN_POINT('Ctrl Pts',(47.4856949747266,-46.7057769703188,
-61.0158724995589));
#165510=CARTESIAN_POINT('Ctrl Pts',(47.5016056905473,-46.710324966154,-60.9977415259233));
#165511=CARTESIAN_POINT('Ctrl Pts',(47.5239116638849,-46.7167010132775,
-60.9723228697762));
#165512=CARTESIAN_POINT('Ctrl Pts',(47.5478688873049,-46.7235628876405,
-60.9476070723277));
#165513=CARTESIAN_POINT('Ctrl Pts',(47.5734743527693,-46.730899683852,-60.9238278542592));
#165514=CARTESIAN_POINT('Ctrl Pts',(47.5843973344877,-46.7340294723341,
-60.9136839275807));
#165515=CARTESIAN_POINT('Ctrl Pts',(47.5956197393021,-46.7372455183854,
-60.9037107396086));
#165516=CARTESIAN_POINT('Ctrl Pts',(47.6071388613982,-46.7405461742288,
-60.893927797046));
#165517=CARTESIAN_POINT('Ctrl Pts',(47.6263998861775,-46.7460651724177,
-60.8775698231016));
#165518=CARTESIAN_POINT('Ctrl Pts',(47.6464923548891,-46.7518206541896,
-60.8617425255592));
#165519=CARTESIAN_POINT('Ctrl Pts',(47.6674021178734,-46.7578004809242,
-60.8465384000143));
#165520=CARTESIAN_POINT('Ctrl Pts',(47.6778569993656,-46.7607903942915,
-60.8389363372419));
#165521=CARTESIAN_POINT('Ctrl Pts',(47.6885162039648,-46.7638363936609,
-60.8314900530784));
#165522=CARTESIAN_POINT('Ctrl Pts',(47.6993772512914,-46.7669364419737,
-60.8242117420372));
#165523=CARTESIAN_POINT('Ctrl Pts',(47.7048077749548,-46.7684864661302,
-60.8205725865165));
#165524=CARTESIAN_POINT('Ctrl Pts',(47.7102887588547,-46.770050002197,-60.8169754248191));
#165525=CARTESIAN_POINT('Ctrl Pts',(47.7158198685113,-46.7716267778854,
-60.813421808391));
#165526=CARTESIAN_POINT('Ctrl Pts',(47.7193727027062,-46.7726395986269,
-60.8111391904815));
#165527=CARTESIAN_POINT('Ctrl Pts',(47.7234224734296,-46.7737934320202,
-60.8085741529328));
#165528=CARTESIAN_POINT('Ctrl Pts',(47.7270524255314,-46.7748272671279,
-60.8063084769865));
#165529=CARTESIAN_POINT('Ctrl Pts',(47.7290736414891,-46.7754029232134,
-60.8050469120267));
#165530=CARTESIAN_POINT('Ctrl Pts',(47.7309642340686,-46.7759412474452,
-60.8038771214381));
#165531=CARTESIAN_POINT('Ctrl Pts',(47.732563241915,-46.7763964389912,-60.8028931958203));
#165532=CARTESIAN_POINT('Ctrl Pts',(47.7372961730498,-46.7777437683652,
-60.7999808572715));
#165533=CARTESIAN_POINT('Ctrl Pts',(47.7420952026095,-46.7791092300362,
-60.7970812943398));
#165534=CARTESIAN_POINT('Ctrl Pts',(47.7469605871675,-46.7804929909258,
-60.7941971932464));
#165535=CARTESIAN_POINT('Ctrl Pts',(47.772543208461,-46.7877689277767,-60.7790323352242));
#165536=CARTESIAN_POINT('Ctrl Pts',(47.7999356062372,-46.7955435956083,
-60.7642777177594));
#165537=CARTESIAN_POINT('Ctrl Pts',(47.8292061473077,-46.8038519743165,
-60.7503187372695));
#165538=CARTESIAN_POINT('Ctrl Pts',(47.8364355740346,-46.8059040311933,
-60.7468710583765));
#165539=CARTESIAN_POINT('Ctrl Pts',(47.8437794265727,-46.8079886144811,
-60.7434721114416));
#165540=CARTESIAN_POINT('Ctrl Pts',(47.8512384246683,-46.8101061839473,
-60.740128093106));
#165541=CARTESIAN_POINT('Ctrl Pts',(47.8729397082559,-46.8162670617104,
-60.730398972748));
#165542=CARTESIAN_POINT('Ctrl Pts',(47.8956133919344,-46.8227056078164,
-60.7211360160641));
#165543=CARTESIAN_POINT('Ctrl Pts',(47.9192598675699,-46.8294193228067,
-60.7125029350349));
#165544=CARTESIAN_POINT('Ctrl Pts',(47.9310831053876,-46.8327761803018,
-60.7081863945204));
#165545=CARTESIAN_POINT('Ctrl Pts',(47.9431492874975,-46.8362016470855,
-60.7040274877552));
#165546=CARTESIAN_POINT('Ctrl Pts',(47.9554568133423,-46.8396942255108,
-60.7000475267255));
#165547=CARTESIAN_POINT('Ctrl Pts',(47.9616105762647,-46.8414405147234,
-60.6980575462106));
#165548=CARTESIAN_POINT('Ctrl Pts',(47.9678246742073,-46.8432035812128,
-60.6961123029493));
#165549=CARTESIAN_POINT('Ctrl Pts',(47.9740987753576,-46.8449831434372,
-60.6942145099447));
#165550=CARTESIAN_POINT('Ctrl Pts',(47.9772358259328,-46.8458729245494,
-60.6932656134423));
#165551=CARTESIAN_POINT('Ctrl Pts',(47.980387877244,-46.8467668295495,-60.6923285794147));
#165552=CARTESIAN_POINT('Ctrl Pts',(47.9835548832028,-46.8476648199627,
-60.6914037480275));
#165553=CARTESIAN_POINT('Ctrl Pts',(47.9859651476109,-46.8483482396846,
-60.6906999008591));
#165554=CARTESIAN_POINT('Ctrl Pts',(47.9892214896772,-46.8492713977441,
-60.6897640113346));
#165555=CARTESIAN_POINT('Ctrl Pts',(47.991412150968,-46.8498923749228,-60.6891431809423));
#165556=CARTESIAN_POINT('Ctrl Pts',(47.992099944563,-46.8500873407662,-60.6889482611849));
#165557=CARTESIAN_POINT('Ctrl Pts',(47.9926825870611,-46.8502524924943,
-60.6887839277128));
#165558=CARTESIAN_POINT('Ctrl Pts',(47.9931007164342,-46.8503710071843,
-60.6886662023885));
#165559=CARTESIAN_POINT('Ctrl Pts',(48.0053033073781,-46.8538297124931,
-60.6852305337442));
#165560=CARTESIAN_POINT('Ctrl Pts',(48.0192692831386,-46.8577875919822,
-60.6815376280838));
#165561=CARTESIAN_POINT('Ctrl Pts',(48.0350282325568,-46.8622516984632,
-60.6778086356672));
#165562=CARTESIAN_POINT('Ctrl Pts',(48.0507543703039,-46.8667065102387,
-60.6740874073769));
#165563=CARTESIAN_POINT('Ctrl Pts',(48.0682665960331,-46.871665608229,-60.6703303471326));
#165564=CARTESIAN_POINT('Ctrl Pts',(48.0875881985635,-46.8771339372435,
-60.6668083564069));
#165565=CARTESIAN_POINT('Ctrl Pts',(48.1067263400268,-46.8825503437803,
-60.6633198074299));
#165566=CARTESIAN_POINT('Ctrl Pts',(48.1276403019889,-46.8884665410566,
-60.6600620547269));
#165567=CARTESIAN_POINT('Ctrl Pts',(48.1503376798541,-46.8948827095381,
-60.6573464342638));
#165568=CARTESIAN_POINT('Ctrl Pts',(48.17240731422,-46.9011214254487,-60.6547059199695));
#165569=CARTESIAN_POINT('Ctrl Pts',(48.1961636602219,-46.9078330051241,
-60.6525782551135));
#165570=CARTESIAN_POINT('Ctrl Pts',(48.2215905577363,-46.9150106839736,
-60.6512917365203));
#165571=CARTESIAN_POINT('Ctrl Pts',(48.238560647475,-46.91980111718,-60.6504331049879));
#165572=CARTESIAN_POINT('Ctrl Pts',(48.2562743795194,-46.9247990237211,
-60.64995));
#165573=CARTESIAN_POINT('Ctrl Pts',(48.2747189347426,-46.93000002,-60.64995));
#165574=CARTESIAN_POINT('Origin',(-83.2809572255632,-46.9300000199999,-61.14995));
#165575=CARTESIAN_POINT('',(51.1565772669927,-46.43000002,-61.14995));
#165576=CARTESIAN_POINT('',(-83.2809572255632,-46.4300000199999,-61.14995));
#165577=CARTESIAN_POINT('',(51.1565772669927,-46.93000002,-60.64995));
#165578=CARTESIAN_POINT('Origin',(51.1565772669927,-46.93000002,-61.14995));
#165579=CARTESIAN_POINT('',(-1.41965171211599E-14,-46.93000002,-60.64995));
#165580=CARTESIAN_POINT('Origin',(0.,-12.9675000200281,-61.64995));
#165581=CARTESIAN_POINT('',(43.7578534463097,-52.58000002,-60.64995));
#165582=CARTESIAN_POINT('Origin',(0.,-12.9675000200281,-60.64995));
#165583=CARTESIAN_POINT('Ctrl Pts',(43.7578534463096,-52.58000002,-60.64995));
#165584=CARTESIAN_POINT('Ctrl Pts',(43.7326047098007,-52.5718933448815,
-60.64995));
#165585=CARTESIAN_POINT('Ctrl Pts',(43.7087430193938,-52.5642265504434,
-60.6508231664889));
#165586=CARTESIAN_POINT('Ctrl Pts',(43.6862857190865,-52.5570071197507,
-60.6522980719393));
#165587=CARTESIAN_POINT('Ctrl Pts',(43.6788113190536,-52.5546042969595,
-60.6527889605678));
#165588=CARTESIAN_POINT('Ctrl Pts',(43.6714922008008,-52.5522509345212,
-60.6533468213481));
#165589=CARTESIAN_POINT('Ctrl Pts',(43.6643282149358,-52.5499470452909,
-60.6539625815365));
#165590=CARTESIAN_POINT('Ctrl Pts',(43.6417273860358,-52.5426787721148,
-60.6559051720056));
#165591=CARTESIAN_POINT('Ctrl Pts',(43.6206746206964,-52.5359042274634,
-60.658421247948));
#165592=CARTESIAN_POINT('Ctrl Pts',(43.6011861995931,-52.5296303175985,
-60.66124704236));
#165593=CARTESIAN_POINT('Ctrl Pts',(43.5812552623538,-52.523213948458,-60.6641370010067));
#165594=CARTESIAN_POINT('Ctrl Pts',(43.5629639926385,-52.5173223267036,
-60.6673497529415));
#165595=CARTESIAN_POINT('Ctrl Pts',(43.5462866787648,-52.5119486088649,
-60.6706467221525));
#165596=CARTESIAN_POINT('Ctrl Pts',(43.5285676330368,-52.5062392270762,
-60.6741496332721));
#165597=CARTESIAN_POINT('Ctrl Pts',(43.5126732014012,-52.5011153502927,
-60.6777467267745));
#165598=CARTESIAN_POINT('Ctrl Pts',(43.4985738697311,-52.496568816543,-60.681200460083));
#165599=CARTESIAN_POINT('Ctrl Pts',(43.493624271658,-52.4949727469411,-60.6824128999439));
#165600=CARTESIAN_POINT('Ctrl Pts',(43.4888958518418,-52.4934478097891,
-60.6836081329837));
#165601=CARTESIAN_POINT('Ctrl Pts',(43.4843871673709,-52.4919935882829,
-60.6847773996288));
#165602=CARTESIAN_POINT('Ctrl Pts',(43.4825117041136,-52.4913886803502,
-60.6852637757869));
#165603=CARTESIAN_POINT('Ctrl Pts',(43.480674260163,-52.490796007527,-60.6857456694553));
#165604=CARTESIAN_POINT('Ctrl Pts',(43.478874708603,-52.4902161677162,-60.6862223751517));
#165605=CARTESIAN_POINT('Ctrl Pts',(43.4774063456389,-52.4897430413429,
-60.686611348163));
#165606=CARTESIAN_POINT('Ctrl Pts',(43.4769880700405,-52.4896084617891,
-60.6867221277077));
#165607=CARTESIAN_POINT('Ctrl Pts',(43.4751110601863,-52.4890030432867,
-60.6872267061947));
#165608=CARTESIAN_POINT('Ctrl Pts',(43.4746877014711,-52.48886649142,-60.687340513642));
#165609=CARTESIAN_POINT('Ctrl Pts',(43.4741901615202,-52.4887059950551,
-60.6874745159787));
#165610=CARTESIAN_POINT('Ctrl Pts',(43.4735897327294,-52.4885122903053,
-60.6876368692356));
#165611=CARTESIAN_POINT('Ctrl Pts',(43.440872946168,-52.4779575050367,-60.6964833418455));
#165612=CARTESIAN_POINT('Ctrl Pts',(43.4096715539944,-52.4678833667465,
-60.7065709859225));
#165613=CARTESIAN_POINT('Ctrl Pts',(43.3800156571783,-52.4583018043552,
-60.717578197336));
#165614=CARTESIAN_POINT('Ctrl Pts',(43.3623552478449,-52.4525958796639,
-60.724133111537));
#165615=CARTESIAN_POINT('Ctrl Pts',(43.3452419651281,-52.4470643237979,
-60.7310145708574));
#165616=CARTESIAN_POINT('Ctrl Pts',(43.328674854676,-52.4417072470008,-60.7381585903407));
#165617=CARTESIAN_POINT('Ctrl Pts',(43.3085530794791,-52.4352007475521,
-60.7468354416517));
#165618=CARTESIAN_POINT('Ctrl Pts',(43.2892379670008,-52.428951803686,-60.7558991768847));
#165619=CARTESIAN_POINT('Ctrl Pts',(43.270721116452,-52.422958340144,-60.7652397187937));
#165620=CARTESIAN_POINT('Ctrl Pts',(43.2585405932486,-52.4190157948634,
-60.7713839973336));
#165621=CARTESIAN_POINT('Ctrl Pts',(43.2467055435055,-52.4151838158481,
-60.7776480399122));
#165622=CARTESIAN_POINT('Ctrl Pts',(43.2352112538791,-52.4114610468223,
-60.7840021349292));
#165623=CARTESIAN_POINT('Ctrl Pts',(43.2322460380483,-52.4105006731057,
-60.7856413195806));
#165624=CARTESIAN_POINT('Ctrl Pts',(43.2293030096678,-52.4095474084892,
-60.7872867762851));
#165625=CARTESIAN_POINT('Ctrl Pts',(43.2263834511929,-52.4086016712105,
-60.7889372301596));
#165626=CARTESIAN_POINT('Ctrl Pts',(43.224616894102,-52.408029427527,-60.7899358815037));
#165627=CARTESIAN_POINT('Ctrl Pts',(43.2228583502841,-52.4074597533364,
-60.7909367527273));
#165628=CARTESIAN_POINT('Ctrl Pts',(43.2211081357598,-52.4068927518434,
-60.7919395425494));
#165629=CARTESIAN_POINT('Ctrl Pts',(43.218074199461,-52.4059098743805,-60.793677843997));
#165630=CARTESIAN_POINT('Ctrl Pts',(43.2155965839684,-52.4051071765678,
-60.7951131541398));
#165631=CARTESIAN_POINT('Ctrl Pts',(43.2126453552502,-52.4041510156181,
-60.7968407012197));
#165632=CARTESIAN_POINT('Ctrl Pts',(43.2110245994186,-52.4036259111334,
-60.7977894355509));
#165633=CARTESIAN_POINT('Ctrl Pts',(43.2092611714391,-52.4030545742235,
-60.7988269575869));
#165634=CARTESIAN_POINT('Ctrl Pts',(43.2071863268825,-52.4023823129085,
-60.8000583398207));
#165635=CARTESIAN_POINT('Ctrl Pts',(43.1791498868442,-52.393298348528,-60.8166974533641));
#165636=CARTESIAN_POINT('Ctrl Pts',(43.1522144188923,-52.3845643830934,
-60.8344485377384));
#165637=CARTESIAN_POINT('Ctrl Pts',(43.1264895714976,-52.3762177436116,
-60.8531177508924));
#165638=CARTESIAN_POINT('Ctrl Pts',(43.0995702971012,-52.3674835624112,
-60.8726537918239));
#165639=CARTESIAN_POINT('Ctrl Pts',(43.0739765262997,-52.359173462109,-60.8931951091248));
#165640=CARTESIAN_POINT('Ctrl Pts',(43.0497792324109,-52.3513121589382,
-60.9145307982532));
#165641=CARTESIAN_POINT('Ctrl Pts',(43.0298661553644,-52.3448427274206,
-60.9320889278279));
#165642=CARTESIAN_POINT('Ctrl Pts',(43.0108976759893,-52.338676858853,-60.9501852458894));
#165643=CARTESIAN_POINT('Ctrl Pts',(42.9928889905782,-52.3328202776169,
-60.9687080860286));
#165644=CARTESIAN_POINT('Ctrl Pts',(42.9682605971059,-52.3248109097041,
-60.9940396293788));
#165645=CARTESIAN_POINT('Ctrl Pts',(42.9455081131276,-52.3174064822144,
-61.0199852010191));
#165646=CARTESIAN_POINT('Ctrl Pts',(42.9245492686285,-52.3105824389046,
-61.0464447313357));
#165647=CARTESIAN_POINT('Ctrl Pts',(42.9014578882856,-52.3030640578437,
-61.0755964853009));
#165648=CARTESIAN_POINT('Ctrl Pts',(42.8805436006627,-52.2962501412606,
-61.1053719350892));
#165649=CARTESIAN_POINT('Ctrl Pts',(42.8616512181442,-52.2900924335603,
-61.1355876054117));
#165650=CARTESIAN_POINT('Ctrl Pts',(42.8427588356257,-52.2839347258599,
-61.1658032757343));
#165651=CARTESIAN_POINT('Ctrl Pts',(42.8258875244576,-52.2784329474316,
-61.1964582058417));
#165652=CARTESIAN_POINT('Ctrl Pts',(42.8108476403352,-52.2735270043159,
-61.2273317382593));
#165653=CARTESIAN_POINT('Origin',(57.,-53.58000002,-174.34995));
#165654=CARTESIAN_POINT('',(57.,-53.08000002,-176.84995));
#165655=CARTESIAN_POINT('Origin',(57.,-53.58000002,-176.84995));
#165656=CARTESIAN_POINT('',(59.5,-53.08000002,-174.34995));
#165657=CARTESIAN_POINT('Origin',(57.,-53.08000002,-174.34995));
#165658=CARTESIAN_POINT('Origin',(59.5,-53.58000002,-174.34995));
#165659=CARTESIAN_POINT('Origin',(59.5,-53.58000002,-55.2499500000008));
#165660=CARTESIAN_POINT('',(59.5,-53.08000002,-58.24995));
#165661=CARTESIAN_POINT('',(59.5,-53.08000002,-174.34995));
#165662=CARTESIAN_POINT('Origin',(59.5,-53.58000002,-58.24995));
#165663=CARTESIAN_POINT('Origin',(-1.65582490824295E-14,-52.58000002,-61.14995));
#165664=CARTESIAN_POINT('',(50.6622663180714,-52.58000002,-60.64995));
#165665=CARTESIAN_POINT('',(50.6622663180714,-53.08000002,-61.14995));
#165666=CARTESIAN_POINT('Origin',(50.6622663180714,-52.58000002,-61.14995));
#165667=CARTESIAN_POINT('',(43.7578534463097,-53.08000002,-61.14995));
#165668=CARTESIAN_POINT('',(-83.2809572255632,-53.0800000199999,-61.14995));
#165669=CARTESIAN_POINT('Origin',(43.7578534463097,-52.58000002,-61.14995));
#165670=CARTESIAN_POINT('',(-1.65582490824295E-14,-52.58000002,-60.64995));
#165671=CARTESIAN_POINT('Ctrl Pts',(43.7578534463097,-52.58000002,-60.64995));
#165672=CARTESIAN_POINT('Ctrl Pts',(43.7578534463096,-53.0800000199999,
-60.64995));
#165673=CARTESIAN_POINT('Ctrl Pts',(43.7578534463097,-53.08000002,-61.14995));
#165674=CARTESIAN_POINT('Ctrl Pts',(43.5763740160895,-52.5217319642193,
-60.64995));
#165675=CARTESIAN_POINT('Ctrl Pts',(43.5651337625656,-53.08000002,-60.5880729855648));
#165676=CARTESIAN_POINT('Ctrl Pts',(43.6407450400032,-53.08000002,-61.1499500212049));
#165677=CARTESIAN_POINT('Ctrl Pts',(43.3921532801741,-52.4622997588847,
-60.6952259861921));
#165678=CARTESIAN_POINT('Ctrl Pts',(43.3529851647999,-53.0800000199999,
-60.5541186415154));
#165679=CARTESIAN_POINT('Ctrl Pts',(43.5216142225441,-53.08000002,-61.1725879738646));
#165680=CARTESIAN_POINT('Ctrl Pts',(43.1434985367023,-52.3817526273734,
-60.8357928521433));
#165681=CARTESIAN_POINT('Ctrl Pts',(43.0017618884342,-53.08000002,-60.5701748148313));
#165682=CARTESIAN_POINT('Ctrl Pts',(43.3605400154948,-53.08000002,-61.2428714356874));
#165683=CARTESIAN_POINT('Ctrl Pts',(43.0639517713831,-52.3559271119108,
-60.8956186757958));
#165684=CARTESIAN_POINT('Ctrl Pts',(42.8669014498658,-53.0800000199996,
-60.5905012094869));
#165685=CARTESIAN_POINT('Ctrl Pts',(43.3089610591665,-53.08000002,-61.2727843293231));
#165686=CARTESIAN_POINT('Ctrl Pts',(42.9218280041301,-52.3097083637374,
-61.0417997602761));
#165687=CARTESIAN_POINT('Ctrl Pts',(42.577778492926,-53.0800000200004,-60.6851892310921));
#165688=CARTESIAN_POINT('Ctrl Pts',(43.2167397054761,-53.08000002,-61.3458748887128));
#165689=CARTESIAN_POINT('Ctrl Pts',(42.8599235980017,-52.2895352828276,
-61.126589843371));
#165690=CARTESIAN_POINT('Ctrl Pts',(42.4244093202802,-53.0800000199984,
-60.7623557509217));
#165691=CARTESIAN_POINT('Ctrl Pts',(43.1765485703954,-53.08000002,-61.3882486178711));
#165692=CARTESIAN_POINT('Ctrl Pts',(42.8108476403352,-52.2735270043159,
-61.2273317382593));
#165693=CARTESIAN_POINT('Ctrl Pts',(42.2822348911901,-53.08000002,-60.8926985768511));
#165694=CARTESIAN_POINT('Ctrl Pts',(43.1446480925044,-53.08000002,-61.4386408691297));
#165695=CARTESIAN_POINT('',(43.1446480925044,-53.08000002,-61.4386408691297));
#165696=CARTESIAN_POINT('Ctrl Pts',(43.1446480925044,-53.08000002,-61.4386408691297));
#165697=CARTESIAN_POINT('Ctrl Pts',(43.1765609373872,-53.08000002,-61.3882288400421));
#165698=CARTESIAN_POINT('Ctrl Pts',(43.2167516388878,-53.08000002,-61.3458652617053));
#165699=CARTESIAN_POINT('Ctrl Pts',(43.2628503174202,-53.08000002,-61.3093295271296));
#165700=CARTESIAN_POINT('Ctrl Pts',(43.3089610210815,-53.08000002,-61.2727842619789));
#165701=CARTESIAN_POINT('Ctrl Pts',(43.3605330051287,-53.08000002,-61.2428744748387));
#165702=CARTESIAN_POINT('Ctrl Pts',(43.414231413078,-53.08000002,-61.2194436041558));
#165703=CARTESIAN_POINT('Ctrl Pts',(43.4456262415641,-53.08000002,-61.205744721927));
#165704=CARTESIAN_POINT('Ctrl Pts',(43.477917759742,-53.08000002,-61.1941576093824));
#165705=CARTESIAN_POINT('Ctrl Pts',(43.5108494925037,-53.08000002,-61.1845858141908));
#165706=CARTESIAN_POINT('Ctrl Pts',(43.5447058226299,-53.08000002,-61.1747452795231));
#165707=CARTESIAN_POINT('Ctrl Pts',(43.5792402145377,-53.08000002,-61.1670347524206));
#165708=CARTESIAN_POINT('Ctrl Pts',(43.6141927055654,-53.08000002,-61.1614020099222));
#165709=CARTESIAN_POINT('Ctrl Pts',(43.648904945801,-53.08000002,-61.1558079848602));
#165710=CARTESIAN_POINT('Ctrl Pts',(43.6840310643504,-53.08000002,-61.1522634649487));
#165711=CARTESIAN_POINT('Ctrl Pts',(43.719312634701,-53.08000002,-61.1507670586125));
#165712=CARTESIAN_POINT('Ctrl Pts',(43.7321435462895,-53.08000002,-61.1502228578524));
#165713=CARTESIAN_POINT('Ctrl Pts',(43.7449948697402,-53.08000002,-61.14995));
#165714=CARTESIAN_POINT('Ctrl Pts',(43.7578534463097,-53.08000002,-61.14995));
#165715=CARTESIAN_POINT('Origin',(43.1446480925044,-52.58000002,-61.4386408691297));
#165716=CARTESIAN_POINT('Ctrl Pts',(41.0647116264215,-53.08000002,-64.6870793282409));
#165717=CARTESIAN_POINT('Ctrl Pts',(40.1851006581956,-53.08000002,-64.1171767326871));
#165718=CARTESIAN_POINT('Ctrl Pts',(40.7385684738022,-52.2653905871942,
-64.4757701973706));
#165719=CARTESIAN_POINT('Ctrl Pts',(41.7638515954828,-53.08000002,-63.6079981134234));
#165720=CARTESIAN_POINT('Ctrl Pts',(40.8849497704992,-53.0800000200001,
-63.0545757298723));
#165721=CARTESIAN_POINT('Ctrl Pts',(41.4350320326697,-52.2681651349568,
-63.3966889540178));
#165722=CARTESIAN_POINT('Ctrl Pts',(42.4569204735311,-53.08000002,-62.5250292766735));
#165723=CARTESIAN_POINT('Ctrl Pts',(41.584202382955,-53.08000002,-61.9790488279059));
#165724=CARTESIAN_POINT('Ctrl Pts',(42.125553749702,-52.2708762823431,-62.3137201227713));
#165725=CARTESIAN_POINT('Ctrl Pts',(43.1446480925044,-53.08000002,-61.4386408691297));
#165726=CARTESIAN_POINT('Ctrl Pts',(42.2822348911901,-53.08000002,-60.8926985768511));
#165727=CARTESIAN_POINT('Ctrl Pts',(42.8108476403353,-52.2735270043159,
-61.2273317382593));
#165728=CARTESIAN_POINT('',(41.0647116264214,-53.08000002,-64.687079328241));
#165729=CARTESIAN_POINT('Ctrl Pts',(41.0647116264215,-53.08000002,-64.6870793282409));
#165730=CARTESIAN_POINT('Ctrl Pts',(41.7638515954828,-53.08000002,-63.6079981134234));
#165731=CARTESIAN_POINT('Ctrl Pts',(42.4569204735311,-53.08000002,-62.5250292766735));
#165732=CARTESIAN_POINT('Ctrl Pts',(43.1446480925044,-53.08000002,-61.4386408691297));
#165733=CARTESIAN_POINT('Origin',(41.0647116264214,-52.58000002,-64.687079328241));
#165734=CARTESIAN_POINT('Ctrl Pts',(40.7385684738017,-52.2653905871946,
-64.4757701973708));
#165735=CARTESIAN_POINT('Ctrl Pts',(40.1851006581961,-53.08000002,-64.117176732689));
#165736=CARTESIAN_POINT('Ctrl Pts',(41.0647116264215,-53.08000002,-64.6870793282409));
#165737=CARTESIAN_POINT('Ctrl Pts',(40.4169533529343,-52.2886158160728,
-64.9375850416414));
#165738=CARTESIAN_POINT('Ctrl Pts',(39.9350648871364,-53.08000002,-64.6424135397739));
#165739=CARTESIAN_POINT('Ctrl Pts',(40.7752331041961,-53.08000002,-65.1338723319862));
#165740=CARTESIAN_POINT('Ctrl Pts',(40.1571532317284,-52.3131117923589,
-65.4245685478069));
#165741=CARTESIAN_POINT('Ctrl Pts',(39.7292916509907,-53.0800000199999,
-65.1967116799));
#165742=CARTESIAN_POINT('Ctrl Pts',(40.5414379096314,-53.08000002,-65.6048227505322));
#165743=CARTESIAN_POINT('Ctrl Pts',(39.8302312493672,-52.3511206237746,
-66.1800801057477));
#165744=CARTESIAN_POINT('Ctrl Pts',(39.4809642231373,-53.0800000199999,
-66.0439398517176));
#165745=CARTESIAN_POINT('Ctrl Pts',(40.2472081238925,-53.08000002,-66.3353006309098));
#165746=CARTESIAN_POINT('Ctrl Pts',(39.7320550320644,-52.3640100073116,
-66.4362687474843));
#165747=CARTESIAN_POINT('Ctrl Pts',(39.4096807156913,-53.08000002,-66.3196295939567));
#165748=CARTESIAN_POINT('Ctrl Pts',(40.158849529204,-53.08000002,-66.5829654036754));
#165749=CARTESIAN_POINT('Ctrl Pts',(39.5550747922058,-52.3901835262345,
-66.9564695443705));
#165750=CARTESIAN_POINT('Ctrl Pts',(39.2851434780251,-53.0800000199999,
-66.8724334008892));
#165751=CARTESIAN_POINT('Ctrl Pts',(39.9995673126391,-53.08000002,-67.0857801567948));
#165752=CARTESIAN_POINT('Ctrl Pts',(39.4760999841222,-52.4035086843654,
-67.2212970006122));
#165753=CARTESIAN_POINT('Ctrl Pts',(39.2309126715885,-53.08000002,-67.1508200729254));
#165754=CARTESIAN_POINT('Ctrl Pts',(39.9284899861158,-53.08000002,-67.341717845364));
#165755=CARTESIAN_POINT('Ctrl Pts',(39.2683842506574,-52.4436252670713,
-68.0185730582879));
#165756=CARTESIAN_POINT('Ctrl Pts',(39.096874254798,-53.08000002,-67.9652916099918));
#165757=CARTESIAN_POINT('Ctrl Pts',(39.7415458247801,-53.08000002,-68.1121058873989));
#165758=CARTESIAN_POINT('Ctrl Pts',(39.1678647718912,-52.4706085083894,
-68.5548226317846));
#165759=CARTESIAN_POINT('Ctrl Pts',(39.0356546500978,-53.08000002,-68.5171438238431));
#165760=CARTESIAN_POINT('Ctrl Pts',(39.6510782949347,-53.08000002,-68.6301060216833));
#165761=CARTESIAN_POINT('Ctrl Pts',(39.0336224576287,-52.5249919887119,
-69.6357261726145));
#165762=CARTESIAN_POINT('Ctrl Pts',(38.9750254916822,-53.0800000199999,
-69.6153526806455));
#165763=CARTESIAN_POINT('Ctrl Pts',(39.5302602116332,-53.08000002,-69.6738635266831));
#165764=CARTESIAN_POINT('Ctrl Pts',(39.,-52.5523936264783,-70.1804078085674));
#165765=CARTESIAN_POINT('Ctrl Pts',(38.9716079589828,-53.0800000199999,
-70.1647867514408));
#165766=CARTESIAN_POINT('Ctrl Pts',(39.500000000531,-53.08000002,-70.1996476853715));
#165767=CARTESIAN_POINT('Ctrl Pts',(39.,-52.58000002,-70.7293062304687));
#165768=CARTESIAN_POINT('Ctrl Pts',(38.9999999999999,-53.08000002,-70.7293062304687));
#165769=CARTESIAN_POINT('Ctrl Pts',(39.5,-53.08000002,-70.7293062304687));
#165770=CARTESIAN_POINT('',(39.5,-53.08000002,-70.7293062304687));
#165771=CARTESIAN_POINT('Ctrl Pts',(39.5,-53.08000002,-70.7293062304687));
#165772=CARTESIAN_POINT('Ctrl Pts',(39.5,-53.08000002,-70.1996325547074));
#165773=CARTESIAN_POINT('Ctrl Pts',(39.5302602116353,-53.08000002,-69.6738635266889));
#165774=CARTESIAN_POINT('Ctrl Pts',(39.5906692531643,-53.08000002,-69.1519847741694));
#165775=CARTESIAN_POINT('Ctrl Pts',(39.6510782946932,-53.08000002,-68.6301060216499));
#165776=CARTESIAN_POINT('Ctrl Pts',(39.7415458248093,-53.08000002,-68.1121058873188));
#165777=CARTESIAN_POINT('Ctrl Pts',(39.8661752652165,-53.08000002,-67.5985138592655));
#165778=CARTESIAN_POINT('Ctrl Pts',(39.9284899854243,-53.08000002,-67.3417178452216));
#165779=CARTESIAN_POINT('Ctrl Pts',(39.9995673120589,-53.08000002,-67.0857801566515));
#165780=CARTESIAN_POINT('Ctrl Pts',(40.0792084204325,-53.08000002,-66.8343727800802));
#165781=CARTESIAN_POINT('Ctrl Pts',(40.1588495287955,-53.08000002,-66.5829654035428));
#165782=CARTESIAN_POINT('Ctrl Pts',(40.2472081235396,-53.08000002,-66.3353006307905));
#165783=CARTESIAN_POINT('Ctrl Pts',(40.3452847184367,-53.08000002,-66.0918080038346));
#165784=CARTESIAN_POINT('Ctrl Pts',(40.4725149961137,-53.08000002,-65.7759361633367));
#165785=CARTESIAN_POINT('Ctrl Pts',(40.6155606032197,-53.08000002,-65.4668542003479));
#165786=CARTESIAN_POINT('Ctrl Pts',(40.7793840759628,-53.08000002,-65.1666925984976));
#165787=CARTESIAN_POINT('Ctrl Pts',(40.868130174949,-53.08000002,-65.0040897017112));
#165788=CARTESIAN_POINT('Ctrl Pts',(40.9629743342362,-53.08000002,-64.8441048248465));
#165789=CARTESIAN_POINT('Ctrl Pts',(41.0647116264214,-53.08000002,-64.687079328241));
#165790=CARTESIAN_POINT('Origin',(39.5,-52.58000002,-70.7293062304687));
#165791=CARTESIAN_POINT('Origin',(39.5,-52.58000002,-55.2499500000008));
#165792=CARTESIAN_POINT('',(39.5,-53.08000002,-161.329336741015));
#165793=CARTESIAN_POINT('',(39.5,-53.08000002,-55.2499500000008));
#165794=CARTESIAN_POINT('Origin',(39.5,-52.58000002,-161.329336741016));
#165795=CARTESIAN_POINT('Ctrl Pts',(39.,-52.5800000200011,-161.329336741014));
#165796=CARTESIAN_POINT('Ctrl Pts',(39.0000000000011,-53.08000002,-161.329336741014));
#165797=CARTESIAN_POINT('Ctrl Pts',(39.5,-53.08000002,-161.329336741015));
#165798=CARTESIAN_POINT('Ctrl Pts',(38.999999999999,-52.5523928630554,-161.878250342061));
#165799=CARTESIAN_POINT('Ctrl Pts',(38.971607175397,-53.08000002,-161.893871800581));
#165800=CARTESIAN_POINT('Ctrl Pts',(39.5000000005568,-53.08000002,-161.859009936371));
#165801=CARTESIAN_POINT('Ctrl Pts',(39.0336246233085,-52.5250040247996,
-162.422677519451));
#165802=CARTESIAN_POINT('Ctrl Pts',(38.9750364187576,-53.08000002,-162.443018289978));
#165803=CARTESIAN_POINT('Ctrl Pts',(39.5302621607567,-53.08000002,-162.384548554576));
#165804=CARTESIAN_POINT('Ctrl Pts',(39.1676758409912,-52.4706721515367,
-163.50255544994));
#165805=CARTESIAN_POINT('Ctrl Pts',(39.0355537948544,-53.0800000199999,
-163.540173111977));
#165806=CARTESIAN_POINT('Ctrl Pts',(39.650908257113,-53.08000002,-163.427315362947));
#165807=CARTESIAN_POINT('Ctrl Pts',(39.2680076006075,-52.4437276611465,
-164.038034987594));
#165808=CARTESIAN_POINT('Ctrl Pts',(39.0966358008681,-53.08000002,-164.091177104404));
#165809=CARTESIAN_POINT('Ctrl Pts',(39.7412068397501,-53.08000002,-163.944571422167));
#165810=CARTESIAN_POINT('Ctrl Pts',(39.5441113151659,-52.3903440317307,
-165.098979928026));
#165811=CARTESIAN_POINT('Ctrl Pts',(39.2784275950098,-53.0800000199999,
-165.197323336931));
#165812=CARTESIAN_POINT('Ctrl Pts',(39.9897001844459,-53.08000002,-164.969734884811));
#165813=CARTESIAN_POINT('Ctrl Pts',(39.7204443742655,-52.3638938128861,
-165.624666922963));
#165814=CARTESIAN_POINT('Ctrl Pts',(39.4053566676027,-53.08000002,-165.756550564755));
#165815=CARTESIAN_POINT('Ctrl Pts',(40.1483999357838,-53.08000002,-165.477859388262));
#165816=CARTESIAN_POINT('Ctrl Pts',(40.1569686920085,-52.3131241972374,
-166.633827745735));
#165817=CARTESIAN_POINT('Ctrl Pts',(39.7291683816592,-53.08000002,-166.861730184891));
#165818=CARTESIAN_POINT('Ctrl Pts',(40.5412718238628,-53.08000002,-166.453581502202));
#165819=CARTESIAN_POINT('Ctrl Pts',(40.4170614047767,-52.2886080120764,
-167.121213082449));
#165820=CARTESIAN_POINT('Ctrl Pts',(39.9351413271735,-53.08000002,-167.416390015348));
#165821=CARTESIAN_POINT('Ctrl Pts',(40.7753307309704,-53.08000002,-166.924921320909));
#165822=CARTESIAN_POINT('Ctrl Pts',(40.7385684738071,-52.2653905871942,
-167.582872774143));
#165823=CARTESIAN_POINT('Ctrl Pts',(40.1851006582006,-53.08000002,-167.941466238826));
#165824=CARTESIAN_POINT('Ctrl Pts',(41.0647116264263,-53.08000002,-167.371563643272));
#165825=CARTESIAN_POINT('',(41.0647116264263,-53.08000002,-167.371563643272));
#165826=CARTESIAN_POINT('Origin',(41.0647116264263,-52.58000002,-167.371563643272));
#165827=CARTESIAN_POINT('Ctrl Pts',(41.0647116264263,-53.08000002,-167.371563643272));
#165828=CARTESIAN_POINT('Ctrl Pts',(40.873027927483,-53.08000002,-167.075711184737));
#165829=CARTESIAN_POINT('Ctrl Pts',(40.7056641754959,-53.08000002,-166.769103902006));
#165830=CARTESIAN_POINT('Ctrl Pts',(40.5574162968375,-53.08000002,-166.454043185673));
#165831=CARTESIAN_POINT('Ctrl Pts',(40.4818120706116,-53.08000002,-166.293366878611));
#165832=CARTESIAN_POINT('Ctrl Pts',(40.4111805199837,-53.08000002,-166.130491546345));
#165833=CARTESIAN_POINT('Ctrl Pts',(40.3448358791345,-53.08000002,-165.965720445509));
#165834=CARTESIAN_POINT('Ctrl Pts',(40.1483999357586,-53.08000002,-165.477859388165));
#165835=CARTESIAN_POINT('Ctrl Pts',(39.9897001835278,-53.08000002,-164.969734884954));
#165836=CARTESIAN_POINT('Ctrl Pts',(39.8654535116526,-53.08000002,-164.457153153597));
#165837=CARTESIAN_POINT('Ctrl Pts',(39.7412068397774,-53.08000002,-163.94457142224));
#165838=CARTESIAN_POINT('Ctrl Pts',(39.6509082568844,-53.08000002,-163.427315362986));
#165839=CARTESIAN_POINT('Ctrl Pts',(39.5905852088212,-53.08000002,-162.905931958774));
#165840=CARTESIAN_POINT('Ctrl Pts',(39.530262160758,-53.08000002,-162.384548554563));
#165841=CARTESIAN_POINT('Ctrl Pts',(39.4999999999991,-53.08000002,-161.85902605313));
#165842=CARTESIAN_POINT('Ctrl Pts',(39.5,-53.08000002,-161.329336741015));
#165843=CARTESIAN_POINT('Ctrl Pts',(43.2972503047852,-53.08000002,-170.861259130871));
#165844=CARTESIAN_POINT('Ctrl Pts',(42.4360603595898,-53.08000002,-171.405549026075));
#165845=CARTESIAN_POINT('Ctrl Pts',(42.9629113790828,-52.2741145284007,
-171.07256826174));
#165846=CARTESIAN_POINT('Ctrl Pts',(42.5594745131554,-53.08000002,-169.693930655453));
#165847=CARTESIAN_POINT('Ctrl Pts',(41.6869083931944,-53.0800000201158,
-170.237641125793));
#165848=CARTESIAN_POINT('Ctrl Pts',(42.2277314430405,-52.2712772274341,
-169.905239816447));
#165849=CARTESIAN_POINT('Ctrl Pts',(41.8155944388483,-53.08000002,-168.530506878352));
#165850=CARTESIAN_POINT('Ctrl Pts',(40.9363322060061,-53.08000002,-169.082082669019));
#165851=CARTESIAN_POINT('Ctrl Pts',(41.4865768015737,-52.2683704772926,
-168.741816047102));
#165852=CARTESIAN_POINT('Ctrl Pts',(41.0647116264263,-53.08000002,-167.371563643272));
#165853=CARTESIAN_POINT('Ctrl Pts',(40.1851006582006,-53.0800000199999,
-167.941466238826));
#165854=CARTESIAN_POINT('Ctrl Pts',(40.738568473807,-52.2653905871942,-167.582872774143));
#165855=CARTESIAN_POINT('',(43.2972503047852,-53.08000002,-170.861259130871));
#165856=CARTESIAN_POINT('Origin',(43.2972503047852,-52.58000002,-170.861259130871));
#165857=CARTESIAN_POINT('Ctrl Pts',(43.2972503047852,-53.08000002,-170.861259130871));
#165858=CARTESIAN_POINT('Ctrl Pts',(42.5594745131554,-53.08000002,-169.693930655453));
#165859=CARTESIAN_POINT('Ctrl Pts',(41.8155944388483,-53.08000002,-168.530506878352));
#165860=CARTESIAN_POINT('Ctrl Pts',(41.0647116264263,-53.08000002,-167.371563643272));
#165861=CARTESIAN_POINT('Ctrl Pts',(42.9629113790828,-52.2741145284007,
-171.07256826174));
#165862=CARTESIAN_POINT('Ctrl Pts',(42.4360603595898,-53.08000002,-171.405549026075));
#165863=CARTESIAN_POINT('Ctrl Pts',(43.2972503047852,-53.08000002,-170.861259130871));
#165864=CARTESIAN_POINT('Ctrl Pts',(43.0118891450524,-52.2900672717484,
-171.173154953435));
#165865=CARTESIAN_POINT('Ctrl Pts',(42.5775224401932,-53.080000020001,-171.535704796364));
#165866=CARTESIAN_POINT('Ctrl Pts',(43.3290496999002,-53.08000002,-170.911572751073));
#165867=CARTESIAN_POINT('Ctrl Pts',(43.073894673874,-52.3102438041593,-171.258275237078));
#165868=CARTESIAN_POINT('Ctrl Pts',(42.7308220084871,-53.0800000200015,
-171.613444114474));
#165869=CARTESIAN_POINT('Ctrl Pts',(43.3692611707715,-53.08000002,-170.954112611118));
#165870=CARTESIAN_POINT('Ctrl Pts',(43.2170017360461,-52.3567135560047,
-171.405295505501));
#165871=CARTESIAN_POINT('Ctrl Pts',(43.0212179754289,-53.0800000199986,
-171.708873691595));
#165872=CARTESIAN_POINT('Ctrl Pts',(43.4620142194198,-53.08000002,-171.027622760172));
#165873=CARTESIAN_POINT('Ctrl Pts',(43.2956718648015,-52.3822166623249,
-171.464307358546));
#165874=CARTESIAN_POINT('Ctrl Pts',(43.154321777956,-53.080000020001,-171.728961938884));
#165875=CARTESIAN_POINT('Ctrl Pts',(43.512966485493,-53.08000002,-171.057128671245));
#165876=CARTESIAN_POINT('Ctrl Pts',(43.4617135157955,-52.4359237144093,
-171.55811115512));
#165877=CARTESIAN_POINT('Ctrl Pts',(43.3978292274293,-53.080000019999,-171.740357884216));
#165878=CARTESIAN_POINT('Ctrl Pts',(43.6204035532382,-53.08000002,-171.104030585588));
#165879=CARTESIAN_POINT('Ctrl Pts',(43.5499633272225,-52.4644105712997,
-171.592966290451));
#165880=CARTESIAN_POINT('Ctrl Pts',(43.5113479697337,-53.080000019999,-171.733309812026));
#165881=CARTESIAN_POINT('Ctrl Pts',(43.6774556997061,-53.08000002,-171.121458138538));
#165882=CARTESIAN_POINT('Ctrl Pts',(43.7274774238083,-52.5215797867686,
-171.638576841342));
#165883=CARTESIAN_POINT('Ctrl Pts',(43.718452515944,-53.080000020001,-171.702758245039));
#165884=CARTESIAN_POINT('Ctrl Pts',(43.7921030708942,-53.08000002,-171.144263427359));
#165885=CARTESIAN_POINT('Ctrl Pts',(43.8177416070106,-52.5505863340359,
-171.64995));
#165886=CARTESIAN_POINT('Ctrl Pts',(43.8149201055142,-53.08000002,-171.680268286151));
#165887=CARTESIAN_POINT('Ctrl Pts',(43.8503459614229,-53.08000002,-171.149949987963));
#165888=CARTESIAN_POINT('Ctrl Pts',(43.9094855672884,-52.58000002,-171.64995));
#165889=CARTESIAN_POINT('Ctrl Pts',(43.9094855672884,-53.0800000199999,
-171.64995));
#165890=CARTESIAN_POINT('Ctrl Pts',(43.9094855672884,-53.08000002,-171.14995));
#165891=CARTESIAN_POINT('',(43.9094855672884,-53.08000002,-171.14995));
#165892=CARTESIAN_POINT('Origin',(43.9094855672884,-52.58000002,-171.14995));
#165893=CARTESIAN_POINT('Ctrl Pts',(43.9094855672884,-53.08000002,-171.14995));
#165894=CARTESIAN_POINT('Ctrl Pts',(43.8503415173364,-53.08000002,-171.14995));
#165895=CARTESIAN_POINT('Ctrl Pts',(43.7921001974326,-53.08000002,-171.144262868806));
#165896=CARTESIAN_POINT('Ctrl Pts',(43.7347793831646,-53.08000002,-171.132860793684));
#165897=CARTESIAN_POINT('Ctrl Pts',(43.6774556974662,-53.08000002,-171.121458147386));
#165898=CARTESIAN_POINT('Ctrl Pts',(43.6204048981063,-53.08000002,-171.104031177905));
#165899=CARTESIAN_POINT('Ctrl Pts',(43.5666850153843,-53.08000002,-171.080579637536));
#165900=CARTESIAN_POINT('Ctrl Pts',(43.5129605101707,-53.08000002,-171.057126079209));
#165901=CARTESIAN_POINT('Ctrl Pts',(43.4620141840633,-53.08000002,-171.02762282191));
#165902=CARTESIAN_POINT('Ctrl Pts',(43.4156376346715,-53.08000002,-170.990867761886));
#165903=CARTESIAN_POINT('Ctrl Pts',(43.3692713886891,-53.08000002,-170.95412086768));
#165904=CARTESIAN_POINT('Ctrl Pts',(43.3290601923967,-53.08000002,-170.911589580894));
#165905=CARTESIAN_POINT('Ctrl Pts',(43.2972503047852,-53.08000002,-170.861259130871));
#165906=CARTESIAN_POINT('Origin',(-83.2809572255632,-52.5800000199999,-171.14995));
#165907=CARTESIAN_POINT('',(49.6300753314849,-53.08000002,-171.14995));
#165908=CARTESIAN_POINT('Origin',(49.6300753314849,-52.58000002,-171.14995));
#165909=CARTESIAN_POINT('',(43.4531980731446,-53.08000002,-171.14995));
#165910=CARTESIAN_POINT('Ctrl Pts',(51.1448166902628,-53.08000002,-172.64995));
#165911=CARTESIAN_POINT('Ctrl Pts',(50.5696324866524,-53.08000002,-172.64995));
#165912=CARTESIAN_POINT('Ctrl Pts',(50.6496826558921,-52.51041346952,-172.64995));
#165913=CARTESIAN_POINT('Ctrl Pts',(51.1448166902479,-53.08000002,-172.453565067926));
#165914=CARTESIAN_POINT('Ctrl Pts',(50.5696324866503,-53.080000020002,-172.529650273729));
#165915=CARTESIAN_POINT('Ctrl Pts',(50.6496826558917,-52.5104134695225,
-172.51902671195));
#165916=CARTESIAN_POINT('Ctrl Pts',(51.1053920215496,-53.08000002,-172.257328160063));
#165917=CARTESIAN_POINT('Ctrl Pts',(50.5479627709917,-53.08000002,-172.409726298163));
#165918=CARTESIAN_POINT('Ctrl Pts',(50.6231450026166,-52.5122246214263,
-172.38820210671));
#165919=CARTESIAN_POINT('Ctrl Pts',(50.9536357182667,-53.08000002,-171.894521542842));
#165920=CARTESIAN_POINT('Ctrl Pts',(50.4615294415736,-53.08000002,-172.182182441317));
#165921=CARTESIAN_POINT('Ctrl Pts',(50.5209943367899,-52.5191962391206,
-172.14633102856));
#165922=CARTESIAN_POINT('Ctrl Pts',(50.8413637606251,-53.08000002,-171.728129909852));
#165923=CARTESIAN_POINT('Ctrl Pts',(50.3972583757626,-53.0800000199979,
-172.075215659168));
#165924=CARTESIAN_POINT('Ctrl Pts',(50.4454214941564,-52.5243539633763,
-172.035403273235));
#165925=CARTESIAN_POINT('Ctrl Pts',(50.5609546754159,-53.08000002,-171.450449746589));
#165926=CARTESIAN_POINT('Ctrl Pts',(50.2296016046087,-53.080000020002,-171.888983273332));
#165927=CARTESIAN_POINT('Ctrl Pts',(50.256671675285,-52.537235833176,-171.850283164392));
#165928=CARTESIAN_POINT('Ctrl Pts',(50.3929278167739,-53.08000002,-171.339270411997));
#165929=CARTESIAN_POINT('Ctrl Pts',(50.1270268918696,-53.0800000200001,
-171.809929875206));
#165930=CARTESIAN_POINT('Ctrl Pts',(50.1435689235997,-52.5449549130127,
-171.776163607997));
#165931=CARTESIAN_POINT('Ctrl Pts',(50.0265556908409,-53.08000002,-171.18899099047));
#165932=CARTESIAN_POINT('Ctrl Pts',(49.8942480960507,-53.08000002,-171.69520402023));
#165933=CARTESIAN_POINT('Ctrl Pts',(49.8969554005076,-52.561785887019,-171.675977326981));
#165934=CARTESIAN_POINT('Ctrl Pts',(49.8283902508599,-53.08000002,-171.149950000016));
#165935=CARTESIAN_POINT('Ctrl Pts',(49.7648572777959,-53.08000002,-171.659148653595));
#165936=CARTESIAN_POINT('Ctrl Pts',(49.7635656750098,-52.5708895200013,
-171.64995));
#165937=CARTESIAN_POINT('Ctrl Pts',(49.6300753314849,-53.08000002,-171.14995));
#165938=CARTESIAN_POINT('Ctrl Pts',(49.6300753314848,-53.0800000199999,
-171.64995));
#165939=CARTESIAN_POINT('Ctrl Pts',(49.6300753314849,-52.58000002,-171.64995));
#165940=CARTESIAN_POINT('',(51.1448166902628,-53.08000002,-172.64995));
#165941=CARTESIAN_POINT('',(50.6448166902628,-52.58000002,-172.64995));
#165942=CARTESIAN_POINT('Origin',(51.1448166902628,-52.58000002,-172.64995));
#165943=CARTESIAN_POINT('Origin',(51.1448166902628,-52.58000002,-172.64995));
#165944=CARTESIAN_POINT('Ctrl Pts',(51.1448166902628,-53.08000002,-172.64995));
#165945=CARTESIAN_POINT('Ctrl Pts',(51.1448166902479,-53.08000002,-172.453565067926));
#165946=CARTESIAN_POINT('Ctrl Pts',(51.1053920215496,-53.08000002,-172.257328160063));
#165947=CARTESIAN_POINT('Ctrl Pts',(50.9536357182667,-53.08000002,-171.894521542842));
#165948=CARTESIAN_POINT('Ctrl Pts',(50.8413637606251,-53.08000002,-171.728129909852));
#165949=CARTESIAN_POINT('Ctrl Pts',(50.5609546754159,-53.08000002,-171.450449746589));
#165950=CARTESIAN_POINT('Ctrl Pts',(50.3929278167739,-53.08000002,-171.339270411997));
#165951=CARTESIAN_POINT('Ctrl Pts',(50.0265556908409,-53.08000002,-171.18899099047));
#165952=CARTESIAN_POINT('Ctrl Pts',(49.8283902508599,-53.08000002,-171.149950000016));
#165953=CARTESIAN_POINT('Ctrl Pts',(49.6300753314849,-53.08000002,-171.14995));
#165954=CARTESIAN_POINT('Origin',(51.1448166902628,-52.58000002,-171.64995));
#165955=CARTESIAN_POINT('',(51.1448166902628,-53.08000002,-55.2499500000008));
#165956=CARTESIAN_POINT('',(50.6496826558921,-52.51041346952,-171.64995));
#165957=CARTESIAN_POINT('Origin',(60.,-53.58000002,-176.84995));
#165958=CARTESIAN_POINT('',(-83.2809572255632,-53.0800000199999,-176.84995));
#165959=CARTESIAN_POINT('Origin',(57.,-53.58000002,-58.24995));
#165960=CARTESIAN_POINT('',(57.,-53.08000002,-55.74995));
#165961=CARTESIAN_POINT('Origin',(57.,-53.08000002,-58.24995));
#165962=CARTESIAN_POINT('',(57.,-53.58000002,-55.24995));
#165963=CARTESIAN_POINT('Origin',(57.,-53.58000002,-55.74995));
#165964=CARTESIAN_POINT('Origin',(57.,-53.58000002,-58.24995));
#165965=CARTESIAN_POINT('Origin',(57.,-2.42462934179819E-14,-58.24995));
#165966=CARTESIAN_POINT('',(57.,-54.08000002,-55.24995));
#165967=CARTESIAN_POINT('',(57.,28.41999998,-55.24995));
#165968=CARTESIAN_POINT('Origin',(57.,-54.08000002,-58.24995));
#165969=CARTESIAN_POINT('Origin',(60.,-55.08000002,-171.14995));
#165970=CARTESIAN_POINT('',(45.8586217441902,-54.58000002,-171.14995));
#165971=CARTESIAN_POINT('',(45.8586217441902,-55.08000002,-171.64995));
#165972=CARTESIAN_POINT('Origin',(45.8586217441902,-55.08000002,-171.14995));
#165973=CARTESIAN_POINT('',(42.5,-55.08000002,-171.64995));
#165974=CARTESIAN_POINT('',(49.2787232447289,-54.58000002,-171.14995));
#165975=CARTESIAN_POINT('Origin',(49.2787232447289,-55.08000002,-171.14995));
#165976=CARTESIAN_POINT('',(49.3489936620801,-54.58000002,-171.14995));
#165977=CARTESIAN_POINT('Origin',(60.,-55.08000002,-171.14995));
#165978=CARTESIAN_POINT('',(43.1572831724514,-55.08000002,-171.64995));
#165979=CARTESIAN_POINT('',(42.5,-55.08000002,-171.64995));
#165980=CARTESIAN_POINT('',(43.1572831724514,-54.58000002,-171.14995));
#165981=CARTESIAN_POINT('Origin',(43.1572831724514,-55.08000002,-171.14995));
#165982=CARTESIAN_POINT('',(49.3489936620801,-54.58000002,-171.14995));
#165983=CARTESIAN_POINT('Origin',(-1.8445455022812E-14,-55.08000002,-61.14995));
#165984=CARTESIAN_POINT('',(43.1572831724516,-54.58000002,-61.14995));
#165985=CARTESIAN_POINT('',(60.,-54.58000002,-61.14995));
#165986=CARTESIAN_POINT('Origin',(43.1572831724516,-55.08000002,-61.14995));
#165987=CARTESIAN_POINT('Ctrl Pts',(43.1572831724516,-55.080148121506,-60.6499500219341));
#165988=CARTESIAN_POINT('Ctrl Pts',(43.1572831724515,-54.58000002,-60.6498018765534));
#165989=CARTESIAN_POINT('Ctrl Pts',(43.1572831724516,-54.58000002,-61.14995));
#165990=CARTESIAN_POINT('Ctrl Pts',(43.3271185292341,-54.9843723315207,
-60.6499212610322));
#165991=CARTESIAN_POINT('Ctrl Pts',(43.3143913613969,-54.58000002,-60.7384339405188));
#165992=CARTESIAN_POINT('Ctrl Pts',(43.3817682803708,-54.58000002,-61.1499499438652));
#165993=CARTESIAN_POINT('Ctrl Pts',(43.5299471737832,-54.8943395876963,
-60.6499049353895));
#165994=CARTESIAN_POINT('Ctrl Pts',(43.5407821982001,-54.58000002,-60.7796882578927));
#165995=CARTESIAN_POINT('Ctrl Pts',(43.6059648750607,-54.58000002,-61.1139843549936));
#165996=CARTESIAN_POINT('Ctrl Pts',(43.9881565230544,-54.764616113509,-60.6498916468796));
#165997=CARTESIAN_POINT('Ctrl Pts',(44.0046317151094,-54.58000002,-60.8040236126605));
#165998=CARTESIAN_POINT('Ctrl Pts',(44.0540062919343,-54.58000002,-61.0395265773532));
#165999=CARTESIAN_POINT('Ctrl Pts',(44.2440095987556,-54.7260645641703,
-60.6498933522812));
#166000=CARTESIAN_POINT('Ctrl Pts',(44.2580491347896,-54.58000002,-60.7962448835176));
#166001=CARTESIAN_POINT('Ctrl Pts',(44.2780419706101,-54.58000002,-61.0029930876918));
#166002=CARTESIAN_POINT('Ctrl Pts',(44.7601884828712,-54.7249655177495,
-60.6498933671498));
#166003=CARTESIAN_POINT('Ctrl Pts',(44.7466180387413,-54.58000002,-60.7961110321462));
#166004=CARTESIAN_POINT('Ctrl Pts',(44.7276655629963,-54.58000002,-61.0020306983307));
#166005=CARTESIAN_POINT('Ctrl Pts',(45.0183788445834,-54.7626525929477,
-60.6498915741979));
#166006=CARTESIAN_POINT('Ctrl Pts',(45.0021140860289,-54.58000002,-60.8040311529128));
#166007=CARTESIAN_POINT('Ctrl Pts',(44.9532637149968,-54.58000002,-61.0380773886891));
#166008=CARTESIAN_POINT('Ctrl Pts',(45.4809398893316,-54.8922510295825,
-60.6499045972125));
#166009=CARTESIAN_POINT('Ctrl Pts',(45.4698465063657,-54.58000002,-60.7804647582867));
#166010=CARTESIAN_POINT('Ctrl Pts',(45.4045230317319,-54.58000002,-61.1130978438444));
#166011=CARTESIAN_POINT('Ctrl Pts',(45.6855420836461,-54.9825427397825,
-60.6499207098429));
#166012=CARTESIAN_POINT('Ctrl Pts',(45.6987517183194,-54.58000002,-60.7399919909284));
#166013=CARTESIAN_POINT('Ctrl Pts',(45.6299507757142,-54.58000002,-61.149949944621));
#166014=CARTESIAN_POINT('Ctrl Pts',(45.8586217441897,-55.080148121506,-60.6499500219341));
#166015=CARTESIAN_POINT('Ctrl Pts',(45.8586217441896,-54.58000002,-60.6498018765534));
#166016=CARTESIAN_POINT('Ctrl Pts',(45.8586217441897,-54.58000002,-61.14995));
#166017=CARTESIAN_POINT('',(45.8586217441897,-54.58000002,-61.14995));
#166018=CARTESIAN_POINT('Ctrl Pts',(45.8586217441897,-54.58000002,-61.14995));
#166019=CARTESIAN_POINT('Ctrl Pts',(45.7594843223744,-54.58000002,-61.1499499759911));
#166020=CARTESIAN_POINT('Ctrl Pts',(45.6608556134178,-54.58000002,-61.1430183938606));
#166021=CARTESIAN_POINT('Ctrl Pts',(45.5625314448154,-54.58000002,-61.1320945152429));
#166022=CARTESIAN_POINT('Ctrl Pts',(45.4342876572929,-54.58000002,-61.1178465476446));
#166023=CARTESIAN_POINT('Ctrl Pts',(45.3065614560444,-54.58000002,-61.0968118490375));
#166024=CARTESIAN_POINT('Ctrl Pts',(45.1788934332666,-54.5800000200001,
-61.075587255946));
#166025=CARTESIAN_POINT('Ctrl Pts',(45.1788516209101,-54.5800000200001,
-61.0755803047123));
#166026=CARTESIAN_POINT('Ctrl Pts',(45.1788098085678,-54.5800000200001,
-61.0755733535311));
#166027=CARTESIAN_POINT('Ctrl Pts',(45.1787679962398,-54.5800000200001,
-61.0755664024026));
#166028=CARTESIAN_POINT('Ctrl Pts',(44.9531807615356,-54.5800000200004,
-61.0380634472604));
#166029=CARTESIAN_POINT('Ctrl Pts',(44.7276252028241,-54.58000002,-61.0020307849363));
#166030=CARTESIAN_POINT('Ctrl Pts',(44.5028537665277,-54.58000002,-61.0025117642945));
#166031=CARTESIAN_POINT('Ctrl Pts',(44.5028486075311,-54.58000002,-61.002511775334));
#166032=CARTESIAN_POINT('Ctrl Pts',(44.5028434485348,-54.58000002,-61.0025117863925));
#166033=CARTESIAN_POINT('Ctrl Pts',(44.502838289539,-54.58000002,-61.00251179747));
#166034=CARTESIAN_POINT('Ctrl Pts',(44.3506760857094,-54.58000002,-61.0028385232137));
#166035=CARTESIAN_POINT('Ctrl Pts',(44.1989241833573,-54.5800000200001,
-61.0196754576622));
#166036=CARTESIAN_POINT('Ctrl Pts',(44.0472833113082,-54.5800000200001,
-61.042061298072));
#166037=CARTESIAN_POINT('Ctrl Pts',(43.9748362264932,-54.5800000200001,
-61.0527562304929));
#166038=CARTESIAN_POINT('Ctrl Pts',(43.9024145037602,-54.58000002,-61.0647186315174));
#166039=CARTESIAN_POINT('Ctrl Pts',(43.8299855489727,-54.58000002,-61.0767552584245));
#166040=CARTESIAN_POINT('Ctrl Pts',(43.7015244308355,-54.58000002,-61.0981036066869));
#166041=CARTESIAN_POINT('Ctrl Pts',(43.5729778197502,-54.58000002,-61.1190439724882));
#166042=CARTESIAN_POINT('Ctrl Pts',(43.4442858805782,-54.58000002,-61.1330238652827));
#166043=CARTESIAN_POINT('Ctrl Pts',(43.3487066835599,-54.58000002,-61.143406698398));
#166044=CARTESIAN_POINT('Ctrl Pts',(43.2530473192975,-54.58000002,-61.1499499760532));
#166045=CARTESIAN_POINT('Ctrl Pts',(43.1572831724516,-54.58000002,-61.14995));
#166046=CARTESIAN_POINT('',(45.8586217441897,-55.08000002,-60.64995));
#166047=CARTESIAN_POINT('Origin',(45.8586217441897,-55.08000002,-61.14995));
#166048=CARTESIAN_POINT('Ctrl Pts',(45.8586217441897,-55.08000002,-60.64995));
#166049=CARTESIAN_POINT('Ctrl Pts',(45.7689536596558,-55.029440916946,-60.64995));
#166050=CARTESIAN_POINT('Ctrl Pts',(45.6765174633164,-54.9839564622373,
-60.6499624250156));
#166051=CARTESIAN_POINT('Ctrl Pts',(45.4778485953844,-54.8996925932592,
-60.6499736157096));
#166052=CARTESIAN_POINT('Ctrl Pts',(45.3713338603102,-54.8620619965581,
-60.649952959783));
#166053=CARTESIAN_POINT('Ctrl Pts',(45.185760202174,-54.8090884744683,-60.6499481945182));
#166054=CARTESIAN_POINT('Ctrl Pts',(45.1077985401425,-54.7904750984749,
-60.6500611432134));
#166055=CARTESIAN_POINT('Ctrl Pts',(44.9203791059894,-54.7542997329155,
-60.6502857315348));
#166056=CARTESIAN_POINT('Ctrl Pts',(44.8104650288099,-54.7398986265098,
-60.6502931678836));
#166057=CARTESIAN_POINT('Ctrl Pts',(44.6361116415848,-54.7276946232681,
-60.6500701126525));
#166058=CARTESIAN_POINT('Ctrl Pts',(44.5721214250066,-54.7254562445459,
-60.6499575033559));
#166059=CARTESIAN_POINT('Ctrl Pts',(44.4919713617192,-54.7254515344577,
-60.6499485324377));
#166060=CARTESIAN_POINT('Ctrl Pts',(44.4758287519404,-54.7255927281287,
-60.6499538101927));
#166061=CARTESIAN_POINT('Ctrl Pts',(44.3973353016915,-54.726970533525,-60.6500007005379));
#166062=CARTESIAN_POINT('Ctrl Pts',(44.3350361171944,-54.7301856687748,
-60.6500992062372));
#166063=CARTESIAN_POINT('Ctrl Pts',(44.2458944853161,-54.7378330706298,
-60.6501868928199));
#166064=CARTESIAN_POINT('Ctrl Pts',(44.2189296557646,-54.7405484163116,
-60.6502073540677));
#166065=CARTESIAN_POINT('Ctrl Pts',(44.1669378685651,-54.746561490262,-60.650229174244));
#166066=CARTESIAN_POINT('Ctrl Pts',(44.141907947471,-54.7498060612269,-60.6502317923741));
#166067=CARTESIAN_POINT('Ctrl Pts',(44.0251905251394,-54.7665726407089,
-60.6502071425432));
#166068=CARTESIAN_POINT('Ctrl Pts',(43.9341908339756,-54.7843774385812,
-60.6500644239801));
#166069=CARTESIAN_POINT('Ctrl Pts',(43.7178584587808,-54.8381778103589,
-60.6498839791579));
#166070=CARTESIAN_POINT('Ctrl Pts',(43.5938526567529,-54.8785531161367,
-60.6499834288654));
#166071=CARTESIAN_POINT('Ctrl Pts',(43.3647423777244,-54.9716018333708,
-60.6499762216949));
#166072=CARTESIAN_POINT('Ctrl Pts',(43.2592299860172,-55.0225175893237,
-60.64995));
#166073=CARTESIAN_POINT('Ctrl Pts',(43.1572831724516,-55.08000002,-60.64995));
#166074=CARTESIAN_POINT('Origin',(57.,-54.08000002,-58.24995));
#166075=CARTESIAN_POINT('',(59.5,-54.58000002,-58.24995));
#166076=CARTESIAN_POINT('Origin',(59.5,-54.08000002,-58.24995));
#166077=CARTESIAN_POINT('',(57.,-54.58000002,-55.74995));
#166078=CARTESIAN_POINT('Origin',(57.,-54.08000002,-55.74995));
#166079=CARTESIAN_POINT('Origin',(57.,-54.58000002,-58.24995));
#166080=CARTESIAN_POINT('Origin',(59.5,-54.08000002,0.));
#166081=CARTESIAN_POINT('',(59.5,-54.58000002,-174.34995));
#166082=CARTESIAN_POINT('Origin',(59.5,-54.08000002,-174.34995));
#166083=CARTESIAN_POINT('',(59.5,-54.58000002,-58.24995));
#166084=CARTESIAN_POINT('Origin',(57.,-54.08000002,-174.34995));
#166085=CARTESIAN_POINT('',(57.,-54.58000002,-176.84995));
#166086=CARTESIAN_POINT('Origin',(57.,-54.08000002,-176.84995));
#166087=CARTESIAN_POINT('Origin',(57.,-54.58000002,-174.34995));
#166088=CARTESIAN_POINT('Origin',(60.,-54.08000002,-176.84995));
#166089=CARTESIAN_POINT('',(60.,-54.58000002,-176.84995));
#166090=CARTESIAN_POINT('Origin',(50.7934646035069,-55.08000002,-171.64995));
#166091=CARTESIAN_POINT('',(50.7934646035069,-54.58000002,-172.64995));
#166092=CARTESIAN_POINT('Origin',(50.7934646035069,-55.08000002,-172.64995));
#166093=CARTESIAN_POINT('',(50.2983305691361,-55.0104134695199,-171.64995));
#166094=CARTESIAN_POINT('',(50.7934646035069,-54.58000002,-55.24995));
#166095=CARTESIAN_POINT('Ctrl Pts',(49.2787232447289,-54.58000002,-171.14995));
#166096=CARTESIAN_POINT('Ctrl Pts',(49.2787232447289,-54.58000002,-171.64995));
#166097=CARTESIAN_POINT('Ctrl Pts',(49.2787232447289,-55.08000002,-171.64995));
#166098=CARTESIAN_POINT('Ctrl Pts',(49.477038164104,-54.58000002,-171.149950000016));
#166099=CARTESIAN_POINT('Ctrl Pts',(49.4109716734917,-54.58000002,-171.640924254979));
#166100=CARTESIAN_POINT('Ctrl Pts',(49.4122135882539,-55.0708895200012,
-171.64995));
#166101=CARTESIAN_POINT('Ctrl Pts',(49.6752036040849,-54.58000002,-171.18899099047));
#166102=CARTESIAN_POINT('Ctrl Pts',(49.548241251645,-54.58000002,-171.658003579003));
#166103=CARTESIAN_POINT('Ctrl Pts',(49.5456033137516,-55.061785887019,-171.675977326981));
#166104=CARTESIAN_POINT('Ctrl Pts',(50.0415757300179,-54.58000002,-171.339270411997));
#166105=CARTESIAN_POINT('Ctrl Pts',(49.8066765125445,-54.5800000199999,
-171.746711574348));
#166106=CARTESIAN_POINT('Ctrl Pts',(49.7922168368437,-55.0449549130127,
-171.776163607997));
#166107=CARTESIAN_POINT('Ctrl Pts',(50.2096025886599,-54.58000002,-171.450449746589));
#166108=CARTESIAN_POINT('Ctrl Pts',(49.9282402287017,-54.5800000199992,
-171.817687494207));
#166109=CARTESIAN_POINT('Ctrl Pts',(49.9053195885289,-55.037235833176,-171.850283164392));
#166110=CARTESIAN_POINT('Ctrl Pts',(50.4900116738692,-54.58000002,-171.728129909852));
#166111=CARTESIAN_POINT('Ctrl Pts',(50.1326854480763,-54.5800000200006,
-172.003556970024));
#166112=CARTESIAN_POINT('Ctrl Pts',(50.0940694074005,-55.0243539633763,
-172.035403273235));
#166113=CARTESIAN_POINT('Ctrl Pts',(50.6022836315107,-54.58000002,-171.894521542842));
#166114=CARTESIAN_POINT('Ctrl Pts',(50.2162545403414,-54.58000002,-172.118296873734));
#166115=CARTESIAN_POINT('Ctrl Pts',(50.1696422500339,-55.0191962391206,
-172.14633102856));
#166116=CARTESIAN_POINT('Ctrl Pts',(50.7540399347937,-54.58000002,-172.257328160063));
#166117=CARTESIAN_POINT('Ctrl Pts',(50.3290655494749,-54.58000002,-172.371853931892));
#166118=CARTESIAN_POINT('Ctrl Pts',(50.2717929158607,-55.0122246214262,
-172.38820210671));
#166119=CARTESIAN_POINT('Ctrl Pts',(50.7934646034919,-54.58000002,-172.453565067926));
#166120=CARTESIAN_POINT('Ctrl Pts',(50.3588212345858,-54.5800000199993,
-172.511015867073));
#166121=CARTESIAN_POINT('Ctrl Pts',(50.2983305691357,-55.0104134695225,
-172.51902671195));
#166122=CARTESIAN_POINT('Ctrl Pts',(50.7934646035069,-54.58000002,-172.64995));
#166123=CARTESIAN_POINT('Ctrl Pts',(50.3588212345988,-54.5800000199999,
-172.64995));
#166124=CARTESIAN_POINT('Ctrl Pts',(50.2983305691361,-55.0104134695199,
-172.64995));
#166125=CARTESIAN_POINT('Ctrl Pts',(49.2787232447289,-54.58000002,-171.14995));
#166126=CARTESIAN_POINT('Ctrl Pts',(49.477038164104,-54.58000002,-171.149950000016));
#166127=CARTESIAN_POINT('Ctrl Pts',(49.6752036040849,-54.58000002,-171.18899099047));
#166128=CARTESIAN_POINT('Ctrl Pts',(50.0415757300179,-54.58000002,-171.339270411997));
#166129=CARTESIAN_POINT('Ctrl Pts',(50.2096025886599,-54.58000002,-171.450449746589));
#166130=CARTESIAN_POINT('Ctrl Pts',(50.4900116738692,-54.58000002,-171.728129909852));
#166131=CARTESIAN_POINT('Ctrl Pts',(50.6022836315107,-54.58000002,-171.894521542842));
#166132=CARTESIAN_POINT('Ctrl Pts',(50.7540399347937,-54.58000002,-172.257328160063));
#166133=CARTESIAN_POINT('Ctrl Pts',(50.7934646034919,-54.58000002,-172.453565067926));
#166134=CARTESIAN_POINT('Ctrl Pts',(50.7934646035069,-54.58000002,-172.64995));
#166135=CARTESIAN_POINT('Ctrl Pts',(52.4185037433787,-38.6078427661476,
-171.271207239029));
#166136=CARTESIAN_POINT('Ctrl Pts',(52.5086485179119,-38.28000002,-171.191647032251));
#166137=CARTESIAN_POINT('Ctrl Pts',(52.7704579175044,-38.28000002,-170.960578619515));
#166138=CARTESIAN_POINT('Ctrl Pts',(52.370156234462,-38.5972036761564,-171.210531232685));
#166139=CARTESIAN_POINT('Ctrl Pts',(52.4702729319568,-38.2800000200013,
-171.135526834247));
#166140=CARTESIAN_POINT('Ctrl Pts',(52.7436831755344,-38.28000002,-170.930241803514));
#166141=CARTESIAN_POINT('Ctrl Pts',(52.3288572922619,-38.5881022353565,
-171.144413209532));
#166142=CARTESIAN_POINT('Ctrl Pts',(52.4376229301059,-38.2800000199995,
-171.075889787111));
#166143=CARTESIAN_POINT('Ctrl Pts',(52.7208049303309,-38.28000002,-170.897181907961));
#166144=CARTESIAN_POINT('Ctrl Pts',(52.2951895046066,-38.58067735034,-171.072568261741));
#166145=CARTESIAN_POINT('Ctrl Pts',(52.4111831155989,-38.28000002,-171.012340412829));
#166146=CARTESIAN_POINT('Ctrl Pts',(52.7021525552272,-38.28000002,-170.861259130871));
#166147=CARTESIAN_POINT('',(52.7021525552272,-38.28000002,-170.861259130871));
#166148=CARTESIAN_POINT('Origin',(52.7021525552272,-38.78000002,-170.861259130871));
#166149=CARTESIAN_POINT('',(52.7704579175045,-38.28000002,-170.960578619515));
#166150=CARTESIAN_POINT('Origin',(52.7704579175045,-38.78000002,-170.960578619515));
#166151=CARTESIAN_POINT('Ctrl Pts',(52.7021525552272,-38.28000002,-170.861259130871));
#166152=CARTESIAN_POINT('Ctrl Pts',(52.7208104423973,-38.28000002,-170.897192602603));
#166153=CARTESIAN_POINT('Ctrl Pts',(52.7436752534113,-38.28000002,-170.930232830913));
#166154=CARTESIAN_POINT('Ctrl Pts',(52.7704579175045,-38.28000002,-170.960578619515));
#166155=CARTESIAN_POINT('Ctrl Pts',(40.5593018105247,-38.28000002,-148.113408860656));
#166156=CARTESIAN_POINT('Ctrl Pts',(40.3021382496555,-38.28000002,-148.255551254414));
#166157=CARTESIAN_POINT('Ctrl Pts',(40.1770020116941,-38.5366991465431,
-148.324717991527));
#166158=CARTESIAN_POINT('Ctrl Pts',(42.6385250759047,-38.28000002,-151.875132894361));
#166159=CARTESIAN_POINT('Ctrl Pts',(42.3869374257262,-38.280000019955,-152.041577619703));
#166160=CARTESIAN_POINT('Ctrl Pts',(42.2505775009144,-38.5455762523402,
-152.086445166823));
#166161=CARTESIAN_POINT('Ctrl Pts',(44.6827387638399,-38.28000002,-155.655552720034));
#166162=CARTESIAN_POINT('Ctrl Pts',(44.4227143745257,-38.2800000199852,
-155.82004311619));
#166163=CARTESIAN_POINT('Ctrl Pts',(44.2901446089557,-38.5535332680681,
-155.866861850893));
#166164=CARTESIAN_POINT('Ctrl Pts',(48.7243729558795,-38.28000002,-163.241363066864));
#166165=CARTESIAN_POINT('Ctrl Pts',(48.4532973709855,-38.280000020015,-163.409015135176));
#166166=CARTESIAN_POINT('Ctrl Pts',(48.3237478755738,-38.5680639323333,
-163.452672197745));
#166167=CARTESIAN_POINT('Ctrl Pts',(50.7215899998133,-38.28000002,-167.046867503852));
#166168=CARTESIAN_POINT('Ctrl Pts',(50.4437502527583,-38.2800000199406,
-167.213058728775));
#166169=CARTESIAN_POINT('Ctrl Pts',(50.3175866645898,-38.5746359826999,
-167.258178117331));
#166170=CARTESIAN_POINT('Ctrl Pts',(52.7021525552272,-38.28000002,-170.861259130871));
#166171=CARTESIAN_POINT('Ctrl Pts',(52.4111831155989,-38.28000002,-171.012340412829));
#166172=CARTESIAN_POINT('Ctrl Pts',(52.2951895046066,-38.58067735034,-171.07256826174));
#166173=CARTESIAN_POINT('',(40.5593018105246,-38.28000002,-148.113408860656));
#166174=CARTESIAN_POINT('Origin',(40.5593018105246,-38.78000002,-148.113408860656));
#166175=CARTESIAN_POINT('Ctrl Pts',(40.5593018105247,-38.28000002,-148.113408860656));
#166176=CARTESIAN_POINT('Ctrl Pts',(42.6385266988695,-38.28000002,-151.875135830624));
#166177=CARTESIAN_POINT('Ctrl Pts',(44.6827387638261,-38.28000002,-155.655552720007));
#166178=CARTESIAN_POINT('Ctrl Pts',(46.7035558598462,-38.28000002,-159.448457893456));
#166179=CARTESIAN_POINT('Ctrl Pts',(48.7243729558662,-38.28000002,-163.241363066904));
#166180=CARTESIAN_POINT('Ctrl Pts',(50.7215893876843,-38.28000002,-167.046866324983));
#166181=CARTESIAN_POINT('Ctrl Pts',(52.7021525552272,-38.28000002,-170.86125913087));
#166182=CARTESIAN_POINT('Ctrl Pts',(40.2402032265086,-38.5310516260855,
-148.430476962511));
#166183=CARTESIAN_POINT('Ctrl Pts',(40.3651906300648,-38.28000002,-148.358692119651));
#166184=CARTESIAN_POINT('Ctrl Pts',(40.6162128330585,-38.28000002,-148.214500674674));
#166185=CARTESIAN_POINT('Ctrl Pts',(39.7977899207324,-38.5702096309806,
-147.703924195849));
#166186=CARTESIAN_POINT('Ctrl Pts',(39.9124625700216,-38.28000002,-147.631198453379));
#166187=CARTESIAN_POINT('Ctrl Pts',(40.2179805560823,-38.28000002,-147.519873800225));
#166188=CARTESIAN_POINT('Ctrl Pts',(39.4932042804462,-38.6117726883092,
-146.929953925225));
#166189=CARTESIAN_POINT('Ctrl Pts',(39.6018856406274,-38.28000002,-146.86744228999));
#166190=CARTESIAN_POINT('Ctrl Pts',(39.9439021523076,-38.28000002,-146.780824095429));
#166191=CARTESIAN_POINT('Ctrl Pts',(39.1932776445035,-38.6754317541046,
-145.737338799595));
#166192=CARTESIAN_POINT('Ctrl Pts',(39.2753128801367,-38.28000002,-145.71515188289));
#166193=CARTESIAN_POINT('Ctrl Pts',(39.6739630147418,-38.28000002,-145.64333076277));
#166194=CARTESIAN_POINT('Ctrl Pts',(39.1206267323737,-38.6963627685879,
-145.344127129863));
#166195=CARTESIAN_POINT('Ctrl Pts',(39.1901218279244,-38.28000002,-145.326713623533));
#166196=CARTESIAN_POINT('Ctrl Pts',(39.6085749933904,-38.28000002,-145.268506383101));
#166197=CARTESIAN_POINT('Ctrl Pts',(39.0193613209311,-38.7402648896269,
-144.516661028813));
#166198=CARTESIAN_POINT('Ctrl Pts',(39.0555238762964,-38.28000002,-144.505704693498));
#166199=CARTESIAN_POINT('Ctrl Pts',(39.5174306634401,-38.28000002,-144.480224304407));
#166200=CARTESIAN_POINT('Ctrl Pts',(38.9953087866826,-38.763347780271,-144.080042595184));
#166201=CARTESIAN_POINT('Ctrl Pts',(39.0120467208245,-38.28000002,-144.07044288467));
#166202=CARTESIAN_POINT('Ctrl Pts',(39.4957803914547,-38.28000002,-144.064560626685));
#166203=CARTESIAN_POINT('Ctrl Pts',(39.0007543400766,-38.7864872879417,
-143.640515939691));
#166204=CARTESIAN_POINT('Ctrl Pts',(38.994184744005,-38.2800000199999,-143.64044055047));
#166205=CARTESIAN_POINT('Ctrl Pts',(39.5006779618633,-38.28000002,-143.646429119223));
#166206=CARTESIAN_POINT('',(39.5,-38.28000002,-143.762156710948));
#166207=CARTESIAN_POINT('Origin',(39.5,-38.78000002,-143.762156710948));
#166208=CARTESIAN_POINT('Ctrl Pts',(39.5,-38.28000002,-143.762156710948));
#166209=CARTESIAN_POINT('Ctrl Pts',(39.5,-38.28000002,-144.141283590664));
#166210=CARTESIAN_POINT('Ctrl Pts',(39.5218408888636,-38.28000002,-144.518367123251));
#166211=CARTESIAN_POINT('Ctrl Pts',(39.5652079410422,-38.28000002,-144.893436753186));
#166212=CARTESIAN_POINT('Ctrl Pts',(39.6085749932207,-38.28000002,-145.26850638312));
#166213=CARTESIAN_POINT('Ctrl Pts',(39.6739630147302,-38.28000002,-145.643330762739));
#166214=CARTESIAN_POINT('Ctrl Pts',(39.7609941006785,-38.28000002,-146.010070025021));
#166215=CARTESIAN_POINT('Ctrl Pts',(39.8480251866268,-38.28000002,-146.376809287303));
#166216=CARTESIAN_POINT('Ctrl Pts',(39.9556757536423,-38.28000002,-146.736297755287));
#166217=CARTESIAN_POINT('Ctrl Pts',(40.0875243805731,-38.28000002,-147.087277124802));
#166218=CARTESIAN_POINT('Ctrl Pts',(40.206517035942,-38.28000002,-147.404034061377));
#166219=CARTESIAN_POINT('Ctrl Pts',(40.3452186968614,-38.28000002,-147.713860479176));
#166220=CARTESIAN_POINT('Ctrl Pts',(40.5063035885383,-38.28000002,-148.015815905681));
#166221=CARTESIAN_POINT('Ctrl Pts',(40.5237072071063,-38.28000002,-148.04843918284));
#166222=CARTESIAN_POINT('Ctrl Pts',(40.5413721449718,-38.28000002,-148.080970567499));
#166223=CARTESIAN_POINT('Ctrl Pts',(40.5593018105246,-38.28000002,-148.113408860656));
#166224=CARTESIAN_POINT('Origin',(39.5,-38.78000002,-55.2499500000007));
#166225=CARTESIAN_POINT('',(39.5,-38.28000002,-88.296486260558));
#166226=CARTESIAN_POINT('Origin',(39.5,-38.78000002,-88.296486260558));
#166227=CARTESIAN_POINT('',(39.5,-38.28000002,-55.2499500000007));
#166228=CARTESIAN_POINT('Ctrl Pts',(39.,-38.78000002,-88.296486260558));
#166229=CARTESIAN_POINT('Ctrl Pts',(39.,-38.2800000199999,-88.296486260558));
#166230=CARTESIAN_POINT('Ctrl Pts',(39.5,-38.28000002,-88.296486260558));
#166231=CARTESIAN_POINT('Ctrl Pts',(39.,-38.7380050653939,-87.4993525996999));
#166232=CARTESIAN_POINT('Ctrl Pts',(39.0402973596559,-38.2800000199999,
-87.5315757932098));
#166233=CARTESIAN_POINT('Ctrl Pts',(39.500000001834,-38.28000002,-87.5380528917837));
#166234=CARTESIAN_POINT('Ctrl Pts',(39.094978232517,-38.6964757448679,-86.7169698827889));
#166235=CARTESIAN_POINT('Ctrl Pts',(39.1607938862687,-38.2800000199999,
-86.7517814461085));
#166236=CARTESIAN_POINT('Ctrl Pts',(39.5854804081441,-38.28000002,-86.7926795341198));
#166237=CARTESIAN_POINT('Ctrl Pts',(39.4784350964048,-38.6146030713812,
-85.1828476912075));
#166238=CARTESIAN_POINT('Ctrl Pts',(39.5865447970557,-38.28000002,-85.2418413411644));
#166239=CARTESIAN_POINT('Ctrl Pts',(39.9305915878855,-38.28000002,-85.3294730611686));
#166240=CARTESIAN_POINT('Ctrl Pts',(39.7704847917915,-38.5740029030169,
-84.4264431605892));
#166241=CARTESIAN_POINT('Ctrl Pts',(39.8855744697273,-38.28000002,-84.495834401995));
#166242=CARTESIAN_POINT('Ctrl Pts',(40.1934239997695,-38.28000002,-84.6071790833831));
#166243=CARTESIAN_POINT('Ctrl Pts',(40.1770020116941,-38.5366991465431,
-83.7339249799794));
#166244=CARTESIAN_POINT('Ctrl Pts',(40.3021382496555,-38.2800000199999,
-83.8030917170923));
#166245=CARTESIAN_POINT('Ctrl Pts',(40.5593018105246,-38.28000002,-83.9452341108497));
#166246=CARTESIAN_POINT('',(40.5593018105246,-38.28000002,-83.9452341108497));
#166247=CARTESIAN_POINT('Origin',(40.5593018105246,-38.78000002,-83.9452341108497));
#166248=CARTESIAN_POINT('Ctrl Pts',(40.5593018105246,-38.28000002,-83.9452341108497));
#166249=CARTESIAN_POINT('Ctrl Pts',(40.495353484328,-38.28000002,-84.0609292165926));
#166250=CARTESIAN_POINT('Ctrl Pts',(40.4347639681506,-38.28000002,-84.1780768945292));
#166251=CARTESIAN_POINT('Ctrl Pts',(40.377316900473,-38.28000002,-84.2965776208551));
#166252=CARTESIAN_POINT('Ctrl Pts',(40.3173964789327,-38.28000002,-84.42018033482));
#166253=CARTESIAN_POINT('Ctrl Pts',(40.2608947873256,-38.28000002,-84.5452556205672));
#166254=CARTESIAN_POINT('Ctrl Pts',(40.2076155462081,-38.28000002,-84.6717210755965));
#166255=CARTESIAN_POINT('Ctrl Pts',(40.1651845073099,-38.28000002,-84.7724368615026));
#166256=CARTESIAN_POINT('Ctrl Pts',(40.1247982681521,-38.28000002,-84.8740350854921));
#166257=CARTESIAN_POINT('Ctrl Pts',(40.086379235959,-38.28000002,-84.9764835369928));
#166258=CARTESIAN_POINT('Ctrl Pts',(40.0265153547945,-38.28000002,-85.1361169680304));
#166259=CARTESIAN_POINT('Ctrl Pts',(39.9714555367521,-38.28000002,-85.2977643783891));
#166260=CARTESIAN_POINT('Ctrl Pts',(39.9211479365403,-38.28000002,-85.4606561619587));
#166261=CARTESIAN_POINT('Ctrl Pts',(39.8688810993165,-38.28000002,-85.6298917903942));
#166262=CARTESIAN_POINT('Ctrl Pts',(39.821743908823,-38.28000002,-85.8004696290636));
#166263=CARTESIAN_POINT('Ctrl Pts',(39.7796250224716,-38.28000002,-85.9715109372544));
#166264=CARTESIAN_POINT('Ctrl Pts',(39.7722762919973,-38.28000002,-86.0013535229146));
#166265=CARTESIAN_POINT('Ctrl Pts',(39.7650802005722,-38.28000002,-86.0312102022424));
#166266=CARTESIAN_POINT('Ctrl Pts',(39.758035997616,-38.28000002,-86.0610762975502));
#166267=CARTESIAN_POINT('Ctrl Pts',(39.6557558157219,-38.28000002,-86.4947250268074));
#166268=CARTESIAN_POINT('Ctrl Pts',(39.5840763701744,-38.28000002,-86.9331589876102));
#166269=CARTESIAN_POINT('Ctrl Pts',(39.5426478307206,-38.28000002,-87.3763235090859));
#166270=CARTESIAN_POINT('Ctrl Pts',(39.5141828100108,-38.28000002,-87.6808161957216));
#166271=CARTESIAN_POINT('Ctrl Pts',(39.5,-38.28000002,-87.9875423033778));
#166272=CARTESIAN_POINT('Ctrl Pts',(39.5,-38.28000002,-88.296486260558));
#166273=CARTESIAN_POINT('Ctrl Pts',(52.5768547844511,-38.28000002,-61.4386408691297));
#166274=CARTESIAN_POINT('Ctrl Pts',(52.2861787013546,-38.28000002,-61.287642251635));
#166275=CARTESIAN_POINT('Ctrl Pts',(52.1700794675439,-38.5802945048887,
-61.2273317382593));
#166276=CARTESIAN_POINT('Ctrl Pts',(50.6164606414324,-38.28000002,-65.2124482077584));
#166277=CARTESIAN_POINT('Ctrl Pts',(50.3387340734665,-38.2800000200587,
-65.0466233854387));
#166278=CARTESIAN_POINT('Ctrl Pts',(50.2126317933694,-38.5742944332221,
-65.0011376410615));
#166279=CARTESIAN_POINT('Ctrl Pts',(48.6396458371624,-38.28000002,-68.9774905161504));
#166280=CARTESIAN_POINT('Ctrl Pts',(48.3685987197966,-38.28000002,-68.8102729799503));
#166281=CARTESIAN_POINT('Ctrl Pts',(48.239176789686,-38.5677719010369,-68.7661813852757));
#166282=CARTESIAN_POINT('Ctrl Pts',(44.6396194153305,-38.28000002,-76.4827983330569));
#166283=CARTESIAN_POINT('Ctrl Pts',(44.3795316629781,-38.28000002,-76.3187098252974));
#166284=CARTESIAN_POINT('Ctrl Pts',(44.247123664849,-38.5533652514423,-76.2714892021909));
#166285=CARTESIAN_POINT('Ctrl Pts',(42.6166022657662,-38.28000002,-80.2231727548289));
#166286=CARTESIAN_POINT('Ctrl Pts',(42.3648252555903,-38.2800000199999,
-80.0572213824928));
#166287=CARTESIAN_POINT('Ctrl Pts',(42.228714191533,-38.5454826541321,-80.0118606023558));
#166288=CARTESIAN_POINT('Ctrl Pts',(40.5593018105246,-38.28000002,-83.9452341108497));
#166289=CARTESIAN_POINT('Ctrl Pts',(40.3021382496555,-38.28000002,-83.8030917170923));
#166290=CARTESIAN_POINT('Ctrl Pts',(40.177002011694,-38.5366991465431,-83.7339249799794));
#166291=CARTESIAN_POINT('',(52.5768547844511,-38.28000002,-61.4386408691297));
#166292=CARTESIAN_POINT('',(52.1700794675439,-38.5802945048887,-61.2273317382593));
#166293=CARTESIAN_POINT('Origin',(52.5768547844511,-38.78000002,-61.4386408691297));
#166294=CARTESIAN_POINT('Ctrl Pts',(40.177002011694,-38.536699146543,-83.7339249799794));
#166295=CARTESIAN_POINT('Ctrl Pts',(40.7446447656533,-38.5391292605099,
-82.7041495102648));
#166296=CARTESIAN_POINT('Ctrl Pts',(41.3204916041055,-38.5415363980795,
-81.6534564475751));
#166297=CARTESIAN_POINT('Ctrl Pts',(41.9045140297048,-38.5439178456464,
-80.5818101170486));
#166298=CARTESIAN_POINT('Ctrl Pts',(42.4744069545298,-38.5462416778483,
-79.536090578017));
#166299=CARTESIAN_POINT('Ctrl Pts',(43.0520848743935,-38.5485410462409,
-78.4704186258952));
#166300=CARTESIAN_POINT('Ctrl Pts',(43.6375626153468,-38.5508142186263,
-77.3847870051934));
#166301=CARTESIAN_POINT('Ctrl Pts',(44.2084182209449,-38.5530306191961,
-76.3262687167217));
#166302=CARTESIAN_POINT('Ctrl Pts',(44.7866884417665,-38.5552221118789,
-75.2487758893125));
#166303=CARTESIAN_POINT('Ctrl Pts',(45.3724279863849,-38.5573878910057,
-74.1523290357761));
#166304=CARTESIAN_POINT('Ctrl Pts',(45.6528382846118,-38.5584247115113,
-73.6274285198132));
#166305=CARTESIAN_POINT('Ctrl Pts',(45.9349610406077,-38.5594556511644,
-73.0981844964864));
#166306=CARTESIAN_POINT('Ctrl Pts',(46.2188059022254,-38.5604806919717,
-72.5646014397013));
#166307=CARTESIAN_POINT('Ctrl Pts',(46.2269016349262,-38.560509927859,-72.5493827537727));
#166308=CARTESIAN_POINT('Ctrl Pts',(46.23585120676,-38.5605422353004,-72.5325579056226));
#166309=CARTESIAN_POINT('Ctrl Pts',(46.2431502305807,-38.5605685685527,
-72.5188352954991));
#166310=CARTESIAN_POINT('Ctrl Pts',(46.2433044757766,-38.5605691250351,
-72.5185453051197));
#166311=CARTESIAN_POINT('Ctrl Pts',(46.2434579839114,-38.5605696788504,
-72.5182567001373));
#166312=CARTESIAN_POINT('Ctrl Pts',(46.2436107313547,-38.5605702299136,
-72.5179695249877));
#166313=CARTESIAN_POINT('Ctrl Pts',(46.8939219586432,-38.562916341634,-71.2953420301694));
#166314=CARTESIAN_POINT('Ctrl Pts',(47.5544270166758,-38.5652360394503,
-70.0477205124839));
#166315=CARTESIAN_POINT('Ctrl Pts',(48.2251016678356,-38.5675266745615,
-68.7750796691625));
#166316=CARTESIAN_POINT('Ctrl Pts',(48.873376566188,-38.5697408051259,-67.5449435488894));
#166317=CARTESIAN_POINT('Ctrl Pts',(49.5311530209752,-38.5719277795132,
-66.2914313855809));
#166318=CARTESIAN_POINT('Ctrl Pts',(50.1984508815467,-38.5740861349683,
-65.0145434284377));
#166319=CARTESIAN_POINT('Ctrl Pts',(50.846656328617,-38.5761827365691,-63.7741891908119));
#166320=CARTESIAN_POINT('Ctrl Pts',(51.5038460529118,-38.5782523311409,
-62.5117776143721));
#166321=CARTESIAN_POINT('Ctrl Pts',(52.1700794675439,-38.5802945048887,
-61.2273317382593));
#166322=CARTESIAN_POINT('Ctrl Pts',(52.5768547844511,-38.28000002,-61.4386408691297));
#166323=CARTESIAN_POINT('Ctrl Pts',(50.6164600523975,-38.28000002,-65.2124493416261));
#166324=CARTESIAN_POINT('Ctrl Pts',(48.6396458371541,-38.28000002,-68.9774905161615));
#166325=CARTESIAN_POINT('Ctrl Pts',(46.6396326262455,-38.28000002,-72.7301444246032));
#166326=CARTESIAN_POINT('Ctrl Pts',(44.6396194153369,-38.28000002,-76.4827983330449));
#166327=CARTESIAN_POINT('Ctrl Pts',(42.6166038138442,-38.28000002,-80.2231699540513));
#166328=CARTESIAN_POINT('Ctrl Pts',(40.5593018105246,-38.28000002,-83.9452341108497));
#166329=CARTESIAN_POINT('Origin',(59.5,-37.78000002,-55.2499500000007));
#166330=CARTESIAN_POINT('',(59.5,-38.28000002,-58.24995));
#166331=CARTESIAN_POINT('Origin',(59.5,-37.78000002,-58.24995));
#166332=CARTESIAN_POINT('',(59.5,-38.28000002,-174.34995));
#166333=CARTESIAN_POINT('',(59.5,-38.28000002,-58.24995));
#166334=CARTESIAN_POINT('Origin',(59.5,-37.78000002,-174.34995));
#166335=CARTESIAN_POINT('Origin',(57.,-37.78000002,-174.34995));
#166336=CARTESIAN_POINT('',(57.,-38.28000002,-176.84995));
#166337=CARTESIAN_POINT('Origin',(57.,-38.28000002,-174.34995));
#166338=CARTESIAN_POINT('Origin',(57.,-37.78000002,-176.84995));
#166339=CARTESIAN_POINT('Origin',(-83.2809572255632,-37.78000002,-176.84995));
#166340=CARTESIAN_POINT('',(-83.2809572255632,-38.28000002,-176.84995));
#166341=CARTESIAN_POINT('Origin',(53.1262583325313,-38.78000002,-179.64995));
#166342=CARTESIAN_POINT('',(53.1262583325313,-38.28000002,-171.916267709546));
#166343=CARTESIAN_POINT('Origin',(53.1262583325313,-38.78000002,-171.916267709546));
#166344=CARTESIAN_POINT('',(52.6451348158641,-38.6439112191758,-179.64995));
#166345=CARTESIAN_POINT('',(53.1262583325313,-38.28000002,-176.84995));
#166346=CARTESIAN_POINT('Ctrl Pts',(52.7704579175044,-38.28000002,-170.960578619515));
#166347=CARTESIAN_POINT('Ctrl Pts',(52.508648517912,-38.28000002,-171.191647032252));
#166348=CARTESIAN_POINT('Ctrl Pts',(52.418503743379,-38.6078427661477,-171.27120723903));
#166349=CARTESIAN_POINT('Ctrl Pts',(52.8865885798003,-38.28000002,-171.092159149585));
#166350=CARTESIAN_POINT('Ctrl Pts',(52.5972087752045,-38.2800000200018,
-171.289280606396));
#166351=CARTESIAN_POINT('Ctrl Pts',(52.4966135335128,-38.6055762491043,
-171.358452481822));
#166352=CARTESIAN_POINT('Ctrl Pts',(52.9752899136351,-38.28000002,-171.24095231752));
#166353=CARTESIAN_POINT('Ctrl Pts',(52.6638881026927,-38.2800000200005,
-171.402873892562));
#166354=CARTESIAN_POINT('Ctrl Pts',(52.5554277399439,-38.6065951776351,
-171.457851777602));
#166355=CARTESIAN_POINT('Ctrl Pts',(53.0969739026007,-38.28000002,-171.570371861396));
#166356=CARTESIAN_POINT('Ctrl Pts',(52.7468873373812,-38.2800000199994,
-171.654013242837));
#166357=CARTESIAN_POINT('Ctrl Pts',(52.6330841414732,-38.6181228329597,
-171.679920679702));
#166358=CARTESIAN_POINT('Ctrl Pts',(53.1262583244907,-38.28000002,-171.740763530748));
#166359=CARTESIAN_POINT('Ctrl Pts',(52.7606056378773,-38.28000002,-171.785522775662));
#166360=CARTESIAN_POINT('Ctrl Pts',(52.6495272179227,-38.6283824768232,
-171.795722243821));
#166361=CARTESIAN_POINT('Ctrl Pts',(53.1262583325313,-38.28000002,-171.916267709546));
#166362=CARTESIAN_POINT('Ctrl Pts',(52.748069378376,-38.28000002,-171.916267709546));
#166363=CARTESIAN_POINT('Ctrl Pts',(52.6451348158641,-38.6439112191758,
-171.916267709546));
#166364=CARTESIAN_POINT('Ctrl Pts',(52.7704579175044,-38.28000002,-170.960578619515));
#166365=CARTESIAN_POINT('Ctrl Pts',(52.8285971612714,-38.28000002,-171.026452630405));
#166366=CARTESIAN_POINT('Ctrl Pts',(52.8797920295936,-38.28000002,-171.096554170654));
#166367=CARTESIAN_POINT('Ctrl Pts',(52.9240704508372,-38.28000002,-171.170767761981));
#166368=CARTESIAN_POINT('Ctrl Pts',(52.9683488720808,-38.28000002,-171.244981353309));
#166369=CARTESIAN_POINT('Ctrl Pts',(53.0057109090821,-38.28000002,-171.323307205357));
#166370=CARTESIAN_POINT('Ctrl Pts',(53.0361319037073,-38.28000002,-171.405662091088));
#166371=CARTESIAN_POINT('Ctrl Pts',(53.0782642785414,-38.28000002,-171.519721705435));
#166372=CARTESIAN_POINT('Ctrl Pts',(53.1052589026234,-38.28000002,-171.636480608475));
#166373=CARTESIAN_POINT('Ctrl Pts',(53.1178820115773,-38.28000002,-171.755802197906));
#166374=CARTESIAN_POINT('Ctrl Pts',(53.1234875228305,-38.28000002,-171.808789026646));
#166375=CARTESIAN_POINT('Ctrl Pts',(53.126258330058,-38.28000002,-171.862281331534));
#166376=CARTESIAN_POINT('Ctrl Pts',(53.1262583325313,-38.28000002,-171.916267709546));
#166377=CARTESIAN_POINT('Ctrl Pts',(49.940073970993,-44.4295309128427,-60.6499502200616));
#166378=CARTESIAN_POINT('Ctrl Pts',(49.940073970993,-44.93000002,-60.6494806725745));
#166379=CARTESIAN_POINT('Ctrl Pts',(49.940073970993,-44.93000002,-61.14995));
#166380=CARTESIAN_POINT('Ctrl Pts',(49.8479774404557,-44.4053128313032,
-60.6499729431522));
#166381=CARTESIAN_POINT('Ctrl Pts',(49.8456458072228,-44.93000002,-60.6246358503761));
#166382=CARTESIAN_POINT('Ctrl Pts',(49.8863992897437,-44.93000002,-61.1499500208808));
#166383=CARTESIAN_POINT('Ctrl Pts',(49.7578649778778,-44.3815585116814,
-60.662149119638));
#166384=CARTESIAN_POINT('Ctrl Pts',(49.7496066417035,-44.93000002,-60.6099006060758));
#166385=CARTESIAN_POINT('Ctrl Pts',(49.8338483436824,-44.93000002,-61.1560263819637));
#166386=CARTESIAN_POINT('Ctrl Pts',(49.5816013859087,-44.3349893071918,
-60.7103063370538));
#166387=CARTESIAN_POINT('Ctrl Pts',(49.5465928271943,-44.93000002,-60.6009208199127));
#166388=CARTESIAN_POINT('Ctrl Pts',(49.7309938571501,-44.93000002,-61.1800821203567));
#166389=CARTESIAN_POINT('Ctrl Pts',(49.4941735011919,-44.3118347483412,
-60.7471802581384));
#166390=CARTESIAN_POINT('Ctrl Pts',(49.4370815776501,-44.9300000199997,
-60.6082512678975));
#166391=CARTESIAN_POINT('Ctrl Pts',(49.6799439551145,-44.93000002,-61.1985082982007));
#166392=CARTESIAN_POINT('Ctrl Pts',(49.3328045849881,-44.269009574368,-60.8440382106835));
#166393=CARTESIAN_POINT('Ctrl Pts',(49.2133831268095,-44.9300000200003,
-60.653509168894));
#166394=CARTESIAN_POINT('Ctrl Pts',(49.5856644732959,-44.93000002,-61.2469206297));
#166395=CARTESIAN_POINT('Ctrl Pts',(49.2582348505417,-44.2491742563957,
-60.9036717632631));
#166396=CARTESIAN_POINT('Ctrl Pts',(49.0983969745462,-44.9300000200002,
-60.6926283936834));
#166397=CARTESIAN_POINT('Ctrl Pts',(49.5420691606389,-44.93000002,-61.2767318781126));
#166398=CARTESIAN_POINT('Ctrl Pts',(49.1235836593332,-44.2132994481138,
-61.0495884892673));
#166399=CARTESIAN_POINT('Ctrl Pts',(48.8650295486972,-44.9300000199998,
-60.8202676220942));
#166400=CARTESIAN_POINT('Ctrl Pts',(49.4633104246523,-44.93000002,-61.3496883835064));
#166401=CARTESIAN_POINT('Ctrl Pts',(49.0660606187868,-44.1979416296537,
-61.1334940119936));
#166402=CARTESIAN_POINT('Ctrl Pts',(48.7523385355526,-44.93000002,-60.9091191391034));
#166403=CARTESIAN_POINT('Ctrl Pts',(49.4296447656355,-44.93000002,-61.3916439172571));
#166404=CARTESIAN_POINT('Ctrl Pts',(49.0216817963636,-44.1860823027988,
-61.2274665920928));
#166405=CARTESIAN_POINT('Ctrl Pts',(48.6578457649038,-44.93000002,-61.0263236351359));
#166406=CARTESIAN_POINT('Ctrl Pts',(49.4036629110189,-44.93000002,-61.4386408691297));
#166407=CARTESIAN_POINT('Ctrl Pts',(49.940073970993,-44.43000002,-60.64995));
#166408=CARTESIAN_POINT('Ctrl Pts',(49.8114787093223,-44.3961999235187,
-60.64995));
#166409=CARTESIAN_POINT('Ctrl Pts',(49.7009578626629,-44.366496043485,-60.6737266630953));
#166410=CARTESIAN_POINT('Ctrl Pts',(49.5662681479033,-44.3309458928829,
-60.7193269101808));
#166411=CARTESIAN_POINT('Ctrl Pts',(49.5264094220829,-44.320504982567,-60.7362560379875));
#166412=CARTESIAN_POINT('Ctrl Pts',(49.4738000033418,-44.306750375621,-60.7618373723648));
#166413=CARTESIAN_POINT('Ctrl Pts',(49.4574561560657,-44.302480786915,-60.7704020732091));
#166414=CARTESIAN_POINT('Ctrl Pts',(49.4346580763186,-44.2965074132954,
-60.7830608683784));
#166415=CARTESIAN_POINT('Ctrl Pts',(49.4236882926368,-44.293628364449,-60.789343778841));
#166416=CARTESIAN_POINT('Ctrl Pts',(49.411624548949,-44.2904477727066,-60.7965449436944));
#166417=CARTESIAN_POINT('Ctrl Pts',(49.4066098784319,-44.2891217552102,
-60.7995988132645));
#166418=CARTESIAN_POINT('Ctrl Pts',(49.4033011158289,-44.2882458627272,
-60.8016270235086));
#166419=CARTESIAN_POINT('Ctrl Pts',(49.4028309549621,-44.2881216419612,
-60.8019125086144));
#166420=CARTESIAN_POINT('Ctrl Pts',(49.2216643765893,-44.2400505684977,
-60.9144220519661));
#166421=CARTESIAN_POINT('Ctrl Pts',(49.0958707926624,-44.2064653114064,
-61.0697892923834));
#166422=CARTESIAN_POINT('Ctrl Pts',(49.0214378669496,-44.1865817238571,
-61.2273317382593));
#166423=CARTESIAN_POINT('Ctrl Pts',(49.4036629110189,-44.93000002,-61.4386408691297));
#166424=CARTESIAN_POINT('Ctrl Pts',(49.421292954971,-44.93000002,-61.4067508873822));
#166425=CARTESIAN_POINT('Ctrl Pts',(49.4424088019263,-44.93000002,-61.3772666862021));
#166426=CARTESIAN_POINT('Ctrl Pts',(49.4663885772137,-44.93000002,-61.3502540659085));
#166427=CARTESIAN_POINT('Ctrl Pts',(49.4778548596161,-44.93000002,-61.33733758404));
#166428=CARTESIAN_POINT('Ctrl Pts',(49.4899767151879,-44.93000002,-61.3249865422103));
#166429=CARTESIAN_POINT('Ctrl Pts',(49.5026897554816,-44.93000002,-61.3132100906898));
#166430=CARTESIAN_POINT('Ctrl Pts',(49.5320647115447,-44.93000002,-61.2859992317605));
#166431=CARTESIAN_POINT('Ctrl Pts',(49.563760885477,-44.93000002,-61.2625146831493));
#166432=CARTESIAN_POINT('Ctrl Pts',(49.597554081752,-44.93000002,-61.2422777750133));
#166433=CARTESIAN_POINT('Ctrl Pts',(49.6090633503044,-44.93000002,-61.2353854997602));
#166434=CARTESIAN_POINT('Ctrl Pts',(49.6208161109919,-44.93000002,-61.2288703265774));
#166435=CARTESIAN_POINT('Ctrl Pts',(49.6328042123455,-44.93000002,-61.2227144603287));
#166436=CARTESIAN_POINT('Ctrl Pts',(49.679945666351,-44.93000002,-61.1985074172725));
#166437=CARTESIAN_POINT('Ctrl Pts',(49.7309938530465,-44.93000002,-61.1800821085049));
#166438=CARTESIAN_POINT('Ctrl Pts',(49.7824210964939,-44.93000002,-61.1680542343897));
#166439=CARTESIAN_POINT('Ctrl Pts',(49.833844605741,-44.93000002,-61.1560272336343));
#166440=CARTESIAN_POINT('Ctrl Pts',(49.8863934436428,-44.93000002,-61.14995));
#166441=CARTESIAN_POINT('Ctrl Pts',(49.940073970993,-44.93000002,-61.14995));
#166442=CARTESIAN_POINT('Ctrl Pts',(52.1700794675439,-38.5802945048887,
-61.2273317382593));
#166443=CARTESIAN_POINT('Ctrl Pts',(52.2861787013546,-38.28000002,-61.287642251635));
#166444=CARTESIAN_POINT('Ctrl Pts',(52.5768547844511,-38.28000002,-61.4386408691297));
#166445=CARTESIAN_POINT('Ctrl Pts',(52.238210979969,-38.595348210897,-61.0819498253042));
#166446=CARTESIAN_POINT('Ctrl Pts',(52.3399181230539,-38.28000002,-61.1584857199633));
#166447=CARTESIAN_POINT('Ctrl Pts',(52.6146146074011,-38.28000002,-61.3659524750795));
#166448=CARTESIAN_POINT('Ctrl Pts',(52.3391546482515,-38.6176244716287,
-60.958102271836));
#166449=CARTESIAN_POINT('Ctrl Pts',(52.4211494089633,-38.28000002,-61.0428817134857));
#166450=CARTESIAN_POINT('Ctrl Pts',(52.6705520955624,-38.28000002,-61.3040259447327));
#166451=CARTESIAN_POINT('Ctrl Pts',(52.4601060488528,-38.6442121687577,
-60.8635779995782));
#166452=CARTESIAN_POINT('Ctrl Pts',(52.5193575501107,-38.28000002,-60.9475523661893));
#166453=CARTESIAN_POINT('Ctrl Pts',(52.7375342894722,-38.28000002,-61.2567639997891));
#166454=CARTESIAN_POINT('',(52.7375342894721,-38.28000002,-61.2567639997892));
#166455=CARTESIAN_POINT('',(52.4601061170824,-38.6442121641745,-60.8635778131262));
#166456=CARTESIAN_POINT('Origin',(52.7375342894721,-38.78000002,-61.2567639997892));
#166457=CARTESIAN_POINT('Origin',(53.0240343600242,-38.7671930235723,-61.6028141108652));
#166458=CARTESIAN_POINT('Origin',(53.0468858549885,-38.28000002,-61.6241485284279));
#166459=CARTESIAN_POINT('Origin',(0.,-12.9675000200281,-60.64995));
#166460=CARTESIAN_POINT('Origin',(0.,-12.9675000200281,-61.2273317382593));
#166461=CARTESIAN_POINT('Origin',(57.,19.76999998,-174.34995));
#166462=CARTESIAN_POINT('',(57.,20.26999998,-176.84995));
#166463=CARTESIAN_POINT('Origin',(57.,19.76999998,-176.84995));
#166464=CARTESIAN_POINT('',(59.5,20.26999998,-174.34995));
#166465=CARTESIAN_POINT('Origin',(57.,20.26999998,-174.34995));
#166466=CARTESIAN_POINT('Origin',(59.5,19.76999998,-174.34995));
#166467=CARTESIAN_POINT('Origin',(59.5,19.76999998,-55.24995));
#166468=CARTESIAN_POINT('',(59.5,20.26999998,-58.24995));
#166469=CARTESIAN_POINT('',(59.5,20.26999998,-174.34995));
#166470=CARTESIAN_POINT('Origin',(59.5,19.76999998,-58.24995));
#166471=CARTESIAN_POINT('Ctrl Pts',(48.5401663778083,20.8005163310888,-60.6557251999476));
#166472=CARTESIAN_POINT('Ctrl Pts',(48.5428568992146,20.2699999800004,-60.6233186082983));
#166473=CARTESIAN_POINT('Ctrl Pts',(48.4967141407694,20.26999998,-61.1528286091218));
#166474=CARTESIAN_POINT('Ctrl Pts',(48.3258603491075,20.7405626834577,-60.6326588680102));
#166475=CARTESIAN_POINT('Ctrl Pts',(48.3312760425999,20.2699999799993,-60.6648966748951));
#166476=CARTESIAN_POINT('Ctrl Pts',(48.368727227854,20.26999998,-61.1413140584609));
#166477=CARTESIAN_POINT('Ctrl Pts',(48.0997023590435,20.6768759439098,-60.6786895616851));
#166478=CARTESIAN_POINT('Ctrl Pts',(48.123617249358,20.2699999800005,-60.7558947672151));
#166479=CARTESIAN_POINT('Ctrl Pts',(48.2334071498883,20.26999998,-61.1643439345927));
#166480=CARTESIAN_POINT('Ctrl Pts',(47.710945097327,20.5668610319491,-60.9089307872898));
#166481=CARTESIAN_POINT('Ctrl Pts',(47.7976044540999,20.2699999799995,-61.0163559243911));
#166482=CARTESIAN_POINT('Ctrl Pts',(48.000500083877,20.26999998,-61.2794769780549));
#166483=CARTESIAN_POINT('Ctrl Pts',(47.5431247912797,20.5190619893355,-61.0949662257924));
#166484=CARTESIAN_POINT('Ctrl Pts',(47.662880268204,20.2699999800005,-61.1871235536955));
#166485=CARTESIAN_POINT('Ctrl Pts',(47.8998003386288,20.26999998,-61.3724531273306));
#166486=CARTESIAN_POINT('Ctrl Pts',(47.4601025565285,20.4953747916186,-61.3483411114119));
#166487=CARTESIAN_POINT('Ctrl Pts',(47.5983464794385,20.2699999799998,-61.4016832893902));
#166488=CARTESIAN_POINT('Ctrl Pts',(47.8499146758921,20.26999998,-61.4991870244405));
#166489=CARTESIAN_POINT('',(47.878929697957,20.26999998,-61.4386408691297));
#166490=CARTESIAN_POINT('Origin',(47.878929697957,20.76999998,-61.4386408691297));
#166491=CARTESIAN_POINT('',(48.4322308821779,20.76999998,-60.64995));
#166492=CARTESIAN_POINT('Ctrl Pts',(48.4322308821779,20.76999998,-60.64995));
#166493=CARTESIAN_POINT('Ctrl Pts',(48.399722578391,20.7608881764303,-60.64995));
#166494=CARTESIAN_POINT('Ctrl Pts',(48.3683266666299,20.7520242857188,-60.6514739673707));
#166495=CARTESIAN_POINT('Ctrl Pts',(48.3381385205148,20.7434793708773,-60.6542240356935));
#166496=CARTESIAN_POINT('Ctrl Pts',(48.3071065638243,20.7346956109777,-60.6570509731531));
#166497=CARTESIAN_POINT('Ctrl Pts',(48.277350510797,20.7262486977711,-60.6611729491662));
#166498=CARTESIAN_POINT('Ctrl Pts',(48.2489294698721,20.7181846607773,-60.6662816822899));
#166499=CARTESIAN_POINT('Ctrl Pts',(48.2196862185314,20.709887334115,-60.6715382092119));
#166500=CARTESIAN_POINT('Ctrl Pts',(48.1918559318809,20.7019950860821,-60.6778389168705));
#166501=CARTESIAN_POINT('Ctrl Pts',(48.1654622162443,20.6945292505851,-60.6848721910989));
#166502=CARTESIAN_POINT('Ctrl Pts',(48.1378677797617,20.6867237742267,-60.6922254278175));
#166503=CARTESIAN_POINT('Ctrl Pts',(48.1118431759175,20.6793841107777,-60.7003788836451));
#166504=CARTESIAN_POINT('Ctrl Pts',(48.0873777720132,20.6725078124747,-60.7090106282434));
#166505=CARTESIAN_POINT('Ctrl Pts',(48.062292478069,20.6654572865626,-60.7178610789184));
#166506=CARTESIAN_POINT('Ctrl Pts',(48.038845789214,20.658893486969,-60.7272140672987));
#166507=CARTESIAN_POINT('Ctrl Pts',(48.016995772979,20.6527917612606,-60.7367639150856));
#166508=CARTESIAN_POINT('Ctrl Pts',(47.9943585023737,20.6464701908538,-60.7466578431389));
#166509=CARTESIAN_POINT('Ctrl Pts',(47.9734344086814,20.6406441600918,-60.756762814792));
#166510=CARTESIAN_POINT('Ctrl Pts',(47.9541541175128,20.6352694937039,-60.7667871712989));
#166511=CARTESIAN_POINT('Ctrl Pts',(47.9467623633479,20.6332089328799,-60.770630348682));
#166512=CARTESIAN_POINT('Ctrl Pts',(47.9396120395958,20.6312145793529,-60.77446218704));
#166513=CARTESIAN_POINT('Ctrl Pts',(47.9326986888512,20.6292835269848,-60.7782681307328));
#166514=CARTESIAN_POINT('Ctrl Pts',(47.9250776896262,20.6271548126834,-60.7824636496649));
#166515=CARTESIAN_POINT('Ctrl Pts',(47.9177446558436,20.6251030197031,-60.7866276814552));
#166516=CARTESIAN_POINT('Ctrl Pts',(47.9106933592237,20.623124049625,-60.7907421586884));
#166517=CARTESIAN_POINT('Ctrl Pts',(47.9071677109137,20.6221345645859,-60.7927993973051));
#166518=CARTESIAN_POINT('Ctrl Pts',(47.9037125043225,20.6211632904805,-60.7948442623793));
#166519=CARTESIAN_POINT('Ctrl Pts',(47.9003269328935,20.6202096924913,-60.7968746421038));
#166520=CARTESIAN_POINT('Ctrl Pts',(47.8986341471789,20.6197328934967,-60.797889831966));
#166521=CARTESIAN_POINT('Ctrl Pts',(47.8969587707282,20.619260513863,-60.7989014014781));
#166522=CARTESIAN_POINT('Ctrl Pts',(47.8953007039598,20.6187924875234,-60.7999090937751));
#166523=CARTESIAN_POINT('Ctrl Pts',(47.8939271861499,20.6184047814762,-60.8007438510618));
#166524=CARTESIAN_POINT('Ctrl Pts',(47.893382665496,20.6182516173075,-60.8010750695854));
#166525=CARTESIAN_POINT('Ctrl Pts',(47.8916362218411,20.6177573754894,-60.8021469852348));
#166526=CARTESIAN_POINT('Ctrl Pts',(47.8912744145753,20.6176549843929,-60.8023690518724));
#166527=CARTESIAN_POINT('Ctrl Pts',(47.8908610878189,20.6175379989838,-60.8026230349715));
#166528=CARTESIAN_POINT('Ctrl Pts',(47.8903783339695,20.6174014028689,-60.8029202868589));
#166529=CARTESIAN_POINT('Ctrl Pts',(47.8567603545224,20.6078891319896,-60.8236202934009));
#166530=CARTESIAN_POINT('Ctrl Pts',(47.8249183854607,20.5988369606764,-60.8459276154961));
#166531=CARTESIAN_POINT('Ctrl Pts',(47.7949209542359,20.5903002472954,-60.8695267047893));
#166532=CARTESIAN_POINT('Ctrl Pts',(47.7643887817459,20.5816113564535,-60.8935464769994));
#166533=CARTESIAN_POINT('Ctrl Pts',(47.7357672715377,20.5734563241395,-60.918903986338));
#166534=CARTESIAN_POINT('Ctrl Pts',(47.7090862256909,20.5658629872418,-60.9452797566578));
#166535=CARTESIAN_POINT('Ctrl Pts',(47.6816764704408,20.558062262072,-60.9723758987336));
#166536=CARTESIAN_POINT('Ctrl Pts',(47.6563143907701,20.5508541852985,-61.0005461949134));
#166537=CARTESIAN_POINT('Ctrl Pts',(47.6329913081009,20.5442391521648,-61.0294657761639));
#166538=CARTESIAN_POINT('Ctrl Pts',(47.6092897534091,20.5375167745173,-61.0588546458253));
#166539=CARTESIAN_POINT('Ctrl Pts',(47.5876935481731,20.5314065997584,-61.089016935168));
#166540=CARTESIAN_POINT('Ctrl Pts',(47.5681564806293,20.5258817901274,-61.1196402525177));
#166541=CARTESIAN_POINT('Ctrl Pts',(47.5481621754662,20.5202276800885,-61.1509802655888));
#166542=CARTESIAN_POINT('Ctrl Pts',(47.5303241501823,20.5151864019244,-61.1828027952977));
#166543=CARTESIAN_POINT('Ctrl Pts',(47.5145598665705,20.5107046588175,-61.2148083010891));
#166544=CARTESIAN_POINT('Ctrl Pts',(47.512505186092,20.510120518726,-61.2189798251225));
#166545=CARTESIAN_POINT('Ctrl Pts',(47.5104856938792,20.5095458537873,-61.2231545095474));
#166546=CARTESIAN_POINT('Ctrl Pts',(47.508501172308,20.508980519813,-61.2273317382593));
#166547=CARTESIAN_POINT('',(48.4322308821779,20.26999998,-61.14995));
#166548=CARTESIAN_POINT('Origin',(48.4322308821779,20.76999998,-61.14995));
#166549=CARTESIAN_POINT('Ctrl Pts',(47.878929697957,20.26999998,-61.4386408691297));
#166550=CARTESIAN_POINT('Ctrl Pts',(47.8974331987387,20.26999998,-61.4062039153374));
#166551=CARTESIAN_POINT('Ctrl Pts',(47.919537961559,20.26999998,-61.3763755387993));
#166552=CARTESIAN_POINT('Ctrl Pts',(47.9444691614871,20.26999998,-61.3492604871255));
#166553=CARTESIAN_POINT('Ctrl Pts',(47.972080538841,20.26999998,-61.319230487531));
#166554=CARTESIAN_POINT('Ctrl Pts',(48.003157746836,20.26999998,-61.2925292835119));
#166555=CARTESIAN_POINT('Ctrl Pts',(48.0365924563169,20.26999998,-61.2692603439464));
#166556=CARTESIAN_POINT('Ctrl Pts',(48.0621704908697,20.26999998,-61.2514592698694));
#166557=CARTESIAN_POINT('Ctrl Pts',(48.0891267715872,20.26999998,-61.2356661036975));
#166558=CARTESIAN_POINT('Ctrl Pts',(48.1169536143029,20.26999998,-61.2219104511051));
#166559=CARTESIAN_POINT('Ctrl Pts',(48.1430951909369,20.26999998,-61.2089878766662));
#166560=CARTESIAN_POINT('Ctrl Pts',(48.1700747212765,20.26999998,-61.1978560977682));
#166561=CARTESIAN_POINT('Ctrl Pts',(48.1976781569078,20.26999998,-61.1884510370574));
#166562=CARTESIAN_POINT('Ctrl Pts',(48.2258927336206,20.26999998,-61.1788377479562));
#166563=CARTESIAN_POINT('Ctrl Pts',(48.2547605141936,20.26999998,-61.171028311645));
#166564=CARTESIAN_POINT('Ctrl Pts',(48.2840750385862,20.26999998,-61.1650052516751));
#166565=CARTESIAN_POINT('Ctrl Pts',(48.3128848180535,20.26999998,-61.1590858982813));
#166566=CARTESIAN_POINT('Ctrl Pts',(48.3421274958275,20.26999998,-61.1548920321836));
#166567=CARTESIAN_POINT('Ctrl Pts',(48.3716073656792,20.26999998,-61.1524557732793));
#166568=CARTESIAN_POINT('Ctrl Pts',(48.391727124007,20.26999998,-61.1507930474726));
#166569=CARTESIAN_POINT('Ctrl Pts',(48.4119573716396,20.26999998,-61.14995));
#166570=CARTESIAN_POINT('Ctrl Pts',(48.4322308821779,20.26999998,-61.14995));
#166571=CARTESIAN_POINT('Ctrl Pts',(40.8552491802306,20.26999998,-73.4195575571114));
#166572=CARTESIAN_POINT('Ctrl Pts',(40.6336903802598,20.26999998,-73.2855702871256));
#166573=CARTESIAN_POINT('Ctrl Pts',(40.5058324224785,20.4814581622114,-73.2082484262411));
#166574=CARTESIAN_POINT('Ctrl Pts',(43.2510347775237,20.26999998,-69.4579320833189));
#166575=CARTESIAN_POINT('Ctrl Pts',(43.0367110660153,20.26999998,-69.2967901887638));
#166576=CARTESIAN_POINT('Ctrl Pts',(42.8933128344149,20.4915183317059,-69.2466191256953));
#166577=CARTESIAN_POINT('Ctrl Pts',(45.5849829096511,20.26999998,-65.4599688790667));
#166578=CARTESIAN_POINT('Ctrl Pts',(45.3606391668745,20.269999980008,-65.3006916020456));
#166579=CARTESIAN_POINT('Ctrl Pts',(45.2204439541918,20.5006239318743,-65.2486577002759));
#166580=CARTESIAN_POINT('Ctrl Pts',(47.878929697957,20.26999998,-61.4386408691297));
#166581=CARTESIAN_POINT('Ctrl Pts',(47.6355531845903,20.26999998,-61.2998079338862));
#166582=CARTESIAN_POINT('Ctrl Pts',(47.508501172308,20.508980519813,-61.2273317382593));
#166583=CARTESIAN_POINT('',(40.8552491802306,20.26999998,-73.4195575571114));
#166584=CARTESIAN_POINT('Origin',(40.8552491802306,20.76999998,-73.4195575571114));
#166585=CARTESIAN_POINT('Ctrl Pts',(40.8552491802306,20.26999998,-73.4195575571114));
#166586=CARTESIAN_POINT('Ctrl Pts',(43.2510477030711,20.26999998,-69.4579107098797));
#166587=CARTESIAN_POINT('Ctrl Pts',(45.5849708137067,20.26999998,-65.4599900833935));
#166588=CARTESIAN_POINT('Ctrl Pts',(47.878929697957,20.26999998,-61.4386408691297));
#166589=CARTESIAN_POINT('Ctrl Pts',(40.5057626875991,20.4815735279761,-73.2082062542032));
#166590=CARTESIAN_POINT('Ctrl Pts',(40.6336137367886,20.26999998,-73.2855239371297));
#166591=CARTESIAN_POINT('Ctrl Pts',(40.8552491802306,20.26999998,-73.4195575571114));
#166592=CARTESIAN_POINT('Ctrl Pts',(40.2348040052479,20.5032631524898,-73.6266590242966));
#166593=CARTESIAN_POINT('Ctrl Pts',(40.36273680226,20.26999998,-73.7004454481632));
#166594=CARTESIAN_POINT('Ctrl Pts',(40.611373197132,20.26999998,-73.8228262549259));
#166595=CARTESIAN_POINT('Ctrl Pts',(40.0115963838279,20.5258775774689,-74.0630752877361));
#166596=CARTESIAN_POINT('Ctrl Pts',(40.140116113121,20.26999998,-74.1289328806859));
#166597=CARTESIAN_POINT('Ctrl Pts',(40.4104980509131,20.26999998,-74.2432272518665));
#166598=CARTESIAN_POINT('Ctrl Pts',(39.6351601117623,20.5724303588935,-74.9618949473625));
#166599=CARTESIAN_POINT('Ctrl Pts',(39.75639920405,20.26999998,-75.0104621522509));
#166600=CARTESIAN_POINT('Ctrl Pts',(40.0717001001047,20.26999998,-75.1087680536759));
#166601=CARTESIAN_POINT('Ctrl Pts',(39.4823650047626,20.5963820683904,-75.4245552669206));
#166602=CARTESIAN_POINT('Ctrl Pts',(39.5971879815112,20.26999998,-75.4662299884762));
#166603=CARTESIAN_POINT('Ctrl Pts',(39.9341806290214,20.26999998,-75.5541367565536));
#166604=CARTESIAN_POINT('Ctrl Pts',(39.116363283268,20.6699824412149,-76.8472597580483));
#166605=CARTESIAN_POINT('Ctrl Pts',(39.1910923623951,20.26999998,-76.8948600995692));
#166606=CARTESIAN_POINT('Ctrl Pts',(39.6047590085956,20.26999998,-76.9230972788123));
#166607=CARTESIAN_POINT('Ctrl Pts',(38.999978189647,20.7198888639429,-77.8132651533063));
#166608=CARTESIAN_POINT('Ctrl Pts',(39.0477122635571,20.2699999800001,-77.8601979059779));
#166609=CARTESIAN_POINT('Ctrl Pts',(39.5000000011617,20.26999998,-77.8518474726923));
#166610=CARTESIAN_POINT('Ctrl Pts',(39.0000000471688,20.7702171638925,-78.7897987614795));
#166611=CARTESIAN_POINT('Ctrl Pts',(38.9997827689182,20.26999998,-78.7897987614795));
#166612=CARTESIAN_POINT('Ctrl Pts',(39.5,20.26999998,-78.7897987614789));
#166613=CARTESIAN_POINT('',(39.5,20.26999998,-78.7897987614789));
#166614=CARTESIAN_POINT('Origin',(39.5,20.76999998,-78.7897987614789));
#166615=CARTESIAN_POINT('Ctrl Pts',(39.5,20.26999998,-78.7897987614789));
#166616=CARTESIAN_POINT('Ctrl Pts',(39.4999999999996,20.26999998,-78.4276754534812));
#166617=CARTESIAN_POINT('Ctrl Pts',(39.5156108303728,20.26999998,-78.0671937952867));
#166618=CARTESIAN_POINT('Ctrl Pts',(39.5473687221686,20.26999998,-77.7085899056868));
#166619=CARTESIAN_POINT('Ctrl Pts',(39.5782679790923,20.26999998,-77.3596815527704));
#166620=CARTESIAN_POINT('Ctrl Pts',(39.6244528955633,20.26999998,-77.0125506150102));
#166621=CARTESIAN_POINT('Ctrl Pts',(39.6864661720935,20.26999998,-76.6674187362214));
#166622=CARTESIAN_POINT('Ctrl Pts',(39.725963031717,20.26999998,-76.4476008821939));
#166623=CARTESIAN_POINT('Ctrl Pts',(39.7718817094829,20.26999998,-76.2285940465882));
#166624=CARTESIAN_POINT('Ctrl Pts',(39.8243734219799,20.26999998,-76.0104569305838));
#166625=CARTESIAN_POINT('Ctrl Pts',(39.9341806286948,20.26999998,-75.5541367564111));
#166626=CARTESIAN_POINT('Ctrl Pts',(40.0717001000673,20.26999998,-75.1087680536983));
#166627=CARTESIAN_POINT('Ctrl Pts',(40.2410990749131,20.26999998,-74.6759976525381));
#166628=CARTESIAN_POINT('Ctrl Pts',(40.3724674808252,20.26999998,-74.3403854814604));
#166629=CARTESIAN_POINT('Ctrl Pts',(40.5227478579286,20.26999998,-74.0122470450776));
#166630=CARTESIAN_POINT('Ctrl Pts',(40.6973553852854,20.26999998,-73.6937223220652));
#166631=CARTESIAN_POINT('Ctrl Pts',(40.7479034874671,20.26999998,-73.60151083216));
#166632=CARTESIAN_POINT('Ctrl Pts',(40.800490685591,20.26999998,-73.510105161834));
#166633=CARTESIAN_POINT('Ctrl Pts',(40.8552491802306,20.26999998,-73.4195575571114));
#166634=CARTESIAN_POINT('Origin',(39.5,20.76999998,-55.24995));
#166635=CARTESIAN_POINT('',(39.5,20.26999998,-153.26884421004));
#166636=CARTESIAN_POINT('Origin',(39.5,20.76999998,-153.26884421004));
#166637=CARTESIAN_POINT('',(39.5,20.26999998,-55.24995));
#166638=CARTESIAN_POINT('Ctrl Pts',(39.,20.76999998,-153.26884421004));
#166639=CARTESIAN_POINT('Ctrl Pts',(39.,20.26999998,-153.26884421004));
#166640=CARTESIAN_POINT('Ctrl Pts',(39.5,20.26999998,-153.26884421004));
#166641=CARTESIAN_POINT('Ctrl Pts',(39.,20.7196410046276,-154.246185133485));
#166642=CARTESIAN_POINT('Ctrl Pts',(39.0479377066243,20.26999998,-154.199194380993));
#166643=CARTESIAN_POINT('Ctrl Pts',(39.5000000013484,20.26999998,-154.20759288104));
#166644=CARTESIAN_POINT('Ctrl Pts',(39.1162573309359,20.6699959324755,-155.207409347787));
#166645=CARTESIAN_POINT('Ctrl Pts',(39.1910773834404,20.26999998,-155.160229045822));
#166646=CARTESIAN_POINT('Ctrl Pts',(39.6046315964214,20.26999998,-155.13174861728));
#166647=CARTESIAN_POINT('Ctrl Pts',(39.4789868412919,20.5968217552646,-156.622386886066));
#166648=CARTESIAN_POINT('Ctrl Pts',(39.5936890623428,20.26999998,-156.580982897093));
#166649=CARTESIAN_POINT('Ctrl Pts',(39.9310881578732,20.26999998,-156.493265246185));
#166650=CARTESIAN_POINT('Ctrl Pts',(39.6331118787012,20.5725600557084,-157.091220397978));
#166651=CARTESIAN_POINT('Ctrl Pts',(39.7543133491109,20.26999998,-157.042666916184));
#166652=CARTESIAN_POINT('Ctrl Pts',(40.0698006899404,20.26999998,-156.944576655439));
#166653=CARTESIAN_POINT('Ctrl Pts',(40.0111570472454,20.5257809479637,-157.994781653225));
#166654=CARTESIAN_POINT('Ctrl Pts',(40.1396850110498,20.26999998,-157.928861059881));
#166655=CARTESIAN_POINT('Ctrl Pts',(40.4100413434116,20.26999998,-157.81469163798));
#166656=CARTESIAN_POINT('Ctrl Pts',(40.2350800433575,20.5031211311407,-158.43226426538));
#166657=CARTESIAN_POINT('Ctrl Pts',(40.3630340966184,20.26999998,-158.358476471872));
#166658=CARTESIAN_POINT('Ctrl Pts',(40.6115602809737,20.26999998,-158.236126075511));
#166659=CARTESIAN_POINT('Ctrl Pts',(40.5058324224674,20.4814581622123,-158.850394545248));
#166660=CARTESIAN_POINT('Ctrl Pts',(40.6336903802489,20.26999998,-158.773072684364));
#166661=CARTESIAN_POINT('Ctrl Pts',(40.8552491802207,20.26999998,-158.639085414378));
#166662=CARTESIAN_POINT('',(40.8552491802207,20.26999998,-158.639085414378));
#166663=CARTESIAN_POINT('Origin',(40.8552491802207,20.76999998,-158.639085414378));
#166664=CARTESIAN_POINT('Ctrl Pts',(40.8552491802207,20.26999998,-158.639085414378));
#166665=CARTESIAN_POINT('Ctrl Pts',(40.6523563183102,20.26999998,-158.303585638821));
#166666=CARTESIAN_POINT('Ctrl Pts',(40.4787269326948,20.26999998,-157.955339387382));
#166667=CARTESIAN_POINT('Ctrl Pts',(40.3280973119772,20.26999998,-157.597074989874));
#166668=CARTESIAN_POINT('Ctrl Pts',(40.2977909470356,20.26999998,-157.524992941704));
#166669=CARTESIAN_POINT('Ctrl Pts',(40.2684157827767,20.26999998,-157.452505284537));
#166670=CARTESIAN_POINT('Ctrl Pts',(40.2399210161217,20.26999998,-157.379634146926));
#166671=CARTESIAN_POINT('Ctrl Pts',(40.0698006898873,20.26999998,-156.944576655372));
#166672=CARTESIAN_POINT('Ctrl Pts',(39.9310881570987,20.26999998,-156.493265246319));
#166673=CARTESIAN_POINT('Ctrl Pts',(39.8222693035354,20.26999998,-156.039426370008));
#166674=CARTESIAN_POINT('Ctrl Pts',(39.7053251420368,20.26999998,-155.551700161656));
#166675=CARTESIAN_POINT('Ctrl Pts',(39.6210196491341,20.26999998,-155.059280307642));
#166676=CARTESIAN_POINT('Ctrl Pts',(39.5680311845015,20.26999998,-154.562356823708));
#166677=CARTESIAN_POINT('Ctrl Pts',(39.5224060219208,20.26999998,-154.134486061611));
#166678=CARTESIAN_POINT('Ctrl Pts',(39.5,20.26999998,-153.703276192992));
#166679=CARTESIAN_POINT('Ctrl Pts',(39.5,20.26999998,-153.26884421004));
#166680=CARTESIAN_POINT('Ctrl Pts',(48.0164881467928,20.26999998,-170.861259130871));
#166681=CARTESIAN_POINT('Ctrl Pts',(47.7727200234913,20.26999998,-171.000183411942));
#166682=CARTESIAN_POINT('Ctrl Pts',(47.6457075325507,20.5094809071607,-171.07256826174));
#166683=CARTESIAN_POINT('Ctrl Pts',(45.6783453674058,20.26999998,-166.758558919217));
#166684=CARTESIAN_POINT('Ctrl Pts',(45.4541703457615,20.2699999799837,-166.918724083766));
#166685=CARTESIAN_POINT('Ctrl Pts',(45.3135333962397,20.5009878795767,-166.96987023406));
#166686=CARTESIAN_POINT('Ctrl Pts',(43.2989471172158,20.26999998,-162.679937821406));
#166687=CARTESIAN_POINT('Ctrl Pts',(43.0850828436089,20.26999998,-162.842145218595));
#166688=CARTESIAN_POINT('Ctrl Pts',(42.941059217223,20.4917195215043,-162.891251079751));
#166689=CARTESIAN_POINT('Ctrl Pts',(40.8552491802207,20.26999998,-158.639085414378));
#166690=CARTESIAN_POINT('Ctrl Pts',(40.6336903802499,20.26999998,-158.773072684364));
#166691=CARTESIAN_POINT('Ctrl Pts',(40.5058324224685,20.4814581622113,-158.850394545248));
#166692=CARTESIAN_POINT('',(48.0164881467928,20.26999998,-170.861259130871));
#166693=CARTESIAN_POINT('Origin',(48.0164881467928,20.76999998,-170.861259130871));
#166694=CARTESIAN_POINT('Ctrl Pts',(48.0164881467928,20.26999998,-170.861259130871));
#166695=CARTESIAN_POINT('Ctrl Pts',(45.678332174125,20.26999998,-166.758535769278));
#166696=CARTESIAN_POINT('Ctrl Pts',(43.29896123138,20.26999998,-162.67996116032));
#166697=CARTESIAN_POINT('Ctrl Pts',(40.8552491802207,20.26999998,-158.639085414378));
#166698=CARTESIAN_POINT('Ctrl Pts',(47.5981304714751,20.4959940009177,-170.953449037984));
#166699=CARTESIAN_POINT('Ctrl Pts',(47.7361803032393,20.2699999799996,-170.899850076481));
#166700=CARTESIAN_POINT('Ctrl Pts',(47.9879536642768,20.26999998,-170.801687503914));
#166701=CARTESIAN_POINT('Ctrl Pts',(47.6795757723456,20.5191819878533,-171.201996012878));
#166702=CARTESIAN_POINT('Ctrl Pts',(47.7994410651643,20.2699999800006,-171.110340027154));
#166703=CARTESIAN_POINT('Ctrl Pts',(48.0368367588952,20.26999998,-170.925976258083));
#166704=CARTESIAN_POINT('Ctrl Pts',(47.8461118288466,20.5665218710759,-171.389416721024));
#166705=CARTESIAN_POINT('Ctrl Pts',(47.9331941373512,20.26999998,-171.282098957825));
#166706=CARTESIAN_POINT('Ctrl Pts',(48.1367170179081,20.26999998,-171.019673785838));
#166707=CARTESIAN_POINT('Ctrl Pts',(48.2369635182516,20.6769092692865,-171.621547588333));
#166708=CARTESIAN_POINT('Ctrl Pts',(48.2608982797316,20.26999998,-171.544336769923));
#166709=CARTESIAN_POINT('Ctrl Pts',(48.370721955878,20.26999998,-171.135742484204));
#166710=CARTESIAN_POINT('Ctrl Pts',(48.4597228298326,20.7395177616212,-171.667100514749));
#166711=CARTESIAN_POINT('Ctrl Pts',(48.4654155591074,20.2699999799989,-171.633931058418));
#166712=CARTESIAN_POINT('Ctrl Pts',(48.5039132591497,20.26999998,-171.158522665518));
#166713=CARTESIAN_POINT('Ctrl Pts',(48.6790987479349,20.8007757752918,-171.644223713054));
#166714=CARTESIAN_POINT('Ctrl Pts',(48.6818136557496,20.2699999800007,-171.676865614123));
#166715=CARTESIAN_POINT('Ctrl Pts',(48.6348374950401,20.26999998,-171.147089237505));
#166716=CARTESIAN_POINT('',(48.5692718988023,20.26999998,-171.14995));
#166717=CARTESIAN_POINT('Origin',(48.5692718988023,20.76999998,-171.14995));
#166718=CARTESIAN_POINT('Ctrl Pts',(48.5692718988023,20.26999998,-171.14995));
#166719=CARTESIAN_POINT('Ctrl Pts',(48.5047948684884,20.26999998,-171.14995));
#166720=CARTESIAN_POINT('Ctrl Pts',(48.4405703346722,20.26999998,-171.141645130582));
#166721=CARTESIAN_POINT('Ctrl Pts',(48.3787338163827,20.26999998,-171.124930042697));
#166722=CARTESIAN_POINT('Ctrl Pts',(48.3356628951308,20.26999998,-171.113287501138));
#166723=CARTESIAN_POINT('Ctrl Pts',(48.2937500450339,20.26999998,-171.097563680329));
#166724=CARTESIAN_POINT('Ctrl Pts',(48.2537194844918,20.26999998,-171.077708139862));
#166725=CARTESIAN_POINT('Ctrl Pts',(48.2190067257616,20.26999998,-171.060490279898));
#166726=CARTESIAN_POINT('Ctrl Pts',(48.1858587814802,20.26999998,-171.04016650214));
#166727=CARTESIAN_POINT('Ctrl Pts',(48.1550885346326,20.26999998,-171.016846515546));
#166728=CARTESIAN_POINT('Ctrl Pts',(48.127107857359,20.26999998,-170.995640672702));
#166729=CARTESIAN_POINT('Ctrl Pts',(48.1010921834753,20.26999998,-170.971956505701));
#166730=CARTESIAN_POINT('Ctrl Pts',(48.0776779540546,20.26999998,-170.945845192496));
#166731=CARTESIAN_POINT('Ctrl Pts',(48.0545175809095,20.26999998,-170.920016977257));
#166732=CARTESIAN_POINT('Ctrl Pts',(48.0339013190985,20.26999998,-170.891813734436));
#166733=CARTESIAN_POINT('Ctrl Pts',(48.0164881467928,20.26999998,-170.861259130871));
#166734=CARTESIAN_POINT('Origin',(1.41024658483895E-14,20.76999998,-171.14995));
#166735=CARTESIAN_POINT('',(50.4557527353536,20.26999998,-171.14995));
#166736=CARTESIAN_POINT('Origin',(50.4557527353536,20.76999998,-171.14995));
#166737=CARTESIAN_POINT('',(48.9127966158122,20.26999998,-171.14995));
#166738=CARTESIAN_POINT('Ctrl Pts',(51.9704940941315,20.26999998,-172.64995));
#166739=CARTESIAN_POINT('Ctrl Pts',(51.5358507252234,20.26999998,-172.64995));
#166740=CARTESIAN_POINT('Ctrl Pts',(51.4753600597607,20.70041342952,-172.64995));
#166741=CARTESIAN_POINT('Ctrl Pts',(51.9704940941145,20.26999998,-172.453565067926));
#166742=CARTESIAN_POINT('Ctrl Pts',(51.5358507252071,20.26999998,-172.511015867074));
#166743=CARTESIAN_POINT('Ctrl Pts',(51.4753600597603,20.7004134295229,-172.51902671195));
#166744=CARTESIAN_POINT('Ctrl Pts',(51.9310694254183,20.26999998,-172.257328160063));
#166745=CARTESIAN_POINT('Ctrl Pts',(51.5060950400989,20.26999998,-172.371853931892));
#166746=CARTESIAN_POINT('Ctrl Pts',(51.4488224064852,20.7022245814263,-172.38820210671));
#166747=CARTESIAN_POINT('Ctrl Pts',(51.7793131221354,20.26999998,-171.894521542842));
#166748=CARTESIAN_POINT('Ctrl Pts',(51.3932840309667,20.26999998,-172.118296873734));
#166749=CARTESIAN_POINT('Ctrl Pts',(51.3466717406587,20.7091961991206,-172.14633102856));
#166750=CARTESIAN_POINT('Ctrl Pts',(51.6670411644938,20.26999998,-171.728129909852));
#166751=CARTESIAN_POINT('Ctrl Pts',(51.3097149387001,20.2699999800017,-172.003556970023));
#166752=CARTESIAN_POINT('Ctrl Pts',(51.2710988980251,20.7143539233764,-172.035403273235));
#166753=CARTESIAN_POINT('Ctrl Pts',(51.3866320792846,20.26999998,-171.450449746589));
#166754=CARTESIAN_POINT('Ctrl Pts',(51.105269719327,20.2699999799983,-171.817687494207));
#166755=CARTESIAN_POINT('Ctrl Pts',(51.0823490791536,20.727235793176,-171.850283164392));
#166756=CARTESIAN_POINT('Ctrl Pts',(51.2186052206426,20.26999998,-171.339270411997));
#166757=CARTESIAN_POINT('Ctrl Pts',(50.9837060031699,20.26999998,-171.746711574348));
#166758=CARTESIAN_POINT('Ctrl Pts',(50.9692463274684,20.7349548730131,-171.776163607997));
#166759=CARTESIAN_POINT('Ctrl Pts',(50.8522330947096,20.26999998,-171.18899099047));
#166760=CARTESIAN_POINT('Ctrl Pts',(50.725270742269,20.26999998,-171.658003579003));
#166761=CARTESIAN_POINT('Ctrl Pts',(50.7226328043762,20.7517858470187,-171.675977326981));
#166762=CARTESIAN_POINT('Ctrl Pts',(50.6540676547286,20.26999998,-171.149950000016));
#166763=CARTESIAN_POINT('Ctrl Pts',(50.5880011641168,20.26999998,-171.640924254979));
#166764=CARTESIAN_POINT('Ctrl Pts',(50.5892430788785,20.760889480001,-171.64995));
#166765=CARTESIAN_POINT('Ctrl Pts',(50.4557527353536,20.26999998,-171.14995));
#166766=CARTESIAN_POINT('Ctrl Pts',(50.4557527353535,20.26999998,-171.64995));
#166767=CARTESIAN_POINT('Ctrl Pts',(50.4557527353536,20.76999998,-171.64995));
#166768=CARTESIAN_POINT('',(51.9704940941315,20.26999998,-172.64995));
#166769=CARTESIAN_POINT('Origin',(51.9704940941315,20.76999998,-172.64995));
#166770=CARTESIAN_POINT('Ctrl Pts',(51.9704940941315,20.26999998,-172.64995));
#166771=CARTESIAN_POINT('Ctrl Pts',(51.9704940941145,20.26999998,-172.453565067926));
#166772=CARTESIAN_POINT('Ctrl Pts',(51.9310694254183,20.26999998,-172.257328160063));
#166773=CARTESIAN_POINT('Ctrl Pts',(51.7793131221354,20.26999998,-171.894521542842));
#166774=CARTESIAN_POINT('Ctrl Pts',(51.6670411644938,20.26999998,-171.728129909852));
#166775=CARTESIAN_POINT('Ctrl Pts',(51.3866320792846,20.26999998,-171.450449746589));
#166776=CARTESIAN_POINT('Ctrl Pts',(51.2186052206426,20.26999998,-171.339270411997));
#166777=CARTESIAN_POINT('Ctrl Pts',(50.8522330947096,20.26999998,-171.18899099047));
#166778=CARTESIAN_POINT('Ctrl Pts',(50.6540676547286,20.26999998,-171.149950000016));
#166779=CARTESIAN_POINT('Ctrl Pts',(50.4557527353536,20.26999998,-171.14995));
#166780=CARTESIAN_POINT('Origin',(51.9704940941315,20.76999998,-171.64995));
#166781=CARTESIAN_POINT('',(51.4753600597607,20.70041342952,-171.64995));
#166782=CARTESIAN_POINT('',(51.9704940941315,20.26999998,-55.24995));
#166783=CARTESIAN_POINT('Origin',(60.,19.76999998,-176.84995));
#166784=CARTESIAN_POINT('',(-83.2809572255632,20.2699999800001,-176.84995));
#166785=CARTESIAN_POINT('Origin',(57.,19.76999998,-58.24995));
#166786=CARTESIAN_POINT('',(57.,20.26999998,-55.74995));
#166787=CARTESIAN_POINT('Origin',(57.,20.26999998,-58.24995));
#166788=CARTESIAN_POINT('',(57.,19.76999998,-55.24995));
#166789=CARTESIAN_POINT('Origin',(57.,19.76999998,-55.74995));
#166790=CARTESIAN_POINT('Origin',(57.,19.76999998,-58.24995));
#166791=CARTESIAN_POINT('Origin',(57.,-2.42462934179819E-14,-58.24995));
#166792=CARTESIAN_POINT('',(57.,19.26999998,-55.24995));
#166793=CARTESIAN_POINT('',(57.,28.41999998,-55.24995));
#166794=CARTESIAN_POINT('Origin',(57.,19.26999998,-58.24995));
#166795=CARTESIAN_POINT('Origin',(57.,19.26999998,-58.24995));
#166796=CARTESIAN_POINT('',(57.,18.76999998,-55.74995));
#166797=CARTESIAN_POINT('Origin',(57.,19.26999998,-55.74995));
#166798=CARTESIAN_POINT('',(59.5,18.76999998,-58.24995));
#166799=CARTESIAN_POINT('Origin',(57.,18.76999998,-58.24995));
#166800=CARTESIAN_POINT('Origin',(59.5,19.26999998,-58.24995));
#166801=CARTESIAN_POINT('Origin',(59.5,19.26999998,-55.24995));
#166802=CARTESIAN_POINT('',(59.5,18.76999998,-174.34995));
#166803=CARTESIAN_POINT('',(59.5,18.76999998,-58.24995));
#166804=CARTESIAN_POINT('Origin',(59.5,19.26999998,-174.34995));
#166805=CARTESIAN_POINT('Origin',(57.,19.26999998,-174.34995));
#166806=CARTESIAN_POINT('',(57.,18.76999998,-176.84995));
#166807=CARTESIAN_POINT('Origin',(57.,18.76999998,-174.34995));
#166808=CARTESIAN_POINT('Origin',(57.,19.26999998,-176.84995));
#166809=CARTESIAN_POINT('Origin',(-83.2809572255632,19.26999998,-176.84995));
#166810=CARTESIAN_POINT('',(-83.2809572255632,18.7699999800001,-176.84995));
#166811=CARTESIAN_POINT('Origin',(52.3218461808875,18.26999998,-171.64995));
#166812=CARTESIAN_POINT('',(52.3218461808875,18.76999998,-172.64995));
#166813=CARTESIAN_POINT('',(52.3218461808875,18.76999998,-55.24995));
#166814=CARTESIAN_POINT('Origin',(52.3218461808875,18.26999998,-172.64995));
#166815=CARTESIAN_POINT('',(51.8267121465167,18.20041342952,-171.64995));
#166816=CARTESIAN_POINT('Ctrl Pts',(50.8069033782914,18.76999998,-171.149950013428));
#166817=CARTESIAN_POINT('Ctrl Pts',(50.8069691716108,18.76999998,-171.65003477338));
#166818=CARTESIAN_POINT('Ctrl Pts',(50.8069692256435,18.2699152183756,-171.649950001854));
#166819=CARTESIAN_POINT('Ctrl Pts',(51.0052855451476,18.76999998,-171.149923566191));
#166820=CARTESIAN_POINT('Ctrl Pts',(50.9417879142081,18.76999998,-171.659221103016));
#166821=CARTESIAN_POINT('Ctrl Pts',(50.9405045947988,18.2608007878192,-171.649930655763));
#166822=CARTESIAN_POINT('Ctrl Pts',(51.2035231560588,18.76999998,-171.188965548735));
#166823=CARTESIAN_POINT('Ctrl Pts',(51.071213531544,18.7699999800004,-171.695281914067));
#166824=CARTESIAN_POINT('Ctrl Pts',(51.0739436419031,18.251693043142,-171.675956808334));
#166825=CARTESIAN_POINT('Ctrl Pts',(51.5699573073986,18.76999998,-171.339270411997));
#166826=CARTESIAN_POINT('Ctrl Pts',(51.3040045310345,18.7699999799997,-171.81002165518));
#166827=CARTESIAN_POINT('Ctrl Pts',(51.3206014184843,18.2348578535175,-171.776157476854));
#166828=CARTESIAN_POINT('Ctrl Pts',(51.7379841660413,18.76999998,-171.450449746589));
#166829=CARTESIAN_POINT('Ctrl Pts',(51.406565936193,18.7699999800021,-171.889069508912));
#166830=CARTESIAN_POINT('Ctrl Pts',(51.4337060393708,18.2271381960672,-171.850276197782));
#166831=CARTESIAN_POINT('Ctrl Pts',(52.0183932512491,18.76999998,-171.728129909852));
#166832=CARTESIAN_POINT('Ctrl Pts',(51.5741992781134,18.769999979998,-172.075284894373));
#166833=CARTESIAN_POINT('Ctrl Pts',(51.6224595301836,18.2142554277381,-172.035396209825));
#166834=CARTESIAN_POINT('Ctrl Pts',(52.1306652088914,18.76999998,-171.894521542842));
#166835=CARTESIAN_POINT('Ctrl Pts',(51.6384601923106,18.76999998,-172.182240159754));
#166836=CARTESIAN_POINT('Ctrl Pts',(51.6980343154967,18.2090973697629,-172.14632470545));
#166837=CARTESIAN_POINT('Ctrl Pts',(52.282447203939,18.76999998,-172.257389581842));
#166838=CARTESIAN_POINT('Ctrl Pts',(51.7248942642808,18.76999998,-172.409795949396));
#166839=CARTESIAN_POINT('Ctrl Pts',(51.8002049408554,18.2021241406569,-172.388239289312));
#166840=CARTESIAN_POINT('Ctrl Pts',(52.3218728744769,18.76999998,-172.453697958274));
#166841=CARTESIAN_POINT('Ctrl Pts',(51.7465600943494,18.769999979999,-172.529747068593));
#166842=CARTESIAN_POINT('Ctrl Pts',(51.8267440903201,18.2003128369917,-172.519113452117));
#166843=CARTESIAN_POINT('Ctrl Pts',(52.3218461673279,18.76999998,-172.650149483381));
#166844=CARTESIAN_POINT('Ctrl Pts',(51.746545387842,18.76999998,-172.650072180543));
#166845=CARTESIAN_POINT('Ctrl Pts',(51.8267261127284,18.2003140627874,-172.650082990805));
#166846=CARTESIAN_POINT('',(50.8071048221096,18.76999998,-171.14995));
#166847=CARTESIAN_POINT('Ctrl Pts',(50.8071048221096,18.76999998,-171.14995));
#166848=CARTESIAN_POINT('Ctrl Pts',(51.0054197414846,18.76999998,-171.149950000016));
#166849=CARTESIAN_POINT('Ctrl Pts',(51.2035851814656,18.76999998,-171.18899099047));
#166850=CARTESIAN_POINT('Ctrl Pts',(51.5699573073986,18.76999998,-171.339270411997));
#166851=CARTESIAN_POINT('Ctrl Pts',(51.7379841660413,18.76999998,-171.450449746589));
#166852=CARTESIAN_POINT('Ctrl Pts',(52.0183932512491,18.76999998,-171.728129909852));
#166853=CARTESIAN_POINT('Ctrl Pts',(52.1306652088914,18.76999998,-171.894521542842));
#166854=CARTESIAN_POINT('Ctrl Pts',(52.2824215121743,18.76999998,-172.257328160063));
#166855=CARTESIAN_POINT('Ctrl Pts',(52.3218461808705,18.76999998,-172.453565067926));
#166856=CARTESIAN_POINT('Ctrl Pts',(52.3218461808875,18.76999998,-172.64995));
#166857=CARTESIAN_POINT('Origin',(50.8071048221096,18.26999998,-171.14995));
#166858=CARTESIAN_POINT('Origin',(1.30574517062348E-14,18.26999998,-171.14995));
#166859=CARTESIAN_POINT('',(50.2136602208993,18.76999998,-171.14995));
#166860=CARTESIAN_POINT('',(50.7368344047584,18.76999998,-171.14995));
#166861=CARTESIAN_POINT('Origin',(50.2136602208993,18.26999998,-171.14995));
#166862=CARTESIAN_POINT('Ctrl Pts',(50.2136602208993,18.2695361161168,-171.64994978483));
#166863=CARTESIAN_POINT('Ctrl Pts',(50.2136602208993,18.76999998,-171.650414079253));
#166864=CARTESIAN_POINT('Ctrl Pts',(50.2136602208993,18.76999998,-171.14995));
#166865=CARTESIAN_POINT('Ctrl Pts',(50.1215246544275,18.2455129162615,-171.649927496752));
#166866=CARTESIAN_POINT('Ctrl Pts',(50.1192121820986,18.769999979997,-171.675053529555));
#166867=CARTESIAN_POINT('Ctrl Pts',(50.1601223770514,18.76999998,-171.149949978729));
#166868=CARTESIAN_POINT('Ctrl Pts',(50.0313961658949,18.2219555745979,-171.637727684223));
#166869=CARTESIAN_POINT('Ctrl Pts',(50.0231831602898,18.76999998,-171.689509542455));
#166870=CARTESIAN_POINT('Ctrl Pts',(50.1077189781947,18.76999998,-171.143861566653));
#166871=CARTESIAN_POINT('Ctrl Pts',(49.8551417349348,18.175783311066,-171.589506214496));
#166872=CARTESIAN_POINT('Ctrl Pts',(49.8203496880657,18.76999998,-171.697765173689));
#166873=CARTESIAN_POINT('Ctrl Pts',(50.005178217729,18.76999998,-171.11977321611));
#166874=CARTESIAN_POINT('Ctrl Pts',(49.7677248232621,18.1528278677084,-171.552585380948));
#166875=CARTESIAN_POINT('Ctrl Pts',(49.7110176447319,18.7699999800001,-171.68998153823));
#166876=CARTESIAN_POINT('Ctrl Pts',(49.9542884930289,18.76999998,-171.101323338366));
#166877=CARTESIAN_POINT('Ctrl Pts',(49.6064083377552,18.1103795873091,-171.455624893693));
#166878=CARTESIAN_POINT('Ctrl Pts',(49.4879820896889,18.7699999799999,-171.643731626876));
#166879=CARTESIAN_POINT('Ctrl Pts',(49.8603247967136,18.76999998,-171.052859322317));
#166880=CARTESIAN_POINT('Ctrl Pts',(49.5319078591071,18.0907307659146,-171.395951487152));
#166881=CARTESIAN_POINT('Ctrl Pts',(49.3735536061473,18.76999998,-171.604097554333));
#166882=CARTESIAN_POINT('Ctrl Pts',(49.8169023670873,18.76999998,-171.023027979234));
#166883=CARTESIAN_POINT('Ctrl Pts',(49.3974552840491,18.0552129145183,-171.250061441532));
#166884=CARTESIAN_POINT('Ctrl Pts',(49.1418918710281,18.76999998,-171.475750795187));
#166885=CARTESIAN_POINT('Ctrl Pts',(49.7384998091177,18.76999998,-170.950084676266));
#166886=CARTESIAN_POINT('Ctrl Pts',(49.3400748423115,18.0400232861332,-171.166250453495));
#166887=CARTESIAN_POINT('Ctrl Pts',(49.0303787392063,18.7699999799994,-171.386822745588));
#166888=CARTESIAN_POINT('Ctrl Pts',(49.7050206304183,18.76999998,-170.908176521547));
#166889=CARTESIAN_POINT('Ctrl Pts',(49.295796129512,18.0282912758315,-171.072436686249));
#166890=CARTESIAN_POINT('Ctrl Pts',(48.9370286803265,18.76999998,-171.270056405085));
#166891=CARTESIAN_POINT('Ctrl Pts',(49.6791770659623,18.76999998,-170.861259130871));
#166892=CARTESIAN_POINT('',(49.6791770659623,18.76999998,-170.861259130871));
#166893=CARTESIAN_POINT('Ctrl Pts',(49.6791770659623,18.76999998,-170.861259130871));
#166894=CARTESIAN_POINT('Ctrl Pts',(49.6968576580123,18.76999998,-170.893357248139));
#166895=CARTESIAN_POINT('Ctrl Pts',(49.7180606234586,18.76999998,-170.923027065572));
#166896=CARTESIAN_POINT('Ctrl Pts',(49.7421669681709,18.76999998,-170.950201836129));
#166897=CARTESIAN_POINT('Ctrl Pts',(49.7534002577178,18.76999998,-170.962864978123));
#166898=CARTESIAN_POINT('Ctrl Pts',(49.7652647303594,18.76999998,-170.974986007307));
#166899=CARTESIAN_POINT('Ctrl Pts',(49.7777010515148,18.76999998,-170.986556367076));
#166900=CARTESIAN_POINT('Ctrl Pts',(49.8071230954839,18.76999998,-171.013929705992));
#166901=CARTESIAN_POINT('Ctrl Pts',(49.8388986066918,18.76999998,-171.037546210365));
#166902=CARTESIAN_POINT('Ctrl Pts',(49.8728019101421,18.76999998,-171.057883544606));
#166903=CARTESIAN_POINT('Ctrl Pts',(49.8840707206928,18.76999998,-171.064643286087));
#166904=CARTESIAN_POINT('Ctrl Pts',(49.8955748425992,18.76999998,-171.071040378572));
#166905=CARTESIAN_POINT('Ctrl Pts',(49.9073066431081,18.76999998,-171.07709133376));
#166906=CARTESIAN_POINT('Ctrl Pts',(49.9542902216173,18.76999998,-171.101324232019));
#166907=CARTESIAN_POINT('Ctrl Pts',(50.0051782135404,18.76999998,-171.119773228098));
#166908=CARTESIAN_POINT('Ctrl Pts',(50.0564485939595,18.76999998,-171.131817408419));
#166909=CARTESIAN_POINT('Ctrl Pts',(50.1077152012182,18.76999998,-171.143860702368));
#166910=CARTESIAN_POINT('Ctrl Pts',(50.1601164670163,18.76999998,-171.14995));
#166911=CARTESIAN_POINT('Ctrl Pts',(50.2136602208993,18.76999998,-171.14995));
#166912=CARTESIAN_POINT('Origin',(49.6791770659623,18.26999998,-170.861259130871));
#166913=CARTESIAN_POINT('Ctrl Pts',(40.7628307834967,18.76999998,-155.145469613787));
#166914=CARTESIAN_POINT('Ctrl Pts',(39.9612665046713,18.76999998,-155.616375074053));
#166915=CARTESIAN_POINT('Ctrl Pts',(40.4031453149964,17.9943646866131,-155.356778744658));
#166916=CARTESIAN_POINT('Ctrl Pts',(43.8140202568649,18.76999998,-160.339133090562));
#166917=CARTESIAN_POINT('Ctrl Pts',(42.9502082118644,18.76999998,-160.637466725898));
#166918=CARTESIAN_POINT('Ctrl Pts',(43.4443793123589,18.0073632340302,-160.550451772752));
#166919=CARTESIAN_POINT('Ctrl Pts',(46.773026135633,18.76999998,-165.585306091383));
#166920=CARTESIAN_POINT('Ctrl Pts',(45.9568836537051,18.7699999799361,-165.904661000913));
#166921=CARTESIAN_POINT('Ctrl Pts',(46.3957674250336,18.0186733043079,-165.796619822254));
#166922=CARTESIAN_POINT('Ctrl Pts',(49.6791770659623,18.76999998,-170.861259130871));
#166923=CARTESIAN_POINT('Ctrl Pts',(48.9379852680023,18.76999998,-171.26952948831));
#166924=CARTESIAN_POINT('Ctrl Pts',(49.2955572616308,18.0287857662076,-171.07256826174));
#166925=CARTESIAN_POINT('',(40.7628307834967,18.76999998,-155.145469613787));
#166926=CARTESIAN_POINT('Ctrl Pts',(40.7628307834967,18.76999998,-155.145469613787));
#166927=CARTESIAN_POINT('Ctrl Pts',(43.8140512781903,18.76999998,-160.339185894338));
#166928=CARTESIAN_POINT('Ctrl Pts',(46.7729974319751,18.76999998,-165.585253981682));
#166929=CARTESIAN_POINT('Ctrl Pts',(49.6791770659623,18.76999998,-170.861259130871));
#166930=CARTESIAN_POINT('Origin',(40.7628307834967,18.26999998,-155.145469613787));
#166931=CARTESIAN_POINT('Ctrl Pts',(40.4031453149963,17.9943646866131,-155.356778744658));
#166932=CARTESIAN_POINT('Ctrl Pts',(39.9612665046713,18.76999998,-155.616375074053));
#166933=CARTESIAN_POINT('Ctrl Pts',(40.7628307834967,18.76999998,-155.145469613787));
#166934=CARTESIAN_POINT('Ctrl Pts',(40.1535949024652,18.0152331222464,-154.959221008645));
#166935=CARTESIAN_POINT('Ctrl Pts',(39.7648410678857,18.76999998,-155.176920406762));
#166936=CARTESIAN_POINT('Ctrl Pts',(40.5382265796732,18.76999998,-154.763153570891));
#166937=CARTESIAN_POINT('Ctrl Pts',(39.9463699385113,18.0368966498548,-154.546270136328));
#166938=CARTESIAN_POINT('Ctrl Pts',(39.5997667004894,18.76999998,-154.717664579548));
#166939=CARTESIAN_POINT('Ctrl Pts',(40.3517329455581,18.76999998,-154.366209991013));
#166940=CARTESIAN_POINT('Ctrl Pts',(39.5960425666541,18.0813960858844,-153.697271402021));
#166941=CARTESIAN_POINT('Ctrl Pts',(39.3360417060011,18.76999998,-153.799575452297));
#166942=CARTESIAN_POINT('Ctrl Pts',(40.0364383090907,18.76999998,-153.550444480173));
#166943=CARTESIAN_POINT('Ctrl Pts',(39.4532556977585,18.1042418116532,-153.261037480867));
#166944=CARTESIAN_POINT('Ctrl Pts',(39.23220455254,18.76999998,-153.338508255374));
#166945=CARTESIAN_POINT('Ctrl Pts',(39.9079301282699,18.76999998,-153.131458232674));
#166946=CARTESIAN_POINT('Ctrl Pts',(39.2248664505887,18.1509702537189,-152.367727156036));
#166947=CARTESIAN_POINT('Ctrl Pts',(39.0797143668984,18.76999998,-152.409570079113));
#166948=CARTESIAN_POINT('Ctrl Pts',(39.7023798052426,18.76999998,-152.273874561686));
#166949=CARTESIAN_POINT('Ctrl Pts',(39.1404609620539,18.1746678021094,-151.914185519153));
#166950=CARTESIAN_POINT('Ctrl Pts',(39.0281802867267,18.76999998,-151.943644934638));
#166951=CARTESIAN_POINT('Ctrl Pts',(39.6264148660465,18.76999998,-151.83867201801));
#166952=CARTESIAN_POINT('Ctrl Pts',(39.0282127872062,18.2221486757409,-151.004139862532));
#166953=CARTESIAN_POINT('Ctrl Pts',(38.9776025606259,18.76999998,-151.019307709025));
#166954=CARTESIAN_POINT('Ctrl Pts',(39.5253915082876,18.76999998,-150.965860868517));
#166955=CARTESIAN_POINT('Ctrl Pts',(39.,18.2460151034934,-150.546047809514));
#166956=CARTESIAN_POINT('Ctrl Pts',(38.9754245522527,18.76999998,-150.557403393481));
#166957=CARTESIAN_POINT('Ctrl Pts',(39.5000000006086,18.76999998,-150.526727576342));
#166958=CARTESIAN_POINT('Ctrl Pts',(39.,18.26999998,-150.084863924608));
#166959=CARTESIAN_POINT('Ctrl Pts',(39.,18.76999998,-150.084863924608));
#166960=CARTESIAN_POINT('Ctrl Pts',(39.5,18.76999998,-150.084863924608));
#166961=CARTESIAN_POINT('',(39.5,18.76999998,-150.084863924608));
#166962=CARTESIAN_POINT('Ctrl Pts',(39.5,18.76999998,-150.084863924608));
#166963=CARTESIAN_POINT('Ctrl Pts',(39.5,18.76999998,-150.526736484781));
#166964=CARTESIAN_POINT('Ctrl Pts',(39.5253915082895,18.76999998,-150.965860868514));
#166965=CARTESIAN_POINT('Ctrl Pts',(39.5759031870658,18.76999998,-151.402266443275));
#166966=CARTESIAN_POINT('Ctrl Pts',(39.6264148658422,18.76999998,-151.838672018036));
#166967=CARTESIAN_POINT('Ctrl Pts',(39.7023798052339,18.76999998,-152.273874561637));
#166968=CARTESIAN_POINT('Ctrl Pts',(39.8051549665991,18.76999998,-152.702666397218));
#166969=CARTESIAN_POINT('Ctrl Pts',(39.9079301279644,18.76999998,-153.131458232799));
#166970=CARTESIAN_POINT('Ctrl Pts',(40.0364383090913,18.76999998,-153.550444480149));
#166971=CARTESIAN_POINT('Ctrl Pts',(40.1940856267786,18.76999998,-153.958327235804));
#166972=CARTESIAN_POINT('Ctrl Pts',(40.3268328904507,18.76999998,-154.301785789407));
#166973=CARTESIAN_POINT('Ctrl Pts',(40.4800174576109,18.76999998,-154.637456687545));
#166974=CARTESIAN_POINT('Ctrl Pts',(40.6592112616996,18.76999998,-154.963216752103));
#166975=CARTESIAN_POINT('Ctrl Pts',(40.6928235206461,18.76999998,-155.024321161935));
#166976=CARTESIAN_POINT('Ctrl Pts',(40.7273510343294,18.76999998,-155.085076813206));
#166977=CARTESIAN_POINT('Ctrl Pts',(40.7628307834967,18.76999998,-155.145469613787));
#166978=CARTESIAN_POINT('Origin',(39.5,18.26999998,-150.084863924608));
#166979=CARTESIAN_POINT('Origin',(39.5,18.26999998,-55.24995));
#166980=CARTESIAN_POINT('',(39.5,18.76999998,-81.9737790469184));
#166981=CARTESIAN_POINT('',(39.5,18.76999998,-55.24995));
#166982=CARTESIAN_POINT('Origin',(39.5,18.26999998,-81.9737790469175));
#166983=CARTESIAN_POINT('Ctrl Pts',(39.,18.2699999800011,-81.9737790469193));
#166984=CARTESIAN_POINT('Ctrl Pts',(39.0000000000011,18.76999998,-81.9737790469193));
#166985=CARTESIAN_POINT('Ctrl Pts',(39.5,18.76999998,-81.9737790469184));
#166986=CARTESIAN_POINT('Ctrl Pts',(38.9999999999983,18.2220313158448,-81.0514322138321));
#166987=CARTESIAN_POINT('Ctrl Pts',(38.9495856510588,18.76999998,-81.0044062795137));
#166988=CARTESIAN_POINT('Ctrl Pts',(39.5000000014778,18.76999998,-81.0900715307985));
#166989=CARTESIAN_POINT('Ctrl Pts',(39.1098638639319,18.1747125385734,-80.1448153615248));
#166990=CARTESIAN_POINT('Ctrl Pts',(39.0100135050444,18.76999998,-80.0786830893324));
#166991=CARTESIAN_POINT('Ctrl Pts',(39.5988774762002,18.76999998,-80.2205083311056));
#166992=CARTESIAN_POINT('Ctrl Pts',(39.4494341483978,18.1049192927842,-78.810548635267));
#166993=CARTESIAN_POINT('Ctrl Pts',(39.229508253648,18.7699999800001,-78.7338553009239));
#166994=CARTESIAN_POINT('Ctrl Pts',(39.9044907342272,18.76999998,-78.9396134649389));
#166995=CARTESIAN_POINT('Ctrl Pts',(39.5935190801229,18.0817455339462,-78.3680408652321));
#166996=CARTESIAN_POINT('Ctrl Pts',(39.3342349384753,18.76999998,-78.2659886991342));
#166997=CARTESIAN_POINT('Ctrl Pts',(40.0341671712988,18.76999998,-78.514605681855));
#166998=CARTESIAN_POINT('Ctrl Pts',(39.9457414385913,18.036947832209,-77.5133471330197));
#166999=CARTESIAN_POINT('Ctrl Pts',(39.5993180096537,18.76999998,-77.3418642254583));
#167000=CARTESIAN_POINT('Ctrl Pts',(40.3511672955439,18.76999998,-77.6933701733068));
#167001=CARTESIAN_POINT('Ctrl Pts',(40.1537986734602,18.0152160834001,-77.0990973343972));
#167002=CARTESIAN_POINT('Ctrl Pts',(39.7649903796933,18.76999998,-76.8813885224012));
#167003=CARTESIAN_POINT('Ctrl Pts',(40.5384105179099,18.76999998,-77.2951763044633));
#167004=CARTESIAN_POINT('Ctrl Pts',(40.4031453149964,17.9943646866131,-76.7018642268486));
#167005=CARTESIAN_POINT('Ctrl Pts',(39.9612665046713,18.76999998,-76.4422678974524));
#167006=CARTESIAN_POINT('Ctrl Pts',(40.7628307834967,18.76999998,-76.913173357719));
#167007=CARTESIAN_POINT('',(40.7628307834967,18.76999998,-76.9131733577189));
#167008=CARTESIAN_POINT('Ctrl Pts',(40.7628307834967,18.76999998,-76.913173357719));
#167009=CARTESIAN_POINT('Ctrl Pts',(40.5548564785643,18.76999998,-77.267182363376));
#167010=CARTESIAN_POINT('Ctrl Pts',(40.3788354530892,18.76999998,-77.6350438334274));
#167011=CARTESIAN_POINT('Ctrl Pts',(40.2280138947792,18.76999998,-78.013829837117));
#167012=CARTESIAN_POINT('Ctrl Pts',(40.2160748553597,18.76999998,-78.043814549384));
#167013=CARTESIAN_POINT('Ctrl Pts',(40.2042937476386,18.76999998,-78.073867728607));
#167014=CARTESIAN_POINT('Ctrl Pts',(40.1926672329271,18.76999998,-78.1039879273901));
#167015=CARTESIAN_POINT('Ctrl Pts',(40.0341671712826,18.76999998,-78.5146056819203));
#167016=CARTESIAN_POINT('Ctrl Pts',(39.9044907334798,18.76999998,-78.9396134648084));
#167017=CARTESIAN_POINT('Ctrl Pts',(39.802619647733,18.76999998,-79.366578420212));
#167018=CARTESIAN_POINT('Ctrl Pts',(39.6899907885241,18.76999998,-79.8386316578581));
#167019=CARTESIAN_POINT('Ctrl Pts',(39.6094172115555,18.76999998,-80.3154017457566));
#167020=CARTESIAN_POINT('Ctrl Pts',(39.5598665237953,18.76999998,-80.7967368113108));
#167021=CARTESIAN_POINT('Ctrl Pts',(39.5197815285328,18.76999998,-81.1861222001839));
#167022=CARTESIAN_POINT('Ctrl Pts',(39.4999999999993,18.76999998,-81.5784952288498));
#167023=CARTESIAN_POINT('Ctrl Pts',(39.5,18.76999998,-81.9737790469184));
#167024=CARTESIAN_POINT('Origin',(40.7628307834967,18.26999998,-76.9131733577189));
#167025=CARTESIAN_POINT('Ctrl Pts',(49.5462350640495,18.76999998,-61.4386408691297));
#167026=CARTESIAN_POINT('Ctrl Pts',(48.8042785465888,18.76999998,-61.0296382684995));
#167027=CARTESIAN_POINT('Ctrl Pts',(49.1629069712534,18.0283224583225,-61.2273317382593));
#167028=CARTESIAN_POINT('Ctrl Pts',(46.6827176097033,18.76999998,-66.6332421622494));
#167029=CARTESIAN_POINT('Ctrl Pts',(45.867410270929,18.769999980105,-66.3106234612426));
#167030=CARTESIAN_POINT('Ctrl Pts',(46.3056933853622,18.0183276393305,-66.4219286454218));
#167031=CARTESIAN_POINT('Ctrl Pts',(43.7675014857899,18.76999998,-71.7986930470318));
#167032=CARTESIAN_POINT('Ctrl Pts',(42.9058979134104,18.76999998004,-71.4956126488948));
#167033=CARTESIAN_POINT('Ctrl Pts',(43.3980120961201,18.0071650557604,-71.5873748987318));
#167034=CARTESIAN_POINT('Ctrl Pts',(40.7628307834967,18.76999998,-76.913173357719));
#167035=CARTESIAN_POINT('Ctrl Pts',(39.9612665046713,18.76999998,-76.4422678974524));
#167036=CARTESIAN_POINT('Ctrl Pts',(40.4031453149964,17.9943646866131,-76.7018642268486));
#167037=CARTESIAN_POINT('',(49.5462350640495,18.76999998,-61.4386408691297));
#167038=CARTESIAN_POINT('Ctrl Pts',(49.5462350640495,18.76999998,-61.4386408691297));
#167039=CARTESIAN_POINT('Ctrl Pts',(46.6826907236407,18.76999998,-66.6332909352423));
#167040=CARTESIAN_POINT('Ctrl Pts',(43.7675305143725,18.76999998,-71.7986436352564));
#167041=CARTESIAN_POINT('Ctrl Pts',(40.7628307834967,18.76999998,-76.9131733577189));
#167042=CARTESIAN_POINT('',(49.1629069712534,18.0283224583225,-61.2273317382593));
#167043=CARTESIAN_POINT('Origin',(49.5462350640495,18.26999998,-61.4386408691297));
#167044=CARTESIAN_POINT('Ctrl Pts',(40.4031453149964,17.9943646866131,-76.7018642268486));
#167045=CARTESIAN_POINT('Ctrl Pts',(40.9712467296026,17.9967928105837,-75.7316879770719));
#167046=CARTESIAN_POINT('Ctrl Pts',(41.5465254248927,17.9992060627235,-74.7420551953058));
#167047=CARTESIAN_POINT('Ctrl Pts',(42.128923600295,18.0016015174866,-73.7329075612711));
#167048=CARTESIAN_POINT('Ctrl Pts',(42.6901148582909,18.0039097463388,-72.7605061112557));
#167049=CARTESIAN_POINT('Ctrl Pts',(43.2579165046237,18.0062014493159,-71.7699850988452));
#167050=CARTESIAN_POINT('Ctrl Pts',(43.8323178965797,18.0084744664279,-70.7613168444979));
#167051=CARTESIAN_POINT('Ctrl Pts',(44.3962696818231,18.0107061324303,-69.7709984526495));
#167052=CARTESIAN_POINT('Ctrl Pts',(44.966583117755,18.0129197841333,-68.7631869984356));
#167053=CARTESIAN_POINT('Ctrl Pts',(45.5432901010871,18.0151138514758,-67.7378813099146));
#167054=CARTESIAN_POINT('Ctrl Pts',(46.1330667662012,18.0173576420969,-66.6893395249608));
#167055=CARTESIAN_POINT('Ctrl Pts',(46.7295295612902,18.0195809446279,-65.6225012995692));
#167056=CARTESIAN_POINT('Ctrl Pts',(47.3327621588231,18.0217826463812,-64.5373949188219));
#167057=CARTESIAN_POINT('Ctrl Pts',(47.8996793987642,18.0238518029325,-63.5176133007002));
#167058=CARTESIAN_POINT('Ctrl Pts',(48.4725760817027,18.0259018832755,-62.481696975236));
#167059=CARTESIAN_POINT('Ctrl Pts',(49.0515658068575,18.0279324735353,-61.4296957260205));
#167060=CARTESIAN_POINT('Ctrl Pts',(49.0886544988738,18.0280625482732,-61.3623070511654));
#167061=CARTESIAN_POINT('Ctrl Pts',(49.1257682082662,18.0281925432139,-61.2948523829536));
#167062=CARTESIAN_POINT('Ctrl Pts',(49.1629069712534,18.0283224583225,-61.2273317382593));
#167063=CARTESIAN_POINT('Origin',(-83.2809572255632,18.26999998,-61.14995));
#167064=CARTESIAN_POINT('',(50.0811190791972,18.26999998,-60.64995));
#167065=CARTESIAN_POINT('',(50.0811190791972,18.76999998,-61.14995));
#167066=CARTESIAN_POINT('Origin',(50.0811190791972,18.26999998,-61.14995));
#167067=CARTESIAN_POINT('',(51.394983875096,18.76999998,-61.14995));
#167068=CARTESIAN_POINT('',(-83.2809572255632,18.7699999800001,-61.14995));
#167069=CARTESIAN_POINT('',(51.394983875096,18.26999998,-60.64995));
#167070=CARTESIAN_POINT('Origin',(51.394983875096,18.26999998,-61.14995));
#167071=CARTESIAN_POINT('',(1.30574517062348E-14,18.26999998,-60.64995));
#167072=CARTESIAN_POINT('Ctrl Pts',(49.1629069712534,18.0283224583225,-61.2273317382593));
#167073=CARTESIAN_POINT('Ctrl Pts',(48.8042785465888,18.76999998,-61.0296382684994));
#167074=CARTESIAN_POINT('Ctrl Pts',(49.5462350640495,18.76999998,-61.4386408691297));
#167075=CARTESIAN_POINT('Ctrl Pts',(49.2072136788996,18.0400790290492,-61.1335104039183));
#167076=CARTESIAN_POINT('Ctrl Pts',(48.8976639972856,18.7699999800003,-60.912976735742));
#167077=CARTESIAN_POINT('Ctrl Pts',(49.5720983755525,18.76999998,-61.3917233465932));
#167078=CARTESIAN_POINT('Ctrl Pts',(49.2636489250068,18.0550404895701,-61.0510932718963));
#167079=CARTESIAN_POINT('Ctrl Pts',(49.0074625403989,18.7699999800005,-60.8254916046238));
#167080=CARTESIAN_POINT('Ctrl Pts',(49.6050257059303,18.76999998,-61.3505216375984));
#167081=CARTESIAN_POINT('Ctrl Pts',(49.3970153298707,18.0903238932961,-60.9057963508575));
#167082=CARTESIAN_POINT('Ctrl Pts',(49.2376424762765,18.7699999799996,-60.6973789326117));
#167083=CARTESIAN_POINT('Ctrl Pts',(49.6828096124638,18.76999998,-61.2778731737785));
#167084=CARTESIAN_POINT('Ctrl Pts',(49.4723725947842,18.1102284712985,-60.8450701877959));
#167085=CARTESIAN_POINT('Ctrl Pts',(49.3535760550633,18.7699999800002,-60.656860805429));
#167086=CARTESIAN_POINT('Ctrl Pts',(49.7267438680042,18.76999998,-61.2475100972213));
#167087=CARTESIAN_POINT('Ctrl Pts',(49.7151670266325,18.1742094267258,-60.6988289354793));
#167088=CARTESIAN_POINT('Ctrl Pts',(49.6800903574717,18.7699999799997,-60.5889551600382));
#167089=CARTESIAN_POINT('Ctrl Pts',(49.8682179142305,18.76999998,-61.1743894610928));
#167090=CARTESIAN_POINT('Ctrl Pts',(49.897617121419,18.2220908968247,-60.64995));
#167091=CARTESIAN_POINT('Ctrl Pts',(49.8890563478339,18.76999998,-60.5998057785282));
#167092=CARTESIAN_POINT('Ctrl Pts',(49.9744290136678,18.76999998,-61.1499500118827));
#167093=CARTESIAN_POINT('Ctrl Pts',(50.0811190791972,18.26999998,-60.64995));
#167094=CARTESIAN_POINT('Ctrl Pts',(50.0811190791972,18.76999998,-60.64995));
#167095=CARTESIAN_POINT('Ctrl Pts',(50.0811190791972,18.76999998,-61.14995));
#167096=CARTESIAN_POINT('Ctrl Pts',(50.0811190791972,18.76999998,-61.14995));
#167097=CARTESIAN_POINT('Ctrl Pts',(50.0253653304668,18.76999998,-61.14995));
#167098=CARTESIAN_POINT('Ctrl Pts',(49.9698122997697,18.76999998,-61.156619759286));
#167099=CARTESIAN_POINT('Ctrl Pts',(49.9160272892494,18.76999998,-61.1699168656484));
#167100=CARTESIAN_POINT('Ctrl Pts',(49.8667673647609,18.76999998,-61.1820952486029));
#167101=CARTESIAN_POINT('Ctrl Pts',(49.8189890147709,18.76999998,-61.1998333372795));
#167102=CARTESIAN_POINT('Ctrl Pts',(49.7739018815407,18.76999998,-61.2231365482226));
#167103=CARTESIAN_POINT('Ctrl Pts',(49.7267405569306,18.76999998,-61.2475118015823));
#167104=CARTESIAN_POINT('Ctrl Pts',(49.6828095888518,18.76999998,-61.2778731395778));
#167105=CARTESIAN_POINT('Ctrl Pts',(49.6439176192587,18.76999998,-61.3141973629269));
#167106=CARTESIAN_POINT('Ctrl Pts',(49.6050311049514,18.76999998,-61.3505164911619));
#167107=CARTESIAN_POINT('Ctrl Pts',(49.572103750808,18.76999998,-61.3917134395509));
#167108=CARTESIAN_POINT('Ctrl Pts',(49.5462350640495,18.76999998,-61.4386408691297));
#167109=CARTESIAN_POINT('Ctrl Pts',(49.1629069712534,18.0283224583225,-61.2273317382593));
#167110=CARTESIAN_POINT('Ctrl Pts',(49.1758556443986,18.0317583367506,-61.1999123610635));
#167111=CARTESIAN_POINT('Ctrl Pts',(49.1902712257389,18.0355823155541,-61.1725636295363));
#167112=CARTESIAN_POINT('Ctrl Pts',(49.2062471139611,18.0398182108422,-61.1455207345201));
#167113=CARTESIAN_POINT('Ctrl Pts',(49.2132121160929,18.0416649325582,-61.1337308534933));
#167114=CARTESIAN_POINT('Ctrl Pts',(49.2204732095182,18.0435898179205,-61.121998672147));
#167115=CARTESIAN_POINT('Ctrl Pts',(49.2280358572725,18.0455942231795,-61.1103416139779));
#167116=CARTESIAN_POINT('Ctrl Pts',(49.242774003619,18.0495004236274,-61.0876242489957));
#167117=CARTESIAN_POINT('Ctrl Pts',(49.2586567334235,18.0537084504928,-61.0651969160208));
#167118=CARTESIAN_POINT('Ctrl Pts',(49.2757017806171,18.0582222363407,-61.0431801156955));
#167119=CARTESIAN_POINT('Ctrl Pts',(49.2863389361599,18.0610391157312,-61.0294402810704));
#167120=CARTESIAN_POINT('Ctrl Pts',(49.297428296039,18.0639749488797,-61.015859905788));
#167121=CARTESIAN_POINT('Ctrl Pts',(49.3089695099989,18.0670294385391,-61.0024639978232));
#167122=CARTESIAN_POINT('Ctrl Pts',(49.3159220123172,18.068869482967,-60.9943942157791));
#167123=CARTESIAN_POINT('Ctrl Pts',(49.3230396086335,18.070752883333,-60.9863896947236));
#167124=CARTESIAN_POINT('Ctrl Pts',(49.3303321274388,18.0726821914331,-60.9784448113769));
#167125=CARTESIAN_POINT('Ctrl Pts',(49.3443907684802,18.0764015442057,-60.9631285309434));
#167126=CARTESIAN_POINT('Ctrl Pts',(49.3590252215099,18.0802718191738,-60.9481340775816));
#167127=CARTESIAN_POINT('Ctrl Pts',(49.3742621817036,18.0842997443489,-60.93348331691));
#167128=CARTESIAN_POINT('Ctrl Pts',(49.3852323673815,18.0871997379504,-60.9229351785118));
#167129=CARTESIAN_POINT('Ctrl Pts',(49.3965149012616,18.0901814586669,-60.9125653703328));
#167130=CARTESIAN_POINT('Ctrl Pts',(49.4081198851036,18.093247433935,-60.9023849264265));
#167131=CARTESIAN_POINT('Ctrl Pts',(49.4184695181154,18.0959817521625,-60.8933057359888));
#167132=CARTESIAN_POINT('Ctrl Pts',(49.4290760983762,18.0987832097414,-60.8843771910698));
#167133=CARTESIAN_POINT('Ctrl Pts',(49.4399282538534,18.1016486941697,-60.8756225366125));
#167134=CARTESIAN_POINT('Ctrl Pts',(49.4666824192631,18.1087130644264,-60.8540394074407));
#167135=CARTESIAN_POINT('Ctrl Pts',(49.4949459316395,18.1161710329613,-60.8335002902348));
#167136=CARTESIAN_POINT('Ctrl Pts',(49.5246636596379,18.1240062279754,-60.8142280794331));
#167137=CARTESIAN_POINT('Ctrl Pts',(49.5282089615409,18.1249409606641,-60.8119289196308));
#167138=CARTESIAN_POINT('Ctrl Pts',(49.5322455216986,18.1260051114224,-60.8093481622553));
#167139=CARTESIAN_POINT('Ctrl Pts',(49.5358597613694,18.1269578466203,-60.8070708522197));
#167140=CARTESIAN_POINT('Ctrl Pts',(49.5378245064206,18.1274757651691,-60.8058328785295));
#167141=CARTESIAN_POINT('Ctrl Pts',(49.5396639643064,18.1279606345221,-60.804683593521));
#167142=CARTESIAN_POINT('Ctrl Pts',(49.5412286251171,18.1283730633644,-60.8037112597476));
#167143=CARTESIAN_POINT('Ctrl Pts',(49.5452063921231,18.1294215627134,-60.8012393392033));
#167144=CARTESIAN_POINT('Ctrl Pts',(49.5492314114211,18.130482391578,-60.7987761186316));
#167145=CARTESIAN_POINT('Ctrl Pts',(49.5533040478086,18.1315556397923,-60.7963230567551));
#167146=CARTESIAN_POINT('Ctrl Pts',(49.5780259154611,18.1380705106986,-60.7814323900504));
#167147=CARTESIAN_POINT('Ctrl Pts',(49.60446489505,18.1450328864082,-60.7669291728874));
#167148=CARTESIAN_POINT('Ctrl Pts',(49.6326921477065,18.1524603198153,-60.7531665994733));
#167149=CARTESIAN_POINT('Ctrl Pts',(49.6413659131076,18.1547426466039,-60.7489375894962));
#167150=CARTESIAN_POINT('Ctrl Pts',(49.6502083083206,18.1570688241963,-60.7447787940001));
#167151=CARTESIAN_POINT('Ctrl Pts',(49.6592207458122,18.1594391838299,-60.7407012135605));
#167152=CARTESIAN_POINT('Ctrl Pts',(49.6808075021014,18.1651167128864,-60.7309345177824));
#167153=CARTESIAN_POINT('Ctrl Pts',(49.7033660875626,18.1710466103037,-60.7216353832497));
#167154=CARTESIAN_POINT('Ctrl Pts',(49.7268958138618,18.177227889774,-60.7129654588309));
#167155=CARTESIAN_POINT('Ctrl Pts',(49.7386606770114,18.1803185295091,-60.7086304966215));
#167156=CARTESIAN_POINT('Ctrl Pts',(49.7506680691111,18.1834719459986,-60.70445298761));
#167157=CARTESIAN_POINT('Ctrl Pts',(49.7629162642643,18.1866875763887,-60.7004539866541));
#167158=CARTESIAN_POINT('Ctrl Pts',(49.7690403618409,18.1882953915837,-60.6984544861761));
#167159=CARTESIAN_POINT('Ctrl Pts',(49.7752246606936,18.1899187602925,-60.6964996152323));
#167160=CARTESIAN_POINT('Ctrl Pts',(49.7814688141369,18.191557577201,-60.6945920612596));
#167161=CARTESIAN_POINT('Ctrl Pts',(49.7845908908586,18.1923769856553,-60.6936382842732));
#167162=CARTESIAN_POINT('Ctrl Pts',(49.7877279312615,18.1932002561623,-60.6926963366154));
#167163=CARTESIAN_POINT('Ctrl Pts',(49.7908798877155,18.1940273743939,-60.6917665561795));
#167164=CARTESIAN_POINT('Ctrl Pts',(49.7932848752266,18.1946584773442,-60.6910571205102));
#167165=CARTESIAN_POINT('Ctrl Pts',(49.7965271499009,18.1955092358784,-60.6901157621523));
#167166=CARTESIAN_POINT('Ctrl Pts',(49.7987102115137,18.1960820260968,-60.6894907266843));
#167167=CARTESIAN_POINT('Ctrl Pts',(49.7993882521346,18.1962599299329,-60.689296595912));
#167168=CARTESIAN_POINT('Ctrl Pts',(49.7999640076789,18.1964109931631,-60.6891325221658));
#167169=CARTESIAN_POINT('Ctrl Pts',(49.80038045534,18.1965202573161,-60.6890140555969));
#167170=CARTESIAN_POINT('Ctrl Pts',(49.8126406245812,18.199736980888,-60.6855264140025));
#167171=CARTESIAN_POINT('Ctrl Pts',(49.8266384353679,18.2034086307252,-60.6817886559558));
#167172=CARTESIAN_POINT('Ctrl Pts',(49.8424059506839,18.2075426297223,-60.6780206105999));
#167173=CARTESIAN_POINT('Ctrl Pts',(49.8580179662976,18.2116358590989,-60.6742897258186));
#167174=CARTESIAN_POINT('Ctrl Pts',(49.8753655394232,18.2161825187496,-60.6705292559762));
#167175=CARTESIAN_POINT('Ctrl Pts',(49.8944728359148,18.2211877040932,-60.6670026654773));
#167176=CARTESIAN_POINT('Ctrl Pts',(49.9133107617609,18.226122327387,-60.6635257921092));
#167177=CARTESIAN_POINT('Ctrl Pts',(49.9338597788633,18.2315028072817,-60.6602763839452));
#167178=CARTESIAN_POINT('Ctrl Pts',(49.9561272211008,18.2373295727274,-60.6575539969875));
#167179=CARTESIAN_POINT('Ctrl Pts',(49.9776524699926,18.2429621269792,-60.6549223495706));
#167180=CARTESIAN_POINT('Ctrl Pts',(50.0007840434222,18.2490118557362,-60.6527834311557));
#167181=CARTESIAN_POINT('Ctrl Pts',(50.0255051992595,18.2554727154041,-60.6514490823613));
#167182=CARTESIAN_POINT('Ctrl Pts',(50.0432317550206,18.2601055404193,-60.6504922740119));
#167183=CARTESIAN_POINT('Ctrl Pts',(50.0617751943528,18.2649496372297,-60.64995));
#167184=CARTESIAN_POINT('Ctrl Pts',(50.0811190791972,18.26999998,-60.64995));
#167185=CARTESIAN_POINT('Origin',(0.,-12.9675000200281,-60.64995));
#167186=CARTESIAN_POINT('',(52.2790965136749,12.4220352393542,-61.2273317382593));
#167187=CARTESIAN_POINT('Origin',(0.,-12.9675000200281,-61.2273317382593));
#167188=CARTESIAN_POINT('Ctrl Pts',(52.2790965136749,12.4220352393542,-61.2273317382593));
#167189=CARTESIAN_POINT('Ctrl Pts',(51.5940499967886,12.4199494071951,-62.5507730638401));
#167190=CARTESIAN_POINT('Ctrl Pts',(50.9185870393202,12.4178348117833,-63.8509234010523));
#167191=CARTESIAN_POINT('Ctrl Pts',(50.2526456556148,12.4156916222119,-65.1277560842965));
#167192=CARTESIAN_POINT('Ctrl Pts',(49.5653893074062,12.413479834997,-66.4454566937362));
#167193=CARTESIAN_POINT('Ctrl Pts',(48.8882741342398,12.4112375970648,-67.7383226701546));
#167194=CARTESIAN_POINT('Ctrl Pts',(48.2212806269929,12.40896625095,-69.0063541135337));
#167195=CARTESIAN_POINT('Ctrl Pts',(47.5767619469032,12.4067714394803,-70.2316583231239));
#167196=CARTESIAN_POINT('Ctrl Pts',(46.9416949320218,12.4045494617144,-71.4337735851211));
#167197=CARTESIAN_POINT('Ctrl Pts',(46.3161001760333,12.4023024545041,-72.6127259072083));
#167198=CARTESIAN_POINT('Ctrl Pts',(46.3086478819023,12.4022756874021,-72.6267699818853));
#167199=CARTESIAN_POINT('Ctrl Pts',(46.3021038939964,12.4022521764144,-72.6391017563987));
#167200=CARTESIAN_POINT('Ctrl Pts',(46.2937473313732,12.4022221332078,-72.654848273595));
#167201=CARTESIAN_POINT('Ctrl Pts',(46.293595489273,12.4022215873107,-72.6551343941387));
#167202=CARTESIAN_POINT('Ctrl Pts',(46.2934436476664,12.4022210414119,-72.6554205134396));
#167203=CARTESIAN_POINT('Ctrl Pts',(46.2932918065534,12.4022204955114,-72.6557066314977));
#167204=CARTESIAN_POINT('Ctrl Pts',(45.6957923828427,12.4000723603874,-73.7815899406001));
#167205=CARTESIAN_POINT('Ctrl Pts',(45.1059485933711,12.3978983023915,-74.888236379866));
#167206=CARTESIAN_POINT('Ctrl Pts',(44.5236810068234,12.3956984861845,-75.9756149755482));
#167207=CARTESIAN_POINT('Ctrl Pts',(43.930487601711,12.3934573920611,-77.0833974225216));
#167208=CARTESIAN_POINT('Ctrl Pts',(43.3451575554821,12.3911895674979,-78.1711822389739));
#167209=CARTESIAN_POINT('Ctrl Pts',(42.7676550803754,12.3888961308826,-79.2389632317658));
#167210=CARTESIAN_POINT('Ctrl Pts',(42.1723207719999,12.3865318786758,-80.3397146332603));
#167211=CARTESIAN_POINT('Ctrl Pts',(41.5853049906506,12.3841404106341,-81.4192078583826));
#167212=CARTESIAN_POINT('Ctrl Pts',(41.0066173579777,12.3817239039064,-82.4774630287889));
#167213=CARTESIAN_POINT('Ctrl Pts',(40.7249794558944,12.3805478292045,-82.9924986874662));
#167214=CARTESIAN_POINT('Ctrl Pts',(40.4453148819667,12.3793658376879,-83.5025042696471));
#167215=CARTESIAN_POINT('Ctrl Pts',(40.1676286103916,12.3781782553103,-84.0074842249685));
#167216=CARTESIAN_POINT('Origin',(57.,11.61999998,-174.34995));
#167217=CARTESIAN_POINT('',(57.,12.11999998,-176.84995));
#167218=CARTESIAN_POINT('Origin',(57.,11.61999998,-176.84995));
#167219=CARTESIAN_POINT('',(59.5,12.11999998,-174.34995));
#167220=CARTESIAN_POINT('Origin',(57.,12.11999998,-174.34995));
#167221=CARTESIAN_POINT('Origin',(59.5,11.61999998,-174.34995));
#167222=CARTESIAN_POINT('Origin',(59.5,11.61999998,-55.24995));
#167223=CARTESIAN_POINT('',(59.5,12.11999998,-58.24995));
#167224=CARTESIAN_POINT('',(59.5,12.11999998,-174.34995));
#167225=CARTESIAN_POINT('Origin',(59.5,11.61999998,-58.24995));
#167226=CARTESIAN_POINT('Ctrl Pts',(52.8224784153175,12.11999998,-61.2752041600839));
#167227=CARTESIAN_POINT('Ctrl Pts',(52.5913010098385,12.11999998,-60.9843891047178));
#167228=CARTESIAN_POINT('Ctrl Pts',(52.5245819708698,12.4756972986233,-60.9004583201698));
#167229=CARTESIAN_POINT('Ctrl Pts',(53.0127900201976,12.11999998,-61.1239198608288));
#167230=CARTESIAN_POINT('Ctrl Pts',(52.7297264322295,12.1199999799996,-60.865773772671));
#167231=CARTESIAN_POINT('Ctrl Pts',(52.6505629615106,12.4839221309077,-60.7971452199062));
#167232=CARTESIAN_POINT('Ctrl Pts',(53.1625689933938,12.11999998,-60.9259844495965));
#167233=CARTESIAN_POINT('Ctrl Pts',(52.8314129775774,12.1199999800002,-60.7072763762979));
#167234=CARTESIAN_POINT('Ctrl Pts',(52.7486445377005,12.4996864767879,-60.660571058145));
#167235=CARTESIAN_POINT('Ctrl Pts',(53.2607580814926,12.11999998,-60.7033966151602));
#167236=CARTESIAN_POINT('Ctrl Pts',(52.8857929788878,12.11999998,-60.5379900686008));
#167237=CARTESIAN_POINT('Ctrl Pts',(52.81219032515,12.5218539749099,-60.5055220850798));
#167238=CARTESIAN_POINT('',(52.81219032515,12.5218539749099,-60.5055220850798));
#167239=CARTESIAN_POINT('',(53.2607580814926,12.11999998,-60.7033966151602));
#167240=CARTESIAN_POINT('Origin',(53.2607580814926,12.61999998,-60.7033966151602));
#167241=CARTESIAN_POINT('',(52.8224784153176,12.11999998,-61.275204160084));
#167242=CARTESIAN_POINT('Origin',(52.0615368275759,12.11999998,-60.1416270042854));
#167243=CARTESIAN_POINT('',(52.5245819708686,12.4756972986232,-60.9004583201709));
#167244=CARTESIAN_POINT('Origin',(52.8224784153158,12.6199999800056,-61.2752041600831));
#167245=CARTESIAN_POINT('Ctrl Pts',(52.81219032515,12.5218539749099,-60.5055220850798));
#167246=CARTESIAN_POINT('Ctrl Pts',(52.7933411307666,12.5152785668795,-60.5515133041606));
#167247=CARTESIAN_POINT('Ctrl Pts',(52.7716003070881,12.5093184856134,-60.5955155162472));
#167248=CARTESIAN_POINT('Ctrl Pts',(52.7473030826718,12.5039798383895,-60.6371999655705));
#167249=CARTESIAN_POINT('Ctrl Pts',(52.7233801432051,12.4987234299955,-60.6782422896143));
#167250=CARTESIAN_POINT('Ctrl Pts',(52.6969791694599,12.4940694538365,-60.7170375441058));
#167251=CARTESIAN_POINT('Ctrl Pts',(52.6684211908199,12.4900172284755,-60.753321423101));
#167252=CARTESIAN_POINT('Ctrl Pts',(52.6403779947413,12.4860380480235,-60.7889512534185));
#167253=CARTESIAN_POINT('Ctrl Pts',(52.6102550306507,12.4826391084701,-60.8221593620841));
#167254=CARTESIAN_POINT('Ctrl Pts',(52.5783544676246,12.4798135521224,-60.8527452424381));
#167255=CARTESIAN_POINT('Ctrl Pts',(52.560943652773,12.4782714088574,-60.8694385246063));
#167256=CARTESIAN_POINT('Ctrl Pts',(52.543003279237,12.4768999569538,-60.8853515771895));
#167257=CARTESIAN_POINT('Ctrl Pts',(52.5245819708698,12.4756972986233,-60.9004583201698));
#167258=CARTESIAN_POINT('Ctrl Pts',(52.5554920964233,12.4824531775908,-60.8743475621314));
#167259=CARTESIAN_POINT('Ctrl Pts',(52.6167804214063,12.1199999799999,-60.9580152164686));
#167260=CARTESIAN_POINT('Ctrl Pts',(52.8395656282165,12.11999998,-61.2621516547499));
#167261=CARTESIAN_POINT('Ctrl Pts',(52.4298097977004,12.4550534422725,-60.9763291407645));
#167262=CARTESIAN_POINT('Ctrl Pts',(52.5149863535236,12.1199999800004,-61.0598572644291));
#167263=CARTESIAN_POINT('Ctrl Pts',(52.7700980531444,12.11999998,-61.3131374124818));
#167264=CARTESIAN_POINT('Ctrl Pts',(52.3281854015479,12.4328072501504,-61.1077415231532));
#167265=CARTESIAN_POINT('Ctrl Pts',(52.4334636056902,12.1199999799999,-61.181393614378));
#167266=CARTESIAN_POINT('Ctrl Pts',(52.7138825713227,12.11999998,-61.378844307496));
#167267=CARTESIAN_POINT('Ctrl Pts',(52.2617577785881,12.4182503522228,-61.266432315258));
#167268=CARTESIAN_POINT('Ctrl Pts',(52.3811794250381,12.11999998,-61.3215576504461));
#167269=CARTESIAN_POINT('Ctrl Pts',(52.6771323647535,12.11999998,-61.4581932772117));
#167270=CARTESIAN_POINT('',(52.6867218473722,12.11999998,-61.4386408691297));
#167271=CARTESIAN_POINT('Origin',(53.5608834560411,12.11999998,-61.897804091577));
#167272=CARTESIAN_POINT('Origin',(52.6867218473722,12.61999998,-61.4386408691297));
#167273=CARTESIAN_POINT('Origin',(53.1708541764071,12.6169987765688,-61.636054659934));
#167274=CARTESIAN_POINT('Ctrl Pts',(40.5508657493525,12.11999998,-84.2187933558389));
#167275=CARTESIAN_POINT('Ctrl Pts',(40.2925576369006,12.11999998,-84.0763675385317));
#167276=CARTESIAN_POINT('Ctrl Pts',(40.1676286103916,12.3781782553103,-84.0074842249685));
#167277=CARTESIAN_POINT('Ctrl Pts',(42.6282131590433,12.11999998,-80.4512482683356));
#167278=CARTESIAN_POINT('Ctrl Pts',(42.3754889509591,12.11999998,-80.2844795011615));
#167279=CARTESIAN_POINT('Ctrl Pts',(42.2393869130494,12.3870385552721,-80.2399360160109));
#167280=CARTESIAN_POINT('Ctrl Pts',(44.6709958246245,12.11999998,-76.6652818249261));
#167281=CARTESIAN_POINT('Ctrl Pts',(44.4098483480378,12.11999998,-76.5004916194052));
#167282=CARTESIAN_POINT('Ctrl Pts',(44.2775738677864,12.39497584134,-76.4539726940548));
#167283=CARTESIAN_POINT('Ctrl Pts',(48.710372157466,12.11999998,-69.0687496953211));
#167284=CARTESIAN_POINT('Ctrl Pts',(48.4382080167511,12.11999998,-68.9007945866128));
#167285=CARTESIAN_POINT('Ctrl Pts',(48.3090097368786,12.4094651694423,-68.8574405644517));
#167286=CARTESIAN_POINT('Ctrl Pts',(50.7067648613536,12.11999998,-65.2580717844373));
#167287=CARTESIAN_POINT('Ctrl Pts',(50.4278516292118,12.1199999800037,-65.0915922935902));
#167288=CARTESIAN_POINT('Ctrl Pts',(50.3020637690764,12.4160155627679,-65.046761180979));
#167289=CARTESIAN_POINT('Ctrl Pts',(52.6867218473722,12.11999998,-61.4386408691297));
#167290=CARTESIAN_POINT('Ctrl Pts',(52.3947118718251,12.11999998,-61.287265650179));
#167291=CARTESIAN_POINT('Ctrl Pts',(52.2790965136749,12.4220352393542,-61.2273317382593));
#167292=CARTESIAN_POINT('',(40.5508657493525,12.11999998,-84.2187933558389));
#167293=CARTESIAN_POINT('Ctrl Pts',(40.5508657493525,12.11999998,-84.2187933558389));
#167294=CARTESIAN_POINT('Ctrl Pts',(42.6282147356021,12.11999998,-80.4512454090371));
#167295=CARTESIAN_POINT('Ctrl Pts',(44.6709958246292,12.11999998,-76.6652818249174));
#167296=CARTESIAN_POINT('Ctrl Pts',(46.6906839910419,12.11999998,-72.8670157601218));
#167297=CARTESIAN_POINT('Ctrl Pts',(48.7103721574547,12.11999998,-69.0687496953263));
#167298=CARTESIAN_POINT('Ctrl Pts',(50.7067642663818,12.11999998,-65.2580729321624));
#167299=CARTESIAN_POINT('Ctrl Pts',(52.6867218473722,12.11999998,-61.4386408691297));
#167300=CARTESIAN_POINT('Origin',(40.5508657493525,12.61999998,-84.2187933558389));
#167301=CARTESIAN_POINT('Ctrl Pts',(40.2331730433337,12.3723044963979,-83.8975858343799));
#167302=CARTESIAN_POINT('Ctrl Pts',(40.3579731063027,12.1199999799991,-83.9691999731268));
#167303=CARTESIAN_POINT('Ctrl Pts',(40.6098865790299,12.11999998,-84.1137766207722));
#167304=CARTESIAN_POINT('Ctrl Pts',(39.7931688569455,12.411333626796,-84.6210795875556));
#167305=CARTESIAN_POINT('Ctrl Pts',(39.9075805796616,12.1199999800059,-84.6935233019318));
#167306=CARTESIAN_POINT('Ctrl Pts',(40.2138237094928,12.11999998,-84.8052710236263));
#167307=CARTESIAN_POINT('Ctrl Pts',(39.4900144732213,12.4527389916394,-85.3915160553928));
#167308=CARTESIAN_POINT('Ctrl Pts',(39.5983305176353,12.11999998,-85.4536873863572));
#167309=CARTESIAN_POINT('Ctrl Pts',(39.9410319396356,12.11999998,-85.5407202621882));
#167310=CARTESIAN_POINT('Ctrl Pts',(39.1919178464122,12.5160949947626,-86.5777828047161));
#167311=CARTESIAN_POINT('Ctrl Pts',(39.2735548943734,12.11999998,-86.5998107325698));
#167312=CARTESIAN_POINT('Ctrl Pts',(39.6727396192083,12.11999998,-86.6717926677035));
#167313=CARTESIAN_POINT('Ctrl Pts',(39.1197796418649,12.5368967075763,-86.9683794640772));
#167314=CARTESIAN_POINT('Ctrl Pts',(39.1889101666761,12.11999998,-86.985650574818));
#167315=CARTESIAN_POINT('Ctrl Pts',(39.6078129604692,12.11999998,-87.0440021565177));
#167316=CARTESIAN_POINT('Ctrl Pts',(39.0190067195619,12.5806200665905,-87.7921667079605));
#167317=CARTESIAN_POINT('Ctrl Pts',(39.0548711280315,12.11999998,-87.8030567622564));
#167318=CARTESIAN_POINT('Ctrl Pts',(39.5171116805788,12.11999998,-87.8285181369117));
#167319=CARTESIAN_POINT('Ctrl Pts',(38.9951427354958,12.6036514403655,-88.2277009984956));
#167320=CARTESIAN_POINT('Ctrl Pts',(39.011598340781,12.11999998,-88.2372397284706));
#167321=CARTESIAN_POINT('Ctrl Pts',(39.495630995299,12.11999998,-88.2430081536419));
#167322=CARTESIAN_POINT('Ctrl Pts',(39.0008182748242,12.6267359883438,-88.6661338308315));
#167323=CARTESIAN_POINT('Ctrl Pts',(38.9939934962203,12.11999998,-88.6662158548394));
#167324=CARTESIAN_POINT('Ctrl Pts',(39.5007354296681,12.11999998,-88.6599531506585));
#167325=CARTESIAN_POINT('',(39.5,12.11999998,-88.5398461374725));
#167326=CARTESIAN_POINT('Ctrl Pts',(39.5,12.11999998,-88.5398461374725));
#167327=CARTESIAN_POINT('Ctrl Pts',(39.5,12.11999998,-88.1633801721072));
#167328=CARTESIAN_POINT('Ctrl Pts',(39.5216886477936,12.11999998,-87.7889298981599));
#167329=CARTESIAN_POINT('Ctrl Pts',(39.5647508040475,12.11999998,-87.4164660273289));
#167330=CARTESIAN_POINT('Ctrl Pts',(39.6078129603014,12.11999998,-87.0440021564979));
#167331=CARTESIAN_POINT('Ctrl Pts',(39.672739619198,12.11999998,-86.6717926677294));
#167332=CARTESIAN_POINT('Ctrl Pts',(39.7591103506482,12.11999998,-86.3076691214426));
#167333=CARTESIAN_POINT('Ctrl Pts',(39.8454810820984,12.11999998,-85.9435455751558));
#167334=CARTESIAN_POINT('Ctrl Pts',(39.9523131981843,12.11999998,-85.5865932598647));
#167335=CARTESIAN_POINT('Ctrl Pts',(40.0830988504763,12.11999998,-85.2380360010512));
#167336=CARTESIAN_POINT('Ctrl Pts',(40.2020523584852,12.11999998,-84.9210126276826));
#167337=CARTESIAN_POINT('Ctrl Pts',(40.3408210453828,12.11999998,-84.6109338991013));
#167338=CARTESIAN_POINT('Ctrl Pts',(40.5020760733001,12.11999998,-84.3087360817111));
#167339=CARTESIAN_POINT('Ctrl Pts',(40.5181158924583,12.11999998,-84.2786768742337));
#167340=CARTESIAN_POINT('Ctrl Pts',(40.5343782322704,12.11999998,-84.248695655134));
#167341=CARTESIAN_POINT('Ctrl Pts',(40.5508657493524,12.11999998,-84.2187933558389));
#167342=CARTESIAN_POINT('Origin',(39.5,12.61999998,-88.5398461374725));
#167343=CARTESIAN_POINT('Origin',(39.5,12.61999998,-55.24995));
#167344=CARTESIAN_POINT('',(39.5,12.11999998,-143.518796834034));
#167345=CARTESIAN_POINT('',(39.5,12.11999998,-55.24995));
#167346=CARTESIAN_POINT('Origin',(39.5,12.61999998,-143.518796834034));
#167347=CARTESIAN_POINT('Ctrl Pts',(39.,12.61999998,-143.518796834034));
#167348=CARTESIAN_POINT('Ctrl Pts',(39.,12.11999998,-143.518796834033));
#167349=CARTESIAN_POINT('Ctrl Pts',(39.5,12.11999998,-143.518796834034));
#167350=CARTESIAN_POINT('Ctrl Pts',(39.,12.5782777425004,-144.310620782824));
#167351=CARTESIAN_POINT('Ctrl Pts',(39.0400461849957,12.11999998,-144.278811846669));
#167352=CARTESIAN_POINT('Ctrl Pts',(39.5000000018526,12.11999998,-144.271919993373));
#167353=CARTESIAN_POINT('Ctrl Pts',(39.0943364399906,12.5370121096574,-145.08773908462));
#167354=CARTESIAN_POINT('Ctrl Pts',(39.1598342511364,12.11999998,-145.053286643925));
#167355=CARTESIAN_POINT('Ctrl Pts',(39.5849027948822,12.11999998,-145.01203141024));
#167356=CARTESIAN_POINT('Ctrl Pts',(39.4748832666623,12.4556479161234,-146.611482622671));
#167357=CARTESIAN_POINT('Ctrl Pts',(39.5826034488757,12.11999998,-146.552938806615));
#167358=CARTESIAN_POINT('Ctrl Pts',(39.9273949411055,12.11999998,-146.464868936119));
#167359=CARTESIAN_POINT('Ctrl Pts',(39.7646907193389,12.4152882936363,-147.362846081219));
#167360=CARTESIAN_POINT('Ctrl Pts',(39.8795078356987,12.11999998,-147.293857468464));
#167361=CARTESIAN_POINT('Ctrl Pts',(40.1882099383814,12.11999998,-147.182125180442));
#167362=CARTESIAN_POINT('Ctrl Pts',(40.1676286103828,12.3781782553111,-148.051158746522));
#167363=CARTESIAN_POINT('Ctrl Pts',(40.2925576368918,12.11999998,-147.98227543296));
#167364=CARTESIAN_POINT('Ctrl Pts',(40.5508657493446,12.11999998,-147.839849615653));
#167365=CARTESIAN_POINT('',(40.5508657493446,12.11999998,-147.839849615653));
#167366=CARTESIAN_POINT('Ctrl Pts',(40.5508657493446,12.11999998,-147.839849615653));
#167367=CARTESIAN_POINT('Ctrl Pts',(40.4872051775684,12.11999998,-147.72439272417));
#167368=CARTESIAN_POINT('Ctrl Pts',(40.4268911487416,12.11999998,-147.607488691345));
#167369=CARTESIAN_POINT('Ctrl Pts',(40.3697096603118,12.11999998,-147.489235888512));
#167370=CARTESIAN_POINT('Ctrl Pts',(40.3100900049243,12.11999998,-147.365940893102));
#167371=CARTESIAN_POINT('Ctrl Pts',(40.2538755845826,12.11999998,-147.241179143609));
#167372=CARTESIAN_POINT('Ctrl Pts',(40.2008730860125,12.11999998,-147.115031779943));
#167373=CARTESIAN_POINT('Ctrl Pts',(40.1592698126766,12.11999998,-147.016014877103));
#167374=CARTESIAN_POINT('Ctrl Pts',(40.1196464719309,12.11999998,-146.916143544358));
#167375=CARTESIAN_POINT('Ctrl Pts',(40.0819301037035,12.11999998,-146.815448147357));
#167376=CARTESIAN_POINT('Ctrl Pts',(40.0215352750628,12.11999998,-146.654205654174));
#167377=CARTESIAN_POINT('Ctrl Pts',(39.9660661346645,12.11999998,-146.490922340265));
#167378=CARTESIAN_POINT('Ctrl Pts',(39.9154672964456,12.11999998,-146.326388038909));
#167379=CARTESIAN_POINT('Ctrl Pts',(39.8629240743821,12.11999998,-146.15553110548));
#167380=CARTESIAN_POINT('Ctrl Pts',(39.8156327203445,12.11999998,-145.983326186387));
#167381=CARTESIAN_POINT('Ctrl Pts',(39.7734780737246,12.11999998,-145.810672966349));
#167382=CARTESIAN_POINT('Ctrl Pts',(39.767602077948,12.11999998,-145.786606589968));
#167383=CARTESIAN_POINT('Ctrl Pts',(39.7618258061273,12.11999998,-145.762531511883));
#167384=CARTESIAN_POINT('Ctrl Pts',(39.7561488675992,12.11999998,-145.738450173272));
#167385=CARTESIAN_POINT('Ctrl Pts',(39.6543246883703,12.11999998,-145.306516213334));
#167386=CARTESIAN_POINT('Ctrl Pts',(39.5830357134782,12.11999998,-144.869793515157));
#167387=CARTESIAN_POINT('Ctrl Pts',(39.5419615359765,12.11999998,-144.428332293124));
#167388=CARTESIAN_POINT('Ctrl Pts',(39.5139579007142,12.11999998,-144.127351974194));
#167389=CARTESIAN_POINT('Ctrl Pts',(39.5,12.11999998,-143.824168887311));
#167390=CARTESIAN_POINT('Ctrl Pts',(39.5,12.11999998,-143.518796834034));
#167391=CARTESIAN_POINT('Origin',(40.5508657493455,12.6199999799991,-147.839849615653));
#167392=CARTESIAN_POINT('Ctrl Pts',(52.811758955289,12.11999998,-170.861259130871));
#167393=CARTESIAN_POINT('Ctrl Pts',(52.5194581681217,12.11999998,-171.0127167027));
#167394=CARTESIAN_POINT('Ctrl Pts',(52.4039495302269,12.4224147476539,-171.07256826174));
#167395=CARTESIAN_POINT('Ctrl Pts',(50.8116692616976,12.11999998,-167.001248800573));
#167396=CARTESIAN_POINT('Ctrl Pts',(50.5326451268968,12.11999998,-167.168095406566));
#167397=CARTESIAN_POINT('Ctrl Pts',(50.4067968770089,12.4163544181458,-167.212559451309));
#167398=CARTESIAN_POINT('Ctrl Pts',(48.7949136859973,12.11999998,-163.150111451781));
#167399=CARTESIAN_POINT('Ctrl Pts',(48.5227235736013,12.1199999799924,-163.318503470872));
#167400=CARTESIAN_POINT('Ctrl Pts',(48.3933978906048,12.4097551621214,-163.361420582663));
#167401=CARTESIAN_POINT('Ctrl Pts',(44.7140165615046,12.11999998,-155.473076929555));
#167402=CARTESIAN_POINT('Ctrl Pts',(44.4529340155615,12.1199999800075,-155.63827143996));
#167403=CARTESIAN_POINT('Ctrl Pts',(44.3204976166945,12.3951430089669,-155.684386060413));
#167404=CARTESIAN_POINT('Ctrl Pts',(42.6500851427248,12.11999998,-151.647062446733));
#167405=CARTESIAN_POINT('Ctrl Pts',(42.3975527923274,12.11999998,-151.814329756678));
#167406=CARTESIAN_POINT('Ctrl Pts',(42.2612000992887,12.3871318438137,-151.858374821466));
#167407=CARTESIAN_POINT('Ctrl Pts',(40.5508657493446,12.11999998,-147.839849615653));
#167408=CARTESIAN_POINT('Ctrl Pts',(40.2925576368927,12.11999998,-147.98227543296));
#167409=CARTESIAN_POINT('Ctrl Pts',(40.1676286103837,12.3781782553102,-148.051158746523));
#167410=CARTESIAN_POINT('',(52.811758955289,12.11999998,-170.861259130871));
#167411=CARTESIAN_POINT('Ctrl Pts',(52.811758955289,12.11999998,-170.861259130871));
#167412=CARTESIAN_POINT('Ctrl Pts',(50.8116686437173,12.11999998,-167.001247608061));
#167413=CARTESIAN_POINT('Ctrl Pts',(48.794913685955,12.11999998,-163.150111451771));
#167414=CARTESIAN_POINT('Ctrl Pts',(46.7544651237368,12.11999998,-159.311594190676));
#167415=CARTESIAN_POINT('Ctrl Pts',(44.7140165615186,12.11999998,-155.47307692958));
#167416=CARTESIAN_POINT('Ctrl Pts',(42.6500867945137,12.11999998,-151.647065442471));
#167417=CARTESIAN_POINT('Ctrl Pts',(40.5508657493446,12.11999998,-147.839849615653));
#167418=CARTESIAN_POINT('Origin',(52.811758955289,12.61999998,-170.861259130871));
#167419=CARTESIAN_POINT('Ctrl Pts',(52.4039495302269,12.4224147476539,-171.07256826174));
#167420=CARTESIAN_POINT('Ctrl Pts',(52.5194581681217,12.11999998,-171.0127167027));
#167421=CARTESIAN_POINT('Ctrl Pts',(52.811758955289,12.11999998,-170.861259130871));
#167422=CARTESIAN_POINT('Ctrl Pts',(52.4335834030071,12.4288943780099,-171.135818022105));
#167423=CARTESIAN_POINT('Ctrl Pts',(52.5427333133061,12.1199999800001,-171.068676662146));
#167424=CARTESIAN_POINT('Ctrl Pts',(52.8281457246307,12.11999998,-170.892884198111));
#167425=CARTESIAN_POINT('Ctrl Pts',(52.4691942899059,12.4366759982665,-171.194717391534));
#167426=CARTESIAN_POINT('Ctrl Pts',(52.5708615508922,12.11999998,-171.121670121752));
#167427=CARTESIAN_POINT('Ctrl Pts',(52.8478360402188,12.11999998,-170.922334416373));
#167428=CARTESIAN_POINT('Ctrl Pts',(52.5103993792154,12.4456688476555,-171.249463186897));
#167429=CARTESIAN_POINT('Ctrl Pts',(52.6035237155536,12.11999998,-171.171968757444));
#167430=CARTESIAN_POINT('Ctrl Pts',(52.8706140943225,12.11999998,-170.949706593448));
#167431=CARTESIAN_POINT('',(52.8706140943225,12.11999998,-170.949706593448));
#167432=CARTESIAN_POINT('Ctrl Pts',(52.8706140943225,12.11999998,-170.949706593448));
#167433=CARTESIAN_POINT('Ctrl Pts',(52.8478318703964,12.11999998,-170.92232940649));
#167434=CARTESIAN_POINT('Ctrl Pts',(52.8281487108054,12.11999998,-170.892890025127));
#167435=CARTESIAN_POINT('Ctrl Pts',(52.811758955289,12.11999998,-170.861259130871));
#167436=CARTESIAN_POINT('Origin',(52.8706140943225,12.61999998,-170.949706593448));
#167437=CARTESIAN_POINT('Ctrl Pts',(53.1963133798215,12.11999998,-171.855638188259));
#167438=CARTESIAN_POINT('Ctrl Pts',(52.8383133487074,12.11999998,-171.855638188259));
#167439=CARTESIAN_POINT('Ctrl Pts',(52.7229737572976,12.4589111791821,-171.855638188259));
#167440=CARTESIAN_POINT('Ctrl Pts',(53.1963133729203,12.11999998,-171.690331848712));
#167441=CARTESIAN_POINT('Ctrl Pts',(52.8469882490941,12.1199999799987,-171.731583871386));
#167442=CARTESIAN_POINT('Ctrl Pts',(52.7266981809109,12.4479674186086,-171.743571468459));
#167443=CARTESIAN_POINT('Ctrl Pts',(53.1690734716394,12.11999998,-171.529660295248));
#167444=CARTESIAN_POINT('Ctrl Pts',(52.8308498854142,12.11999998,-171.608042739796));
#167445=CARTESIAN_POINT('Ctrl Pts',(52.7105385127756,12.4423260364225,-171.635556218068));
#167446=CARTESIAN_POINT('Ctrl Pts',(53.0574449276732,12.11999998,-171.218309959504));
#167447=CARTESIAN_POINT('Ctrl Pts',(52.7491850652078,12.11999998,-171.372054509995));
#167448=CARTESIAN_POINT('Ctrl Pts',(52.6373539450168,12.4388109638705,-171.427428053892));
#167449=CARTESIAN_POINT('Ctrl Pts',(52.9763399384659,12.11999998,-171.076756377445));
#167450=CARTESIAN_POINT('Ctrl Pts',(52.6858882090128,12.1199999799997,-171.265152468682));
#167451=CARTESIAN_POINT('Ctrl Pts',(52.5825160219714,12.4409678748685,-171.333391115642));
#167452=CARTESIAN_POINT('Ctrl Pts',(52.8706140943225,12.11999998,-170.949706593448));
#167453=CARTESIAN_POINT('Ctrl Pts',(52.6035237155536,12.11999998,-171.171968757444));
#167454=CARTESIAN_POINT('Ctrl Pts',(52.5103993792154,12.4456688476555,-171.249463186897));
#167455=CARTESIAN_POINT('',(53.1963133798215,12.11999998,-171.855638188259));
#167456=CARTESIAN_POINT('Ctrl Pts',(53.1963133798215,12.11999998,-171.855638188259));
#167457=CARTESIAN_POINT('Ctrl Pts',(53.196313374732,12.11999998,-171.733726928708));
#167458=CARTESIAN_POINT('Ctrl Pts',(53.1815021190221,12.11999998,-171.614382981078));
#167459=CARTESIAN_POINT('Ctrl Pts',(53.1513539482,12.11999998,-171.497697478305));
#167460=CARTESIAN_POINT('Ctrl Pts',(53.140611776948,12.11999998,-171.456120970701));
#167461=CARTESIAN_POINT('Ctrl Pts',(53.1279219841141,12.11999998,-171.414882055051));
#167462=CARTESIAN_POINT('Ctrl Pts',(53.1132591959952,12.11999998,-171.373985128688));
#167463=CARTESIAN_POINT('Ctrl Pts',(53.0817091112244,12.11999998,-171.285986755994));
#167464=CARTESIAN_POINT('Ctrl Pts',(53.0420949559002,12.11999998,-171.202535400932));
#167465=CARTESIAN_POINT('Ctrl Pts',(52.9945125852617,12.11999998,-171.123638976886));
#167466=CARTESIAN_POINT('Ctrl Pts',(52.9579184729549,12.11999998,-171.062962205985));
#167467=CARTESIAN_POINT('Ctrl Pts',(52.9166104754401,12.11999998,-171.00498002572));
#167468=CARTESIAN_POINT('Ctrl Pts',(52.8706140943225,12.11999998,-170.949706593448));
#167469=CARTESIAN_POINT('Origin',(53.1963133798215,12.61999998,-171.855638188259));
#167470=CARTESIAN_POINT('Origin',(53.1963133798215,12.61999998,-179.64995));
#167471=CARTESIAN_POINT('',(53.1963133798215,12.11999998,-171.806096612245));
#167472=CARTESIAN_POINT('',(52.7229737572976,12.4589111791821,-179.64995));
#167473=CARTESIAN_POINT('Origin',(60.,11.61999998,-176.84995));
#167474=CARTESIAN_POINT('',(-83.2809572255632,12.1199999800001,-176.84995));
#167475=CARTESIAN_POINT('Origin',(60.,28.91999998,-171.14995));
#167476=CARTESIAN_POINT('',(43.6738487993976,28.91999998,-171.64995));
#167477=CARTESIAN_POINT('',(49.3806153498803,28.91999998,-171.64995));
#167478=CARTESIAN_POINT('',(43.6738487993976,28.41999998,-171.14995));
#167479=CARTESIAN_POINT('',(41.7558360441701,28.41999998,-171.14995));
#167480=CARTESIAN_POINT('Origin',(43.6738487993976,28.91999998,-171.14995));
#167481=CARTESIAN_POINT('Origin',(60.,28.91999998,-171.14995));
#167482=CARTESIAN_POINT('',(49.3103449325291,28.41999998,-171.14995));
#167483=CARTESIAN_POINT('Origin',(49.3103449325291,28.91999998,-171.14995));
#167484=CARTESIAN_POINT('',(45.342056117244,28.91999998,-171.64995));
#167485=CARTESIAN_POINT('',(49.3806153498803,28.91999998,-171.64995));
#167486=CARTESIAN_POINT('',(45.342056117244,28.41999998,-171.14995));
#167487=CARTESIAN_POINT('Origin',(45.342056117244,28.91999998,-171.14995));
#167488=CARTESIAN_POINT('',(41.7558360441701,28.41999998,-171.14995));
#167489=CARTESIAN_POINT('Ctrl Pts',(50.825086291307,28.41999998,-172.64995));
#167490=CARTESIAN_POINT('Ctrl Pts',(50.3904429223989,28.41999998,-172.64995));
#167491=CARTESIAN_POINT('Ctrl Pts',(50.3299522569362,28.85041342952,-172.64995));
#167492=CARTESIAN_POINT('Ctrl Pts',(50.82508629129,28.41999998,-172.453565067926));
#167493=CARTESIAN_POINT('Ctrl Pts',(50.3904429223853,28.4199999800017,-172.511015867074));
#167494=CARTESIAN_POINT('Ctrl Pts',(50.3299522569358,28.8504134295228,-172.51902671195));
#167495=CARTESIAN_POINT('Ctrl Pts',(50.7856616225938,28.41999998,-172.257328160063));
#167496=CARTESIAN_POINT('Ctrl Pts',(50.3606872372737,28.41999998,-172.371853931892));
#167497=CARTESIAN_POINT('Ctrl Pts',(50.3034146036607,28.8522245814264,-172.38820210671));
#167498=CARTESIAN_POINT('Ctrl Pts',(50.6339053193109,28.41999998,-171.894521542842));
#167499=CARTESIAN_POINT('Ctrl Pts',(50.247876228143,28.41999998,-172.118296873734));
#167500=CARTESIAN_POINT('Ctrl Pts',(50.2012639378342,28.8591961991206,-172.14633102856));
#167501=CARTESIAN_POINT('Ctrl Pts',(50.5216333616693,28.41999998,-171.728129909852));
#167502=CARTESIAN_POINT('Ctrl Pts',(50.1643071358756,28.4199999800017,-172.003556970023));
#167503=CARTESIAN_POINT('Ctrl Pts',(50.1256910952006,28.8643539233763,-172.035403273235));
#167504=CARTESIAN_POINT('Ctrl Pts',(50.2412242764601,28.41999998,-171.450449746589));
#167505=CARTESIAN_POINT('Ctrl Pts',(49.9598619165025,28.4199999799983,-171.817687494207));
#167506=CARTESIAN_POINT('Ctrl Pts',(49.9369412763291,28.8772357931761,-171.850283164392));
#167507=CARTESIAN_POINT('Ctrl Pts',(50.0731974178181,28.41999998,-171.339270411997));
#167508=CARTESIAN_POINT('Ctrl Pts',(49.8382982003454,28.4199999800004,-171.746711574348));
#167509=CARTESIAN_POINT('Ctrl Pts',(49.8238385246439,28.8849548730131,-171.776163607997));
#167510=CARTESIAN_POINT('Ctrl Pts',(49.7068252918851,28.41999998,-171.18899099047));
#167511=CARTESIAN_POINT('Ctrl Pts',(49.5798629394444,28.4199999799996,-171.658003579003));
#167512=CARTESIAN_POINT('Ctrl Pts',(49.5772250015517,28.9017858470187,-171.675977326981));
#167513=CARTESIAN_POINT('Ctrl Pts',(49.5086598519041,28.41999998,-171.149950000016));
#167514=CARTESIAN_POINT('Ctrl Pts',(49.4425933612922,28.41999998,-171.640924254978));
#167515=CARTESIAN_POINT('Ctrl Pts',(49.443835276054,28.9108894800008,-171.64995));
#167516=CARTESIAN_POINT('Ctrl Pts',(49.3103449325291,28.41999998,-171.14995));
#167517=CARTESIAN_POINT('Ctrl Pts',(49.3103449325291,28.41999998,-171.64995));
#167518=CARTESIAN_POINT('Ctrl Pts',(49.3103449325291,28.91999998,-171.64995));
#167519=CARTESIAN_POINT('',(50.825086291307,28.41999998,-172.64995));
#167520=CARTESIAN_POINT('Origin',(50.825086291307,28.91999998,-172.64995));
#167521=CARTESIAN_POINT('Ctrl Pts',(50.825086291307,28.41999998,-172.64995));
#167522=CARTESIAN_POINT('Ctrl Pts',(50.82508629129,28.41999998,-172.453565067926));
#167523=CARTESIAN_POINT('Ctrl Pts',(50.7856616225938,28.41999998,-172.257328160063));
#167524=CARTESIAN_POINT('Ctrl Pts',(50.6339053193109,28.41999998,-171.894521542842));
#167525=CARTESIAN_POINT('Ctrl Pts',(50.5216333616693,28.41999998,-171.728129909852));
#167526=CARTESIAN_POINT('Ctrl Pts',(50.2412242764601,28.41999998,-171.450449746589));
#167527=CARTESIAN_POINT('Ctrl Pts',(50.0731974178181,28.41999998,-171.339270411997));
#167528=CARTESIAN_POINT('Ctrl Pts',(49.7068252918851,28.41999998,-171.18899099047));
#167529=CARTESIAN_POINT('Ctrl Pts',(49.5086598519041,28.41999998,-171.149950000016));
#167530=CARTESIAN_POINT('Ctrl Pts',(49.3103449325291,28.41999998,-171.14995));
#167531=CARTESIAN_POINT('Origin',(50.825086291307,28.91999998,-171.64995));
#167532=CARTESIAN_POINT('',(50.3299522569362,28.85041342952,-171.64995));
#167533=CARTESIAN_POINT('',(50.825086291307,28.41999998,-55.24995));
#167534=CARTESIAN_POINT('Origin',(60.,27.91999998,-176.84995));
#167535=CARTESIAN_POINT('',(57.,28.41999998,-176.84995));
#167536=CARTESIAN_POINT('',(60.,28.41999998,-176.84995));
#167537=CARTESIAN_POINT('Origin',(57.,27.91999998,-176.84995));
#167538=CARTESIAN_POINT('Origin',(57.,27.91999998,-174.34995));
#167539=CARTESIAN_POINT('',(59.5,28.41999998,-174.34995));
#167540=CARTESIAN_POINT('Origin',(57.,28.41999998,-174.34995));
#167541=CARTESIAN_POINT('Origin',(59.5,27.91999998,-174.34995));
#167542=CARTESIAN_POINT('Origin',(59.5,27.91999998,0.));
#167543=CARTESIAN_POINT('',(59.5,28.41999998,-58.24995));
#167544=CARTESIAN_POINT('',(59.5,28.41999998,-174.34995));
#167545=CARTESIAN_POINT('Origin',(59.5,27.91999998,-58.24995));
#167546=CARTESIAN_POINT('Ctrl Pts',(45.342056117244,28.9200050678813,-60.6499500000259));
#167547=CARTESIAN_POINT('Ctrl Pts',(45.342056117244,28.41999998,-60.6499449120928));
#167548=CARTESIAN_POINT('Ctrl Pts',(45.342056117244,28.41999998,-61.14995));
#167549=CARTESIAN_POINT('Ctrl Pts',(45.2161093325487,28.8799153348109,-60.6499495913736));
#167550=CARTESIAN_POINT('Ctrl Pts',(45.2207546457868,28.41999998,-60.6885563794559));
#167551=CARTESIAN_POINT('Ctrl Pts',(45.2032855852163,28.41999998,-61.1499499725599));
#167552=CARTESIAN_POINT('Ctrl Pts',(45.0809055449378,28.8470468727513,-60.6499493090119));
#167553=CARTESIAN_POINT('Ctrl Pts',(45.0814092233342,28.4199999800006,-60.7134256454893));
#167554=CARTESIAN_POINT('Ctrl Pts',(45.0642313709311,28.41999998,-61.1448442113686));
#167555=CARTESIAN_POINT('Ctrl Pts',(44.7999542633237,28.8023061531432,-60.6499489465081));
#167556=CARTESIAN_POINT('Ctrl Pts',(44.7998786663716,28.4199999799995,-60.7430249240652));
#167557=CARTESIAN_POINT('Ctrl Pts',(44.7862672310244,28.41999998,-61.1362430899869));
#167558=CARTESIAN_POINT('Ctrl Pts',(44.6541596767004,28.7904721518728,-60.6499488654503));
#167559=CARTESIAN_POINT('Ctrl Pts',(44.6527441767019,28.41999998,-60.7493138199263));
#167560=CARTESIAN_POINT('Ctrl Pts',(44.647272115325,28.41999998,-61.1328798677618));
#167561=CARTESIAN_POINT('Ctrl Pts',(44.36232828092,28.7904412154038,-60.6499488652048));
#167562=CARTESIAN_POINT('Ctrl Pts',(44.3637416796284,28.41999998,-60.7493310407855));
#167563=CARTESIAN_POINT('Ctrl Pts',(44.3691883762669,28.41999998,-61.1328719599062));
#167564=CARTESIAN_POINT('Ctrl Pts',(44.2164190292987,28.8022526047183,-60.6499489461074));
#167565=CARTESIAN_POINT('Ctrl Pts',(44.2164931090599,28.41999998,-60.7430562060495));
#167566=CARTESIAN_POINT('Ctrl Pts',(44.2300913879779,28.41999998,-61.1362301431742));
#167567=CARTESIAN_POINT('Ctrl Pts',(43.9353228646302,28.8469743774063,-60.6499493083947));
#167568=CARTESIAN_POINT('Ctrl Pts',(43.9348222136893,28.41999998,-60.7134784063315));
#167569=CARTESIAN_POINT('Ctrl Pts',(43.952003265591,28.41999998,-61.1448329195507));
#167570=CARTESIAN_POINT('Ctrl Pts',(43.800108709594,28.8798156648005,-60.6499495903585));
#167571=CARTESIAN_POINT('Ctrl Pts',(43.7954409326636,28.4199999800005,-60.688648899859));
#167572=CARTESIAN_POINT('Ctrl Pts',(43.812959462792,28.41999998,-61.149949972467));
#167573=CARTESIAN_POINT('Ctrl Pts',(43.6738487993976,28.9200050678813,-60.6499500000259));
#167574=CARTESIAN_POINT('Ctrl Pts',(43.6738487993976,28.41999998,-60.6499449120928));
#167575=CARTESIAN_POINT('Ctrl Pts',(43.6738487993976,28.41999998,-61.14995));
#167576=CARTESIAN_POINT('',(45.342056117244,28.41999998,-61.14995));
#167577=CARTESIAN_POINT('',(45.342056117244,28.91999998,-60.64995));
#167578=CARTESIAN_POINT('Origin',(45.342056117244,28.91999998,-61.14995));
#167579=CARTESIAN_POINT('',(43.6738487993976,28.41999998,-61.14995));
#167580=CARTESIAN_POINT('Ctrl Pts',(43.6738487993976,28.41999998,-61.14995));
#167581=CARTESIAN_POINT('Ctrl Pts',(43.8129691638245,28.41999998,-61.1499499724651));
#167582=CARTESIAN_POINT('Ctrl Pts',(43.9520102350777,28.41999998,-61.1448326154154));
#167583=CARTESIAN_POINT('Ctrl Pts',(44.0910473222173,28.41999998,-61.1405313837273));
#167584=CARTESIAN_POINT('Ctrl Pts',(44.2300643593017,28.41999998,-61.1362307723049));
#167585=CARTESIAN_POINT('Ctrl Pts',(44.3691300592233,28.4199999800001,-61.1328730966358));
#167586=CARTESIAN_POINT('Ctrl Pts',(44.5081446038248,28.41999998,-61.1328757503145));
#167587=CARTESIAN_POINT('Ctrl Pts',(44.5081731511562,28.41999998,-61.1328757508594));
#167588=CARTESIAN_POINT('Ctrl Pts',(44.5082016984814,28.41999998,-61.1328757515461));
#167589=CARTESIAN_POINT('Ctrl Pts',(44.5082302458005,28.41999998,-61.1328757523744));
#167590=CARTESIAN_POINT('Ctrl Pts',(44.6473090834153,28.41999998,-61.1328797881197));
#167591=CARTESIAN_POINT('Ctrl Pts',(44.7862513535664,28.41999998,-61.1362425571023));
#167592=CARTESIAN_POINT('Ctrl Pts',(44.9252493016292,28.41999998,-61.140543629625));
#167593=CARTESIAN_POINT('Ctrl Pts',(45.0447391053956,28.41999998,-61.1442410533561));
#167594=CARTESIAN_POINT('Ctrl Pts',(45.1643332045563,28.41999998,-61.1485385900918));
#167595=CARTESIAN_POINT('Ctrl Pts',(45.283905320582,28.41999998,-61.1496673946892));
#167596=CARTESIAN_POINT('Ctrl Pts',(45.3032896860489,28.41999998,-61.1498503902034));
#167597=CARTESIAN_POINT('Ctrl Pts',(45.3226734672926,28.41999998,-61.1499499961673));
#167598=CARTESIAN_POINT('Ctrl Pts',(45.342056117244,28.41999998,-61.14995));
#167599=CARTESIAN_POINT('',(43.6738487993976,28.91999998,-60.64995));
#167600=CARTESIAN_POINT('Origin',(43.6738487993998,28.91999998,-61.1499500000012));
#167601=CARTESIAN_POINT('',(44.5079483622449,28.7904524382955,-60.6499500000782));
#167602=CARTESIAN_POINT('Ctrl Pts',(43.6738487993976,28.91999998,-60.64995));
#167603=CARTESIAN_POINT('Ctrl Pts',(43.7715300191691,28.8889075392417,-60.64995));
#167604=CARTESIAN_POINT('Ctrl Pts',(43.8708734141984,28.863301217625,-60.6499548134033));
#167605=CARTESIAN_POINT('Ctrl Pts',(44.0765991739498,28.8223766210739,-60.6499497946885));
#167606=CARTESIAN_POINT('Ctrl Pts',(44.1829187602502,28.8076233386194,-60.6499592865054));
#167607=CARTESIAN_POINT('Ctrl Pts',(44.3623912990614,28.7933428984955,-60.6499605228612));
#167608=CARTESIAN_POINT('Ctrl Pts',(44.4351555237859,28.7904525467191,-60.6499500385495));
#167609=CARTESIAN_POINT('Ctrl Pts',(44.5079483622449,28.7904524382955,-60.6499500000782));
#167610=CARTESIAN_POINT('Ctrl Pts',(44.5079524583208,28.7904524382925,-60.6499500000761));
#167611=CARTESIAN_POINT('Ctrl Pts',(44.5807739260483,28.7904524382925,-60.6499499621218));
#167612=CARTESIAN_POINT('Ctrl Pts',(44.6535626787506,28.7933447394316,-60.6499600878182));
#167613=CARTESIAN_POINT('Ctrl Pts',(44.8330844822752,28.8076342035688,-60.6499589653179));
#167614=CARTESIAN_POINT('Ctrl Pts',(44.9394245210754,28.8223946394281,-60.6499497574468));
#167615=CARTESIAN_POINT('Ctrl Pts',(45.1451227360793,28.8633247324819,-60.6499554518237));
#167616=CARTESIAN_POINT('Ctrl Pts',(45.2444197705189,28.8889218225659,-60.64995));
#167617=CARTESIAN_POINT('Ctrl Pts',(45.342056117244,28.91999998,-60.64995));
#167618=CARTESIAN_POINT('Origin',(41.7558360441701,29.41999998,-179.64995));
#167619=CARTESIAN_POINT('',(41.7558360441701,28.41999998,-94.0656090587062));
#167620=CARTESIAN_POINT('',(41.7558360441701,28.41999998,-61.14995));
#167621=CARTESIAN_POINT('',(41.7558360441701,28.41999998,-60.64995));
#167622=CARTESIAN_POINT('Ctrl Pts',(41.7558360441699,28.41999998,-94.0656090587062));
#167623=CARTESIAN_POINT('Ctrl Pts',(41.7308060590876,28.41999998,-94.0338832438937));
#167624=CARTESIAN_POINT('Ctrl Pts',(41.7052809909715,28.4208804787712,-94.0028874559655));
#167625=CARTESIAN_POINT('Ctrl Pts',(41.6793664879697,28.4228182439003,-93.9726174435406));
#167626=CARTESIAN_POINT('Ctrl Pts',(41.6537132083297,28.4247364759703,-93.9426525588816));
#167627=CARTESIAN_POINT('Ctrl Pts',(41.6276783059325,28.4276905003979,-93.9133988823568));
#167628=CARTESIAN_POINT('Ctrl Pts',(41.6013615267512,28.4318016725001,-93.8848511812043));
#167629=CARTESIAN_POINT('Ctrl Pts',(41.5745345322137,28.435992549764,-93.8557500127976));
#167630=CARTESIAN_POINT('Ctrl Pts',(41.5474143379969,28.441386237443,-93.827382397737));
#167631=CARTESIAN_POINT('Ctrl Pts',(41.5201155936462,28.4480570335741,-93.7997531157501));
#167632=CARTESIAN_POINT('Ctrl Pts',(41.4978025199057,28.4535095175445,-93.7771698716841));
#167633=CARTESIAN_POINT('Ctrl Pts',(41.4753698984777,28.4598141851721,-93.7550795761226));
#167634=CARTESIAN_POINT('Ctrl Pts',(41.4528781441728,28.4669860146366,-93.7334824827062));
#167635=CARTESIAN_POINT('Ctrl Pts',(41.4463031679536,28.4690825433261,-93.7271690411804));
#167636=CARTESIAN_POINT('Ctrl Pts',(41.4399116489738,28.4711911056978,-93.7210776132016));
#167637=CARTESIAN_POINT('Ctrl Pts',(41.4334563878741,28.4733895230503,-93.7149684859755));
#167638=CARTESIAN_POINT('Ctrl Pts',(41.4261104488557,28.4758912715558,-93.7080164393634));
#167639=CARTESIAN_POINT('Ctrl Pts',(41.4186813966183,28.4785040045918,-93.7010438416435));
#167640=CARTESIAN_POINT('Ctrl Pts',(41.4107916508638,28.4813867845025,-93.6937059454966));
#167641=CARTESIAN_POINT('Ctrl Pts',(41.4099071063804,28.4817099821246,-93.6928832706273));
#167642=CARTESIAN_POINT('Ctrl Pts',(41.4090167534851,28.4820366245984,-93.6920560131081));
#167643=CARTESIAN_POINT('Ctrl Pts',(41.4081200467408,28.4823669762365,-93.6912236943418));
#167644=CARTESIAN_POINT('Ctrl Pts',(41.3849837120793,28.4908905276703,-93.6697486629028));
#167645=CARTESIAN_POINT('Ctrl Pts',(41.361944000301,28.5002943094801,-93.6489194763972));
#167646=CARTESIAN_POINT('Ctrl Pts',(41.3391424940239,28.5106357860759,-93.6287624230044));
#167647=CARTESIAN_POINT('Ctrl Pts',(41.3154766201132,28.5213692910556,-93.6078412488412));
#167648=CARTESIAN_POINT('Ctrl Pts',(41.2920672370986,28.5331126675112,-93.587644051536));
#167649=CARTESIAN_POINT('Ctrl Pts',(41.2690384601266,28.5458882035334,-93.5681847612561));
#167650=CARTESIAN_POINT('Ctrl Pts',(41.2445672529732,28.5594639478674,-93.5475066191177));
#167651=CARTESIAN_POINT('Ctrl Pts',(41.2205258064017,28.5742050230276,-93.5276616732026));
#167652=CARTESIAN_POINT('Ctrl Pts',(41.1970260426481,28.5900949563365,-93.5086504182702));
#167653=CARTESIAN_POINT('Ctrl Pts',(41.1718083285525,28.6071465232962,-93.4882493454546));
#167654=CARTESIAN_POINT('Ctrl Pts',(41.1472143849228,28.6255208325304,-93.4688082580181));
#167655=CARTESIAN_POINT('Ctrl Pts',(41.1233412664623,28.6451524244045,-93.4503104059951));
#167656=CARTESIAN_POINT('Ctrl Pts',(41.0995082258377,28.6647510590544,-93.4318436078908));
#167657=CARTESIAN_POINT('Ctrl Pts',(41.0763931215648,28.6856020390434,-93.41431663479));
#167658=CARTESIAN_POINT('Ctrl Pts',(41.0540572871253,28.7076050220164,-93.3976987687948));
#167659=CARTESIAN_POINT('Origin',(41.7558360441701,29.41999998,-61.14995));
#167660=CARTESIAN_POINT('Origin',(57.,27.91999998,-58.24995));
#167661=CARTESIAN_POINT('',(57.,28.41999998,-55.74995));
#167662=CARTESIAN_POINT('Origin',(57.,28.41999998,-58.24995));
#167663=CARTESIAN_POINT('',(57.,27.91999998,-55.24995));
#167664=CARTESIAN_POINT('Origin',(57.,27.91999998,-55.74995));
#167665=CARTESIAN_POINT('Origin',(57.,27.91999998,-58.24995));
#167666=CARTESIAN_POINT('Origin',(57.,-2.42462934179819E-14,-58.24995));
#167667=CARTESIAN_POINT('',(57.,27.41999998,-55.24995));
#167668=CARTESIAN_POINT('',(57.,28.41999998,-55.24995));
#167669=CARTESIAN_POINT('Origin',(57.,27.41999998,-58.24995));
#167670=CARTESIAN_POINT('Origin',(-83.2809572255632,26.4199999800001,-171.14995));
#167671=CARTESIAN_POINT('',(44.1114262156583,26.91999998,-171.14995));
#167672=CARTESIAN_POINT('Origin',(44.1114262156583,26.41999998,-171.14995));
#167673=CARTESIAN_POINT('',(49.6616970192851,26.91999998,-171.14995));
#167674=CARTESIAN_POINT('Origin',(49.6616970192851,26.41999998,-171.14995));
#167675=CARTESIAN_POINT('',(49.5914266019339,26.91999998,-171.14995));
#167676=CARTESIAN_POINT('Ctrl Pts',(44.1114262156583,26.41999998,-171.64995));
#167677=CARTESIAN_POINT('Ctrl Pts',(44.1114262156583,26.91999998,-171.64995));
#167678=CARTESIAN_POINT('Ctrl Pts',(44.1114262156583,26.91999998,-171.14995));
#167679=CARTESIAN_POINT('Ctrl Pts',(43.9300489743418,26.362103375035,-171.64995));
#167680=CARTESIAN_POINT('Ctrl Pts',(43.9189401667911,26.91999998,-171.71139261988));
#167681=CARTESIAN_POINT('Ctrl Pts',(43.9948946430299,26.91999998,-171.149949978158));
#167682=CARTESIAN_POINT('Ctrl Pts',(43.7459157865524,26.3030441696697,-171.604534812847));
#167683=CARTESIAN_POINT('Ctrl Pts',(43.7068322349107,26.91999998,-171.744547621103));
#167684=CARTESIAN_POINT('Ctrl Pts',(43.8763450763459,26.91999998,-171.127242425404));
#167685=CARTESIAN_POINT('Ctrl Pts',(43.4976348610037,26.2230846254426,-171.46374657232));
#167686=CARTESIAN_POINT('Ctrl Pts',(43.3564708632233,26.91999998,-171.726334995184));
#167687=CARTESIAN_POINT('Ctrl Pts',(43.7162275365378,26.91999998,-171.05684827667));
#167688=CARTESIAN_POINT('Ctrl Pts',(43.4182794830488,26.1974705898599,-171.403866413424));
#167689=CARTESIAN_POINT('Ctrl Pts',(43.2222824786043,26.91999998,-171.705069685313));
#167690=CARTESIAN_POINT('Ctrl Pts',(43.665002290469,26.91999998,-171.026908215035));
#167691=CARTESIAN_POINT('Ctrl Pts',(43.2765868661323,26.1516592710682,-171.257703672334));
#167692=CARTESIAN_POINT('Ctrl Pts',(42.9355727403744,26.91999998,-171.608576267085));
#167693=CARTESIAN_POINT('Ctrl Pts',(43.5734725485514,26.91999998,-170.953826827844));
#167694=CARTESIAN_POINT('Ctrl Pts',(43.2149501334587,26.1316898999239,-171.173001781957));
#167695=CARTESIAN_POINT('Ctrl Pts',(42.7841822677167,26.9199999800006,-171.530641542159));
#167696=CARTESIAN_POINT('Ctrl Pts',(43.5336346878404,26.91999998,-170.91149625204));
#167697=CARTESIAN_POINT('Ctrl Pts',(43.1661128544364,26.1158519257145,-171.07256826174));
#167698=CARTESIAN_POINT('Ctrl Pts',(42.6444458925863,26.91999998,-171.400720533971));
#167699=CARTESIAN_POINT('Ctrl Pts',(43.5020331013479,26.91999998,-170.861259130871));
#167700=CARTESIAN_POINT('',(43.5020331013479,26.91999998,-170.861259130871));
#167701=CARTESIAN_POINT('Origin',(43.5020331013479,26.41999998,-170.861259130871));
#167702=CARTESIAN_POINT('Ctrl Pts',(43.5020331013479,26.91999998,-170.861259130871));
#167703=CARTESIAN_POINT('Ctrl Pts',(43.5336466193108,26.91999998,-170.911515457779));
#167704=CARTESIAN_POINT('Ctrl Pts',(43.5734840835972,26.91999998,-170.953836204196));
#167705=CARTESIAN_POINT('Ctrl Pts',(43.61923735557,26.91999998,-170.99036760152));
#167706=CARTESIAN_POINT('Ctrl Pts',(43.6650022527906,26.91999998,-171.026908280947));
#167707=CARTESIAN_POINT('Ctrl Pts',(43.7162207484477,26.91999998,-171.056845311872));
#167708=CARTESIAN_POINT('Ctrl Pts',(43.7696000450754,26.91999998,-171.080313003677));
#167709=CARTESIAN_POINT('Ctrl Pts',(43.8006630727512,26.91999998,-171.093969563544));
#167710=CARTESIAN_POINT('Ctrl Pts',(43.8326179990561,26.91999998,-171.105532778688));
#167711=CARTESIAN_POINT('Ctrl Pts',(43.8652115257656,26.91999998,-171.115097339925));
#167712=CARTESIAN_POINT('Ctrl Pts',(43.8987093663281,26.91999998,-171.124927271807));
#167713=CARTESIAN_POINT('Ctrl Pts',(43.9328831236168,26.91999998,-171.132646173148));
#167714=CARTESIAN_POINT('Ctrl Pts',(43.9674767132985,26.91999998,-171.138304320373));
#167715=CARTESIAN_POINT('Ctrl Pts',(44.0018197383426,26.91999998,-171.143921485104));
#167716=CARTESIAN_POINT('Ctrl Pts',(44.0365780353938,26.91999998,-171.147507459409));
#167717=CARTESIAN_POINT('Ctrl Pts',(44.0714975023725,26.91999998,-171.149061689887));
#167718=CARTESIAN_POINT('Ctrl Pts',(44.084788827213,26.91999998,-171.149653273435));
#167719=CARTESIAN_POINT('Ctrl Pts',(44.0981033481739,26.91999998,-171.14995));
#167720=CARTESIAN_POINT('Ctrl Pts',(44.1114262156583,26.91999998,-171.14995));
#167721=CARTESIAN_POINT('Ctrl Pts',(41.0569324495328,26.91999998,-167.025025538602));
#167722=CARTESIAN_POINT('Ctrl Pts',(40.1792441039419,26.91999998,-167.592179375447));
#167723=CARTESIAN_POINT('Ctrl Pts',(40.7299249439265,26.10628905815,-167.236334669472));
#167724=CARTESIAN_POINT('Ctrl Pts',(41.879954591083,26.91999998,-168.29867810854));
#167725=CARTESIAN_POINT('Ctrl Pts',(41.0020315723371,26.9199999800235,-168.844852386549));
#167726=CARTESIAN_POINT('Ctrl Pts',(41.5498055229506,26.1095638122232,-168.509987294195));
#167727=CARTESIAN_POINT('Ctrl Pts',(42.6945981803054,26.91999998,-169.577671730211));
#167728=CARTESIAN_POINT('Ctrl Pts',(41.8241014260219,26.9199999799921,-170.115499778852));
#167729=CARTESIAN_POINT('Ctrl Pts',(42.361486708359,26.1127497675934,-169.788980903725));
#167730=CARTESIAN_POINT('Ctrl Pts',(43.502033101348,26.91999998,-170.861259130871));
#167731=CARTESIAN_POINT('Ctrl Pts',(42.6444458925864,26.91999998,-171.400720533971));
#167732=CARTESIAN_POINT('Ctrl Pts',(43.1661128544364,26.1158519257145,-171.07256826174));
#167733=CARTESIAN_POINT('',(41.0569324495328,26.91999998,-167.025025538602));
#167734=CARTESIAN_POINT('Origin',(41.0569324495328,26.41999998,-167.025025538602));
#167735=CARTESIAN_POINT('Ctrl Pts',(41.0569324495328,26.91999998,-167.025025538602));
#167736=CARTESIAN_POINT('Ctrl Pts',(41.879954591083,26.91999998,-168.29867810854));
#167737=CARTESIAN_POINT('Ctrl Pts',(42.6945981803054,26.91999998,-169.577671730211));
#167738=CARTESIAN_POINT('Ctrl Pts',(43.502033101348,26.91999998,-170.861259130871));
#167739=CARTESIAN_POINT('Ctrl Pts',(40.7299249439254,26.1062890581509,-167.236334669472));
#167740=CARTESIAN_POINT('Ctrl Pts',(40.1792441039429,26.91999998,-167.592179375443));
#167741=CARTESIAN_POINT('Ctrl Pts',(41.0569324495329,26.91999998,-167.025025538602));
#167742=CARTESIAN_POINT('Ctrl Pts',(40.4102462106017,26.1294636129469,-166.776026902216));
#167743=CARTESIAN_POINT('Ctrl Pts',(39.9306704790183,26.9199999799922,-167.069096608359));
#167744=CARTESIAN_POINT('Ctrl Pts',(40.7691972872111,26.91999998,-166.579746336928));
#167745=CARTESIAN_POINT('Ctrl Pts',(40.151813332835,26.1538945559334,-166.290857209798));
#167746=CARTESIAN_POINT('Ctrl Pts',(39.7259665151012,26.91999998,-166.517209541042));
#167747=CARTESIAN_POINT('Ctrl Pts',(40.5366320006225,26.91999998,-166.110608556751));
#167748=CARTESIAN_POINT('Ctrl Pts',(39.8265523607132,26.1917953794806,-165.538288752884));
#167749=CARTESIAN_POINT('Ctrl Pts',(39.4788563322456,26.91999998,-165.67366929337));
#167750=CARTESIAN_POINT('Ctrl Pts',(40.2438971241064,26.91999998,-165.383070268286));
#167751=CARTESIAN_POINT('Ctrl Pts',(39.7288584282001,26.2046468301746,-165.283122127771));
#167752=CARTESIAN_POINT('Ctrl Pts',(39.4079009250289,26.91999998,-165.399136176622));
#167753=CARTESIAN_POINT('Ctrl Pts',(40.1559725857258,26.91999998,-165.136425734968));
#167754=CARTESIAN_POINT('Ctrl Pts',(39.5527294533689,26.2307412681496,-164.765032944851));
#167755=CARTESIAN_POINT('Ctrl Pts',(39.2839209216265,26.91999998,-164.848652791671));
#167756=CARTESIAN_POINT('Ctrl Pts',(39.9974565076864,26.91999998,-164.635718209756));
#167757=CARTESIAN_POINT('Ctrl Pts',(39.4741198514661,26.2440255255985,-164.501291002302));
#167758=CARTESIAN_POINT('Ctrl Pts',(39.2299261071797,26.91999998,-164.57143444594));
#167759=CARTESIAN_POINT('Ctrl Pts',(39.9267078667251,26.91999998,-164.380863661625));
#167760=CARTESIAN_POINT('Ctrl Pts',(39.2672961864197,26.2840285028959,-163.707086385033));
#167761=CARTESIAN_POINT('Ctrl Pts',(39.0964160674726,26.91999998,-163.760078926904));
#167762=CARTESIAN_POINT('Ctrl Pts',(39.7405665669667,26.91999998,-163.613547303229));
#167763=CARTESIAN_POINT('Ctrl Pts',(39.1671866999672,26.3109338019081,-163.172923345691));
#167764=CARTESIAN_POINT('Ctrl Pts',(39.0354484142071,26.919999979999,-163.210393447583));
#167765=CARTESIAN_POINT('Ctrl Pts',(39.6504680302044,26.91999998,-163.097634164455));
#167766=CARTESIAN_POINT('Ctrl Pts',(39.0334891635878,26.3651575479723,-162.096254993545));
#167767=CARTESIAN_POINT('Ctrl Pts',(38.9750776668959,26.9199999800009,-162.116493741208));
#167768=CARTESIAN_POINT('Ctrl Pts',(39.530140246995,26.91999998,-162.058113878045));
#167769=CARTESIAN_POINT('Ctrl Pts',(39.,26.3924773748256,-161.553722423305));
#167770=CARTESIAN_POINT('Ctrl Pts',(38.9716965848467,26.9199999800009,-161.56923273356));
#167771=CARTESIAN_POINT('Ctrl Pts',(39.5000000005343,26.91999998,-161.534480343589));
#167772=CARTESIAN_POINT('Ctrl Pts',(39.,26.41999998,-161.0070032805));
#167773=CARTESIAN_POINT('Ctrl Pts',(39.,26.91999998,-161.0070032805));
#167774=CARTESIAN_POINT('Ctrl Pts',(39.5,26.91999998,-161.0070032805));
#167775=CARTESIAN_POINT('',(39.5,26.91999998,-161.0070032805));
#167776=CARTESIAN_POINT('Origin',(39.5,26.41999998,-161.0070032805));
#167777=CARTESIAN_POINT('Ctrl Pts',(39.5,26.91999998,-161.0070032805));
#167778=CARTESIAN_POINT('Ctrl Pts',(39.5,26.91999998,-161.534495292789));
#167779=CARTESIAN_POINT('Ctrl Pts',(39.5301402469972,26.91999998,-162.058113878039));
#167780=CARTESIAN_POINT('Ctrl Pts',(39.5903041384792,26.91999998,-162.577874021264));
#167781=CARTESIAN_POINT('Ctrl Pts',(39.6504680299611,26.91999998,-163.097634164489));
#167782=CARTESIAN_POINT('Ctrl Pts',(39.7405665669947,26.91999998,-163.613547303305));
#167783=CARTESIAN_POINT('Ctrl Pts',(39.864660766352,26.91999998,-164.12509154227));
#167784=CARTESIAN_POINT('Ctrl Pts',(39.9267078660346,26.91999998,-164.380863661769));
#167785=CARTESIAN_POINT('Ctrl Pts',(39.997456507107,26.91999998,-164.6357182099));
#167786=CARTESIAN_POINT('Ctrl Pts',(40.0767145462179,26.91999998,-164.886071972517));
#167787=CARTESIAN_POINT('Ctrl Pts',(40.1559725853186,26.91999998,-165.136425735101));
#167788=CARTESIAN_POINT('Ctrl Pts',(40.2438971237555,26.91999998,-165.383070268404));
#167789=CARTESIAN_POINT('Ctrl Pts',(40.3414754155803,26.91999998,-165.625583031388));
#167790=CARTESIAN_POINT('Ctrl Pts',(40.4688793539733,26.91999998,-165.942221912198));
#167791=CARTESIAN_POINT('Ctrl Pts',(40.6122052010724,26.91999998,-166.252046258612));
#167792=CARTESIAN_POINT('Ctrl Pts',(40.7764339005761,26.91999998,-166.552924284035));
#167793=CARTESIAN_POINT('Ctrl Pts',(40.863769731484,26.91999998,-166.712929401482));
#167794=CARTESIAN_POINT('Ctrl Pts',(40.9570176103072,26.91999998,-166.870404192076));
#167795=CARTESIAN_POINT('Ctrl Pts',(41.0569324495328,26.91999998,-167.025025538601));
#167796=CARTESIAN_POINT('Origin',(39.5,26.41999998,-55.24995));
#167797=CARTESIAN_POINT('',(39.5,26.91999998,-71.0516396909898));
#167798=CARTESIAN_POINT('Origin',(39.5,26.41999998,-71.0516396909898));
#167799=CARTESIAN_POINT('',(39.5,26.91999998,-55.24995));
#167800=CARTESIAN_POINT('Ctrl Pts',(39.,26.4199999799992,-71.0516396909892));
#167801=CARTESIAN_POINT('Ctrl Pts',(38.9999999999991,26.91999998,-71.0516396909893));
#167802=CARTESIAN_POINT('Ctrl Pts',(39.5,26.91999998,-71.0516396909898));
#167803=CARTESIAN_POINT('Ctrl Pts',(39.0000000000007,26.3924765441606,-70.5049040476121));
#167804=CARTESIAN_POINT('Ctrl Pts',(38.9716957320515,26.91999998,-70.4893932974167));
#167805=CARTESIAN_POINT('Ctrl Pts',(39.5000000005637,26.91999998,-70.5241467046182));
#167806=CARTESIAN_POINT('Ctrl Pts',(39.033491503913,26.3651705337364,-69.9626458947041));
#167807=CARTESIAN_POINT('Ctrl Pts',(38.9750894758337,26.91999998,-69.9424423105591));
#167808=CARTESIAN_POINT('Ctrl Pts',(39.530142353303,26.91999998,-70.0007779304057));
#167809=CARTESIAN_POINT('Ctrl Pts',(39.1669830003526,26.3110025024839,-68.8870836756328));
#167810=CARTESIAN_POINT('Ctrl Pts',(39.0353396916727,26.91999998,-68.8496793569739));
#167811=CARTESIAN_POINT('Ctrl Pts',(39.6502847005361,26.91999998,-68.962325974017));
#167812=CARTESIAN_POINT('Ctrl Pts',(39.2668900453864,26.2841390411479,-68.3537511575017));
#167813=CARTESIAN_POINT('Ctrl Pts',(39.096159008118,26.91999998,-68.300908425027));
#167814=CARTESIAN_POINT('Ctrl Pts',(39.7402010400563,26.91999998,-68.4472152479348));
#167815=CARTESIAN_POINT('Ctrl Pts',(39.5417383881002,26.2309152444135,-67.2970652120671));
#167816=CARTESIAN_POINT('Ctrl Pts',(39.2771671667713,26.9199999800001,-67.1992781955699));
#167817=CARTESIAN_POINT('Ctrl Pts',(39.9875645500817,26.91999998,-67.4263054007275));
#167818=CARTESIAN_POINT('Ctrl Pts',(39.717260119628,26.2045403217606,-66.7734209576797));
#167819=CARTESIAN_POINT('Ctrl Pts',(39.4035340747194,26.91999998,-66.6423091570439));
#167820=CARTESIAN_POINT('Ctrl Pts',(40.1455341066151,26.91999998,-66.9202222962256));
#167821=CARTESIAN_POINT('Ctrl Pts',(40.1516150766926,26.1539079466874,-65.7680517499882));
#167822=CARTESIAN_POINT('Ctrl Pts',(39.7258338602466,26.91999998,-65.5416509613312));
#167823=CARTESIAN_POINT('Ctrl Pts',(40.5364535700734,26.91999998,-65.9482917889975));
#167824=CARTESIAN_POINT('Ctrl Pts',(40.4103610815574,26.1294552845028,-65.2824506673441));
#167825=CARTESIAN_POINT('Ctrl Pts',(39.9307518154148,26.91999998,-64.9893751942709));
#167826=CARTESIAN_POINT('Ctrl Pts',(40.7693010717051,26.91999998,-65.4787360246525));
#167827=CARTESIAN_POINT('Ctrl Pts',(40.7299249439368,26.1062890581501,-64.8223083020179));
#167828=CARTESIAN_POINT('Ctrl Pts',(40.1792441039523,26.91999998,-64.466463596043));
#167829=CARTESIAN_POINT('Ctrl Pts',(41.0569324495432,26.91999998,-65.0336174328882));
#167830=CARTESIAN_POINT('',(41.0569324495432,26.91999998,-65.0336174328882));
#167831=CARTESIAN_POINT('Origin',(41.0569324495432,26.41999998,-65.0336174328882));
#167832=CARTESIAN_POINT('Ctrl Pts',(41.0569324495432,26.91999998,-65.0336174328882));
#167833=CARTESIAN_POINT('Ctrl Pts',(40.8648408575287,26.91999998,-65.3308851945503));
#167834=CARTESIAN_POINT('Ctrl Pts',(40.6972294070544,26.91999998,-65.6389714709824));
#167835=CARTESIAN_POINT('Ctrl Pts',(40.5488568184269,26.91999998,-65.9555599509455));
#167836=CARTESIAN_POINT('Ctrl Pts',(40.4750173837555,26.91999998,-66.1131140827442));
#167837=CARTESIAN_POINT('Ctrl Pts',(40.4059436807378,26.91999998,-66.2727743327563));
#167838=CARTESIAN_POINT('Ctrl Pts',(40.3409938376608,26.91999998,-66.4342570423367));
#167839=CARTESIAN_POINT('Ctrl Pts',(40.1455341065928,26.91999998,-66.9202222963147));
#167840=CARTESIAN_POINT('Ctrl Pts',(39.9875645491708,26.91999998,-67.4263054005813));
#167841=CARTESIAN_POINT('Ctrl Pts',(39.8638827946265,26.91999998,-67.936760324224));
#167842=CARTESIAN_POINT('Ctrl Pts',(39.7402010400822,26.91999998,-68.4472152478667));
#167843=CARTESIAN_POINT('Ctrl Pts',(39.6502847003092,26.91999998,-68.9623259739815));
#167844=CARTESIAN_POINT('Ctrl Pts',(39.5902135268069,26.91999998,-69.4815519521983));
#167845=CARTESIAN_POINT('Ctrl Pts',(39.5301423533046,26.91999998,-70.0007779304152));
#167846=CARTESIAN_POINT('Ctrl Pts',(39.5000000000007,26.91999998,-70.5241306955437));
#167847=CARTESIAN_POINT('Ctrl Pts',(39.5,26.91999998,-71.0516396909898));
#167848=CARTESIAN_POINT('Ctrl Pts',(43.3501517762232,26.91999998,-61.4386408691297));
#167849=CARTESIAN_POINT('Ctrl Pts',(42.4913556541499,26.91999998,-60.8975655472507));
#167850=CARTESIAN_POINT('Ctrl Pts',(43.0147613882085,26.1152677387813,-61.2273317382593));
#167851=CARTESIAN_POINT('Ctrl Pts',(42.5924607769204,26.91999998,-62.641249943458));
#167852=CARTESIAN_POINT('Ctrl Pts',(41.7218722762073,26.9199999800149,-62.1010809579055));
#167853=CARTESIAN_POINT('Ctrl Pts',(42.2597213352523,26.1123501122717,-62.4299407790815));
#167854=CARTESIAN_POINT('Ctrl Pts',(41.828377509759,26.91999998,-63.839782013441));
#167855=CARTESIAN_POINT('Ctrl Pts',(40.950890457431,26.91999998,-63.291651632712));
#167856=CARTESIAN_POINT('Ctrl Pts',(41.4984253110313,26.1093585902154,-63.6284728402189));
#167857=CARTESIAN_POINT('Ctrl Pts',(41.0569324495432,26.91999998,-65.0336174328882));
#167858=CARTESIAN_POINT('Ctrl Pts',(40.1792441039523,26.91999998,-64.466463596043));
#167859=CARTESIAN_POINT('Ctrl Pts',(40.7299249439368,26.1062890581501,-64.8223083020179));
#167860=CARTESIAN_POINT('',(43.3501517762232,26.91999998,-61.4386408691297));
#167861=CARTESIAN_POINT('Origin',(43.3501517762232,26.41999998,-61.4386408691297));
#167862=CARTESIAN_POINT('Ctrl Pts',(43.3501517762232,26.91999998,-61.4386408691297));
#167863=CARTESIAN_POINT('Ctrl Pts',(42.5924607769204,26.91999998,-62.641249943458));
#167864=CARTESIAN_POINT('Ctrl Pts',(41.828377509759,26.91999998,-63.839782013441));
#167865=CARTESIAN_POINT('Ctrl Pts',(41.0569324495432,26.91999998,-65.0336174328882));
#167866=CARTESIAN_POINT('Ctrl Pts',(43.0147613882086,26.1152677387813,-61.2273317382593));
#167867=CARTESIAN_POINT('Ctrl Pts',(42.4913556541499,26.91999998,-60.8975655472507));
#167868=CARTESIAN_POINT('Ctrl Pts',(43.3501517762232,26.91999998,-61.4386408691297));
#167869=CARTESIAN_POINT('Ctrl Pts',(43.0636216624014,26.1311367864154,-61.1268955825468));
#167870=CARTESIAN_POINT('Ctrl Pts',(42.6316122966568,26.9199999800009,-60.7676176413114));
#167871=CARTESIAN_POINT('Ctrl Pts',(43.3818037825525,26.91999998,-61.3884029511195));
#167872=CARTESIAN_POINT('Ctrl Pts',(43.1254911751643,26.1512115744493,-61.0418249229491));
#167873=CARTESIAN_POINT('Ctrl Pts',(42.7839211391678,26.91999998,-60.6895038034116));
#167874=CARTESIAN_POINT('Ctrl Pts',(43.4218378639138,26.91999998,-61.3458874687825));
#167875=CARTESIAN_POINT('Ctrl Pts',(43.2683662178942,26.1974732479793,-60.8948259755643));
#167876=CARTESIAN_POINT('Ctrl Pts',(43.0730867590013,26.91999998,-60.5931776502515));
#167877=CARTESIAN_POINT('Ctrl Pts',(43.5142348068871,26.91999998,-61.2723879804742));
#167878=CARTESIAN_POINT('Ctrl Pts',(43.3469540657763,26.2228767030678,-60.8357750676355));
#167879=CARTESIAN_POINT('Ctrl Pts',(43.2058848140176,26.9199999800003,-60.57262210769));
#167880=CARTESIAN_POINT('Ctrl Pts',(43.5650210354047,26.91999998,-61.2428625417913));
#167881=CARTESIAN_POINT('Ctrl Pts',(43.512870268579,26.2763890014657,-60.7418969884463));
#167882=CARTESIAN_POINT('Ctrl Pts',(43.4490485146957,26.9199999799997,-60.5604852270767));
#167883=CARTESIAN_POINT('Ctrl Pts',(43.6721398787422,26.91999998,-61.1959234862494));
#167884=CARTESIAN_POINT('Ctrl Pts',(43.6010803778225,26.3047810522968,-60.7070015638854));
#167885=CARTESIAN_POINT('Ctrl Pts',(43.5624944559174,26.91999998,-60.5672455602404));
#167886=CARTESIAN_POINT('Ctrl Pts',(43.7290408259741,26.91999998,-61.1784757886431));
#167887=CARTESIAN_POINT('Ctrl Pts',(43.7785234711652,26.3617623367046,-60.6613392327119));
#167888=CARTESIAN_POINT('Ctrl Pts',(43.7695073126827,26.9199999800001,-60.5973801431191));
#167889=CARTESIAN_POINT('Ctrl Pts',(43.8433908708859,26.91999998,-61.1556446096555));
#167890=CARTESIAN_POINT('Ctrl Pts',(43.8687620016371,26.3906766531834,-60.64995));
#167891=CARTESIAN_POINT('Ctrl Pts',(43.8659505814334,26.91999998,-60.6197279239548));
#167892=CARTESIAN_POINT('Ctrl Pts',(43.901489846726,26.91999998,-61.1499500121981));
#167893=CARTESIAN_POINT('Ctrl Pts',(43.9604906504041,26.41999998,-60.64995));
#167894=CARTESIAN_POINT('Ctrl Pts',(43.9604906504041,26.91999998,-60.64995));
#167895=CARTESIAN_POINT('Ctrl Pts',(43.9604906504041,26.91999998,-61.14995));
#167896=CARTESIAN_POINT('',(43.9604906504041,26.91999998,-61.14995));
#167897=CARTESIAN_POINT('',(43.9604906504041,26.41999998,-60.64995));
#167898=CARTESIAN_POINT('Origin',(43.9604906504041,26.41999998,-61.14995));
#167899=CARTESIAN_POINT('Ctrl Pts',(43.0147613882085,26.1152677387814,-61.2273317382593));
#167900=CARTESIAN_POINT('Ctrl Pts',(43.0274763575341,26.1193973798922,-61.2011950859334));
#167901=CARTESIAN_POINT('Ctrl Pts',(43.0415632309696,26.1239712727001,-61.1750984307868));
#167902=CARTESIAN_POINT('Ctrl Pts',(43.0571164447522,26.1290191152281,-61.1492627867981));
#167903=CARTESIAN_POINT('Ctrl Pts',(43.0651699639752,26.131632909226,-61.1358849821584));
#167904=CARTESIAN_POINT('Ctrl Pts',(43.0736161127961,26.1343736036103,-61.1225765741374));
#167905=CARTESIAN_POINT('Ctrl Pts',(43.0824643698387,26.1372441135223,-61.1093641997718));
#167906=CARTESIAN_POINT('Ctrl Pts',(43.0987837821055,26.1425383804549,-61.0849957639026));
#167907=CARTESIAN_POINT('Ctrl Pts',(43.1164700502224,26.148273918697,-61.0609616514732));
#167908=CARTESIAN_POINT('Ctrl Pts',(43.1355429762965,26.1544559569961,-61.0374154010505));
#167909=CARTESIAN_POINT('Ctrl Pts',(43.1465990107172,26.1580395093026,-61.0237663073487));
#167910=CARTESIAN_POINT('Ctrl Pts',(43.1581203006806,26.161772866853,-61.0102803672665));
#167911=CARTESIAN_POINT('Ctrl Pts',(43.1701048827302,26.1656551276577,-60.9969808939406));
#167912=CARTESIAN_POINT('Ctrl Pts',(43.1787950777989,26.1684702115346,-60.9873372520484));
#167913=CARTESIAN_POINT('Ctrl Pts',(43.1877316752268,26.1713644971657,-60.9777879307699));
#167914=CARTESIAN_POINT('Ctrl Pts',(43.1969286965292,26.1743424112143,-60.9683254492567));
#167915=CARTESIAN_POINT('Ctrl Pts',(43.2109826450054,26.1788929552686,-60.9538658516032));
#167916=CARTESIAN_POINT('Ctrl Pts',(43.2255507321307,26.1836083308442,-60.939720140068));
#167917=CARTESIAN_POINT('Ctrl Pts',(43.240679422296,26.1885032267772,-60.92589299095));
#167918=CARTESIAN_POINT('Ctrl Pts',(43.2502919812774,26.1916133754649,-60.917107413019));
#167919=CARTESIAN_POINT('Ctrl Pts',(43.2601309161905,26.1947960145932,-60.9084506542873));
#167920=CARTESIAN_POINT('Ctrl Pts',(43.2702085065296,26.1980550109063,-60.8999260702465));
#167921=CARTESIAN_POINT('Ctrl Pts',(43.2793934354622,26.2010253290599,-60.8921565840934));
#167922=CARTESIAN_POINT('Ctrl Pts',(43.2887784322572,26.2040596634157,-60.8844958212145));
#167923=CARTESIAN_POINT('Ctrl Pts',(43.2983502312506,26.2071536395938,-60.8769643387686));
#167924=CARTESIAN_POINT('Ctrl Pts',(43.3244804473604,26.2155999375393,-60.8564040173416));
#167925=CARTESIAN_POINT('Ctrl Pts',(43.3520269426161,26.2244985424302,-60.8367910129159));
#167926=CARTESIAN_POINT('Ctrl Pts',(43.3809428948479,26.2338324224914,-60.8183059987373));
#167927=CARTESIAN_POINT('Ctrl Pts',(43.384685235144,26.2350404254371,-60.8159136440647));
#167928=CARTESIAN_POINT('Ctrl Pts',(43.3884504656939,26.2362557032945,-60.8135401319426));
#167929=CARTESIAN_POINT('Ctrl Pts',(43.3922384457186,26.2374782060985,-60.8111858058261));
#167930=CARTESIAN_POINT('Ctrl Pts',(43.3958601516481,26.2386470469122,-60.8089348232969));
#167931=CARTESIAN_POINT('Ctrl Pts',(43.4000029195312,26.2399839248036,-60.8063959387213));
#167932=CARTESIAN_POINT('Ctrl Pts',(43.4037184370012,26.2411828803464,-60.8041517225798));
#167933=CARTESIAN_POINT('Ctrl Pts',(43.4058774798864,26.2418795791118,-60.8028476353477));
#167934=CARTESIAN_POINT('Ctrl Pts',(43.4078918169659,26.2425295698655,-60.8016419018772));
#167935=CARTESIAN_POINT('Ctrl Pts',(43.4095725805353,26.2430719505222,-60.8006413710886));
#167936=CARTESIAN_POINT('Ctrl Pts',(43.4162296669324,26.2452201853826,-60.7966785175239));
#167937=CARTESIAN_POINT('Ctrl Pts',(43.4230090840535,26.2474073661611,-60.7927415272842));
#167938=CARTESIAN_POINT('Ctrl Pts',(43.4299120181182,26.24963387702,-60.7888356878748));
#167939=CARTESIAN_POINT('Ctrl Pts',(43.4520200484725,26.2567647244526,-60.7763264540602));
#167940=CARTESIAN_POINT('Ctrl Pts',(43.4754609305302,26.2643201821782,-60.7641300208485));
#167941=CARTESIAN_POINT('Ctrl Pts',(43.5002298509359,26.2722988221321,-60.7524745840402));
#167942=CARTESIAN_POINT('Ctrl Pts',(43.5102299430492,26.2755200822101,-60.7477688705979));
#167943=CARTESIAN_POINT('Ctrl Pts',(43.5204460297338,26.2788101645169,-60.743151597115));
#167944=CARTESIAN_POINT('Ctrl Pts',(43.5308756725033,26.2821682775036,-60.7386388333542));
#167945=CARTESIAN_POINT('Ctrl Pts',(43.5566971886473,26.2904822313576,-60.7274662165276));
#167946=CARTESIAN_POINT('Ctrl Pts',(43.5838500463463,26.299219566432,-60.7169226589352));
#167947=CARTESIAN_POINT('Ctrl Pts',(43.6123323823145,26.3083779270718,-60.7072553544966));
#167948=CARTESIAN_POINT('Ctrl Pts',(43.6266343653468,26.3129766621832,-60.7024010607968));
#167949=CARTESIAN_POINT('Ctrl Pts',(43.6412713379323,26.3176814759652,-60.6977682056505));
#167950=CARTESIAN_POINT('Ctrl Pts',(43.6562406894801,26.3224912600696,-60.6933921846514));
#167951=CARTESIAN_POINT('Ctrl Pts',(43.6594393144061,26.3235190063468,-60.6924571241179));
#167952=CARTESIAN_POINT('Ctrl Pts',(43.6626531147166,26.3245515451493,-60.6915338002814));
#167953=CARTESIAN_POINT('Ctrl Pts',(43.6658820550481,26.3255889226458,-60.6906225673019));
#167954=CARTESIAN_POINT('Ctrl Pts',(43.6683132129433,26.3263699926664,-60.6899364749542));
#167955=CARTESIAN_POINT('Ctrl Pts',(43.6716206439064,26.3274324944764,-60.6890177374869));
#167956=CARTESIAN_POINT('Ctrl Pts',(43.6738444898251,26.3281468390294,-60.6884086503619));
#167957=CARTESIAN_POINT('Ctrl Pts',(43.6745742430091,26.3283812505988,-60.6882087789296));
#167958=CARTESIAN_POINT('Ctrl Pts',(43.6751872771554,26.3285781630476,-60.6880417202069));
#167959=CARTESIAN_POINT('Ctrl Pts',(43.6756142713164,26.3287153133704,-60.6879255590549));
#167960=CARTESIAN_POINT('Ctrl Pts',(43.6800859617517,26.3301516182259,-60.6867090629997));
#167961=CARTESIAN_POINT('Ctrl Pts',(43.6848158056741,26.331670679367,-60.6854534743842));
#167962=CARTESIAN_POINT('Ctrl Pts',(43.6898019198389,26.3332718294864,-60.6841703749843));
#167963=CARTESIAN_POINT('Ctrl Pts',(43.7032213047287,26.3375810869581,-60.6807171037335));
#167964=CARTESIAN_POINT('Ctrl Pts',(43.7185191369564,26.3424921433827,-60.6770466408939));
#167965=CARTESIAN_POINT('Ctrl Pts',(43.735693185848,26.3480028948378,-60.6734097222796));
#167966=CARTESIAN_POINT('Ctrl Pts',(43.7533010892254,26.3536528600713,-60.6696809270516));
#167967=CARTESIAN_POINT('Ctrl Pts',(43.7728812161057,26.3599332090448,-60.6659874477524));
#167968=CARTESIAN_POINT('Ctrl Pts',(43.7944381567387,26.3668435503401,-60.662653882105));
#167969=CARTESIAN_POINT('Ctrl Pts',(43.8163462038058,26.3738664431023,-60.659266021353));
#167970=CARTESIAN_POINT('Ctrl Pts',(43.8402960134949,26.3815400288333,-60.6562500536345));
#167971=CARTESIAN_POINT('Ctrl Pts',(43.8662991796198,26.3898656652239,-60.6540003957982));
#167972=CARTESIAN_POINT('Ctrl Pts',(43.8929368536722,26.3983944569635,-60.651695843657));
#167973=CARTESIAN_POINT('Ctrl Pts',(43.9217293432544,26.4076075212788,-60.6501955756524));
#167974=CARTESIAN_POINT('Ctrl Pts',(43.9526957322241,26.4175079798945,-60.6499774413423));
#167975=CARTESIAN_POINT('Ctrl Pts',(43.9552789029716,26.4183338616306,-60.6499592448981));
#167976=CARTESIAN_POINT('Ctrl Pts',(43.9578772047001,26.419164527574,-60.64995));
#167977=CARTESIAN_POINT('Ctrl Pts',(43.9604906504041,26.41999998,-60.64995));
#167978=CARTESIAN_POINT('Ctrl Pts',(43.9604906504041,26.91999998,-61.14995));
#167979=CARTESIAN_POINT('Ctrl Pts',(43.9014853731981,26.91999998,-61.14995));
#167980=CARTESIAN_POINT('Ctrl Pts',(43.8433879790802,26.91999998,-61.1556451738328));
#167981=CARTESIAN_POINT('Ctrl Pts',(43.7862158462631,26.91999998,-61.1670601882964));
#167982=CARTESIAN_POINT('Ctrl Pts',(43.7290408237003,26.91999998,-61.178475779728));
#167983=CARTESIAN_POINT('Ctrl Pts',(43.6721412316922,26.91999998,-61.1959228882129));
#167984=CARTESIAN_POINT('Ctrl Pts',(43.6185804531072,26.91999998,-61.2193930049692));
#167985=CARTESIAN_POINT('Ctrl Pts',(43.5650151406998,26.91999998,-61.2428651084281));
#167986=CARTESIAN_POINT('Ctrl Pts',(43.5142347717189,26.91999998,-61.2723879193617));
#167987=CARTESIAN_POINT('Ctrl Pts',(43.4680362753946,26.91999998,-61.3091376491944));
#167988=CARTESIAN_POINT('Ctrl Pts',(43.4218479344169,26.91999998,-61.345879300707));
#167989=CARTESIAN_POINT('Ctrl Pts',(43.3818141153598,26.91999998,-61.3883863242137));
#167990=CARTESIAN_POINT('Ctrl Pts',(43.3501517762232,26.91999998,-61.4386408691297));
#167991=CARTESIAN_POINT('Origin',(57.,27.41999998,-58.24995));
#167992=CARTESIAN_POINT('',(57.,26.91999998,-55.74995));
#167993=CARTESIAN_POINT('Origin',(57.,27.41999998,-55.74995));
#167994=CARTESIAN_POINT('',(59.5,26.91999998,-58.24995));
#167995=CARTESIAN_POINT('Origin',(57.,26.91999998,-58.24995));
#167996=CARTESIAN_POINT('Origin',(59.5,27.41999998,-58.24995));
#167997=CARTESIAN_POINT('Origin',(59.5,27.41999998,-55.24995));
#167998=CARTESIAN_POINT('',(59.5,26.91999998,-174.34995));
#167999=CARTESIAN_POINT('',(59.5,26.91999998,-58.24995));
#168000=CARTESIAN_POINT('Origin',(59.5,27.41999998,-174.34995));
#168001=CARTESIAN_POINT('Origin',(57.,27.41999998,-174.34995));
#168002=CARTESIAN_POINT('',(57.,26.91999998,-176.84995));
#168003=CARTESIAN_POINT('Origin',(57.,26.91999998,-174.34995));
#168004=CARTESIAN_POINT('Origin',(57.,27.41999998,-176.84995));
#168005=CARTESIAN_POINT('Origin',(-83.2809572255632,27.41999998,-176.84995));
#168006=CARTESIAN_POINT('',(-83.2809572255632,26.9199999800001,-176.84995));
#168007=CARTESIAN_POINT('Origin',(51.176438378063,26.41999998,-55.24995));
#168008=CARTESIAN_POINT('',(50.676438378063,26.41999998,-172.64995));
#168009=CARTESIAN_POINT('Origin',(51.176438378063,26.41999998,-172.64995));
#168010=CARTESIAN_POINT('',(50.6813043436922,26.35041342952,-171.64995));
#168011=CARTESIAN_POINT('',(51.176438378063,26.91999998,-172.64995));
#168012=CARTESIAN_POINT('',(51.176438378063,26.91999998,-55.24995));
#168013=CARTESIAN_POINT('Origin',(51.176438378063,26.41999998,-172.64995));
#168014=CARTESIAN_POINT('Ctrl Pts',(49.6614955754677,26.91999998,-171.149950013428));
#168015=CARTESIAN_POINT('Ctrl Pts',(49.6615613687869,26.91999998,-171.65003477338));
#168016=CARTESIAN_POINT('Ctrl Pts',(49.6615614228195,26.419915218376,-171.649950001854));
#168017=CARTESIAN_POINT('Ctrl Pts',(49.8598777423236,26.91999998,-171.149923566191));
#168018=CARTESIAN_POINT('Ctrl Pts',(49.7963801113845,26.91999998,-171.659221103016));
#168019=CARTESIAN_POINT('Ctrl Pts',(49.7950967919746,26.4108007878185,-171.649930655763));
#168020=CARTESIAN_POINT('Ctrl Pts',(50.0581153532345,26.91999998,-171.188965548735));
#168021=CARTESIAN_POINT('Ctrl Pts',(49.925805728719,26.91999998,-171.695281914066));
#168022=CARTESIAN_POINT('Ctrl Pts',(49.9285358390788,26.4016930431424,-171.675956808335));
#168023=CARTESIAN_POINT('Ctrl Pts',(50.4245495045741,26.91999998,-171.339270411997));
#168024=CARTESIAN_POINT('Ctrl Pts',(50.158596728211,26.91999998,-171.81002165518));
#168025=CARTESIAN_POINT('Ctrl Pts',(50.1751936156598,26.3848578535179,-171.776157476854));
#168026=CARTESIAN_POINT('Ctrl Pts',(50.5925763632168,26.91999998,-171.450449746589));
#168027=CARTESIAN_POINT('Ctrl Pts',(50.2611581333694,26.9199999800027,-171.889069508911));
#168028=CARTESIAN_POINT('Ctrl Pts',(50.2882982365463,26.3771381960673,-171.850276197782));
#168029=CARTESIAN_POINT('Ctrl Pts',(50.8729854484245,26.91999998,-171.728129909852));
#168030=CARTESIAN_POINT('Ctrl Pts',(50.4287914752885,26.9199999799973,-172.075284894372));
#168031=CARTESIAN_POINT('Ctrl Pts',(50.4770517273591,26.3642554277389,-172.035396209825));
#168032=CARTESIAN_POINT('Ctrl Pts',(50.9852574060669,26.91999998,-171.894521542842));
#168033=CARTESIAN_POINT('Ctrl Pts',(50.4930523894858,26.91999998,-172.182240159756));
#168034=CARTESIAN_POINT('Ctrl Pts',(50.5526265126722,26.3590973697634,-172.14632470545));
#168035=CARTESIAN_POINT('Ctrl Pts',(51.1370394011144,26.91999998,-172.257389581842));
#168036=CARTESIAN_POINT('Ctrl Pts',(50.5794864614573,26.91999998,-172.409795949393));
#168037=CARTESIAN_POINT('Ctrl Pts',(50.6547971380307,26.3521241406573,-172.388239289312));
#168038=CARTESIAN_POINT('Ctrl Pts',(51.1764650716523,26.91999998,-172.453697958273));
#168039=CARTESIAN_POINT('Ctrl Pts',(50.601152291526,26.91999998,-172.529747068595));
#168040=CARTESIAN_POINT('Ctrl Pts',(50.6813362874954,26.350312836992,-172.519113452117));
#168041=CARTESIAN_POINT('Ctrl Pts',(51.1764383645034,26.91999998,-172.65014948338));
#168042=CARTESIAN_POINT('Ctrl Pts',(50.601137585018,26.91999998,-172.650072180543));
#168043=CARTESIAN_POINT('Ctrl Pts',(50.6813183099038,26.3503140627879,-172.650082990804));
#168044=CARTESIAN_POINT('Ctrl Pts',(49.6616970192851,26.91999998,-171.14995));
#168045=CARTESIAN_POINT('Ctrl Pts',(49.8600119386601,26.91999998,-171.149950000016));
#168046=CARTESIAN_POINT('Ctrl Pts',(50.058177378641,26.91999998,-171.18899099047));
#168047=CARTESIAN_POINT('Ctrl Pts',(50.4245495045741,26.91999998,-171.339270411997));
#168048=CARTESIAN_POINT('Ctrl Pts',(50.5925763632168,26.91999998,-171.450449746589));
#168049=CARTESIAN_POINT('Ctrl Pts',(50.8729854484245,26.91999998,-171.728129909852));
#168050=CARTESIAN_POINT('Ctrl Pts',(50.9852574060669,26.91999998,-171.894521542842));
#168051=CARTESIAN_POINT('Ctrl Pts',(51.1370137093498,26.91999998,-172.257328160063));
#168052=CARTESIAN_POINT('Ctrl Pts',(51.176438378046,26.91999998,-172.453565067926));
#168053=CARTESIAN_POINT('Ctrl Pts',(51.176438378063,26.91999998,-172.64995));
#168054=CARTESIAN_POINT('Origin',(-83.2809572255632,20.76999998,-61.14995));
#168055=CARTESIAN_POINT('',(51.1762622162812,20.76999998,-60.64995));
#168056=CARTESIAN_POINT('',(1.41024658483895E-14,20.76999998,-60.64995));
#168057=CARTESIAN_POINT('',(51.1762622162812,20.26999998,-61.14995));
#168058=CARTESIAN_POINT('Origin',(51.1762622162812,20.76999998,-61.14995));
#168059=CARTESIAN_POINT('',(-83.2809572255632,20.2699999800001,-61.14995));
#168060=CARTESIAN_POINT('Origin',(1.64641978096591E-14,26.4199999800001,
-61.14995));
#168061=CARTESIAN_POINT('',(50.6819512673597,26.91999998,-61.14995));
#168062=CARTESIAN_POINT('',(50.6819512673597,26.41999998,-60.64995));
#168063=CARTESIAN_POINT('Origin',(50.6819512673597,26.41999998,-61.14995));
#168064=CARTESIAN_POINT('',(1.64641978096591E-14,26.4199999800001,-60.64995));
#168065=CARTESIAN_POINT('',(-83.2809572255632,26.9199999800001,-61.14995));
#168066=CARTESIAN_POINT('Origin',(0.,-12.9675000200281,-61.64995));
#168067=CARTESIAN_POINT('Origin',(0.,-12.9675000200281,-60.64995));
#168068=CARTESIAN_POINT('Ctrl Pts',(37.,33.02054075664,-60.64995));
#168069=CARTESIAN_POINT('Ctrl Pts',(37.5,33.0205407566399,-60.64995));
#168070=CARTESIAN_POINT('Ctrl Pts',(37.5,33.02054075664,-61.14995));
#168071=CARTESIAN_POINT('Ctrl Pts',(36.9450144953722,32.8396166159335,-60.64995));
#168072=CARTESIAN_POINT('Ctrl Pts',(37.4999999999984,32.829451263505,-60.5918750690658));
#168073=CARTESIAN_POINT('Ctrl Pts',(37.5,32.9079637588407,-61.149950027061));
#168074=CARTESIAN_POINT('Ctrl Pts',(36.8889168804295,32.6559426968113,-60.6963841656953));
#168075=CARTESIAN_POINT('Ctrl Pts',(37.5,32.6176893530803,-60.5649300622629));
#168076=CARTESIAN_POINT('Ctrl Pts',(37.5,32.7934674553098,-61.173167066129));
#168077=CARTESIAN_POINT('Ctrl Pts',(36.8135029743542,32.4100449984504,-60.8387768064376));
#168078=CARTESIAN_POINT('Ctrl Pts',(37.5,32.2741011266166,-60.5989161145872));
#168079=CARTESIAN_POINT('Ctrl Pts',(37.5,32.6399623596936,-61.2443634115781));
#168080=CARTESIAN_POINT('Ctrl Pts',(36.7895122380439,32.3319990572285,-60.8990185151424));
#168081=CARTESIAN_POINT('Ctrl Pts',(37.5,32.1451108386466,-60.6268090630372));
#168082=CARTESIAN_POINT('Ctrl Pts',(37.5,32.5912011068259,-61.27448425119));
#168083=CARTESIAN_POINT('Ctrl Pts',(36.7467810375704,32.1932186054134,-61.0450197081848));
#168084=CARTESIAN_POINT('Ctrl Pts',(37.4999999999999,31.876172903305,-60.7353807030111));
#168085=CARTESIAN_POINT('Ctrl Pts',(37.5,32.5044425233165,-61.3474848604736));
#168086=CARTESIAN_POINT('Ctrl Pts',(36.7283245477951,32.1334017245463,-61.1290643654114));
#168087=CARTESIAN_POINT('Ctrl Pts',(37.5,31.7388049050588,-60.8179479783099));
#168088=CARTESIAN_POINT('Ctrl Pts',(37.5,32.4670287634048,-61.3894925929396));
#168089=CARTESIAN_POINT('Ctrl Pts',(36.7137393100582,32.0861766206928,-61.2273317382593));
#168090=CARTESIAN_POINT('Ctrl Pts',(37.5,31.6156971887288,-60.9443257831194));
#168091=CARTESIAN_POINT('Ctrl Pts',(37.5,32.4374646344434,-61.4386408691296));
#168092=CARTESIAN_POINT('',(37.,33.02054075664,-60.64995));
#168093=CARTESIAN_POINT('',(37.5,33.02054075664,-61.14995));
#168094=CARTESIAN_POINT('Origin',(37.,33.02054075664,-61.14995));
#168095=CARTESIAN_POINT('',(37.5,32.4374646344434,-61.4386408691296));
#168096=CARTESIAN_POINT('Ctrl Pts',(37.5,32.4374646344434,-61.4386408691296));
#168097=CARTESIAN_POINT('Ctrl Pts',(37.5,32.4670379954265,-61.3894770341505));
#168098=CARTESIAN_POINT('Ctrl Pts',(37.5,32.5044515673201,-61.3474771045912));
#168099=CARTESIAN_POINT('Ctrl Pts',(37.5,32.5478217582305,-61.3109844882787));
#168100=CARTESIAN_POINT('Ctrl Pts',(37.5,32.5912010725173,-61.2744841953601));
#168101=CARTESIAN_POINT('Ctrl Pts',(37.5,32.6399569706336,-61.2443658937749));
#168102=CARTESIAN_POINT('Ctrl Pts',(37.5,32.6911307205588,-61.2206312870705));
#168103=CARTESIAN_POINT('Ctrl Pts',(37.5,32.7200261312687,-61.2072294705187));
#168104=CARTESIAN_POINT('Ctrl Pts',(37.5,32.7497820420349,-61.1958060470671));
#168105=CARTESIAN_POINT('Ctrl Pts',(37.5,32.7801663767935,-61.1862777806123));
#168106=CARTESIAN_POINT('Ctrl Pts',(37.5,32.8113193812835,-61.1765084659306));
#168107=CARTESIAN_POINT('Ctrl Pts',(37.5,32.8431343593208,-61.168731309436));
#168108=CARTESIAN_POINT('Ctrl Pts',(37.5,32.8753810744804,-61.1629086143648));
#168109=CARTESIAN_POINT('Ctrl Pts',(37.5,32.9073189135582,-61.1571416921447));
#168110=CARTESIAN_POINT('Ctrl Pts',(37.5,32.9396816981555,-61.1532921099755));
#168111=CARTESIAN_POINT('Ctrl Pts',(37.5,32.9722439056898,-61.1513728702169));
#168112=CARTESIAN_POINT('Ctrl Pts',(37.5,32.9883041294273,-61.1504262691642));
#168113=CARTESIAN_POINT('Ctrl Pts',(37.5,33.0044127038512,-61.14995));
#168114=CARTESIAN_POINT('Ctrl Pts',(37.5,33.02054075664,-61.14995));
#168115=CARTESIAN_POINT('Origin',(37.,32.4374646344434,-61.4386408691297));
#168116=CARTESIAN_POINT('Ctrl Pts',(37.,33.02054075664,-60.64995));
#168117=CARTESIAN_POINT('Ctrl Pts',(36.9924666287437,32.9957529741621,-60.64995));
#168118=CARTESIAN_POINT('Ctrl Pts',(36.985335089206,32.9723043403195,-60.6508183507148));
#168119=CARTESIAN_POINT('Ctrl Pts',(36.9786128679924,32.9502135923693,-60.6522871953885));
#168120=CARTESIAN_POINT('Ctrl Pts',(36.9763217634444,32.942684501688,-60.6527878151398));
#168121=CARTESIAN_POINT('Ctrl Pts',(36.9740781118526,32.9353128465307,-60.6533585216106));
#168122=CARTESIAN_POINT('Ctrl Pts',(36.971881941803,32.9280985200821,-60.6539897266455));
#168123=CARTESIAN_POINT('Ctrl Pts',(36.965231374082,32.9062516842166,-60.6559011778243));
#168124=CARTESIAN_POINT('Ctrl Pts',(36.9590174442728,32.8858515293307,-60.6583648678132));
#168125=CARTESIAN_POINT('Ctrl Pts',(36.9532466191212,32.8669144251051,-60.66113439231));
#168126=CARTESIAN_POINT('Ctrl Pts',(36.9471591964415,32.8469383983284,-60.6640558577488));
#168127=CARTESIAN_POINT('Ctrl Pts',(36.9415662354112,32.8285949580227,-60.6673161203253));
#168128=CARTESIAN_POINT('Ctrl Pts',(36.9364609481188,32.811857241149,-60.6706709359492));
#168129=CARTESIAN_POINT('Ctrl Pts',(36.9310729056594,32.7941925096614,-60.6742115572677));
#168130=CARTESIAN_POINT('Ctrl Pts',(36.9262289085405,32.778319104586,-60.6778566924258));
#168131=CARTESIAN_POINT('Ctrl Pts',(36.9219209635135,32.7642065999614,-60.6813681849314));
#168132=CARTESIAN_POINT('Ctrl Pts',(36.9216127929121,32.7631970561973,-60.6816193809775));
#168133=CARTESIAN_POINT('Ctrl Pts',(36.9213073643478,32.7621965203486,-60.6818699150514));
#168134=CARTESIAN_POINT('Ctrl Pts',(36.9210046743457,32.7612049796934,-60.6821197101778));
#168135=CARTESIAN_POINT('Ctrl Pts',(36.9197702682111,32.7571613579714,-60.6831384046648));
#168136=CARTESIAN_POINT('Ctrl Pts',(36.9185820051841,32.7532673571459,-60.6841446812285));
#168137=CARTESIAN_POINT('Ctrl Pts',(36.9174407986844,32.7495220389772,-60.6851333445339));
#168138=CARTESIAN_POINT('Ctrl Pts',(36.9168701954346,32.7476493798929,-60.6856276761866));
#168139=CARTESIAN_POINT('Ctrl Pts',(36.9163106727964,32.745813915541,-60.6861177217765));
#168140=CARTESIAN_POINT('Ctrl Pts',(36.9157621566578,32.744015541504,-60.6866029019919));
#168141=CARTESIAN_POINT('Ctrl Pts',(36.9153143472532,32.7425473462224,-60.6869990038531));
#168142=CARTESIAN_POINT('Ctrl Pts',(36.9151803653871,32.7421075257166,-60.6871177040467));
#168143=CARTESIAN_POINT('Ctrl Pts',(36.9146094848417,32.7402377771945,-60.687629668855));
#168144=CARTESIAN_POINT('Ctrl Pts',(36.9144811009473,32.7398172941379,-60.6877448033369));
#168145=CARTESIAN_POINT('Ctrl Pts',(36.9143306295394,32.7393245233921,-60.6878799880567));
#168146=CARTESIAN_POINT('Ctrl Pts',(36.9141495553194,32.7387315882737,-60.6880432899671));
#168147=CARTESIAN_POINT('Ctrl Pts',(36.9043380451416,32.7066033872109,-60.696891807198));
#168148=CARTESIAN_POINT('Ctrl Pts',(36.8949659479171,32.6759477413478,-60.7069683211716));
#168149=CARTESIAN_POINT('Ctrl Pts',(36.8860481049607,32.646796740842,-60.7179589785711));
#168150=CARTESIAN_POINT('Ctrl Pts',(36.880623229728,32.6290636924553,-60.7246447820114));
#168151=CARTESIAN_POINT('Ctrl Pts',(36.8753661521547,32.6118864586659,-60.7316693183976));
#168152=CARTESIAN_POINT('Ctrl Pts',(36.870277794653,32.5952643697575,-60.7389662185715));
#168153=CARTESIAN_POINT('Ctrl Pts',(36.8634689774476,32.5730220715484,-60.7487303240677));
#168154=CARTESIAN_POINT('Ctrl Pts',(36.8569610178916,32.5517753515799,-60.7589817870678));
#168155=CARTESIAN_POINT('Ctrl Pts',(36.850751208167,32.5315126220667,-60.7695692092458));
#168156=CARTESIAN_POINT('Ctrl Pts',(36.8469896993187,32.519238745775,-60.7759823980503));
#168157=CARTESIAN_POINT('Ctrl Pts',(36.8433375714303,32.5073258680656,-60.7825189042054));
#168158=CARTESIAN_POINT('Ctrl Pts',(36.8397933289186,32.4957685477639,-60.7891471100307));
#168159=CARTESIAN_POINT('Ctrl Pts',(36.8394079005284,32.4945117152125,-60.789867912485));
#168160=CARTESIAN_POINT('Ctrl Pts',(36.8390237657356,32.4932591453848,-60.790589766835));
#168161=CARTESIAN_POINT('Ctrl Pts',(36.838640943046,32.492010897904,-60.7913125928568));
#168162=CARTESIAN_POINT('Ctrl Pts',(36.8383083204172,32.4909263348163,-60.7919406337175));
#168163=CARTESIAN_POINT('Ctrl Pts',(36.8379766343786,32.4898448569959,-60.7925695226016));
#168164=CARTESIAN_POINT('Ctrl Pts',(36.837645899059,32.4887665099017,-60.7931992041001));
#168165=CARTESIAN_POINT('Ctrl Pts',(36.8367126023148,32.485723539367,-60.7949760923178));
#168166=CARTESIAN_POINT('Ctrl Pts',(36.8359448549989,32.4832205295986,-60.7964541280974));
#168167=CARTESIAN_POINT('Ctrl Pts',(36.8350327265731,32.4802468787299,-60.7982289031365));
#168168=CARTESIAN_POINT('Ctrl Pts',(36.8345500410079,32.4786732644123,-60.799168089186));
#168169=CARTESIAN_POINT('Ctrl Pts',(36.8340269806588,32.4769680487848,-60.8001910085464));
#168170=CARTESIAN_POINT('Ctrl Pts',(36.8334181657035,32.4749833371142,-60.8013915861747));
#168171=CARTESIAN_POINT('Ctrl Pts',(36.8245987446436,32.4462323878243,-60.8187834053606));
#168172=CARTESIAN_POINT('Ctrl Pts',(36.8161386112744,32.4186750863256,-60.8373693003596));
#168173=CARTESIAN_POINT('Ctrl Pts',(36.8080717737016,32.3924160926302,-60.8569388251974));
#168174=CARTESIAN_POINT('Ctrl Pts',(36.7996545921008,32.3650166666973,-60.8773582575852));
#168175=CARTESIAN_POINT('Ctrl Pts',(36.7916655629267,32.3390306165208,-60.8988485370896));
#168176=CARTESIAN_POINT('Ctrl Pts',(36.7841265152786,32.3145232383288,-60.9211850004421));
#168177=CARTESIAN_POINT('Ctrl Pts',(36.778553909317,32.296408223251,-60.9376953495804));
#168178=CARTESIAN_POINT('Ctrl Pts',(36.7732267926098,32.2790999388228,-60.9546683305905));
#168179=CARTESIAN_POINT('Ctrl Pts',(36.7681487604643,32.2626081160615,-60.9720182616034));
#168180=CARTESIAN_POINT('Ctrl Pts',(36.7599928054858,32.2361201852846,-60.9998844215971));
#168181=CARTESIAN_POINT('Ctrl Pts',(36.7525209698787,32.2118726247007,-61.0284772793722));
#168182=CARTESIAN_POINT('Ctrl Pts',(36.7456966945039,32.1897381268672,-61.057655954971));
#168183=CARTESIAN_POINT('Ctrl Pts',(36.7381722170941,32.16533252777,-61.089828496865));
#168184=CARTESIAN_POINT('Ctrl Pts',(36.7314349486327,32.1434956696669,-61.1227130004321));
#168185=CARTESIAN_POINT('Ctrl Pts',(36.7254206591586,32.1240104384723,-61.1560745996167));
#168186=CARTESIAN_POINT('Ctrl Pts',(36.721175758641,32.1102577136761,-61.1796212995642));
#168187=CARTESIAN_POINT('Ctrl Pts',(36.7172906773545,32.0976754369519,-61.2034046454934));
#168188=CARTESIAN_POINT('Ctrl Pts',(36.7137393100582,32.0861766206928,-61.2273317382593));
#168189=CARTESIAN_POINT('Ctrl Pts',(37.5,30.3198029183591,-64.9254179945063));
#168190=CARTESIAN_POINT('Ctrl Pts',(37.5,29.4819543139165,-64.4114488783587));
#168191=CARTESIAN_POINT('Ctrl Pts',(36.7055659807482,29.9753365781776,-64.714108863636));
#168192=CARTESIAN_POINT('Ctrl Pts',(37.5,31.0308541172825,-63.7662953234662));
#168193=CARTESIAN_POINT('Ctrl Pts',(37.5000000000047,30.1937476367692,-63.2670920970213));
#168194=CARTESIAN_POINT('Ctrl Pts',(36.7083606505135,30.6839990376866,-63.5549861665061));
#168195=CARTESIAN_POINT('Ctrl Pts',(37.5,31.7365266751429,-62.6039057229559));
#168196=CARTESIAN_POINT('Ctrl Pts',(37.5,30.9051975556495,-62.1106946535587));
#168197=CARTESIAN_POINT('Ctrl Pts',(36.7110836457466,31.3874027455588,-62.3925965705953));
#168198=CARTESIAN_POINT('Ctrl Pts',(37.5,32.4374646344434,-61.4386408691296));
#168199=CARTESIAN_POINT('Ctrl Pts',(37.5,31.6156971887288,-60.9443257831195));
#168200=CARTESIAN_POINT('Ctrl Pts',(36.7137393100582,32.0861766206928,-61.2273317382593));
#168201=CARTESIAN_POINT('',(37.5,30.3198029183596,-64.9254179945056));
#168202=CARTESIAN_POINT('Ctrl Pts',(37.5,30.3198029183591,-64.9254179945063));
#168203=CARTESIAN_POINT('Ctrl Pts',(37.5,31.0308541172825,-63.7662953234662));
#168204=CARTESIAN_POINT('Ctrl Pts',(37.5,31.7365266751429,-62.6039057229559));
#168205=CARTESIAN_POINT('Ctrl Pts',(37.5,32.4374646344434,-61.4386408691296));
#168206=CARTESIAN_POINT('Origin',(37.,30.3198029183592,-64.9254179945062));
#168207=CARTESIAN_POINT('Ctrl Pts',(36.7055659807485,29.9753365781889,-64.7141088636423));
#168208=CARTESIAN_POINT('Ctrl Pts',(37.5,29.4819543139285,-64.4114488783659));
#168209=CARTESIAN_POINT('Ctrl Pts',(37.5,30.3198029183707,-64.9254179945125));
#168210=CARTESIAN_POINT('Ctrl Pts',(36.7276066422259,29.6936558584646,-65.1425806750807));
#168211=CARTESIAN_POINT('Ctrl Pts',(37.5,29.2617307842025,-64.8907595368038));
#168212=CARTESIAN_POINT('Ctrl Pts',(37.5,30.066275812609,-65.3387061138468));
#168213=CARTESIAN_POINT('Ctrl Pts',(36.7506399492972,29.4626112609503,-65.5904100084171));
#168214=CARTESIAN_POINT('Ctrl Pts',(37.4999999999999,29.0782932545581,-65.3939122854256));
#168215=CARTESIAN_POINT('Ctrl Pts',(37.5,29.8583501338385,-65.770493027413));
#168216=CARTESIAN_POINT('Ctrl Pts',(36.7981064172734,29.0734767074675,-66.5135522731121));
#168217=CARTESIAN_POINT('Ctrl Pts',(37.5,28.7875108426025,-66.3978618624443));
#168218=CARTESIAN_POINT('Ctrl Pts',(37.5,29.5081290337376,-66.6603034853058));
#168219=CARTESIAN_POINT('Ctrl Pts',(36.8225713421442,28.9158110192433,-66.9894827414662));
#168220=CARTESIAN_POINT('Ctrl Pts',(37.5,28.6734901542511,-66.902255679337));
#168221=CARTESIAN_POINT('Ctrl Pts',(37.5,29.3662299161008,-67.1188991703195));
#168222=CARTESIAN_POINT('Ctrl Pts',(36.8977082013987,28.5389562140588,-68.4518423383231));
#168223=CARTESIAN_POINT('Ctrl Pts',(37.5,28.43212483966,-68.3736721849867));
#168224=CARTESIAN_POINT('Ctrl Pts',(37.5,29.0270605890893,-68.5274557979285));
#168225=CARTESIAN_POINT('Ctrl Pts',(36.9485508209842,28.41999998,-69.4422434553462));
#168226=CARTESIAN_POINT('Ctrl Pts',(37.5,28.3657190858733,-69.3869874906105));
#168227=CARTESIAN_POINT('Ctrl Pts',(37.5,28.9199999811121,-69.4807175010263));
#168228=CARTESIAN_POINT('Ctrl Pts',(37.,28.41999998,-70.4461836365688));
#168229=CARTESIAN_POINT('Ctrl Pts',(37.5,28.41999998,-70.4461836365687));
#168230=CARTESIAN_POINT('Ctrl Pts',(37.5,28.91999998,-70.4461836365688));
#168231=CARTESIAN_POINT('',(37.5,28.91999998,-70.4461836365688));
#168232=CARTESIAN_POINT('Ctrl Pts',(37.5,28.91999998,-70.4461836365688));
#168233=CARTESIAN_POINT('Ctrl Pts',(37.5,28.91999998,-69.912174657427));
#168234=CARTESIAN_POINT('Ctrl Pts',(37.5,28.9527491161422,-69.3820227305296));
#168235=CARTESIAN_POINT('Ctrl Pts',(37.5,29.0202545273658,-68.8559643077838));
#168236=CARTESIAN_POINT('Ctrl Pts',(37.5,29.074821691239,-68.4307314910276));
#168237=CARTESIAN_POINT('Ctrl Pts',(37.5,29.1520996751838,-68.0081734812178));
#168238=CARTESIAN_POINT('Ctrl Pts',(37.5,29.2531734731887,-67.5884180460506));
#168239=CARTESIAN_POINT('Ctrl Pts',(37.5,29.3662299152087,-67.1188991701865));
#168240=CARTESIAN_POINT('Ctrl Pts',(37.5,29.5081290337322,-66.6603034853492));
#168241=CARTESIAN_POINT('Ctrl Pts',(37.5,29.6832395831696,-66.2153982561153));
#168242=CARTESIAN_POINT('Ctrl Pts',(37.5,29.8137242360819,-65.8838745152443));
#168243=CARTESIAN_POINT('Ctrl Pts',(37.5,29.9624113407221,-65.5596714884955));
#168244=CARTESIAN_POINT('Ctrl Pts',(37.5,30.1346313217786,-65.24493295738));
#168245=CARTESIAN_POINT('Ctrl Pts',(37.5,30.1935307469803,-65.1372920294355));
#168246=CARTESIAN_POINT('Ctrl Pts',(37.5,30.255183072144,-65.0307582682231));
#168247=CARTESIAN_POINT('Ctrl Pts',(37.5,30.3198029183595,-64.9254179945056));
#168248=CARTESIAN_POINT('Origin',(37.,28.91999998,-70.4461836365688));
#168249=CARTESIAN_POINT('Origin',(37.,28.91999998,-55.24995));
#168250=CARTESIAN_POINT('',(37.5,28.91999998,-91.34995));
#168251=CARTESIAN_POINT('',(37.5,28.91999998,-69.7748183683767));
#168252=CARTESIAN_POINT('',(37.,28.41999998,-91.34995));
#168253=CARTESIAN_POINT('Origin',(37.,28.91999998,-91.34995));
#168254=CARTESIAN_POINT('',(37.,28.41999998,-91.34995));
#168255=CARTESIAN_POINT('Origin',(38.,43.91999998,-58.24995));
#168256=CARTESIAN_POINT('',(38.,46.91999998,-58.24995));
#168257=CARTESIAN_POINT('',(37.5,46.41999998,-58.24995));
#168258=CARTESIAN_POINT('Origin',(38.,46.41999998,-58.24995));
#168259=CARTESIAN_POINT('',(37.5,43.91999998,-55.74995));
#168260=CARTESIAN_POINT('Origin',(37.5,43.91999998,-58.24995));
#168261=CARTESIAN_POINT('',(38.,43.91999998,-55.24995));
#168262=CARTESIAN_POINT('Origin',(38.,43.91999998,-55.74995));
#168263=CARTESIAN_POINT('Origin',(38.,43.91999998,-58.24995));
#168264=CARTESIAN_POINT('Origin',(0.,43.91999998,-58.24995));
#168265=CARTESIAN_POINT('',(38.5,43.91999998,-55.24995));
#168266=CARTESIAN_POINT('',(0.,43.91999998,-55.24995));
#168267=CARTESIAN_POINT('',(38.5,46.91999998,-58.24995));
#168268=CARTESIAN_POINT('Origin',(38.5,43.91999998,-58.24995));
#168269=CARTESIAN_POINT('',(-39.,46.91999998,-58.24995));
#168270=CARTESIAN_POINT('Origin',(38.5,43.91999998,-58.24995));
#168271=CARTESIAN_POINT('',(39.,43.91999998,-55.74995));
#168272=CARTESIAN_POINT('Origin',(38.5,43.91999998,-55.74995));
#168273=CARTESIAN_POINT('',(39.,46.41999998,-58.24995));
#168274=CARTESIAN_POINT('Origin',(39.,43.91999998,-58.24995));
#168275=CARTESIAN_POINT('Origin',(38.5,46.41999998,-58.24995));
#168276=CARTESIAN_POINT('Origin',(38.5,46.41999998,-129.34995));
#168277=CARTESIAN_POINT('',(39.,46.41999998,-91.9958480337503));
#168278=CARTESIAN_POINT('',(39.,46.41999998,-129.34995));
#168279=CARTESIAN_POINT('',(38.5,46.91999998,-91.84995));
#168280=CARTESIAN_POINT('Ctrl Pts',(39.,46.41999998,-91.9958480337503));
#168281=CARTESIAN_POINT('Ctrl Pts',(39.,46.4383593062444,-91.9958480337503));
#168282=CARTESIAN_POINT('Ctrl Pts',(38.9989710148889,46.4572833490541,-91.9952104626986));
#168283=CARTESIAN_POINT('Ctrl Pts',(38.9967508671932,46.4766440820793,-91.9938816236437));
#168284=CARTESIAN_POINT('Ctrl Pts',(38.9953313980197,46.4890225214778,-91.9930320197733));
#168285=CARTESIAN_POINT('Ctrl Pts',(38.9934248666238,46.5015785833831,-91.9919000447932));
#168286=CARTESIAN_POINT('Ctrl Pts',(38.9909875853142,46.5142679203736,-91.9904744337629));
#168287=CARTESIAN_POINT('Ctrl Pts',(38.9879236812039,46.5302196743252,-91.9886822994377));
#168288=CARTESIAN_POINT('Ctrl Pts',(38.9840210150448,46.5463837492805,-91.9864258165825));
#168289=CARTESIAN_POINT('Ctrl Pts',(38.9791896661436,46.5626525596803,-91.9836879413693));
#168290=CARTESIAN_POINT('Ctrl Pts',(38.9767739916931,46.5707869648802,-91.9823190037628));
#168291=CARTESIAN_POINT('Ctrl Pts',(38.9741260943782,46.5789471626428,-91.9808298188763));
#168292=CARTESIAN_POINT('Ctrl Pts',(38.9712345064629,46.5871170280941,-91.9792189642192));
#168293=CARTESIAN_POINT('Ctrl Pts',(38.9697887125053,46.5912019608197,-91.9784135368906));
#168294=CARTESIAN_POINT('Ctrl Pts',(38.9682819877514,46.5952892977622,-91.9775776967405));
#168295=CARTESIAN_POINT('Ctrl Pts',(38.9667128998072,46.5993768111374,-91.9767113231393));
#168296=CARTESIAN_POINT('Ctrl Pts',(38.9665488507948,46.5998041629213,-91.9766207433001));
#168297=CARTESIAN_POINT('Ctrl Pts',(38.9663841201167,46.6002315164782,-91.9765298297484));
#168298=CARTESIAN_POINT('Ctrl Pts',(38.9662187061398,46.6006588691706,-91.976438582373));
#168299=CARTESIAN_POINT('Ctrl Pts',(38.9660815493286,46.6010132185049,-91.9763629225087));
#168300=CARTESIAN_POINT('Ctrl Pts',(38.9659442495352,46.6013667545193,-91.9762872126274));
#168301=CARTESIAN_POINT('Ctrl Pts',(38.9658014814792,46.6017330596689,-91.9762085198219));
#168302=CARTESIAN_POINT('Ctrl Pts',(38.964878272724,46.6041017696637,-91.9756996532795));
#168303=CARTESIAN_POINT('Ctrl Pts',(38.9637824718195,46.6068475079059,-91.9750972858545));
#168304=CARTESIAN_POINT('Ctrl Pts',(38.9628075054374,46.6092327396235,-91.9745628844117));
#168305=CARTESIAN_POINT('Ctrl Pts',(38.9623758791192,46.6102887029911,-91.9743263001239));
#168306=CARTESIAN_POINT('Ctrl Pts',(38.9619686005258,46.611274297802,-91.9741033520448));
#168307=CARTESIAN_POINT('Ctrl Pts',(38.9616138110508,46.6121267335955,-91.9739093074448));
#168308=CARTESIAN_POINT('Ctrl Pts',(38.9614200658218,46.6125922360406,-91.9738033425893));
#168309=CARTESIAN_POINT('Ctrl Pts',(38.9612419963564,46.6130180505684,-91.973706020483));
#168310=CARTESIAN_POINT('Ctrl Pts',(38.9610842933711,46.6133939988585,-91.9736198702739));
#168311=CARTESIAN_POINT('Ctrl Pts',(38.9610119987885,46.6135663419795,-91.9735803770874));
#168312=CARTESIAN_POINT('Ctrl Pts',(38.9609443960246,46.6137272414247,-91.9735434559988));
#168313=CARTESIAN_POINT('Ctrl Pts',(38.9608751120365,46.6138919016539,-91.973505625203));
#168314=CARTESIAN_POINT('Ctrl Pts',(38.9567213876535,46.6237636372138,-91.9712375874808));
#168315=CARTESIAN_POINT('Ctrl Pts',(38.9518680842499,46.6344001787413,-91.9686174080448));
#168316=CARTESIAN_POINT('Ctrl Pts',(38.946177595039,46.6456366502153,-91.9656152575245));
#168317=CARTESIAN_POINT('Ctrl Pts',(38.9401988073236,46.657442397511,-91.9624610083931));
#168318=CARTESIAN_POINT('Ctrl Pts',(38.9333015040993,46.6699024228789,-91.9588870343257));
#168319=CARTESIAN_POINT('Ctrl Pts',(38.9252978398083,46.6828446406519,-91.9548765239483));
#168320=CARTESIAN_POINT('Ctrl Pts',(38.9201412478996,46.6911830382935,-91.9522926367924));
#168321=CARTESIAN_POINT('Ctrl Pts',(38.9145249398867,46.6997211758053,-91.949528013274));
#168322=CARTESIAN_POINT('Ctrl Pts',(38.9083979295449,46.7084008365676,-91.9465877544647));
#168323=CARTESIAN_POINT('Ctrl Pts',(38.9009630650995,46.7189332328916,-91.9430198764193));
#168324=CARTESIAN_POINT('Ctrl Pts',(38.892777050832,46.7296758500678,-91.9391926280371));
#168325=CARTESIAN_POINT('Ctrl Pts',(38.8837164293804,46.7405353151116,-91.9351210844034));
#168326=CARTESIAN_POINT('Ctrl Pts',(38.8751108750016,46.7508493666871,-91.9312540328625));
#168327=CARTESIAN_POINT('Ctrl Pts',(38.8657161059638,46.7612691278656,-91.9271661831289));
#168328=CARTESIAN_POINT('Ctrl Pts',(38.8554209343761,46.7716757316366,-91.9228953364302));
#168329=CARTESIAN_POINT('Ctrl Pts',(38.8548765192935,46.7722260393225,-91.922669491398));
#168330=CARTESIAN_POINT('Ctrl Pts',(38.8543295855841,46.7727763000726,-91.9224431416288));
#168331=CARTESIAN_POINT('Ctrl Pts',(38.8537801165802,46.7733264928175,-91.9222162951506));
#168332=CARTESIAN_POINT('Ctrl Pts',(38.8536544843425,46.7734522905335,-91.9221644282928));
#168333=CARTESIAN_POINT('Ctrl Pts',(38.85352882043,46.7735779836955,-91.9221125901406));
#168334=CARTESIAN_POINT('Ctrl Pts',(38.8534031249738,46.7737035723748,-91.9220607807091));
#168335=CARTESIAN_POINT('Ctrl Pts',(38.8462316750874,46.7808689301918,-91.9191048366159));
#168336=CARTESIAN_POINT('Ctrl Pts',(38.8389362233865,46.7877118845293,-91.9162395555616));
#168337=CARTESIAN_POINT('Ctrl Pts',(38.8315472950243,46.7942461691172,-91.9134652859837));
#168338=CARTESIAN_POINT('Ctrl Pts',(38.8181190696914,46.8061212126327,-91.9084234835463));
#168339=CARTESIAN_POINT('Ctrl Pts',(38.804374545969,46.8169853430965,-91.9036748558894));
#168340=CARTESIAN_POINT('Ctrl Pts',(38.7904695579344,46.8269040598907,-91.8992337321801));
#168341=CARTESIAN_POINT('Ctrl Pts',(38.7771257367623,46.8364224847054,-91.8949718399416));
#168342=CARTESIAN_POINT('Ctrl Pts',(38.7636334875039,46.8450704493382,-91.8909923724618));
#168343=CARTESIAN_POINT('Ctrl Pts',(38.7500931237289,46.8529065841947,-91.887282952442));
#168344=CARTESIAN_POINT('Ctrl Pts',(38.7362680437785,46.8609074911639,-91.8834955336402));
#168345=CARTESIAN_POINT('Ctrl Pts',(38.7223990660432,46.8680567950519,-91.8799962545976));
#168346=CARTESIAN_POINT('Ctrl Pts',(38.7086077471669,46.8743998864685,-91.8767851783845));
#168347=CARTESIAN_POINT('Ctrl Pts',(38.7029413913131,46.8770060341112,-91.8754658629034));
#168348=CARTESIAN_POINT('Ctrl Pts',(38.697284315972,46.8794776843018,-91.8741947680128));
#168349=CARTESIAN_POINT('Ctrl Pts',(38.6916560145369,46.8818135523074,-91.8729730791622));
#168350=CARTESIAN_POINT('Ctrl Pts',(38.690434966776,46.8823203137933,-91.8727080364219));
#168351=CARTESIAN_POINT('Ctrl Pts',(38.6892145306102,46.8828209021287,-91.8724452601857));
#168352=CARTESIAN_POINT('Ctrl Pts',(38.6879949385285,46.8833153304816,-91.8721847293447));
#168353=CARTESIAN_POINT('Ctrl Pts',(38.6845743466761,46.8847020544697,-91.8714540180803));
#168354=CARTESIAN_POINT('Ctrl Pts',(38.6811624576419,46.8860394931494,-91.870741323611));
#168355=CARTESIAN_POINT('Ctrl Pts',(38.6777616037319,46.8873292507991,-91.8700466429565));
#168356=CARTESIAN_POINT('Ctrl Pts',(38.6743607498219,46.8886190084487,-91.8693519623019));
#168357=CARTESIAN_POINT('Ctrl Pts',(38.6709709301683,46.8898610847578,-91.8686752954307));
#168358=CARTESIAN_POINT('Ctrl Pts',(38.6675943952643,46.8910570583194,-91.8680166390568));
#168359=CARTESIAN_POINT('Ctrl Pts',(38.6521588071316,46.8965243660297,-91.8650056384902));
#168360=CARTESIAN_POINT('Ctrl Pts',(38.6369789277987,46.9010399726731,-91.8623722770382));
#168361=CARTESIAN_POINT('Ctrl Pts',(38.6221553104875,46.9047591974349,-91.8601140144284));
#168362=CARTESIAN_POINT('Ctrl Pts',(38.6073316931762,46.9084784221968,-91.8578557518186));
#168363=CARTESIAN_POINT('Ctrl Pts',(38.5928631234692,46.9114011072647,-91.8559725211624));
#168364=CARTESIAN_POINT('Ctrl Pts',(38.5788026188502,46.9136563357898,-91.8544668874172));
#168365=CARTESIAN_POINT('Ctrl Pts',(38.5647421142311,46.915911564315,-91.8529612536721));
#168366=CARTESIAN_POINT('Ctrl Pts',(38.5510974137732,46.917496438632,-91.8518320044153));
#168367=CARTESIAN_POINT('Ctrl Pts',(38.5379391593889,46.918518762006,-91.851079193558));
#168368=CARTESIAN_POINT('Ctrl Pts',(38.5313600321968,46.919029923693,-91.8507027881294));
#168369=CARTESIAN_POINT('Ctrl Pts',(38.5249025899683,46.9194002702488,-91.8504204897178));
#168370=CARTESIAN_POINT('Ctrl Pts',(38.5185762063117,46.9196427903307,-91.8502322928751));
#168371=CARTESIAN_POINT('Ctrl Pts',(38.512249822655,46.9198853104125,-91.8500440960323));
#168372=CARTESIAN_POINT('Ctrl Pts',(38.5060545004698,46.91999998,-91.8499500002645));
#168373=CARTESIAN_POINT('Ctrl Pts',(38.5,46.91999998,-91.84995));
#168374=CARTESIAN_POINT('',(38.5,46.91999998,-129.34995));
#168375=CARTESIAN_POINT('Origin',(40.,31.080768958446,-179.64995));
#168376=CARTESIAN_POINT('',(39.,31.080768958446,-91.9958480337503));
#168377=CARTESIAN_POINT('Ctrl Pts',(39.3277310924369,30.3404619167909,-92.0491293459315));
#168378=CARTESIAN_POINT('Ctrl Pts',(39.2886346270581,30.3759652101421,-92.0422366709188));
#168379=CARTESIAN_POINT('Ctrl Pts',(39.2523153224603,30.4148006640942,-92.0360096476917));
#168380=CARTESIAN_POINT('Ctrl Pts',(39.219197064997,30.4564585863616,-92.0304533816565));
#168381=CARTESIAN_POINT('Ctrl Pts',(39.1844077477968,30.5002184572809,-92.024616761123));
#168382=CARTESIAN_POINT('Ctrl Pts',(39.1531513695584,30.5470922331216,-92.0195203571601));
#168383=CARTESIAN_POINT('Ctrl Pts',(39.125895733847,30.5964367240933,-92.0151624600667));
#168384=CARTESIAN_POINT('Ctrl Pts',(39.112241386304,30.6211569997895,-92.0129792696946));
#168385=CARTESIAN_POINT('Ctrl Pts',(39.099590693715,30.6464966177574,-92.0109813029423));
#168386=CARTESIAN_POINT('Ctrl Pts',(39.0879995509094,30.6723709176288,-92.0091676111272));
#168387=CARTESIAN_POINT('Ctrl Pts',(39.067970142895,30.7170815141512,-92.0060335652451));
#168388=CARTESIAN_POINT('Ctrl Pts',(39.0510881489839,30.7634337254292,-92.0034479181842));
#168389=CARTESIAN_POINT('Ctrl Pts',(39.0376514204517,30.8109406522508,-92.0014180562603));
#168390=CARTESIAN_POINT('Ctrl Pts',(39.0245645049345,30.857210779411,-91.9994410399468));
#168391=CARTESIAN_POINT('Ctrl Pts',(39.0147461926495,30.9045752998721,-91.9979911959902));
#168392=CARTESIAN_POINT('Ctrl Pts',(39.0084275646637,30.9525664602203,-91.9970678562248));
#168393=CARTESIAN_POINT('Ctrl Pts',(39.0028510130954,30.9949214115026,-91.9962529559286));
#168394=CARTESIAN_POINT('Ctrl Pts',(39.,31.0377638135206,-91.9958480382673));
#168395=CARTESIAN_POINT('Ctrl Pts',(39.,31.080768958446,-91.9958480337503));
#168396=CARTESIAN_POINT('',(39.,31.080768958446,-61.14995));
#168397=CARTESIAN_POINT('',(39.,31.080768958446,-129.34995));
#168398=CARTESIAN_POINT('Origin',(40.,31.080768958446,-61.14995));
#168399=CARTESIAN_POINT('Ctrl Pts',(29.,30.0207919771236,-76.4370443259982));
#168400=CARTESIAN_POINT('Ctrl Pts',(29.,29.2642096076976,-76.0137531166873));
#168401=CARTESIAN_POINT('Ctrl Pts',(28.2496025504691,29.6431021990262,-76.2257351951278));
#168402=CARTESIAN_POINT('Ctrl Pts',(29.,32.8015320477175,-71.4668042994815));
#168403=CARTESIAN_POINT('Ctrl Pts',(29.,32.0024463153694,-71.1716406391234));
#168404=CARTESIAN_POINT('Ctrl Pts',(28.2608542879989,32.4163856120597,-71.2554899486297));
#168405=CARTESIAN_POINT('Ctrl Pts',(29.,35.5206920342409,-66.4628921538691));
#168406=CARTESIAN_POINT('Ctrl Pts',(28.9999999999899,34.7556963975018,-66.1533445021367));
#168407=CARTESIAN_POINT('Ctrl Pts',(28.2706820191605,35.1297158291743,-66.2515800426151));
#168408=CARTESIAN_POINT('Ctrl Pts',(29.,38.2024209812184,-61.4386408691297));
#168409=CARTESIAN_POINT('Ctrl Pts',(29.,37.4942143736512,-61.0606306836509));
#168410=CARTESIAN_POINT('Ctrl Pts',(28.2795019009908,37.8065307949999,-61.2273317382593));
#168411=CARTESIAN_POINT('',(28.2795019009908,37.8065307949999,-61.2273317382593));
#168412=CARTESIAN_POINT('',(29.,38.2024209812184,-61.4386408691297));
#168413=CARTESIAN_POINT('Origin',(28.5,38.2024209812184,-61.4386408691297));
#168414=CARTESIAN_POINT('',(29.,30.0207919771236,-76.4370443259982));
#168415=CARTESIAN_POINT('Ctrl Pts',(29.,30.0207919771236,-76.4370443259982));
#168416=CARTESIAN_POINT('Ctrl Pts',(29.,32.8015436034469,-71.4667836449984));
#168417=CARTESIAN_POINT('Ctrl Pts',(29.,35.5206811754595,-66.4629124977081));
#168418=CARTESIAN_POINT('Ctrl Pts',(29.,38.2024209812184,-61.4386408691297));
#168419=CARTESIAN_POINT('Origin',(28.5,30.0207919771236,-76.4370443259982));
#168420=CARTESIAN_POINT('Ctrl Pts',(28.2795019009908,37.8065307949999,-61.2273317382593));
#168421=CARTESIAN_POINT('Ctrl Pts',(28.277453635604,37.1848867012263,-62.3941267255567));
#168422=CARTESIAN_POINT('Ctrl Pts',(28.275381852787,36.5706479594793,-63.5422196084077));
#168423=CARTESIAN_POINT('Ctrl Pts',(28.2732866240955,35.9637160883466,-64.6715679822654));
#168424=CARTESIAN_POINT('Ctrl Pts',(28.2711270058156,35.3381322707528,-65.8356229622629));
#168425=CARTESIAN_POINT('Ctrl Pts',(28.2689424796447,34.7203113773663,-66.9797636636303));
#168426=CARTESIAN_POINT('Ctrl Pts',(28.2667339239111,34.1101940280727,-68.1039712769445));
#168427=CARTESIAN_POINT('Ctrl Pts',(28.2644834413072,33.4884943082005,-69.2495206685244));
#168428=CARTESIAN_POINT('Ctrl Pts',(28.2622080112682,32.8747935600169,-70.3743730692533));
#168429=CARTESIAN_POINT('Ctrl Pts',(28.2599093458026,32.2690767258885,-71.4785358153589));
#168430=CARTESIAN_POINT('Ctrl Pts',(28.257539766533,31.6446735341878,-72.616761969858));
#168431=CARTESIAN_POINT('Ctrl Pts',(28.2551454983198,31.0287545675081,-73.7330022870964));
#168432=CARTESIAN_POINT('Ctrl Pts',(28.2527292012792,30.4213516569412,-74.827292366658));
#168433=CARTESIAN_POINT('Ctrl Pts',(28.2516909581113,30.1603605985564,-75.2974908478906));
#168434=CARTESIAN_POINT('Ctrl Pts',(28.2506486572428,29.900942426465,-75.76363703424));
#168435=CARTESIAN_POINT('Ctrl Pts',(28.2496025504691,29.6431021990262,-76.2257351951278));
#168436=CARTESIAN_POINT('Ctrl Pts',(28.2496025504691,29.6431021990262,-76.2257351951279));
#168437=CARTESIAN_POINT('Ctrl Pts',(29.,29.2642096076976,-76.0137531166872));
#168438=CARTESIAN_POINT('Ctrl Pts',(29.,30.0207919771236,-76.4370443259982));
#168439=CARTESIAN_POINT('Ctrl Pts',(28.2688173873502,29.4296103781281,-76.5845570406398));
#168440=CARTESIAN_POINT('Ctrl Pts',(29.,29.0941349251779,-76.4054204039549));
#168441=CARTESIAN_POINT('Ctrl Pts',(29.,29.8286446521612,-76.7804846793283));
#168442=CARTESIAN_POINT('Ctrl Pts',(28.2886273449575,29.2500516159651,-76.9550303093546));
#168443=CARTESIAN_POINT('Ctrl Pts',(29.,28.9500939111529,-76.8125874626777));
#168444=CARTESIAN_POINT('Ctrl Pts',(29.,29.6670464531659,-77.134908720041));
#168445=CARTESIAN_POINT('Ctrl Pts',(28.3291630969748,28.9452627171061,-77.7145350708491));
#168446=CARTESIAN_POINT('Ctrl Pts',(29.,28.7180119748831,-77.6282159000457));
#168447=CARTESIAN_POINT('Ctrl Pts',(29.,29.392736442598,-77.861168463682));
#168448=CARTESIAN_POINT('Ctrl Pts',(28.3498943566417,28.8202033592585,-78.1036672968219));
#168449=CARTESIAN_POINT('Ctrl Pts',(29.,28.6262186304227,-78.0380158313972));
#168450=CARTESIAN_POINT('Ctrl Pts',(29.,29.2801830215621,-78.2330925203216));
#168451=CARTESIAN_POINT('Ctrl Pts',(28.3921729695334,28.6196836802033,-78.89905271603));
#168452=CARTESIAN_POINT('Ctrl Pts',(29.,28.4907909944947,-78.8635806040775));
#168453=CARTESIAN_POINT('Ctrl Pts',(29.,29.0997153099535,-78.9928975231766));
#168454=CARTESIAN_POINT('Ctrl Pts',(28.4137198127509,28.544609722815,-79.3053090810168));
#168455=CARTESIAN_POINT('Ctrl Pts',(29.,28.4446634876444,-79.2803896999264));
#168456=CARTESIAN_POINT('Ctrl Pts',(29.,29.0321487487139,-79.3807788748604));
#168457=CARTESIAN_POINT('Ctrl Pts',(28.4567512459693,28.4450459981447,-80.1187974753391));
#168458=CARTESIAN_POINT('Ctrl Pts',(29.,28.3995314322135,-80.1063804977281));
#168459=CARTESIAN_POINT('Ctrl Pts',(29.,28.9425413961498,-80.1570353641513));
#168460=CARTESIAN_POINT('Ctrl Pts',(28.4783422408471,28.41999998,-80.5280280808492));
#168461=CARTESIAN_POINT('Ctrl Pts',(29.,28.3978619671205,-80.5188978169702));
#168462=CARTESIAN_POINT('Ctrl Pts',(29.,28.9199999806373,-80.547320361459));
#168463=CARTESIAN_POINT('Ctrl Pts',(28.5,28.41999998,-80.9397703408579));
#168464=CARTESIAN_POINT('Ctrl Pts',(29.,28.41999998,-80.9397703408578));
#168465=CARTESIAN_POINT('Ctrl Pts',(29.,28.91999998,-80.9397703408579));
#168466=CARTESIAN_POINT('',(29.,28.91999998,-80.9397703408579));
#168467=CARTESIAN_POINT('Ctrl Pts',(29.,28.91999998,-80.9397703408579));
#168468=CARTESIAN_POINT('Ctrl Pts',(29.,28.9199999800001,-80.5473141158908));
#168469=CARTESIAN_POINT('Ctrl Pts',(29.,28.9425413961516,-80.1570353641503));
#168470=CARTESIAN_POINT('Ctrl Pts',(29.,28.98734507234,-79.7689071194953));
#168471=CARTESIAN_POINT('Ctrl Pts',(29.,29.0321487485283,-79.3807788748402));
#168472=CARTESIAN_POINT('Ctrl Pts',(29.,29.0997153099481,-78.9928975232084));
#168473=CARTESIAN_POINT('Ctrl Pts',(29.,29.1899491656343,-78.6129950217198));
#168474=CARTESIAN_POINT('Ctrl Pts',(29.,29.2801830213205,-78.2330925202312));
#168475=CARTESIAN_POINT('Ctrl Pts',(29.,29.3927364426023,-77.8611684636915));
#168476=CARTESIAN_POINT('Ctrl Pts',(29.,29.5298914474149,-77.498038591685));
#168477=CARTESIAN_POINT('Ctrl Pts',(29.,29.6670464522275,-77.1349087196785));
#168478=CARTESIAN_POINT('Ctrl Pts',(29.,29.8286298518252,-76.7805111234986));
#168479=CARTESIAN_POINT('Ctrl Pts',(29.,30.0207919771236,-76.4370443259982));
#168480=CARTESIAN_POINT('Origin',(28.5,28.91999998,-80.9397703408579));
#168481=CARTESIAN_POINT('Origin',(28.5,28.91999998,-55.24995));
#168482=CARTESIAN_POINT('',(29.,28.91999998,-91.34995));
#168483=CARTESIAN_POINT('',(29.,28.91999998,-80.3749072158811));
#168484=CARTESIAN_POINT('',(28.5,28.41999998,-91.34995));
#168485=CARTESIAN_POINT('Origin',(28.5,28.91999998,-91.34995));
#168486=CARTESIAN_POINT('',(28.5,28.41999998,-91.34995));
#168487=CARTESIAN_POINT('Origin',(29.5,43.91999998,-58.24995));
#168488=CARTESIAN_POINT('',(29.5,46.91999998,-58.24995));
#168489=CARTESIAN_POINT('',(29.,46.41999998,-58.24995));
#168490=CARTESIAN_POINT('Origin',(29.5,46.41999998,-58.24995));
#168491=CARTESIAN_POINT('',(29.,43.91999998,-55.74995));
#168492=CARTESIAN_POINT('Origin',(29.,43.91999998,-58.24995));
#168493=CARTESIAN_POINT('',(29.5,43.91999998,-55.24995));
#168494=CARTESIAN_POINT('Origin',(29.5,43.91999998,-55.74995));
#168495=CARTESIAN_POINT('Origin',(29.5,43.91999998,-58.24995));
#168496=CARTESIAN_POINT('Origin',(0.,43.91999998,-58.24995));
#168497=CARTESIAN_POINT('',(30.,46.91999998,-58.24995));
#168498=CARTESIAN_POINT('',(-39.,46.91999998,-58.24995));
#168499=CARTESIAN_POINT('',(30.,43.91999998,-55.24995));
#168500=CARTESIAN_POINT('',(0.,43.91999998,-55.24995));
#168501=CARTESIAN_POINT('Origin',(30.,43.91999998,-58.24995));
#168502=CARTESIAN_POINT('Origin',(30.,43.91999998,-58.24995));
#168503=CARTESIAN_POINT('',(30.5,43.91999998,-55.74995));
#168504=CARTESIAN_POINT('Origin',(30.,43.91999998,-55.74995));
#168505=CARTESIAN_POINT('',(30.5,46.41999998,-58.24995));
#168506=CARTESIAN_POINT('Origin',(30.5,43.91999998,-58.24995));
#168507=CARTESIAN_POINT('Origin',(30.,46.41999998,-58.24995));
#168508=CARTESIAN_POINT('Origin',(31.,28.91999998,-55.24995));
#168509=CARTESIAN_POINT('',(30.5,28.91999998,-78.0460091084363));
#168510=CARTESIAN_POINT('Origin',(31.,28.91999998,-78.0460091084363));
#168511=CARTESIAN_POINT('',(31.,28.41999998,-91.34995));
#168512=CARTESIAN_POINT('',(31.,28.41999998,-78.6384479219785));
#168513=CARTESIAN_POINT('',(30.5,28.91999998,-91.34995));
#168514=CARTESIAN_POINT('Origin',(31.,28.91999998,-91.34995));
#168515=CARTESIAN_POINT('',(30.5,28.91999998,-91.34995));
#168516=CARTESIAN_POINT('Ctrl Pts',(31.,28.41999998,-78.0460091084363));
#168517=CARTESIAN_POINT('Ctrl Pts',(30.5,28.4199999800001,-78.0460091084362));
#168518=CARTESIAN_POINT('Ctrl Pts',(30.5,28.91999998,-78.0460091084363));
#168519=CARTESIAN_POINT('Ctrl Pts',(30.9540427885061,28.41999998,-77.1674732790134));
#168520=CARTESIAN_POINT('Ctrl Pts',(30.4999999999986,28.4639319715929,-77.2061881935471));
#168521=CARTESIAN_POINT('Ctrl Pts',(30.5,28.9199999815576,-77.20604216556));
#168522=CARTESIAN_POINT('Ctrl Pts',(30.9086864990993,28.524456817556,-76.3042505917732));
#168523=CARTESIAN_POINT('Ctrl Pts',(30.5,28.594723031989,-76.3445661605256));
#168524=CARTESIAN_POINT('Ctrl Pts',(30.5,29.0140111325264,-76.3798194513939));
#168525=CARTESIAN_POINT('Ctrl Pts',(30.8417479231147,28.8453484758852,-75.0340652196707));
#168526=CARTESIAN_POINT('Ctrl Pts',(30.5,28.9540243183721,-75.0718611408805));
#168527=CARTESIAN_POINT('Ctrl Pts',(30.5,29.3028136269337,-75.1629449138939));
#168528=CARTESIAN_POINT('Ctrl Pts',(30.8195011122979,28.9813539161962,-74.6125811736547));
#168529=CARTESIAN_POINT('Ctrl Pts',(30.5,29.0970986774549,-74.6573700140041));
#168530=CARTESIAN_POINT('Ctrl Pts',(30.5,29.4252185218281,-74.758955076818));
#168531=CARTESIAN_POINT('Ctrl Pts',(30.7763886958648,29.3132233924744,-73.7967725466866));
#168532=CARTESIAN_POINT('Ctrl Pts',(30.5,29.4381839095486,-73.8581557735759));
#168533=CARTESIAN_POINT('Ctrl Pts',(30.5,29.7239010519754,-73.9766691906993));
#168534=CARTESIAN_POINT('Ctrl Pts',(30.7554505056092,29.508874874601,-73.4010655029222));
#168535=CARTESIAN_POINT('Ctrl Pts',(30.5,29.6348298970151,-73.4702277561984));
#168536=CARTESIAN_POINT('Ctrl Pts',(30.5,29.8999811721136,-73.5970610003643));
#168537=CARTESIAN_POINT('Ctrl Pts',(30.7353076117354,29.7418701453453,-73.0207363867646));
#168538=CARTESIAN_POINT('Ctrl Pts',(30.5,29.8691857803932,-73.0938794170476));
#168539=CARTESIAN_POINT('Ctrl Pts',(30.5,30.1096831288108,-73.2320455176344));
#168540=CARTESIAN_POINT('',(30.5,30.1096831288108,-73.2320455176344));
#168541=CARTESIAN_POINT('Origin',(31.,30.1096831288108,-73.2320455176344));
#168542=CARTESIAN_POINT('Ctrl Pts',(30.5,30.1096831288108,-73.2320455176344));
#168543=CARTESIAN_POINT('Ctrl Pts',(30.5,29.8999686314803,-73.5970828192481));
#168544=CARTESIAN_POINT('Ctrl Pts',(30.5,29.7239010511178,-73.976669190304));
#168545=CARTESIAN_POINT('Ctrl Pts',(30.5,29.5745597864535,-74.3678121335876));
#168546=CARTESIAN_POINT('Ctrl Pts',(30.5,29.4252185217892,-74.7589550768712));
#168547=CARTESIAN_POINT('Ctrl Pts',(30.5,29.3028136262495,-75.1629449137757));
#168548=CARTESIAN_POINT('Ctrl Pts',(30.5,29.2065461283391,-75.5685697596184));
#168549=CARTESIAN_POINT('Ctrl Pts',(30.5,29.0974180990883,-76.0283826871664));
#168550=CARTESIAN_POINT('Ctrl Pts',(30.5,29.0199506911356,-76.492948109106));
#168551=CARTESIAN_POINT('Ctrl Pts',(30.5,28.9733024240056,-76.9621397516276));
#168552=CARTESIAN_POINT('Ctrl Pts',(30.5,28.9376489765477,-77.3207447031834));
#168553=CARTESIAN_POINT('Ctrl Pts',(30.5,28.91999998,-77.6820522875113));
#168554=CARTESIAN_POINT('Ctrl Pts',(30.5,28.91999998,-78.0460091084363));
#168555=CARTESIAN_POINT('Ctrl Pts',(30.5,36.7276789742547,-61.4386408691296));
#168556=CARTESIAN_POINT('Ctrl Pts',(30.5,36.4678387256643,-61.2958335593366));
#168557=CARTESIAN_POINT('Ctrl Pts',(30.7601599624812,36.3431985357226,-61.2273317382593));
#168558=CARTESIAN_POINT('Ctrl Pts',(30.5,34.5564303542403,-65.3892634389964));
#168559=CARTESIAN_POINT('Ctrl Pts',(30.5,34.3134045700868,-65.2278638132481));
#168560=CARTESIAN_POINT('Ctrl Pts',(30.7526164452201,34.1766563796975,-65.1779528603621));
#168561=CARTESIAN_POINT('Ctrl Pts',(30.5,32.3553350664733,-69.3231754387568));
#168562=CARTESIAN_POINT('Ctrl Pts',(30.5,32.1210861733241,-69.1599841087648));
#168563=CARTESIAN_POINT('Ctrl Pts',(30.7443983582191,31.9809814038522,-69.1118639196982));
#168564=CARTESIAN_POINT('Ctrl Pts',(30.5,30.1096831288108,-73.2320455176344));
#168565=CARTESIAN_POINT('Ctrl Pts',(30.5,29.8691857803939,-73.0938794170475));
#168566=CARTESIAN_POINT('Ctrl Pts',(30.7353076117347,29.741870145346,-73.0207363867641));
#168567=CARTESIAN_POINT('',(30.5,36.7276789742547,-61.4386408691296));
#168568=CARTESIAN_POINT('Origin',(31.,36.7276789742547,-61.4386408691296));
#168569=CARTESIAN_POINT('Ctrl Pts',(30.5,36.7276789742547,-61.4386408691296));
#168570=CARTESIAN_POINT('Ctrl Pts',(30.5,34.5564250420216,-65.3892731044285));
#168571=CARTESIAN_POINT('Ctrl Pts',(30.5,32.355340677558,-69.3231656718822));
#168572=CARTESIAN_POINT('Ctrl Pts',(30.5,30.1096831288108,-73.2320455176344));
#168573=CARTESIAN_POINT('Ctrl Pts',(30.7601599624812,36.3431985357226,-61.2273317382593));
#168574=CARTESIAN_POINT('Ctrl Pts',(30.5,36.4678387256643,-61.2958335593366));
#168575=CARTESIAN_POINT('Ctrl Pts',(30.5,36.7276789742547,-61.4386408691297));
#168576=CARTESIAN_POINT('Ctrl Pts',(30.7833440352389,36.4311997587239,-61.0408976853214));
#168577=CARTESIAN_POINT('Ctrl Pts',(30.5,36.536757012545,-61.1328271281761));
#168578=CARTESIAN_POINT('Ctrl Pts',(30.5,36.7789093803379,-61.3454266101228));
#168579=CARTESIAN_POINT('Ctrl Pts',(30.820204224048,36.5713423922847,-60.8940610213177));
#168580=CARTESIAN_POINT('Ctrl Pts',(30.5000000000002,36.6495790716841,-60.9942767827739));
#168581=CARTESIAN_POINT('Ctrl Pts',(30.5,36.8604662025248,-61.2720055170969));
#168582=CARTESIAN_POINT('Ctrl Pts',(30.9048607560821,36.8949030802612,-60.6989334962026));
#168583=CARTESIAN_POINT('Ctrl Pts',(30.4999999999998,36.921160791843,-60.7754981362285));
#168584=CARTESIAN_POINT('Ctrl Pts',(30.5,37.0485310665384,-61.1744417416632));
#168585=CARTESIAN_POINT('Ctrl Pts',(30.9524183405754,37.0774198714491,-60.64995));
#168586=CARTESIAN_POINT('Ctrl Pts',(30.5,37.0857740751484,-60.6953661941756));
#168587=CARTESIAN_POINT('Ctrl Pts',(30.5,37.1545174137893,-61.1499500119967));
#168588=CARTESIAN_POINT('Ctrl Pts',(31.,37.2609769076718,-60.64995));
#168589=CARTESIAN_POINT('Ctrl Pts',(30.5,37.2609769076718,-60.64995));
#168590=CARTESIAN_POINT('Ctrl Pts',(30.5,37.2609769076718,-61.14995));
#168591=CARTESIAN_POINT('',(30.5,37.2609769076718,-61.14995));
#168592=CARTESIAN_POINT('',(31.,37.2609769076718,-60.64995));
#168593=CARTESIAN_POINT('Origin',(31.,37.2609769076718,-61.14995));
#168594=CARTESIAN_POINT('Ctrl Pts',(30.7601599624812,36.3431985357226,-61.2273317382593));
#168595=CARTESIAN_POINT('Ctrl Pts',(30.763965363455,36.3576429322361,-61.1967307159962));
#168596=CARTESIAN_POINT('Ctrl Pts',(30.7682373320678,36.3739555244459,-61.1662491652629));
#168597=CARTESIAN_POINT('Ctrl Pts',(30.773014719755,36.3922097826873,-61.1361721037419));
#168598=CARTESIAN_POINT('Ctrl Pts',(30.7743832716099,36.3974389791877,-61.1275560941091));
#168599=CARTESIAN_POINT('Ctrl Pts',(30.7757932280396,36.4028272069756,-61.1189733621298));
#168600=CARTESIAN_POINT('Ctrl Pts',(30.7772453313422,36.4083754424347,-61.1104308162074));
#168601=CARTESIAN_POINT('Ctrl Pts',(30.7822566925532,36.4275229864965,-61.0809495918337));
#168602=CARTESIAN_POINT('Ctrl Pts',(30.7877692333939,36.4485775577365,-61.0519471656573));
#168603=CARTESIAN_POINT('Ctrl Pts',(30.7938075568224,36.4715887509763,-61.0236793562699));
#168604=CARTESIAN_POINT('Ctrl Pts',(30.7956267481173,36.4785214307048,-61.0151629935126));
#168605=CARTESIAN_POINT('Ctrl Pts',(30.7974936059083,36.4856314523552,-61.0067135459256));
#168606=CARTESIAN_POINT('Ctrl Pts',(30.7994086489996,36.4929194816368,-60.9983386454677));
#168607=CARTESIAN_POINT('Ctrl Pts',(30.8053381175456,36.5154851046153,-60.9724077883165));
#168608=CARTESIAN_POINT('Ctrl Pts',(30.8117244764344,36.5397508645177,-60.9472021615385));
#168609=CARTESIAN_POINT('Ctrl Pts',(30.8185588211127,36.5657140442116,-60.9229694331518));
#168610=CARTESIAN_POINT('Ctrl Pts',(30.8212582864498,36.5759691172173,-60.9133978628872));
#168611=CARTESIAN_POINT('Ctrl Pts',(30.8240275191732,36.5864885832815,-60.9039784112583));
#168612=CARTESIAN_POINT('Ctrl Pts',(30.8268654522856,36.5972705027269,-60.8947276746678));
#168613=CARTESIAN_POINT('Ctrl Pts',(30.8318768733917,36.6163099714291,-60.8783920759203));
#168614=CARTESIAN_POINT('Ctrl Pts',(30.8371024716969,36.6361694013684,-60.8625813969166));
#168615=CARTESIAN_POINT('Ctrl Pts',(30.8425326224079,36.6568361342905,-60.8473901690906));
#168616=CARTESIAN_POINT('Ctrl Pts',(30.8452476977634,36.6671695007516,-60.8397945551776));
#168617=CARTESIAN_POINT('Ctrl Pts',(30.8480139129425,36.6777046960906,-60.8323538223576));
#168618=CARTESIAN_POINT('Ctrl Pts',(30.8508295920009,36.6884393999272,-60.8250806072626));
#168619=CARTESIAN_POINT('Ctrl Pts',(30.8522374315301,36.6938067518455,-60.8214439997151));
#168620=CARTESIAN_POINT('Ctrl Pts',(30.8536576365094,36.6992239800803,-60.8178492742012));
#168621=CARTESIAN_POINT('Ctrl Pts',(30.8550899796344,36.7046907663651,-60.814298049174));
#168622=CARTESIAN_POINT('Ctrl Pts',(30.8560154879301,36.7082231295039,-60.8120034256547));
#168623=CARTESIAN_POINT('Ctrl Pts',(30.8570682094331,36.7122433277919,-60.8094291323204));
#168624=CARTESIAN_POINT('Ctrl Pts',(30.8580115255638,36.7158468637295,-60.8071553682941));
#168625=CARTESIAN_POINT('Ctrl Pts',(30.8585281124733,36.7178202631368,-60.8059101900415));
#168626=CARTESIAN_POINT('Ctrl Pts',(30.8590117680525,36.7196682301612,-60.8047541406749));
#168627=CARTESIAN_POINT('Ctrl Pts',(30.8594229432602,36.7212394976976,-60.8037765840641));
#168628=CARTESIAN_POINT('Ctrl Pts',(30.8604475203524,36.7251548230705,-60.8013406830395));
#168629=CARTESIAN_POINT('Ctrl Pts',(30.8614836657748,36.7291158819178,-60.7989137988806));
#168630=CARTESIAN_POINT('Ctrl Pts',(30.8625314764417,36.7331228697491,-60.7964975160502));
#168631=CARTESIAN_POINT('Ctrl Pts',(30.8690570966094,36.7580778367397,-60.7814492401846));
#168632=CARTESIAN_POINT('Ctrl Pts',(30.8760300291748,36.784795266773,-60.7667926107252));
#168633=CARTESIAN_POINT('Ctrl Pts',(30.8834787244378,36.8133365487953,-60.7528950405293));
#168634=CARTESIAN_POINT('Ctrl Pts',(30.8856856098912,36.8217927062689,-60.7487774945135));
#168635=CARTESIAN_POINT('Ctrl Pts',(30.8879342100648,36.8304087431804,-60.7447268360333));
#168636=CARTESIAN_POINT('Ctrl Pts',(30.8902251321549,36.8391856521961,-60.7407532768451));
#168637=CARTESIAN_POINT('Ctrl Pts',(30.8958575471384,36.8607643842102,-60.730983964128));
#168638=CARTESIAN_POINT('Ctrl Pts',(30.9017446838295,36.8833145238806,-60.7216812541265));
#168639=CARTESIAN_POINT('Ctrl Pts',(30.9078839561844,36.9068356960058,-60.7130073200878));
#168640=CARTESIAN_POINT('Ctrl Pts',(30.9109535923618,36.9185962820684,-60.7086703530685));
#168641=CARTESIAN_POINT('Ctrl Pts',(30.9140861029083,36.9305993739776,-60.7044907499071));
#168642=CARTESIAN_POINT('Ctrl Pts',(30.9172801297012,36.9428432830316,-60.7004897073433));
#168643=CARTESIAN_POINT('Ctrl Pts',(30.9188771430977,36.9489652375587,-60.6984891860615));
#168644=CARTESIAN_POINT('Ctrl Pts',(30.9204895355962,36.9551473964347,-60.6965333068457));
#168645=CARTESIAN_POINT('Ctrl Pts',(30.9221170541162,36.9613894159181,-60.6946247772135));
#168646=CARTESIAN_POINT('Ctrl Pts',(30.9229308133762,36.9645104256597,-60.6936705123975));
#168647=CARTESIAN_POINT('Ctrl Pts',(30.9237483541366,36.967646400545,-60.6927280849868));
#168648=CARTESIAN_POINT('Ctrl Pts',(30.9245696419522,36.9707972931077,-60.6917978351345));
#168649=CARTESIAN_POINT('Ctrl Pts',(30.9251964133939,36.9732019184251,-60.6910879085654));
#168650=CARTESIAN_POINT('Ctrl Pts',(30.9260411033132,36.9764431639241,-60.6901460669173));
#168651=CARTESIAN_POINT('Ctrl Pts',(30.9266098300196,36.9786257121803,-60.6895206596725));
#168652=CARTESIAN_POINT('Ctrl Pts',(30.9267863324083,36.9793030585691,-60.6893265666725));
#168653=CARTESIAN_POINT('Ctrl Pts',(30.9269362296689,36.9798783303591,-60.6891624942613));
#168654=CARTESIAN_POINT('Ctrl Pts',(30.9270447106142,36.9802946739586,-60.6890439593315));
#168655=CARTESIAN_POINT('Ctrl Pts',(30.9302404200775,36.9925596222182,-60.6855520723829));
#168656=CARTESIAN_POINT('Ctrl Pts',(30.9338876720354,37.0065603067294,-60.6818105517145));
#168657=CARTESIAN_POINT('Ctrl Pts',(30.9379937153134,37.0223289997633,-60.6780391759794));
#168658=CARTESIAN_POINT('Ctrl Pts',(30.9420570063409,37.0379335086743,-60.6743070679258));
#168659=CARTESIAN_POINT('Ctrl Pts',(30.9465697396705,37.0552699885961,-60.6705458315636));
#168660=CARTESIAN_POINT('Ctrl Pts',(30.9515368184822,37.0743626826108,-60.6670184499722));
#168661=CARTESIAN_POINT('Ctrl Pts',(30.9564323410571,37.0931803253556,-60.6635418841948));
#168662=CARTESIAN_POINT('Ctrl Pts',(30.961769379885,37.1137045804594,-60.6602926154819));
#168663=CARTESIAN_POINT('Ctrl Pts',(30.9675481761194,37.135942761274,-60.6575694262484));
#168664=CARTESIAN_POINT('Ctrl Pts',(30.9731323446384,37.1574319684012,-60.654937953019));
#168665=CARTESIAN_POINT('Ctrl Pts',(30.9791291569654,37.1805221375206,-60.6527979719705));
#168666=CARTESIAN_POINT('Ctrl Pts',(30.9855324226127,37.2051964674286,-60.6514602685091));
#168667=CARTESIAN_POINT('Ctrl Pts',(30.9901458013928,37.2229736511785,-60.6504964895403));
#168668=CARTESIAN_POINT('Ctrl Pts',(30.9949700422445,37.2415727055254,-60.64995));
#168669=CARTESIAN_POINT('Ctrl Pts',(31.,37.2609769076718,-60.64995));
#168670=CARTESIAN_POINT('Ctrl Pts',(30.5,37.2609769076718,-61.14995));
#168671=CARTESIAN_POINT('Ctrl Pts',(30.5,37.2057964810293,-61.14995));
#168672=CARTESIAN_POINT('Ctrl Pts',(30.5,37.1508139868675,-61.156525590466));
#168673=CARTESIAN_POINT('Ctrl Pts',(30.5,37.0975659565498,-61.1696247206416));
#168674=CARTESIAN_POINT('Ctrl Pts',(30.5,37.0479567714747,-61.1818286870481));
#168675=CARTESIAN_POINT('Ctrl Pts',(30.5,36.9998515275001,-61.1996955772651));
#168676=CARTESIAN_POINT('Ctrl Pts',(30.5,36.9544986327132,-61.223223625875));
#168677=CARTESIAN_POINT('Ctrl Pts',(30.5,36.9220640062062,-61.2400499711984));
#168678=CARTESIAN_POINT('Ctrl Pts',(30.5,36.8911731746046,-61.2597722334506));
#168679=CARTESIAN_POINT('Ctrl Pts',(30.5,36.8624864317525,-61.2822151380553));
#168680=CARTESIAN_POINT('Ctrl Pts',(30.5,36.8352464003273,-61.3035262164813));
#168681=CARTESIAN_POINT('Ctrl Pts',(30.5,36.8099924249355,-61.3272911886641));
#168682=CARTESIAN_POINT('Ctrl Pts',(30.5,36.7873187400317,-61.3533954059166));
#168683=CARTESIAN_POINT('Ctrl Pts',(30.5,36.7660341218412,-61.377900390428));
#168684=CARTESIAN_POINT('Ctrl Pts',(30.5,36.7470225594145,-61.4044673363617));
#168685=CARTESIAN_POINT('Ctrl Pts',(30.5,36.7308159346661,-61.4330244036173));
#168686=CARTESIAN_POINT('Ctrl Pts',(30.5,36.7297582655658,-61.4348880814713));
#168687=CARTESIAN_POINT('Ctrl Pts',(30.5,36.7287125602851,-61.4367602423503));
#168688=CARTESIAN_POINT('Ctrl Pts',(30.5,36.7276789742547,-61.4386408691296));
#168689=CARTESIAN_POINT('Origin',(37.,-12.9675000200281,-61.14995));
#168690=CARTESIAN_POINT('',(37.,37.923330431502,-60.64995));
#168691=CARTESIAN_POINT('',(37.5,37.923330431502,-61.14995));
#168692=CARTESIAN_POINT('Origin',(37.,37.923330431502,-61.14995));
#168693=CARTESIAN_POINT('',(37.5,-9.33460238845303,-61.14995));
#168694=CARTESIAN_POINT('',(37.,-12.9675000200281,-60.64995));
#168695=CARTESIAN_POINT('Origin',(31.,-9.33460238845303,-61.14995));
#168696=CARTESIAN_POINT('',(30.5,38.4482624126576,-61.14995));
#168697=CARTESIAN_POINT('',(31.,38.4482624126576,-60.64995));
#168698=CARTESIAN_POINT('Origin',(31.,38.4482624126576,-61.14995));
#168699=CARTESIAN_POINT('',(31.,-12.9675000200281,-60.64995));
#168700=CARTESIAN_POINT('',(30.5,-9.33460238845303,-61.14995));
#168701=CARTESIAN_POINT('Origin',(0.,-12.9675000200281,-61.64995));
#168702=CARTESIAN_POINT('Origin',(0.,-12.9675000200281,-60.64995));
#168703=CARTESIAN_POINT('Origin',(32.85,-70.08000002,-174.34995));
#168704=CARTESIAN_POINT('',(33.35,-70.08000002,-176.84995));
#168705=CARTESIAN_POINT('Origin',(32.85,-70.08000002,-176.84995));
#168706=CARTESIAN_POINT('',(33.35,-72.58000002,-174.34995));
#168707=CARTESIAN_POINT('Origin',(33.35,-70.08000002,-174.34995));
#168708=CARTESIAN_POINT('Origin',(32.85,-72.58000002,-174.34995));
#168709=CARTESIAN_POINT('Origin',(32.85,-72.58000002,-55.24995));
#168710=CARTESIAN_POINT('',(33.35,-72.58000002,-58.24995));
#168711=CARTESIAN_POINT('',(33.35,-72.58000002,-174.34995));
#168712=CARTESIAN_POINT('Origin',(32.85,-72.58000002,-58.24995));
#168713=CARTESIAN_POINT('Ctrl Pts',(33.8806075480013,-61.4290931059938,
-60.6557206474106));
#168714=CARTESIAN_POINT('Ctrl Pts',(33.3500000000017,-61.4317841533,-60.6232112509527));
#168715=CARTESIAN_POINT('Ctrl Pts',(33.35,-61.3857298748211,-61.15282619958));
#168716=CARTESIAN_POINT('Ctrl Pts',(33.8204813483267,-61.214817269187,-60.6326735238177));
#168717=CARTESIAN_POINT('Ctrl Pts',(33.3499999999973,-61.2202673099084,
-60.6650058644588));
#168718=CARTESIAN_POINT('Ctrl Pts',(33.35,-61.2575945542474,-61.141321528844));
#168719=CARTESIAN_POINT('Ctrl Pts',(33.7566015486364,-60.9886558736888,
-60.6786599271601));
#168720=CARTESIAN_POINT('Ctrl Pts',(33.35,-61.0126032841866,-60.7560614808116));
#168721=CARTESIAN_POINT('Ctrl Pts',(33.35,-61.1220945388604,-61.1643294714043));
#168722=CARTESIAN_POINT('Ctrl Pts',(33.6462317574322,-60.5998176841187,
-60.9087900837106));
#168723=CARTESIAN_POINT('Ctrl Pts',(33.35,-60.6865246086057,-61.01647290262));
#168724=CARTESIAN_POINT('Ctrl Pts',(33.35,-60.8888304023229,-61.2794071648862));
#168725=CARTESIAN_POINT('Ctrl Pts',(33.5982385932668,-60.4318222621551,
-61.0947839923052));
#168726=CARTESIAN_POINT('Ctrl Pts',(33.3499999999994,-60.5516411453185,
-61.1871692827256));
#168727=CARTESIAN_POINT('Ctrl Pts',(33.35,-60.7878913738886,-61.3723612907971));
#168728=CARTESIAN_POINT('Ctrl Pts',(33.5744465072952,-60.3486837713638,
-61.3484667599621));
#168729=CARTESIAN_POINT('Ctrl Pts',(33.3500000000003,-60.4870054034178,
-61.4019031189409));
#168730=CARTESIAN_POINT('Ctrl Pts',(33.35,-60.7378676393038,-61.4992508410464));
#168731=CARTESIAN_POINT('',(33.35,-60.7669593817595,-61.4386408691297));
#168732=CARTESIAN_POINT('Origin',(33.85,-60.7669593817595,-61.4386408691297));
#168733=CARTESIAN_POINT('',(33.85,-61.3211699373828,-60.64995));
#168734=CARTESIAN_POINT('Ctrl Pts',(33.85,-61.3211699373828,-60.64995));
#168735=CARTESIAN_POINT('Ctrl Pts',(33.8408946232257,-61.2887822220266,
-60.64995));
#168736=CARTESIAN_POINT('Ctrl Pts',(33.8320360329935,-61.2574987712952,
-60.6514617262184));
#168737=CARTESIAN_POINT('Ctrl Pts',(33.8234947330584,-61.2274137239541,
-60.6541908134115));
#168738=CARTESIAN_POINT('Ctrl Pts',(33.8147158384926,-61.1964917963056,
-60.6569958160353));
#168739=CARTESIAN_POINT('Ctrl Pts',(33.8062719252371,-61.1668355547361,
-60.6610862959292));
#168740=CARTESIAN_POINT('Ctrl Pts',(33.7982087688177,-61.1385034904715,
-60.6661576313229));
#168741=CARTESIAN_POINT('Ctrl Pts',(33.7897805562155,-61.1088887033258,
-60.6714585693988));
#168742=CARTESIAN_POINT('Ctrl Pts',(33.7817681532881,-61.0807203975373,
-60.6778306117877));
#168743=CARTESIAN_POINT('Ctrl Pts',(33.7741937721167,-61.0540230202112,
-60.6849510110676));
#168744=CARTESIAN_POINT('Ctrl Pts',(33.7664268947605,-61.0266471527007,
-60.6922523689849));
#168745=CARTESIAN_POINT('Ctrl Pts',(33.7591202239172,-61.0008173969275,
-60.7003402004141));
#168746=CARTESIAN_POINT('Ctrl Pts',(33.7522713515567,-60.976523346829,-60.7088999701646));
#168747=CARTESIAN_POINT('Ctrl Pts',(33.7451537939754,-60.9512762271051,
-60.7177955446293));
#168748=CARTESIAN_POINT('Ctrl Pts',(33.7385302859764,-60.9276871255218,
-60.7272004222153));
#168749=CARTESIAN_POINT('Ctrl Pts',(33.7323756813871,-60.9057134546262,
-60.7368036104378));
#168750=CARTESIAN_POINT('Ctrl Pts',(33.7289765914216,-60.8935777466109,
-60.7421072981484));
#168751=CARTESIAN_POINT('Ctrl Pts',(33.7257201687046,-60.8819342854479,
-60.7474722461951));
#168752=CARTESIAN_POINT('Ctrl Pts',(33.7226000576368,-60.8707730258723,
-60.752851779779));
#168753=CARTESIAN_POINT('Ctrl Pts',(33.7176811117149,-60.8531769752573,
-60.7613327710671));
#168754=CARTESIAN_POINT('Ctrl Pts',(33.7131011490807,-60.836779646766,-60.7698488054675));
#168755=CARTESIAN_POINT('Ctrl Pts',(33.7088302172017,-60.8215350129312,
-60.77823724668));
#168756=CARTESIAN_POINT('Ctrl Pts',(33.7066947512622,-60.8139126960137,
-60.7824314672863));
#168757=CARTESIAN_POINT('Ctrl Pts',(33.7046364618188,-60.8065784470663,
-60.7865941739577));
#168758=CARTESIAN_POINT('Ctrl Pts',(33.7026512377244,-60.7995260481909,
-60.7907073021494));
#168759=CARTESIAN_POINT('Ctrl Pts',(33.7016586256772,-60.7959998487532,
-60.7927638662452));
#168760=CARTESIAN_POINT('Ctrl Pts',(33.700684285193,-60.7925441192497,-60.7948080508209));
#168761=CARTESIAN_POINT('Ctrl Pts',(33.6997276798046,-60.7891580545039,
-60.7968377444204));
#168762=CARTESIAN_POINT('Ctrl Pts',(33.6992493771104,-60.787465022131,-60.7978525912201));
#168763=CARTESIAN_POINT('Ctrl Pts',(33.6987755085231,-60.78578940642,-60.7988638162632));
#168764=CARTESIAN_POINT('Ctrl Pts',(33.6983060077729,-60.784131107961,-60.799871162729));
#168765=CARTESIAN_POINT('Ctrl Pts',(33.6979171366822,-60.7827575972046,
-60.8007055126608));
#168766=CARTESIAN_POINT('Ctrl Pts',(33.6977636893367,-60.7822136993763,
-60.8010361890538));
#168767=CARTESIAN_POINT('Ctrl Pts',(33.6972679602333,-60.780467262921,-60.802107581507));
#168768=CARTESIAN_POINT('Ctrl Pts',(33.6971651743236,-60.7801051517227,
-60.8023297271247));
#168769=CARTESIAN_POINT('Ctrl Pts',(33.697047717804,-60.7796914074066,-60.8025838438696));
#168770=CARTESIAN_POINT('Ctrl Pts',(33.6969105433143,-60.7792080657786,
-60.8028813142771));
#168771=CARTESIAN_POINT('Ctrl Pts',(33.687366364001,-60.7455786411208,-60.8235783907874));
#168772=CARTESIAN_POINT('Ctrl Pts',(33.6782837661359,-60.7137258174839,
-60.8458827892109));
#168773=CARTESIAN_POINT('Ctrl Pts',(33.6697182991571,-60.6837179852912,
-60.869478970828));
#168774=CARTESIAN_POINT('Ctrl Pts',(33.6610001352008,-60.653175202081,-60.89349580267));
#168775=CARTESIAN_POINT('Ctrl Pts',(33.6528175632848,-60.6245435544086,
-60.9188503903528));
#168776=CARTESIAN_POINT('Ctrl Pts',(33.6451985198799,-60.5978527728285,
-60.94522326713));
#168777=CARTESIAN_POINT('Ctrl Pts',(33.6373713547231,-60.5704329059907,
-60.9723165452788));
#168778=CARTESIAN_POINT('Ctrl Pts',(33.6301387768433,-60.5450611554622,
-61.0004840158148));
#168779=CARTESIAN_POINT('Ctrl Pts',(33.6235011899514,-60.5217288367252,
-61.0294008158947));
#168780=CARTESIAN_POINT('Ctrl Pts',(33.616755885099,-60.49801786987,-61.0587868917486));
#168781=CARTESIAN_POINT('Ctrl Pts',(33.6106247947373,-60.4764127066887,
-61.0889464349294));
#168782=CARTESIAN_POINT('Ctrl Pts',(33.6050809985361,-60.4568671948489,
-61.1195670593001));
#168783=CARTESIAN_POINT('Ctrl Pts',(33.5994074183963,-60.4368641096391,
-61.1509045327563));
#168784=CARTESIAN_POINT('Ctrl Pts',(33.5943486981784,-60.4190178726719,
-61.1827245851904));
#168785=CARTESIAN_POINT('Ctrl Pts',(33.5898513690894,-60.403246067445,-61.2147276758847));
#168786=CARTESIAN_POINT('Ctrl Pts',(33.5892613820072,-60.4011770257618,
-61.2189260366736));
#168787=CARTESIAN_POINT('Ctrl Pts',(33.5886810256773,-60.3991436438934,
-61.2231276001908));
#168788=CARTESIAN_POINT('Ctrl Pts',(33.5881101525802,-60.3971457002532,
-61.2273317382593));
#168789=CARTESIAN_POINT('',(33.35,-61.3211699373828,-61.14995));
#168790=CARTESIAN_POINT('Origin',(33.85,-61.3211699373828,-61.14995));
#168791=CARTESIAN_POINT('Ctrl Pts',(33.35,-60.7669593817595,-61.4386408691297));
#168792=CARTESIAN_POINT('Ctrl Pts',(33.35,-60.7854255655574,-61.4063230635264));
#168793=CARTESIAN_POINT('Ctrl Pts',(33.35,-60.8074669942766,-61.3766005831691));
#168794=CARTESIAN_POINT('Ctrl Pts',(33.35,-60.832315928212,-61.3495741724077));
#168795=CARTESIAN_POINT('Ctrl Pts',(33.35,-60.8598479301247,-61.3196295802289));
#168796=CARTESIAN_POINT('Ctrl Pts',(33.35,-60.8908254879517,-61.2929954345219));
#168797=CARTESIAN_POINT('Ctrl Pts',(33.35,-60.924148426403,-61.269769822738));
#168798=CARTESIAN_POINT('Ctrl Pts',(33.35,-60.9500168068532,-61.2517399313257));
#168799=CARTESIAN_POINT('Ctrl Pts',(33.35,-60.9772970763437,-61.2357633244769));
#168800=CARTESIAN_POINT('Ctrl Pts',(33.35,-61.0054624679791,-61.2218683128495));
#168801=CARTESIAN_POINT('Ctrl Pts',(33.35,-61.0316582964252,-61.2089449583455));
#168802=CARTESIAN_POINT('Ctrl Pts',(33.35,-61.0586931044519,-61.1978139207404));
#168803=CARTESIAN_POINT('Ctrl Pts',(33.35,-61.0863521110361,-61.1884108897488));
#168804=CARTESIAN_POINT('Ctrl Pts',(33.35,-61.1146264284014,-61.1787986760331));
#168805=CARTESIAN_POINT('Ctrl Pts',(33.35,-61.1435543947087,-61.1709920371076));
#168806=CARTESIAN_POINT('Ctrl Pts',(33.35,-61.1729286914007,-61.1649732421567));
#168807=CARTESIAN_POINT('Ctrl Pts',(33.35,-61.2017965294043,-61.1590582206179));
#168808=CARTESIAN_POINT('Ctrl Pts',(33.35,-61.2310968493209,-61.1548700235783));
#168809=CARTESIAN_POINT('Ctrl Pts',(33.35,-61.2606330881678,-61.1524405238988));
#168810=CARTESIAN_POINT('Ctrl Pts',(33.35,-61.2807251508687,-61.1507878537622));
#168811=CARTESIAN_POINT('Ctrl Pts',(33.35,-61.3009263849489,-61.14995));
#168812=CARTESIAN_POINT('Ctrl Pts',(33.35,-61.3211699373828,-61.14995));
#168813=CARTESIAN_POINT('Ctrl Pts',(33.35,-56.3642045114132,-69.0177323827589));
#168814=CARTESIAN_POINT('Ctrl Pts',(33.35,-56.134778922778,-68.8820528924306));
#168815=CARTESIAN_POINT('Ctrl Pts',(33.5712930253538,-56.006893899348,-68.8064232518886));
#168816=CARTESIAN_POINT('Ctrl Pts',(33.35,-57.8514943778664,-66.5028176210733));
#168817=CARTESIAN_POINT('Ctrl Pts',(33.35,-57.623019767821,-66.3564728841549));
#168818=CARTESIAN_POINT('Ctrl Pts',(33.5772316679252,-57.489551829777,-66.2915080112617));
#168819=CARTESIAN_POINT('Ctrl Pts',(33.35,-59.3174222737568,-63.975486542669));
#168820=CARTESIAN_POINT('Ctrl Pts',(33.35,-59.0838703919199,-63.828995910853));
#168821=CARTESIAN_POINT('Ctrl Pts',(33.5828208370019,-58.9513545007691,
-63.7641770795492));
#168822=CARTESIAN_POINT('Ctrl Pts',(33.35,-60.7669593817595,-61.4386408691297));
#168823=CARTESIAN_POINT('Ctrl Pts',(33.35,-60.5242644024533,-61.2999665374096));
#168824=CARTESIAN_POINT('Ctrl Pts',(33.5881101525803,-60.3971457002532,
-61.2273317382593));
#168825=CARTESIAN_POINT('',(33.35,-56.3642045114132,-69.0177323827589));
#168826=CARTESIAN_POINT('Origin',(33.85,-56.3642045114132,-69.0177323827589));
#168827=CARTESIAN_POINT('Ctrl Pts',(33.35,-56.3642045114132,-69.0177323827589));
#168828=CARTESIAN_POINT('Ctrl Pts',(33.35,-57.8514954063616,-66.5028158819518));
#168829=CARTESIAN_POINT('Ctrl Pts',(33.35,-59.3174212852614,-63.975488272466));
#168830=CARTESIAN_POINT('Ctrl Pts',(33.35,-60.7669593817595,-61.4386408691297));
#168831=CARTESIAN_POINT('Ctrl Pts',(33.5694121272515,-56.0311308231553,
-68.7681930766575));
#168832=CARTESIAN_POINT('Ctrl Pts',(33.35,-56.1587194716786,-68.8446841104126));
#168833=CARTESIAN_POINT('Ctrl Pts',(33.35,-56.3860793134489,-68.980989400591));
#168834=CARTESIAN_POINT('Ctrl Pts',(33.5910952109519,-55.7655514639883,
-69.1827326666124));
#168835=CARTESIAN_POINT('Ctrl Pts',(33.35,-55.8926720909797,-69.2555053068349));
#168836=CARTESIAN_POINT('Ctrl Pts',(33.35,-56.1470456681896,-69.379827229092));
#168837=CARTESIAN_POINT('Ctrl Pts',(33.6136638920077,-55.5467927199511,
-69.6144308420505));
#168838=CARTESIAN_POINT('Ctrl Pts',(33.35,-55.6739612204769,-69.6790964973634));
#168839=CARTESIAN_POINT('Ctrl Pts',(33.35,-55.9501721297621,-69.7949917247217));
#168840=CARTESIAN_POINT('Ctrl Pts',(33.659375070679,-55.1847160495168,-70.489496195354));
#168841=CARTESIAN_POINT('Ctrl Pts',(33.35,-55.3038384109907,-70.536501599542));
#168842=CARTESIAN_POINT('Ctrl Pts',(33.35,-55.6242976847011,-70.6362303826783));
#168843=CARTESIAN_POINT('Ctrl Pts',(33.682489279096,-55.039631648896,-70.9322999995547));
#168844=CARTESIAN_POINT('Ctrl Pts',(33.35,-55.152089096076,-70.9724572353069));
#168845=CARTESIAN_POINT('Ctrl Pts',(33.35,-55.4937179039915,-71.0617579129361));
#168846=CARTESIAN_POINT('Ctrl Pts',(33.7541801885443,-54.6881003351372,
-72.3070874300299));
#168847=CARTESIAN_POINT('Ctrl Pts',(33.35,-54.7604537006047,-72.352581791756));
#168848=CARTESIAN_POINT('Ctrl Pts',(33.35,-55.1773203769037,-72.3823434918717));
#168849=CARTESIAN_POINT('Ctrl Pts',(33.8033026557133,-54.5764726761907,
-73.2509483926675));
#168850=CARTESIAN_POINT('Ctrl Pts',(33.3499999999908,-54.6214526391974,
-73.2954399089219));
#168851=CARTESIAN_POINT('Ctrl Pts',(33.35,-55.076843343761,-73.2882195565875));
#168852=CARTESIAN_POINT('Ctrl Pts',(33.8525101260014,-54.580084950057,-74.1994042577821));
#168853=CARTESIAN_POINT('Ctrl Pts',(33.3500000000004,-54.5775630671305,
-74.1994064437527));
#168854=CARTESIAN_POINT('Ctrl Pts',(33.35,-55.0800755412332,-74.1975793503824));
#168855=CARTESIAN_POINT('',(33.35,-55.08000002,-74.155095361993));
#168856=CARTESIAN_POINT('Origin',(33.85,-55.08000002,-74.155095361993));
#168857=CARTESIAN_POINT('Ctrl Pts',(33.35,-55.08000002,-74.155095361993));
#168858=CARTESIAN_POINT('Ctrl Pts',(33.35,-55.0800000199996,-73.9307666441726));
#168859=CARTESIAN_POINT('Ctrl Pts',(33.35,-55.0863156531016,-73.7071338026571));
#168860=CARTESIAN_POINT('Ctrl Pts',(33.35,-55.099013419779,-73.4842001164092));
#168861=CARTESIAN_POINT('Ctrl Pts',(33.35,-55.1117111864564,-73.2612664301613));
#168862=CARTESIAN_POINT('Ctrl Pts',(33.35,-55.1307909278358,-73.0390315071252));
#168863=CARTESIAN_POINT('Ctrl Pts',(33.35,-55.1563760274665,-72.8175000855932));
#168864=CARTESIAN_POINT('Ctrl Pts',(33.35,-55.1806216024911,-72.6075670863644));
#168865=CARTESIAN_POINT('Ctrl Pts',(33.35,-55.2107500142178,-72.3979880684073));
#168866=CARTESIAN_POINT('Ctrl Pts',(33.35,-55.2468600350683,-72.1892231805732));
#168867=CARTESIAN_POINT('Ctrl Pts',(33.35,-55.2824608236504,-71.9834023457995));
#168868=CARTESIAN_POINT('Ctrl Pts',(33.35,-55.3238757306222,-71.7783731405225));
#168869=CARTESIAN_POINT('Ctrl Pts',(33.35,-55.3711489449075,-71.5745698720748));
#168870=CARTESIAN_POINT('Ctrl Pts',(33.35,-55.3771233770104,-71.5488130284138));
#168871=CARTESIAN_POINT('Ctrl Pts',(33.35,-55.3831913115128,-71.5230757533215));
#168872=CARTESIAN_POINT('Ctrl Pts',(33.35,-55.3893527788882,-71.4973589120773));
#168873=CARTESIAN_POINT('Ctrl Pts',(33.35,-55.49371790368,-71.061757912807));
#168874=CARTESIAN_POINT('Ctrl Pts',(33.35,-55.62429768467,-70.6362303826932));
#168875=CARTESIAN_POINT('Ctrl Pts',(33.35,-55.7846973533805,-70.2221616988514));
#168876=CARTESIAN_POINT('Ctrl Pts',(33.35,-55.9170285274604,-69.8805512982628));
#168877=CARTESIAN_POINT('Ctrl Pts',(33.35,-56.0694235889258,-69.5466508244303));
#168878=CARTESIAN_POINT('Ctrl Pts',(33.35,-56.2474267878585,-69.2225907452635));
#168879=CARTESIAN_POINT('Ctrl Pts',(33.35,-56.2851826822517,-69.1538550247853));
#168880=CARTESIAN_POINT('Ctrl Pts',(33.35,-56.3240908525654,-69.0855620876847));
#168881=CARTESIAN_POINT('Ctrl Pts',(33.35,-56.3642045114132,-69.0177323827589));
#168882=CARTESIAN_POINT('Origin',(33.85,-55.08000002,-55.24995));
#168883=CARTESIAN_POINT('',(33.35,-55.08000002,-157.903547609535));
#168884=CARTESIAN_POINT('Origin',(33.85,-55.08000002,-157.903547609535));
#168885=CARTESIAN_POINT('',(33.35,-55.08000002,-74.7820934264633));
#168886=CARTESIAN_POINT('Ctrl Pts',(33.85,-54.58000002,-157.903547609535));
#168887=CARTESIAN_POINT('Ctrl Pts',(33.35,-54.58000002,-157.903547609535));
#168888=CARTESIAN_POINT('Ctrl Pts',(33.35,-55.08000002,-157.903547609535));
#168889=CARTESIAN_POINT('Ctrl Pts',(33.801455552521,-54.58000002,-158.839330848163));
#168890=CARTESIAN_POINT('Ctrl Pts',(33.35,-54.6262905574736,-158.795882575748));
#168891=CARTESIAN_POINT('Ctrl Pts',(33.35,-55.0800000214226,-158.800807467734));
#168892=CARTESIAN_POINT('Ctrl Pts',(33.7535837781314,-54.6911524904427,
-159.759384984053));
#168893=CARTESIAN_POINT('Ctrl Pts',(33.3500000000032,-54.7641489713074,
-159.715131975651));
#168894=CARTESIAN_POINT('Ctrl Pts',(33.35,-55.180037242033,-159.683846218103));
#168895=CARTESIAN_POINT('Ctrl Pts',(33.6829913348673,-55.0359328654928,
-161.113586648345));
#168896=CARTESIAN_POINT('Ctrl Pts',(33.3499999999985,-55.1482360556977,
-161.073701561693));
#168897=CARTESIAN_POINT('Ctrl Pts',(33.35,-55.4903395816263,-160.984647645179));
#168898=CARTESIAN_POINT('Ctrl Pts',(33.6595586460473,-55.182326049271,-161.562665253801));
#168899=CARTESIAN_POINT('Ctrl Pts',(33.3499999999999,-55.3013905829052,
-161.515682361465));
#168900=CARTESIAN_POINT('Ctrl Pts',(33.35,-55.6220934455112,-161.416204912461));
#168901=CARTESIAN_POINT('Ctrl Pts',(33.6142892652062,-55.5406109894237,
-162.429616508549));
#168902=CARTESIAN_POINT('Ctrl Pts',(33.35,-55.6678404697842,-162.365570451247));
#168903=CARTESIAN_POINT('Ctrl Pts',(33.35,-55.9445498933141,-162.249650631001));
#168904=CARTESIAN_POINT('Ctrl Pts',(33.5923371961949,-55.7524367209228,
-162.849704728299));
#168905=CARTESIAN_POINT('Ctrl Pts',(33.3500000000047,-55.8797778942332,
-162.777810522451));
#168906=CARTESIAN_POINT('Ctrl Pts',(33.35,-56.1351840325082,-162.653651176326));
#168907=CARTESIAN_POINT('Ctrl Pts',(33.571293025353,-56.0068938993578,-163.252219719633));
#168908=CARTESIAN_POINT('Ctrl Pts',(33.35,-56.1347789227877,-163.176590079091));
#168909=CARTESIAN_POINT('Ctrl Pts',(33.35,-56.364204511422,-163.040910588762));
#168910=CARTESIAN_POINT('',(33.35,-56.3642045114216,-163.040910588762));
#168911=CARTESIAN_POINT('Origin',(33.85,-56.3642045114216,-163.040910588762));
#168912=CARTESIAN_POINT('Ctrl Pts',(33.35,-56.3642045114216,-163.040910588762));
#168913=CARTESIAN_POINT('Ctrl Pts',(33.35,-56.1574464964891,-162.691295630997));
#168914=CARTESIAN_POINT('Ctrl Pts',(33.35,-55.982001331389,-162.328090330229));
#168915=CARTESIAN_POINT('Ctrl Pts',(33.35,-55.8312183865757,-161.95418118213));
#168916=CARTESIAN_POINT('Ctrl Pts',(33.35,-55.8149691192272,-161.91388650743));
#168917=CARTESIAN_POINT('Ctrl Pts',(33.35,-55.7990063112411,-161.873467504156));
#168918=CARTESIAN_POINT('Ctrl Pts',(33.35,-55.7833216689026,-161.832927771927));
#168919=CARTESIAN_POINT('Ctrl Pts',(33.35,-55.6220934454647,-161.4162049124));
#168920=CARTESIAN_POINT('Ctrl Pts',(33.35,-55.4903395808871,-160.984647645305));
#168921=CARTESIAN_POINT('Ctrl Pts',(33.35,-55.3869054679322,-160.551047169605));
#168922=CARTESIAN_POINT('Ctrl Pts',(33.35,-55.2731785652169,-160.074298854097));
#168923=CARTESIAN_POINT('Ctrl Pts',(33.35,-55.1917492545591,-159.592825164626));
#168924=CARTESIAN_POINT('Ctrl Pts',(33.35,-55.141467476699,-159.106794321393));
#168925=CARTESIAN_POINT('Ctrl Pts',(33.35,-55.1002871472374,-158.70873937774));
#168926=CARTESIAN_POINT('Ctrl Pts',(33.35,-55.08000002,-158.307627565795));
#168927=CARTESIAN_POINT('Ctrl Pts',(33.35,-55.08000002,-157.903547609535));
#168928=CARTESIAN_POINT('Ctrl Pts',(33.35,-60.9047458754482,-170.861259130871));
#168929=CARTESIAN_POINT('Ctrl Pts',(33.35,-60.6616577186179,-171.000024903864));
#168930=CARTESIAN_POINT('Ctrl Pts',(33.5886122085038,-60.5345771657124,
-171.07256826174));
#168931=CARTESIAN_POINT('Ctrl Pts',(33.35,-59.4103431251365,-168.243382962268));
#168932=CARTESIAN_POINT('Ctrl Pts',(33.3499999999583,-59.1768144406969,
-168.390475993822));
#168933=CARTESIAN_POINT('Ctrl Pts',(33.5831748521597,-59.0440141159766,
-168.454692464379));
#168934=CARTESIAN_POINT('Ctrl Pts',(33.35,-57.8986390322929,-165.635544032027));
#168935=CARTESIAN_POINT('Ctrl Pts',(33.3500000000315,-57.6703808898087,
-165.782543034447));
#168936=CARTESIAN_POINT('Ctrl Pts',(33.5774199132796,-57.5365496870091,
-165.846853703856));
#168937=CARTESIAN_POINT('Ctrl Pts',(33.35,-56.364204511422,-163.040910588762));
#168938=CARTESIAN_POINT('Ctrl Pts',(33.35,-56.1347789227867,-163.176590079091));
#168939=CARTESIAN_POINT('Ctrl Pts',(33.5712930253539,-56.0068938993568,
-163.252219719633));
#168940=CARTESIAN_POINT('',(33.35,-60.9047458754482,-170.861259130871));
#168941=CARTESIAN_POINT('Origin',(33.85,-60.9047458754482,-170.861259130871));
#168942=CARTESIAN_POINT('Ctrl Pts',(33.35,-60.9047458754482,-170.861259130871));
#168943=CARTESIAN_POINT('Ctrl Pts',(33.35,-59.4103419837617,-168.243380962845));
#168944=CARTESIAN_POINT('Ctrl Pts',(33.35,-57.8986402212887,-165.635546042559));
#168945=CARTESIAN_POINT('Ctrl Pts',(33.35,-56.3642045114219,-163.040910588762));
#168946=CARTESIAN_POINT('Ctrl Pts',(33.5750675957151,-60.4869407444486,
-170.953330140827));
#168947=CARTESIAN_POINT('Ctrl Pts',(33.35,-60.6250690696869,-170.899634921035));
#168948=CARTESIAN_POINT('Ctrl Pts',(33.35,-60.8761373158519,-170.801627468756));
#168949=CARTESIAN_POINT('Ctrl Pts',(33.5983572986425,-60.5684969171355,
-171.202165692941));
#168950=CARTESIAN_POINT('Ctrl Pts',(33.3499999999999,-60.6884266834228,
-171.110284935414));
#168951=CARTESIAN_POINT('Ctrl Pts',(33.35,-60.9251533634944,-170.926061957919));
#168952=CARTESIAN_POINT('Ctrl Pts',(33.645886928716,-60.7351980774689,-171.389554331221));
#168953=CARTESIAN_POINT('Ctrl Pts',(33.35,-60.8223319990726,-171.281977972795));
#168954=CARTESIAN_POINT('Ctrl Pts',(33.35,-61.0252654854184,-171.01974252204));
#168955=CARTESIAN_POINT('Ctrl Pts',(33.7566428569643,-61.1261755253357,
-171.621593660576));
#168956=CARTESIAN_POINT('Ctrl Pts',(33.35,-61.1501400117675,-171.544190338249));
#168957=CARTESIAN_POINT('Ctrl Pts',(33.35,-61.2596546585114,-171.135765475889));
#168958=CARTESIAN_POINT('Ctrl Pts',(33.8194265539495,-61.3488867187904,
-171.667078490997));
#168959=CARTESIAN_POINT('Ctrl Pts',(33.35,-61.354614484144,-171.633806784439));
#168960=CARTESIAN_POINT('Ctrl Pts',(33.35,-61.3929914759312,-171.158511634364));
#168961=CARTESIAN_POINT('Ctrl Pts',(33.8808666646521,-61.5682521131594,
-171.644230663833));
#168962=CARTESIAN_POINT('Ctrl Pts',(33.35,-61.5709679425831,-171.67697447423));
#168963=CARTESIAN_POINT('Ctrl Pts',(33.35,-61.5240790589959,-171.147092730284));
#168964=CARTESIAN_POINT('',(33.35,-61.4584329769396,-171.14995));
#168965=CARTESIAN_POINT('Origin',(33.85,-61.4584329769396,-171.14995));
#168966=CARTESIAN_POINT('Ctrl Pts',(33.35,-61.4584329769396,-171.14995));
#168967=CARTESIAN_POINT('Ctrl Pts',(33.35,-61.3933512658348,-171.14995));
#168968=CARTESIAN_POINT('Ctrl Pts',(33.35,-61.3285261814807,-171.141518537402));
#168969=CARTESIAN_POINT('Ctrl Pts',(33.35,-61.2661398376647,-171.12453960829));
#168970=CARTESIAN_POINT('Ctrl Pts',(33.35,-61.2235444953656,-171.112946954302));
#168971=CARTESIAN_POINT('Ctrl Pts',(33.35,-61.1820855819996,-171.097368683161));
#168972=CARTESIAN_POINT('Ctrl Pts',(33.35,-61.1424600695408,-171.077754003862));
#168973=CARTESIAN_POINT('Ctrl Pts',(33.35,-61.1076390364327,-171.06051754798));
#168974=CARTESIAN_POINT('Ctrl Pts',(33.35,-61.0743836755039,-171.040165282673));
#168975=CARTESIAN_POINT('Ctrl Pts',(33.35,-61.0435144499423,-171.016803427715));
#168976=CARTESIAN_POINT('Ctrl Pts',(33.35,-61.0154640589458,-170.995574869044));
#168977=CARTESIAN_POINT('Ctrl Pts',(33.35,-60.989382795281,-170.971860522155));
#168978=CARTESIAN_POINT('Ctrl Pts',(33.35,-60.9659114268316,-170.94570880678));
#168979=CARTESIAN_POINT('Ctrl Pts',(33.35,-60.9427675971707,-170.919922033959));
#168980=CARTESIAN_POINT('Ctrl Pts',(33.35,-60.9221601342061,-170.891765212973));
#168981=CARTESIAN_POINT('Ctrl Pts',(33.35,-60.9047458754482,-170.861259130871));
#168982=CARTESIAN_POINT('Origin',(33.85,-12.9675000200281,-171.14995));
#168983=CARTESIAN_POINT('',(33.35,-63.4074419114814,-171.14995));
#168984=CARTESIAN_POINT('Origin',(33.85,-63.4074419114814,-171.14995));
#168985=CARTESIAN_POINT('',(33.35,-61.8036605881122,-171.14995));
#168986=CARTESIAN_POINT('Ctrl Pts',(33.35,-64.9221832702593,-172.64995));
#168987=CARTESIAN_POINT('Ctrl Pts',(33.3499999999999,-64.4875399013512,
-172.64995));
#168988=CARTESIAN_POINT('Ctrl Pts',(33.7804134495199,-64.4270492358885,
-172.64995));
#168989=CARTESIAN_POINT('Ctrl Pts',(33.35,-64.922183270247,-172.453565067926));
#168990=CARTESIAN_POINT('Ctrl Pts',(33.35,-64.4875399013443,-172.511015867074));
#168991=CARTESIAN_POINT('Ctrl Pts',(33.7804134495211,-64.4270492358883,
-172.51902671195));
#168992=CARTESIAN_POINT('Ctrl Pts',(33.35,-64.8827586015461,-172.257328160063));
#168993=CARTESIAN_POINT('Ctrl Pts',(33.35,-64.4577842162266,-172.371853931892));
#168994=CARTESIAN_POINT('Ctrl Pts',(33.7822246014263,-64.4005115826131,
-172.38820210671));
#168995=CARTESIAN_POINT('Ctrl Pts',(33.35,-64.7310022982632,-171.894521542842));
#168996=CARTESIAN_POINT('Ctrl Pts',(33.35,-64.3449732070946,-172.118296873734));
#168997=CARTESIAN_POINT('Ctrl Pts',(33.7891962191206,-64.2983609167864,
-172.14633102856));
#168998=CARTESIAN_POINT('Ctrl Pts',(33.35,-64.6187303406215,-171.728129909852));
#168999=CARTESIAN_POINT('Ctrl Pts',(33.3500000000013,-64.2614041148292,
-172.003556970023));
#169000=CARTESIAN_POINT('Ctrl Pts',(33.7943539433762,-64.2227880741536,
-172.035403273235));
#169001=CARTESIAN_POINT('Ctrl Pts',(33.35,-64.3383212554124,-171.450449746589));
#169002=CARTESIAN_POINT('Ctrl Pts',(33.3499999999986,-64.0569588954535,
-171.817687494207));
#169003=CARTESIAN_POINT('Ctrl Pts',(33.8072358131761,-64.0340382552807,
-171.850283164391));
#169004=CARTESIAN_POINT('Ctrl Pts',(33.35,-64.1702943967697,-171.339270411997));
#169005=CARTESIAN_POINT('Ctrl Pts',(33.3499999999999,-63.9353951792977,
-171.746711574348));
#169006=CARTESIAN_POINT('Ctrl Pts',(33.8149548930127,-63.9209355035967,
-171.776163607997));
#169007=CARTESIAN_POINT('Ctrl Pts',(33.35,-63.8039222708381,-171.18899099047));
#169008=CARTESIAN_POINT('Ctrl Pts',(33.3499999999999,-63.6769599183967,
-171.658003579003));
#169009=CARTESIAN_POINT('Ctrl Pts',(33.831785867019,-63.6743219805034,-171.675977326981));
#169010=CARTESIAN_POINT('Ctrl Pts',(33.35,-63.6057568308558,-171.149950000016));
#169011=CARTESIAN_POINT('Ctrl Pts',(33.35,-63.5396903402446,-171.640924254979));
#169012=CARTESIAN_POINT('Ctrl Pts',(33.8408895000012,-63.5409322550068,
-171.64995));
#169013=CARTESIAN_POINT('Ctrl Pts',(33.35,-63.4074419114814,-171.14995));
#169014=CARTESIAN_POINT('Ctrl Pts',(33.35,-63.4074419114814,-171.64995));
#169015=CARTESIAN_POINT('Ctrl Pts',(33.85,-63.4074419114814,-171.64995));
#169016=CARTESIAN_POINT('',(33.35,-64.9221832702593,-172.64995));
#169017=CARTESIAN_POINT('Origin',(33.85,-64.9221832702593,-172.64995));
#169018=CARTESIAN_POINT('Ctrl Pts',(33.35,-64.9221832702593,-172.64995));
#169019=CARTESIAN_POINT('Ctrl Pts',(33.35,-64.922183270247,-172.453565067926));
#169020=CARTESIAN_POINT('Ctrl Pts',(33.35,-64.8827586015461,-172.257328160063));
#169021=CARTESIAN_POINT('Ctrl Pts',(33.35,-64.7310022982632,-171.894521542842));
#169022=CARTESIAN_POINT('Ctrl Pts',(33.35,-64.6187303406215,-171.728129909852));
#169023=CARTESIAN_POINT('Ctrl Pts',(33.35,-64.3383212554124,-171.450449746589));
#169024=CARTESIAN_POINT('Ctrl Pts',(33.35,-64.1702943967697,-171.339270411997));
#169025=CARTESIAN_POINT('Ctrl Pts',(33.35,-63.8039222708381,-171.18899099047));
#169026=CARTESIAN_POINT('Ctrl Pts',(33.35,-63.6057568308558,-171.149950000016));
#169027=CARTESIAN_POINT('Ctrl Pts',(33.35,-63.4074419114814,-171.14995));
#169028=CARTESIAN_POINT('Origin',(33.85,-64.9221832702593,-171.64995));
#169029=CARTESIAN_POINT('',(33.7804134495199,-64.4270492358885,-171.64995));
#169030=CARTESIAN_POINT('',(33.35,-64.9221832702593,-55.24995));
#169031=CARTESIAN_POINT('Origin',(32.85,-73.08000002,-176.84995));
#169032=CARTESIAN_POINT('',(33.35,67.7009572055632,-176.84995));
#169033=CARTESIAN_POINT('Origin',(32.85,-70.08000002,-58.24995));
#169034=CARTESIAN_POINT('',(33.35,-70.08000002,-55.74995));
#169035=CARTESIAN_POINT('Origin',(33.35,-70.08000002,-58.24995));
#169036=CARTESIAN_POINT('',(32.85,-70.08000002,-55.24995));
#169037=CARTESIAN_POINT('Origin',(32.85,-70.08000002,-55.74995));
#169038=CARTESIAN_POINT('Origin',(32.85,-70.08000002,-58.24995));
#169039=CARTESIAN_POINT('Origin',(-3.3975957231091E-14,-70.08000002,-58.24995));
#169040=CARTESIAN_POINT('',(32.35,-70.08000002,-55.24995));
#169041=CARTESIAN_POINT('',(41.5,-70.08000002,-55.24995));
#169042=CARTESIAN_POINT('Origin',(32.35,-70.08000002,-58.24995));
#169043=CARTESIAN_POINT('Origin',(32.35,-70.08000002,-58.24995));
#169044=CARTESIAN_POINT('',(31.85,-70.08000002,-55.74995));
#169045=CARTESIAN_POINT('Origin',(32.35,-70.08000002,-55.74995));
#169046=CARTESIAN_POINT('',(31.85,-72.58000002,-58.24995));
#169047=CARTESIAN_POINT('Origin',(31.85,-70.08000002,-58.24995));
#169048=CARTESIAN_POINT('Origin',(32.35,-72.58000002,-58.24995));
#169049=CARTESIAN_POINT('Origin',(32.35,-72.58000002,-55.24995));
#169050=CARTESIAN_POINT('',(31.85,-72.58000002,-174.34995));
#169051=CARTESIAN_POINT('',(31.85,-72.58000002,-58.24995));
#169052=CARTESIAN_POINT('Origin',(32.35,-72.58000002,-174.34995));
#169053=CARTESIAN_POINT('Origin',(32.35,-70.08000002,-174.34995));
#169054=CARTESIAN_POINT('',(31.85,-70.08000002,-176.84995));
#169055=CARTESIAN_POINT('Origin',(31.85,-70.08000002,-174.34995));
#169056=CARTESIAN_POINT('Origin',(32.35,-70.08000002,-176.84995));
#169057=CARTESIAN_POINT('Origin',(32.35,67.7009572055632,-176.84995));
#169058=CARTESIAN_POINT('',(31.85,67.7009572055632,-176.84995));
#169059=CARTESIAN_POINT('Origin',(31.35,-65.2735353570153,-171.64995));
#169060=CARTESIAN_POINT('',(31.85,-65.2735353570153,-172.64995));
#169061=CARTESIAN_POINT('',(31.85,-65.2735353570153,-55.24995));
#169062=CARTESIAN_POINT('Origin',(31.35,-65.2735353570153,-172.64995));
#169063=CARTESIAN_POINT('',(31.28041344952,-64.7784013226445,-171.64995));
#169064=CARTESIAN_POINT('Ctrl Pts',(31.85,-63.7585925544192,-171.149950013428));
#169065=CARTESIAN_POINT('Ctrl Pts',(31.8499999999999,-63.7586583477387,
-171.65003477338));
#169066=CARTESIAN_POINT('Ctrl Pts',(31.3499152383757,-63.7586584017713,
-171.649950001854));
#169067=CARTESIAN_POINT('Ctrl Pts',(31.85,-63.9569747212759,-171.149923566191));
#169068=CARTESIAN_POINT('Ctrl Pts',(31.85,-63.8934770903365,-171.659221103016));
#169069=CARTESIAN_POINT('Ctrl Pts',(31.3408008078195,-63.8921937709272,
-171.649930655763));
#169070=CARTESIAN_POINT('Ctrl Pts',(31.85,-64.1552123321859,-171.188965548735));
#169071=CARTESIAN_POINT('Ctrl Pts',(31.85,-64.0229027076712,-171.695281914067));
#169072=CARTESIAN_POINT('Ctrl Pts',(31.3316930631424,-64.0256328180304,
-171.675956808334));
#169073=CARTESIAN_POINT('Ctrl Pts',(31.85,-64.521646483527,-171.339270411997));
#169074=CARTESIAN_POINT('Ctrl Pts',(31.85,-64.2556937071631,-171.81002165518));
#169075=CARTESIAN_POINT('Ctrl Pts',(31.3148578735171,-64.2722905946127,
-171.776157476854));
#169076=CARTESIAN_POINT('Ctrl Pts',(31.85,-64.6896733421684,-171.450449746589));
#169077=CARTESIAN_POINT('Ctrl Pts',(31.850000000002,-64.3582551123188,-171.889069508912));
#169078=CARTESIAN_POINT('Ctrl Pts',(31.3071382160674,-64.3853952154975,
-171.850276197781));
#169079=CARTESIAN_POINT('Ctrl Pts',(31.85,-64.9700824273775,-171.728129909852));
#169080=CARTESIAN_POINT('Ctrl Pts',(31.8499999999979,-64.5258884542433,
-172.075284894373));
#169081=CARTESIAN_POINT('Ctrl Pts',(31.294255447738,-64.5741487063124,-172.035396209826));
#169082=CARTESIAN_POINT('Ctrl Pts',(31.85,-65.0823543850191,-171.894521542842));
#169083=CARTESIAN_POINT('Ctrl Pts',(31.85,-64.5901493684385,-172.182240159754));
#169084=CARTESIAN_POINT('Ctrl Pts',(31.289097389763,-64.6497234916245,-172.14632470545));
#169085=CARTESIAN_POINT('Ctrl Pts',(31.85,-65.2341363800668,-172.257389581842));
#169086=CARTESIAN_POINT('Ctrl Pts',(31.8499999999999,-64.6765834404086,
-172.409795949396));
#169087=CARTESIAN_POINT('Ctrl Pts',(31.2821241606569,-64.7518941169831,
-172.388239289312));
#169088=CARTESIAN_POINT('Ctrl Pts',(31.85,-65.2735620506093,-172.453697958274));
#169089=CARTESIAN_POINT('Ctrl Pts',(31.85,-64.6982492704848,-172.529747068593));
#169090=CARTESIAN_POINT('Ctrl Pts',(31.2803128569907,-64.7784332664479,
-172.519113452117));
#169091=CARTESIAN_POINT('Ctrl Pts',(31.85,-65.2735353434557,-172.650149483381));
#169092=CARTESIAN_POINT('Ctrl Pts',(31.8499999999999,-64.6982345639698,
-172.650072180543));
#169093=CARTESIAN_POINT('Ctrl Pts',(31.2803140827874,-64.7784152888562,
-172.650082990805));
#169094=CARTESIAN_POINT('',(31.85,-63.7587939982373,-171.14995));
#169095=CARTESIAN_POINT('Ctrl Pts',(31.85,-63.7587939982373,-171.14995));
#169096=CARTESIAN_POINT('Ctrl Pts',(31.85,-63.9571089176128,-171.149950000016));
#169097=CARTESIAN_POINT('Ctrl Pts',(31.85,-64.1552743575927,-171.18899099047));
#169098=CARTESIAN_POINT('Ctrl Pts',(31.85,-64.521646483527,-171.339270411997));
#169099=CARTESIAN_POINT('Ctrl Pts',(31.85,-64.6896733421684,-171.450449746589));
#169100=CARTESIAN_POINT('Ctrl Pts',(31.85,-64.9700824273775,-171.728129909852));
#169101=CARTESIAN_POINT('Ctrl Pts',(31.85,-65.0823543850191,-171.894521542842));
#169102=CARTESIAN_POINT('Ctrl Pts',(31.85,-65.2341106883021,-172.257328160063));
#169103=CARTESIAN_POINT('Ctrl Pts',(31.85,-65.273535357003,-172.453565067926));
#169104=CARTESIAN_POINT('Ctrl Pts',(31.85,-65.2735353570153,-172.64995));
#169105=CARTESIAN_POINT('Origin',(31.35,-63.7587939982373,-171.14995));
#169106=CARTESIAN_POINT('Origin',(31.35,-12.9675000200281,-171.14995));
#169107=CARTESIAN_POINT('',(31.85,-63.1109998882233,-171.14995));
#169108=CARTESIAN_POINT('',(31.85,-63.6885235808861,-171.14995));
#169109=CARTESIAN_POINT('Origin',(31.35,-63.1109998882233,-171.14995));
#169110=CARTESIAN_POINT('Ctrl Pts',(31.3495340997183,-63.1109998882233,
-171.649949782937));
#169111=CARTESIAN_POINT('Ctrl Pts',(31.8499999999999,-63.1109998882232,
-171.650416117547));
#169112=CARTESIAN_POINT('Ctrl Pts',(31.85,-63.1109998882233,-171.14995));
#169113=CARTESIAN_POINT('Ctrl Pts',(31.3254339042549,-63.0188799316811,
-171.649927325175));
#169114=CARTESIAN_POINT('Ctrl Pts',(31.8499999999969,-63.0165598996745,
-171.675136694187));
#169115=CARTESIAN_POINT('Ctrl Pts',(31.85,-63.0574084096236,-171.149949978884));
#169116=CARTESIAN_POINT('Ctrl Pts',(31.301798787247,-62.9287579316647,-171.63773683985));
#169117=CARTESIAN_POINT('Ctrl Pts',(31.8500000000009,-62.9205269518794,
-171.689702894937));
#169118=CARTESIAN_POINT('Ctrl Pts',(31.85,-63.0049471542817,-171.14386632127));
#169119=CARTESIAN_POINT('Ctrl Pts',(31.2554698848903,-62.7525001587558,
-171.589540674115));
#169120=CARTESIAN_POINT('Ctrl Pts',(31.8499999999991,-62.7176222625568,
-171.698243814111));
#169121=CARTESIAN_POINT('Ctrl Pts',(31.85,-62.9022833467989,-171.11979081221));
#169122=CARTESIAN_POINT('Ctrl Pts',(31.2324358840903,-62.6650789422019,
-171.552638259287));
#169123=CARTESIAN_POINT('Ctrl Pts',(31.8499999999999,-62.6082192965497,
-171.690638470313));
#169124=CARTESIAN_POINT('Ctrl Pts',(31.85,-62.8513307506207,-171.101350238814));
#169125=CARTESIAN_POINT('Ctrl Pts',(31.1898390398577,-62.5037420018705,
-171.455718071437));
#169126=CARTESIAN_POINT('Ctrl Pts',(31.85,-62.384922264433,-171.644778100208));
#169127=CARTESIAN_POINT('Ctrl Pts',(31.85,-62.7572432252394,-171.052906534958));
#169128=CARTESIAN_POINT('Ctrl Pts',(31.1701167672829,-62.4292143353616,
-171.396060292184));
#169129=CARTESIAN_POINT('Ctrl Pts',(31.8499999999993,-62.2702741424481,
-171.605345720721));
#169130=CARTESIAN_POINT('Ctrl Pts',(31.85,-62.7137529944933,-171.02308307076));
#169131=CARTESIAN_POINT('Ctrl Pts',(31.1344584332459,-62.2946837716206,
-171.25015961779));
#169132=CARTESIAN_POINT('Ctrl Pts',(31.8500000000008,-62.0379421582966,
-171.477274777814));
#169133=CARTESIAN_POINT('Ctrl Pts',(31.85,-62.6352107798375,-170.950134506763));
#169134=CARTESIAN_POINT('Ctrl Pts',(31.1192027095743,-62.2372474415666,
-171.166311520395));
#169135=CARTESIAN_POINT('Ctrl Pts',(31.8499999999999,-61.9259673058959,
-171.38837548536));
#169136=CARTESIAN_POINT('Ctrl Pts',(31.85,-62.6016585634489,-170.908207754234));
#169137=CARTESIAN_POINT('Ctrl Pts',(31.1074206615884,-62.1929294743655,
-171.072435409621));
#169138=CARTESIAN_POINT('Ctrl Pts',(31.85,-61.8321698700148,-171.271436537469));
#169139=CARTESIAN_POINT('Ctrl Pts',(31.85,-62.5757608260974,-170.861259130871));
#169140=CARTESIAN_POINT('',(31.85,-62.5757608260974,-170.861259130871));
#169141=CARTESIAN_POINT('Ctrl Pts',(31.85,-62.5757608260974,-170.861259130871));
#169142=CARTESIAN_POINT('Ctrl Pts',(31.85,-62.5934214847794,-170.893275292324));
#169143=CARTESIAN_POINT('Ctrl Pts',(31.85,-62.6145900881585,-170.922872024471));
#169144=CARTESIAN_POINT('Ctrl Pts',(31.85,-62.6386464997605,-170.949982960699));
#169145=CARTESIAN_POINT('Ctrl Pts',(31.85,-62.6499713199274,-170.962745731906));
#169146=CARTESIAN_POINT('Ctrl Pts',(31.85,-62.6619368642692,-170.974957283073));
#169147=CARTESIAN_POINT('Ctrl Pts',(31.85,-62.6744818503514,-170.986608828398));
#169148=CARTESIAN_POINT('Ctrl Pts',(31.85,-62.7038852881232,-171.013918184158));
#169149=CARTESIAN_POINT('Ctrl Pts',(31.85,-62.7356294724137,-171.037482725823));
#169150=CARTESIAN_POINT('Ctrl Pts',(31.85,-62.7694892975018,-171.057780531265));
#169151=CARTESIAN_POINT('Ctrl Pts',(31.85,-62.780852617915,-171.064592452659));
#169152=CARTESIAN_POINT('Ctrl Pts',(31.85,-62.7924544589394,-171.071036069574));
#169153=CARTESIAN_POINT('Ctrl Pts',(31.85,-62.8042869861286,-171.077128390385));
#169154=CARTESIAN_POINT('Ctrl Pts',(31.85,-62.8513324723594,-171.10135112744));
#169155=CARTESIAN_POINT('Ctrl Pts',(31.85,-62.9022833426441,-171.119790824143));
#169156=CARTESIAN_POINT('Ctrl Pts',(31.85,-62.9536152465698,-171.131828583671));
#169157=CARTESIAN_POINT('Ctrl Pts',(31.85,-63.0049433927144,-171.143865461968));
#169158=CARTESIAN_POINT('Ctrl Pts',(31.85,-63.0574025248319,-171.14995));
#169159=CARTESIAN_POINT('Ctrl Pts',(31.85,-63.1109998882233,-171.14995));
#169160=CARTESIAN_POINT('Origin',(31.35,-62.5757608260974,-170.861259130871));
#169161=CARTESIAN_POINT('Ctrl Pts',(31.85,-56.2763252281792,-159.66866755714));
#169162=CARTESIAN_POINT('Ctrl Pts',(31.8499999999999,-55.4929314270088,
-160.119633364362));
#169163=CARTESIAN_POINT('Ctrl Pts',(31.0842850915597,-55.9092502513102,
-159.879976688011));
#169164=CARTESIAN_POINT('Ctrl Pts',(31.85,-58.4122993941661,-163.37916820794));
#169165=CARTESIAN_POINT('Ctrl Pts',(31.8500000000875,-57.6056192097127,
-163.747040286917));
#169166=CARTESIAN_POINT('Ctrl Pts',(31.0928842088245,-58.0390008802754,
-163.590479273921));
#169167=CARTESIAN_POINT('Ctrl Pts',(31.85,-60.5078533703316,-167.112448841938));
#169168=CARTESIAN_POINT('Ctrl Pts',(31.8499999999999,-59.7238064590067,
-167.480553670321));
#169169=CARTESIAN_POINT('Ctrl Pts',(31.1007058108654,-60.129339000976,-167.323759171684));
#169170=CARTESIAN_POINT('Ctrl Pts',(31.85,-62.5757608260975,-170.861259130871));
#169171=CARTESIAN_POINT('Ctrl Pts',(31.8499999999999,-61.8331341426276,
-171.27090462831));
#169172=CARTESIAN_POINT('Ctrl Pts',(31.1079170675507,-62.1926886331265,
-171.07256826174));
#169173=CARTESIAN_POINT('',(31.85,-56.2763252281792,-159.66866755714));
#169174=CARTESIAN_POINT('Ctrl Pts',(31.85,-56.2763252281792,-159.66866755714));
#169175=CARTESIAN_POINT('Ctrl Pts',(31.85,-58.4123038607033,-163.37917596697));
#169176=CARTESIAN_POINT('Ctrl Pts',(31.85,-60.5078491316876,-167.112441157955));
#169177=CARTESIAN_POINT('Ctrl Pts',(31.85,-62.5757608260974,-170.861259130871));
#169178=CARTESIAN_POINT('Origin',(31.35,-56.2763252281792,-159.66866755714));
#169179=CARTESIAN_POINT('Ctrl Pts',(31.0842850915597,-55.9092502513102,
-159.879976688011));
#169180=CARTESIAN_POINT('Ctrl Pts',(31.85,-55.4929314270087,-160.119633364362));
#169181=CARTESIAN_POINT('Ctrl Pts',(31.85,-56.2763252281792,-159.66866755714));
#169182=CARTESIAN_POINT('Ctrl Pts',(31.1045100388203,-55.6745659332473,
-159.497727845842));
#169183=CARTESIAN_POINT('Ctrl Pts',(31.8499999999999,-55.3073385167954,
-159.699359913876));
#169184=CARTESIAN_POINT('Ctrl Pts',(31.85,-56.0651024669579,-159.301742606223));
#169185=CARTESIAN_POINT('Ctrl Pts',(31.1254451190221,-55.4786764778281,
-159.101707988136));
#169186=CARTESIAN_POINT('Ctrl Pts',(31.85,-55.150888528242,-159.261095570535));
#169187=CARTESIAN_POINT('Ctrl Pts',(31.85,-55.8888088329065,-158.921766047559));
#169188=CARTESIAN_POINT('Ctrl Pts',(31.1683825098781,-55.1470153257944,
-158.288497370345));
#169189=CARTESIAN_POINT('Ctrl Pts',(31.8499999999999,-54.9001304967853,
-158.384215791274));
#169190=CARTESIAN_POINT('Ctrl Pts',(31.85,-55.5903137943537,-158.141820520556));
#169191=CARTESIAN_POINT('Ctrl Pts',(31.1903926108665,-55.0114922210667,
-157.871160476353));
#169192=CARTESIAN_POINT('Ctrl Pts',(31.8499999999999,-54.8012512449405,
-157.943770771097));
#169193=CARTESIAN_POINT('Ctrl Pts',(31.85,-55.4683430012288,-157.741722853926));
#169194=CARTESIAN_POINT('Ctrl Pts',(31.235360609423,-54.7945396526329,-157.017225985171));
#169195=CARTESIAN_POINT('Ctrl Pts',(31.8499999999999,-54.6558194805957,
-157.05645039125));
#169196=CARTESIAN_POINT('Ctrl Pts',(31.85,-55.2730856891008,-156.923456306516));
#169197=CARTESIAN_POINT('Ctrl Pts',(31.2582224016427,-54.7139233464081,
-156.582445743712));
#169198=CARTESIAN_POINT('Ctrl Pts',(31.8500000000015,-54.6065272690148,
-156.610041402948));
#169199=CARTESIAN_POINT('Ctrl Pts',(31.85,-55.2005310139637,-156.507030856831));
#169200=CARTESIAN_POINT('Ctrl Pts',(31.3039546551071,-54.6068982720801,
-155.711146263543));
#169201=CARTESIAN_POINT('Ctrl Pts',(31.8499999999985,-54.5582899067328,
-155.725181694391));
#169202=CARTESIAN_POINT('Ctrl Pts',(31.85,-55.1042084466757,-155.672936697905));
#169203=CARTESIAN_POINT('Ctrl Pts',(31.3269276470654,-54.58000002,-155.272681199498));
#169204=CARTESIAN_POINT('Ctrl Pts',(31.85,-54.5563817475358,-155.28312293345));
#169205=CARTESIAN_POINT('Ctrl Pts',(31.85,-55.0800000206076,-155.253403124156));
#169206=CARTESIAN_POINT('Ctrl Pts',(31.35,-54.58000002,-154.831379798159));
#169207=CARTESIAN_POINT('Ctrl Pts',(31.8499999999999,-54.58000002,-154.831379798158));
#169208=CARTESIAN_POINT('Ctrl Pts',(31.85,-55.08000002,-154.831379798159));
#169209=CARTESIAN_POINT('',(31.85,-55.08000002,-154.831379798159));
#169210=CARTESIAN_POINT('Ctrl Pts',(31.85,-55.08000002,-154.831379798159));
#169211=CARTESIAN_POINT('Ctrl Pts',(31.85,-55.08000002,-155.253410854053));
#169212=CARTESIAN_POINT('Ctrl Pts',(31.85,-55.1042084466772,-155.6729366979));
#169213=CARTESIAN_POINT('Ctrl Pts',(31.85,-55.1523697302198,-156.089983777379));
#169214=CARTESIAN_POINT('Ctrl Pts',(31.85,-55.2005310137623,-156.507030856859));
#169215=CARTESIAN_POINT('Ctrl Pts',(31.85,-55.2730856890926,-156.92345630647));
#169216=CARTESIAN_POINT('Ctrl Pts',(31.85,-55.3707143450195,-157.332589580255));
#169217=CARTESIAN_POINT('Ctrl Pts',(31.85,-55.4683430009464,-157.74172285404));
#169218=CARTESIAN_POINT('Ctrl Pts',(31.85,-55.5903137943579,-158.141820520543));
#169219=CARTESIAN_POINT('Ctrl Pts',(31.85,-55.7395613131142,-158.531793284255));
#169220=CARTESIAN_POINT('Ctrl Pts',(31.85,-55.8729496111504,-158.880327073396));
#169221=CARTESIAN_POINT('Ctrl Pts',(31.85,-56.0279262450874,-159.220847441937));
#169222=CARTESIAN_POINT('Ctrl Pts',(31.85,-56.2101595914815,-159.551250340852));
#169223=CARTESIAN_POINT('Ctrl Pts',(31.85,-56.2318262511927,-159.590533640643));
#169224=CARTESIAN_POINT('Ctrl Pts',(31.85,-56.2538782710457,-159.629673897772));
#169225=CARTESIAN_POINT('Ctrl Pts',(31.85,-56.2763252281792,-159.66866755714));
#169226=CARTESIAN_POINT('Origin',(31.35,-55.08000002,-154.831379798159));
#169227=CARTESIAN_POINT('Origin',(31.35,-55.08000002,-55.24995));
#169228=CARTESIAN_POINT('',(31.85,-55.08000002,-77.227263173365));
#169229=CARTESIAN_POINT('',(31.85,-55.08000002,-155.433057559267));
#169230=CARTESIAN_POINT('Origin',(31.35,-55.08000002,-77.2272631733642));
#169231=CARTESIAN_POINT('Ctrl Pts',(31.3500000000009,-54.58000002,-77.2272631733658));
#169232=CARTESIAN_POINT('Ctrl Pts',(31.85,-54.5800000200009,-77.2272631733658));
#169233=CARTESIAN_POINT('Ctrl Pts',(31.85,-55.08000002,-77.227263173365));
#169234=CARTESIAN_POINT('Ctrl Pts',(31.3038531467957,-54.5800000199985,
-76.3446192991014));
#169235=CARTESIAN_POINT('Ctrl Pts',(31.85,-54.5315963664815,-76.3014537863538));
#169236=CARTESIAN_POINT('Ctrl Pts',(31.85,-55.0800000215433,-76.3831770294161));
#169237=CARTESIAN_POINT('Ctrl Pts',(31.258313471615,-54.6849196157793,-75.4773117729577));
#169238=CARTESIAN_POINT('Ctrl Pts',(31.85,-54.5888070575115,-75.4165208091089));
#169239=CARTESIAN_POINT('Ctrl Pts',(31.85,-55.1744276549191,-75.5528673220433));
#169240=CARTESIAN_POINT('Ctrl Pts',(31.1911093410829,-55.0074869144856,
-74.2010813719198));
#169241=CARTESIAN_POINT('Ctrl Pts',(31.85,-54.7984161464127,-74.129239130374));
#169242=CARTESIAN_POINT('Ctrl Pts',(31.85,-55.4647382256782,-74.3299545388963));
#169243=CARTESIAN_POINT('Ctrl Pts',(31.1687759778426,-55.1442253086702,
-73.7776011027959));
#169244=CARTESIAN_POINT('Ctrl Pts',(31.85,-54.8981200391591,-73.6821630179211));
#169245=CARTESIAN_POINT('Ctrl Pts',(31.85,-55.5878027790484,-73.9239717796963));
#169246=CARTESIAN_POINT('Ctrl Pts',(31.1255062785665,-55.4779574226737,
-72.9580899132975));
#169247=CARTESIAN_POINT('Ctrl Pts',(31.85,-55.1503671712329,-72.798619733739));
#169248=CARTESIAN_POINT('Ctrl Pts',(31.85,-55.8881616831611,-73.1379857970122));
#169249=CARTESIAN_POINT('Ctrl Pts',(31.1044941422599,-55.6747504070549,
-72.5606146570313));
#169250=CARTESIAN_POINT('Ctrl Pts',(31.8500000000028,-55.3074747056296,
-72.358974665281));
#169251=CARTESIAN_POINT('Ctrl Pts',(31.85,-56.0652689851553,-72.7566110978467));
#169252=CARTESIAN_POINT('Ctrl Pts',(31.0842850915597,-55.9092502513102,
-72.178666283495));
#169253=CARTESIAN_POINT('Ctrl Pts',(31.85,-55.4929314270087,-71.9390096071439));
#169254=CARTESIAN_POINT('Ctrl Pts',(31.85,-56.2763252281792,-72.3899754143654));
#169255=CARTESIAN_POINT('',(31.85,-56.2763252281792,-72.3899754143654));
#169256=CARTESIAN_POINT('Ctrl Pts',(31.85,-56.2763252281792,-72.3899754143654));
#169257=CARTESIAN_POINT('Ctrl Pts',(31.85,-56.0652560607924,-72.7566335394409));
#169258=CARTESIAN_POINT('Ctrl Pts',(31.85,-55.8881616822718,-73.1379857966025));
#169259=CARTESIAN_POINT('Ctrl Pts',(31.85,-55.737982230652,-73.5309787881812));
#169260=CARTESIAN_POINT('Ctrl Pts',(31.85,-55.5878027790321,-73.9239717797599));
#169261=CARTESIAN_POINT('Ctrl Pts',(31.85,-55.4647382249676,-74.3299545387688));
#169262=CARTESIAN_POINT('Ctrl Pts',(31.85,-55.367968034963,-74.7375921331689));
#169263=CARTESIAN_POINT('Ctrl Pts',(31.85,-55.2585018339704,-75.1987107776467));
#169264=CARTESIAN_POINT('Ctrl Pts',(31.85,-55.1807511519299,-75.664581041178));
#169265=CARTESIAN_POINT('Ctrl Pts',(31.85,-55.1338484059999,-76.1350729813846));
#169266=CARTESIAN_POINT('Ctrl Pts',(31.85,-55.0978253247024,-76.4964285710373));
#169267=CARTESIAN_POINT('Ctrl Pts',(31.85,-55.0800000199994,-76.8605105831137));
#169268=CARTESIAN_POINT('Ctrl Pts',(31.85,-55.08000002,-77.227263173365));
#169269=CARTESIAN_POINT('Origin',(31.35,-56.2763252281792,-72.3899754143654));
#169270=CARTESIAN_POINT('Ctrl Pts',(31.85,-62.4426282692182,-61.4386408691297));
#169271=CARTESIAN_POINT('Ctrl Pts',(31.85,-61.6992317916068,-61.0282555233051));
#169272=CARTESIAN_POINT('Ctrl Pts',(31.1074520910898,-62.0598503138784,
-61.2273317382593));
#169273=CARTESIAN_POINT('Ctrl Pts',(31.85,-60.4178950612392,-65.1063632921145));
#169274=CARTESIAN_POINT('Ctrl Pts',(31.8500000000147,-59.6343590655212,
-64.7356884621635));
#169275=CARTESIAN_POINT('Ctrl Pts',(31.1003696873064,-60.0396054978548,
-64.8950530477878));
#169276=CARTESIAN_POINT('Ctrl Pts',(31.85,-58.3664713365843,-68.7590848262753));
#169277=CARTESIAN_POINT('Ctrl Pts',(31.85,-57.56108933629,-68.3880588333245));
#169278=CARTESIAN_POINT('Ctrl Pts',(31.0926997115701,-57.9933062860146,
-68.5477739147732));
#169279=CARTESIAN_POINT('Ctrl Pts',(31.85,-56.2763252281792,-72.3899754143654));
#169280=CARTESIAN_POINT('Ctrl Pts',(31.85,-55.4929314270087,-71.9390096071439));
#169281=CARTESIAN_POINT('Ctrl Pts',(31.0842850915597,-55.9092502513102,
-72.178666283495));
#169282=CARTESIAN_POINT('',(31.85,-62.4426282692182,-61.4386408691297));
#169283=CARTESIAN_POINT('Ctrl Pts',(31.85,-62.4426282692182,-61.4386408691297));
#169284=CARTESIAN_POINT('Ctrl Pts',(31.85,-60.41789121461,-65.1063702600533));
#169285=CARTESIAN_POINT('Ctrl Pts',(31.85,-58.3664753860174,-68.7590777918155));
#169286=CARTESIAN_POINT('Ctrl Pts',(31.85,-56.2763252281792,-72.3899754143654));
#169287=CARTESIAN_POINT('',(31.1074520910898,-62.0598503138784,-61.2273317382593));
#169288=CARTESIAN_POINT('Origin',(31.35,-62.4426282692182,-61.4386408691297));
#169289=CARTESIAN_POINT('Ctrl Pts',(31.0842850915597,-55.9092502513102,
-72.178666283495));
#169290=CARTESIAN_POINT('Ctrl Pts',(31.0866188993887,-56.4872664046269,
-71.1716326888473));
#169291=CARTESIAN_POINT('Ctrl Pts',(31.0889358110602,-57.0723871813429,
-70.1454736819142));
#169292=CARTESIAN_POINT('Ctrl Pts',(31.0912335136878,-57.6645912286248,
-69.1001560516859));
#169293=CARTESIAN_POINT('Ctrl Pts',(31.0934878913511,-58.2456288094846,
-68.0745486957657));
#169294=CARTESIAN_POINT('Ctrl Pts',(31.0957237752392,-58.8334849007926,
-67.0304983146088));
#169295=CARTESIAN_POINT('Ctrl Pts',(31.0979394902314,-59.428182062844,-65.9679985255963));
#169296=CARTESIAN_POINT('Ctrl Pts',(31.1000978632644,-60.007488662236,-64.9329958739871));
#169297=CARTESIAN_POINT('Ctrl Pts',(31.1022370964783,-60.5932867432086,
-63.8804863393331));
#169298=CARTESIAN_POINT('Ctrl Pts',(31.1043561549919,-61.1856397486797,
-62.8104889207958));
#169299=CARTESIAN_POINT('Ctrl Pts',(31.1053929798596,-61.4754695587821,
-62.2869545658413));
#169300=CARTESIAN_POINT('Ctrl Pts',(31.1064249829176,-61.7668692831667,
-61.7592339914446));
#169301=CARTESIAN_POINT('Ctrl Pts',(31.1074520910898,-62.0598503138784,
-61.2273317382593));
#169302=CARTESIAN_POINT('Origin',(31.35,67.7009572055632,-61.14995));
#169303=CARTESIAN_POINT('',(31.35,-62.9782728042642,-60.64995));
#169304=CARTESIAN_POINT('',(31.85,-62.9782728042642,-61.14995));
#169305=CARTESIAN_POINT('Origin',(31.35,-62.9782728042642,-61.14995));
#169306=CARTESIAN_POINT('',(31.85,-64.3526414204797,-61.14995));
#169307=CARTESIAN_POINT('',(31.85,67.7009572055632,-61.14995));
#169308=CARTESIAN_POINT('',(31.35,-64.3526414204797,-60.64995));
#169309=CARTESIAN_POINT('Origin',(31.35,-64.3526414204797,-61.14995));
#169310=CARTESIAN_POINT('',(31.35,-12.9675000200281,-60.64995));
#169311=CARTESIAN_POINT('Ctrl Pts',(31.1074520910898,-62.0598503138784,
-61.2273317382593));
#169312=CARTESIAN_POINT('Ctrl Pts',(31.8499999999999,-61.6992317916067,
-61.028255523305));
#169313=CARTESIAN_POINT('Ctrl Pts',(31.85,-62.4426282692183,-61.4386408691297));
#169314=CARTESIAN_POINT('Ctrl Pts',(31.1192593280084,-62.1041984096607,
-61.1334442002736));
#169315=CARTESIAN_POINT('Ctrl Pts',(31.8500000000001,-61.7930681218295,
-60.9114185604269));
#169316=CARTESIAN_POINT('Ctrl Pts',(31.85,-62.4685470764636,-61.3916901534439));
#169317=CARTESIAN_POINT('Ctrl Pts',(31.1342845229578,-62.1606836378221,
-61.0509981549565));
#169318=CARTESIAN_POINT('Ctrl Pts',(31.8499999999998,-61.9033127772783,
-60.8239692453656));
#169319=CARTESIAN_POINT('Ctrl Pts',(31.85,-62.5015432853809,-61.3504740791978));
#169320=CARTESIAN_POINT('Ctrl Pts',(31.1697097530512,-62.2941363459118,
-60.9056817830676));
#169321=CARTESIAN_POINT('Ctrl Pts',(31.8500000000002,-62.1341758421231,
-60.6961222616711));
#169322=CARTESIAN_POINT('Ctrl Pts',(31.85,-62.5794711033445,-61.2778158898142));
#169323=CARTESIAN_POINT('Ctrl Pts',(31.1896892584046,-62.369523292851,-60.8449704353912));
#169324=CARTESIAN_POINT('Ctrl Pts',(31.8500000000001,-62.2503354665,-60.6558084251244));
#169325=CARTESIAN_POINT('Ctrl Pts',(31.85,-62.6234753527752,-61.2474602210686));
#169326=CARTESIAN_POINT('Ctrl Pts',(31.2539016024624,-62.6123775685824,
-60.6987791235328));
#169327=CARTESIAN_POINT('Ctrl Pts',(31.8499999999996,-62.5772240699999,
-60.5884818802849));
#169328=CARTESIAN_POINT('Ctrl Pts',(31.85,-62.765153261125,-61.1743645550205));
#169329=CARTESIAN_POINT('Ctrl Pts',(31.3019361194217,-62.7947963971694,
-60.64995));
#169330=CARTESIAN_POINT('Ctrl Pts',(31.85,-62.7861985042763,-60.599633723582));
#169331=CARTESIAN_POINT('Ctrl Pts',(31.85,-62.8714721065165,-61.1499500118284));
#169332=CARTESIAN_POINT('Ctrl Pts',(31.35,-62.9782728042642,-60.64995));
#169333=CARTESIAN_POINT('Ctrl Pts',(31.8499999999999,-62.9782728042642,
-60.64995));
#169334=CARTESIAN_POINT('Ctrl Pts',(31.85,-62.9782728042642,-61.14995));
#169335=CARTESIAN_POINT('Ctrl Pts',(31.85,-62.9782728042642,-61.14995));
#169336=CARTESIAN_POINT('Ctrl Pts',(31.85,-62.9222361461989,-61.14995));
#169337=CARTESIAN_POINT('Ctrl Pts',(31.85,-62.8664016141293,-61.1566668506652));
#169338=CARTESIAN_POINT('Ctrl Pts',(31.85,-62.8123519766769,-61.1700628877857));
#169339=CARTESIAN_POINT('Ctrl Pts',(31.85,-62.7632675286839,-61.1822283179041));
#169340=CARTESIAN_POINT('Ctrl Pts',(31.85,-62.7156536890988,-61.1999027909616));
#169341=CARTESIAN_POINT('Ctrl Pts',(31.85,-62.6707013203275,-61.2230949953743));
#169342=CARTESIAN_POINT('Ctrl Pts',(31.85,-62.6234720220053,-61.2474619324435));
#169343=CARTESIAN_POINT('Ctrl Pts',(31.85,-62.5794710795978,-61.2778158553603));
#169344=CARTESIAN_POINT('Ctrl Pts',(31.85,-62.5405071542091,-61.3141449414402));
#169345=CARTESIAN_POINT('Ctrl Pts',(31.85,-62.5015487187516,-61.350468908832));
#169346=CARTESIAN_POINT('Ctrl Pts',(31.85,-62.4685524875291,-61.3916801947947));
#169347=CARTESIAN_POINT('Ctrl Pts',(31.85,-62.4426282692182,-61.4386408691297));
#169348=CARTESIAN_POINT('Ctrl Pts',(31.1074520910898,-62.0598503138784,
-61.2273317382593));
#169349=CARTESIAN_POINT('Ctrl Pts',(31.1108987502867,-62.072795958949,-61.1999250308078));
#169350=CARTESIAN_POINT('Ctrl Pts',(31.1147345475847,-62.0872074931539,
-61.1725886690502));
#169351=CARTESIAN_POINT('Ctrl Pts',(31.1189833805676,-62.1031783133733,
-61.1455576859644));
#169352=CARTESIAN_POINT('Ctrl Pts',(31.1208390286195,-62.1101534572652,
-61.1337520933918));
#169353=CARTESIAN_POINT('Ctrl Pts',(31.1227733311916,-62.1174255501541,
-61.1220043179659));
#169354=CARTESIAN_POINT('Ctrl Pts',(31.1247876568115,-62.1250000854343,
-61.1103318592589));
#169355=CARTESIAN_POINT('Ctrl Pts',(31.1287109590604,-62.1397530086992,
-61.0875974100488));
#169356=CARTESIAN_POINT('Ctrl Pts',(31.1329376519543,-62.1556525802205,
-61.0651534254741));
#169357=CARTESIAN_POINT('Ctrl Pts',(31.1374716858149,-62.1727165590761,
-61.0431207160486));
#169358=CARTESIAN_POINT('Ctrl Pts',(31.1403005099853,-62.1833629276993,
-61.0293743121004));
#169359=CARTESIAN_POINT('Ctrl Pts',(31.1432488445812,-62.1944620910562,
-61.0157875755612));
#169360=CARTESIAN_POINT('Ctrl Pts',(31.146316387066,-62.2060136847393,-61.0023855422076));
#169361=CARTESIAN_POINT('Ctrl Pts',(31.1481654956904,-62.2129769628714,
-60.9943068226528));
#169362=CARTESIAN_POINT('Ctrl Pts',(31.1500582276936,-62.2201057956471,
-60.986293492844));
#169363=CARTESIAN_POINT('Ctrl Pts',(31.1519971380045,-62.227409991867,-60.9783399690121));
#169364=CARTESIAN_POINT('Ctrl Pts',(31.1557249806558,-62.2414533924559,
-60.9630481397807));
#169365=CARTESIAN_POINT('Ctrl Pts',(31.1596037700658,-62.2560707690401,
-60.9480773991703));
#169366=CARTESIAN_POINT('Ctrl Pts',(31.1636402857178,-62.2712889198747,
-60.9334493797663));
#169367=CARTESIAN_POINT('Ctrl Pts',(31.166544145986,-62.2822368233077,-60.9229260155553));
#169368=CARTESIAN_POINT('Ctrl Pts',(31.1695296424351,-62.2934956800733,
-60.9125801941714));
#169369=CARTESIAN_POINT('Ctrl Pts',(31.1725993165996,-62.3050756093665,
-60.9024228237426));
#169370=CARTESIAN_POINT('Ctrl Pts',(31.1753410923218,-62.3154185862757,
-60.8933504498841));
#169371=CARTESIAN_POINT('Ctrl Pts',(31.1781501655449,-62.3260182489252,
-60.8844284021417));
#169372=CARTESIAN_POINT('Ctrl Pts',(31.1810233977105,-62.3368631657002,
-60.8756799581451));
#169373=CARTESIAN_POINT('Ctrl Pts',(31.1881225361094,-62.3636586213652,
-60.8540644355817));
#169374=CARTESIAN_POINT('Ctrl Pts',(31.1956178552882,-62.3919682155818,
-60.8334957734164));
#169375=CARTESIAN_POINT('Ctrl Pts',(31.2034928509274,-62.4217365557345,
-60.8141976243507));
#169376=CARTESIAN_POINT('Ctrl Pts',(31.2044308739207,-62.4252823846867,
-60.8118989427538));
#169377=CARTESIAN_POINT('Ctrl Pts',(31.2054988244701,-62.4293197487863,
-60.8093185870448));
#169378=CARTESIAN_POINT('Ctrl Pts',(31.2064549723818,-62.4329347477781,
-60.8070416049354));
#169379=CARTESIAN_POINT('Ctrl Pts',(31.206975096698,-62.434901231055,-60.8058029746481));
#169380=CARTESIAN_POINT('Ctrl Pts',(31.2074620124814,-62.4367422457334,
-60.8046531307694));
#169381=CARTESIAN_POINT('Ctrl Pts',(31.2078761028582,-62.4383079307552,
-60.8036805117118));
#169382=CARTESIAN_POINT('Ctrl Pts',(31.2089360045458,-62.4423154428585,
-60.801191005463));
#169383=CARTESIAN_POINT('Ctrl Pts',(31.210008459837,-62.4463709054711,-60.7987103220674));
#169384=CARTESIAN_POINT('Ctrl Pts',(31.21109356135,-62.4504746931321,-60.7962399497209));
#169385=CARTESIAN_POINT('Ctrl Pts',(31.2176343274827,-62.4752114712354,
-60.7813490592517));
#169386=CARTESIAN_POINT('Ctrl Pts',(31.2246242218186,-62.5016658401879,
-60.7668461547674));
#169387=CARTESIAN_POINT('Ctrl Pts',(31.2320809775905,-62.5299093892021,
-60.7530846416116));
#169388=CARTESIAN_POINT('Ctrl Pts',(31.2343612993462,-62.5385464401189,
-60.7488762862891));
#169389=CARTESIAN_POINT('Ctrl Pts',(31.2366852199439,-62.5473505889011,
-60.7447375430121));
#169390=CARTESIAN_POINT('Ctrl Pts',(31.2390530712776,-62.5563232432806,
-60.7406792618884));
#169391=CARTESIAN_POINT('Ctrl Pts',(31.2447507611333,-62.5779138731933,
-60.7309139413801));
#169392=CARTESIAN_POINT('Ctrl Pts',(31.2507016754884,-62.6004763561987,
-60.721616180738));
#169393=CARTESIAN_POINT('Ctrl Pts',(31.2569048308005,-62.6240100284728,
-60.7129476795834));
#169394=CARTESIAN_POINT('Ctrl Pts',(31.2600064084566,-62.6357768646099,
-60.7086134290061));
#169395=CARTESIAN_POINT('Ctrl Pts',(31.2631709773321,-62.6477862416905,
-60.7044366435674));
#169396=CARTESIAN_POINT('Ctrl Pts',(31.2663979733409,-62.6600364364823,
-60.7004383808229));
#169397=CARTESIAN_POINT('Ctrl Pts',(31.2680114713453,-62.6661615338782,
-60.6984392494507));
#169398=CARTESIAN_POINT('Ctrl Pts',(31.2696405761633,-62.6723468361821,
-60.6964847512362));
#169399=CARTESIAN_POINT('Ctrl Pts',(31.2712851822209,-62.678591997083,-60.6945775736112));
#169400=CARTESIAN_POINT('Ctrl Pts',(31.2721074852497,-62.6817145775334,
-60.6936239847987));
#169401=CARTESIAN_POINT('Ctrl Pts',(31.2729336635908,-62.6848521226649,
-60.6926822262165));
#169402=CARTESIAN_POINT('Ctrl Pts',(31.2737637028789,-62.6880045848913,
-60.6917526357354));
#169403=CARTESIAN_POINT('Ctrl Pts',(31.2743969734453,-62.6904097259108,
-60.6910434135348));
#169404=CARTESIAN_POINT('Ctrl Pts',(31.2752507214592,-62.6936524636479,
-60.6901022655063));
#169405=CARTESIAN_POINT('Ctrl Pts',(31.2758255067016,-62.6958357698216,
-60.6894773904497));
#169406=CARTESIAN_POINT('Ctrl Pts',(31.2760041029658,-62.6965141628936,
-60.6892832303661));
#169407=CARTESIAN_POINT('Ctrl Pts',(31.2761557406995,-62.6970901666106,
-60.6891191468964));
#169408=CARTESIAN_POINT('Ctrl Pts',(31.276265388598,-62.6975066730064,-60.6890007076171));
#169409=CARTESIAN_POINT('Ctrl Pts',(31.2794923723847,-62.7097646314778,
-60.6855149897932));
#169410=CARTESIAN_POINT('Ctrl Pts',(31.2831760644004,-62.7237611744023,
-60.6817788945145));
#169411=CARTESIAN_POINT('Ctrl Pts',(31.287323887984,-62.7395282728487,-60.6780123031017));
#169412=CARTESIAN_POINT('Ctrl Pts',(31.2914319889272,-62.7551443738452,
-60.674281783367));
#169413=CARTESIAN_POINT('Ctrl Pts',(31.2959955302348,-62.7724978666158,
-60.6705214565164));
#169414=CARTESIAN_POINT('Ctrl Pts',(31.301019614512,-62.791612885044,-60.6669950606601));
#169415=CARTESIAN_POINT('Ctrl Pts',(31.3059736788063,-62.8104615000466,
-60.6635178117056));
#169416=CARTESIAN_POINT('Ctrl Pts',(31.3113757072995,-62.8310235174328,
-60.6602681537048));
#169417=CARTESIAN_POINT('Ctrl Pts',(31.3172261299313,-62.8533062793187,
-60.6575460641314));
#169418=CARTESIAN_POINT('Ctrl Pts',(31.3228826744743,-62.8748506092043,
-60.6549141823186));
#169419=CARTESIAN_POINT('Ctrl Pts',(31.3289585309402,-62.898004070122,-60.6527757376979));
#169420=CARTESIAN_POINT('Ctrl Pts',(31.3354476363654,-62.9227499384764,
-60.6514431409284));
#169421=CARTESIAN_POINT('Ctrl Pts',(31.3400888166132,-62.9404488396189,
-60.6504900323873));
#169422=CARTESIAN_POINT('Ctrl Pts',(31.3449412714657,-62.9589618928917,
-60.64995));
#169423=CARTESIAN_POINT('Ctrl Pts',(31.35,-62.9782728042642,-60.64995));
#169424=CARTESIAN_POINT('Origin',(0.,-12.9675000200281,-60.64995));
#169425=CARTESIAN_POINT('',(25.5011648721215,-65.1922357602732,-61.2273317382593));
#169426=CARTESIAN_POINT('Origin',(0.,-12.9675000200281,-61.2273317382593));
#169427=CARTESIAN_POINT('Ctrl Pts',(25.5011648721215,-65.1922357602732,
-61.2273317382594));
#169428=CARTESIAN_POINT('Ctrl Pts',(25.4991627264348,-64.5368797680873,
-62.4921139271883));
#169429=CARTESIAN_POINT('Ctrl Pts',(25.4971342104485,-63.8900461478545,
-63.7361686020899));
#169430=CARTESIAN_POINT('Ctrl Pts',(25.4950786388046,-63.2516311374157,
-64.9594484662041));
#169431=CARTESIAN_POINT('Ctrl Pts',(25.4929314940811,-62.5847755573274,
-66.2372238788364));
#169432=CARTESIAN_POINT('Ctrl Pts',(25.4907548287261,-61.9271053228049,
-67.4923322416149));
#169433=CARTESIAN_POINT('Ctrl Pts',(25.488548990673,-61.2785535158614,-68.7247481694799));
#169434=CARTESIAN_POINT('Ctrl Pts',(25.4863229332212,-60.6240568810712,
-69.968460805562));
#169435=CARTESIAN_POINT('Ctrl Pts',(25.4840671719797,-59.9788468670033,
-71.1890632334062));
#169436=CARTESIAN_POINT('Ctrl Pts',(25.4817831377555,-59.3429037702644,
-72.3865566306907));
#169437=CARTESIAN_POINT('Ctrl Pts',(25.4794165618636,-58.6839786169288,
-73.6273256939456));
#169438=CARTESIAN_POINT('Ctrl Pts',(25.4770196348699,-58.0350023501894,
-74.8432853373019));
#169439=CARTESIAN_POINT('Ctrl Pts',(25.4745950365093,-57.3960031446104,
-76.0344647149628));
#169440=CARTESIAN_POINT('Ctrl Pts',(25.4724033328441,-56.8183829813483,
-77.1112254066692));
#169441=CARTESIAN_POINT('Ctrl Pts',(25.4701890367985,-56.2489160726328,
-78.1677381930187));
#169442=CARTESIAN_POINT('Ctrl Pts',(25.4679548160676,-55.6876551762764,
-79.2040423737711));
#169443=CARTESIAN_POINT('Origin',(24.7,-70.08000002,-174.34995));
#169444=CARTESIAN_POINT('',(25.2,-70.08000002,-176.84995));
#169445=CARTESIAN_POINT('Origin',(24.7,-70.08000002,-176.84995));
#169446=CARTESIAN_POINT('',(25.2,-72.58000002,-174.34995));
#169447=CARTESIAN_POINT('Origin',(25.2,-70.08000002,-174.34995));
#169448=CARTESIAN_POINT('Origin',(24.7,-72.58000002,-174.34995));
#169449=CARTESIAN_POINT('Origin',(24.7,-72.58000002,-55.24995));
#169450=CARTESIAN_POINT('',(25.2,-72.58000002,-58.24995));
#169451=CARTESIAN_POINT('',(25.2,-72.58000002,-174.34995));
#169452=CARTESIAN_POINT('Origin',(24.7,-72.58000002,-58.24995));
#169453=CARTESIAN_POINT('Ctrl Pts',(25.2,-56.0768896606488,-79.4153515046414));
#169454=CARTESIAN_POINT('Ctrl Pts',(25.2,-55.8110355215084,-79.2710235754996));
#169455=CARTESIAN_POINT('Ctrl Pts',(25.4679548160676,-55.6876551762764,
-79.2040423737711));
#169456=CARTESIAN_POINT('Ctrl Pts',(25.2,-59.3123390931711,-73.4556067153995));
#169457=CARTESIAN_POINT('Ctrl Pts',(25.2000000000118,-59.0651351497249,
-73.255975182323));
#169458=CARTESIAN_POINT('Ctrl Pts',(25.4808037502955,-58.9154492031739,
-73.2442891352868));
#169459=CARTESIAN_POINT('Ctrl Pts',(25.2,-62.4759645157842,-67.4577026174502));
#169460=CARTESIAN_POINT('Ctrl Pts',(25.200000000035,-62.2130344026582,-67.2677845851136));
#169461=CARTESIAN_POINT('Ctrl Pts',(25.4916367264251,-62.0734180747052,
-67.2463887183684));
#169462=CARTESIAN_POINT('Ctrl Pts',(25.2,-65.5994372375941,-61.4386408691297));
#169463=CARTESIAN_POINT('Ctrl Pts',(25.1999999999999,-65.3080942147003,
-61.2874541854323));
#169464=CARTESIAN_POINT('Ctrl Pts',(25.5011648721215,-65.1922357602732,
-61.2273317382594));
#169465=CARTESIAN_POINT('',(25.2,-56.0768896606488,-79.4153515046414));
#169466=CARTESIAN_POINT('Origin',(25.7,-56.0768896606488,-79.4153515046414));
#169467=CARTESIAN_POINT('',(25.2,-65.5994372375942,-61.4386408691297));
#169468=CARTESIAN_POINT('Origin',(25.7,-65.5994372375942,-61.4386408691297));
#169469=CARTESIAN_POINT('Ctrl Pts',(25.2,-56.0768896606488,-79.4153515046414));
#169470=CARTESIAN_POINT('Ctrl Pts',(25.2,-59.3123551324919,-73.4555771707379));
#169471=CARTESIAN_POINT('Ctrl Pts',(25.2,-62.4759494901776,-67.4577315724186));
#169472=CARTESIAN_POINT('Ctrl Pts',(25.2,-65.5994372375941,-61.4386408691297));
#169473=CARTESIAN_POINT('Ctrl Pts',(25.4545017719006,-55.8438706635705,
-78.943998453909));
#169474=CARTESIAN_POINT('Ctrl Pts',(25.2000000000001,-55.9670041176591,
-79.0175935267739));
#169475=CARTESIAN_POINT('Ctrl Pts',(25.2,-56.2177692725606,-79.1675127966822));
#169476=CARTESIAN_POINT('Ctrl Pts',(25.4946642550745,-55.3775661721662,
-79.6840646292403));
#169477=CARTESIAN_POINT('Ctrl Pts',(25.1999999999996,-55.4896073847247,
-79.7583704081732));
#169478=CARTESIAN_POINT('Ctrl Pts',(25.2,-55.7980013963185,-79.8734371403239));
#169479=CARTESIAN_POINT('Ctrl Pts',(25.5373410788309,-55.060286146179,-80.4743302772342));
#169480=CARTESIAN_POINT('Ctrl Pts',(25.2000000000013,-55.1662734412503,
-80.5380010629174));
#169481=CARTESIAN_POINT('Ctrl Pts',(25.2,-55.5124752416472,-80.6262357014044));
#169482=CARTESIAN_POINT('Ctrl Pts',(25.6012210394754,-54.7627355327589,
-81.6666848695308));
#169483=CARTESIAN_POINT('Ctrl Pts',(25.1999999999993,-54.8412314292706,
-81.6875787444334));
#169484=CARTESIAN_POINT('Ctrl Pts',(25.2,-55.2446154752418,-81.7605756924265));
#169485=CARTESIAN_POINT('Ctrl Pts',(25.6211910848485,-54.694018420619,-82.0406920440613));
#169486=CARTESIAN_POINT('Ctrl Pts',(25.2,-54.7601766884843,-82.0569617949468));
#169487=CARTESIAN_POINT('Ctrl Pts',(25.2,-55.1827439360829,-82.1162012744658));
#169488=CARTESIAN_POINT('Ctrl Pts',(25.6662757795504,-54.5909095821962,
-82.8883828751549));
#169489=CARTESIAN_POINT('Ctrl Pts',(25.2,-54.6218448035381,-82.9004000920468));
#169490=CARTESIAN_POINT('Ctrl Pts',(25.2,-55.0898763101586,-82.9217439686801));
#169491=CARTESIAN_POINT('Ctrl Pts',(25.6914944489404,-54.5694774201419,
-83.364867732155));
#169492=CARTESIAN_POINT('Ctrl Pts',(25.2,-54.5787849570664,-83.3759856193062));
#169493=CARTESIAN_POINT('Ctrl Pts',(25.2,-55.0705472464169,-83.3741940098927));
#169494=CARTESIAN_POINT('Ctrl Pts',(25.7167531711063,-54.5847952699482,
-83.8448396592079));
#169495=CARTESIAN_POINT('Ctrl Pts',(25.1999999999999,-54.5674926027507,
-83.8453670198231));
#169496=CARTESIAN_POINT('Ctrl Pts',(25.2,-55.0842863948154,-83.8295657569677));
#169497=CARTESIAN_POINT('',(25.2,-55.08000002,-83.5456386250819));
#169498=CARTESIAN_POINT('Origin',(25.7,-55.08000002,-83.5456386250819));
#169499=CARTESIAN_POINT('Ctrl Pts',(25.2,-55.08000002,-83.5456386250819));
#169500=CARTESIAN_POINT('Ctrl Pts',(25.2,-55.08000002,-83.1859931739116));
#169501=CARTESIAN_POINT('Ctrl Pts',(25.2,-55.1006621337637,-82.8281867002424));
#169502=CARTESIAN_POINT('Ctrl Pts',(25.2,-55.1417030348396,-82.4721939873445));
#169503=CARTESIAN_POINT('Ctrl Pts',(25.2,-55.1827439359154,-82.1162012744465));
#169504=CARTESIAN_POINT('Ctrl Pts',(25.2,-55.2446154752336,-81.7605756924466));
#169505=CARTESIAN_POINT('Ctrl Pts',(25.2,-55.3267103680732,-81.4129179556859));
#169506=CARTESIAN_POINT('Ctrl Pts',(25.2,-55.4088052609128,-81.0652602189252));
#169507=CARTESIAN_POINT('Ctrl Pts',(25.2,-55.5103655940696,-80.7242806574902));
#169508=CARTESIAN_POINT('Ctrl Pts',(25.2,-55.6343884585548,-80.3910074402699));
#169509=CARTESIAN_POINT('Ctrl Pts',(25.2,-55.75841132304,-80.0577342230496));
#169510=CARTESIAN_POINT('Ctrl Pts',(25.2,-55.9048956589413,-79.7321669507792));
#169511=CARTESIAN_POINT('Ctrl Pts',(25.2,-56.0768896606488,-79.4153515046414));
#169512=CARTESIAN_POINT('Origin',(25.7,-55.08000002,-55.24995));
#169513=CARTESIAN_POINT('',(25.2,-55.08000002,-148.513004346424));
#169514=CARTESIAN_POINT('Origin',(25.7,-55.08000002,-148.513004346424));
#169515=CARTESIAN_POINT('',(25.2,-55.08000002,-84.0594740639255));
#169516=CARTESIAN_POINT('Ctrl Pts',(25.7,-54.58000002,-148.513004346424));
#169517=CARTESIAN_POINT('Ctrl Pts',(25.2,-54.58000002,-148.513004346424));
#169518=CARTESIAN_POINT('Ctrl Pts',(25.2,-55.08000002,-148.513004346424));
#169519=CARTESIAN_POINT('Ctrl Pts',(25.6600482417947,-54.58000002,-149.271156587884));
#169520=CARTESIAN_POINT('Ctrl Pts',(25.2000000000095,-54.6184124317501,
-149.241944845519));
#169521=CARTESIAN_POINT('Ctrl Pts',(25.2,-55.0800000219098,-149.232572052747));
#169522=CARTESIAN_POINT('Ctrl Pts',(25.6205133511944,-54.6700019565425,
-150.014998643991));
#169523=CARTESIAN_POINT('Ctrl Pts',(25.1999999999999,-54.7333981827002,
-149.982853405445));
#169524=CARTESIAN_POINT('Ctrl Pts',(25.2,-55.161001761834,-149.939471833849));
#169525=CARTESIAN_POINT('Ctrl Pts',(25.5425103305472,-55.0316743873447,
-151.47324255767));
#169526=CARTESIAN_POINT('Ctrl Pts',(25.2,-55.1367600846321,-151.417636910868));
#169527=CARTESIAN_POINT('Ctrl Pts',(25.2,-55.4865069516644,-151.326860933587));
#169528=CARTESIAN_POINT('Ctrl Pts',(25.5037571210995,-55.3070348279188,
-152.192808028705));
#169529=CARTESIAN_POINT('Ctrl Pts',(25.2,-55.4199215048179,-152.126493092391));
#169530=CARTESIAN_POINT('Ctrl Pts',(25.2,-55.7343229434107,-152.012278589766));
#169531=CARTESIAN_POINT('Ctrl Pts',(25.4679548160676,-55.6876551762764,
-152.854600597735));
#169532=CARTESIAN_POINT('Ctrl Pts',(25.2,-55.8110355215084,-152.787619396006));
#169533=CARTESIAN_POINT('Ctrl Pts',(25.2,-56.0768896606487,-152.643291466864));
#169534=CARTESIAN_POINT('',(25.2,-56.0768896606488,-152.643291466864));
#169535=CARTESIAN_POINT('Origin',(25.7,-56.0768896606488,-152.643291466864));
#169536=CARTESIAN_POINT('Ctrl Pts',(25.2,-56.0768896606487,-152.643291466864));
#169537=CARTESIAN_POINT('Ctrl Pts',(25.2,-56.014966929036,-152.529228896965));
#169538=CARTESIAN_POINT('Ctrl Pts',(25.2,-55.9563289964364,-152.41374598058));
#169539=CARTESIAN_POINT('Ctrl Pts',(25.2,-55.9007756544418,-152.296934067097));
#169540=CARTESIAN_POINT('Ctrl Pts',(25.2,-55.8430042328461,-152.175458201579));
#169541=CARTESIAN_POINT('Ctrl Pts',(25.2,-55.7885684933974,-152.052544547972));
#169542=CARTESIAN_POINT('Ctrl Pts',(25.2,-55.7372926676245,-151.928266900595));
#169543=CARTESIAN_POINT('Ctrl Pts',(25.2,-55.7009775154016,-151.84024956271));
#169544=CARTESIAN_POINT('Ctrl Pts',(25.2,-55.6662483997963,-151.75154742078));
#169545=CARTESIAN_POINT('Ctrl Pts',(25.2,-55.6330574644204,-151.662180878469));
#169546=CARTESIAN_POINT('Ctrl Pts',(25.2,-55.563802642011,-151.475712375941));
#169547=CARTESIAN_POINT('Ctrl Pts',(25.2,-55.5013746560331,-151.286675000308));
#169548=CARTESIAN_POINT('Ctrl Pts',(25.2,-55.4456440455194,-151.096220906466));
#169549=CARTESIAN_POINT('Ctrl Pts',(25.2,-55.400687777678,-150.94258711033));
#169550=CARTESIAN_POINT('Ctrl Pts',(25.2,-55.3600885309574,-150.78803223373));
#169551=CARTESIAN_POINT('Ctrl Pts',(25.2,-55.323754356376,-150.633166383806));
#169552=CARTESIAN_POINT('Ctrl Pts',(25.2,-55.224809284665,-150.211436351325));
#169553=CARTESIAN_POINT('Ctrl Pts',(25.2,-55.1560866851019,-149.784875950094));
#169554=CARTESIAN_POINT('Ctrl Pts',(25.2,-55.1174016248576,-149.353514705437));
#169555=CARTESIAN_POINT('Ctrl Pts',(25.2,-55.0924544716307,-149.075339228945));
#169556=CARTESIAN_POINT('Ctrl Pts',(25.2,-55.0800000200004,-148.795167064065));
#169557=CARTESIAN_POINT('Ctrl Pts',(25.2,-55.08000002,-148.513004346424));
#169558=CARTESIAN_POINT('Ctrl Pts',(25.2,-65.7246041881209,-170.861259130871));
#169559=CARTESIAN_POINT('Ctrl Pts',(25.2,-65.4329690822618,-171.012528323755));
#169560=CARTESIAN_POINT('Ctrl Pts',(25.5015460489969,-65.317216804244,-171.07256826174));
#169561=CARTESIAN_POINT('Ctrl Pts',(25.2,-62.5605386715726,-164.761189683274));
#169562=CARTESIAN_POINT('Ctrl Pts',(25.1999999998579,-62.297876586317,-164.952133926682));
#169563=CARTESIAN_POINT('Ctrl Pts',(25.4919266567716,-62.1578398412392,
-164.972503788787));
#169564=CARTESIAN_POINT('Ctrl Pts',(25.2,-59.3555677916457,-158.682664145768));
#169565=CARTESIAN_POINT('Ctrl Pts',(25.2,-59.109002613422,-158.883754709366));
#169566=CARTESIAN_POINT('Ctrl Pts',(25.4809754250192,-58.9585757861229,
-158.893982149016));
#169567=CARTESIAN_POINT('Ctrl Pts',(25.2,-56.0768896606488,-152.643291466864));
#169568=CARTESIAN_POINT('Ctrl Pts',(25.2,-55.8110355215084,-152.787619396006));
#169569=CARTESIAN_POINT('Ctrl Pts',(25.4679548160676,-55.6876551762764,
-152.854600597735));
#169570=CARTESIAN_POINT('',(25.2,-65.7246041881209,-170.861259130871));
#169571=CARTESIAN_POINT('Origin',(25.7,-65.7246041881209,-170.861259130871));
#169572=CARTESIAN_POINT('Ctrl Pts',(25.2,-65.7246041881209,-170.861259130871));
#169573=CARTESIAN_POINT('Ctrl Pts',(25.2,-62.5605227754587,-164.761159036905));
#169574=CARTESIAN_POINT('Ctrl Pts',(25.2,-59.3555847723563,-158.682695424483));
#169575=CARTESIAN_POINT('Ctrl Pts',(25.2,-56.0768896606488,-152.643291466864));
#169576=CARTESIAN_POINT('Ctrl Pts',(25.5015460489969,-65.3172168042439,
-171.07256826174));
#169577=CARTESIAN_POINT('Ctrl Pts',(25.2,-65.4329690822618,-171.012528323755));
#169578=CARTESIAN_POINT('Ctrl Pts',(25.2,-65.7246041881209,-170.861259130871));
#169579=CARTESIAN_POINT('Ctrl Pts',(25.5078751098564,-65.3460382794916,
-171.13407782586));
#169580=CARTESIAN_POINT('Ctrl Pts',(25.2,-65.4555942264487,-171.066917428723));
#169581=CARTESIAN_POINT('Ctrl Pts',(25.2,-65.7405566104338,-170.892014084856));
#169582=CARTESIAN_POINT('Ctrl Pts',(25.5154426820321,-65.380521047679,-171.191481806562));
#169583=CARTESIAN_POINT('Ctrl Pts',(25.1999999999994,-65.4828113676634,
-171.118510663779));
#169584=CARTESIAN_POINT('Ctrl Pts',(25.2,-65.7596409576893,-170.920716557309));
#169585=CARTESIAN_POINT('Ctrl Pts',(25.5241645957028,-65.4203114663335,
-171.244965273984));
#169586=CARTESIAN_POINT('Ctrl Pts',(25.2,-65.5143246899125,-171.167561256232));
#169587=CARTESIAN_POINT('Ctrl Pts',(25.2,-65.7816577220592,-170.947457636992));
#169588=CARTESIAN_POINT('',(25.2,-65.7816577220592,-170.947457636992));
#169589=CARTESIAN_POINT('Origin',(25.7,-65.7816577220592,-170.947457636992));
#169590=CARTESIAN_POINT('Ctrl Pts',(25.2,-65.7816577220592,-170.947457636992));
#169591=CARTESIAN_POINT('Ctrl Pts',(25.2,-65.759637326036,-170.920712146581));
#169592=CARTESIAN_POINT('Ctrl Pts',(25.2,-65.7405592277015,-170.892019192244));
#169593=CARTESIAN_POINT('Ctrl Pts',(25.2,-65.7246041881209,-170.861259130871));
#169594=CARTESIAN_POINT('Ctrl Pts',(25.2,-66.1031295107182,-171.854014632589));
#169595=CARTESIAN_POINT('Ctrl Pts',(25.1999999999999,-65.7373527968364,
-171.85401463259));
#169596=CARTESIAN_POINT('Ctrl Pts',(25.5486065204957,-65.6266003779639,
-171.854014632591));
#169597=CARTESIAN_POINT('Ctrl Pts',(25.2,-66.1031295051642,-171.688945996574));
#169598=CARTESIAN_POINT('Ctrl Pts',(25.2,-65.7495636563843,-171.730197187823));
#169599=CARTESIAN_POINT('Ctrl Pts',(25.5332781069629,-65.6314702205409,
-171.740892625582));
#169600=CARTESIAN_POINT('Ctrl Pts',(25.2,-66.0766766441701,-171.528325399449));
#169601=CARTESIAN_POINT('Ctrl Pts',(25.2,-65.7357529125625,-171.605967390697));
#169602=CARTESIAN_POINT('Ctrl Pts',(25.5254918386358,-65.6165368852731,
-171.632443841085));
#169603=CARTESIAN_POINT('Ctrl Pts',(25.2,-65.9668265905144,-171.216885108557));
#169604=CARTESIAN_POINT('Ctrl Pts',(25.1999999999999,-65.6576340206492,
-171.369178819378));
#169605=CARTESIAN_POINT('Ctrl Pts',(25.5190396326646,-65.5455021430107,
-171.42367336987));
#169606=CARTESIAN_POINT('Ctrl Pts',(25.2,-65.8865499901975,-171.074857506769));
#169607=CARTESIAN_POINT('Ctrl Pts',(25.2,-65.5955175213768,-171.261530708485));
#169608=CARTESIAN_POINT('Ctrl Pts',(25.5204167023824,-65.4915081760158,
-171.329224126564));
#169609=CARTESIAN_POINT('Ctrl Pts',(25.2,-65.7816577220592,-170.947457636992));
#169610=CARTESIAN_POINT('Ctrl Pts',(25.1999999999999,-65.5143246899125,
-171.167561256232));
#169611=CARTESIAN_POINT('Ctrl Pts',(25.5241645957028,-65.4203114663335,
-171.244965273984));
#169612=CARTESIAN_POINT('',(25.2,-66.1031295107175,-171.854014632589));
#169613=CARTESIAN_POINT('',(25.5486065204179,-65.6266003779886,-171.854014632026));
#169614=CARTESIAN_POINT('Origin',(25.7,-66.1031295107182,-171.854014632589));
#169615=CARTESIAN_POINT('Ctrl Pts',(25.5241645957028,-65.4203114663335,
-171.244965273985));
#169616=CARTESIAN_POINT('Ctrl Pts',(25.5231299263541,-65.4399665220691,
-171.268226355155));
#169617=CARTESIAN_POINT('Ctrl Pts',(25.522294585227,-65.4579784931356,-171.291877835995));
#169618=CARTESIAN_POINT('Ctrl Pts',(25.5216840617807,-65.474386214064,-171.315718493851));
#169619=CARTESIAN_POINT('Ctrl Pts',(25.5210735383344,-65.4907939349924,
-171.339559151708));
#169620=CARTESIAN_POINT('Ctrl Pts',(25.5206879562631,-65.5055976477405,
-171.363588766213));
#169621=CARTESIAN_POINT('Ctrl Pts',(25.5205350576004,-65.5188821404571,
-171.387584492607));
#169622=CARTESIAN_POINT('Ctrl Pts',(25.5203772443314,-65.5325936352857,
-171.412351511218));
#169623=CARTESIAN_POINT('Ctrl Pts',(25.5204670406992,-65.5446917115373,
-171.437087091981));
#169624=CARTESIAN_POINT('Ctrl Pts',(25.5207940342398,-65.555334013505,-171.46158698178));
#169625=CARTESIAN_POINT('Ctrl Pts',(25.5210214587905,-65.5627357521982,
-171.478626695825));
#169626=CARTESIAN_POINT('Ctrl Pts',(25.5213632022661,-65.5694346066928,
-171.495553194624));
#169627=CARTESIAN_POINT('Ctrl Pts',(25.5218116495206,-65.5754939001744,
-171.512310512318));
#169628=CARTESIAN_POINT('Ctrl Pts',(25.5219110299368,-65.5768367004739,
-171.516024102242));
#169629=CARTESIAN_POINT('Ctrl Pts',(25.5220026056098,-65.5779873853903,
-171.519273109632));
#169630=CARTESIAN_POINT('Ctrl Pts',(25.5221106011063,-65.5792558272748,
-171.522927038886));
#169631=CARTESIAN_POINT('Ctrl Pts',(25.5221580914876,-65.5798136170971,
-171.524533832681));
#169632=CARTESIAN_POINT('Ctrl Pts',(25.5222088848793,-65.5803936558672,
-171.526219210179));
#169633=CARTESIAN_POINT('Ctrl Pts',(25.5222657314613,-65.5810195156442,
-171.528058604948));
#169634=CARTESIAN_POINT('Ctrl Pts',(25.5222827629558,-65.5812070260796,
-171.528609695986));
#169635=CARTESIAN_POINT('Ctrl Pts',(25.5223003400726,-65.5813985772047,
-171.529174456282));
#169636=CARTESIAN_POINT('Ctrl Pts',(25.5223185463672,-65.5815947553066,
-171.529754907915));
#169637=CARTESIAN_POINT('Ctrl Pts',(25.5233919437605,-65.5931609233538,
-171.56397687794));
#169638=CARTESIAN_POINT('Ctrl Pts',(25.5249423650029,-65.602329155868,-171.598090812457));
#169639=CARTESIAN_POINT('Ctrl Pts',(25.5270085019446,-65.6093231945859,
-171.631964042931));
#169640=CARTESIAN_POINT('Ctrl Pts',(25.5290969526855,-65.6163927672979,
-171.66620309643));
#169641=CARTESIAN_POINT('Ctrl Pts',(25.5317125482548,-65.621241287655,-171.700196223063));
#169642=CARTESIAN_POINT('Ctrl Pts',(25.5348601544508,-65.6241378124208,
-171.733792453079));
#169643=CARTESIAN_POINT('Ctrl Pts',(25.5380761467274,-65.6270972681774,
-171.768118607474));
#169644=CARTESIAN_POINT('Ctrl Pts',(25.5418477161118,-65.6280193673831,
-171.802030424976));
#169645=CARTESIAN_POINT('Ctrl Pts',(25.5461401976557,-65.6272249998709,
-171.835352357183));
#169646=CARTESIAN_POINT('Ctrl Pts',(25.5469442697997,-65.6270761981156,
-171.841594256466));
#169647=CARTESIAN_POINT('Ctrl Pts',(25.5477665059252,-65.6268672508965,
-171.8478154174));
#169648=CARTESIAN_POINT('Ctrl Pts',(25.5486065204168,-65.626600377989,-171.854014632026));
#169649=CARTESIAN_POINT('Ctrl Pts',(25.2,-66.1031295107175,-171.854014632589));
#169650=CARTESIAN_POINT('Ctrl Pts',(25.2,-66.1031295063964,-171.725572055906));
#169651=CARTESIAN_POINT('Ctrl Pts',(25.2,-66.0871173562523,-171.599865253242));
#169652=CARTESIAN_POINT('Ctrl Pts',(25.2,-66.0541497294318,-171.477055409759));
#169653=CARTESIAN_POINT('Ctrl Pts',(25.2,-66.0447396524369,-171.442001322027));
#169654=CARTESIAN_POINT('Ctrl Pts',(25.2,-66.0339478541516,-171.407183310008));
#169655=CARTESIAN_POINT('Ctrl Pts',(25.2,-66.0217516132152,-171.372605255459));
#169656=CARTESIAN_POINT('Ctrl Pts',(25.2,-65.9940406295861,-171.294040728197));
#169657=CARTESIAN_POINT('Ctrl Pts',(25.2,-65.9598967243537,-171.219005811922));
#169658=CARTESIAN_POINT('Ctrl Pts',(25.2,-65.9193893860855,-171.147550497276));
#169659=CARTESIAN_POINT('Ctrl Pts',(25.2,-65.8796084720222,-171.077376601561));
#169660=CARTESIAN_POINT('Ctrl Pts',(25.2,-65.8336900811296,-171.010655009758));
#169661=CARTESIAN_POINT('Ctrl Pts',(25.2,-65.7816577220592,-170.947457636992));
#169662=CARTESIAN_POINT('Ctrl Pts',(25.567270247017,-65.4932347742778,-60.8550643728577));
#169663=CARTESIAN_POINT('Ctrl Pts',(25.2,-65.5504599379798,-60.9384440262482));
#169664=CARTESIAN_POINT('Ctrl Pts',(25.2,-65.76604051674,-61.2525142085044));
#169665=CARTESIAN_POINT('Ctrl Pts',(25.5372515674752,-65.3560756313885,
-60.9593757850282));
#169666=CARTESIAN_POINT('Ctrl Pts',(25.1999999999999,-65.4390463676049,
-61.0441607188783));
#169667=CARTESIAN_POINT('Ctrl Pts',(25.2,-65.6901622771225,-61.3046675609273));
#169668=CARTESIAN_POINT('Ctrl Pts',(25.5126788498768,-65.2443062807722,
-61.0990698192377));
#169669=CARTESIAN_POINT('Ctrl Pts',(25.2,-65.3491857740292,-61.1739405307172));
#169670=CARTESIAN_POINT('Ctrl Pts',(25.2,-65.6282820810228,-61.3745120488097));
#169671=CARTESIAN_POINT('Ctrl Pts',(25.4971432604052,-65.1737221584172,
-61.2692230181219));
#169672=CARTESIAN_POINT('Ctrl Pts',(25.2,-65.293642201641,-61.3241535201351));
#169673=CARTESIAN_POINT('Ctrl Pts',(25.2,-65.5891959094587,-61.4595920393833));
#169674=CARTESIAN_POINT('',(25.5598256884619,-65.45949290163,-60.8818893816432));
#169675=CARTESIAN_POINT('Ctrl Pts',(25.5598256882386,-65.4594929016689,
-60.8818893816956));
#169676=CARTESIAN_POINT('Ctrl Pts',(25.5531049092406,-65.4288008059568,
-60.9073497695154));
#169677=CARTESIAN_POINT('Ctrl Pts',(25.5467989300454,-65.4000883723788,
-60.934263332496));
#169678=CARTESIAN_POINT('Ctrl Pts',(25.5409376948429,-65.3734073767371,
-60.9622975884069));
#169679=CARTESIAN_POINT('Ctrl Pts',(25.5349907014394,-65.3463360002097,
-60.9907420253246));
#169680=CARTESIAN_POINT('Ctrl Pts',(25.5295014264852,-65.3213556457941,
-61.0203397151011));
#169681=CARTESIAN_POINT('Ctrl Pts',(25.5244779293711,-65.2984740811048,
-61.0507610829557));
#169682=CARTESIAN_POINT('Ctrl Pts',(25.51932958311,-65.2750238400988,-61.0819385141152));
#169683=CARTESIAN_POINT('Ctrl Pts',(25.5146703184022,-65.2537777129736,
-61.113980610906));
#169684=CARTESIAN_POINT('Ctrl Pts',(25.5104866316509,-65.2347002082,-61.1465583656441));
#169685=CARTESIAN_POINT('Ctrl Pts',(25.5070679032027,-65.2191108937587,
-61.1731795023406));
#169686=CARTESIAN_POINT('Ctrl Pts',(25.5039662672152,-65.2049687286471,
-61.2001587559061));
#169687=CARTESIAN_POINT('Ctrl Pts',(25.5011648721215,-65.1922357602732,
-61.2273317382593));
#169688=CARTESIAN_POINT('',(25.2,-65.7473676730073,-61.2659196908498));
#169689=CARTESIAN_POINT('Origin',(25.7,-65.7473676730073,-61.2659196908498));
#169690=CARTESIAN_POINT('Origin',(25.2,-66.2733246934326,-61.766045927512));
#169691=CARTESIAN_POINT('Origin',(42.,-73.08000002,-171.14995));
#169692=CARTESIAN_POINT('',(41.5,-62.2620341086569,-171.14995));
#169693=CARTESIAN_POINT('Origin',(42.,-62.2620341086569,-171.14995));
#169694=CARTESIAN_POINT('',(42.,-58.6035812240168,-171.64995));
#169695=CARTESIAN_POINT('',(42.,-62.3323045260081,-171.64995));
#169696=CARTESIAN_POINT('',(41.5,-58.6035812240168,-171.14995));
#169697=CARTESIAN_POINT('Origin',(42.,-58.6035812240168,-171.14995));
#169698=CARTESIAN_POINT('',(41.5,-55.58000002,-171.14995));
#169699=CARTESIAN_POINT('Ctrl Pts',(41.5,-63.7767754674349,-172.64995));
#169700=CARTESIAN_POINT('Ctrl Pts',(41.5,-63.3421320985268,-172.64995));
#169701=CARTESIAN_POINT('Ctrl Pts',(41.9304134495199,-63.2816414330641,
-172.64995));
#169702=CARTESIAN_POINT('Ctrl Pts',(41.5,-63.7767754674226,-172.453565067926));
#169703=CARTESIAN_POINT('Ctrl Pts',(41.5,-63.3421320985213,-172.511015867074));
#169704=CARTESIAN_POINT('Ctrl Pts',(41.9304134495211,-63.2816414330639,
-172.51902671195));
#169705=CARTESIAN_POINT('Ctrl Pts',(41.5,-63.7373507987217,-172.257328160063));
#169706=CARTESIAN_POINT('Ctrl Pts',(41.4999999999999,-63.3123764134035,
-172.371853931892));
#169707=CARTESIAN_POINT('Ctrl Pts',(41.9322246014262,-63.2551037797886,
-172.38820210671));
#169708=CARTESIAN_POINT('Ctrl Pts',(41.5,-63.5855944954388,-171.894521542842));
#169709=CARTESIAN_POINT('Ctrl Pts',(41.5,-63.1995654042688,-172.118296873734));
#169710=CARTESIAN_POINT('Ctrl Pts',(41.9391962191206,-63.152953113962,-172.14633102856));
#169711=CARTESIAN_POINT('Ctrl Pts',(41.5,-63.4733225377971,-171.728129909852));
#169712=CARTESIAN_POINT('Ctrl Pts',(41.500000000002,-63.1159963120049,-172.003556970023));
#169713=CARTESIAN_POINT('Ctrl Pts',(41.9443539433762,-63.0773802713291,
-172.035403273235));
#169714=CARTESIAN_POINT('Ctrl Pts',(41.5,-63.192913452588,-171.450449746589));
#169715=CARTESIAN_POINT('Ctrl Pts',(41.499999999998,-62.9115510926292,-171.817687494207));
#169716=CARTESIAN_POINT('Ctrl Pts',(41.9572358131761,-62.8886304524563,
-171.850283164391));
#169717=CARTESIAN_POINT('Ctrl Pts',(41.5,-63.0248865939453,-171.339270411997));
#169718=CARTESIAN_POINT('Ctrl Pts',(41.4999999999999,-62.7899873764732,
-171.746711574348));
#169719=CARTESIAN_POINT('Ctrl Pts',(41.9649548930126,-62.7755277007723,
-171.776163607997));
#169720=CARTESIAN_POINT('Ctrl Pts',(41.5,-62.6585144680136,-171.18899099047));
#169721=CARTESIAN_POINT('Ctrl Pts',(41.5,-62.5315521155723,-171.658003579003));
#169722=CARTESIAN_POINT('Ctrl Pts',(41.981785867019,-62.528914177679,-171.675977326981));
#169723=CARTESIAN_POINT('Ctrl Pts',(41.5,-62.4603490280314,-171.149950000016));
#169724=CARTESIAN_POINT('Ctrl Pts',(41.4999999999999,-62.3942825374201,
-171.640924254979));
#169725=CARTESIAN_POINT('Ctrl Pts',(41.9908895000012,-62.3955244521823,
-171.64995));
#169726=CARTESIAN_POINT('Ctrl Pts',(41.5,-62.2620341086569,-171.14995));
#169727=CARTESIAN_POINT('Ctrl Pts',(41.4999999999999,-62.2620341086569,
-171.64995));
#169728=CARTESIAN_POINT('Ctrl Pts',(42.,-62.2620341086569,-171.64995));
#169729=CARTESIAN_POINT('',(41.5,-63.7767754674349,-172.64995));
#169730=CARTESIAN_POINT('Origin',(42.,-63.7767754674349,-172.64995));
#169731=CARTESIAN_POINT('Ctrl Pts',(41.5,-63.7767754674349,-172.64995));
#169732=CARTESIAN_POINT('Ctrl Pts',(41.5,-63.7767754674226,-172.453565067926));
#169733=CARTESIAN_POINT('Ctrl Pts',(41.5,-63.7373507987217,-172.257328160063));
#169734=CARTESIAN_POINT('Ctrl Pts',(41.5,-63.5855944954388,-171.894521542842));
#169735=CARTESIAN_POINT('Ctrl Pts',(41.5,-63.4733225377971,-171.728129909852));
#169736=CARTESIAN_POINT('Ctrl Pts',(41.5,-63.192913452588,-171.450449746589));
#169737=CARTESIAN_POINT('Ctrl Pts',(41.5,-63.0248865939453,-171.339270411997));
#169738=CARTESIAN_POINT('Ctrl Pts',(41.5,-62.6585144680136,-171.18899099047));
#169739=CARTESIAN_POINT('Ctrl Pts',(41.5,-62.4603490280314,-171.149950000016));
#169740=CARTESIAN_POINT('Ctrl Pts',(41.5,-62.2620341086569,-171.14995));
#169741=CARTESIAN_POINT('Origin',(42.,-63.7767754674349,-171.64995));
#169742=CARTESIAN_POINT('',(41.9304134495199,-63.2816414330641,-171.64995));
#169743=CARTESIAN_POINT('',(41.5,-63.7767754674349,-177.34995));
#169744=CARTESIAN_POINT('Origin',(41.,-73.08000002,-176.84995));
#169745=CARTESIAN_POINT('',(41.5,-70.08000002,-176.84995));
#169746=CARTESIAN_POINT('',(41.5,-73.08000002,-176.84995));
#169747=CARTESIAN_POINT('Origin',(41.,-70.08000002,-176.84995));
#169748=CARTESIAN_POINT('Origin',(41.,-70.08000002,-174.34995));
#169749=CARTESIAN_POINT('',(41.5,-72.58000002,-174.34995));
#169750=CARTESIAN_POINT('Origin',(41.,-72.58000002,-174.34995));
#169751=CARTESIAN_POINT('Origin',(41.5,-70.08000002,-174.34995));
#169752=CARTESIAN_POINT('Origin',(41.,-72.58000002,-4.66002702801304E-15));
#169753=CARTESIAN_POINT('',(41.5,-72.58000002,-58.24995));
#169754=CARTESIAN_POINT('Origin',(41.,-72.58000002,-58.24995));
#169755=CARTESIAN_POINT('',(41.5,-72.58000002,-174.34995));
#169756=CARTESIAN_POINT('Ctrl Pts',(42.0000617764046,-58.6035812240174,
-60.6499500038163));
#169757=CARTESIAN_POINT('Ctrl Pts',(41.5,-58.6035812240175,-60.6498882197787));
#169758=CARTESIAN_POINT('Ctrl Pts',(41.5,-58.6035812240174,-61.14995));
#169759=CARTESIAN_POINT('Ctrl Pts',(41.9298643117028,-58.4475344566847,
-60.6499412757882));
#169760=CARTESIAN_POINT('Ctrl Pts',(41.4999999999957,-58.4568531764755,
-60.7159032420905));
#169761=CARTESIAN_POINT('Ctrl Pts',(41.5,-58.4156885491981,-61.1499499554112));
#169762=CARTESIAN_POINT('Ctrl Pts',(41.8681695534325,-58.2705723212611,
-60.6499357694868));
#169763=CARTESIAN_POINT('Ctrl Pts',(41.5000000000007,-58.2676804549562,
-60.7523419094271));
#169764=CARTESIAN_POINT('Ctrl Pts',(41.5,-58.2277855029442,-61.1325395579243));
#169765=CARTESIAN_POINT('Ctrl Pts',(41.7820591277972,-57.8880263314595,
-60.6499295039941));
#169766=CARTESIAN_POINT('Ctrl Pts',(41.4999999999994,-57.8827900893775,
-60.7882832533183));
#169767=CARTESIAN_POINT('Ctrl Pts',(41.5,-57.8520667952968,-61.1008454187365));
#169768=CARTESIAN_POINT('Ctrl Pts',(41.7580490411453,-57.6823964313119,
-60.6499285241464));
#169769=CARTESIAN_POINT('Ctrl Pts',(41.5000000000007,-57.6764631965609,
-60.7926167355675));
#169770=CARTESIAN_POINT('Ctrl Pts',(41.5,-57.6641810084401,-61.0874868365943));
#169771=CARTESIAN_POINT('Ctrl Pts',(41.7579337455089,-57.270046180586,-60.6499285183491));
#169772=CARTESIAN_POINT('Ctrl Pts',(41.4999999999994,-57.2759508310879,
-60.7926435723737));
#169773=CARTESIAN_POINT('Ctrl Pts',(41.5,-57.2881262594113,-61.0874286718719));
#169774=CARTESIAN_POINT('Ctrl Pts',(41.7818539242553,-57.0640562802561,
-60.6499294916166));
#169775=CARTESIAN_POINT('Ctrl Pts',(41.5,-57.0692704467339,-60.7883470172518));
#169776=CARTESIAN_POINT('Ctrl Pts',(41.5,-57.0999570266671,-61.1007545617424));
#169777=CARTESIAN_POINT('Ctrl Pts',(41.8680165447744,-56.6807474451004,
-60.6499357558287));
#169778=CARTESIAN_POINT('Ctrl Pts',(41.5,-56.6836417097814,-60.7524277281085));
#169779=CARTESIAN_POINT('Ctrl Pts',(41.5,-56.7235644715484,-61.1324985063765));
#169780=CARTESIAN_POINT('Ctrl Pts',(41.9298158029953,-56.5034783375499,
-60.6499412695179));
#169781=CARTESIAN_POINT('Ctrl Pts',(41.5000000000006,-56.4941497059427,
-60.7159472955962));
#169782=CARTESIAN_POINT('Ctrl Pts',(41.5,-56.5353526996978,-61.1499499536044));
#169783=CARTESIAN_POINT('Ctrl Pts',(42.0000617764046,-56.3473237326805,
-60.6499500038163));
#169784=CARTESIAN_POINT('Ctrl Pts',(41.5,-56.3473237326805,-60.6498882197787));
#169785=CARTESIAN_POINT('Ctrl Pts',(41.5,-56.3473237326805,-61.14995));
#169786=CARTESIAN_POINT('',(42.,-58.6035812240174,-60.64995));
#169787=CARTESIAN_POINT('',(41.5,-58.6035812240174,-61.14995));
#169788=CARTESIAN_POINT('Origin',(42.,-58.6035812240174,-61.14995));
#169789=CARTESIAN_POINT('',(41.5,-56.3473237326805,-61.14995));
#169790=CARTESIAN_POINT('Ctrl Pts',(41.5,-56.3473237326805,-61.14995));
#169791=CARTESIAN_POINT('Ctrl Pts',(41.5,-56.4247882486864,-61.1499499808859));
#169792=CARTESIAN_POINT('Ctrl Pts',(41.5,-56.5020743317104,-61.146992865599));
#169793=CARTESIAN_POINT('Ctrl Pts',(41.5,-56.5792618257267,-61.1424262748502));
#169794=CARTESIAN_POINT('Ctrl Pts',(41.5,-56.6823474618059,-61.1363274900916));
#169795=CARTESIAN_POINT('Ctrl Pts',(41.5,-56.7852572696793,-61.1273561280415));
#169796=CARTESIAN_POINT('Ctrl Pts',(41.5000000000002,-56.8881825068221,
-61.1186215077307));
#169797=CARTESIAN_POINT('Ctrl Pts',(41.5000000000002,-56.8960417889422,
-61.1179545396756));
#169798=CARTESIAN_POINT('Ctrl Pts',(41.5000000000002,-56.9039011612641,
-61.1172889307083));
#169799=CARTESIAN_POINT('Ctrl Pts',(41.5000000000002,-56.9117607090172,
-61.1166260587005));
#169800=CARTESIAN_POINT('Ctrl Pts',(41.5000000000002,-56.9118309970963,
-61.116620130624));
#169801=CARTESIAN_POINT('Ctrl Pts',(41.5000000000002,-56.9119012851879,
-61.1166142029013));
#169802=CARTESIAN_POINT('Ctrl Pts',(41.5000000000002,-56.9119715732919,
-61.1166082755328));
#169803=CARTESIAN_POINT('Ctrl Pts',(41.5000000000007,-57.0997257526663,
-61.1007750386643));
#169804=CARTESIAN_POINT('Ctrl Pts',(41.4999999999977,-57.2880101287523,
-61.0874286525006));
#169805=CARTESIAN_POINT('Ctrl Pts',(41.5000000000023,-57.4761536341596,
-61.0874562423818));
#169806=CARTESIAN_POINT('Ctrl Pts',(41.5000000000023,-57.476328431569,-61.0874562680146));
#169807=CARTESIAN_POINT('Ctrl Pts',(41.5000000000023,-57.4765032288573,
-61.087456305165));
#169808=CARTESIAN_POINT('Ctrl Pts',(41.5000000000023,-57.4766780260241,
-61.0874563538243));
#169809=CARTESIAN_POINT('Ctrl Pts',(41.500000000005,-57.5875579724867,-61.0874872201067));
#169810=CARTESIAN_POINT('Ctrl Pts',(41.5000000000027,-57.6982145368478,
-61.092146664679));
#169811=CARTESIAN_POINT('Ctrl Pts',(41.5000000000012,-57.8087551935517,
-61.0991963488612));
#169812=CARTESIAN_POINT('Ctrl Pts',(41.5000000000001,-57.8858564168504,
-61.1041134471535));
#169813=CARTESIAN_POINT('Ctrl Pts',(41.5,-57.9629012529644,-61.1101948863674));
#169814=CARTESIAN_POINT('Ctrl Pts',(41.5,-58.039926161923,-61.1166923365635));
#169815=CARTESIAN_POINT('Ctrl Pts',(41.5,-58.0400259760021,-61.1167007563983));
#169816=CARTESIAN_POINT('Ctrl Pts',(41.5,-58.0401257900677,-61.1167091766712));
#169817=CARTESIAN_POINT('Ctrl Pts',(41.5,-58.0402256041196,-61.1167175973794));
#169818=CARTESIAN_POINT('Ctrl Pts',(41.5,-58.1358345616343,-61.1247835471794));
#169819=CARTESIAN_POINT('Ctrl Pts',(41.5,-58.2314235934534,-61.1332503625509));
#169820=CARTESIAN_POINT('Ctrl Pts',(41.5,-58.3271142909743,-61.1396237955238));
#169821=CARTESIAN_POINT('Ctrl Pts',(41.5,-58.4115316341054,-61.1452463721392));
#169822=CARTESIAN_POINT('Ctrl Pts',(41.5,-58.4960281098057,-61.1492419515511));
#169823=CARTESIAN_POINT('Ctrl Pts',(41.5,-58.5806871719383,-61.1498651031255));
#169824=CARTESIAN_POINT('Ctrl Pts',(41.5,-58.5883171817128,-61.149921265484));
#169825=CARTESIAN_POINT('Ctrl Pts',(41.5,-58.5959485120592,-61.1499499981887));
#169826=CARTESIAN_POINT('Ctrl Pts',(41.5,-58.6035812240174,-61.14995));
#169827=CARTESIAN_POINT('Origin',(42.,-56.3473237326805,-61.14995));
#169828=CARTESIAN_POINT('Ctrl Pts',(42.,-58.6035812240174,-60.64995));
#169829=CARTESIAN_POINT('Ctrl Pts',(41.9586127577212,-58.5115728992453,
-60.64995));
#169830=CARTESIAN_POINT('Ctrl Pts',(41.9223200866005,-58.4173567491328,
-60.6499639595534));
#169831=CARTESIAN_POINT('Ctrl Pts',(41.8579031946498,-58.2180944893025,
-60.6499671932779));
#169832=CARTESIAN_POINT('Ctrl Pts',(41.8306620008004,-58.1129431414189,
-60.6499312309338));
#169833=CARTESIAN_POINT('Ctrl Pts',(41.7951274186657,-57.9323775711288,
-60.6499828894707));
#169834=CARTESIAN_POINT('Ctrl Pts',(41.7836058362703,-57.8577298063973,
-60.6500200799918));
#169835=CARTESIAN_POINT('Ctrl Pts',(41.763699988371,-57.6806798505208,-60.6500271654877));
#169836=CARTESIAN_POINT('Ctrl Pts',(41.7579524619679,-57.578105462568,-60.6499494618776));
#169837=CARTESIAN_POINT('Ctrl Pts',(41.7579524619679,-57.3728595819392,
-60.6499505378071));
#169838=CARTESIAN_POINT('Ctrl Pts',(41.7636932451376,-57.2703453579393,
-60.6500300767565));
#169839=CARTESIAN_POINT('Ctrl Pts',(41.7835828980495,-57.0933348984408,
-60.6500220919564));
#169840=CARTESIAN_POINT('Ctrl Pts',(41.7951032511139,-57.0186677636549,
-60.6499835586185));
#169841=CARTESIAN_POINT('Ctrl Pts',(41.8306429216694,-56.838033533205,-60.6499306306421));
#169842=CARTESIAN_POINT('Ctrl Pts',(41.857894634129,-56.7328337987607,-60.6499676698703));
#169843=CARTESIAN_POINT('Ctrl Pts',(41.9223259722372,-56.5335329279257,
-60.6499642647307));
#169844=CARTESIAN_POINT('Ctrl Pts',(41.9586161144828,-56.4393245950077,
-60.64995));
#169845=CARTESIAN_POINT('Ctrl Pts',(42.,-56.3473237326805,-60.64995));
#169846=CARTESIAN_POINT('Origin',(42.,-12.9675000200281,-61.14995));
#169847=CARTESIAN_POINT('',(41.5,-73.08000002,-61.14995));
#169848=CARTESIAN_POINT('Origin',(42.5,-55.58000002,-177.34995));
#169849=CARTESIAN_POINT('',(41.5,-55.58000002,-60.64995));
#169850=CARTESIAN_POINT('',(42.5,-54.58000002,-171.64995));
#169851=CARTESIAN_POINT('Origin',(42.,-73.08000002,-171.14995));
#169852=CARTESIAN_POINT('',(41.5,-56.3473237326807,-171.14995));
#169853=CARTESIAN_POINT('',(42.,-56.3473237326807,-171.64995));
#169854=CARTESIAN_POINT('Origin',(42.,-56.3473237326807,-171.14995));
#169855=CARTESIAN_POINT('',(42.,-62.3323045260081,-171.64995));
#169856=CARTESIAN_POINT('',(41.5,-55.58000002,-171.14995));
#169857=CARTESIAN_POINT('Origin',(41.,-70.08000002,-58.24995));
#169858=CARTESIAN_POINT('',(41.5,-70.08000002,-55.74995));
#169859=CARTESIAN_POINT('',(41.,-70.08000002,-55.24995));
#169860=CARTESIAN_POINT('Origin',(41.,-70.08000002,-55.74995));
#169861=CARTESIAN_POINT('Origin',(41.,-70.08000002,-58.24995));
#169862=CARTESIAN_POINT('Origin',(41.5,-70.08000002,-58.24995));
#169863=CARTESIAN_POINT('Origin',(-3.3975957231091E-14,-70.08000002,-58.24995));
#169864=CARTESIAN_POINT('',(40.5,-70.08000002,-55.24995));
#169865=CARTESIAN_POINT('',(41.5,-70.08000002,-55.24995));
#169866=CARTESIAN_POINT('Origin',(40.5,-70.08000002,-58.24995));
#169867=CARTESIAN_POINT('Origin',(39.5,67.7009572055632,-171.14995));
#169868=CARTESIAN_POINT('',(40.,-56.978215522411,-171.14995));
#169869=CARTESIAN_POINT('Origin',(39.5,-56.978215522411,-171.14995));
#169870=CARTESIAN_POINT('',(40.,-62.6133861954129,-171.14995));
#169871=CARTESIAN_POINT('Origin',(39.5,-62.6133861954129,-171.14995));
#169872=CARTESIAN_POINT('',(40.,-62.5431157780617,-171.14995));
#169873=CARTESIAN_POINT('Ctrl Pts',(39.5,-56.978215522411,-171.64995));
#169874=CARTESIAN_POINT('Ctrl Pts',(40.,-56.9782155224109,-171.64995));
#169875=CARTESIAN_POINT('Ctrl Pts',(40.,-56.978215522411,-171.14995));
#169876=CARTESIAN_POINT('Ctrl Pts',(39.4660557514084,-56.8721092179034,
-171.64995));
#169877=CARTESIAN_POINT('Ctrl Pts',(40.,-56.8683451300554,-171.685098426659));
#169878=CARTESIAN_POINT('Ctrl Pts',(40.,-56.9099188320733,-171.149949989769));
#169879=CARTESIAN_POINT('Ctrl Pts',(39.4324273161011,-56.7672721138937,
-171.634782634301));
#169880=CARTESIAN_POINT('Ctrl Pts',(40.0000000000047,-56.7549311731639,
-171.710009011284));
#169881=CARTESIAN_POINT('Ctrl Pts',(40.,-56.8423993478631,-171.142369716128));
#169882=CARTESIAN_POINT('Ctrl Pts',(39.399271366643,-56.6641713142698,-171.60362375617));
#169883=CARTESIAN_POINT('Ctrl Pts',(40.,-56.6359876224365,-171.723920704752));
#169884=CARTESIAN_POINT('Ctrl Pts',(40.,-56.7758867300387,-171.126786878085));
#169885=CARTESIAN_POINT('',(40.,-56.7758867300388,-171.126786878085));
#169886=CARTESIAN_POINT('Origin',(39.5,-56.7758867300388,-171.126786878085));
#169887=CARTESIAN_POINT('Ctrl Pts',(40.,-56.7758867300388,-171.126786878085));
#169888=CARTESIAN_POINT('Ctrl Pts',(40.,-56.8424288281835,-171.142376649979));
#169889=CARTESIAN_POINT('Ctrl Pts',(40.,-56.909888666977,-171.14995));
#169890=CARTESIAN_POINT('Ctrl Pts',(40.,-56.978215522411,-171.14995));
#169891=CARTESIAN_POINT('Ctrl Pts',(40.,-56.3715344108516,-170.85018387548));
#169892=CARTESIAN_POINT('Ctrl Pts',(39.9999999999999,-55.5316163075193,
-171.321942247435));
#169893=CARTESIAN_POINT('Ctrl Pts',(39.2122207971108,-56.0150382320575,
-171.05041775096));
#169894=CARTESIAN_POINT('Ctrl Pts',(40.,-56.4127345596313,-170.923536275602));
#169895=CARTESIAN_POINT('Ctrl Pts',(40.0000000000016,-55.7019737694774,
-171.520946951432));
#169896=CARTESIAN_POINT('Ctrl Pts',(39.2305303132587,-56.0826793050571,
-171.197160563313));
#169897=CARTESIAN_POINT('Ctrl Pts',(40.,-56.4743979142815,-170.984396086855));
#169898=CARTESIAN_POINT('Ctrl Pts',(40.0000000000015,-55.9148019306841,
-171.629811017638));
#169899=CARTESIAN_POINT('Ctrl Pts',(39.2581734308863,-56.1834313742016,
-171.318842218969));
#169900=CARTESIAN_POINT('Ctrl Pts',(40.,-56.6150166715838,-171.07608877299));
#169901=CARTESIAN_POINT('Ctrl Pts',(39.9999999999985,-56.2996107654989,
-171.733927689933));
#169902=CARTESIAN_POINT('Ctrl Pts',(39.3228477027581,-56.4100322256565,
-171.502227500722));
#169903=CARTESIAN_POINT('Ctrl Pts',(40.,-56.6951614830789,-171.107874245193));
#169904=CARTESIAN_POINT('Ctrl Pts',(39.9999999999952,-56.4773256662664,
-171.740119136472));
#169905=CARTESIAN_POINT('Ctrl Pts',(39.3604560080182,-56.5377771955238,
-171.565812105304));
#169906=CARTESIAN_POINT('Ctrl Pts',(40.,-56.7758867300388,-171.126786878085));
#169907=CARTESIAN_POINT('Ctrl Pts',(40.,-56.6359876224367,-171.723920704753));
#169908=CARTESIAN_POINT('Ctrl Pts',(39.399271366643,-56.6641713142699,-171.60362375617));
#169909=CARTESIAN_POINT('',(40.,-56.3715344108516,-170.85018387548));
#169910=CARTESIAN_POINT('Origin',(39.5,-56.3715344108516,-170.85018387548));
#169911=CARTESIAN_POINT('Ctrl Pts',(40.,-56.3715344108516,-170.85018387548));
#169912=CARTESIAN_POINT('Ctrl Pts',(40.,-56.3837583326097,-170.871947332768));
#169913=CARTESIAN_POINT('Ctrl Pts',(40.,-56.3977040563911,-170.892479579619));
#169914=CARTESIAN_POINT('Ctrl Pts',(39.9999999999999,-56.4130583083892,
-170.911803741317));
#169915=CARTESIAN_POINT('Ctrl Pts',(39.9999999999997,-56.4292409786972,
-170.93217051254));
#169916=CARTESIAN_POINT('Ctrl Pts',(39.9999999999994,-56.4469891868553,
-170.951195798844));
#169917=CARTESIAN_POINT('Ctrl Pts',(39.9999999999991,-56.4659895184394,
-170.968879578562));
#169918=CARTESIAN_POINT('Ctrl Pts',(39.9999999999989,-56.4862759122394,
-170.987760307967));
#169919=CARTESIAN_POINT('Ctrl Pts',(39.9999999999988,-56.5079910115911,
-171.005112575639));
#169920=CARTESIAN_POINT('Ctrl Pts',(39.9999999999991,-56.5307948409885,
-171.020896071163));
#169921=CARTESIAN_POINT('Ctrl Pts',(39.9999999999992,-56.5352406042452,
-171.023973172086));
#169922=CARTESIAN_POINT('Ctrl Pts',(39.9999999999993,-56.5397278285598,
-171.026990509393));
#169923=CARTESIAN_POINT('Ctrl Pts',(39.9999999999994,-56.5442540887154,
-171.029947579459));
#169924=CARTESIAN_POINT('Ctrl Pts',(39.9999999999994,-56.5444049748233,
-171.030046155496));
#169925=CARTESIAN_POINT('Ctrl Pts',(39.9999999999994,-56.5445558983641,
-171.030144660686));
#169926=CARTESIAN_POINT('Ctrl Pts',(39.9999999999994,-56.5447068592425,
-171.030243095025));
#169927=CARTESIAN_POINT('Ctrl Pts',(39.9999999999998,-56.5677583970533,
-171.045273895852));
#169928=CARTESIAN_POINT('Ctrl Pts',(39.9999999999999,-56.5918056322569,
-171.058759052615));
#169929=CARTESIAN_POINT('Ctrl Pts',(40.,-56.616614889125,-171.070798762234));
#169930=CARTESIAN_POINT('Ctrl Pts',(40.,-56.6425070267789,-171.083363984176));
#169931=CARTESIAN_POINT('Ctrl Pts',(40.,-56.6692310020633,-171.094354961296));
#169932=CARTESIAN_POINT('Ctrl Pts',(40.,-56.6965412231968,-171.103832593435));
#169933=CARTESIAN_POINT('Ctrl Pts',(40.,-56.7225306079875,-171.112851847704));
#169934=CARTESIAN_POINT('Ctrl Pts',(40.,-56.7490526547637,-171.120500083882));
#169935=CARTESIAN_POINT('Ctrl Pts',(40.,-56.7758867300388,-171.126786878085));
#169936=CARTESIAN_POINT('Ctrl Pts',(39.2122207971107,-56.0150382320573,
-171.05041775096));
#169937=CARTESIAN_POINT('Ctrl Pts',(40.,-55.5316163075182,-171.321942247434));
#169938=CARTESIAN_POINT('Ctrl Pts',(40.,-56.3715344108516,-170.85018387548));
#169939=CARTESIAN_POINT('Ctrl Pts',(39.2341040930243,-55.7557644506258,
-170.620257995618));
#169940=CARTESIAN_POINT('Ctrl Pts',(39.999999999956,-55.3341015490071,-170.847929211526));
#169941=CARTESIAN_POINT('Ctrl Pts',(40.,-56.1381771304993,-170.434714809241));
#169942=CARTESIAN_POINT('Ctrl Pts',(39.2567881498609,-55.5425920931993,
-170.174365095598));
#169943=CARTESIAN_POINT('Ctrl Pts',(39.9999999999967,-55.1686346470297,
-170.352236872778));
#169944=CARTESIAN_POINT('Ctrl Pts',(40.,-55.946332886798,-170.004198915545));
#169945=CARTESIAN_POINT('Ctrl Pts',(39.3033074404025,-55.1837352900438,
-169.25987708718));
#169946=CARTESIAN_POINT('Ctrl Pts',(40.0000000000031,-54.9062023418216,
-169.365343244152));
#169947=CARTESIAN_POINT('Ctrl Pts',(40.,-55.6233617621208,-169.121472747772));
#169948=CARTESIAN_POINT('Ctrl Pts',(39.3271543017018,-55.0384654852052,
-168.791053495007));
#169949=CARTESIAN_POINT('Ctrl Pts',(39.9999999999966,-54.803396468199,-168.870754981701));
#169950=CARTESIAN_POINT('Ctrl Pts',(40.,-55.4926189390281,-168.669060842998));
#169951=CARTESIAN_POINT('Ctrl Pts',(39.3758587707466,-54.8068569180214,
-167.833341194373));
#169952=CARTESIAN_POINT('Ctrl Pts',(40.0000000000032,-54.6536169628087,
-167.876849546978));
#169953=CARTESIAN_POINT('Ctrl Pts',(40.,-55.2841712278759,-167.745175405929));
#169954=CARTESIAN_POINT('Ctrl Pts',(39.4005707712209,-54.7215461590296,
-167.347314197405));
#169955=CARTESIAN_POINT('Ctrl Pts',(39.9999999999983,-54.6033362561509,
-167.378205061485));
#169956=CARTESIAN_POINT('Ctrl Pts',(40.,-55.2073915453443,-167.276463616742));
#169957=CARTESIAN_POINT('Ctrl Pts',(39.4500853482271,-54.6083104675451,
-166.373147921324));
#169958=CARTESIAN_POINT('Ctrl Pts',(40.0000000000016,-54.5553362422517,
-166.389752651669));
#169959=CARTESIAN_POINT('Ctrl Pts',(40.,-55.1054794225729,-166.337325121725));
#169960=CARTESIAN_POINT('Ctrl Pts',(39.4749775493875,-54.58000002,-165.883246469104));
#169961=CARTESIAN_POINT('Ctrl Pts',(40.,-54.5543340703016,-165.895917381598));
#169962=CARTESIAN_POINT('Ctrl Pts',(40.,-55.0800000204413,-165.865198337359));
#169963=CARTESIAN_POINT('Ctrl Pts',(39.5,-54.58000002,-165.390538702986));
#169964=CARTESIAN_POINT('Ctrl Pts',(40.,-54.58000002,-165.390538702985));
#169965=CARTESIAN_POINT('Ctrl Pts',(40.,-55.08000002,-165.390538702986));
#169966=CARTESIAN_POINT('',(40.,-55.08000002,-165.390538702986));
#169967=CARTESIAN_POINT('Origin',(39.5,-55.08000002,-165.390538702986));
#169968=CARTESIAN_POINT('Ctrl Pts',(40.,-55.08000002,-165.390538702986));
#169969=CARTESIAN_POINT('Ctrl Pts',(40.,-55.08000002,-165.865206657822));
#169970=CARTESIAN_POINT('Ctrl Pts',(40.,-55.1054794225748,-166.33732512172));
#169971=CARTESIAN_POINT('Ctrl Pts',(40.,-55.1564354838472,-166.806894369245));
#169972=CARTESIAN_POINT('Ctrl Pts',(40.,-55.2073915451197,-167.27646361677));
#169973=CARTESIAN_POINT('Ctrl Pts',(40.,-55.2841712278673,-167.745175405874));
#169974=CARTESIAN_POINT('Ctrl Pts',(40.,-55.3883950832632,-168.207118124506));
#169975=CARTESIAN_POINT('Ctrl Pts',(40.,-55.4926189386592,-168.669060843138));
#169976=CARTESIAN_POINT('Ctrl Pts',(40.,-55.6233617621227,-169.121472747749));
#169977=CARTESIAN_POINT('Ctrl Pts',(40.,-55.7848473238897,-169.562835831867));
#169978=CARTESIAN_POINT('Ctrl Pts',(40.,-55.9143897222853,-169.916893692237));
#169979=CARTESIAN_POINT('Ctrl Pts',(40.,-56.0634514912202,-170.263936360661));
#169980=CARTESIAN_POINT('Ctrl Pts',(40.,-56.2378305483017,-170.601880104207));
#169981=CARTESIAN_POINT('Ctrl Pts',(40.,-56.280829742217,-170.685211834545));
#169982=CARTESIAN_POINT('Ctrl Pts',(40.,-56.325368553705,-170.767990232551));
#169983=CARTESIAN_POINT('Ctrl Pts',(40.,-56.3715344108516,-170.85018387548));
#169984=CARTESIAN_POINT('Origin',(39.5,-55.08000002,-55.24995));
#169985=CARTESIAN_POINT('',(40.,-55.08000002,-66.6681042685293));
#169986=CARTESIAN_POINT('',(40.,-55.08000002,-166.086292363451));
#169987=CARTESIAN_POINT('Origin',(39.5,-55.08000002,-66.6681042685293));
#169988=CARTESIAN_POINT('Ctrl Pts',(39.5,-54.58000002,-66.6681042685296));
#169989=CARTESIAN_POINT('Ctrl Pts',(39.9999999999999,-54.5800000200005,
-66.6681042685296));
#169990=CARTESIAN_POINT('Ctrl Pts',(40.,-55.08000002,-66.6681042685293));
#169991=CARTESIAN_POINT('Ctrl Pts',(39.4524759569592,-54.5800000199993,
-65.7323260169345));
#169992=CARTESIAN_POINT('Ctrl Pts',(40.000000000023,-54.5300790303385,-65.6851286065597));
#169993=CARTESIAN_POINT('Ctrl Pts',(40.,-55.0800000210321,-65.7666038778627));
#169994=CARTESIAN_POINT('Ctrl Pts',(39.4055862633018,-54.6797418208431,
-64.8099001089231));
#169995=CARTESIAN_POINT('Ctrl Pts',(40.,-54.5798306201335,-64.744699921287));
#169996=CARTESIAN_POINT('Ctrl Pts',(40.,-55.1697676396346,-64.8773517277477));
#169997=CARTESIAN_POINT('Ctrl Pts',(39.336341776171,-54.9893440187367,-63.4482326198876));
#169998=CARTESIAN_POINT('Ctrl Pts',(40.,-54.7700293023446,-63.3785482937886));
#169999=CARTESIAN_POINT('Ctrl Pts',(40.,-55.4484096194251,-63.5638700072085));
#170000=CARTESIAN_POINT('Ctrl Pts',(39.3133286552319,-55.1206346051679,
-62.9957806797004));
#170001=CARTESIAN_POINT('Ctrl Pts',(40.,-54.8613740727702,-62.9031901152049));
#170002=CARTESIAN_POINT('Ctrl Pts',(40.,-55.5665711459207,-63.1272943707367));
#170003=CARTESIAN_POINT('Ctrl Pts',(39.2684369452391,-55.4440915465439,
-62.113263414855));
#170004=CARTESIAN_POINT('Ctrl Pts',(40.,-55.0944248813133,-61.958211698159));
#170005=CARTESIAN_POINT('Ctrl Pts',(40.,-55.8576823946199,-62.2755058384848));
#170006=CARTESIAN_POINT('Ctrl Pts',(39.2465526403215,-55.635643675915,-61.6830846593873));
#170007=CARTESIAN_POINT('Ctrl Pts',(39.9999999999954,-55.2406041652953,
-61.4857700511268));
#170008=CARTESIAN_POINT('Ctrl Pts',(40.,-56.0300729172808,-61.8601972461309));
#170009=CARTESIAN_POINT('Ctrl Pts',(39.2253966502057,-55.8655297208508,
-61.2672223984388));
#170010=CARTESIAN_POINT('Ctrl Pts',(39.9999999999999,-55.4129915017042,
-61.0340816633138));
#170011=CARTESIAN_POINT('Ctrl Pts',(40.,-56.2369767507657,-61.4585861992193));
#170012=CARTESIAN_POINT('',(40.,-56.2369767507657,-61.4585861992193));
#170013=CARTESIAN_POINT('Ctrl Pts',(40.,-56.2369767507657,-61.4585861992193));
#170014=CARTESIAN_POINT('Ctrl Pts',(40.,-56.0300621110256,-61.860218211459));
#170015=CARTESIAN_POINT('Ctrl Pts',(40.,-55.8576823937473,-62.2755058381188));
#170016=CARTESIAN_POINT('Ctrl Pts',(40.,-55.7121267698271,-62.7014001044593));
#170017=CARTESIAN_POINT('Ctrl Pts',(40.,-55.566571145907,-63.1272943707998));
#170018=CARTESIAN_POINT('Ctrl Pts',(40.,-55.4484096188021,-63.563870007102));
#170019=CARTESIAN_POINT('Ctrl Pts',(40.,-55.355528959088,-64.0016972473019));
#170020=CARTESIAN_POINT('Ctrl Pts',(40.,-55.2432744366405,-64.5308503337935));
#170021=CARTESIAN_POINT('Ctrl Pts',(40.,-55.1660815895368,-65.0649117752156));
#170022=CARTESIAN_POINT('Ctrl Pts',(40.,-55.1225595401114,-65.6036868919934));
#170023=CARTESIAN_POINT('Ctrl Pts',(40.,-55.0940603190417,-65.9564890086819));
#170024=CARTESIAN_POINT('Ctrl Pts',(40.,-55.0800000199998,-66.3113124768404));
#170025=CARTESIAN_POINT('Ctrl Pts',(40.,-55.08000002,-66.6681042685293));
#170026=CARTESIAN_POINT('Origin',(39.5,-56.2369767507657,-61.4585861992193));
#170027=CARTESIAN_POINT('Ctrl Pts',(39.2250415490953,-55.8657373699498,
-61.2673293760636));
#170028=CARTESIAN_POINT('Ctrl Pts',(40.,-55.4121526631459,-61.0336495065824));
#170029=CARTESIAN_POINT('Ctrl Pts',(40.,-56.2369767507698,-61.4585861992214));
#170030=CARTESIAN_POINT('Ctrl Pts',(39.2367912602697,-55.9110350177183,
-61.1625123459351));
#170031=CARTESIAN_POINT('Ctrl Pts',(39.9999999999999,-55.5203773908674,
-60.8902955679075));
#170032=CARTESIAN_POINT('Ctrl Pts',(40.,-56.2639883391117,-61.4061555156247));
#170033=CARTESIAN_POINT('Ctrl Pts',(39.2526254167108,-55.9715434068114,
-61.0715217947418));
#170034=CARTESIAN_POINT('Ctrl Pts',(40.0000000000002,-55.6518298350008,
-60.7886660066872));
#170035=CARTESIAN_POINT('Ctrl Pts',(40.,-56.3001438773882,-61.3606672793622));
#170036=CARTESIAN_POINT('Ctrl Pts',(39.2913939492583,-56.1161109922439,
-60.9128192370848));
#170037=CARTESIAN_POINT('Ctrl Pts',(39.9999999999997,-55.923525557992,-60.6494230275178));
#170038=CARTESIAN_POINT('Ctrl Pts',(40.,-56.3871674054812,-61.2813159675772));
#170039=CARTESIAN_POINT('Ctrl Pts',(39.3134274873215,-56.1967830839396,
-60.8489419701753));
#170040=CARTESIAN_POINT('Ctrl Pts',(40.0000000000002,-56.055303527311,-60.6118369663638));
#170041=CARTESIAN_POINT('Ctrl Pts',(40.,-56.4359944422203,-61.2493819347541));
#170042=CARTESIAN_POINT('Ctrl Pts',(39.3621229995535,-56.3701234141287,
-60.7467866067772));
#170043=CARTESIAN_POINT('Ctrl Pts',(39.9999999999998,-56.3052253871045,
-60.5760036964908));
#170044=CARTESIAN_POINT('Ctrl Pts',(40.,-56.5418574657904,-61.1983186977834));
#170045=CARTESIAN_POINT('Ctrl Pts',(39.3878798646771,-56.459572422833,-60.710431798962));
#170046=CARTESIAN_POINT('Ctrl Pts',(40.0000000000002,-56.4197432892716,
-60.5759049037901));
#170047=CARTESIAN_POINT('Ctrl Pts',(40.,-56.5969271200065,-61.1801504966336));
#170048=CARTESIAN_POINT('Ctrl Pts',(39.4420692078983,-56.6422525387301,
-60.6618822224814));
#170049=CARTESIAN_POINT('Ctrl Pts',(39.9999999999997,-56.6329760211049,
-60.5982183614686));
#170050=CARTESIAN_POINT('Ctrl Pts',(40.,-56.7105746147406,-61.1558957215692));
#170051=CARTESIAN_POINT('Ctrl Pts',(39.4706843681677,-56.7360270779361,
-60.6499699008789));
#170052=CARTESIAN_POINT('Ctrl Pts',(40.,-56.7332871432547,-60.6197584771857));
#170053=CARTESIAN_POINT('Ctrl Pts',(40.,-56.769502228095,-61.1499499952173));
#170054=CARTESIAN_POINT('Ctrl Pts',(39.4996584737974,-56.8280459100727,
-60.6499501166402));
#170055=CARTESIAN_POINT('Ctrl Pts',(40.,-56.8280459100727,-60.6496083570775));
#170056=CARTESIAN_POINT('Ctrl Pts',(40.,-56.8280459100727,-61.14995));
#170057=CARTESIAN_POINT('',(40.,-56.8280459100727,-61.14995));
#170058=CARTESIAN_POINT('Ctrl Pts',(40.,-56.8280459100727,-61.14995));
#170059=CARTESIAN_POINT('Ctrl Pts',(40.,-56.7775257469882,-61.1499499958728));
#170060=CARTESIAN_POINT('Ctrl Pts',(40.,-56.7268325166741,-61.15437366761));
#170061=CARTESIAN_POINT('Ctrl Pts',(40.,-56.6774814901229,-61.1633382145163));
#170062=CARTESIAN_POINT('Ctrl Pts',(40.,-56.6695344165968,-61.1647817896225));
#170063=CARTESIAN_POINT('Ctrl Pts',(40.,-56.6616221088455,-61.1663432172134));
#170064=CARTESIAN_POINT('Ctrl Pts',(40.,-56.6537508667182,-61.1680231060305));
#170065=CARTESIAN_POINT('Ctrl Pts',(40.,-56.6068413991698,-61.1780345741922));
#170066=CARTESIAN_POINT('Ctrl Pts',(40.,-56.5611509800564,-61.1921536886351));
#170067=CARTESIAN_POINT('Ctrl Pts',(40.,-56.5168370445334,-61.2111466189142));
#170068=CARTESIAN_POINT('Ctrl Pts',(40.,-56.5074712818004,-61.2151607800691));
#170069=CARTESIAN_POINT('Ctrl Pts',(40.,-56.4981670562378,-61.2193928254492));
#170070=CARTESIAN_POINT('Ctrl Pts',(40.,-56.4889259423713,-61.2238502921498));
#170071=CARTESIAN_POINT('Ctrl Pts',(40.,-56.4359851254178,-61.2493863835865));
#170072=CARTESIAN_POINT('Ctrl Pts',(40.,-56.3871673636495,-61.2813158980448));
#170073=CARTESIAN_POINT('Ctrl Pts',(40.,-56.3436555786936,-61.3209915546623));
#170074=CARTESIAN_POINT('Ctrl Pts',(40.,-56.3001590827628,-61.3606532701805));
#170075=CARTESIAN_POINT('Ctrl Pts',(40.,-56.2640024859216,-61.4061278501816));
#170076=CARTESIAN_POINT('Ctrl Pts',(40.,-56.2369767507657,-61.4585861992193));
#170077=CARTESIAN_POINT('',(39.4999994911522,-56.8280450701521,-60.6499500000002));
#170078=CARTESIAN_POINT('Origin',(39.5,-56.8280459100727,-61.14995));
#170079=CARTESIAN_POINT('Ctrl Pts',(39.2253966502054,-55.865529720851,-61.2672223984388));
#170080=CARTESIAN_POINT('Ctrl Pts',(39.234911163723,-55.9022177765805,-61.1823557659019));
#170081=CARTESIAN_POINT('Ctrl Pts',(39.2479974736944,-55.9538728824452,
-61.0971743824038));
#170082=CARTESIAN_POINT('Ctrl Pts',(39.2746238713045,-56.0536593475906,
-60.9796220178071));
#170083=CARTESIAN_POINT('Ctrl Pts',(39.2846341785973,-56.0905800623539,
-60.942170208689));
#170084=CARTESIAN_POINT('Ctrl Pts',(39.3012162205084,-56.1508612956915,
-60.8899544631596));
#170085=CARTESIAN_POINT('Ctrl Pts',(39.3070019925557,-56.1717675923896,
-60.8732084043496));
#170086=CARTESIAN_POINT('Ctrl Pts',(39.3160276366305,-56.2042376975661,
-60.8492301021309));
#170087=CARTESIAN_POINT('Ctrl Pts',(39.3206269620396,-56.220750075716,-60.8375258888386));
#170088=CARTESIAN_POINT('Ctrl Pts',(39.3253463010804,-56.2376553063615,
-60.8262748915364));
#170089=CARTESIAN_POINT('Ctrl Pts',(39.3285179752611,-56.2490100114614,
-60.8188775954966));
#170090=CARTESIAN_POINT('Ctrl Pts',(39.3303914962528,-56.2557130146439,
-60.8146171211701));
#170091=CARTESIAN_POINT('Ctrl Pts',(39.3424129108038,-56.2987074019437,
-60.7877930361237));
#170092=CARTESIAN_POINT('Ctrl Pts',(39.3542789664704,-56.340825775592,-60.7649606346162));
#170093=CARTESIAN_POINT('Ctrl Pts',(39.3739744074941,-56.4094606619384,
-60.7340965930491));
#170094=CARTESIAN_POINT('Ctrl Pts',(39.3808520215394,-56.4332428662801,
-60.7243742045393));
#170095=CARTESIAN_POINT('Ctrl Pts',(39.3916159549907,-56.4701691837868,
-60.7108731089427));
#170096=CARTESIAN_POINT('Ctrl Pts',(39.3971093785701,-56.4889450165438,
-60.704393079611));
#170097=CARTESIAN_POINT('Ctrl Pts',(39.4037042050758,-56.5113687814886,
-60.69735570514));
#170098=CARTESIAN_POINT('Ctrl Pts',(39.4065690926056,-56.5210866631315,
-60.6944567729941));
#170099=CARTESIAN_POINT('Ctrl Pts',(39.4084874292263,-56.5275887919521,
-60.692550727735));
#170100=CARTESIAN_POINT('Ctrl Pts',(39.4099873539432,-56.5326675243218,
-60.6910973649265));
#170101=CARTESIAN_POINT('Ctrl Pts',(39.4242087195643,-56.5807982407849,
-60.6774835249891));
#170102=CARTESIAN_POINT('Ctrl Pts',(39.4543205885197,-56.6829255755301,
-60.6499501150941));
#170103=CARTESIAN_POINT('Ctrl Pts',(39.4999997135809,-56.8280450001391,
-60.6499500000004));
#170104=CARTESIAN_POINT('Origin',(40.5,-70.08000002,-58.24995));
#170105=CARTESIAN_POINT('',(40.,-70.08000002,-55.74995));
#170106=CARTESIAN_POINT('Origin',(40.5,-70.08000002,-55.74995));
#170107=CARTESIAN_POINT('',(40.,-72.58000002,-58.24995));
#170108=CARTESIAN_POINT('Origin',(40.,-70.08000002,-58.24995));
#170109=CARTESIAN_POINT('Origin',(40.5,-72.58000002,-58.24995));
#170110=CARTESIAN_POINT('Origin',(40.5,-72.58000002,-55.24995));
#170111=CARTESIAN_POINT('',(40.,-72.58000002,-174.34995));
#170112=CARTESIAN_POINT('',(40.,-72.58000002,-58.24995));
#170113=CARTESIAN_POINT('Origin',(40.5,-72.58000002,-174.34995));
#170114=CARTESIAN_POINT('Origin',(40.5,-70.08000002,-174.34995));
#170115=CARTESIAN_POINT('',(40.,-70.08000002,-176.84995));
#170116=CARTESIAN_POINT('Origin',(40.,-70.08000002,-174.34995));
#170117=CARTESIAN_POINT('Origin',(40.5,-70.08000002,-176.84995));
#170118=CARTESIAN_POINT('Origin',(40.5,67.7009572055632,-176.84995));
#170119=CARTESIAN_POINT('',(40.,67.7009572055632,-176.84995));
#170120=CARTESIAN_POINT('Origin',(39.5,-64.1281275541909,-55.24995));
#170121=CARTESIAN_POINT('',(39.5,-63.6281275541908,-172.64995));
#170122=CARTESIAN_POINT('Origin',(39.5,-64.1281275541908,-172.64995));
#170123=CARTESIAN_POINT('',(39.43041344952,-63.63299351982,-171.64995));
#170124=CARTESIAN_POINT('',(40.,-64.1281275541908,-172.64995));
#170125=CARTESIAN_POINT('',(40.,-64.1281275541909,-55.24995));
#170126=CARTESIAN_POINT('Origin',(39.5,-64.1281275541908,-172.64995));
#170127=CARTESIAN_POINT('Ctrl Pts',(40.,-62.6131847515953,-171.149950013428));
#170128=CARTESIAN_POINT('Ctrl Pts',(40.,-62.6132505449146,-171.65003477338));
#170129=CARTESIAN_POINT('Ctrl Pts',(39.4999152383759,-62.6132505989472,
-171.649950001854));
#170130=CARTESIAN_POINT('Ctrl Pts',(40.,-62.8115669184518,-171.149923566191));
#170131=CARTESIAN_POINT('Ctrl Pts',(40.,-62.7480692875133,-171.659221103016));
#170132=CARTESIAN_POINT('Ctrl Pts',(39.4908008078197,-62.7467859681038,
-171.649930655763));
#170133=CARTESIAN_POINT('Ctrl Pts',(40.,-63.0098045293616,-171.188965548735));
#170134=CARTESIAN_POINT('Ctrl Pts',(40.,-62.8774949048455,-171.695281914067));
#170135=CARTESIAN_POINT('Ctrl Pts',(39.4816930631427,-62.8802250152049,
-171.675956808334));
#170136=CARTESIAN_POINT('Ctrl Pts',(40.,-63.3762386807026,-171.339270411997));
#170137=CARTESIAN_POINT('Ctrl Pts',(40.0000000000001,-63.1102859043402,
-171.81002165518));
#170138=CARTESIAN_POINT('Ctrl Pts',(39.4648578735174,-63.1268827917894,
-171.776157476855));
#170139=CARTESIAN_POINT('Ctrl Pts',(40.,-63.5442655393439,-171.450449746589));
#170140=CARTESIAN_POINT('Ctrl Pts',(40.000000000002,-63.2128473094945,-171.889069508911));
#170141=CARTESIAN_POINT('Ctrl Pts',(39.4571382160676,-63.2399874126731,
-171.850276197781));
#170142=CARTESIAN_POINT('Ctrl Pts',(40.,-63.8246746245531,-171.728129909852));
#170143=CARTESIAN_POINT('Ctrl Pts',(39.9999999999979,-63.3804806514191,
-172.075284894372));
#170144=CARTESIAN_POINT('Ctrl Pts',(39.4442554477382,-63.428740903488,-172.035396209826));
#170145=CARTESIAN_POINT('Ctrl Pts',(40.,-63.9369465821947,-171.894521542842));
#170146=CARTESIAN_POINT('Ctrl Pts',(40.,-63.4447415656143,-172.182240159753));
#170147=CARTESIAN_POINT('Ctrl Pts',(39.4390973897632,-63.5043156888,-172.14632470545));
#170148=CARTESIAN_POINT('Ctrl Pts',(40.,-64.0887285772422,-172.257389581842));
#170149=CARTESIAN_POINT('Ctrl Pts',(40.,-63.5311756375845,-172.409795949395));
#170150=CARTESIAN_POINT('Ctrl Pts',(39.4321241606571,-63.6064863141587,
-172.388239289312));
#170151=CARTESIAN_POINT('Ctrl Pts',(40.,-64.1281542477849,-172.453697958273));
#170152=CARTESIAN_POINT('Ctrl Pts',(40.,-63.5528414676591,-172.529747068593));
#170153=CARTESIAN_POINT('Ctrl Pts',(39.4303128569903,-63.6330254636236,
-172.519113452117));
#170154=CARTESIAN_POINT('Ctrl Pts',(40.,-64.1281275406312,-172.65014948338));
#170155=CARTESIAN_POINT('Ctrl Pts',(40.,-63.5528267611457,-172.650072180543));
#170156=CARTESIAN_POINT('Ctrl Pts',(39.4303140827877,-63.6330074860316,
-172.650082990804));
#170157=CARTESIAN_POINT('Ctrl Pts',(40.,-62.6133861954129,-171.14995));
#170158=CARTESIAN_POINT('Ctrl Pts',(40.,-62.8117011147884,-171.149950000016));
#170159=CARTESIAN_POINT('Ctrl Pts',(40.,-63.0098665547682,-171.18899099047));
#170160=CARTESIAN_POINT('Ctrl Pts',(40.,-63.3762386807026,-171.339270411997));
#170161=CARTESIAN_POINT('Ctrl Pts',(40.,-63.5442655393439,-171.450449746589));
#170162=CARTESIAN_POINT('Ctrl Pts',(40.,-63.8246746245531,-171.728129909852));
#170163=CARTESIAN_POINT('Ctrl Pts',(40.,-63.9369465821947,-171.894521542842));
#170164=CARTESIAN_POINT('Ctrl Pts',(40.,-64.0887028854776,-172.257328160063));
#170165=CARTESIAN_POINT('Ctrl Pts',(40.,-64.1281275541786,-172.453565067926));
#170166=CARTESIAN_POINT('Ctrl Pts',(40.,-64.1281275541908,-172.64995));
#170167=CARTESIAN_POINT('Origin',(0.,-12.9675000200281,-61.64995));
#170168=CARTESIAN_POINT('',(39.4379155619868,-56.882767417621,-60.64995));
#170169=CARTESIAN_POINT('Origin',(0.,-12.9675000200281,-60.64995));
#170170=CARTESIAN_POINT('Origin',(39.4379155619868,-56.882767417621,-61.64995));
#170171=CARTESIAN_POINT('Origin',(33.85,67.7009572055632,-61.14995));
#170172=CARTESIAN_POINT('',(33.85,-64.1339197616649,-60.64995));
#170173=CARTESIAN_POINT('',(33.85,-12.9675000200281,-60.64995));
#170174=CARTESIAN_POINT('',(33.35,-64.133919761665,-61.14995));
#170175=CARTESIAN_POINT('Origin',(33.85,-64.133919761665,-61.14995));
#170176=CARTESIAN_POINT('',(33.35,67.7009572055632,-61.14995));
#170177=CARTESIAN_POINT('Origin',(39.5,-12.9675000200281,-61.14995));
#170178=CARTESIAN_POINT('',(40.,-63.6396088127436,-61.14995));
#170179=CARTESIAN_POINT('',(40.,67.7009572055632,-61.14995));
#170180=CARTESIAN_POINT('',(39.5,-63.6396088127436,-60.64995));
#170181=CARTESIAN_POINT('Origin',(39.5,-63.6396088127436,-61.14995));
#170182=CARTESIAN_POINT('',(39.5,-12.9675000200281,-60.64995));
#170183=CARTESIAN_POINT('Ctrl Pts',(39.4379155619868,-56.882767417621,-60.64995));
#170184=CARTESIAN_POINT('Ctrl Pts',(39.0122500629964,-56.4087764892537,
-60.6499500000001));
#170185=CARTESIAN_POINT('Ctrl Pts',(38.8323560497301,-56.2084592670262,
-61.2273317382593));
#170186=CARTESIAN_POINT('Ctrl Pts',(39.5470561894999,-56.7847541538272,
-60.64995));
#170187=CARTESIAN_POINT('Ctrl Pts',(39.1308890120013,-56.2886813392436,
-60.64995));
#170188=CARTESIAN_POINT('Ctrl Pts',(38.9597499727218,-56.0859430057577,
-61.2402727589806));
#170189=CARTESIAN_POINT('Ctrl Pts',(39.6600993514669,-56.6929757051825,
-60.64995));
#170190=CARTESIAN_POINT('Ctrl Pts',(39.2535572856597,-56.1757390223779,
-60.64995));
#170191=CARTESIAN_POINT('Ctrl Pts',(39.0917129041016,-55.9712198429402,
-61.2536666704059));
#170192=CARTESIAN_POINT('Ctrl Pts',(39.7766890844069,-56.606882728875,-60.64995));
#170193=CARTESIAN_POINT('Ctrl Pts',(39.3796800351166,-56.0692409848678,
-60.64995));
#170194=CARTESIAN_POINT('Ctrl Pts',(39.2278317447683,-55.8636034060938,
-61.2674693219905));
#170195=CARTESIAN_POINT('Ctrl Pts',(39.4379155619868,-56.882767417621,-60.64995));
#170196=CARTESIAN_POINT('Ctrl Pts',(39.4584539679692,-56.8643229911399,
-60.64995));
#170197=CARTESIAN_POINT('Ctrl Pts',(39.4791489724441,-56.8460828416128,
-60.64995));
#170198=CARTESIAN_POINT('Ctrl Pts',(39.4999988314732,-56.8280445593217,
-60.64995));
#170199=CARTESIAN_POINT('Ctrl Pts',(40.4577925858907,10.61999998,-144.90822241383));
#170200=CARTESIAN_POINT('Ctrl Pts',(39.7432392475336,10.61999998,-145.291860254625));
#170201=CARTESIAN_POINT('Ctrl Pts',(40.064213984323,9.8954018152728,-145.1195315447));
#170202=CARTESIAN_POINT('Ctrl Pts',(42.7973905232547,10.61999998,-149.265893474329));
#170203=CARTESIAN_POINT('Ctrl Pts',(42.0569998298599,10.61999998,-149.560052788611));
#170204=CARTESIAN_POINT('Ctrl Pts',(42.3982233528881,9.90519935947367,-149.477207192598));
#170205=CARTESIAN_POINT('Ctrl Pts',(45.0988060523808,10.61999998,-153.643419067924));
#170206=CARTESIAN_POINT('Ctrl Pts',(44.3825306854435,10.6199999800261,-153.946076900384));
#170207=CARTESIAN_POINT('Ctrl Pts',(44.6952062210366,9.91377387366803,-153.854728198786));
#170208=CARTESIAN_POINT('Ctrl Pts',(49.6533413888222,10.61999998,-162.423562369795));
#170209=CARTESIAN_POINT('Ctrl Pts',(48.9599089008669,10.6199999799746,-162.709726895544));
#170210=CARTESIAN_POINT('Ctrl Pts',(49.2422260788803,9.92919580612355,-162.634871500674));
#170211=CARTESIAN_POINT('Ctrl Pts',(51.9061633492443,10.61999998,-166.826341244199));
#170212=CARTESIAN_POINT('Ctrl Pts',(51.2291869847762,10.6199999797401,-167.117625919029));
#170213=CARTESIAN_POINT('Ctrl Pts',(51.491975374397,9.936039246645,-167.037652347168));
#170214=CARTESIAN_POINT('Ctrl Pts',(54.1424378198232,10.61999998,-171.237717270032));
#170215=CARTESIAN_POINT('Ctrl Pts',(53.4956787755832,10.61999998,-171.565581122671));
#170216=CARTESIAN_POINT('Ctrl Pts',(53.7255998841352,9.94225131873298,-171.449026400902));
#170217=CARTESIAN_POINT('',(40.4577925858907,10.61999998,-144.90822241383));
#170218=CARTESIAN_POINT('Origin',(40.4577925858907,10.11999998,-144.90822241383));
#170219=CARTESIAN_POINT('',(54.1424378198232,10.61999998,-171.237717270032));
#170220=CARTESIAN_POINT('Origin',(54.1424378198232,10.11999998,-171.237717270032));
#170221=CARTESIAN_POINT('Ctrl Pts',(40.4577925858907,10.61999998,-144.90822241383));
#170222=CARTESIAN_POINT('Ctrl Pts',(42.7973924930771,10.61999998,-149.265897143292));
#170223=CARTESIAN_POINT('Ctrl Pts',(45.0988060523871,10.61999998,-153.643419067936));
#170224=CARTESIAN_POINT('Ctrl Pts',(47.3760737205892,10.61999998,-158.033490718866));
#170225=CARTESIAN_POINT('Ctrl Pts',(49.6533413887914,10.61999998,-162.423562369795));
#170226=CARTESIAN_POINT('Ctrl Pts',(51.9061626796858,10.61999998,-166.826339923461));
#170227=CARTESIAN_POINT('Ctrl Pts',(54.1424378198232,10.61999998,-171.237717270032));
#170228=CARTESIAN_POINT('Ctrl Pts',(40.1796955375735,9.88440567969849,-145.31549319889));
#170229=CARTESIAN_POINT('Ctrl Pts',(39.8393811074739,10.61999998,-145.511819782235));
#170230=CARTESIAN_POINT('Ctrl Pts',(40.5615971123268,10.61999998,-145.094901201173));
#170231=CARTESIAN_POINT('Ctrl Pts',(39.7529573682649,9.92251944743362,-144.614806037804));
#170232=CARTESIAN_POINT('Ctrl Pts',(39.502953749878,10.61999998,-144.775506187451));
#170233=CARTESIAN_POINT('Ctrl Pts',(40.1775148443164,10.61999998,-144.427612983545));
#170234=CARTESIAN_POINT('Ctrl Pts',(39.4582086878617,9.96279114543498,-143.870271315249));
#170235=CARTESIAN_POINT('Ctrl Pts',(39.2626189761704,10.61999998,-143.977483356653));
#170236=CARTESIAN_POINT('Ctrl Pts',(39.912296049423,10.61999998,-143.719512225762));
#170237=CARTESIAN_POINT('Ctrl Pts',(39.0709388975647,10.0461576545263,-142.315031435705));
#170238=CARTESIAN_POINT('Ctrl Pts',(38.9964277475896,10.61999998,-142.362517500096));
#170239=CARTESIAN_POINT('Ctrl Pts',(39.5638060942237,10.61999998,-142.242424394332));
#170240=CARTESIAN_POINT('Ctrl Pts',(38.9827638115546,10.0893227527421,-141.50278642521));
#170241=CARTESIAN_POINT('Ctrl Pts',(38.9510892610462,10.61999998,-141.53616355362));
#170242=CARTESIAN_POINT('Ctrl Pts',(39.4844701295021,10.61999998,-141.472057475813));
#170243=CARTESIAN_POINT('Ctrl Pts',(39.0027794749889,10.1314228667547,-140.701237361295));
#170244=CARTESIAN_POINT('Ctrl Pts',(39.0139531655019,10.61999998,-140.701380742148));
#170245=CARTESIAN_POINT('Ctrl Pts',(39.5025080143507,10.61999998,-140.713061620781));
#170246=CARTESIAN_POINT('',(39.5,10.61999998,-140.924467062102));
#170247=CARTESIAN_POINT('Origin',(39.5,10.11999998,-140.924467062102));
#170248=CARTESIAN_POINT('Ctrl Pts',(39.5,10.61999998,-140.924467062102));
#170249=CARTESIAN_POINT('Ctrl Pts',(39.5,10.61999998,-141.064641740712));
#170250=CARTESIAN_POINT('Ctrl Pts',(39.503286113677,10.619999980029,-141.204536867586));
#170251=CARTESIAN_POINT('Ctrl Pts',(39.5098002370266,10.6199999796907,-141.344151254401));
#170252=CARTESIAN_POINT('Ctrl Pts',(39.5163738758531,10.6199999793493,-141.485041210679));
#170253=CARTESIAN_POINT('Ctrl Pts',(39.5262347839853,10.6199999785395,-141.625645980312));
#170254=CARTESIAN_POINT('Ctrl Pts',(39.5393758471114,10.6199999780094,-141.765968909083));
#170255=CARTESIAN_POINT('Ctrl Pts',(39.5454296177964,10.6199999777652,-141.830612296339));
#170256=CARTESIAN_POINT('Ctrl Pts',(39.5521802385777,10.6199999776063,-141.895195868191));
#170257=CARTESIAN_POINT('Ctrl Pts',(39.5596307210412,10.6199999776383,-141.959719632822));
#170258=CARTESIAN_POINT('Ctrl Pts',(39.5766960195724,10.6199999777115,-142.107511042463));
#170259=CARTESIAN_POINT('Ctrl Pts',(39.5974615300858,10.6199999785835,-142.255205306997));
#170260=CARTESIAN_POINT('Ctrl Pts',(39.6219007996109,10.6199999791661,-142.402216894669));
#170261=CARTESIAN_POINT('Ctrl Pts',(39.6461342711754,10.6199999797438,-142.547990528609));
#170262=CARTESIAN_POINT('Ctrl Pts',(39.6739797737391,10.6199999799661,-142.693092202931));
#170263=CARTESIAN_POINT('Ctrl Pts',(39.7053613936648,10.6199999799929,-142.836960501111));
#170264=CARTESIAN_POINT('Ctrl Pts',(39.7158636782067,10.6199999800019,-142.885107977489));
#170265=CARTESIAN_POINT('Ctrl Pts',(39.7267615964733,10.61999998,-142.933117442989));
#170266=CARTESIAN_POINT('Ctrl Pts',(39.7380510717141,10.61999998,-142.980968310073));
#170267=CARTESIAN_POINT('Ctrl Pts',(39.8192390703685,10.61999998,-143.325086707917));
#170268=CARTESIAN_POINT('Ctrl Pts',(39.9201606061911,10.61999998,-143.662539288925));
#170269=CARTESIAN_POINT('Ctrl Pts',(40.0436577688824,10.61999998,-143.992366080443));
#170270=CARTESIAN_POINT('Ctrl Pts',(40.1606310196853,10.61999998,-144.304769306275));
#170271=CARTESIAN_POINT('Ctrl Pts',(40.2978572937931,10.61999998,-144.610331317757));
#170272=CARTESIAN_POINT('Ctrl Pts',(40.4577925858907,10.61999998,-144.90822241383));
#170273=CARTESIAN_POINT('Origin',(39.5,10.11999998,-55.24995));
#170274=CARTESIAN_POINT('',(39.5,10.61999998,-91.1341759094044));
#170275=CARTESIAN_POINT('Origin',(39.5,10.11999998,-91.1341759094044));
#170276=CARTESIAN_POINT('',(39.5,10.61999998,-55.24995));
#170277=CARTESIAN_POINT('Ctrl Pts',(39.,10.11999998,-91.1341759094044));
#170278=CARTESIAN_POINT('Ctrl Pts',(39.,10.61999998,-91.1341759094044));
#170279=CARTESIAN_POINT('Ctrl Pts',(39.5,10.61999998,-91.1341759094044));
#170280=CARTESIAN_POINT('Ctrl Pts',(39.,10.0814485101051,-90.4015548889157));
#170281=CARTESIAN_POINT('Ctrl Pts',(38.9598916786063,10.6199999799975,-90.3719688890003));
#170282=CARTESIAN_POINT('Ctrl Pts',(39.5000000020536,10.61999998,-90.4402448608912));
#170283=CARTESIAN_POINT('Ctrl Pts',(39.0871202471367,10.0432464379346,-89.6831085829417));
#170284=CARTESIAN_POINT('Ctrl Pts',(39.0069350308393,10.61999998,-89.6407441936901));
#170285=CARTESIAN_POINT('Ctrl Pts',(39.5784082214306,10.61999998,-89.7587725653299));
#170286=CARTESIAN_POINT('Ctrl Pts',(39.4353702758529,9.96778569102363,-88.2750332292462));
#170287=CARTESIAN_POINT('Ctrl Pts',(39.245797474144,10.61999998,-88.1799493597601));
#170288=CARTESIAN_POINT('Ctrl Pts',(39.89183324926,10.61999998,-88.4214995542899));
#170289=CARTESIAN_POINT('Ctrl Pts',(39.7001621050063,9.93023578241304,-87.580159846776));
#170290=CARTESIAN_POINT('Ctrl Pts',(39.4581171327344,10.61999998,-87.4384896017421));
#170291=CARTESIAN_POINT('Ctrl Pts',(40.1301388343916,10.61999998,-87.7606994776464));
#170292=CARTESIAN_POINT('Ctrl Pts',(40.064213984323,9.8954018152728,-86.9391114268059));
#170293=CARTESIAN_POINT('Ctrl Pts',(39.7432392475336,10.61999998,-86.7667827168808));
#170294=CARTESIAN_POINT('Ctrl Pts',(40.4577925858907,10.61999998,-87.1504205576762));
#170295=CARTESIAN_POINT('',(40.4577925858907,10.61999998,-87.1504205576762));
#170296=CARTESIAN_POINT('',(40.0642139580843,9.89540189669767,-86.9391114694666));
#170297=CARTESIAN_POINT('Origin',(40.4577925858907,10.11999998,-87.1504205576762));
#170298=CARTESIAN_POINT('Ctrl Pts',(39.,10.11999998,-91.1341759094044));
#170299=CARTESIAN_POINT('Ctrl Pts',(39.0000027915595,10.1116886332442,-90.9762294660295));
#170300=CARTESIAN_POINT('Ctrl Pts',(39.0041370161611,10.1028100622757,-90.8063031020809));
#170301=CARTESIAN_POINT('Ctrl Pts',(39.0195460817868,10.088416855121,-90.5336914216223));
#170302=CARTESIAN_POINT('Ctrl Pts',(39.0262224941828,10.0834435553843,-90.4398713106249));
#170303=CARTESIAN_POINT('Ctrl Pts',(39.0389688428197,10.0757342797035,-90.294792834635));
#170304=CARTESIAN_POINT('Ctrl Pts',(39.0460253914765,10.0718178234885,-90.2211670523011));
#170305=CARTESIAN_POINT('Ctrl Pts',(39.0555504742131,10.0671494790069,-90.1333915636446));
#170306=CARTESIAN_POINT('Ctrl Pts',(39.0606484786909,10.0647921444233,-90.0890374660041));
#170307=CARTESIAN_POINT('Ctrl Pts',(39.0632828966796,10.063607905681,-90.0667442610206));
#170308=CARTESIAN_POINT('Ctrl Pts',(39.0644304031572,10.0630992059044,-90.0571651875067));
#170309=CARTESIAN_POINT('Ctrl Pts',(39.0651995305414,10.0627598158354,-90.0507736232742));
#170310=CARTESIAN_POINT('Ctrl Pts',(39.0658473606639,10.0624757851372,-90.045423804078));
#170311=CARTESIAN_POINT('Ctrl Pts',(39.0741342857479,10.0588524738979,-89.9771728188365));
#170312=CARTESIAN_POINT('Ctrl Pts',(39.0892493568576,10.052622511364,-89.8541397133721));
#170313=CARTESIAN_POINT('Ctrl Pts',(39.1330129366525,10.0384158850763,-89.5865583530335));
#170314=CARTESIAN_POINT('Ctrl Pts',(39.1512193030171,10.0328676478481,-89.4835383246356));
#170315=CARTESIAN_POINT('Ctrl Pts',(39.1862174444622,10.0233700821188,-89.3086276329353));
#170316=CARTESIAN_POINT('Ctrl Pts',(39.1991713761146,10.0200103880156,-89.2469300451919));
#170317=CARTESIAN_POINT('Ctrl Pts',(39.220872401986,10.0147117872523,-89.1493691658317));
#170318=CARTESIAN_POINT('Ctrl Pts',(39.2322910073433,10.0119980603492,-89.0993354888038));
#170319=CARTESIAN_POINT('Ctrl Pts',(39.2466865483573,10.0087303108317,-89.0387909591602));
#170320=CARTESIAN_POINT('Ctrl Pts',(39.2530950507342,10.0073095256592,-89.0123804941478));
#170321=CARTESIAN_POINT('Ctrl Pts',(39.2574214878754,10.0063579939484,-88.9946709698606));
#170322=CARTESIAN_POINT('Ctrl Pts',(39.2601341389045,10.0057669940108,-88.9836551782209));
#170323=CARTESIAN_POINT('Ctrl Pts',(39.3160836297246,9.99365749385951,-88.7576909135574));
#170324=CARTESIAN_POINT('Ctrl Pts',(39.3736790817413,9.98295445715858,-88.5614711434704));
#170325=CARTESIAN_POINT('Ctrl Pts',(39.4583129915093,9.96894476384489,-88.3009574359105));
#170326=CARTESIAN_POINT('Ctrl Pts',(39.4862456662361,9.96460148642293,-88.2197448294764));
#170327=CARTESIAN_POINT('Ctrl Pts',(39.527022648588,9.95853825401135,-88.1062286732771));
#170328=CARTESIAN_POINT('Ctrl Pts',(39.5471321967724,9.9556187612689,-88.0515457852448));
#170329=CARTESIAN_POINT('Ctrl Pts',(39.5699677961773,9.95239356302238,-87.9913471515293));
#170330=CARTESIAN_POINT('Ctrl Pts',(39.5812132797666,9.95082387059787,-87.9621429820663));
#170331=CARTESIAN_POINT('Ctrl Pts',(39.585994170109,9.9501600872462,-87.9498182585687));
#170332=CARTESIAN_POINT('Ctrl Pts',(39.5891726689007,9.94971952318801,-87.941644245914));
#170333=CARTESIAN_POINT('Ctrl Pts',(39.5900087473004,9.94960366877689,-87.9394947831222));
#170334=CARTESIAN_POINT('Ctrl Pts',(39.7414059070582,9.92868751729576,-87.552038152988));
#170335=CARTESIAN_POINT('Ctrl Pts',(39.9039311777724,9.91073895422256,-87.2213504986795));
#170336=CARTESIAN_POINT('Ctrl Pts',(40.0642139577648,9.89540181781408,-86.9391114735717));
#170337=CARTESIAN_POINT('Ctrl Pts',(40.4577925858907,10.61999998,-87.1504205576762));
#170338=CARTESIAN_POINT('Ctrl Pts',(40.3970580365442,10.61999998,-87.2635430663923));
#170339=CARTESIAN_POINT('Ctrl Pts',(40.3395672151847,10.61999998,-87.3780682227952));
#170340=CARTESIAN_POINT('Ctrl Pts',(40.285131428432,10.61999998,-87.4939105062397));
#170341=CARTESIAN_POINT('Ctrl Pts',(40.2286629323529,10.61999998,-87.6140785045123));
#170342=CARTESIAN_POINT('Ctrl Pts',(40.1754817433896,10.61999998,-87.7356644050394));
#170343=CARTESIAN_POINT('Ctrl Pts',(40.1254267036649,10.61999998,-87.858600474452));
#170344=CARTESIAN_POINT('Ctrl Pts',(40.0931586145975,10.61999998,-87.9378514761339));
#170345=CARTESIAN_POINT('Ctrl Pts',(40.0621906903531,10.61999998,-88.0176641176421));
#170346=CARTESIAN_POINT('Ctrl Pts',(40.0324904304422,10.61999998,-88.0980242245578));
#170347=CARTESIAN_POINT('Ctrl Pts',(39.9448659684021,10.61999998,-88.3351100668741));
#170348=CARTESIAN_POINT('Ctrl Pts',(39.8685902579799,10.61999998,-88.5761404611087));
#170349=CARTESIAN_POINT('Ctrl Pts',(39.8033297324042,10.61999998,-88.818903429086));
#170350=CARTESIAN_POINT('Ctrl Pts',(39.7790792084132,10.61999998,-88.9091130792095));
#170351=CARTESIAN_POINT('Ctrl Pts',(39.7563491787903,10.61999998,-88.9995618473943));
#170352=CARTESIAN_POINT('Ctrl Pts',(39.735120734996,10.61999998,-89.090136059728));
#170353=CARTESIAN_POINT('Ctrl Pts',(39.6384824206298,10.61999998,-89.5024573438405));
#170354=CARTESIAN_POINT('Ctrl Pts',(39.5716278198238,10.61999998,-89.9196108763147));
#170355=CARTESIAN_POINT('Ctrl Pts',(39.5345653063075,10.61999998,-90.3415980464726));
#170356=CARTESIAN_POINT('Ctrl Pts',(39.5115257817295,10.61999998,-90.6039219650634));
#170357=CARTESIAN_POINT('Ctrl Pts',(39.500000000001,10.61999998,-90.8681139415084));
#170358=CARTESIAN_POINT('Ctrl Pts',(39.5,10.61999998,-91.1341759094044));
#170359=CARTESIAN_POINT('Origin',(59.5,11.11999998,-55.24995));
#170360=CARTESIAN_POINT('',(59.5,10.61999998,-58.24995));
#170361=CARTESIAN_POINT('Origin',(59.5,11.11999998,-58.24995));
#170362=CARTESIAN_POINT('',(59.5,10.61999998,-174.34995));
#170363=CARTESIAN_POINT('',(59.5,10.61999998,-58.24995));
#170364=CARTESIAN_POINT('Origin',(59.5,11.11999998,-174.34995));
#170365=CARTESIAN_POINT('Origin',(57.,11.11999998,-174.34995));
#170366=CARTESIAN_POINT('',(57.,10.61999998,-176.84995));
#170367=CARTESIAN_POINT('Origin',(57.,10.61999998,-174.34995));
#170368=CARTESIAN_POINT('Origin',(57.,11.11999998,-176.84995));
#170369=CARTESIAN_POINT('Origin',(-83.2809572255632,11.1199999800001,-176.84995));
#170370=CARTESIAN_POINT('',(-83.2809572255632,10.6199999800001,-176.84995));
#170371=CARTESIAN_POINT('Origin',(54.2951871140408,10.11999998,-179.64995));
#170372=CARTESIAN_POINT('',(54.2951871140408,10.61999998,-171.871644662643));
#170373=CARTESIAN_POINT('Origin',(54.2951871140408,10.11999998,-171.871644662643));
#170374=CARTESIAN_POINT('',(53.8350584096845,9.92434320033876,-179.64995));
#170375=CARTESIAN_POINT('',(54.2951871140408,10.61999998,-176.84995));
#170376=CARTESIAN_POINT('Ctrl Pts',(54.125256265546,10.6199999790853,-171.204806771037));
#170377=CARTESIAN_POINT('Ctrl Pts',(53.4900212150519,10.6200436404067,-171.547539040477));
#170378=CARTESIAN_POINT('Ctrl Pts',(53.7132658667077,9.94427345761011,-171.4270966421));
#170379=CARTESIAN_POINT('Ctrl Pts',(54.2414728015496,10.6199999790668,-171.420234627159));
#170380=CARTESIAN_POINT('Ctrl Pts',(53.5293152990573,10.6200454840218,-171.669460818781));
#170381=CARTESIAN_POINT('Ctrl Pts',(53.7965641368282,9.93061460392253,-171.570704923157));
#170382=CARTESIAN_POINT('Ctrl Pts',(54.3014296083361,10.6199999790573,-171.661245462922));
#170383=CARTESIAN_POINT('Ctrl Pts',(53.5404438804711,10.6200464809797,-171.777144153386));
#170384=CARTESIAN_POINT('Ctrl Pts',(53.8395077234217,9.92361807935392,-171.73138684676));
#170385=CARTESIAN_POINT('Ctrl Pts',(54.2947083191062,10.6199999790584,-171.909234173486));
#170386=CARTESIAN_POINT('Ctrl Pts',(53.5391294683119,10.6200463684923,-171.888526671109));
#170387=CARTESIAN_POINT('Ctrl Pts',(53.8346934801601,9.92440268025281,-171.896703002619));
#170388=CARTESIAN_POINT('Origin',(52.7058336008317,10.6200000150416,-171.863895229713));
#170389=CARTESIAN_POINT('Ctrl Pts',(54.0353592674108,10.61999998,-61.0321215118284));
#170390=CARTESIAN_POINT('Ctrl Pts',(53.3881607688931,10.6199999799991,-60.7039348782963));
#170391=CARTESIAN_POINT('Ctrl Pts',(53.6186572976477,9.94192748261378,-60.8208168640295));
#170392=CARTESIAN_POINT('Ctrl Pts',(51.8138491393997,10.61999998,-65.4130322530771));
#170393=CARTESIAN_POINT('Ctrl Pts',(51.1366620554546,10.6199999801381,-65.1210166348378));
#170394=CARTESIAN_POINT('Ctrl Pts',(51.3997940829438,9.93573759523097,-65.2017242497444));
#170395=CARTESIAN_POINT('Ctrl Pts',(49.5759233704096,10.61999998,-69.7854123595329));
#170396=CARTESIAN_POINT('Ctrl Pts',(48.8824081932915,10.619999979979,-69.498350907102));
#170397=CARTESIAN_POINT('Ctrl Pts',(49.1649346369347,9.92892193238703,-69.5741060667035));
#170398=CARTESIAN_POINT('Ctrl Pts',(45.0516568115529,10.61999998,-78.5050001236053));
#170399=CARTESIAN_POINT('Ctrl Pts',(44.3353985022919,10.6199999800216,-78.2014831316521));
#170400=CARTESIAN_POINT('Ctrl Pts',(44.6481582889209,9.913573864379,-78.2936943604392));
#170401=CARTESIAN_POINT('Ctrl Pts',(42.7656039747263,10.61999998,-82.8523636293437));
#170402=CARTESIAN_POINT('Ctrl Pts',(42.0255008894278,10.6199999800755,-82.557030405903));
#170403=CARTESIAN_POINT('Ctrl Pts',(42.3665201560454,9.90504529632398,-82.6410530645212));
#170404=CARTESIAN_POINT('Ctrl Pts',(40.4418478052835,10.61999998,-87.1801174602812));
#170405=CARTESIAN_POINT('Ctrl Pts',(39.7271443485661,10.6199999799995,-86.7963620990942));
#170406=CARTESIAN_POINT('Ctrl Pts',(40.0483186661866,9.89530939594053,-86.9688144589263));
#170407=CARTESIAN_POINT('',(54.0201152391274,10.61999998,-61.0621827299711));
#170408=CARTESIAN_POINT('',(53.6034226162473,9.94191093135268,-60.8508735991007));
#170409=CARTESIAN_POINT('Origin',(54.0201152391274,10.11999998,-61.0621827299711));
#170410=CARTESIAN_POINT('Ctrl Pts',(40.064213984323,9.89540181527278,-86.9391114268059));
#170411=CARTESIAN_POINT('Ctrl Pts',(41.1403040225241,9.89991895211768,-84.9300143693684));
#170412=CARTESIAN_POINT('Ctrl Pts',(42.2484592572501,9.90444570038255,-82.8416244158638));
#170413=CARTESIAN_POINT('Ctrl Pts',(43.9590882648639,9.91091969009987,-79.5901001415064));
#170414=CARTESIAN_POINT('Ctrl Pts',(44.5373616193329,9.91303143487921,-78.4864354927038));
#170415=CARTESIAN_POINT('Ctrl Pts',(45.4168857437243,9.91614729047684,-76.8012036834748));
#170416=CARTESIAN_POINT('Ctrl Pts',(45.8596761527945,9.91769289978181,-75.951154069854));
#170417=CARTESIAN_POINT('Ctrl Pts',(46.3815668865533,9.91948502097661,-74.9464205298688));
#170418=CARTESIAN_POINT('Ctrl Pts',(46.6438379037851,9.92038011477212,-74.4408015121859));
#170419=CARTESIAN_POINT('Ctrl Pts',(46.7893905868381,9.92087561089464,-74.1600050945544));
#170420=CARTESIAN_POINT('Ctrl Pts',(46.8599302771651,9.92111540880078,-74.0238636296621));
#170421=CARTESIAN_POINT('Ctrl Pts',(46.8975790657137,9.92124332089142,-73.951187093226));
#170422=CARTESIAN_POINT('Ctrl Pts',(46.902857723862,9.92126125354295,-73.9409969471016));
#170423=CARTESIAN_POINT('Ctrl Pts',(49.024122292157,9.9284670907748,-69.8459140539938));
#170424=CARTESIAN_POINT('Ctrl Pts',(51.2561074478258,9.93535987983753,-65.4852004772353));
#170425=CARTESIAN_POINT('Ctrl Pts',(53.6034226162473,9.94191093135268,-60.8508735991007));
#170426=CARTESIAN_POINT('Ctrl Pts',(54.0201152391274,10.61999998,-61.0621827299711));
#170427=CARTESIAN_POINT('Ctrl Pts',(51.8036107556176,10.61999998,-65.4330353431782));
#170428=CARTESIAN_POINT('Ctrl Pts',(49.570749196272,10.61999998,-69.7953845096745));
#170429=CARTESIAN_POINT('Ctrl Pts',(47.313790090977,10.61999998,-74.1452062415669));
#170430=CARTESIAN_POINT('Ctrl Pts',(45.056830985682,10.61999998,-78.4950279734592));
#170431=CARTESIAN_POINT('Ctrl Pts',(42.7760635123042,10.61999998,-82.8324726037656));
#170432=CARTESIAN_POINT('Ctrl Pts',(40.4577925858907,10.61999998,-87.1504205576762));
#170433=CARTESIAN_POINT('Ctrl Pts',(39.,12.1842625441365,-89.0065976851046));
#170434=CARTESIAN_POINT('Ctrl Pts',(39.,10.9256777712437,-87.8240033916746));
#170435=CARTESIAN_POINT('Ctrl Pts',(40.0658654432757,9.93538940172282,-86.8935063764011));
#170436=CARTESIAN_POINT('Ctrl Pts',(39.,10.9797897629302,-90.28846680179));
#170437=CARTESIAN_POINT('Ctrl Pts',(39.,9.77616182942057,-89.1086695731975));
#170438=CARTESIAN_POINT('Ctrl Pts',(40.0194662171323,8.81210183467955,-88.1753591901201));
#170439=CARTESIAN_POINT('Ctrl Pts',(39.,9.73513866768107,-91.5445844304498));
#170440=CARTESIAN_POINT('Ctrl Pts',(39.,8.58691729751272,-90.3710832422126));
#170441=CARTESIAN_POINT('Ctrl Pts',(39.9723426990601,7.65560021428954,-89.4314931216999));
#170442=CARTESIAN_POINT('Ctrl Pts',(39.,7.14206310577898,-93.9773376754667));
#170443=CARTESIAN_POINT('Ctrl Pts',(39.,6.11218708321155,-92.8159732515183));
#170444=CARTESIAN_POINT('Ctrl Pts',(39.8778703452952,5.25671151505436,-91.8642463668096));
#170445=CARTESIAN_POINT('Ctrl Pts',(39.,5.80730703259943,-95.141285808143));
#170446=CARTESIAN_POINT('Ctrl Pts',(38.9999999999877,4.84006269065046,-93.9862863085864));
#170447=CARTESIAN_POINT('Ctrl Pts',(39.8310091356278,4.02698776925249,-93.0281766935241));
#170448=CARTESIAN_POINT('Ctrl Pts',(39.,4.4206962941175,-96.234166137987));
#170449=CARTESIAN_POINT('Ctrl Pts',(39.,3.51696389869249,-95.0875400976674));
#170450=CARTESIAN_POINT('Ctrl Pts',(39.7856125955649,2.75522821384069,-94.1210748292835));
#170451=CARTESIAN_POINT('',(39.8417543268106,4.28989009189694,-92.7506602165387));
#170452=CARTESIAN_POINT('Ctrl Pts',(39.8417723428441,4.28998413512524,-92.7507162227756));
#170453=CARTESIAN_POINT('Ctrl Pts',(39.8597146560854,4.76916698343337,-92.3070009482122));
#170454=CARTESIAN_POINT('Ctrl Pts',(39.8780875478676,5.25018471631922,-91.8469438750031));
#170455=CARTESIAN_POINT('Ctrl Pts',(39.8968788416962,5.7343155538529,-91.369721820308));
#170456=CARTESIAN_POINT('Ctrl Pts',(39.9061864198051,5.9741120056742,-91.1333473806427));
#170457=CARTESIAN_POINT('Ctrl Pts',(39.9155964941233,6.21467253203749,-90.8927620401306));
#170458=CARTESIAN_POINT('Ctrl Pts',(39.9251065221777,6.45615586467189,-90.6478697442548));
#170459=CARTESIAN_POINT('Ctrl Pts',(39.9416791850316,6.87697711080465,-90.2211078638612));
#170460=CARTESIAN_POINT('Ctrl Pts',(39.9584956321962,7.29904284519804,-89.7828257767047));
#170461=CARTESIAN_POINT('Ctrl Pts',(39.9755525034532,7.72296859045191,-89.332496982478));
#170462=CARTESIAN_POINT('Ctrl Pts',(39.9904670259603,8.09364911993888,-88.9387296358234));
#170463=CARTESIAN_POINT('Ctrl Pts',(40.0055653344074,8.46575119682726,-88.5357514276307));
#170464=CARTESIAN_POINT('Ctrl Pts',(40.0208411411111,8.83969191810781,-88.1232475756398));
#170465=CARTESIAN_POINT('Ctrl Pts',(40.0351460298419,9.18986526826736,-87.736962136304));
#170466=CARTESIAN_POINT('Ctrl Pts',(40.0496065738335,9.54165057206099,-87.3423230586879));
#170467=CARTESIAN_POINT('Ctrl Pts',(40.0642139729082,9.89540198625494,-86.9391115876706));
#170468=CARTESIAN_POINT('Ctrl Pts',(39.8417543268106,4.28989009189694,-92.7506602165387));
#170469=CARTESIAN_POINT('Ctrl Pts',(39.8111499956431,4.29299201950353,-92.8082417354953));
#170470=CARTESIAN_POINT('Ctrl Pts',(39.7802667553935,4.29622413902246,-92.8683179012178));
#170471=CARTESIAN_POINT('Ctrl Pts',(39.7493004842404,4.29958883760676,-92.9309560235319));
#170472=CARTESIAN_POINT('Ctrl Pts',(39.7183256003837,4.30295447202061,-92.9936115674976));
#170473=CARTESIAN_POINT('Ctrl Pts',(39.6872729212866,4.30643631872874,-93.0588330079571));
#170474=CARTESIAN_POINT('Ctrl Pts',(39.6563397338845,4.31006069299538,-93.1266868986523));
#170475=CARTESIAN_POINT('Ctrl Pts',(39.6254065464824,4.31368506726203,-93.1945407893474));
#170476=CARTESIAN_POINT('Ctrl Pts',(39.5945940943932,4.31745491936417,-93.2650236904387));
#170477=CARTESIAN_POINT('Ctrl Pts',(39.5641304981276,4.32136651585282,-93.3381731100622));
#170478=CARTESIAN_POINT('Ctrl Pts',(39.5488986999947,4.32332231409715,-93.3747478198739));
#170479=CARTESIAN_POINT('Ctrl Pts',(39.5337543520915,4.32531328847347,-93.4119889205435));
#170480=CARTESIAN_POINT('Ctrl Pts',(39.5187271516468,4.32733725951214,-93.4498994832949));
#170481=CARTESIAN_POINT('Ctrl Pts',(39.5112135514244,4.32834924503147,-93.4688547646706));
#170482=CARTESIAN_POINT('Ctrl Pts',(39.5037292367631,4.32936947808469,-93.4879774096565));
#170483=CARTESIAN_POINT('Ctrl Pts',(39.4962779863463,4.33039754815179,-93.5072676685439));
#170484=CARTESIAN_POINT('Ctrl Pts',(39.4925523611378,4.33091158318535,-93.5169127979876));
#170485=CARTESIAN_POINT('Ctrl Pts',(39.4888350016951,4.33142757732785,-93.5265998307344));
#170486=CARTESIAN_POINT('Ctrl Pts',(39.4851263808663,4.3319454745947,-93.5363287933278));
#170487=CARTESIAN_POINT('Ctrl Pts',(39.4832720704519,4.33220442322813,-93.5411932746244));
#170488=CARTESIAN_POINT('Ctrl Pts',(39.4814199446683,4.33246384763303,-93.5460682383712));
#170489=CARTESIAN_POINT('Ctrl Pts',(39.4795700627628,4.33272374031367,-93.5509536873952));
#170490=CARTESIAN_POINT('Ctrl Pts',(39.47864512181,4.33285368665399,-93.5533964119072));
#170491=CARTESIAN_POINT('Ctrl Pts',(39.4777207418251,4.33298375006261,-93.5558417577377));
#170492=CARTESIAN_POINT('Ctrl Pts',(39.4767969302229,4.33311392956962,-93.5582897252076));
#170493=CARTESIAN_POINT('Ctrl Pts',(39.4758731186208,4.33324410907663,-93.5607376926775));
#170494=CARTESIAN_POINT('Ctrl Pts',(39.4745077545883,4.33343689447469,-93.5643638035833));
#170495=CARTESIAN_POINT('Ctrl Pts',(39.4740272079786,4.3335048154045,-93.5656414928445));
#170496=CARTESIAN_POINT('Ctrl Pts',(39.4619116443501,4.33521724106759,-93.5978546543312));
#170497=CARTESIAN_POINT('Ctrl Pts',(39.4483615670327,4.33714569186926,-93.6346022140469));
#170498=CARTESIAN_POINT('Ctrl Pts',(39.4335980269417,4.33930934348358,-93.67594212584));
#170499=CARTESIAN_POINT('Ctrl Pts',(39.4185623987223,4.34151287062333,-93.7180439212436));
#170500=CARTESIAN_POINT('Ctrl Pts',(39.4022682265848,4.34396031741693,-93.7649089098956));
#170501=CARTESIAN_POINT('Ctrl Pts',(39.3850008239921,4.34667323458354,-93.8166147001729));
#170502=CARTESIAN_POINT('Ctrl Pts',(39.3761835953417,4.34805852752724,-93.8430171525961));
#170503=CARTESIAN_POINT('Ctrl Pts',(39.3671134251348,4.34951306320326,-93.8706820633472));
#170504=CARTESIAN_POINT('Ctrl Pts',(39.3578332586383,4.35103987466927,-93.8996213409729));
#170505=CARTESIAN_POINT('Ctrl Pts',(39.3382571951746,4.3542606097894,-93.9606673508278));
#170506=CARTESIAN_POINT('Ctrl Pts',(39.3177461102384,4.35779976794404,-94.0273776023551));
#170507=CARTESIAN_POINT('Ctrl Pts',(39.2967677854055,4.36164894682482,-94.0998298524968));
#170508=CARTESIAN_POINT('Ctrl Pts',(39.2934740342213,4.36225329619961,-94.111205388275));
#170509=CARTESIAN_POINT('Ctrl Pts',(39.2901688648655,4.36286528720593,-94.1227225016788));
#170510=CARTESIAN_POINT('Ctrl Pts',(39.2868541959498,4.36348488625061,-94.1343815258526));
#170511=CARTESIAN_POINT('Ctrl Pts',(39.274641085215,4.36576783876756,-94.1773399500328));
#170512=CARTESIAN_POINT('Ctrl Pts',(39.2622991914327,4.36815323253446,-94.2222238784512));
#170513=CARTESIAN_POINT('Ctrl Pts',(39.2499302932482,4.37063298596967,-94.2690438315574));
#170514=CARTESIAN_POINT('Ctrl Pts',(39.2437458441559,4.37187286268728,-94.2924538081105));
#170515=CARTESIAN_POINT('Ctrl Pts',(39.2375547020892,4.37313634560285,-94.3163478101846));
#170516=CARTESIAN_POINT('Ctrl Pts',(39.2313701710456,4.37442178670003,-94.3407266202839));
#170517=CARTESIAN_POINT('Ctrl Pts',(39.2268578943689,4.37535965342608,-94.3585135689532));
#170518=CARTESIAN_POINT('Ctrl Pts',(39.2221531070756,4.37635067920456,-94.3773493160581));
#170519=CARTESIAN_POINT('Ctrl Pts',(39.2176913730843,4.37730344240409,-94.3955037967945));
#170520=CARTESIAN_POINT('Ctrl Pts',(39.2160378498885,4.37765653742357,-94.4022318659857));
#170521=CARTESIAN_POINT('Ctrl Pts',(39.2144172036271,4.37800437246001,-94.4088662101995));
#170522=CARTESIAN_POINT('Ctrl Pts',(39.2128498752563,4.37834227799597,-94.4153182336563));
#170523=CARTESIAN_POINT('Ctrl Pts',(39.2126660218777,4.37838191555729,-94.4160750797219));
#170524=CARTESIAN_POINT('Ctrl Pts',(39.2124823293284,4.37842154399935,-94.4168317672599));
#170525=CARTESIAN_POINT('Ctrl Pts',(39.2122987973978,4.37846116332228,-94.4175882962553));
#170526=CARTESIAN_POINT('Ctrl Pts',(39.1892451767618,4.38343778421844,-94.5126166240753));
#170527=CARTESIAN_POINT('Ctrl Pts',(39.1687677021364,4.38827551589204,-94.6052466993645));
#170528=CARTESIAN_POINT('Ctrl Pts',(39.1505238108285,4.39296972656187,-94.6953494792007));
#170529=CARTESIAN_POINT('Ctrl Pts',(39.1322799195205,4.3976639372317,-94.7854522590368));
#170530=CARTESIAN_POINT('Ctrl Pts',(39.1162696674874,4.40221466077713,-94.8730283767273));
#170531=CARTESIAN_POINT('Ctrl Pts',(39.1021792361851,4.40661979062833,-94.9579995734556));
#170532=CARTESIAN_POINT('Ctrl Pts',(39.0860807420172,4.41165270663333,-95.0550802295142));
#170533=CARTESIAN_POINT('Ctrl Pts',(39.0724902488796,4.41649497941412,-95.1487491592476));
#170534=CARTESIAN_POINT('Ctrl Pts',(39.0609905931823,4.42114241942972,-95.2388722612092));
#170535=CARTESIAN_POINT('Ctrl Pts',(39.0528187821168,4.42444495323986,-95.302914957899));
#170536=CARTESIAN_POINT('Ctrl Pts',(39.0457039565657,4.42764904915551,-95.3651661449135));
#170537=CARTESIAN_POINT('Ctrl Pts',(39.0395083479183,4.43075318936736,-95.4255780326426));
#170538=CARTESIAN_POINT('Ctrl Pts',(39.0350899695047,4.43296689699252,-95.4686605764032));
#170539=CARTESIAN_POINT('Ctrl Pts',(39.0311383113794,4.43513021876868,-95.5108164380876));
#170540=CARTESIAN_POINT('Ctrl Pts',(39.0276053730942,4.43724335335137,-95.5520431268892));
#170541=CARTESIAN_POINT('Ctrl Pts',(39.0205036056785,4.44149108968677,-95.6349153232202));
#170542=CARTESIAN_POINT('Ctrl Pts',(39.0150924157327,4.44553548053849,-95.7140220206559));
#170543=CARTESIAN_POINT('Ctrl Pts',(39.0110141613094,4.4493769408033,-95.7893219652571));
#170544=CARTESIAN_POINT('Ctrl Pts',(39.0067749714961,4.45336999212692,-95.8675933836059));
#170545=CARTESIAN_POINT('Ctrl Pts',(39.003975731844,4.45714380773583,-95.9417521367898));
#170546=CARTESIAN_POINT('Ctrl Pts',(39.0022556585823,4.46070073192571,-96.0117925129403));
#170547=CARTESIAN_POINT('Ctrl Pts',(39.0006677664691,4.46398431989507,-96.0764505501149));
#170548=CARTESIAN_POINT('Ctrl Pts',(39.,4.4670831113137,-96.1375996770293));
#170549=CARTESIAN_POINT('Ctrl Pts',(39.,4.46999998000002,-96.1952589849652));
#170550=CARTESIAN_POINT('Ctrl Pts',(39.8417798628559,4.28988750369336,-92.7506121713693));
#170551=CARTESIAN_POINT('Ctrl Pts',(39.9519009607655,3.96999998000001,-92.8065726369586));
#170552=CARTESIAN_POINT('Ctrl Pts',(40.2576018765703,3.96999998000001,-92.9619213022396));
#170553=CARTESIAN_POINT('Ctrl Pts',(39.558565846057,4.31859237238363,-93.2834642887004));
#170554=CARTESIAN_POINT('Ctrl Pts',(39.6570458949425,3.9699999800025,-93.3357860473751));
#170555=CARTESIAN_POINT('Ctrl Pts',(40.0026978626623,3.96999998000001,-93.4635309699092));
#170556=CARTESIAN_POINT('Ctrl Pts',(39.3523491668799,4.34822838553358,-93.8402926529419));
#170557=CARTESIAN_POINT('Ctrl Pts',(39.4410018196003,3.96999998000002,-93.8819356839734));
#170558=CARTESIAN_POINT('Ctrl Pts',(39.817114250256,3.96999998000002,-93.9870091547076));
#170559=CARTESIAN_POINT('Ctrl Pts',(39.0722484171839,4.40869400027786,-94.9948839370727));
#170560=CARTESIAN_POINT('Ctrl Pts',(39.1236627362708,3.96999998000002,-95.0167026881129));
#170561=CARTESIAN_POINT('Ctrl Pts',(39.5650235754014,3.96999998000002,-95.0708764103351));
#170562=CARTESIAN_POINT('Ctrl Pts',(39.,4.43971662334272,-95.5966316298752));
#170563=CARTESIAN_POINT('Ctrl Pts',(39.0293922558424,3.96999998000002,-95.61424653503));
#170564=CARTESIAN_POINT('Ctrl Pts',(39.500000001452,3.96999998000002,-95.6349699403799));
#170565=CARTESIAN_POINT('Ctrl Pts',(39.,4.46999998000002,-96.1952589849652));
#170566=CARTESIAN_POINT('Ctrl Pts',(39.,3.96999998000001,-96.1952589849652));
#170567=CARTESIAN_POINT('Ctrl Pts',(39.5,3.96999998000002,-96.1952589849652));
#170568=CARTESIAN_POINT('',(39.5,3.96999998000002,-96.1952589849652));
#170569=CARTESIAN_POINT('Origin',(39.5,4.46999998000001,-96.1952589849652));
#170570=CARTESIAN_POINT('',(40.2576018765703,3.96999998000001,-92.9619213022396));
#170571=CARTESIAN_POINT('Origin',(40.2576018765703,4.46999998000001,-92.9619213022396));
#170572=CARTESIAN_POINT('Ctrl Pts',(39.5,3.96999998000002,-96.1952589849652));
#170573=CARTESIAN_POINT('Ctrl Pts',(39.5,3.96999998000001,-95.9142103380175));
#170574=CARTESIAN_POINT('Ctrl Pts',(39.5161227273835,3.96999998000002,-95.6343109988079));
#170575=CARTESIAN_POINT('Ctrl Pts',(39.5801128567305,3.96999998000002,-95.0767752377766));
#170576=CARTESIAN_POINT('Ctrl Pts',(39.6280462441481,3.96999998000002,-94.7999095964395));
#170577=CARTESIAN_POINT('Ctrl Pts',(39.81711425019,3.96999998000002,-93.9870091546851));
#170578=CARTESIAN_POINT('Ctrl Pts',(40.0026450649981,3.96999998000001,-93.4636348550876));
#170579=CARTESIAN_POINT('Ctrl Pts',(40.2576018765703,3.96999998000001,-92.9619213022396));
#170580=CARTESIAN_POINT('Origin',(39.5,4.46999998000002,-55.24995));
#170581=CARTESIAN_POINT('',(39.5,3.96999998000002,-135.863383986541));
#170582=CARTESIAN_POINT('Origin',(39.5,4.46999998000001,-135.863383986541));
#170583=CARTESIAN_POINT('',(39.5,3.96999998000002,-55.24995));
#170584=CARTESIAN_POINT('Ctrl Pts',(39.,4.46999998000002,-135.863383986541));
#170585=CARTESIAN_POINT('Ctrl Pts',(39.,3.96999998000001,-135.863383986541));
#170586=CARTESIAN_POINT('Ctrl Pts',(39.5,3.96999998000002,-135.863383986541));
#170587=CARTESIAN_POINT('Ctrl Pts',(39.,4.43959418388259,-136.464431642573));
#170588=CARTESIAN_POINT('Ctrl Pts',(39.0295065227812,3.96999998000002,-136.446655166649));
#170589=CARTESIAN_POINT('Ctrl Pts',(39.50000000251,3.96999998000002,-136.425947926524));
#170590=CARTESIAN_POINT('Ctrl Pts',(39.0706358339689,4.40924336018453,-137.053149400534));
#170591=CARTESIAN_POINT('Ctrl Pts',(39.1216633961175,3.96999998000002,-137.031492360702));
#170592=CARTESIAN_POINT('Ctrl Pts',(39.5635722498606,3.96999998000002,-136.977817064522));
#170593=CARTESIAN_POINT('Ctrl Pts',(39.3484951732863,4.34886300930159,-138.206349454905));
#170594=CARTESIAN_POINT('Ctrl Pts',(39.4368658200899,3.96999998000001,-138.164990760612));
#170595=CARTESIAN_POINT('Ctrl Pts',(39.813645656669,3.96999998000002,-138.060358011877));
#170596=CARTESIAN_POINT('Ctrl Pts',(39.5585840804945,4.31859052702601,-138.775212992296));
#170597=CARTESIAN_POINT('Ctrl Pts',(39.6570895715147,3.96999997999977,-138.722935325351));
#170598=CARTESIAN_POINT('Ctrl Pts',(40.0027227918541,3.96999998000001,-138.595161064797));
#170599=CARTESIAN_POINT('Ctrl Pts',(39.8417798628559,4.28988750369336,-139.308030800137));
#170600=CARTESIAN_POINT('Ctrl Pts',(39.9519009607655,3.96999998000001,-139.252070334547));
#170601=CARTESIAN_POINT('Ctrl Pts',(40.2576018765703,3.96999998000001,-139.096721669266));
#170602=CARTESIAN_POINT('',(40.2576018765703,3.96999998000001,-139.096721669266));
#170603=CARTESIAN_POINT('Ctrl Pts',(40.2576018765703,3.96999998000001,-139.096721669266));
#170604=CARTESIAN_POINT('Ctrl Pts',(40.1422232489788,3.96999998000001,-138.869675289079));
#170605=CARTESIAN_POINT('Ctrl Pts',(40.0403932052787,3.96999998000002,-138.635953665714));
#170606=CARTESIAN_POINT('Ctrl Pts',(39.9518763029277,3.96999998000002,-138.397956901358));
#170607=CARTESIAN_POINT('Ctrl Pts',(39.858956988463,3.96999998000002,-138.148123303464));
#170608=CARTESIAN_POINT('Ctrl Pts',(39.7807077156263,3.96999998000002,-137.893577344813));
#170609=CARTESIAN_POINT('Ctrl Pts',(39.716907177833,3.96999998000002,-137.637072537694));
#170610=CARTESIAN_POINT('Ctrl Pts',(39.7071356404173,3.96999998000002,-137.597786876369));
#170611=CARTESIAN_POINT('Ctrl Pts',(39.6977031285494,3.96999998000002,-137.558455249076));
#170612=CARTESIAN_POINT('Ctrl Pts',(39.6886089528968,3.96999998000002,-137.519087538285));
#170613=CARTESIAN_POINT('Ctrl Pts',(39.6032792176002,3.96999998000002,-137.149704268227));
#170614=CARTESIAN_POINT('Ctrl Pts',(39.5465796834581,3.96999998000002,-136.775425176616));
#170615=CARTESIAN_POINT('Ctrl Pts',(39.5191682987961,3.96999998000002,-136.396137730917));
#170616=CARTESIAN_POINT('Ctrl Pts',(39.5064128043257,3.96999998000002,-136.219641761233));
#170617=CARTESIAN_POINT('Ctrl Pts',(39.5000000000002,3.96999998000002,-136.042061173853));
#170618=CARTESIAN_POINT('Ctrl Pts',(39.5,3.96999998000002,-135.863383986541));
#170619=CARTESIAN_POINT('Origin',(40.2576018765703,4.46999998000001,-139.096721669266));
#170620=CARTESIAN_POINT('Ctrl Pts',(56.2171666226051,3.96999998000001,-171.237717270032));
#170621=CARTESIAN_POINT('Ctrl Pts',(55.8759673883189,3.96999998,-171.404299214979));
#170622=CARTESIAN_POINT('Ctrl Pts',(55.7843555297028,4.33575017898885,-171.449026400902));
#170623=CARTESIAN_POINT('Ctrl Pts',(53.5931279590331,3.96999998000001,-165.863065274939));
#170624=CARTESIAN_POINT('Ctrl Pts',(53.2681640678716,3.96999998006972,-166.052285867785));
#170625=CARTESIAN_POINT('Ctrl Pts',(53.1620910906406,4.33003381235646,-166.074376691472));
#170626=CARTESIAN_POINT('Ctrl Pts',(50.9564483006955,3.96999998000001,-160.494687880121));
#170627=CARTESIAN_POINT('Ctrl Pts',(50.6399914208629,3.96999998001567,-160.688987094682));
#170628=CARTESIAN_POINT('Ctrl Pts',(50.5275177831741,4.32360860554286,-160.70599701099));
#170629=CARTESIAN_POINT('Ctrl Pts',(45.6433184787346,3.96999998000001,-149.777683344423));
#170630=CARTESIAN_POINT('Ctrl Pts',(45.3382862796144,3.96999997998453,-149.967930534599));
#170631=CARTESIAN_POINT('Ctrl Pts',(45.2197944205701,4.30863333062082,-149.988992475295));
#170632=CARTESIAN_POINT('Ctrl Pts',(42.9672472399765,3.96999998000001,-144.428863195016));
#170633=CARTESIAN_POINT('Ctrl Pts',(42.6741187750921,3.96999998000002,-144.626843683376));
#170634=CARTESIAN_POINT('Ctrl Pts',(42.547006853164,4.30009530891334,-144.640178460294));
#170635=CARTESIAN_POINT('Ctrl Pts',(40.2576018765703,3.96999998000001,-139.096721669266));
#170636=CARTESIAN_POINT('Ctrl Pts',(39.9519009607656,3.96999998000002,-139.252070334547));
#170637=CARTESIAN_POINT('Ctrl Pts',(39.8417798628559,4.28988750369336,-139.308030800137));
#170638=CARTESIAN_POINT('',(56.217166622605,3.96999998000001,-171.237717270032));
#170639=CARTESIAN_POINT('Ctrl Pts',(56.217166622605,3.96999998000001,-171.237717270032));
#170640=CARTESIAN_POINT('Ctrl Pts',(53.5931275135095,3.96999998000001,-165.863064362474));
#170641=CARTESIAN_POINT('Ctrl Pts',(50.9564483006798,3.96999998000001,-160.49468788009));
#170642=CARTESIAN_POINT('Ctrl Pts',(48.2998833897147,3.96999998000001,-155.136185612272));
#170643=CARTESIAN_POINT('Ctrl Pts',(45.6433184787496,3.96999998000001,-149.777683344454));
#170644=CARTESIAN_POINT('Ctrl Pts',(42.9672487496428,3.96999998000001,-144.428866165794));
#170645=CARTESIAN_POINT('Ctrl Pts',(40.2576018765703,3.96999998000001,-139.096721669266));
#170646=CARTESIAN_POINT('Origin',(56.2171666226051,4.46999998000001,-171.237717270032));
#170647=CARTESIAN_POINT('Ctrl Pts',(56.362878117604,3.96999998707827,-171.9375490258));
#170648=CARTESIAN_POINT('Ctrl Pts',(55.9943718457987,3.9699379192599,-171.920606124721));
#170649=CARTESIAN_POINT('Ctrl Pts',(55.8855878616368,4.32236176169507,-171.915575297858));
#170650=CARTESIAN_POINT('Ctrl Pts',(56.3748852598389,3.96999998705621,-171.673567304561));
#170651=CARTESIAN_POINT('Ctrl Pts',(56.0043522879838,3.96993816409121,-171.724641829017));
#170652=CARTESIAN_POINT('Ctrl Pts',(55.8939328694509,4.32126340276226,-171.739613349113));
#170653=CARTESIAN_POINT('Ctrl Pts',(56.3146644389369,3.96999998716678,-171.413359333373));
#170654=CARTESIAN_POINT('Ctrl Pts',(55.9538751380083,3.96993692936927,-171.529346602164));
#170655=CARTESIAN_POINT('Ctrl Pts',(55.8520802190683,4.32676800360642,-171.566123460328));
#170656=CARTESIAN_POINT('Ctrl Pts',(56.1866565229903,3.96999998740382,-171.178434208374));
#170657=CARTESIAN_POINT('Ctrl Pts',(55.8512265932963,3.96993423686634,-171.361424046831));
#170658=CARTESIAN_POINT('Ctrl Pts',(55.7630923089791,4.33856909837021,-171.409535679069));
#170659=CARTESIAN_POINT('',(56.3642936064049,3.96999998000001,-171.871644662643));
#170660=CARTESIAN_POINT('Origin',(54.8887873791231,3.96999970486964,-171.852186214504));
#170661=CARTESIAN_POINT('Origin',(56.3642936064049,4.46999998000001,-171.871644662643));
#170662=CARTESIAN_POINT('Origin',(56.3642936064049,4.46999998000001,-179.64995));
#170663=CARTESIAN_POINT('',(56.3642936064049,3.96999998000001,-171.871644662643));
#170664=CARTESIAN_POINT('',(55.8866301012659,4.32222455627096,-179.64995));
#170665=CARTESIAN_POINT('Origin',(60.,3.46999998000001,-176.84995));
#170666=CARTESIAN_POINT('',(57.,3.96999998000001,-176.84995));
#170667=CARTESIAN_POINT('',(-83.2809572255632,3.96999998000007,-176.84995));
#170668=CARTESIAN_POINT('Origin',(57.,3.46999998000001,-176.84995));
#170669=CARTESIAN_POINT('Origin',(57.,3.46999998000001,-174.34995));
#170670=CARTESIAN_POINT('',(59.5,3.96999998000001,-174.34995));
#170671=CARTESIAN_POINT('Origin',(57.,3.96999998000001,-174.34995));
#170672=CARTESIAN_POINT('Origin',(59.5,3.46999998000001,-174.34995));
#170673=CARTESIAN_POINT('Origin',(59.5,3.46999998000001,-55.24995));
#170674=CARTESIAN_POINT('',(59.5,3.96999998000001,-58.24995));
#170675=CARTESIAN_POINT('',(59.5,3.96999998000001,-174.34995));
#170676=CARTESIAN_POINT('Origin',(59.5,3.46999998000001,-58.24995));
#170677=CARTESIAN_POINT('Ctrl Pts',(40.2576018765703,3.96999998000001,-92.9619213022396));
#170678=CARTESIAN_POINT('Ctrl Pts',(39.9519009607656,3.96999998000002,-92.8065726369586));
#170679=CARTESIAN_POINT('Ctrl Pts',(39.8417798628559,4.28988750369336,-92.7506121713693));
#170680=CARTESIAN_POINT('Ctrl Pts',(42.9469739380577,3.96999998000001,-87.6696743385966));
#170681=CARTESIAN_POINT('Ctrl Pts',(42.6535990616308,3.96999998005189,-87.4723136103566));
#170682=CARTESIAN_POINT('Ctrl Pts',(42.5267665504115,4.30001893486917,-87.4583592347964));
#170683=CARTESIAN_POINT('Ctrl Pts',(45.6032617662856,3.96999998000001,-82.3609901713122));
#170684=CARTESIAN_POINT('Ctrl Pts',(45.2981339154354,3.96999997998722,-82.1711713234106));
#170685=CARTESIAN_POINT('Ctrl Pts',(45.1797873789129,4.30850505828642,-82.1496810404423));
#170686=CARTESIAN_POINT('Ctrl Pts',(50.8772452803079,3.96999998000001,-71.7244637521124));
#170687=CARTESIAN_POINT('Ctrl Pts',(50.5607523082128,3.96999998001296,-71.5306210575042));
#170688=CARTESIAN_POINT('Ctrl Pts',(50.4483866457226,4.32340039588272,-71.5131546212415));
#170689=CARTESIAN_POINT('Ctrl Pts',(53.4945734938964,3.96999998000001,-66.3964343016074));
#170690=CARTESIAN_POINT('Ctrl Pts',(53.1696590969437,3.96999998001539,-66.20755441643));
#170691=CARTESIAN_POINT('Ctrl Pts',(53.0636135580956,4.32979794413352,-66.1851229312852));
#170692=CARTESIAN_POINT('Ctrl Pts',(56.0993680931338,3.96999998000001,-61.0621827299711));
#170693=CARTESIAN_POINT('Ctrl Pts',(55.7583700098454,3.96999998000001,-60.8956682801396));
#170694=CARTESIAN_POINT('Ctrl Pts',(55.6666368275827,4.33549309160632,-60.8508735991007));
#170695=CARTESIAN_POINT('',(55.6666368275827,4.33549309160632,-60.8508735991007));
#170696=CARTESIAN_POINT('Ctrl Pts',(55.6666368275827,4.33549309160632,-60.8508735991007));
#170697=CARTESIAN_POINT('Ctrl Pts',(54.8205608505865,4.33364196429319,-62.5846960616882));
#170698=CARTESIAN_POINT('Ctrl Pts',(53.9903026692869,4.33175386550846,-64.2827945099236));
#170699=CARTESIAN_POINT('Ctrl Pts',(53.1758068650219,4.32982708116484,-65.9451406479148));
#170700=CARTESIAN_POINT('Ctrl Pts',(52.3434513083755,4.32785804750441,-67.6439376678396));
#170701=CARTESIAN_POINT('Ctrl Pts',(51.5275573839763,4.3258486252169,-69.3053969967707));
#170702=CARTESIAN_POINT('Ctrl Pts',(50.7281139966181,4.32379940522285,-70.9295151994433));
#170703=CARTESIAN_POINT('Ctrl Pts',(49.899563188546,4.32167557393118,-72.6127669099562));
#170704=CARTESIAN_POINT('Ctrl Pts',(49.0886828014879,4.31950900276859,-74.2559089319538));
#170705=CARTESIAN_POINT('Ctrl Pts',(48.2955072571905,4.31730276847417,-75.8589672795686));
#170706=CARTESIAN_POINT('Ctrl Pts',(48.1392483326796,4.31686813102153,-76.1747765290183));
#170707=CARTESIAN_POINT('Ctrl Pts',(47.9836766773074,4.31643196122799,-76.4890301985629));
#170708=CARTESIAN_POINT('Ctrl Pts',(47.8287927443473,4.31599429265464,-76.8017286210993));
#170709=CARTESIAN_POINT('Ctrl Pts',(47.824013964662,4.31598078885443,-76.8113765996899));
#170710=CARTESIAN_POINT('Ctrl Pts',(47.8200359612573,4.31596954569576,-76.8194077686504));
#170711=CARTESIAN_POINT('Ctrl Pts',(47.8144583711674,4.31595377082859,-76.8306681161508));
#170712=CARTESIAN_POINT('Ctrl Pts',(47.8143345851444,4.31595342072971,-76.8309180222235));
#170713=CARTESIAN_POINT('Ctrl Pts',(47.8142107994953,4.3159530706297,-76.8311679274349));
#170714=CARTESIAN_POINT('Ctrl Pts',(47.8140870142199,4.31595272052855,-76.8314178317851));
#170715=CARTESIAN_POINT('Ctrl Pts',(47.1001907406593,4.31393361201366,-78.272669901606));
#170716=CARTESIAN_POINT('Ctrl Pts',(46.3987484039203,4.31187755465099,-79.6852882239203));
#170717=CARTESIAN_POINT('Ctrl Pts',(45.7096807250197,4.30978236308995,-81.06923675739));
#170718=CARTESIAN_POINT('Ctrl Pts',(45.015912454009,4.30767287882411,-82.4626261306444));
#170719=CARTESIAN_POINT('Ctrl Pts',(44.3346885815387,4.30552373988916,-83.8269534017042));
#170720=CARTESIAN_POINT('Ctrl Pts',(43.6659786213913,4.30333497175895,-85.16220785781));
#170721=CARTESIAN_POINT('Ctrl Pts',(42.9695469080432,4.30105546699622,-86.5528160497628));
#170722=CARTESIAN_POINT('Ctrl Pts',(42.2866882495013,4.29873298384541,-87.911891050928));
#170723=CARTESIAN_POINT('Ctrl Pts',(41.6174198017565,4.29636985306184,-89.2394474379971));
#170724=CARTESIAN_POINT('Ctrl Pts',(41.0144946503879,4.29424097489616,-90.4354057090332));
#170725=CARTESIAN_POINT('Ctrl Pts',(40.4225998060169,4.2920791485557,-91.6057848751819));
#170726=CARTESIAN_POINT('Ctrl Pts',(39.841779862856,4.28988750369336,-92.7506121713693));
#170727=CARTESIAN_POINT('',(56.0993680931338,3.96999998000001,-61.0621827299711));
#170728=CARTESIAN_POINT('Origin',(56.0993680931338,4.46999998000001,-61.0621827299711));
#170729=CARTESIAN_POINT('Ctrl Pts',(40.2576018765703,3.96999998000001,-92.9619213022396));
#170730=CARTESIAN_POINT('Ctrl Pts',(42.9469753996782,3.96999998000001,-87.669671462365));
#170731=CARTESIAN_POINT('Ctrl Pts',(45.6032617662994,3.96999998000001,-82.3609901712845));
#170732=CARTESIAN_POINT('Ctrl Pts',(48.2402535232915,3.96999998000001,-77.0427269617097));
#170733=CARTESIAN_POINT('Ctrl Pts',(50.8772452802837,3.96999998000001,-71.724463752135));
#170734=CARTESIAN_POINT('Ctrl Pts',(53.4945730592583,3.96999998000001,-66.3964351916018));
#170735=CARTESIAN_POINT('Ctrl Pts',(56.0993680931338,3.96999998000001,-61.0621827299711));
#170736=CARTESIAN_POINT('Origin',(57.,3.46999998000001,-58.24995));
#170737=CARTESIAN_POINT('',(57.,3.96999998000001,-55.74995));
#170738=CARTESIAN_POINT('Origin',(57.,3.96999998000001,-58.24995));
#170739=CARTESIAN_POINT('',(57.,3.46999998000001,-55.24995));
#170740=CARTESIAN_POINT('Origin',(57.,3.46999998000001,-55.74995));
#170741=CARTESIAN_POINT('Origin',(57.,3.46999998000001,-58.24995));
#170742=CARTESIAN_POINT('Origin',(57.,-2.42462934179819E-14,-58.24995));
#170743=CARTESIAN_POINT('',(57.,2.96999998000001,-55.24995));
#170744=CARTESIAN_POINT('',(57.,28.41999998,-55.24995));
#170745=CARTESIAN_POINT('Origin',(57.,2.96999998000001,-58.24995));
#170746=CARTESIAN_POINT('Origin',(57.,2.96999998000001,-58.24995));
#170747=CARTESIAN_POINT('',(57.,2.46999998000001,-55.74995));
#170748=CARTESIAN_POINT('Origin',(57.,2.96999998000001,-55.74995));
#170749=CARTESIAN_POINT('',(59.5,2.46999998000001,-58.24995));
#170750=CARTESIAN_POINT('Origin',(57.,2.46999998000001,-58.24995));
#170751=CARTESIAN_POINT('Origin',(59.5,2.96999998000001,-58.24995));
#170752=CARTESIAN_POINT('Origin',(59.5,2.96999998000001,-55.24995));
#170753=CARTESIAN_POINT('',(59.5,2.46999998000001,-174.34995));
#170754=CARTESIAN_POINT('',(59.5,2.46999998000001,-58.24995));
#170755=CARTESIAN_POINT('Origin',(59.5,2.96999998000001,-174.34995));
#170756=CARTESIAN_POINT('Origin',(57.,2.96999998000001,-174.34995));
#170757=CARTESIAN_POINT('Origin',(57.,2.46999998000001,-174.34995));
#170758=CARTESIAN_POINT('Origin',(57.077763566464,1.96999998000001,-179.64995));
#170759=CARTESIAN_POINT('',(57.077763566464,2.46999998000001,-171.871644662643));
#170760=CARTESIAN_POINT('',(57.077763566464,2.46999998000001,-176.84995));
#170761=CARTESIAN_POINT('Origin',(57.077763566464,1.96999998000001,-171.871644662643));
#170762=CARTESIAN_POINT('',(56.5940537057312,1.84341099694893,-179.64995));
#170763=CARTESIAN_POINT('Ctrl Pts',(56.9026784671178,2.46999996978156,-171.178999526256));
#170764=CARTESIAN_POINT('Ctrl Pts',(56.3489175136905,2.47012711531616,-171.477038599322));
#170765=CARTESIAN_POINT('Ctrl Pts',(56.4736088945599,1.8573874935658,-171.409915902424));
#170766=CARTESIAN_POINT('Ctrl Pts',(57.0276127026275,2.4699999696149,-171.411480993498));
#170767=CARTESIAN_POINT('Ctrl Pts',(56.4096617452283,2.47013088089768,-171.619083147105));
#170768=CARTESIAN_POINT('Ctrl Pts',(56.5595092645592,1.84739527439962,-171.564880044108));
#170769=CARTESIAN_POINT('Ctrl Pts',(57.0884505381248,2.46999996953445,-171.671060999849));
#170770=CARTESIAN_POINT('Ctrl Pts',(56.4344504334064,2.4701327527474,-171.760758212924));
#170771=CARTESIAN_POINT('Ctrl Pts',(56.6013299245167,1.84257107601692,-171.737940501487));
#170772=CARTESIAN_POINT('Ctrl Pts',(57.0763566157493,2.46999996955045,-171.938278709053));
#170773=CARTESIAN_POINT('Ctrl Pts',(56.4294059961933,2.47013238231052,-171.908444781729));
#170774=CARTESIAN_POINT('Ctrl Pts',(56.5930162481435,1.8435307818068,-171.916062071863));
#170775=CARTESIAN_POINT('',(56.9324803875071,2.46999998000001,-171.237717270032));
#170776=CARTESIAN_POINT('Origin',(55.6391139723683,2.47000037313163,-171.847693896014));
#170777=CARTESIAN_POINT('Origin',(56.9324803875071,1.96999998000001,-171.237717270032));
#170778=CARTESIAN_POINT('Ctrl Pts',(40.1772697316389,2.46999998000002,-136.935824627502));
#170779=CARTESIAN_POINT('Ctrl Pts',(39.5564442323333,2.46999998000002,-137.244681069688));
#170780=CARTESIAN_POINT('Ctrl Pts',(39.7525219240432,1.81208306781681,-137.147133758372));
#170781=CARTESIAN_POINT('Ctrl Pts',(43.0113356415696,2.46999998000002,-142.632517793947));
#170782=CARTESIAN_POINT('Ctrl Pts',(42.3628976020159,2.46999998000001,-142.852500243629));
#170783=CARTESIAN_POINT('Ctrl Pts',(42.5829522730059,1.82186961480941,-142.84383290998));
#170784=CARTESIAN_POINT('Ctrl Pts',(45.8169723643538,2.46999998000002,-148.343102920422));
#170785=CARTESIAN_POINT('Ctrl Pts',(45.1914659347836,2.46999998002509,-148.581690034117));
#170786=CARTESIAN_POINT('Ctrl Pts',(45.385956606115,1.82990288117652,-148.554412051289));
#170787=CARTESIAN_POINT('Ctrl Pts',(51.3962007668006,2.46999998000001,-159.779920646508));
#170788=CARTESIAN_POINT('Ctrl Pts',(50.7878173967191,2.46999997997542,-160.008583439984));
#170789=CARTESIAN_POINT('Ctrl Pts',(50.9608945753704,1.84386393970469,-159.991229777381));
#170790=CARTESIAN_POINT('Ctrl Pts',(54.1694331140562,2.46999998000001,-165.506332215193));
#170791=CARTESIAN_POINT('Ctrl Pts',(53.5753070147928,2.46999998000001,-165.745313705806));
#170792=CARTESIAN_POINT('Ctrl Pts',(53.7324859673961,1.84977562860519,-165.717643463624));
#170793=CARTESIAN_POINT('Ctrl Pts',(56.9324803875071,2.46999998000001,-171.237717270032));
#170794=CARTESIAN_POINT('Ctrl Pts',(56.3632322083114,2.46999998,-171.512146507354));
#170795=CARTESIAN_POINT('Ctrl Pts',(56.4941621559325,1.85499746228791,-171.449026400902));
#170796=CARTESIAN_POINT('',(40.1772697316389,2.46999998000002,-136.935824627502));
#170797=CARTESIAN_POINT('Ctrl Pts',(40.1772697316389,2.46999998000002,-136.935824627502));
#170798=CARTESIAN_POINT('Ctrl Pts',(43.0113367121144,2.46999998000002,-142.632519945825));
#170799=CARTESIAN_POINT('Ctrl Pts',(45.8169723643453,2.46999998000002,-148.343102920405));
#170800=CARTESIAN_POINT('Ctrl Pts',(48.6065865655743,2.46999998000001,-154.061511783466));
#170801=CARTESIAN_POINT('Ctrl Pts',(51.3962007668033,2.46999998000001,-159.779920646528));
#170802=CARTESIAN_POINT('Ctrl Pts',(54.1694328122146,2.46999998000001,-165.506331589084));
#170803=CARTESIAN_POINT('Ctrl Pts',(56.9324803874897,2.46999998000001,-171.23771727004));
#170804=CARTESIAN_POINT('Origin',(40.1772697316389,1.96999998000002,-136.935824627502));
#170805=CARTESIAN_POINT('Ctrl Pts',(39.7525219240431,1.81208306781681,-137.147133758372));
#170806=CARTESIAN_POINT('Ctrl Pts',(39.5564442323333,2.46999998000002,-137.244681069688));
#170807=CARTESIAN_POINT('Ctrl Pts',(40.1772697316389,2.46999998000002,-136.935824627502));
#170808=CARTESIAN_POINT('Ctrl Pts',(39.5010130025154,1.83757362466031,-136.660631009723));
#170809=CARTESIAN_POINT('Ctrl Pts',(39.347413825743,2.46999998000002,-136.73953631121));
#170810=CARTESIAN_POINT('Ctrl Pts',(39.950904654581,2.46999998000002,-136.480813185142));
#170811=CARTESIAN_POINT('Ctrl Pts',(39.3161891891914,1.86369282090684,-136.153853436174));
#170812=CARTESIAN_POINT('Ctrl Pts',(39.1941245109705,2.46999998000001,-136.207552272104));
#170813=CARTESIAN_POINT('Ctrl Pts',(39.7845702702201,2.46999998000002,-136.007478819399));
#170814=CARTESIAN_POINT('Ctrl Pts',(39.0651099631573,1.91665698917066,-135.104438767164));
#170815=CARTESIAN_POINT('Ctrl Pts',(39.0102330104275,2.46999998000002,-135.126982248827));
#170816=CARTESIAN_POINT('Ctrl Pts',(39.5585989668938,2.46999998000002,-135.028737339162));
#170817=CARTESIAN_POINT('Ctrl Pts',(39.,1.94368731593243,-134.55780009522));
#170818=CARTESIAN_POINT('Ctrl Pts',(38.9729770085358,2.46999998000002,-134.572511021856));
#170819=CARTESIAN_POINT('Ctrl Pts',(39.5000000000492,2.46999998000002,-134.519624150969));
#170820=CARTESIAN_POINT('Ctrl Pts',(39.,1.96999998000002,-134.012863078852));
#170821=CARTESIAN_POINT('Ctrl Pts',(39.,2.46999998000002,-134.012863078852));
#170822=CARTESIAN_POINT('Ctrl Pts',(39.5,2.46999998000002,-134.012863078852));
#170823=CARTESIAN_POINT('',(39.5,2.46999998000002,-134.012863078852));
#170824=CARTESIAN_POINT('Ctrl Pts',(39.5,2.46999998000002,-134.012863078852));
#170825=CARTESIAN_POINT('Ctrl Pts',(39.5,2.46999998000002,-134.194202123599));
#170826=CARTESIAN_POINT('Ctrl Pts',(39.5074991738613,2.46999998000002,-134.375559257497));
#170827=CARTESIAN_POINT('Ctrl Pts',(39.5222608830473,2.46999998000002,-134.556078177936));
#170828=CARTESIAN_POINT('Ctrl Pts',(39.5372803972934,2.46999998000002,-134.739749761157));
#170829=CARTESIAN_POINT('Ctrl Pts',(39.5598184209786,2.46999998000002,-134.92255477599));
#170830=CARTESIAN_POINT('Ctrl Pts',(39.5896791401065,2.46999998000002,-135.10359544212));
#170831=CARTESIAN_POINT('Ctrl Pts',(39.6126641240196,2.46999998000002,-135.242949647919));
#170832=CARTESIAN_POINT('Ctrl Pts',(39.6399889131326,2.46999998000002,-135.381258722717));
#170833=CARTESIAN_POINT('Ctrl Pts',(39.671584618531,2.46999998000002,-135.518108079287));
#170834=CARTESIAN_POINT('Ctrl Pts',(39.7480265101501,2.46999998000002,-135.849198129379));
#170835=CARTESIAN_POINT('Ctrl Pts',(39.8488754308753,2.46999998000002,-136.172910839316));
#170836=CARTESIAN_POINT('Ctrl Pts',(39.9762245150674,2.46999998000002,-136.488613556872));
#170837=CARTESIAN_POINT('Ctrl Pts',(40.0371049338934,2.46999998000002,-136.639538188888));
#170838=CARTESIAN_POINT('Ctrl Pts',(40.1040424074826,2.46999998000002,-136.788632003769));
#170839=CARTESIAN_POINT('Ctrl Pts',(40.1772697316389,2.46999998000002,-136.935824627502));
#170840=CARTESIAN_POINT('Origin',(39.5,1.96999998000002,-134.012863078852));
#170841=CARTESIAN_POINT('Origin',(39.5,1.96999998000002,-55.24995));
#170842=CARTESIAN_POINT('',(39.5,2.46999998000002,-98.0457798926543));
#170843=CARTESIAN_POINT('',(39.5,2.46999998000002,-55.24995));
#170844=CARTESIAN_POINT('Origin',(39.5,1.96999998000002,-98.0457798926543));
#170845=CARTESIAN_POINT('Ctrl Pts',(39.,1.96999998000002,-98.0457798926543));
#170846=CARTESIAN_POINT('Ctrl Pts',(39.,2.46999998000002,-98.0457798926543));
#170847=CARTESIAN_POINT('Ctrl Pts',(39.5,2.46999998000002,-98.0457798926543));
#170848=CARTESIAN_POINT('Ctrl Pts',(39.,1.9436152588707,-97.4993505936135));
#170849=CARTESIAN_POINT('Ctrl Pts',(38.9728980858888,2.46999998000002,-97.4844974242186));
#170850=CARTESIAN_POINT('Ctrl Pts',(39.5000000026568,2.46999998000002,-97.5376233160284));
#170851=CARTESIAN_POINT('Ctrl Pts',(39.0635968999967,1.91714776114478,-96.9640681661487));
#170852=CARTESIAN_POINT('Ctrl Pts',(39.0092761144151,2.46999998000002,-96.9417291681898));
#170853=CARTESIAN_POINT('Ctrl Pts',(39.5572372093883,2.46999998000002,-97.0390962063516));
#170854=CARTESIAN_POINT('Ctrl Pts',(39.312853918045,1.86422808123875,-95.9152577284902));
#170855=CARTESIAN_POINT('Ctrl Pts',(39.1914722350304,2.46999998000002,-95.8620324116114));
#170856=CARTESIAN_POINT('Ctrl Pts',(39.7815685268491,2.46999998000002,-96.0609362825129));
#170857=CARTESIAN_POINT('Ctrl Pts',(39.5010226636067,1.83757264792979,-95.3979932721737));
#170858=CARTESIAN_POINT('Ctrl Pts',(39.3474064560569,2.46999998000002,-95.3191244694837));
#170859=CARTESIAN_POINT('Ctrl Pts',(39.9509186646822,2.46999998000002,-95.5778016189611));
#170860=CARTESIAN_POINT('Ctrl Pts',(39.7525219240431,1.81208306781681,-94.9115092131337));
#170861=CARTESIAN_POINT('Ctrl Pts',(39.5564442323333,2.46999998000002,-94.8139619018179));
#170862=CARTESIAN_POINT('Ctrl Pts',(40.1772697316389,2.46999998000002,-95.1228183440041));
#170863=CARTESIAN_POINT('',(40.177269731639,2.46999998000002,-95.1228183440042));
#170864=CARTESIAN_POINT('',(39.7525219090133,1.81208319014795,-94.9115093405122));
#170865=CARTESIAN_POINT('Origin',(40.1772697316389,1.96999998000002,-95.1228183440041));
#170866=CARTESIAN_POINT('Ctrl Pts',(39.0000000024628,1.96999998000006,-98.0457798926544));
#170867=CARTESIAN_POINT('Ctrl Pts',(39.0000023795683,1.96570120570202,-97.9567519908293));
#170868=CARTESIAN_POINT('Ctrl Pts',(39.0017233767913,1.96125307100217,-97.8646389244035));
#170869=CARTESIAN_POINT('Ctrl Pts',(39.0055233301077,1.95663173737879,-97.7695025339163));
#170870=CARTESIAN_POINT('Ctrl Pts',(39.006999653108,1.9548362992372,-97.7325410162995));
#170871=CARTESIAN_POINT('Ctrl Pts',(39.0087900561879,1.95301496883546,-97.6951235500827));
#170872=CARTESIAN_POINT('Ctrl Pts',(39.0109166836443,1.95116738479208,-97.657255353352));
#170873=CARTESIAN_POINT('Ctrl Pts',(39.0147168933816,1.94786581598601,-97.5895861950714));
#170874=CARTESIAN_POINT('Ctrl Pts',(39.0195904985651,1.94447998345472,-97.5204771269352));
#170875=CARTESIAN_POINT('Ctrl Pts',(39.025667717316,1.94101327943105,-97.4499659367276));
#170876=CARTESIAN_POINT('Ctrl Pts',(39.0287063266914,1.93927992741922,-97.4147103416238));
#170877=CARTESIAN_POINT('Ctrl Pts',(39.0320459334948,1.93752636333294,-97.3791042242764));
#170878=CARTESIAN_POINT('Ctrl Pts',(39.0357031841201,1.9357538621328,-97.3431535242875));
#170879=CARTESIAN_POINT('Ctrl Pts',(39.0375318094328,1.93486761153271,-97.3251781742931));
#170880=CARTESIAN_POINT('Ctrl Pts',(39.0394398505803,1.93397662688184,-97.3071166789648));
#170881=CARTESIAN_POINT('Ctrl Pts',(39.0414294116136,1.93308109865202,-97.2889698225087));
#170882=CARTESIAN_POINT('Ctrl Pts',(39.0424241921302,1.9326333345371,-97.2798963942806));
#170883=CARTESIAN_POINT('Ctrl Pts',(39.043439352924,1.93218443455118,-97.2708016258043));
#170884=CARTESIAN_POINT('Ctrl Pts',(39.0444751581284,1.93173442564936,-97.2616856194871));
#170885=CARTESIAN_POINT('Ctrl Pts',(39.0449930607306,1.93150942119844,-97.2571276163284));
#170886=CARTESIAN_POINT('Ctrl Pts',(39.0455161244538,1.93128413951999,-97.2525643037117));
#170887=CARTESIAN_POINT('Ctrl Pts',(39.0460443823768,1.93105858419778,-97.2479956947328));
#170888=CARTESIAN_POINT('Ctrl Pts',(39.0465726402997,1.93083302887557,-97.2434270857539));
#170889=CARTESIAN_POINT('Ctrl Pts',(39.0472468859898,1.9305481048655,-97.2376563271244));
#170890=CARTESIAN_POINT('Ctrl Pts',(39.0476447718804,1.93038110095292,-97.2342739919009));
#170891=CARTESIAN_POINT('Ctrl Pts',(39.0547397971647,1.92740311904867,-97.1739608355568));
#170892=CARTESIAN_POINT('Ctrl Pts',(39.0630811872692,1.92424565323167,-97.109804789609));
#170893=CARTESIAN_POINT('Ctrl Pts',(39.0729996746766,1.92088476300344,-97.0418531112313));
#170894=CARTESIAN_POINT('Ctrl Pts',(39.0826231429977,1.91762384031288,-96.9759226122161));
#170895=CARTESIAN_POINT('Ctrl Pts',(39.0937316247875,1.91417106351811,-96.9064185529857));
#170896=CARTESIAN_POINT('Ctrl Pts',(39.1066630521812,1.9105202065299,-96.8334125920886));
#170897=CARTESIAN_POINT('Ctrl Pts',(39.1162799426628,1.90780512406058,-96.7791192562424));
#170898=CARTESIAN_POINT('Ctrl Pts',(39.1269058081946,1.90498076441849,-96.7228896719113));
#170899=CARTESIAN_POINT('Ctrl Pts',(39.1386912625358,1.90205227654554,-96.6647659242202));
#170900=CARTESIAN_POINT('Ctrl Pts',(39.1460189431004,1.90023147074128,-96.6286271175209));
#170901=CARTESIAN_POINT('Ctrl Pts',(39.1537950911084,1.89837054965722,-96.5917562863848));
#170902=CARTESIAN_POINT('Ctrl Pts',(39.1620576208011,1.89647235503082,-96.5541660084023));
#170903=CARTESIAN_POINT('Ctrl Pts',(39.1661888856474,1.89552325771762,-96.5353708694111));
#170904=CARTESIAN_POINT('Ctrl Pts',(39.1704417732556,1.89456484623122,-96.5163958745825));
#170905=CARTESIAN_POINT('Ctrl Pts',(39.1748211237916,1.89359762560557,-96.4972428190492));
#170906=CARTESIAN_POINT('Ctrl Pts',(39.1770107990596,1.89311401529275,-96.4876662912825));
#170907=CARTESIAN_POINT('Ctrl Pts',(39.179232091689,1.89262820293435,-96.4780452486739));
#170908=CARTESIAN_POINT('Ctrl Pts',(39.18148561435,1.89214025762443,-96.4683799240122));
#170909=CARTESIAN_POINT('Ctrl Pts',(39.1826123756804,1.89189628496947,-96.4635472616813));
#170910=CARTESIAN_POINT('Ctrl Pts',(39.1837471946203,1.89165177909316,-96.4587035288602));
#170911=CARTESIAN_POINT('Ctrl Pts',(39.1848901481332,1.89140674918914,-96.4538487554583));
#170912=CARTESIAN_POINT('Ctrl Pts',(39.1854616248896,1.89128423423713,-96.4514213687574));
#170913=CARTESIAN_POINT('Ctrl Pts',(39.1860351352956,1.89116158827922,-96.4489912219127));
#170914=CARTESIAN_POINT('Ctrl Pts',(39.1866106889937,1.89103881250212,-96.4465583187171));
#170915=CARTESIAN_POINT('Ctrl Pts',(39.1871862426919,1.89091603672502,-96.4441254155214));
#170916=CARTESIAN_POINT('Ctrl Pts',(39.1874086280478,1.89086852694691,-96.4431840239398));
#170917=CARTESIAN_POINT('Ctrl Pts',(39.1883434896272,1.89067009691365,-96.4392513438899));
#170918=CARTESIAN_POINT('Ctrl Pts',(39.2039030113169,1.88736749418148,-96.373797139888));
#170919=CARTESIAN_POINT('Ctrl Pts',(39.2194686344583,1.88423223388531,-96.3125811755131));
#170920=CARTESIAN_POINT('Ctrl Pts',(39.234696896302,1.8812995042039,-96.2555688744947));
#170921=CARTESIAN_POINT('Ctrl Pts',(39.2500971432766,1.87833365282396,-96.1979126872501));
#170922=CARTESIAN_POINT('Ctrl Pts',(39.2651521559665,1.87557453440026,-96.1445550998185));
#170923=CARTESIAN_POINT('Ctrl Pts',(39.2795546795664,1.87303882497464,-96.0954463781737));
#170924=CARTESIAN_POINT('Ctrl Pts',(39.2940772709897,1.8704819763987,-96.045928257629));
#170925=CARTESIAN_POINT('Ctrl Pts',(39.3079363553328,1.86815189115088,-96.0007296292346));
#170926=CARTESIAN_POINT('Ctrl Pts',(39.3208676806068,1.86605171503959,-95.9597934618329));
#170927=CARTESIAN_POINT('Ctrl Pts',(39.3338976046489,1.86393552550563,-95.9185451643449));
#170928=CARTESIAN_POINT('Ctrl Pts',(39.3459855447184,1.86205241809051,-95.8816241304791));
#170929=CARTESIAN_POINT('Ctrl Pts',(39.3569133198007,1.86039707135961,-95.8489731675027));
#170930=CARTESIAN_POINT('Ctrl Pts',(39.3678631601099,1.85873838217327,-95.8162562761098));
#170931=CARTESIAN_POINT('Ctrl Pts',(39.3776482049348,1.85730808413837,-95.7878263605496));
#170932=CARTESIAN_POINT('Ctrl Pts',(39.3861007469163,1.85609710073972,-95.7636330869288));
#170933=CARTESIAN_POINT('Ctrl Pts',(39.3945648893821,1.85488445535656,-95.7394066098418));
#170934=CARTESIAN_POINT('Ctrl Pts',(39.401692939157,1.85389150890907,-95.7194281489415));
#170935=CARTESIAN_POINT('Ctrl Pts',(39.4073673786352,1.8531092421283,-95.7036590330933));
#170936=CARTESIAN_POINT('Ctrl Pts',(39.4107258929006,1.85264624412601,-95.6943258115951));
#170937=CARTESIAN_POINT('Ctrl Pts',(39.4135761564115,1.852257070151,-95.6864674008105));
#170938=CARTESIAN_POINT('Ctrl Pts',(39.4159020403612,1.85194027203048,-95.6800782245838));
#170939=CARTESIAN_POINT('Ctrl Pts',(39.4177341500928,1.85169072866027,-95.675045440406));
#170940=CARTESIAN_POINT('Ctrl Pts',(39.4192410137785,1.85148609903756,-95.6709243205286));
#170941=CARTESIAN_POINT('Ctrl Pts',(39.4204173925654,1.85132587896651,-95.6677130149262));
#170942=CARTESIAN_POINT('Ctrl Pts',(39.4210055819589,1.85124576893097,-95.6661073621251));
#170943=CARTESIAN_POINT('Ctrl Pts',(39.4215111848868,1.8511767702981,-95.6647291751866));
#170944=CARTESIAN_POINT('Ctrl Pts',(39.4219337654556,1.85111883252293,-95.6635782981435));
#170945=CARTESIAN_POINT('Ctrl Pts',(39.42214505574,1.85108986363535,-95.6630028596219));
#170946=CARTESIAN_POINT('Ctrl Pts',(39.4223355926106,1.85106366052513,-95.6624842493419));
#170947=CARTESIAN_POINT('Ctrl Pts',(39.4225053348427,1.85104021921531,-95.662022452596));
#170948=CARTESIAN_POINT('Ctrl Pts',(39.4225902059587,1.85102849856041,-95.6617915542231));
#170949=CARTESIAN_POINT('Ctrl Pts',(39.422669878551,1.85101746839093,-95.6615748592819));
#170950=CARTESIAN_POINT('Ctrl Pts',(39.422744348315,1.8510071282838,-95.6613723662314));
#170951=CARTESIAN_POINT('Ctrl Pts',(39.422781583197,1.85100195823023,-95.6612711197062));
#170952=CARTESIAN_POINT('Ctrl Pts',(39.4228175174062,1.85099696069703,-95.6611734236659));
#170953=CARTESIAN_POINT('Ctrl Pts',(39.4228514987551,1.85099222175874,-95.661081052689));
#170954=CARTESIAN_POINT('Ctrl Pts',(39.4228854801041,1.85098748282044,-95.6609886817121));
#170955=CARTESIAN_POINT('Ctrl Pts',(39.4229187089809,1.85098281980264,-95.6608980492788));
#170956=CARTESIAN_POINT('Ctrl Pts',(39.4233430620384,1.85092351009055,-95.6597454129));
#170957=CARTESIAN_POINT('Ctrl Pts',(39.4544661950375,1.84657358489319,-95.5752081280062));
#170958=CARTESIAN_POINT('Ctrl Pts',(39.4861260597182,1.84238472192749,-95.4944667312749));
#170959=CARTESIAN_POINT('Ctrl Pts',(39.5179232619264,1.8383884084295,-95.417491701329));
#170960=CARTESIAN_POINT('Ctrl Pts',(39.5502997984827,1.83431928344136,-95.3391142121822));
#170961=CARTESIAN_POINT('Ctrl Pts',(39.5828183403341,1.8304494528387,-95.264641080767));
#170962=CARTESIAN_POINT('Ctrl Pts',(39.6150932788069,1.82678245847445,-95.1940123862938));
#170963=CARTESIAN_POINT('Ctrl Pts',(39.6482525478298,1.82301498877866,-95.1214484716407));
#170964=CARTESIAN_POINT('Ctrl Pts',(39.6811543457219,1.8194612646841,-95.0529420298684));
#170965=CARTESIAN_POINT('Ctrl Pts',(39.7134238132575,1.8160993657089,-94.9884058941551));
#170966=CARTESIAN_POINT('Ctrl Pts',(39.7265686486177,1.81472990993844,-94.9621173637418));
#170967=CARTESIAN_POINT('Ctrl Pts',(39.7396090786083,1.81339202353714,-94.9364874232129));
#170968=CARTESIAN_POINT('Ctrl Pts',(39.7525219085452,1.81208326361859,-94.911509475135));
#170969=CARTESIAN_POINT('Ctrl Pts',(40.1772697316388,2.46999998000002,-95.1228183440041));
#170970=CARTESIAN_POINT('Ctrl Pts',(40.0557143101432,2.46999998000002,-95.367154206676));
#170971=CARTESIAN_POINT('Ctrl Pts',(39.9506490904769,2.46999998000002,-95.6194942161999));
#170972=CARTESIAN_POINT('Ctrl Pts',(39.862036785698,2.46999998000002,-95.876484568063));
#170973=CARTESIAN_POINT('Ctrl Pts',(39.785571796048,2.46999998000002,-96.0982456953059));
#170974=CARTESIAN_POINT('Ctrl Pts',(39.721358807228,2.46999998000002,-96.3234708895919));
#170975=CARTESIAN_POINT('Ctrl Pts',(39.6694028678064,2.46999998000002,-96.5500162443606));
#170976=CARTESIAN_POINT('Ctrl Pts',(39.5883957972391,2.46999998000002,-96.903234293053));
#170977=CARTESIAN_POINT('Ctrl Pts',(39.5360425809489,2.46999998000002,-97.2613436845068));
#170978=CARTESIAN_POINT('Ctrl Pts',(39.5132030141794,2.46999998000002,-97.624491207193));
#170979=CARTESIAN_POINT('Ctrl Pts',(39.5044179952615,2.46999998000002,-97.7641723968143));
#170980=CARTESIAN_POINT('Ctrl Pts',(39.5,2.46999998000002,-97.9045990595786));
#170981=CARTESIAN_POINT('Ctrl Pts',(39.5,2.46999998000002,-98.0457798926543));
#170982=CARTESIAN_POINT('Ctrl Pts',(56.8241336558648,2.46999998000001,-61.0456553781473));
#170983=CARTESIAN_POINT('Ctrl Pts',(56.2546351764993,2.46999997999971,-60.771071756775));
#170984=CARTESIAN_POINT('Ctrl Pts',(56.3858722762367,1.85477834326924,-60.8343476935333));
#170985=CARTESIAN_POINT('Ctrl Pts',(54.0775409927178,2.46999998000001,-66.7422070144501));
#170986=CARTESIAN_POINT('Ctrl Pts',(53.4833299990046,2.46999998010366,-66.5027538223377));
#170987=CARTESIAN_POINT('Ctrl Pts',(53.6406504195319,1.84956966069372,-66.5308964372918));
#170988=CARTESIAN_POINT('Ctrl Pts',(51.3208277321712,2.46999998000001,-72.433816174677));
#170989=CARTESIAN_POINT('Ctrl Pts',(50.7124694309102,2.46999998,-72.2045026335238));
#170990=CARTESIAN_POINT('Ctrl Pts',(50.8855763842636,1.84367574323028,-72.2225074476142));
#170991=CARTESIAN_POINT('Ctrl Pts',(45.7749111060821,2.46999998000002,-83.8011613014347));
#170992=CARTESIAN_POINT('Ctrl Pts',(45.1494935787875,2.46999998,-83.5619433099981));
#170993=CARTESIAN_POINT('Ctrl Pts',(45.3439391239116,1.82976876705617,-83.5898527848085));
#170994=CARTESIAN_POINT('Ctrl Pts',(42.9860576374377,2.46999998000002,-89.47707155374));
#170995=CARTESIAN_POINT('Ctrl Pts',(42.3379617991063,2.4699999799188,-89.2560712524343));
#170996=CARTESIAN_POINT('Ctrl Pts',(42.5577095805282,1.8217713755538,-89.2657567838175));
#170997=CARTESIAN_POINT('Ctrl Pts',(40.1690969821091,2.46999998000002,-95.1392460099596));
#170998=CARTESIAN_POINT('Ctrl Pts',(39.5482160849935,2.46999998000026,-94.8303544504712));
#170999=CARTESIAN_POINT('Ctrl Pts',(39.7443638707198,1.81204072079829,-94.9279389902309));
#171000=CARTESIAN_POINT('',(56.8161649572467,2.46999998000001,-61.0621827299711));
#171001=CARTESIAN_POINT('',(56.377904566775,1.85477723331148,-60.8508735991007));
#171002=CARTESIAN_POINT('Origin',(56.8161649572467,1.96999998000001,-61.0621827299711));
#171003=CARTESIAN_POINT('Ctrl Pts',(39.7525219240432,1.8120830678168,-94.9115092131337));
#171004=CARTESIAN_POINT('Ctrl Pts',(41.0321872437539,1.8165076616864,-92.3359756573271));
#171005=CARTESIAN_POINT('Ctrl Pts',(42.3688267391817,1.8209983325356,-89.6310450958057));
#171006=CARTESIAN_POINT('Ctrl Pts',(44.4594400294678,1.82716626150394,-85.3795537449517));
#171007=CARTESIAN_POINT('Ctrl Pts',(45.1705837525141,1.82914107837277,-83.9300407099051));
#171008=CARTESIAN_POINT('Ctrl Pts',(46.2587091665782,1.83202090427287,-81.7072472801921));
#171009=CARTESIAN_POINT('Ctrl Pts',(46.808124123156,1.83344150427555,-80.5837195960498));
#171010=CARTESIAN_POINT('Ctrl Pts',(47.4584728770403,1.83508731520312,-79.2517081016338));
#171011=CARTESIAN_POINT('Ctrl Pts',(47.7859880572214,1.8359111325951,-78.5803950553633));
#171012=CARTESIAN_POINT('Ctrl Pts',(47.9679389518065,1.83636798435703,-78.2073063487587));
#171013=CARTESIAN_POINT('Ctrl Pts',(48.0561756206575,1.83658937557106,-78.0263353058769));
#171014=CARTESIAN_POINT('Ctrl Pts',(48.1032839361376,1.83670755389347,-77.9297068476094));
#171015=CARTESIAN_POINT('Ctrl Pts',(48.1100653589499,1.83672456568112,-77.9157965646182));
#171016=CARTESIAN_POINT('Ctrl Pts',(50.6741769084835,1.84315675199189,-72.6561333006624));
#171017=CARTESIAN_POINT('Ctrl Pts',(53.4284137093914,1.84917961846372,-66.9712432304567));
#171018=CARTESIAN_POINT('Ctrl Pts',(56.377904566775,1.85477723331148,-60.8508735991007));
#171019=CARTESIAN_POINT('Ctrl Pts',(56.8161649572467,2.46999998000001,-61.0621827299711));
#171020=CARTESIAN_POINT('Ctrl Pts',(54.0722086604215,2.46999998000001,-66.7532163030615));
#171021=CARTESIAN_POINT('Ctrl Pts',(51.3181460106093,2.46999998000001,-72.4393128412014));
#171022=CARTESIAN_POINT('Ctrl Pts',(48.5478694191173,2.46999998000001,-78.1174887380514));
#171023=CARTESIAN_POINT('Ctrl Pts',(45.7775928276252,2.46999998000002,-83.7956646349013));
#171024=CARTESIAN_POINT('Ctrl Pts',(42.9914528488282,2.46999998000002,-89.4660911391003));
#171025=CARTESIAN_POINT('Ctrl Pts',(40.1772697316389,2.46999998000002,-95.1228183440041));
#171026=CARTESIAN_POINT('Ctrl Pts',(39.,3.43040799630139,-96.9953075914435));
#171027=CARTESIAN_POINT('Ctrl Pts',(39.,2.57465910981969,-95.8526291198646));
#171028=CARTESIAN_POINT('Ctrl Pts',(39.7537608994937,1.84791623342104,-94.8822119187994));
#171029=CARTESIAN_POINT('Ctrl Pts',(39.,2.33014533501219,-97.8192913905431));
#171030=CARTESIAN_POINT('Ctrl Pts',(38.999999999981,1.53000434811038,-96.6793434201897));
#171031=CARTESIAN_POINT('Ctrl Pts',(39.7190156956536,0.840907950229365,
-95.7061778087214));
#171032=CARTESIAN_POINT('Ctrl Pts',(39.,1.18987438490308,-98.6014496888564));
#171033=CARTESIAN_POINT('Ctrl Pts',(39.,0.446333199097853,-97.4659491905239));
#171034=CARTESIAN_POINT('Ctrl Pts',(39.6851690092259,-0.199333099759264,
-96.4883539675537));
#171035=CARTESIAN_POINT('Ctrl Pts',(39.,-0.603530653465397,-99.6882419580977));
#171036=CARTESIAN_POINT('Ctrl Pts',(39.,-1.25780446014918,-98.559487559907));
#171037=CARTESIAN_POINT('Ctrl Pts',(39.6371434881247,-1.8297111910827,-97.5751461950565));
#171038=CARTESIAN_POINT('Ctrl Pts',(39.,-1.21720470538169,-100.036841989918));
#171039=CARTESIAN_POINT('Ctrl Pts',(39.0000000000024,-1.84018826968395,
-98.9100164272499));
#171040=CARTESIAN_POINT('Ctrl Pts',(39.6215593402708,-2.38668766534493,
-97.9237462143533));
#171041=CARTESIAN_POINT('Ctrl Pts',(39.,-2.45808495944723,-100.689411149812));
#171042=CARTESIAN_POINT('Ctrl Pts',(38.9999999999976,-3.01723045502807,
-99.5661131270649));
#171043=CARTESIAN_POINT('Ctrl Pts',(39.5921043556329,-3.51112289490215,
-98.5763153513056));
#171044=CARTESIAN_POINT('Ctrl Pts',(39.,-3.08699664896505,-100.99454469153));
#171045=CARTESIAN_POINT('Ctrl Pts',(39.,-3.61357786082266,-99.8729679343378));
#171046=CARTESIAN_POINT('Ctrl Pts',(39.5781831338039,-4.08013648047372,
-98.8814488059413));
#171047=CARTESIAN_POINT('Ctrl Pts',(39.,-3.72540427022208,-101.27597320326));
#171048=CARTESIAN_POINT('Ctrl Pts',(39.,-4.21906468716858,-100.156127274739));
#171049=CARTESIAN_POINT('Ctrl Pts',(39.565238633238,-4.65691791624337,-99.1628773826332));
#171050=CARTESIAN_POINT('',(39.5857301728914,-3.7824234709496,-98.7152328423687));
#171051=CARTESIAN_POINT('Ctrl Pts',(39.5857305622805,-3.78242133832598,
-98.7152357168537));
#171052=CARTESIAN_POINT('Ctrl Pts',(39.5925013633664,-3.50507902913527,
-98.566659849342));
#171053=CARTESIAN_POINT('Ctrl Pts',(39.5995343541385,-3.22737884836422,
-98.4116495172459));
#171054=CARTESIAN_POINT('Ctrl Pts',(39.6068290975047,-2.94890292239653,
-98.2500352611615));
#171055=CARTESIAN_POINT('Ctrl Pts',(39.6124208939522,-2.73543678447178,
-98.1261496112259));
#171056=CARTESIAN_POINT('Ctrl Pts',(39.6181738810536,-2.52128731141673,
-97.9982124747704));
#171057=CARTESIAN_POINT('Ctrl Pts',(39.6240733158027,-2.30678756415044,
-97.8664764985964));
#171058=CARTESIAN_POINT('Ctrl Pts',(39.6296232126047,-2.10499679740912,
-97.7425457994774));
#171059=CARTESIAN_POINT('Ctrl Pts',(39.6353027291037,-1.90289595837455,
-97.6152528102953));
#171060=CARTESIAN_POINT('Ctrl Pts',(39.6410984012804,-1.70080336620325,
-97.484827319336));
#171061=CARTESIAN_POINT('Ctrl Pts',(39.6450625324154,-1.56257582117692,
-97.3956187282123));
#171062=CARTESIAN_POINT('Ctrl Pts',(39.6490809808139,-1.42435295854234,
-97.3049450480543));
#171063=CARTESIAN_POINT('Ctrl Pts',(39.6531490421426,-1.28624913053006,
-97.212886559647));
#171064=CARTESIAN_POINT('Ctrl Pts',(39.6682655575824,-0.773068900499357,
-96.8708062789114));
#171065=CARTESIAN_POINT('Ctrl Pts',(39.6840971342397,-0.259895270686603,
-96.5089494827552));
#171066=CARTESIAN_POINT('Ctrl Pts',(39.7006573795269,0.255684130879655,
-96.1258675663254));
#171067=CARTESIAN_POINT('Ctrl Pts',(39.7124916438098,0.624126916064151,
-95.8521099883181));
#171068=CARTESIAN_POINT('Ctrl Pts',(39.7246979184353,0.993796081660326,
-95.5675100901926));
#171069=CARTESIAN_POINT('Ctrl Pts',(39.7372758034841,1.36558709194006,-95.2715490323558));
#171070=CARTESIAN_POINT('Ctrl Pts',(39.742298747403,1.5140608128363,-95.1533577951219));
#171071=CARTESIAN_POINT('Ctrl Pts',(39.7473808898758,1.66287325720136,-95.0333550182876));
#171072=CARTESIAN_POINT('Ctrl Pts',(39.7525219085452,1.81208326361858,-94.911509475135));
#171073=CARTESIAN_POINT('Ctrl Pts',(39.5857320339139,-3.78242364196796,
-98.7152337592039));
#171074=CARTESIAN_POINT('Ctrl Pts',(39.5647695935044,-3.78057566286457,
-98.758128723926));
#171075=CARTESIAN_POINT('Ctrl Pts',(39.5426881139166,-3.7785869067278,-98.8046816267017));
#171076=CARTESIAN_POINT('Ctrl Pts',(39.519765128284,-3.77644182021921,-98.8550122588158));
#171077=CARTESIAN_POINT('Ctrl Pts',(39.501693369924,-3.7747507017207,-98.894691340601));
#171078=CARTESIAN_POINT('Ctrl Pts',(39.4830995277155,-3.77296247279516,
-98.9367185702283));
#171079=CARTESIAN_POINT('Ctrl Pts',(39.4641420358889,-3.77107389124137,
-98.9811511179016));
#171080=CARTESIAN_POINT('Ctrl Pts',(39.4426398204678,-3.76893179946144,
-99.0315479858268));
#171081=CARTESIAN_POINT('Ctrl Pts',(39.4206691128835,-3.76666025515081,
-99.0850397431287));
#171082=CARTESIAN_POINT('Ctrl Pts',(39.3984931481515,-3.76426354211129,
-99.1417019859204));
#171083=CARTESIAN_POINT('Ctrl Pts',(39.3874051657855,-3.76306518559153,
-99.1700331073162));
#171084=CARTESIAN_POINT('Ctrl Pts',(39.3762664009185,-3.76183569968917,
-99.199156695867));
#171085=CARTESIAN_POINT('Ctrl Pts',(39.3651129498974,-3.76057674596568,
-99.2290809819656));
#171086=CARTESIAN_POINT('Ctrl Pts',(39.3595362243869,-3.75994726910395,
-99.2440431250149));
#171087=CARTESIAN_POINT('Ctrl Pts',(39.3539558493515,-3.7593104214926,-99.2592054504292));
#171088=CARTESIAN_POINT('Ctrl Pts',(39.3483765482337,-3.75866651196756,
-99.2745688609028));
#171089=CARTESIAN_POINT('Ctrl Pts',(39.3455868976748,-3.75834455720504,
-99.2822505661396));
#171090=CARTESIAN_POINT('Ctrl Pts',(39.3427975168664,-3.75802083673782,
-99.2899825431161));
#171091=CARTESIAN_POINT('Ctrl Pts',(39.3400090065945,-3.75769539178263,
-99.2977649015877));
#171092=CARTESIAN_POINT('Ctrl Pts',(39.3386147514586,-3.75753266930503,
-99.3016560808235));
#171093=CARTESIAN_POINT('Ctrl Pts',(39.3372207140364,-3.75736951569224,
-99.3055598554609));
#171094=CARTESIAN_POINT('Ctrl Pts',(39.335826970206,-3.75720593647556,-99.3094762387292));
#171095=CARTESIAN_POINT('Ctrl Pts',(39.3344332263756,-3.75704235725887,
-99.3133926219975));
#171096=CARTESIAN_POINT('Ctrl Pts',(39.3335565762715,-3.75693935012291,
-99.3158593676638));
#171097=CARTESIAN_POINT('Ctrl Pts',(39.3316466957756,-3.75671392763538,
-99.3212632275588));
#171098=CARTESIAN_POINT('Ctrl Pts',(39.3120453395123,-3.75440038681578,
-99.3767237567527));
#171099=CARTESIAN_POINT('Ctrl Pts',(39.2945611211606,-3.75221686724286,
-99.4288752600496));
#171100=CARTESIAN_POINT('Ctrl Pts',(39.2788945448127,-3.75018391351401,
-99.4775817224279));
#171101=CARTESIAN_POINT('Ctrl Pts',(39.2630442479134,-3.74812711951709,
-99.5268593611707));
#171102=CARTESIAN_POINT('Ctrl Pts',(39.249054055268,-3.7462241551025,-99.5726111325386));
#171103=CARTESIAN_POINT('Ctrl Pts',(39.2366499945523,-3.74448358754834,
-99.6147331608509));
#171104=CARTESIAN_POINT('Ctrl Pts',(39.2240969536772,-3.74272211474086,
-99.657361099819));
#171105=CARTESIAN_POINT('Ctrl Pts',(39.2131680464728,-3.74112669492314,
-99.6962720163725));
#171106=CARTESIAN_POINT('Ctrl Pts',(39.2036218248227,-3.73969751603952,
-99.7313891637658));
#171107=CARTESIAN_POINT('Ctrl Pts',(39.1940360201446,-3.73826241112255,
-99.7666519230126));
#171108=CARTESIAN_POINT('Ctrl Pts',(39.1858442044626,-3.73699469031387,
-99.7980898058902));
#171109=CARTESIAN_POINT('Ctrl Pts',(39.178848316674,-3.7358896890291,-99.82564954893));
#171110=CARTESIAN_POINT('Ctrl Pts',(39.1718273274359,-3.7347807229675,-99.8533081771318));
#171111=CARTESIAN_POINT('Ctrl Pts',(39.1660107449371,-3.73383545695238,
-99.8770611283396));
#171112=CARTESIAN_POINT('Ctrl Pts',(39.1612472807937,-3.73304752251837,
-99.8968733708105));
#171113=CARTESIAN_POINT('Ctrl Pts',(39.1595812339107,-3.73277193826534,
-99.9038028078379));
#171114=CARTESIAN_POINT('Ctrl Pts',(39.1580444579001,-3.73251559828333,
-99.910250327255));
#171115=CARTESIAN_POINT('Ctrl Pts',(39.1566319198793,-3.73227824181624,
-99.9162148626195));
#171116=CARTESIAN_POINT('Ctrl Pts',(39.1551064101022,-3.73202190208881,
-99.922656428709));
#171117=CARTESIAN_POINT('Ctrl Pts',(39.1537257931825,-3.73178770267067,
-99.9285346636997));
#171118=CARTESIAN_POINT('Ctrl Pts',(39.1524847145106,-3.73157534599519,
-99.9338484768152));
#171119=CARTESIAN_POINT('Ctrl Pts',(39.1518641751747,-3.73146916765746,
-99.936505383373));
#171120=CARTESIAN_POINT('Ctrl Pts',(39.15127853624,-3.73136844832386,-99.9390211880862));
#171121=CARTESIAN_POINT('Ctrl Pts',(39.1507272247462,-3.73127315735143,
-99.9413957776894));
#171122=CARTESIAN_POINT('Ctrl Pts',(39.1504515689993,-3.73122551186521,
-99.9425830724911));
#171123=CARTESIAN_POINT('Ctrl Pts',(39.1501844960998,-3.73117922336374,
-99.9437350637426));
#171124=CARTESIAN_POINT('Ctrl Pts',(39.1499259404233,-3.73113428790966,
-99.9448517385624));
#171125=CARTESIAN_POINT('Ctrl Pts',(39.1497966625851,-3.73111182018261,
-99.9454100759722));
#171126=CARTESIAN_POINT('Ctrl Pts',(39.1496695141143,-3.7310896907109,-99.9459595842882));
#171127=CARTESIAN_POINT('Ctrl Pts',(39.1495444871842,-3.73106789902453,
-99.9465002619851));
#171128=CARTESIAN_POINT('Ctrl Pts',(39.1495132304517,-3.73106245110294,
-99.9466354314093));
#171129=CARTESIAN_POINT('Ctrl Pts',(39.1495030287109,-3.73106067541122,
-99.946679562838));
#171130=CARTESIAN_POINT('Ctrl Pts',(39.1494981838382,-3.73105983425694,
-99.9467005194));
#171131=CARTESIAN_POINT('Ctrl Pts',(39.1494945501837,-3.73105920339123,
-99.9467162368216));
#171132=CARTESIAN_POINT('Ctrl Pts',(39.1494939304581,-3.73105909813003,
-99.9467189185376));
#171133=CARTESIAN_POINT('Ctrl Pts',(39.1494897051637,-3.731058363178,-99.94673719502));
#171134=CARTESIAN_POINT('Ctrl Pts',(39.1494770292805,-3.73105615832187,
-99.9467920244674));
#171135=CARTESIAN_POINT('Ctrl Pts',(39.1494318011524,-3.73104829699593,
-99.9469871836392));
#171136=CARTESIAN_POINT('Ctrl Pts',(39.1491757634381,-3.73100353684427,
-99.9480958017481));
#171137=CARTESIAN_POINT('Ctrl Pts',(39.1280875954373,-3.72731693309337,
-100.039405494116));
#171138=CARTESIAN_POINT('Ctrl Pts',(39.109772797189,-3.72369719320944,-100.128756426151));
#171139=CARTESIAN_POINT('Ctrl Pts',(39.0939077592067,-3.72018651132105,
-100.215952276152));
#171140=CARTESIAN_POINT('Ctrl Pts',(39.077695335567,-3.71659895848302,-100.305057392788));
#171141=CARTESIAN_POINT('Ctrl Pts',(39.0640405428947,-3.71312512146226,
-100.391912157614));
#171142=CARTESIAN_POINT('Ctrl Pts',(39.0526011972676,-3.70978648587783,
-100.476356109603));
#171143=CARTESIAN_POINT('Ctrl Pts',(39.0407653272854,-3.70633212249175,
-100.563727159407));
#171144=CARTESIAN_POINT('Ctrl Pts',(39.0313005753357,-3.70302232059837,
-100.648517517554));
#171145=CARTESIAN_POINT('Ctrl Pts',(39.0238403729853,-3.69985856977579,
-100.730599277938));
#171146=CARTESIAN_POINT('Ctrl Pts',(39.0162275336137,-3.69663008806803,
-100.814360445235));
#171147=CARTESIAN_POINT('Ctrl Pts',(39.0107016304485,-3.69355343458246,
-100.89530140222));
#171148=CARTESIAN_POINT('Ctrl Pts',(39.0068940598651,-3.69061080968657,
-100.973333128231));
#171149=CARTESIAN_POINT('Ctrl Pts',(39.0029720963335,-3.68757977788401,
-101.053709204528));
#171150=CARTESIAN_POINT('Ctrl Pts',(39.0008728253103,-3.68469068702846,
-101.130998989905));
#171151=CARTESIAN_POINT('Ctrl Pts',(39.0002225969439,-3.68190774101026,
-101.205148883042));
#171152=CARTESIAN_POINT('Ctrl Pts',(39.0000727567577,-3.68126643224657,
-101.222236162488));
#171153=CARTESIAN_POINT('Ctrl Pts',(39.0000000001679,-3.68063070304705,
-101.239156866278));
#171154=CARTESIAN_POINT('Ctrl Pts',(39.,-3.68000002,-101.255910620448));
#171155=CARTESIAN_POINT('Ctrl Pts',(39.6406521140204,-3.78697803566041,
-98.6057147789936));
#171156=CARTESIAN_POINT('Ctrl Pts',(39.7174896230836,-4.18000001999998,
-98.6445257445324));
#171157=CARTESIAN_POINT('Ctrl Pts',(40.0766182115838,-4.18000001999998,
-98.8259229955145));
#171158=CARTESIAN_POINT('Ctrl Pts',(39.4187804907282,-3.76832519858073,
-99.0363833344201));
#171159=CARTESIAN_POINT('Ctrl Pts',(39.4849150761468,-4.18000001999998,
-99.0700146927968));
#171160=CARTESIAN_POINT('Ctrl Pts',(39.87692608831,-4.18000001999998,-99.2216958278296));
#171161=CARTESIAN_POINT('Ctrl Pts',(39.2562588135465,-3.74954484420426,
-99.4842872473771));
#171162=CARTESIAN_POINT('Ctrl Pts',(39.3129722860326,-4.18000001999998,
-99.5090269233591));
#171163=CARTESIAN_POINT('Ctrl Pts',(39.7306548682082,-4.18000001999998,
-99.6328320937587));
#171164=CARTESIAN_POINT('Ctrl Pts',(39.0420216354292,-3.71207776720274,
-100.41203214575));
#171165=CARTESIAN_POINT('Ctrl Pts',(39.070686775237,-4.18000001999998,-100.423129382882));
#171166=CARTESIAN_POINT('Ctrl Pts',(39.5378302081339,-4.18000001999998,
-100.48343236993));
#171167=CARTESIAN_POINT('Ctrl Pts',(38.9909689698687,-3.69325270187659,
-100.895713807542));
#171168=CARTESIAN_POINT('Ctrl Pts',(39.0043575688645,-4.18000001999998,
-100.903770629911));
#171169=CARTESIAN_POINT('Ctrl Pts',(39.4918770183597,-4.18000001999999,
-100.926406647344));
#171170=CARTESIAN_POINT('Ctrl Pts',(39.0013094879538,-3.6752109923929,-101.378179163766));
#171171=CARTESIAN_POINT('Ctrl Pts',(38.9964768548807,-4.18000001999999,
-101.378270171681));
#171172=CARTESIAN_POINT('Ctrl Pts',(39.5011768353311,-4.18000001999999,
-101.367775593403));
#171173=CARTESIAN_POINT('',(39.5,-4.18000001999998,-101.255910620448));
#171174=CARTESIAN_POINT('Origin',(39.5,-3.68000001999999,-101.255910620448));
#171175=CARTESIAN_POINT('',(40.0271577790679,-4.18000001999998,-98.926539349744));
#171176=CARTESIAN_POINT('Origin',(40.0271577790679,-3.68000001999999,-98.926539349744));
#171177=CARTESIAN_POINT('Ctrl Pts',(39.5,-4.18000001999999,-101.255910620448));
#171178=CARTESIAN_POINT('Ctrl Pts',(39.5,-4.18000001999999,-100.974485528886));
#171179=CARTESIAN_POINT('Ctrl Pts',(39.5222808837194,-4.18000001999999,
-100.693150422405));
#171180=CARTESIAN_POINT('Ctrl Pts',(39.5655905128992,-4.18000001999999,
-100.416810780349));
#171181=CARTESIAN_POINT('Ctrl Pts',(39.5844991865996,-4.18000001999999,
-100.296162873149));
#171182=CARTESIAN_POINT('Ctrl Pts',(39.6074169109172,-4.18000001999998,
-100.176467126241));
#171183=CARTESIAN_POINT('Ctrl Pts',(39.6342425380315,-4.18000001999998,
-100.058132231812));
#171184=CARTESIAN_POINT('Ctrl Pts',(39.7053092693719,-4.18000001999998,
-99.7446381943849));
#171185=CARTESIAN_POINT('Ctrl Pts',(39.8034555232797,-4.18000001999998,
-99.4388673313559));
#171186=CARTESIAN_POINT('Ctrl Pts',(39.930132764858,-4.18000001999998,-99.1412335948014));
#171187=CARTESIAN_POINT('Ctrl Pts',(39.960795555159,-4.18000001999998,-99.0691900237798));
#171188=CARTESIAN_POINT('Ctrl Pts',(39.9931302150563,-4.18000001999998,
-98.9976232754198));
#171189=CARTESIAN_POINT('Ctrl Pts',(40.0271577790679,-4.18000001999998,
-98.926539349744));
#171190=CARTESIAN_POINT('Origin',(39.5,-3.68000001999999,-55.24995));
#171191=CARTESIAN_POINT('',(39.5,-4.18000001999998,-130.802732351058));
#171192=CARTESIAN_POINT('Origin',(39.5,-3.68000001999999,-130.802732351058));
#171193=CARTESIAN_POINT('',(39.5,-4.18000001999998,-55.24995));
#171194=CARTESIAN_POINT('Ctrl Pts',(39.,-3.68000001999999,-130.802732351058));
#171195=CARTESIAN_POINT('Ctrl Pts',(39.,-4.18000001999998,-130.802732351057));
#171196=CARTESIAN_POINT('Ctrl Pts',(39.5,-4.18000001999998,-130.802732351058));
#171197=CARTESIAN_POINT('Ctrl Pts',(39.,-3.69663481492557,-131.244626684237));
#171198=CARTESIAN_POINT('Ctrl Pts',(39.0163626300028,-4.18000001999998,
-131.237396673044));
#171199=CARTESIAN_POINT('Ctrl Pts',(39.5000000028449,-4.18000001999998,
-131.207067934262));
#171200=CARTESIAN_POINT('Ctrl Pts',(39.0498728558349,-3.71353967201765,
-131.677827554702));
#171201=CARTESIAN_POINT('Ctrl Pts',(39.0799719048085,-4.18000001999998,
-131.667492297612));
#171202=CARTESIAN_POINT('Ctrl Pts',(39.5448855698238,-4.18000001999998,
-131.603841024792));
#171203=CARTESIAN_POINT('Ctrl Pts',(39.2448092923438,-3.74782444813235,
-132.527335109052));
#171204=CARTESIAN_POINT('Ctrl Pts',(39.3005991742935,-4.18000001999998,
-132.50452184294));
#171205=CARTESIAN_POINT('Ctrl Pts',(39.720328363537,-4.18000001999998,-132.382704674372));
#171206=CARTESIAN_POINT('Ctrl Pts',(39.391689897628,-3.76532817544854,-132.946345914773));
#171207=CARTESIAN_POINT('Ctrl Pts',(39.4567563186094,-4.18000001999999,
-132.915330450675));
#171208=CARTESIAN_POINT('Ctrl Pts',(39.8525202266285,-4.18000001999998,
-132.767284004423));
#171209=CARTESIAN_POINT('Ctrl Pts',(39.585730865626,-3.78242429107036,-133.343412752622));
#171210=CARTESIAN_POINT('Ctrl Pts',(39.6607823401612,-4.18000001999998,
-133.307485940342));
#171211=CARTESIAN_POINT('Ctrl Pts',(40.0271577790634,-4.18000001999998,
-133.132103621752));
#171212=CARTESIAN_POINT('',(40.0271577790634,-4.18000001999998,-133.132103621752));
#171213=CARTESIAN_POINT('Origin',(40.0271577790634,-3.68000001999999,-133.132103621752));
#171214=CARTESIAN_POINT('Ctrl Pts',(40.0271577790634,-4.18000001999998,
-133.132103621752));
#171215=CARTESIAN_POINT('Ctrl Pts',(39.903504593422,-4.18000001999998,-132.873790865225));
#171216=CARTESIAN_POINT('Ctrl Pts',(39.8011022473334,-4.18000001999999,
-132.605500495487));
#171217=CARTESIAN_POINT('Ctrl Pts',(39.7207150267675,-4.18000001999999,
-132.332596829901));
#171218=CARTESIAN_POINT('Ctrl Pts',(39.6875913562942,-4.18000001999999,
-132.220146479881));
#171219=CARTESIAN_POINT('Ctrl Pts',(39.6582049915466,-4.18000001999998,
-132.106913147221));
#171220=CARTESIAN_POINT('Ctrl Pts',(39.6326069664648,-4.18000001999998,
-131.993272849631));
#171221=CARTESIAN_POINT('Ctrl Pts',(39.5604708508297,-4.18000001999999,
-131.673030580095));
#171222=CARTESIAN_POINT('Ctrl Pts',(39.5173036683663,-4.18000001999998,
-131.347852435203));
#171223=CARTESIAN_POINT('Ctrl Pts',(39.5042396692598,-4.18000001999998,
-131.017545146527));
#171224=CARTESIAN_POINT('Ctrl Pts',(39.5014171427712,-4.18000001999998,
-130.946181005725));
#171225=CARTESIAN_POINT('Ctrl Pts',(39.5,-4.18000001999998,-130.874577408223));
#171226=CARTESIAN_POINT('Ctrl Pts',(39.5,-4.18000001999998,-130.802732351058));
#171227=CARTESIAN_POINT('Ctrl Pts',(58.1221005562789,-4.18000001999999,
-171.237717270032));
#171228=CARTESIAN_POINT('Ctrl Pts',(57.7306096110337,-4.18000001999999,
-171.422588467367));
#171229=CARTESIAN_POINT('Ctrl Pts',(57.6746235421417,-3.75150367745622,
-171.449026400902));
#171230=CARTESIAN_POINT('Ctrl Pts',(52.1178467328245,-4.18000001999999,
-158.52285936551));
#171231=CARTESIAN_POINT('Ctrl Pts',(51.7702631771107,-4.18000001999999,
-158.785894332693));
#171232=CARTESIAN_POINT('Ctrl Pts',(51.6715280616305,-3.75870638021677,
-158.734184170827));
#171233=CARTESIAN_POINT('Ctrl Pts',(46.0984623496487,-4.18000001999998,
-145.815120328436));
#171234=CARTESIAN_POINT('Ctrl Pts',(45.7948164697718,-4.18000001999998,
-146.15085325192));
#171235=CARTESIAN_POINT('Ctrl Pts',(45.6536266465224,-3.76768226491552,
-146.026454114168));
#171236=CARTESIAN_POINT('Ctrl Pts',(40.0271577790634,-4.18000001999998,
-133.132103621752));
#171237=CARTESIAN_POINT('Ctrl Pts',(39.660782340162,-4.18000001999998,-133.307485940342));
#171238=CARTESIAN_POINT('Ctrl Pts',(39.5857308656265,-3.78242429107081,
-133.343412752623));
#171239=CARTESIAN_POINT('',(58.1221005562789,-4.18000001999999,-171.237717270032));
#171240=CARTESIAN_POINT('Origin',(58.1221005562789,-3.68000001999999,-171.237717270032));
#171241=CARTESIAN_POINT('Ctrl Pts',(58.1221005562789,-4.18000001999999,
-171.237717270032));
#171242=CARTESIAN_POINT('Ctrl Pts',(52.1178384024439,-4.18000001999999,
-158.522841724749));
#171243=CARTESIAN_POINT('Ctrl Pts',(46.0984712740486,-4.18000001999998,
-145.815138971718));
#171244=CARTESIAN_POINT('Ctrl Pts',(40.0271577790634,-4.18000001999998,
-133.132103621752));
#171245=CARTESIAN_POINT('Ctrl Pts',(58.2644174754153,-4.18000001999999,
-171.871644662643));
#171246=CARTESIAN_POINT('Ctrl Pts',(57.8378063278745,-4.18000001999999,
-171.871644662643));
#171247=CARTESIAN_POINT('Ctrl Pts',(57.7706512256236,-3.75870764711888,
-171.871644662643));
#171248=CARTESIAN_POINT('Ctrl Pts',(58.2644174584531,-4.18000001999999,
-171.652701076652));
#171249=CARTESIAN_POINT('Ctrl Pts',(57.8378063150439,-4.18000001999999,
-171.715730578987));
#171250=CARTESIAN_POINT('Ctrl Pts',(57.7706512252069,-3.75870764450445,
-171.725685252419));
#171251=CARTESIAN_POINT('Ctrl Pts',(58.2165506240601,-4.18000001999999,
-171.437728673605));
#171252=CARTESIAN_POINT('Ctrl Pts',(57.801183875227,-4.18000002000114,-171.562158552623));
#171253=CARTESIAN_POINT('Ctrl Pts',(57.7383541282856,-3.7562957918519,-171.582363368286));
#171254=CARTESIAN_POINT('Ctrl Pts',(58.1221005562789,-4.18000001999999,
-171.237717270032));
#171255=CARTESIAN_POINT('Ctrl Pts',(57.7306096110337,-4.18000001999999,
-171.422588467367));
#171256=CARTESIAN_POINT('Ctrl Pts',(57.6746235421417,-3.75150367745622,
-171.449026400902));
#171257=CARTESIAN_POINT('',(58.2644174754153,-4.18000001999999,-171.871644662643));
#171258=CARTESIAN_POINT('Origin',(58.2644174754153,-3.68000001999999,-171.871644662643));
#171259=CARTESIAN_POINT('Origin',(56.1314697890424,-4.18000001999999,-172.0066931789));
#171260=CARTESIAN_POINT('Origin',(58.2644174754153,-3.68000001999999,-179.64995));
#171261=CARTESIAN_POINT('',(57.7706512256236,-3.75870764711888,-179.64995));
#171262=CARTESIAN_POINT('',(58.2644174754153,-4.18000001999999,-171.871644662643));
#171263=CARTESIAN_POINT('Ctrl Pts',(60.,-4.68000001999999,-174.488343624884));
#171264=CARTESIAN_POINT('Ctrl Pts',(60.,-4.18000002,-174.488343624884));
#171265=CARTESIAN_POINT('Ctrl Pts',(59.5,-4.18000001999999,-174.488343624884));
#171266=CARTESIAN_POINT('Ctrl Pts',(60.,-4.67777472283721,-174.78368089075));
#171267=CARTESIAN_POINT('Ctrl Pts',(59.9977796185047,-4.18000001999829,
-174.78302738694));
#171268=CARTESIAN_POINT('Ctrl Pts',(59.499999993334,-4.18000001999999,-174.734541991424));
#171269=CARTESIAN_POINT('Ctrl Pts',(59.9573556192874,-4.67559899657361,
-175.071875505894));
#171270=CARTESIAN_POINT('Ctrl Pts',(59.9531694408477,-4.18000002000085,
-175.070632089297));
#171271=CARTESIAN_POINT('Ctrl Pts',(59.4644630183961,-4.18000001999999,
-174.974786360247));
#171272=CARTESIAN_POINT('Ctrl Pts',(59.8306767385091,-4.67241126250759,
-175.493405719049));
#171273=CARTESIAN_POINT('Ctrl Pts',(59.8236519200077,-4.18000001999958,
-175.490806712526));
#171274=CARTESIAN_POINT('Ctrl Pts',(59.3588972809293,-4.18000001999999,
-175.326182058073));
#171275=CARTESIAN_POINT('Ctrl Pts',(59.7776634626824,-4.67136322522169,
-175.631868709625));
#171276=CARTESIAN_POINT('Ctrl Pts',(59.7698424718428,-4.18000001999956,
-175.628550598836));
#171277=CARTESIAN_POINT('Ctrl Pts',(59.3147195516479,-4.18000001999999,
-175.441607525732));
#171278=CARTESIAN_POINT('Ctrl Pts',(59.6537038929485,-4.66936150715186,
-175.896123076728));
#171279=CARTESIAN_POINT('Ctrl Pts',(59.6445293525488,-4.18000002000041,
-175.891155901683));
#171280=CARTESIAN_POINT('Ctrl Pts',(59.2114199113778,-4.18000001999999,
-175.661895244315));
#171281=CARTESIAN_POINT('Ctrl Pts',(59.5824462721252,-4.66839878682381,
-176.023110187492));
#171282=CARTESIAN_POINT('Ctrl Pts',(59.5727342923808,-4.18000002000089,
-176.017245435326));
#171283=CARTESIAN_POINT('Ctrl Pts',(59.1520385607459,-4.18000001999999,
-175.767754281813));
#171284=CARTESIAN_POINT('Ctrl Pts',(59.4213258837533,-4.66655021592386,
-176.266776880891));
#171285=CARTESIAN_POINT('Ctrl Pts',(59.4108028292072,-4.1800000199991,-176.25895171657));
#171286=CARTESIAN_POINT('Ctrl Pts',(59.0177715691528,-4.18000001999999,
-175.970879863896));
#171287=CARTESIAN_POINT('Ctrl Pts',(59.3305935235461,-4.66565781609966,
-176.3843179035));
#171288=CARTESIAN_POINT('Ctrl Pts',(59.3198146755637,-4.18000001999915,
-176.37546218739));
#171289=CARTESIAN_POINT('Ctrl Pts',(58.9421612688066,-4.18000001999999,
-176.06886452411));
#171290=CARTESIAN_POINT('Ctrl Pts',(59.1349023357136,-4.66400011582949,
-176.602528392516));
#171291=CARTESIAN_POINT('Ctrl Pts',(59.1239216856836,-4.18000002000084,
-176.591561815318));
#171292=CARTESIAN_POINT('Ctrl Pts',(58.7790852805764,-4.18000001999999,
-176.250769420981));
#171293=CARTESIAN_POINT('Ctrl Pts',(59.0299133821615,-4.66323171680632,
-176.703607721972));
#171294=CARTESIAN_POINT('Ctrl Pts',(59.0189867750955,-4.18000001999871,
-176.691604703902));
#171295=CARTESIAN_POINT('Ctrl Pts',(58.6915944853457,-4.18000001999999,
-176.33503132506));
#171296=CARTESIAN_POINT('Ctrl Pts',(58.6938786030259,-4.66110543474911,
-176.983174915482));
#171297=CARTESIAN_POINT('Ctrl Pts',(58.6838036746477,-4.18000002000249,
-176.967887143763));
#171298=CARTESIAN_POINT('Ctrl Pts',(58.4115655020993,-4.18000001999999,
-176.56808461344));
#171299=CARTESIAN_POINT('Ctrl Pts',(58.437917085704,-4.65991812350376,-177.139087667033));
#171300=CARTESIAN_POINT('Ctrl Pts',(58.4288067817606,-4.18000002000125,
-177.121996578829));
#171301=CARTESIAN_POINT('Ctrl Pts',(58.1982641486948,-4.18000001999999,
-176.698056997615));
#171302=CARTESIAN_POINT('Ctrl Pts',(58.1703978083756,-4.65905396057624,
-177.252515804372));
#171303=CARTESIAN_POINT('Ctrl Pts',(58.1625546348518,-4.18000002,-177.234024164027));
#171304=CARTESIAN_POINT('Ctrl Pts',(57.9753315069797,-4.18000001999999,
-176.792613205276));
#171305=CARTESIAN_POINT('',(59.5,-4.18000001999999,-174.488343624884));
#171306=CARTESIAN_POINT('Ctrl Pts',(59.5,-4.18000001999999,-174.488343624884));
#171307=CARTESIAN_POINT('Ctrl Pts',(59.5,-4.18000001999999,-174.676432184958));
#171308=CARTESIAN_POINT('Ctrl Pts',(59.4792627601818,-4.18000001935391,
-174.860994953572));
#171309=CARTESIAN_POINT('Ctrl Pts',(59.4381337746112,-4.18000002064829,
-175.042081103196));
#171310=CARTESIAN_POINT('Ctrl Pts',(59.4313812635049,-4.1800000208608,-175.071811625833));
#171311=CARTESIAN_POINT('Ctrl Pts',(59.4240789892375,-4.18000002115769,
-175.101448468711));
#171312=CARTESIAN_POINT('Ctrl Pts',(59.4162283471532,-4.18000002161129,
-175.130991885445));
#171313=CARTESIAN_POINT('Ctrl Pts',(59.4092933860371,-4.18000002201199,
-175.157089425504));
#171314=CARTESIAN_POINT('Ctrl Pts',(59.4019280344311,-4.18000002232545,
-175.183113688583));
#171315=CARTESIAN_POINT('Ctrl Pts',(59.3941336392735,-4.18000002248888,
-175.209064512545));
#171316=CARTESIAN_POINT('Ctrl Pts',(59.3589528015432,-4.18000002322649,
-175.326196337184));
#171317=CARTESIAN_POINT('Ctrl Pts',(59.3147522563139,-4.18000002089879,
-175.441619139941));
#171318=CARTESIAN_POINT('Ctrl Pts',(59.2630854722639,-4.18000002030225,
-175.551758766342));
#171319=CARTESIAN_POINT('Ctrl Pts',(59.2343127518865,-4.18000001997004,
-175.613094433564));
#171320=CARTESIAN_POINT('Ctrl Pts',(59.2031440665131,-4.18000001999999,
-175.673101168879));
#171321=CARTESIAN_POINT('Ctrl Pts',(59.1695814056726,-4.18000001999999,
-175.731779921994));
#171322=CARTESIAN_POINT('Ctrl Pts',(59.1428767576963,-4.18000001999999,
-175.778468575586));
#171323=CARTESIAN_POINT('Ctrl Pts',(59.1146521957298,-4.18000001999991,
-175.824314777934));
#171324=CARTESIAN_POINT('Ctrl Pts',(59.0849057084902,-4.18000002000059,
-175.869317498238));
#171325=CARTESIAN_POINT('Ctrl Pts',(59.0177729179323,-4.18000002000212,
-175.970881026476));
#171326=CARTESIAN_POINT('Ctrl Pts',(58.9421638152095,-4.18000002001086,
-176.068866658213));
#171327=CARTESIAN_POINT('Ctrl Pts',(58.8606254499681,-4.18000002000853,
-176.15981892266));
#171328=CARTESIAN_POINT('Ctrl Pts',(58.8332817762446,-4.18000002000775,
-176.190319522422));
#171329=CARTESIAN_POINT('Ctrl Pts',(58.8052684934466,-4.18000002000547,
-176.220067577769));
#171330=CARTESIAN_POINT('Ctrl Pts',(58.7765893403539,-4.18000002000312,
-176.2490672712));
#171331=CARTESIAN_POINT('Ctrl Pts',(58.7334919025219,-4.18000001999957,
-176.292646399243));
#171332=CARTESIAN_POINT('Ctrl Pts',(58.6887854216327,-4.1800000198565,-176.334637716937));
#171333=CARTESIAN_POINT('Ctrl Pts',(58.6426104314496,-4.18000002015176,
-176.374934331061));
#171334=CARTESIAN_POINT('Ctrl Pts',(58.6279756118803,-4.18000002024535,
-176.387706043077));
#171335=CARTESIAN_POINT('Ctrl Pts',(58.6131935185633,-4.18000002040339,
-176.40030782898));
#171336=CARTESIAN_POINT('Ctrl Pts',(58.5982692931781,-4.18000002077447,
-176.412737145102));
#171337=CARTESIAN_POINT('Ctrl Pts',(58.5771929061033,-4.18000002129852,
-176.430290155116));
#171338=CARTESIAN_POINT('Ctrl Pts',(58.5557921166901,-4.18000002220248,
-176.447510765875));
#171339=CARTESIAN_POINT('Ctrl Pts',(58.5341058949341,-4.18000002446768,
-176.464377473526));
#171340=CARTESIAN_POINT('Ctrl Pts',(58.4881980669412,-4.18000002926289,
-176.500082813181));
#171341=CARTESIAN_POINT('Ctrl Pts',(58.4409815652464,-4.18000004169373,
-176.534222750276));
#171342=CARTESIAN_POINT('Ctrl Pts',(58.3925215548526,-4.18000005349381,
-176.566751049322));
#171343=CARTESIAN_POINT('Ctrl Pts',(58.3507358574757,-4.18000006366869,
-176.59479928227));
#171344=CARTESIAN_POINT('Ctrl Pts',(58.3080246526019,-4.18000007127262,
-176.621648795663));
#171345=CARTESIAN_POINT('Ctrl Pts',(58.2644174754055,-4.18000006545692,
-176.647241333307));
#171346=CARTESIAN_POINT('Origin',(59.5,-4.68000001999999,-174.488343624884));
#171347=CARTESIAN_POINT('Ctrl Pts',(40.0271577790679,-4.18000001999998,
-98.926539349744));
#171348=CARTESIAN_POINT('Ctrl Pts',(39.6607823401664,-4.18000001999998,
-98.7511570311542));
#171349=CARTESIAN_POINT('Ctrl Pts',(39.585730865631,-3.7824242910708,-98.7152302188737));
#171350=CARTESIAN_POINT('Ctrl Pts',(46.0600623067188,-4.18000001999998,
-86.3237407210712));
#171351=CARTESIAN_POINT('Ctrl Pts',(45.7555532717617,-4.18000001999998,
-85.989998533184));
#171352=CARTESIAN_POINT('Ctrl Pts',(45.6152479999264,-3.76777550625849,
-86.1124074338642));
#171353=CARTESIAN_POINT('Ctrl Pts',(52.0416537250564,-4.18000001999999,
-73.6965087765536));
#171354=CARTESIAN_POINT('Ctrl Pts',(51.6938180895878,-4.18000002,-73.4342549076826));
#171355=CARTESIAN_POINT('Ctrl Pts',(51.5953561718106,-3.75882512748543,
-73.4851842533606));
#171356=CARTESIAN_POINT('Ctrl Pts',(58.0081705490647,-4.18000001999999,
-61.0621827299711));
#171357=CARTESIAN_POINT('Ctrl Pts',(57.6167925372613,-4.18000001999999,
-60.8773558160983));
#171358=CARTESIAN_POINT('Ctrl Pts',(57.5607154366947,-3.75164060643487,
-60.8508735991007));
#171359=CARTESIAN_POINT('',(57.5607154366947,-3.75164060643487,-60.8508735991007));
#171360=CARTESIAN_POINT('Ctrl Pts',(57.5607154366947,-3.75164060643487,
-60.8508735991007));
#171361=CARTESIAN_POINT('Ctrl Pts',(55.9461395978097,-3.75358515890381,
-64.27045854236));
#171362=CARTESIAN_POINT('Ctrl Pts',(54.3918375646665,-3.7555208048552,-67.5588600426932));
#171363=CARTESIAN_POINT('Ctrl Pts',(52.1508196005947,-3.75871164726325,
-72.2946871288037));
#171364=CARTESIAN_POINT('Ctrl Pts',(51.4188856818639,-3.75981653600606,
-73.8405002967756));
#171365=CARTESIAN_POINT('Ctrl Pts',(50.3435910299283,-3.76151388746903,
-76.1100262576363));
#171366=CARTESIAN_POINT('Ctrl Pts',(49.8115952016668,-3.76237194900324,
-77.2324907902923));
#171367=CARTESIAN_POINT('Ctrl Pts',(49.2008224325657,-3.76337812834746,
-78.5205104614526));
#171368=CARTESIAN_POINT('Ctrl Pts',(48.8979081133578,-3.76388059401857,
-79.1591397261314));
#171369=CARTESIAN_POINT('Ctrl Pts',(48.7282140480925,-3.76416277298739,
-79.5168554019473));
#171370=CARTESIAN_POINT('Ctrl Pts',(48.6449347296394,-3.76430143017905,
-79.6923933180138));
#171371=CARTESIAN_POINT('Ctrl Pts',(48.6020070309088,-3.76437293568594,
-79.7828734307288));
#171372=CARTESIAN_POINT('Ctrl Pts',(48.5998549578026,-3.76437652051741,
-79.7874094159184));
#171373=CARTESIAN_POINT('Ctrl Pts',(45.3063254247015,-3.76986294272013,
-86.7292502309379));
#171374=CARTESIAN_POINT('Ctrl Pts',(42.3026944142814,-3.775823395277,-93.0362663227149));
#171375=CARTESIAN_POINT('Ctrl Pts',(39.585730865631,-3.78242429107081,-98.7152302188737));
#171376=CARTESIAN_POINT('',(58.0081705490647,-4.18000001999999,-61.0621827299711));
#171377=CARTESIAN_POINT('Origin',(58.0081705490647,-3.68000001999999,-61.0621827299711));
#171378=CARTESIAN_POINT('Ctrl Pts',(40.0271577790679,-4.18000001999998,
-98.926539349744));
#171379=CARTESIAN_POINT('Ctrl Pts',(46.0600710189762,-4.18000001999998,
-86.3237225210772));
#171380=CARTESIAN_POINT('Ctrl Pts',(52.0416455898407,-4.18000001999999,
-73.6965260027483));
#171381=CARTESIAN_POINT('Ctrl Pts',(58.0081705490647,-4.18000001999999,
-61.0621827299711));
#171382=CARTESIAN_POINT('Origin',(59.5,-4.68000001999999,-55.24995));
#171383=CARTESIAN_POINT('',(59.5,-4.18000001999999,-58.1445632485962));
#171384=CARTESIAN_POINT('',(60.,-4.68000002001403,-58.1445632485962));
#171385=CARTESIAN_POINT('Origin',(59.5,-4.68000001999999,-58.1445632485962));
#171386=CARTESIAN_POINT('',(60.,-4.68000001999999,-58.1637190207452));
#171387=CARTESIAN_POINT('',(59.5,-4.18000001999999,-174.466077711105));
#171388=CARTESIAN_POINT('Origin',(60.,-2.55003103885676E-14,0.));
#171389=CARTESIAN_POINT('',(60.,-5.18000001999999,-58.1246434856214));
#171390=CARTESIAN_POINT('Ctrl Pts',(60.,-4.68000002001403,-58.1445632485962));
#171391=CARTESIAN_POINT('Ctrl Pts',(60.,-4.84666977904325,-58.1380335512985));
#171392=CARTESIAN_POINT('Ctrl Pts',(60.,-5.01333597711292,-58.1313769278999));
#171393=CARTESIAN_POINT('Ctrl Pts',(60.,-5.18000001999999,-58.1246434856214));
#171394=CARTESIAN_POINT('',(60.,-5.18000001999999,-174.534521368494));
#171395=CARTESIAN_POINT('Origin',(59.5,-5.18000001999999,-55.24995));
#171396=CARTESIAN_POINT('',(59.5,-5.68000001999999,-58.1246434856214));
#171397=CARTESIAN_POINT('Origin',(59.5,-5.18000001999999,-58.1246434856214));
#171398=CARTESIAN_POINT('',(59.5,-5.68000001999999,-174.511260182693));
#171399=CARTESIAN_POINT('',(59.5,-5.68000001999999,-58.1042606444049));
#171400=CARTESIAN_POINT('Origin',(59.5,-5.18000001999999,-174.511260182693));
#171401=CARTESIAN_POINT('Ctrl Pts',(59.5,-5.68000001999999,-174.511260182693));
#171402=CARTESIAN_POINT('Ctrl Pts',(60.,-5.68000001999998,-174.511260182694));
#171403=CARTESIAN_POINT('Ctrl Pts',(60.,-5.18000001999999,-174.511260182693));
#171404=CARTESIAN_POINT('Ctrl Pts',(59.4999999934949,-5.68000001999999,
-174.751455697725));
#171405=CARTESIAN_POINT('Ctrl Pts',(60.0022233258349,-5.68000002000248,
-174.800030292485));
#171406=CARTESIAN_POINT('Ctrl Pts',(60.,-5.17778160006748,-174.799392136338));
#171407=CARTESIAN_POINT('Ctrl Pts',(59.4661441339012,-5.68000001999999,
-174.985974426754));
#171408=CARTESIAN_POINT('Ctrl Pts',(59.9636195754477,-5.68000001999999,
-175.081942695907));
#171409=CARTESIAN_POINT('Ctrl Pts',(59.9593729581191,-5.1756134281897,-175.080714219829));
#171410=CARTESIAN_POINT('Ctrl Pts',(59.3657005801303,-5.68000001999999,
-175.329231362388));
#171411=CARTESIAN_POINT('Ctrl Pts',(59.8460772881358,-5.68000001999999,
-175.49508011951));
#171412=CARTESIAN_POINT('Ctrl Pts',(59.8388406974375,-5.17243729299778,
-175.492475419334));
#171413=CARTESIAN_POINT('Ctrl Pts',(59.3235784200839,-5.68000001999999,
-175.4423463311));
#171414=CARTESIAN_POINT('Ctrl Pts',(59.7963955952484,-5.68000002000071,
-175.631508024916));
#171415=CARTESIAN_POINT('Ctrl Pts',(59.7882941049042,-5.17139018325129,
-175.628164866621));
#171416=CARTESIAN_POINT('Ctrl Pts',(59.2250283845896,-5.68000001999999,
-175.658495472519));
#171417=CARTESIAN_POINT('Ctrl Pts',(59.6796421793893,-5.68000001999927,
-175.892503005072));
#171418=CARTESIAN_POINT('Ctrl Pts',(59.6700340607039,-5.16938852396119,
-175.887451075324));
#171419=CARTESIAN_POINT('Ctrl Pts',(59.1683759292615,-5.68000001999999,
-175.762481455964));
#171420=CARTESIAN_POINT('Ctrl Pts',(59.6122794132826,-5.6800000200009,-176.018182187565));
#171421=CARTESIAN_POINT('Ctrl Pts',(59.6020511144931,-5.16842516963192,
-176.012189602522));
#171422=CARTESIAN_POINT('Ctrl Pts',(59.0403562655437,-5.68000001999999,
-175.962298484052));
#171423=CARTESIAN_POINT('Ctrl Pts',(59.4596388112852,-5.68000001999906,
-176.259950074275));
#171424=CARTESIAN_POINT('Ctrl Pts',(59.4484275192731,-5.16657340194589,
-176.251884189743));
#171425=CARTESIAN_POINT('Ctrl Pts',(58.9683527741555,-5.68000001999999,
-176.058826880554));
#171426=CARTESIAN_POINT('Ctrl Pts',(59.3735776050024,-5.68000001999968,
-176.376845479805));
#171427=CARTESIAN_POINT('Ctrl Pts',(59.3620233301153,-5.16567852041965,
-176.367676771746));
#171428=CARTESIAN_POINT('Ctrl Pts',(58.8121204079676,-5.68000001999999,
-176.239514776908));
#171429=CARTESIAN_POINT('Ctrl Pts',(59.1864690073094,-5.6800000200003,-176.595885870473));
#171430=CARTESIAN_POINT('Ctrl Pts',(59.1745444884326,-5.16400295101772,
-176.584424539694));
#171431=CARTESIAN_POINT('Ctrl Pts',(58.7283002756348,-5.68000001999999,
-176.3234477233));
#171432=CARTESIAN_POINT('Ctrl Pts',(59.0859070073554,-5.68000001999999,
-176.697708952909));
#171433=CARTESIAN_POINT('Ctrl Pts',(59.0739603306682,-5.16322437006847,
-176.685107962755));
#171434=CARTESIAN_POINT('Ctrl Pts',(58.460151514568,-5.68000001999999,-176.556489535136));
#171435=CARTESIAN_POINT('Ctrl Pts',(58.7634647581383,-5.68000001999999,
-176.980908577071));
#171436=CARTESIAN_POINT('Ctrl Pts',(58.7521818176688,-5.16106213487567,
-176.9646578323));
#171437=CARTESIAN_POINT('Ctrl Pts',(58.2562917522372,-5.68000001999999,
-176.688008530437));
#171438=CARTESIAN_POINT('Ctrl Pts',(58.5179479000405,-5.68000002000953,
-177.140745767071));
#171439=CARTESIAN_POINT('Ctrl Pts',(58.5075501754184,-5.15984115636875,
-177.122423932479));
#171440=CARTESIAN_POINT('Ctrl Pts',(58.0404491789985,-5.68000001999999,
-176.786906275262));
#171441=CARTESIAN_POINT('Ctrl Pts',(58.2576969618386,-5.68000001999996,
-177.261045698521));
#171442=CARTESIAN_POINT('Ctrl Pts',(58.2485390147982,-5.15892282666644,
-177.241058641939));
#171443=CARTESIAN_POINT('Ctrl Pts',(58.6082745331212,-5.6800000199515,-176.427328712824));
#171444=CARTESIAN_POINT('Ctrl Pts',(58.6185667882716,-5.68000001995871,
-176.418676244678));
#171445=CARTESIAN_POINT('Ctrl Pts',(58.628783204882,-5.68000001996413,-176.409943629197));
#171446=CARTESIAN_POINT('Ctrl Pts',(58.6389210444463,-5.68000001996836,
-176.401132572172));
#171447=CARTESIAN_POINT('Ctrl Pts',(58.7108573560273,-5.68000001999836,
-176.338610874188));
#171448=CARTESIAN_POINT('Ctrl Pts',(58.7792948136839,-5.68000001999946,
-176.271947442152));
#171449=CARTESIAN_POINT('Ctrl Pts',(58.8440583693344,-5.68000001994282,
-176.201117847418));
#171450=CARTESIAN_POINT('Ctrl Pts',(58.8596678064668,-5.68000001992916,
-176.184046361842));
#171451=CARTESIAN_POINT('Ctrl Pts',(58.8750639774275,-5.6800000199106,-176.166733035301));
#171452=CARTESIAN_POINT('Ctrl Pts',(58.8902447330317,-5.68000001988414,
-176.149177868712));
#171453=CARTESIAN_POINT('Ctrl Pts',(58.9227212058659,-5.68000001982754,
-176.111621774291));
#171454=CARTESIAN_POINT('Ctrl Pts',(58.9541409398416,-5.68000001973543,
-176.072997877296));
#171455=CARTESIAN_POINT('Ctrl Pts',(58.9843599854969,-5.68000001956972,
-176.033520885199));
#171456=CARTESIAN_POINT('Ctrl Pts',(59.0268866354123,-5.6800000193365,-175.977965715067));
#171457=CARTESIAN_POINT('Ctrl Pts',(59.0670052242283,-5.68000001940972,
-175.920749643185));
#171458=CARTESIAN_POINT('Ctrl Pts',(59.1043833915298,-5.68000001957814,
-175.862401050087));
#171459=CARTESIAN_POINT('Ctrl Pts',(59.1540049590064,-5.68000001980172,
-175.784940092029));
#171460=CARTESIAN_POINT('Ctrl Pts',(59.1991811925137,-5.68000001997513,
-175.705064487821));
#171461=CARTESIAN_POINT('Ctrl Pts',(59.2399658936416,-5.68000001998964,
-175.622670099363));
#171462=CARTESIAN_POINT('Ctrl Pts',(59.2487993257312,-5.68000001999278,
-175.604824553978));
#171463=CARTESIAN_POINT('Ctrl Pts',(59.2574265918442,-5.6800000199934,-175.586860742585));
#171464=CARTESIAN_POINT('Ctrl Pts',(59.2658479718429,-5.68000001999155,
-175.568777423473));
#171465=CARTESIAN_POINT('Ctrl Pts',(59.2686911708562,-5.68000001999092,
-175.5626721919));
#171466=CARTESIAN_POINT('Ctrl Pts',(59.2715106588894,-5.68000001999007,
-175.556553812533));
#171467=CARTESIAN_POINT('Ctrl Pts',(59.2743064287832,-5.68000001998893,
-175.550422281673));
#171468=CARTESIAN_POINT('Ctrl Pts',(59.3235845105522,-5.68000001996885,
-175.44234826609));
#171469=CARTESIAN_POINT('Ctrl Pts',(59.3657187337311,-5.68000001965404,
-175.32923562655));
#171470=CARTESIAN_POINT('Ctrl Pts',(59.3992004790971,-5.68000001961977,
-175.214817860028));
#171471=CARTESIAN_POINT('Ctrl Pts',(59.4149912346775,-5.68000001960361,
-175.160855828914));
#171472=CARTESIAN_POINT('Ctrl Pts',(59.4289384514506,-5.68000001972945,
-175.106577823109));
#171473=CARTESIAN_POINT('Ctrl Pts',(59.4410301448459,-5.68000001987896,
-175.051984501471));
#171474=CARTESIAN_POINT('Ctrl Pts',(59.4606225263251,-5.68000002012122,
-174.963525991253));
#171475=CARTESIAN_POINT('Ctrl Pts',(59.4753677357896,-5.68000001999999,
-174.874236789973));
#171476=CARTESIAN_POINT('Ctrl Pts',(59.485211909548,-5.68000001999999,-174.784118621956));
#171477=CARTESIAN_POINT('Ctrl Pts',(59.4950560833064,-5.68000001999999,
-174.694000453939));
#171478=CARTESIAN_POINT('Ctrl Pts',(59.5,-5.68000001999999,-174.603053692373));
#171479=CARTESIAN_POINT('Ctrl Pts',(59.5,-5.68000001999999,-174.511260182694));
#171480=CARTESIAN_POINT('Origin',(58.6082745331205,-6.18000001999999,-179.64995));
#171481=CARTESIAN_POINT('',(58.6082745331205,-5.68000001999999,-171.871644662643));
#171482=CARTESIAN_POINT('',(58.6082745331205,-5.68000001999999,-176.785131631246));
#171483=CARTESIAN_POINT('Origin',(58.6082745331205,-6.18000001999999,-171.871644662643));
#171484=CARTESIAN_POINT('',(58.1115942404669,-6.2375212064409,-179.64995));
#171485=CARTESIAN_POINT('Ctrl Pts',(58.4667946194619,-5.68000001999999,
-171.237717270032));
#171486=CARTESIAN_POINT('Ctrl Pts',(57.9641288550927,-5.68000002000002,
-171.47368839131));
#171487=CARTESIAN_POINT('Ctrl Pts',(58.0166638356104,-6.23225639415715,
-171.449026400902));
#171488=CARTESIAN_POINT('Ctrl Pts',(58.559801654985,-5.68000001999999,-171.435840927268));
#171489=CARTESIAN_POINT('Ctrl Pts',(58.0192749608379,-5.68000001999239,
-171.600361788065));
#171490=CARTESIAN_POINT('Ctrl Pts',(58.0790703543615,-6.23572556787351,
-171.581106868264));
#171491=CARTESIAN_POINT('Ctrl Pts',(58.608274529079,-5.68000001999999,-171.650520905847));
#171492=CARTESIAN_POINT('Ctrl Pts',(58.0470269895722,-5.68000001999999,
-171.733866658521));
#171493=CARTESIAN_POINT('Ctrl Pts',(58.1115942404139,-6.23752120598293,
-171.724230304954));
#171494=CARTESIAN_POINT('Ctrl Pts',(58.6082745331205,-5.68000001999999,
-171.871644662643));
#171495=CARTESIAN_POINT('Ctrl Pts',(58.0470269915054,-5.68000001999999,
-171.871644662643));
#171496=CARTESIAN_POINT('Ctrl Pts',(58.1115942404669,-6.2375212064409,-171.871644662643));
#171497=CARTESIAN_POINT('',(58.4667946194619,-5.68000001999999,-171.237717270032));
#171498=CARTESIAN_POINT('Origin',(56.431269633621,-5.68000001999999,-172.018134872838));
#171499=CARTESIAN_POINT('Origin',(58.4667946194619,-6.18000001999999,-171.237717270032));
#171500=CARTESIAN_POINT('Ctrl Pts',(39.9791515366304,-5.68000001999998,
-131.975599874271));
#171501=CARTESIAN_POINT('Ctrl Pts',(39.452498014741,-5.68000001999998,-132.224696623613));
#171502=CARTESIAN_POINT('Ctrl Pts',(39.532390596256,-6.25584930059378,-132.186909005141));
#171503=CARTESIAN_POINT('Ctrl Pts',(46.164205183661,-5.68000001999998,-145.052367414711));
#171504=CARTESIAN_POINT('Ctrl Pts',(45.5680069655751,-5.68000001999999,
-145.12303284731));
#171505=CARTESIAN_POINT('Ctrl Pts',(45.7155147614494,-6.24444363034862,
-145.263691191481));
#171506=CARTESIAN_POINT('Ctrl Pts',(52.3196619691199,-5.68000001999999,
-158.143093167052));
#171507=CARTESIAN_POINT('Ctrl Pts',(51.7735675289641,-5.68000001999999,
-158.300965634462));
#171508=CARTESIAN_POINT('Ctrl Pts',(51.870165118292,-6.23767750446664,-158.354412070984));
#171509=CARTESIAN_POINT('Ctrl Pts',(58.4667946194619,-5.68000001999999,
-171.237717270032));
#171510=CARTESIAN_POINT('Ctrl Pts',(57.9641288550927,-5.68000001999999,
-171.47368839131));
#171511=CARTESIAN_POINT('Ctrl Pts',(58.0166638356104,-6.23225639415715,
-171.449026400902));
#171512=CARTESIAN_POINT('',(39.9791515366304,-5.68000001999998,-131.975599874271));
#171513=CARTESIAN_POINT('Ctrl Pts',(39.9791515366304,-5.68000001999998,
-131.975599874271));
#171514=CARTESIAN_POINT('Ctrl Pts',(46.164205183661,-5.68000001999998,-145.052367414711));
#171515=CARTESIAN_POINT('Ctrl Pts',(52.3196619691199,-5.68000001999999,
-158.143093167052));
#171516=CARTESIAN_POINT('Ctrl Pts',(58.4667946194619,-5.68000001999999,
-171.237717270032));
#171517=CARTESIAN_POINT('Origin',(39.9791515366304,-6.18000001999998,-131.975599874271));
#171518=CARTESIAN_POINT('Ctrl Pts',(39.618753076714,-6.26204052658076,-132.359337517737));
#171519=CARTESIAN_POINT('Ctrl Pts',(39.532762793516,-5.68000001999998,-132.403808231301));
#171520=CARTESIAN_POINT('Ctrl Pts',(40.0568611319685,-5.68000001999998,
-132.132760898312));
#171521=CARTESIAN_POINT('Ctrl Pts',(39.3987722978057,-6.2471624346873,-131.938591278504));
#171522=CARTESIAN_POINT('Ctrl Pts',(39.3306902060804,-5.68000001999999,
-131.97378409023));
#171523=CARTESIAN_POINT('Ctrl Pts',(39.8588799388418,-5.68000001999998,
-131.74924323321));
#171524=CARTESIAN_POINT('Ctrl Pts',(39.2388485421598,-6.2323178027174,-131.500725395993));
#171525=CARTESIAN_POINT('Ctrl Pts',(39.184800952389,-5.68000001999998,-131.524152834328));
#171526=CARTESIAN_POINT('Ctrl Pts',(39.7149524852865,-5.68000001999998,
-131.350461425493));
#171527=CARTESIAN_POINT('Ctrl Pts',(39.0323991983154,-6.20294681074234,
-130.592962730002));
#171528=CARTESIAN_POINT('Ctrl Pts',(39.0100410980795,-5.68000001999998,
-130.601991338715));
#171529=CARTESIAN_POINT('Ctrl Pts',(39.5291545030825,-5.68000001999998,
-130.524411418172));
#171530=CARTESIAN_POINT('Ctrl Pts',(38.9864634800499,-6.18831094500166,
-130.119221198789));
#171531=CARTESIAN_POINT('Ctrl Pts',(38.9779951282223,-5.68000001999999,
-130.125131443124));
#171532=CARTESIAN_POINT('Ctrl Pts',(39.4878153045286,-5.68000001999998,
-130.093651490435));
#171533=CARTESIAN_POINT('Ctrl Pts',(39.0034550536173,-6.17442081705026,
-129.647293013264));
#171534=CARTESIAN_POINT('Ctrl Pts',(39.0089685715929,-5.68000001999997,
-129.647466586728));
#171535=CARTESIAN_POINT('Ctrl Pts',(39.5031107769257,-5.68000001999998,
-129.664863321024));
#171536=CARTESIAN_POINT('',(39.5,-5.68000001999998,-129.839692850412));
#171537=CARTESIAN_POINT('Ctrl Pts',(39.5,-5.68000001999998,-129.839692850412));
#171538=CARTESIAN_POINT('Ctrl Pts',(39.5,-5.68000001999998,-130.074011953488));
#171539=CARTESIAN_POINT('Ctrl Pts',(39.5166979118863,-5.68000001999998,
-130.308218863682));
#171540=CARTESIAN_POINT('Ctrl Pts',(39.5492808611194,-5.68000001999998,
-130.539004174579));
#171541=CARTESIAN_POINT('Ctrl Pts',(39.5682253579849,-5.68000001999998,
-130.673188209537));
#171542=CARTESIAN_POINT('Ctrl Pts',(39.592538815617,-5.68000001999998,-130.806215404487));
#171543=CARTESIAN_POINT('Ctrl Pts',(39.6220534778078,-5.68000001999998,
-130.937436349817));
#171544=CARTESIAN_POINT('Ctrl Pts',(39.6907803864138,-5.68000001999998,
-131.242993291602));
#171545=CARTESIAN_POINT('Ctrl Pts',(39.7874256609062,-5.68000001999998,
-131.540730203369));
#171546=CARTESIAN_POINT('Ctrl Pts',(39.9132393368524,-5.68000001999998,
-131.830296953039));
#171547=CARTESIAN_POINT('Ctrl Pts',(39.9343840561751,-5.68000001999998,
-131.878962629492));
#171548=CARTESIAN_POINT('Ctrl Pts',(39.9563527642584,-5.68000001999998,
-131.927397503922));
#171549=CARTESIAN_POINT('Ctrl Pts',(39.9791515366304,-5.68000001999998,
-131.975599874271));
#171550=CARTESIAN_POINT('Origin',(39.5,-6.18000001999998,-129.839692850412));
#171551=CARTESIAN_POINT('Origin',(39.5,-6.18000001999998,-55.24995));
#171552=CARTESIAN_POINT('',(39.5,-5.68000001999998,-102.218950121094));
#171553=CARTESIAN_POINT('',(39.5,-5.68000001999998,-55.24995));
#171554=CARTESIAN_POINT('Origin',(39.5,-6.18000001999998,-102.218950121094));
#171555=CARTESIAN_POINT('Ctrl Pts',(39.,-6.18000001999998,-102.218950121094));
#171556=CARTESIAN_POINT('Ctrl Pts',(39.,-5.68000001999997,-102.218950121094));
#171557=CARTESIAN_POINT('Ctrl Pts',(39.5,-5.68000001999998,-102.218950121094));
#171558=CARTESIAN_POINT('Ctrl Pts',(39.,-6.19216140385576,-101.811197248376));
#171559=CARTESIAN_POINT('Ctrl Pts',(38.9876888787772,-5.68000001999998,
-101.806176686079));
#171560=CARTESIAN_POINT('Ctrl Pts',(39.5000000028438,-5.68000001999998,
-101.848394057804));
#171561=CARTESIAN_POINT('Ctrl Pts',(39.0453283089643,-6.20458878978192,
-101.411268531309));
#171562=CARTESIAN_POINT('Ctrl Pts',(39.0208449410789,-5.68000001999935,
-101.403186844504));
#171563=CARTESIAN_POINT('Ctrl Pts',(39.5407954776771,-5.68000001999998,
-101.484716832152));
#171564=CARTESIAN_POINT('Ctrl Pts',(39.2226569363477,-6.22996106887011,
-100.626634066533));
#171565=CARTESIAN_POINT('Ctrl Pts',(39.1707994584459,-5.68000002000062,
-100.606268005686));
#171566=CARTESIAN_POINT('Ctrl Pts',(39.7003912431037,-5.68000001999998,
-100.770720159946));
#171567=CARTESIAN_POINT('Ctrl Pts',(39.3562549507175,-6.24299658541821,
-100.239515789679));
#171568=CARTESIAN_POINT('Ctrl Pts',(39.2916053087195,-5.68000001999999,
-100.209430566875));
#171569=CARTESIAN_POINT('Ctrl Pts',(39.8206290570768,-5.68000001999998,
-100.418199709297));
#171570=CARTESIAN_POINT('Ctrl Pts',(39.532390596256,-6.25584930059378,-99.8717339663646));
#171571=CARTESIAN_POINT('Ctrl Pts',(39.4524980147409,-5.68000001999997,
-99.8339463478928));
#171572=CARTESIAN_POINT('Ctrl Pts',(39.9791515366304,-5.68000001999998,
-100.083043097235));
#171573=CARTESIAN_POINT('',(39.9791515366304,-5.68000001999998,-100.083043097235));
#171574=CARTESIAN_POINT('Ctrl Pts',(39.9791515366304,-5.68000001999998,
-100.083043097235));
#171575=CARTESIAN_POINT('Ctrl Pts',(39.8867451235786,-5.68000001999998,
-100.278413622974));
#171576=CARTESIAN_POINT('Ctrl Pts',(39.8073027352592,-5.68000001999998,
-100.479790373913));
#171577=CARTESIAN_POINT('Ctrl Pts',(39.7413121766283,-5.68000001999998,
-100.684533556806));
#171578=CARTESIAN_POINT('Ctrl Pts',(39.6941478985853,-5.68000001999998,
-100.830866071725));
#171579=CARTESIAN_POINT('Ctrl Pts',(39.6538540640997,-5.68000001999998,
-100.978917355183));
#171580=CARTESIAN_POINT('Ctrl Pts',(39.6205933601941,-5.68000001999998,
-101.127718496005));
#171581=CARTESIAN_POINT('Ctrl Pts',(39.551582895664,-5.68000001999998,-101.436456274974));
#171582=CARTESIAN_POINT('Ctrl Pts',(39.5117440271939,-5.68000001999998,
-101.750163184502));
#171583=CARTESIAN_POINT('Ctrl Pts',(39.5022324725657,-5.68000001999998,
-102.069036097533));
#171584=CARTESIAN_POINT('Ctrl Pts',(39.5007456673957,-5.68000001999998,
-102.118880935121));
#171585=CARTESIAN_POINT('Ctrl Pts',(39.5,-5.68000001999998,-102.168852019186));
#171586=CARTESIAN_POINT('Ctrl Pts',(39.5,-5.68000001999998,-102.218950121094));
#171587=CARTESIAN_POINT('',(39.5323905862198,-6.25584928266823,-99.8717340064415));
#171588=CARTESIAN_POINT('Origin',(39.9791515366304,-6.18000001999998,-100.083043097235));
#171589=CARTESIAN_POINT('Ctrl Pts',(39.,-6.18000001999998,-102.218950121094));
#171590=CARTESIAN_POINT('Ctrl Pts',(39.,-6.18280348526599,-102.124954155648));
#171591=CARTESIAN_POINT('Ctrl Pts',(39.002404218496,-6.1857384871018,-102.026328836378));
#171592=CARTESIAN_POINT('Ctrl Pts',(39.0079897759941,-6.18884348395754,
-101.923270891007));
#171593=CARTESIAN_POINT('Ctrl Pts',(39.0125734589699,-6.19139154137743,
-101.838698321506));
#171594=CARTESIAN_POINT('Ctrl Pts',(39.0193007259262,-6.19405410413894,
-101.751140850617));
#171595=CARTESIAN_POINT('Ctrl Pts',(39.0286266629022,-6.19685324413035,
-101.660712168677));
#171596=CARTESIAN_POINT('Ctrl Pts',(39.0389718041625,-6.1999582939171,-101.560400801459));
#171597=CARTESIAN_POINT('Ctrl Pts',(39.0525152513023,-6.2032250360155,-101.456576568294));
#171598=CARTESIAN_POINT('Ctrl Pts',(39.0698700180508,-6.20663833765055,
-101.34953622736));
#171599=CARTESIAN_POINT('Ctrl Pts',(39.078547401425,-6.20834498846808,-101.296016056893));
#171600=CARTESIAN_POINT('Ctrl Pts',(39.0881773224577,-6.21008774743007,
-101.241693476407));
#171601=CARTESIAN_POINT('Ctrl Pts',(39.0988327090458,-6.21186142692311,
-101.186615167821));
#171602=CARTESIAN_POINT('Ctrl Pts',(39.1041604023398,-6.21274826666963,
-101.159076013528));
#171603=CARTESIAN_POINT('Ctrl Pts',(39.1097444325043,-6.21364284141544,
-101.131347913177));
#171604=CARTESIAN_POINT('Ctrl Pts',(39.1155935001094,-6.21454424764705,
-101.1034374055));
#171605=CARTESIAN_POINT('Ctrl Pts',(39.1185180339119,-6.21499495076286,
-101.089482151662));
#171606=CARTESIAN_POINT('Ctrl Pts',(39.1215088240554,-6.21544736233241,
-101.075481294353));
#171607=CARTESIAN_POINT('Ctrl Pts',(39.1245669329916,-6.21590136327086,
-101.061435665813));
#171608=CARTESIAN_POINT('Ctrl Pts',(39.1260959874597,-6.21612836374009,
-101.054412851542));
#171609=CARTESIAN_POINT('Ctrl Pts',(39.1276418714215,-6.21635576159457,
-101.047378844344));
#171610=CARTESIAN_POINT('Ctrl Pts',(39.1292047157078,-6.21658354115136,
-101.040333750366));
#171611=CARTESIAN_POINT('Ctrl Pts',(39.129986137851,-6.21669743092976,-101.036811203377));
#171612=CARTESIAN_POINT('Ctrl Pts',(39.1307718000616,-6.21681141613672,
-101.033285884685));
#171613=CARTESIAN_POINT('Ctrl Pts',(39.1315617185623,-6.21692549475772,
-101.0297578077));
#171614=CARTESIAN_POINT('Ctrl Pts',(39.132351637063,-6.21703957337873,-101.026229730715));
#171615=CARTESIAN_POINT('Ctrl Pts',(39.1334695671107,-6.21720007707638,
-101.021266095499));
#171616=CARTESIAN_POINT('Ctrl Pts',(39.133944259014,-6.21726800786083,-101.019165315283));
#171617=CARTESIAN_POINT('Ctrl Pts',(39.1339603748108,-6.21727031411192,
-101.019093993765));
#171618=CARTESIAN_POINT('Ctrl Pts',(39.1339764959978,-6.21727262090659,
-101.019022654972));
#171619=CARTESIAN_POINT('Ctrl Pts',(39.1339926225771,-6.21727492824492,
-101.018951298903));
#171620=CARTESIAN_POINT('Ctrl Pts',(39.1415847113272,-6.21836117952214,
-100.985358210486));
#171621=CARTESIAN_POINT('Ctrl Pts',(39.1503796125988,-6.21956859795788,
-100.947916935796));
#171622=CARTESIAN_POINT('Ctrl Pts',(39.1606238041844,-6.22090460123468,
-100.906695960147));
#171623=CARTESIAN_POINT('Ctrl Pts',(39.17086799577,-6.22224060451149,-100.865474984498));
#171624=CARTESIAN_POINT('Ctrl Pts',(39.1825616354608,-6.22370521203984,
-100.820473748147));
#171625=CARTESIAN_POINT('Ctrl Pts',(39.1959980262754,-6.22530555624786,
-100.771786764605));
#171626=CARTESIAN_POINT('Ctrl Pts',(39.2094486874067,-6.22690760012501,
-100.723048072335));
#171627=CARTESIAN_POINT('Ctrl Pts',(39.2246457230915,-6.22864484024711,
-100.670616186616));
#171628=CARTESIAN_POINT('Ctrl Pts',(39.241924393445,-6.23051375185755,-100.614627493635));
#171629=CARTESIAN_POINT('Ctrl Pts',(39.2505637286217,-6.23144820766277,
-100.586633147144));
#171630=CARTESIAN_POINT('Ctrl Pts',(39.2597240993998,-6.23241542427668,
-100.55775027571));
#171631=CARTESIAN_POINT('Ctrl Pts',(39.2694509482011,-6.23341381238282,
-100.528000444015));
#171632=CARTESIAN_POINT('Ctrl Pts',(39.276025240513,-6.23408861420041,-100.507892792113));
#171633=CARTESIAN_POINT('Ctrl Pts',(39.2826944322007,-6.23476065600126,
-100.487877252101));
#171634=CARTESIAN_POINT('Ctrl Pts',(39.2898035531922,-6.23546318331865,
-100.466971130998));
#171635=CARTESIAN_POINT('Ctrl Pts',(39.2932125749473,-6.23580006475749,
-100.456946062956));
#171636=CARTESIAN_POINT('Ctrl Pts',(39.2967234539788,-6.23614395786301,
-100.446716396379));
#171637=CARTESIAN_POINT('Ctrl Pts',(39.3003783770287,-6.23649853510275,
-100.43617497279));
#171638=CARTESIAN_POINT('Ctrl Pts',(39.3204952758673,-6.23845014786308,
-100.378154393679));
#171639=CARTESIAN_POINT('Ctrl Pts',(39.3404185039594,-6.24028810043805,
-100.323848615045));
#171640=CARTESIAN_POINT('Ctrl Pts',(39.3598170113798,-6.24201123183849,
-100.273176028293));
#171641=CARTESIAN_POINT('Ctrl Pts',(39.3797647162903,-6.24378314737576,
-100.22106883336));
#171642=CARTESIAN_POINT('Ctrl Pts',(39.3991575025057,-6.2454336686,-100.172802869366));
#171643=CARTESIAN_POINT('Ctrl Pts',(39.4176886735397,-6.24696265708752,
-100.128275640437));
#171644=CARTESIAN_POINT('Ctrl Pts',(39.4364188261594,-6.24850806334774,
-100.083270292852));
#171645=CARTESIAN_POINT('Ctrl Pts',(39.454268839455,-6.24992933485546,-100.042083812078));
#171646=CARTESIAN_POINT('Ctrl Pts',(39.4709753783267,-6.25122713146687,
-100.004605647237));
#171647=CARTESIAN_POINT('Ctrl Pts',(39.487832770042,-6.25253664662219,-99.9667890707241));
#171648=CARTESIAN_POINT('Ctrl Pts',(39.5035260267009,-6.25372046637617,
-99.9327475642426));
#171649=CARTESIAN_POINT('Ctrl Pts',(39.5178373919463,-6.25477976690218,
-99.9023711938222));
#171650=CARTESIAN_POINT('Ctrl Pts',(39.5228608944142,-6.25515159717242,
-99.8917086351383));
#171651=CARTESIAN_POINT('Ctrl Pts',(39.5277145979465,-6.25550808835496,
-99.8814977315729));
#171652=CARTESIAN_POINT('Ctrl Pts',(39.5323905785446,-6.25584929930136,
-99.871734003347));
#171653=CARTESIAN_POINT('Ctrl Pts',(58.3535376001277,-5.68000001999999,
-61.0621827299711));
#171654=CARTESIAN_POINT('Ctrl Pts',(57.8507724536939,-5.68000001999999,
-60.826158857425));
#171655=CARTESIAN_POINT('Ctrl Pts',(57.9034184448965,-6.23235646472971,
-60.8508735991007));
#171656=CARTESIAN_POINT('Ctrl Pts',(52.2440275184664,-5.68000001999999,
-74.0763270103718));
#171657=CARTESIAN_POINT('Ctrl Pts',(51.698167660392,-5.68000001999999,-73.9177186732266));
#171658=CARTESIAN_POINT('Ctrl Pts',(51.794541964381,-6.23776491179514,-73.865008277307));
#171659=CARTESIAN_POINT('Ctrl Pts',(46.1262203434603,-5.68000001999998,
-87.0865851147193));
#171660=CARTESIAN_POINT('Ctrl Pts',(45.5309288684318,-5.68000001999999,
-87.0138122441779));
#171661=CARTESIAN_POINT('Ctrl Pts',(45.6775416788308,-6.24451367719405,
-86.8752616229197));
#171662=CARTESIAN_POINT('Ctrl Pts',(39.9791515366304,-5.68000001999998,
-100.083043097235));
#171663=CARTESIAN_POINT('Ctrl Pts',(39.4524980147409,-5.68000001999998,
-99.8339463478929));
#171664=CARTESIAN_POINT('Ctrl Pts',(39.532390596256,-6.25584930059378,-99.8717339663645));
#171665=CARTESIAN_POINT('',(58.3535376001277,-5.68000001999999,-61.0621827299711));
#171666=CARTESIAN_POINT('Ctrl Pts',(58.3535376001277,-5.68000001999999,
-61.0621827299711));
#171667=CARTESIAN_POINT('Ctrl Pts',(52.2440275184664,-5.68000001999999,
-74.0763270103718));
#171668=CARTESIAN_POINT('Ctrl Pts',(46.1262203434603,-5.68000001999998,
-87.0865851147193));
#171669=CARTESIAN_POINT('Ctrl Pts',(39.9791515366304,-5.68000001999998,
-100.083043097235));
#171670=CARTESIAN_POINT('',(57.9034184448965,-6.23235646472971,-60.8508735991007));
#171671=CARTESIAN_POINT('Origin',(58.3535376001277,-6.18000001999999,-61.0621827299711));
#171672=CARTESIAN_POINT('Ctrl Pts',(39.532390596256,-6.25584930059377,-99.8717339663646));
#171673=CARTESIAN_POINT('Ctrl Pts',(40.911961747875,-6.25330448130522,-96.9540582124415));
#171674=CARTESIAN_POINT('Ctrl Pts',(42.3682944181388,-6.25068917191027,
-93.8698701165745));
#171675=CARTESIAN_POINT('Ctrl Pts',(44.6679782761596,-6.24721138579723,
-88.9938194598585));
#171676=CARTESIAN_POINT('Ctrl Pts',(45.4537358898071,-6.24611496597599,
-87.3268411554672));
#171677=CARTESIAN_POINT('Ctrl Pts',(46.6611636792454,-6.24453107456046,
-84.7639315706514));
#171678=CARTESIAN_POINT('Ctrl Pts',(47.2720753433432,-6.24375324528844,
-83.4668662461863));
#171679=CARTESIAN_POINT('Ctrl Pts',(47.9974003487209,-6.24285185802002,
-81.9263049365434));
#171680=CARTESIAN_POINT('Ctrl Pts',(48.3632113198011,-6.24239951385331,
-81.1491946739469));
#171681=CARTESIAN_POINT('Ctrl Pts',(48.5698654666445,-6.24214413381149,
-80.7101493240497));
#171682=CARTESIAN_POINT('Ctrl Pts',(48.6718338188353,-6.24201809389911,
-80.4935007144023));
#171683=CARTESIAN_POINT('Ctrl Pts',(48.7245329191054,-6.24195292792929,
-80.3815296305629));
#171684=CARTESIAN_POINT('Ctrl Pts',(48.7283847105348,-6.24194816478105,
-80.3733456164068));
#171685=CARTESIAN_POINT('Ctrl Pts',(51.5332710940133,-6.23847954177077,
-74.4137117874514));
#171686=CARTESIAN_POINT('Ctrl Pts',(54.5907059876843,-6.23528934935773,
-67.9081592073181));
#171687=CARTESIAN_POINT('Ctrl Pts',(57.9034184448965,-6.23235646472971,
-60.8508735991007));
#171688=CARTESIAN_POINT('Ctrl Pts',(39.,-5.46102446043621,-101.971753092595));
#171689=CARTESIAN_POINT('Ctrl Pts',(39.,-5.86351617202512,-100.855722952121));
#171690=CARTESIAN_POINT('Ctrl Pts',(39.5330007135517,-6.22310220971892,
-99.8586617838914));
#171691=CARTESIAN_POINT('Ctrl Pts',(39.,-6.48207062104881,-102.33998922066));
#171692=CARTESIAN_POINT('Ctrl Pts',(38.9999999999962,-6.82975403393395,
-101.225648609944));
#171693=CARTESIAN_POINT('Ctrl Pts',(39.5158163721933,-7.1434218710037,-100.226898392254));
#171694=CARTESIAN_POINT('Ctrl Pts',(39.,-7.52739464652098,-102.644232481647));
#171695=CARTESIAN_POINT('Ctrl Pts',(39.,-7.81966925102655,-101.531783862877));
#171696=CARTESIAN_POINT('Ctrl Pts',(39.50142226749,-8.08385740698738,-100.53114117287));
#171697=CARTESIAN_POINT('Ctrl Pts',(39.,-9.13906178103241,-102.985482622022));
#171698=CARTESIAN_POINT('Ctrl Pts',(39.,-9.34536808184436,-101.875027810475));
#171699=CARTESIAN_POINT('Ctrl Pts',(39.485193560998,-9.53196095727464,-100.872391313355));
#171700=CARTESIAN_POINT('Ctrl Pts',(39.,-9.68642581410213,-103.080287874832));
#171701=CARTESIAN_POINT('Ctrl Pts',(39.,-9.86335482772211,-101.970380205613));
#171702=CARTESIAN_POINT('Ctrl Pts',(39.4806657492121,-10.0234751165263,
-100.967196566129));
#171703=CARTESIAN_POINT('Ctrl Pts',(39.,-10.7786703656218,-103.225601722724));
#171704=CARTESIAN_POINT('Ctrl Pts',(39.,-10.8967689955421,-102.116504004052));
#171705=CARTESIAN_POINT('Ctrl Pts',(39.4737139394979,-11.0038787161503,
-101.11251041402));
#171706=CARTESIAN_POINT('Ctrl Pts',(39.,-11.32407160958,-103.276476522877));
#171707=CARTESIAN_POINT('Ctrl Pts',(39.0000000000038,-11.4127969575427,
-102.167673995048));
#171708=CARTESIAN_POINT('Ctrl Pts',(39.4712727906473,-11.493239882702,-101.16338521793));
#171709=CARTESIAN_POINT('Ctrl Pts',(39.,-11.8687533077036,-103.305636003273));
#171710=CARTESIAN_POINT('Ctrl Pts',(39.,-11.9281041096302,-102.196998431102));
#171711=CARTESIAN_POINT('Ctrl Pts',(39.4698732852484,-11.9818774403001,
-101.192544694569));
#171712=CARTESIAN_POINT('',(39.470299293038,-11.8429061139822,-101.18366751689));
#171713=CARTESIAN_POINT('Ctrl Pts',(39.4702992602694,-11.8429061149159,
-101.183667501603));
#171714=CARTESIAN_POINT('Ctrl Pts',(39.4714157143871,-11.5010965926809,
-101.160397081716));
#171715=CARTESIAN_POINT('Ctrl Pts',(39.4730376963082,-11.1594525392257,
-101.126547380785));
#171716=CARTESIAN_POINT('Ctrl Pts',(39.4751582271049,-10.8177256429982,
-101.08215692154));
#171717=CARTESIAN_POINT('Ctrl Pts',(39.4757870845495,-10.7163842698549,
-101.068992637007));
#171718=CARTESIAN_POINT('Ctrl Pts',(39.4764598030603,-10.6150355967854,
-101.054900989002));
#171719=CARTESIAN_POINT('Ctrl Pts',(39.4771762399035,-10.5136731096961,
-101.039882102517));
#171720=CARTESIAN_POINT('Ctrl Pts',(39.4773994513674,-10.4820928394407,
-101.035202851763));
#171721=CARTESIAN_POINT('Ctrl Pts',(39.4776269777968,-10.4505092705441,
-101.03043207286));
#171722=CARTESIAN_POINT('Ctrl Pts',(39.4778587715597,-10.418924943814,-101.025570636239));
#171723=CARTESIAN_POINT('Ctrl Pts',(39.4790878128322,-10.2514552042292,
-100.999793815603));
#171724=CARTESIAN_POINT('Ctrl Pts',(39.4804337172402,-10.0839399037763,
-100.971475421647));
#171725=CARTESIAN_POINT('Ctrl Pts',(39.4819042200723,-9.91634393709639,
-100.940630337302));
#171726=CARTESIAN_POINT('Ctrl Pts',(39.4825182652867,-9.8463600519611,-100.927750201326));
#171727=CARTESIAN_POINT('Ctrl Pts',(39.4831540697067,-9.77636222049717,
-100.91442887348));
#171728=CARTESIAN_POINT('Ctrl Pts',(39.4838123356305,-9.70634878432406,
-100.900664901762));
#171729=CARTESIAN_POINT('Ctrl Pts',(39.4849296694305,-9.58750869878921,
-100.877302077913));
#171730=CARTESIAN_POINT('Ctrl Pts',(39.4861104003532,-9.46862238083702,
-100.852667202291));
#171731=CARTESIAN_POINT('Ctrl Pts',(39.4873506398552,-9.34967902011701,
-100.826758874769));
#171732=CARTESIAN_POINT('Ctrl Pts',(39.4879707596062,-9.29020733975701,
-100.813804711008));
#171733=CARTESIAN_POINT('Ctrl Pts',(39.4886056849366,-9.23072140625689,
-100.800532150721));
#171734=CARTESIAN_POINT('Ctrl Pts',(39.4892544851105,-9.17121992545558,
-100.786940815446));
#171735=CARTESIAN_POINT('Ctrl Pts',(39.4895788851974,-9.14146918505491,
-100.780145147809));
#171736=CARTESIAN_POINT('Ctrl Pts',(39.4899067493168,-9.11171455870462,
-100.77326978421));
#171737=CARTESIAN_POINT('Ctrl Pts',(39.4902378654102,-9.08195585995781,
-100.76631480003));
#171738=CARTESIAN_POINT('Ctrl Pts',(39.4903578915464,-9.07116864151043,
-100.76379369068));
#171739=CARTESIAN_POINT('Ctrl Pts',(39.4904803125607,-9.06020644484888,
-100.76122118129));
#171740=CARTESIAN_POINT('Ctrl Pts',(39.4906030413979,-9.04925973560232,
-100.758641447143));
#171741=CARTESIAN_POINT('Ctrl Pts',(39.4908188845949,-9.03000775884592,
-100.754104468886));
#171742=CARTESIAN_POINT('Ctrl Pts',(39.4910357318681,-9.01079978065262,
-100.749544053052));
#171743=CARTESIAN_POINT('Ctrl Pts',(39.4912417658406,-8.99266748358911,
-100.745210479822));
#171744=CARTESIAN_POINT('Ctrl Pts',(39.496412730107,-8.53758981341583,-100.636448065327));
#171745=CARTESIAN_POINT('Ctrl Pts',(39.5024412863883,-8.08236775931935,
-100.509291986928));
#171746=CARTESIAN_POINT('Ctrl Pts',(39.5093071903843,-7.62642775454604,
-100.363713049691));
#171747=CARTESIAN_POINT('Ctrl Pts',(39.5152832138175,-7.22958151925537,
-100.237002402292));
#171748=CARTESIAN_POINT('Ctrl Pts',(39.5218935920656,-6.83219144237864,
-100.096334431291));
#171749=CARTESIAN_POINT('Ctrl Pts',(39.5291209804618,-6.43385878842381,
-99.9417276591744));
#171750=CARTESIAN_POINT('Ctrl Pts',(39.5301971998785,-6.37454367859804,
-99.9187053998219));
#171751=CARTESIAN_POINT('Ctrl Pts',(39.5312870926446,-6.31520762564802,
-99.8953741493161));
#171752=CARTESIAN_POINT('Ctrl Pts',(39.5323905926521,-6.25584926600113,
-99.8717340627362));
#171753=CARTESIAN_POINT('Origin',(46.4732015204142,-11.8458781654969,-103.848204069008));
#171754=CARTESIAN_POINT('Ctrl Pts',(39.4702993039609,-11.842906113671,-101.183667521985));
#171755=CARTESIAN_POINT('Ctrl Pts',(39.4816972464314,-12.33000002,-101.188984626754));
#171756=CARTESIAN_POINT('Ctrl Pts',(39.9232693735648,-12.33000002,-101.394976652855));
#171757=CARTESIAN_POINT('Ctrl Pts',(39.1608544296035,-11.8384595965422,
-101.84673342232));
#171758=CARTESIAN_POINT('Ctrl Pts',(39.1678459389433,-12.3300000200023,
-101.851466764233));
#171759=CARTESIAN_POINT('Ctrl Pts',(39.6447687306727,-12.33000002,-101.991980946201));
#171760=CARTESIAN_POINT('Ctrl Pts',(39.,-11.834085348836,-102.564353929887));
#171761=CARTESIAN_POINT('Ctrl Pts',(39.0040688095373,-12.3300000199977,
-102.567343181294));
#171762=CARTESIAN_POINT('Ctrl Pts',(39.5000000016323,-12.33000002,-102.638067201068));
#171763=CARTESIAN_POINT('Ctrl Pts',(39.,-11.83000002,-103.303524786513));
#171764=CARTESIAN_POINT('Ctrl Pts',(39.,-12.33000002,-103.303524786513));
#171765=CARTESIAN_POINT('Ctrl Pts',(39.5,-12.33000002,-103.303524786513));
#171766=CARTESIAN_POINT('',(39.5,-12.33000002,-103.303524786513));
#171767=CARTESIAN_POINT('Origin',(39.5,-11.83000002,-103.303524786513));
#171768=CARTESIAN_POINT('',(39.9232693735648,-12.33000002,-101.394976652855));
#171769=CARTESIAN_POINT('Origin',(39.9232693735648,-11.83000002,-101.394976652855));
#171770=CARTESIAN_POINT('Origin',(46.190877869282,-12.33000002,-103.784865184748));
#171771=CARTESIAN_POINT('Origin',(39.5,-11.83000002,-55.24995));
#171772=CARTESIAN_POINT('',(39.5,-12.33000002,-128.755118184993));
#171773=CARTESIAN_POINT('Origin',(39.5,-11.83000002,-128.755118184993));
#171774=CARTESIAN_POINT('',(39.5,-12.33000002,-55.24995));
#171775=CARTESIAN_POINT('Ctrl Pts',(39.,-11.83000002,-128.755118184993));
#171776=CARTESIAN_POINT('Ctrl Pts',(39.,-12.33000002,-128.755118184993));
#171777=CARTESIAN_POINT('Ctrl Pts',(39.5,-12.33000002,-128.755118184993));
#171778=CARTESIAN_POINT('Ctrl Pts',(39.,-11.8340442872404,-129.486859645108));
#171779=CARTESIAN_POINT('Ctrl Pts',(39.0040281122736,-12.33000002,-129.483935534574));
#171780=CARTESIAN_POINT('Ctrl Pts',(39.5000000055219,-12.33000002,-129.413887248834));
#171781=CARTESIAN_POINT('Ctrl Pts',(39.1577125252496,-11.8384144493887,
-130.205177204234));
#171782=CARTESIAN_POINT('Ctrl Pts',(39.1646430478985,-12.33000002,-130.200415506093));
#171783=CARTESIAN_POINT('Ctrl Pts',(39.6419410176262,-12.33000002,-130.060600444225));
#171784=CARTESIAN_POINT('Ctrl Pts',(39.4702993039609,-11.8429061136709,
-130.874975449521));
#171785=CARTESIAN_POINT('Ctrl Pts',(39.4816972464314,-12.33000002,-130.869658344752));
#171786=CARTESIAN_POINT('Ctrl Pts',(39.9232693735648,-12.33000002,-130.663666318651));
#171787=CARTESIAN_POINT('',(39.9232693735648,-12.33000002,-130.663666318651));
#171788=CARTESIAN_POINT('Origin',(39.9232693735648,-11.83000002,-130.663666318651));
#171789=CARTESIAN_POINT('Origin',(46.1904260133955,-12.33000002,-128.271059668222));
#171790=CARTESIAN_POINT('Ctrl Pts',(58.8484691650909,-12.33000002,-171.237717270032));
#171791=CARTESIAN_POINT('Ctrl Pts',(58.4031988243933,-12.33000002,-171.445389024352));
#171792=CARTESIAN_POINT('Ctrl Pts',(58.3953999019963,-11.8387575339013,
-171.449026400902));
#171793=CARTESIAN_POINT('Ctrl Pts',(52.5405278046811,-12.33000002,-157.712819732222));
#171794=CARTESIAN_POINT('Ctrl Pts',(52.1019974789428,-12.3300000202716,
-157.93276270106));
#171795=CARTESIAN_POINT('Ctrl Pts',(52.0874768317228,-11.839695897332,-157.924129189572));
#171796=CARTESIAN_POINT('Ctrl Pts',(46.2323452217992,-12.33000002,-144.188034690057));
#171797=CARTESIAN_POINT('Ctrl Pts',(45.801395679434,-12.33000002,-144.421507685211));
#171798=CARTESIAN_POINT('Ctrl Pts',(45.7793173035632,-11.8408682174628,
-144.399344282617));
#171799=CARTESIAN_POINT('Ctrl Pts',(39.9232693735648,-12.33000002,-130.663666318651));
#171800=CARTESIAN_POINT('Ctrl Pts',(39.4816972464314,-12.33000002,-130.869658344752));
#171801=CARTESIAN_POINT('Ctrl Pts',(39.4702993039609,-11.842906113671,-130.874975449521));
#171802=CARTESIAN_POINT('',(58.8484691650909,-12.33000002,-171.237717270032));
#171803=CARTESIAN_POINT('Origin',(58.8484691650909,-11.83000002,-171.237717270032));
#171804=CARTESIAN_POINT('Ctrl Pts',(58.8484691650909,-12.33000002,-171.237717270032));
#171805=CARTESIAN_POINT('Ctrl Pts',(52.5405278046811,-12.33000002,-157.712819732223));
#171806=CARTESIAN_POINT('Ctrl Pts',(46.2323452217992,-12.33000002,-144.188034690057));
#171807=CARTESIAN_POINT('Ctrl Pts',(39.9232693735648,-12.33000002,-130.663666318651));
#171808=CARTESIAN_POINT('Ctrl Pts',(58.9890336736409,-12.33000002,-171.871644662643));
#171809=CARTESIAN_POINT('Ctrl Pts',(58.4985823439911,-12.33000002,-171.871644662643));
#171810=CARTESIAN_POINT('Ctrl Pts',(58.48912660861,-11.8396398505087,-171.871644662643));
#171811=CARTESIAN_POINT('Ctrl Pts',(58.9890336571231,-12.33000002,-171.652832645897));
#171812=CARTESIAN_POINT('Ctrl Pts',(58.4985823327705,-12.33000002,-171.724385262387));
#171813=CARTESIAN_POINT('Ctrl Pts',(58.4891266086039,-11.8396398501934,
-171.725770040011));
#171814=CARTESIAN_POINT('Ctrl Pts',(58.9418960593107,-12.33000002,-171.438034482585));
#171815=CARTESIAN_POINT('Ctrl Pts',(58.46651035226,-12.3300000200013,-171.579769437466));
#171816=CARTESIAN_POINT('Ctrl Pts',(58.4576958292209,-11.8393453695788,
-171.582571135794));
#171817=CARTESIAN_POINT('Ctrl Pts',(58.8484691650909,-12.33000002,-171.237717270032));
#171818=CARTESIAN_POINT('Ctrl Pts',(58.4031988243933,-12.33000002,-171.445389024352));
#171819=CARTESIAN_POINT('Ctrl Pts',(58.3953999019963,-11.8387575339013,
-171.449026400902));
#171820=CARTESIAN_POINT('',(58.9890336736409,-12.33000002,-171.871644662643));
#171821=CARTESIAN_POINT('Origin',(58.9890336736409,-11.83000002,-171.871644662643));
#171822=CARTESIAN_POINT('Origin',(56.7618024059963,-12.33000002,-172.033247591146));
#171823=CARTESIAN_POINT('Origin',(58.9890336736409,-11.83000002,-179.64995));
#171824=CARTESIAN_POINT('',(58.48912660861,-11.8396398505087,-179.64995));
#171825=CARTESIAN_POINT('',(58.9890336736409,-12.33000002,-171.871644662643));
#171826=CARTESIAN_POINT('Ctrl Pts',(60.,-12.83000002,-174.751778045593));
#171827=CARTESIAN_POINT('Ctrl Pts',(60.,-12.33000002,-174.751778045593));
#171828=CARTESIAN_POINT('Ctrl Pts',(59.5,-12.33000002,-174.751778045593));
#171829=CARTESIAN_POINT('Ctrl Pts',(60.,-12.8299432805227,-174.99625355239));
#171830=CARTESIAN_POINT('Ctrl Pts',(59.9999432570754,-12.33000002,-174.996239713811));
#171831=CARTESIAN_POINT('Ctrl Pts',(59.4999999944591,-12.33000002,-174.955507700223));
#171832=CARTESIAN_POINT('Ctrl Pts',(59.9705492201332,-12.8298880430416,
-175.2357685753));
#171833=CARTESIAN_POINT('Ctrl Pts',(59.970440441932,-12.33000002,-175.235742099222));
#171834=CARTESIAN_POINT('Ctrl Pts',(59.4754576845908,-12.33000002,-175.155103617038));
#171835=CARTESIAN_POINT('Ctrl Pts',(59.8547629729398,-12.8297804365705,
-175.705055936053));
#171836=CARTESIAN_POINT('Ctrl Pts',(59.8545561835904,-12.33000002,-175.704977777008));
#171837=CARTESIAN_POINT('Ctrl Pts',(59.3789691429701,-12.33000002,-175.546176541216));
#171838=CARTESIAN_POINT('Ctrl Pts',(59.7670622382429,-12.8297278961218,
-175.935624391263));
#171839=CARTESIAN_POINT('Ctrl Pts',(59.7668149966741,-12.3300000199993,
-175.935510188038));
#171840=CARTESIAN_POINT('Ctrl Pts',(59.3058851982286,-12.33000002,-175.738316981093));
#171841=CARTESIAN_POINT('Ctrl Pts',(59.5424974437338,-12.829631160742,-176.362316424594));
#171842=CARTESIAN_POINT('Ctrl Pts',(59.5421886833106,-12.3300000200007,
-176.362111673427));
#171843=CARTESIAN_POINT('Ctrl Pts',(59.1187478700854,-12.33000002,-176.093893786804));
#171844=CARTESIAN_POINT('Ctrl Pts',(59.4031198237833,-12.8295857148276,
-176.563935060575));
#171845=CARTESIAN_POINT('Ctrl Pts',(59.4027925942033,-12.3300000200005,
-176.563680085108));
#171846=CARTESIAN_POINT('Ctrl Pts',(59.0025998517383,-12.33000002,-176.261909367341));
#171847=CARTESIAN_POINT('Ctrl Pts',(59.0805964717746,-12.8295042980195,
-176.926638521725));
#171848=CARTESIAN_POINT('Ctrl Pts',(59.0802573870172,-12.3300000199995,
-176.926274585031));
#171849=CARTESIAN_POINT('Ctrl Pts',(58.73383039456,-12.33000002,-176.564162347066));
#171850=CARTESIAN_POINT('Ctrl Pts',(58.8998912349101,-12.8294686666967,
-177.086178383746));
#171851=CARTESIAN_POINT('Ctrl Pts',(58.8995591592806,-12.3300000199849,
-177.085762552869));
#171852=CARTESIAN_POINT('Ctrl Pts',(58.5832426931945,-12.33000002,-176.697112268189));
#171853=CARTESIAN_POINT('Ctrl Pts',(58.699732291115,-12.8294380172077,-177.223805132118));
#171854=CARTESIAN_POINT('Ctrl Pts',(58.699414230519,-12.33000002,-177.223342557405));
#171855=CARTESIAN_POINT('Ctrl Pts',(58.4164435759292,-12.33000002,-176.811801263203));
#171856=CARTESIAN_POINT('',(59.5,-12.33000002,-174.751778045594));
#171857=CARTESIAN_POINT('Ctrl Pts',(59.5,-12.33000002,-174.751778045594));
#171858=CARTESIAN_POINT('Ctrl Pts',(59.5,-12.33000002,-174.844927230273));
#171859=CARTESIAN_POINT('Ctrl Pts',(59.4948737621761,-12.3300000199839,
-174.937101433735));
#171860=CARTESIAN_POINT('Ctrl Pts',(59.4847164002782,-12.3300000200162,
-175.028427073489));
#171861=CARTESIAN_POINT('Ctrl Pts',(59.4744815669569,-12.3300000200487,
-175.120449264903));
#171862=CARTESIAN_POINT('Ctrl Pts',(59.4591385334095,-12.3300000199961,
-175.211609900805));
#171863=CARTESIAN_POINT('Ctrl Pts',(59.438732272217,-12.3300000210573,-175.302031274497));
#171864=CARTESIAN_POINT('Ctrl Pts',(59.4350695133288,-12.3300000212478,
-175.318261179968));
#171865=CARTESIAN_POINT('Ctrl Pts',(59.4312434964565,-12.3300000214808,
-175.334467250167));
#171866=CARTESIAN_POINT('Ctrl Pts',(59.4272543062711,-12.330000021774,-175.350650168439));
#171867=CARTESIAN_POINT('Ctrl Pts',(59.4106840236565,-12.3300000229918,
-175.417870711165));
#171868=CARTESIAN_POINT('Ctrl Pts',(59.3911649601375,-12.3300000250948,
-175.484771053152));
#171869=CARTESIAN_POINT('Ctrl Pts',(59.3688362082559,-12.3300000304207,
-175.550947464116));
#171870=CARTESIAN_POINT('Ctrl Pts',(59.3452983767326,-12.330000036035,-175.620707261724));
#171871=CARTESIAN_POINT('Ctrl Pts',(59.318757276387,-12.3300000404266,-175.689252183756));
#171872=CARTESIAN_POINT('Ctrl Pts',(59.2894219594714,-12.3300000414655,
-175.756217087947));
#171873=CARTESIAN_POINT('Ctrl Pts',(59.265578831198,-12.3300000423099,-175.810644752902));
#171874=CARTESIAN_POINT('Ctrl Pts',(59.2398885853161,-12.3300000411891,
-175.864029149378));
#171875=CARTESIAN_POINT('Ctrl Pts',(59.2124386122788,-12.330000039031,-175.916169632722));
#171876=CARTESIAN_POINT('Ctrl Pts',(59.1785809256147,-12.3300000363691,
-175.980481395257));
#171877=CARTESIAN_POINT('Ctrl Pts',(59.1417731864694,-12.3300000322739,
-176.043500821863));
#171878=CARTESIAN_POINT('Ctrl Pts',(59.1021371288072,-12.3300000288604,
-176.105011973128));
#171879=CARTESIAN_POINT('Ctrl Pts',(59.0666804433847,-12.3300000258069,
-176.16003716153));
#171880=CARTESIAN_POINT('Ctrl Pts',(59.0289595515133,-12.3300000233307,
-176.21385559589));
#171881=CARTESIAN_POINT('Ctrl Pts',(58.9890336736408,-12.3300000218957,
-176.26629097911));
#171882=CARTESIAN_POINT('Origin',(59.5,-12.83000002,-174.751778045594));
#171883=CARTESIAN_POINT('Ctrl Pts',(39.9232693735648,-12.33000002,-101.394976652855));
#171884=CARTESIAN_POINT('Ctrl Pts',(39.4816972464314,-12.33000002,-101.188984626754));
#171885=CARTESIAN_POINT('Ctrl Pts',(39.4702993039609,-11.842906113671,-101.183667521985));
#171886=CARTESIAN_POINT('Ctrl Pts',(46.1948314689912,-12.33000002,-87.9510241496856));
#171887=CARTESIAN_POINT('Ctrl Pts',(45.7637467547491,-12.3300000200387,
-87.7178689736084));
#171888=CARTESIAN_POINT('Ctrl Pts',(45.741803891981,-11.8408803347909,-87.7397145657271));
#171889=CARTESIAN_POINT('Ctrl Pts',(52.4655100689676,-12.33000002,-74.5066595330064));
#171890=CARTESIAN_POINT('Ctrl Pts',(52.0269437270063,-12.3300000197686,
-74.2868280745294));
#171891=CARTESIAN_POINT('Ctrl Pts',(52.0124594137882,-11.8397106642502,
-74.2953500811619));
#171892=CARTESIAN_POINT('Ctrl Pts',(58.7359481105893,-12.33000002,-61.0621827299711));
#171893=CARTESIAN_POINT('Ctrl Pts',(58.2906927660831,-12.33000002,-60.8545178210735));
#171894=CARTESIAN_POINT('Ctrl Pts',(58.2828791719688,-11.838774304476,-60.8508735991007));
#171895=CARTESIAN_POINT('',(58.2828791719688,-11.838774304476,-60.8508735991007));
#171896=CARTESIAN_POINT('Ctrl Pts',(58.2828791719688,-11.838774304476,-60.8508735991007));
#171897=CARTESIAN_POINT('Ctrl Pts',(55.3775064758257,-11.8392081628502,
-67.080315389494));
#171898=CARTESIAN_POINT('Ctrl Pts',(52.6531073433158,-11.8396682774539,
-72.921588901895));
#171899=CARTESIAN_POINT('Ctrl Pts',(50.1096592410629,-11.8401779861306,
-78.3746829039473));
#171900=CARTESIAN_POINT('Ctrl Pts',(47.223103444897,-11.8407564538154,-84.5633918792627));
#171901=CARTESIAN_POINT('Ctrl Pts',(44.5696120347148,-11.841398417424,-90.2521277977888));
#171902=CARTESIAN_POINT('Ctrl Pts',(42.149198203414,-11.8420910505548,-95.4408968196894));
#171903=CARTESIAN_POINT('Ctrl Pts',(41.2220298729399,-11.8423563719205,
-97.4285165601807));
#171904=CARTESIAN_POINT('Ctrl Pts',(40.329062911927,-11.8426287216759,-99.3427731426528));
#171905=CARTESIAN_POINT('Ctrl Pts',(39.4702993039609,-11.842906113671,-101.183667521985));
#171906=CARTESIAN_POINT('',(58.7359481105893,-12.33000002,-61.0621827299711));
#171907=CARTESIAN_POINT('Origin',(58.7359481105893,-11.83000002,-61.0621827299711));
#171908=CARTESIAN_POINT('Ctrl Pts',(39.9232693735648,-12.33000002,-101.394976652855));
#171909=CARTESIAN_POINT('Ctrl Pts',(46.1948314689912,-12.33000002,-87.9510241496856));
#171910=CARTESIAN_POINT('Ctrl Pts',(52.4655100689676,-12.33000002,-74.5066595330064));
#171911=CARTESIAN_POINT('Ctrl Pts',(58.7359481105893,-12.33000002,-61.0621827299711));
#171912=CARTESIAN_POINT('Origin',(59.5,-12.83000002,-55.24995));
#171913=CARTESIAN_POINT('',(59.5,-12.33000002,-57.909894348981));
#171914=CARTESIAN_POINT('',(60.,-12.83000002,-57.909894348981));
#171915=CARTESIAN_POINT('Origin',(59.5,-12.83000002,-57.909894348981));
#171916=CARTESIAN_POINT('',(60.,-12.83000002,-57.911664394164));
#171917=CARTESIAN_POINT('',(59.5,-12.33000002,-174.749818876635));
#171918=CARTESIAN_POINT('Origin',(60.,-2.55003103885676E-14,0.));
#171919=CARTESIAN_POINT('',(60.,-13.33000002,-57.9104088126279));
#171920=CARTESIAN_POINT('Origin',(60.,-12.9674754042923,-167.271246742336));
#171921=CARTESIAN_POINT('',(60.,-13.33000002,-174.748117418411));
#171922=CARTESIAN_POINT('Origin',(59.5,-13.33000002,-55.24995));
#171923=CARTESIAN_POINT('',(59.5,-13.83000002,-57.9104088126279));
#171924=CARTESIAN_POINT('Origin',(59.5,-13.33000002,-57.9104088126279));
#171925=CARTESIAN_POINT('',(59.5,-13.83000002,-174.751208632418));
#171926=CARTESIAN_POINT('',(59.5,-13.83000002,-57.9132014677655));
#171927=CARTESIAN_POINT('Origin',(59.5,-13.33000002,-174.751208632418));
#171928=CARTESIAN_POINT('Ctrl Pts',(59.5,-13.83000002,-174.751208632418));
#171929=CARTESIAN_POINT('Ctrl Pts',(60.,-13.83000002,-174.751208632417));
#171930=CARTESIAN_POINT('Ctrl Pts',(60.,-13.33000002,-174.751208632418));
#171931=CARTESIAN_POINT('Ctrl Pts',(59.499999994458,-13.83000002,-174.955005950799));
#171932=CARTESIAN_POINT('Ctrl Pts',(59.9998505155736,-13.83000002,-174.995728395116));
#171933=CARTESIAN_POINT('Ctrl Pts',(60.,-13.3301495200469,-174.995764866376));
#171934=CARTESIAN_POINT('Ctrl Pts',(59.4754418884424,-13.83000002,-175.154666905584));
#171935=CARTESIAN_POINT('Ctrl Pts',(59.9702437452671,-13.8300000199993,
-175.235287718005));
#171936=CARTESIAN_POINT('Ctrl Pts',(59.9705302647519,-13.3302950638363,
-175.235357479373));
#171937=CARTESIAN_POINT('Ctrl Pts',(59.3788903697392,-13.83000002,-175.545864512034));
#171938=CARTESIAN_POINT('Ctrl Pts',(59.8541239849711,-13.8300000200007,
-175.704587709371));
#171939=CARTESIAN_POINT('Ctrl Pts',(59.8546684450659,-13.3305785951146,
-175.704793574078));
#171940=CARTESIAN_POINT('Ctrl Pts',(59.3057599866248,-13.83000002,-175.738059080183));
#171941=CARTESIAN_POINT('Ctrl Pts',(59.7662611489698,-13.8300000199988,
-175.935125812779));
#171942=CARTESIAN_POINT('Ctrl Pts',(59.7669119843163,-13.3307170303008,
-175.935426552567));
#171943=CARTESIAN_POINT('Ctrl Pts',(59.1185058620249,-13.83000002,-176.093723731171));
#171944=CARTESIAN_POINT('Ctrl Pts',(59.5413945721013,-13.8300000200012,
-176.361684206804));
#171945=CARTESIAN_POINT('Ctrl Pts',(59.5422070340633,-13.3309719059141,
-176.362223209373));
#171946=CARTESIAN_POINT('Ctrl Pts',(59.0022803225031,-13.83000002,-176.261780328219));
#171947=CARTESIAN_POINT('Ctrl Pts',(59.4018755020326,-13.8300000199995,
-176.563219594419));
#171948=CARTESIAN_POINT('Ctrl Pts',(59.4027363887007,-13.331091646732,-176.563890694693));
#171949=CARTESIAN_POINT('Ctrl Pts',(58.7333577194631,-13.83000002,-176.564062061699));
#171950=CARTESIAN_POINT('Ctrl Pts',(59.0791375439908,-13.8300000200005,
-176.925670411677));
#171951=CARTESIAN_POINT('Ctrl Pts',(59.0800292616587,-13.3313061338651,
-176.92662799811));
#171952=CARTESIAN_POINT('Ctrl Pts',(58.5826842101506,-13.83000002,-176.697016027753));
#171953=CARTESIAN_POINT('Ctrl Pts',(58.8983479608961,-13.830000020003,-177.085078467603));
#171954=CARTESIAN_POINT('Ctrl Pts',(58.8992210551541,-13.3313999972609,
-177.086172425279));
#171955=CARTESIAN_POINT('Ctrl Pts',(58.4157868605055,-13.83000002,-176.811694866106));
#171956=CARTESIAN_POINT('Ctrl Pts',(58.698108161756,-13.83000002,-177.222569964948));
#171957=CARTESIAN_POINT('Ctrl Pts',(58.6989442326066,-13.3314807280565,
-177.223786737086));
#171958=CARTESIAN_POINT('Ctrl Pts',(58.9842656455839,-13.8300000182384,
-176.2719717603));
#171959=CARTESIAN_POINT('Ctrl Pts',(59.0284765648177,-13.8300000166394,
-176.214285352615));
#171960=CARTESIAN_POINT('Ctrl Pts',(59.0700022374974,-13.8300000137057,
-176.154919321395));
#171961=CARTESIAN_POINT('Ctrl Pts',(59.108769049557,-13.8300000102313,-176.094105263609));
#171962=CARTESIAN_POINT('Ctrl Pts',(59.1458171677547,-13.830000006911,-176.0359873457));
#171963=CARTESIAN_POINT('Ctrl Pts',(59.18034578997,-13.8300000031738,-175.976545944298));
#171964=CARTESIAN_POINT('Ctrl Pts',(59.2122555343191,-13.8300000007997,
-175.915955958697));
#171965=CARTESIAN_POINT('Ctrl Pts',(59.2455714173137,-13.829999998321,-175.852696007478));
#171966=CARTESIAN_POINT('Ctrl Pts',(59.2762989800144,-13.8299999975166,
-175.787603392926));
#171967=CARTESIAN_POINT('Ctrl Pts',(59.3042804787193,-13.8299999996639,
-175.721026919923));
#171968=CARTESIAN_POINT('Ctrl Pts',(59.3272704921691,-13.8300000014281,
-175.666326704402));
#171969=CARTESIAN_POINT('Ctrl Pts',(59.3484061154264,-13.8300000052622,
-175.610623961591));
#171970=CARTESIAN_POINT('Ctrl Pts',(59.3675737697888,-13.8300000097259,
-175.554108016098));
#171971=CARTESIAN_POINT('Ctrl Pts',(59.3904098382371,-13.8300000150439,
-175.486775729355));
#171972=CARTESIAN_POINT('Ctrl Pts',(59.4103356014117,-13.830000017107,-175.418690311177));
#171973=CARTESIAN_POINT('Ctrl Pts',(59.4272061992403,-13.8300000182966,
-175.350275598526));
#171974=CARTESIAN_POINT('Ctrl Pts',(59.449240943989,-13.8300000198503,-175.260918911488));
#171975=CARTESIAN_POINT('Ctrl Pts',(59.4663032629516,-13.8300000198819,
-175.170862100582));
#171976=CARTESIAN_POINT('Ctrl Pts',(59.4783606526567,-13.8300000199558,
-175.079983307972));
#171977=CARTESIAN_POINT('Ctrl Pts',(59.4903258960553,-13.8300000200293,
-174.989799039243));
#171978=CARTESIAN_POINT('Ctrl Pts',(59.4973624498087,-13.83000002,-174.898805302283));
#171979=CARTESIAN_POINT('Ctrl Pts',(59.4993876311079,-13.83000002,-174.806876041458));
#171980=CARTESIAN_POINT('Ctrl Pts',(59.4997955668077,-13.83000002,-174.788358574718));
#171981=CARTESIAN_POINT('Ctrl Pts',(59.5,-13.83000002,-174.769803126625));
#171982=CARTESIAN_POINT('Ctrl Pts',(59.5,-13.83000002,-174.751208632418));
#171983=CARTESIAN_POINT('Origin',(58.9842656455947,-14.33000002,-179.64995));
#171984=CARTESIAN_POINT('',(58.9842656455947,-13.83000002,-171.871644662643));
#171985=CARTESIAN_POINT('',(58.9842656455947,-13.83000002,-176.75597498356));
#171986=CARTESIAN_POINT('Origin',(58.9842656455946,-14.33000002,-171.871644662643));
#171987=CARTESIAN_POINT('',(58.4843989875811,-14.3184534098307,-179.64995));
#171988=CARTESIAN_POINT('Ctrl Pts',(58.8436897472855,-13.83000002,-171.237717270032));
#171989=CARTESIAN_POINT('Ctrl Pts',(58.3999663918639,-13.83000002,-171.444684327491));
#171990=CARTESIAN_POINT('Ctrl Pts',(58.3906572805143,-14.3195102506022,
-171.449026400902));
#171991=CARTESIAN_POINT('Ctrl Pts',(58.9361841983689,-13.83000002,-171.436019148456));
#171992=CARTESIAN_POINT('Ctrl Pts',(58.4628431558437,-13.8300000200007,
-171.577873523862));
#171993=CARTESIAN_POINT('Ctrl Pts',(58.452336355597,-14.3188132239679,-171.581227559315));
#171994=CARTESIAN_POINT('Ctrl Pts',(58.9842656416468,-13.83000002,-171.650610345097));
#171995=CARTESIAN_POINT('Ctrl Pts',(58.4956819559116,-13.83000002,-171.722618633075));
#171996=CARTESIAN_POINT('Ctrl Pts',(58.484398987579,-14.3184534099214,-171.72428852145));
#171997=CARTESIAN_POINT('Ctrl Pts',(58.9842656455947,-13.83000002,-171.871644662643));
#171998=CARTESIAN_POINT('Ctrl Pts',(58.4956819583251,-13.83000002,-171.871644662643));
#171999=CARTESIAN_POINT('Ctrl Pts',(58.4843989875811,-14.3184534098307,
-171.871644662643));
#172000=CARTESIAN_POINT('',(58.8436897472855,-13.83000002,-171.237717270032));
#172001=CARTESIAN_POINT('Origin',(56.7574781748151,-13.83000002,-172.032172120179));
#172002=CARTESIAN_POINT('Origin',(58.8436897472855,-14.33000002,-171.237717270032));
#172003=CARTESIAN_POINT('Ctrl Pts',(39.923987884714,-13.83000002,-130.68030635931));
#172004=CARTESIAN_POINT('Ctrl Pts',(39.4846775617168,-13.83000002,-130.885279386667));
#172005=CARTESIAN_POINT('Ctrl Pts',(39.4710976496822,-14.3145440753934,
-130.89161549018));
#172006=CARTESIAN_POINT('Ctrl Pts',(46.2315241188232,-13.83000002,-144.198991310165));
#172007=CARTESIAN_POINT('Ctrl Pts',(45.8048635488014,-13.83000002,-144.43668735532));
#172008=CARTESIAN_POINT('Ctrl Pts',(45.7785509549148,-14.3169830983588,
-144.410301102566));
#172009=CARTESIAN_POINT('Ctrl Pts',(52.5377799111353,-13.83000002,-157.718273616974));
#172010=CARTESIAN_POINT('Ctrl Pts',(52.1020957034304,-13.8300000200905,
-157.939875120093));
#172011=CARTESIAN_POINT('Ctrl Pts',(52.0847736772191,-14.3183867301138,
-157.929583215096));
#172012=CARTESIAN_POINT('Ctrl Pts',(58.8436897472855,-13.83000002,-171.237717270032));
#172013=CARTESIAN_POINT('Ctrl Pts',(58.3999663918639,-13.83000002,-171.444684327491));
#172014=CARTESIAN_POINT('Ctrl Pts',(58.3906572805143,-14.3195102506022,
-171.449026400902));
#172015=CARTESIAN_POINT('',(39.923987884714,-13.83000002,-130.68030635931));
#172016=CARTESIAN_POINT('Ctrl Pts',(39.923987884714,-13.83000002,-130.68030635931));
#172017=CARTESIAN_POINT('Ctrl Pts',(46.2315241188232,-13.83000002,-144.198991310165));
#172018=CARTESIAN_POINT('Ctrl Pts',(52.5377799111353,-13.83000002,-157.718273616974));
#172019=CARTESIAN_POINT('Ctrl Pts',(58.8436897472855,-13.83000002,-171.237717270032));
#172020=CARTESIAN_POINT('Origin',(39.923987884714,-14.33000002,-130.68030635931));
#172021=CARTESIAN_POINT('Ctrl Pts',(39.4710976496822,-14.3145440753934,
-130.89161549018));
#172022=CARTESIAN_POINT('Ctrl Pts',(39.4846775617168,-13.83000002,-130.885279386667));
#172023=CARTESIAN_POINT('Ctrl Pts',(39.923987884714,-13.83000002,-130.68030635931));
#172024=CARTESIAN_POINT('Ctrl Pts',(39.1611309974652,-14.3198673792142,
-130.227665983087));
#172025=CARTESIAN_POINT('Ctrl Pts',(39.1694803296317,-13.83000002,-130.222011573448));
#172026=CARTESIAN_POINT('Ctrl Pts',(39.6450175280278,-13.83000002,-130.082400567686));
#172027=CARTESIAN_POINT('Ctrl Pts',(39.,-14.325106270286,-129.50903420183));
#172028=CARTESIAN_POINT('Ctrl Pts',(39.0048700588287,-13.83000002,-129.505450476954));
#172029=CARTESIAN_POINT('Ctrl Pts',(39.5000000016417,-13.83000002,-129.435305216167));
#172030=CARTESIAN_POINT('Ctrl Pts',(39.,-14.33000002,-128.768820397718));
#172031=CARTESIAN_POINT('Ctrl Pts',(38.9999999999999,-13.83000002,-128.768820397718));
#172032=CARTESIAN_POINT('Ctrl Pts',(39.5,-13.83000002,-128.768820397718));
#172033=CARTESIAN_POINT('',(39.5,-13.83000002,-128.768820397718));
#172034=CARTESIAN_POINT('Origin',(46.1927888984987,-13.83000002,-128.288325652416));
#172035=CARTESIAN_POINT('Origin',(39.5,-14.33000002,-128.768820397718));
#172036=CARTESIAN_POINT('Origin',(39.5,-14.33000002,-55.24995));
#172037=CARTESIAN_POINT('',(39.5,-13.83000002,-103.289822573788));
#172038=CARTESIAN_POINT('',(39.5,-13.83000002,-55.24995));
#172039=CARTESIAN_POINT('Origin',(39.5,-14.33000002,-103.289822573788));
#172040=CARTESIAN_POINT('Ctrl Pts',(39.,-14.33000002,-103.289822573788));
#172041=CARTESIAN_POINT('Ctrl Pts',(39.,-13.83000002,-103.289822573788));
#172042=CARTESIAN_POINT('Ctrl Pts',(39.5,-13.83000002,-103.289822573788));
#172043=CARTESIAN_POINT('Ctrl Pts',(39.,-14.3251554673834,-102.557050168938));
#172044=CARTESIAN_POINT('Ctrl Pts',(39.0048213824044,-13.83000002,-102.560555788171));
#172045=CARTESIAN_POINT('Ctrl Pts',(39.5000000055327,-13.83000002,-102.630037977128));
#172046=CARTESIAN_POINT('Ctrl Pts',(39.1579830770898,-14.319921441001,-101.837719843386));
#172047=CARTESIAN_POINT('Ctrl Pts',(39.1662598483009,-13.830000019993,-101.843408229318));
#172048=CARTESIAN_POINT('Ctrl Pts',(39.6421844024665,-13.83000002,-101.982314517002));
#172049=CARTESIAN_POINT('Ctrl Pts',(39.4710976496822,-14.3145440753935,
-101.167027481325));
#172050=CARTESIAN_POINT('Ctrl Pts',(39.4846775617168,-13.83000002,-101.173363584839));
#172051=CARTESIAN_POINT('Ctrl Pts',(39.923987884714,-13.83000002,-101.378336612196));
#172052=CARTESIAN_POINT('',(39.923987884714,-13.83000002,-101.378336612196));
#172053=CARTESIAN_POINT('Origin',(46.1924380477474,-13.83000002,-103.773062785038));
#172054=CARTESIAN_POINT('',(39.4710972477948,-14.3145440616689,-101.167027293814));
#172055=CARTESIAN_POINT('Origin',(39.923987884714,-14.33000002,-101.378336612196));
#172056=CARTESIAN_POINT('Origin',(46.4032459150591,-14.3112053351235,-103.821907513578));
#172057=CARTESIAN_POINT('Ctrl Pts',(58.7311595360587,-13.83000002,-61.0621827299711));
#172058=CARTESIAN_POINT('Ctrl Pts',(58.2874540965012,-13.83000002,-60.8552238163692));
#172059=CARTESIAN_POINT('Ctrl Pts',(58.2781275348581,-14.3194901627709,
-60.8508735991007));
#172060=CARTESIAN_POINT('Ctrl Pts',(52.4627544636864,-13.83000002,-74.5012048985427));
#172061=CARTESIAN_POINT('Ctrl Pts',(52.0270272593534,-13.8300000198715,
-74.2797364934824));
#172062=CARTESIAN_POINT('Ctrl Pts',(52.0097486856907,-14.3183690440453,
-74.2898953083048));
#172063=CARTESIAN_POINT('Ctrl Pts',(46.194004389791,-13.83000002,-87.9400661652057));
#172064=CARTESIAN_POINT('Ctrl Pts',(45.7671827316852,-13.8300000198453,
-87.7027488289555));
#172065=CARTESIAN_POINT('Ctrl Pts',(45.7410317152176,-14.3169685900793,
-87.7287563851229));
#172066=CARTESIAN_POINT('Ctrl Pts',(39.923987884714,-13.83000002,-101.378336612196));
#172067=CARTESIAN_POINT('Ctrl Pts',(39.4846775617168,-13.83000002,-101.173363584839));
#172068=CARTESIAN_POINT('Ctrl Pts',(39.4710976496822,-14.3145440753934,
-101.167027481326));
#172069=CARTESIAN_POINT('',(58.7311595360587,-13.83000002,-61.0621827299711));
#172070=CARTESIAN_POINT('Ctrl Pts',(58.7311595360587,-13.83000002,-61.0621827299711));
#172071=CARTESIAN_POINT('Ctrl Pts',(52.4627544636864,-13.83000002,-74.5012048985427));
#172072=CARTESIAN_POINT('Ctrl Pts',(46.194004389791,-13.83000002,-87.9400661652057));
#172073=CARTESIAN_POINT('Ctrl Pts',(39.923987884714,-13.83000002,-101.378336612196));
#172074=CARTESIAN_POINT('',(58.2781275348581,-14.3194901627709,-60.8508735991007));
#172075=CARTESIAN_POINT('Origin',(58.7311595360587,-14.33000002,-61.0621827299711));
#172076=CARTESIAN_POINT('Ctrl Pts',(39.4710976496823,-14.3145440753934,
-101.167027481325));
#172077=CARTESIAN_POINT('Ctrl Pts',(41.5746782641129,-14.3153575069286,
-96.6584495163958));
#172078=CARTESIAN_POINT('Ctrl Pts',(43.8638536657975,-14.3161254468934,
-91.7517222040427));
#172079=CARTESIAN_POINT('Ctrl Pts',(46.3385980299419,-14.3168265117389,
-86.4468333272163));
#172080=CARTESIAN_POINT('Ctrl Pts',(46.751055423966,-14.3169433558798,-85.5626851810786));
#172081=CARTESIAN_POINT('Ctrl Pts',(47.1686676754888,-14.3170546060321,
-84.6674770644942));
#172082=CARTESIAN_POINT('Ctrl Pts',(47.5914346875375,-14.3171629162029,
-83.7612089442138));
#172083=CARTESIAN_POINT('Ctrl Pts',(47.8028181935619,-14.3172170712883,
-83.3080748840737));
#172084=CARTESIAN_POINT('Ctrl Pts',(48.0154903745181,-14.3172711248367,
-82.8521758187235));
#172085=CARTESIAN_POINT('Ctrl Pts',(48.2294512239489,-14.3173253426588,
-82.3935117469702));
#172086=CARTESIAN_POINT('Ctrl Pts',(48.3364316486644,-14.3173524515698,
-82.1641797110936));
#172087=CARTESIAN_POINT('Ctrl Pts',(48.4437342405363,-14.3173796015504,
-81.9341564236338));
#172088=CARTESIAN_POINT('Ctrl Pts',(48.5513589988902,-14.3174068298701,
-81.703441884523));
#172089=CARTESIAN_POINT('Ctrl Pts',(48.6556204835456,-14.3174332073049,
-81.4799371747593));
#172090=CARTESIAN_POINT('Ctrl Pts',(48.7601843138941,-14.317459658259,-81.2557837415226));
#172091=CARTESIAN_POINT('Ctrl Pts',(48.8650504894187,-14.3174862185691,
-81.0309815848041));
#172092=CARTESIAN_POINT('Ctrl Pts',(48.8684332692744,-14.3174870753533,
-81.0237299023293));
#172093=CARTESIAN_POINT('Ctrl Pts',(48.8724050841776,-14.3174880813788,
-81.0152155015906));
#172094=CARTESIAN_POINT('Ctrl Pts',(48.8751997728309,-14.317488789274,-81.0092245122283));
#172095=CARTESIAN_POINT('Ctrl Pts',(51.1015771319527,-14.3180527310343,
-76.2365271818777));
#172096=CARTESIAN_POINT('Ctrl Pts',(53.4929070387879,-14.3185834838436,
-71.1099546195311));
#172097=CARTESIAN_POINT('Ctrl Pts',(56.0492020811948,-14.3190764132052,
-65.6295126793767));
#172098=CARTESIAN_POINT('Ctrl Pts',(56.7787408124601,-14.3192170898701,
-64.065454308388));
#172099=CARTESIAN_POINT('Ctrl Pts',(57.521715671378,-14.3193548761951,-62.4725744724866));
#172100=CARTESIAN_POINT('Ctrl Pts',(58.2781275348581,-14.3194901627709,
-60.8508735991007));
#172101=CARTESIAN_POINT('Ctrl Pts',(39.,-14.2911437666779,-103.292364908221));
#172102=CARTESIAN_POINT('Ctrl Pts',(39.,-14.2196500163134,-102.183653245897));
#172103=CARTESIAN_POINT('Ctrl Pts',(39.4705101402401,-14.154883972851,-101.179273599517));
#172104=CARTESIAN_POINT('Ctrl Pts',(39.,-15.3821188871317,-103.222014874282));
#172105=CARTESIAN_POINT('Ctrl Pts',(38.9999999999962,-15.2519052464411,
-102.112898232639));
#172106=CARTESIAN_POINT('Ctrl Pts',(39.473885603051,-15.1336440339978,-101.108924169704));
#172107=CARTESIAN_POINT('Ctrl Pts',(39.,-16.4753328054123,-103.064008234267));
#172108=CARTESIAN_POINT('Ctrl Pts',(39.,-16.2866475513133,-101.953874758818));
#172109=CARTESIAN_POINT('Ctrl Pts',(39.4814699289176,-16.1148163368312,
-100.950916925651));
#172110=CARTESIAN_POINT('Ctrl Pts',(39.,-18.6473032869024,-102.580339184276));
#172111=CARTESIAN_POINT('Ctrl Pts',(39.,-18.3422738396393,-101.467519549647));
#172112=CARTESIAN_POINT('Ctrl Pts',(39.5044475737172,-18.0667048767241,
-100.467247875485));
#172113=CARTESIAN_POINT('Ctrl Pts',(39.,-19.6982839688054,-102.261854767811));
#172114=CARTESIAN_POINT('Ctrl Pts',(39.,-19.3376015901503,-101.147059506123));
#172115=CARTESIAN_POINT('Ctrl Pts',(39.5194922305763,-19.012479411179,-100.148762913439));
#172116=CARTESIAN_POINT('Ctrl Pts',(39.,-20.7209336217775,-101.88126637264));
#172117=CARTESIAN_POINT('Ctrl Pts',(39.,-20.3054076594241,-100.764738681203));
#172118=CARTESIAN_POINT('Ctrl Pts',(39.5372194307944,-19.9345274212658,
-99.7681750639369));
#172119=CARTESIAN_POINT('',(39.5365899583801,-19.9017174907778,-99.7816873754343));
#172120=CARTESIAN_POINT('Ctrl Pts',(39.5365899564018,-19.9017175093585,
-99.7816874458032));
#172121=CARTESIAN_POINT('Ctrl Pts',(39.530122557743,-19.5639073116448,-99.9204980182519));
#172122=CARTESIAN_POINT('Ctrl Pts',(39.5240916280606,-19.2268288969008,
-100.049342899962));
#172123=CARTESIAN_POINT('Ctrl Pts',(39.5185098148994,-18.8902357403587,
-100.168182990067));
#172124=CARTESIAN_POINT('Ctrl Pts',(39.5124505611178,-18.5248520742067,
-100.297188072209));
#172125=CARTESIAN_POINT('Ctrl Pts',(39.5069205643145,-18.1600421489813,
-100.414403319327));
#172126=CARTESIAN_POINT('Ctrl Pts',(39.5019314566728,-17.7955093298411,
-100.519838481297));
#172127=CARTESIAN_POINT('Ctrl Pts',(39.4994317811217,-17.6128686972832,
-100.572664300168));
#172128=CARTESIAN_POINT('Ctrl Pts',(39.4970678142959,-17.4302977870856,
-100.622533895174));
#172129=CARTESIAN_POINT('Ctrl Pts',(39.4948406453418,-17.2477595012952,
-100.669453192989));
#172130=CARTESIAN_POINT('Ctrl Pts',(39.4945248369439,-17.2218759133065,
-100.676106261785));
#172131=CARTESIAN_POINT('Ctrl Pts',(39.4942244698344,-17.1970497893428,
-100.682432750568));
#172132=CARTESIAN_POINT('Ctrl Pts',(39.4939047480909,-17.1703984768855,
-100.689162165644));
#172133=CARTESIAN_POINT('Ctrl Pts',(39.4938728326357,-17.1677380736302,
-100.689833913341));
#172134=CARTESIAN_POINT('Ctrl Pts',(39.4938407261658,-17.1650594675226,
-100.690509636197));
#172135=CARTESIAN_POINT('Ctrl Pts',(39.4938083953304,-17.1623597805275,
-100.69119003266));
#172136=CARTESIAN_POINT('Ctrl Pts',(39.4935227058336,-17.1385041575733,
-100.697202315387));
#172137=CARTESIAN_POINT('Ctrl Pts',(39.493239218094,-17.1146379939548,-100.703167010794));
#172138=CARTESIAN_POINT('Ctrl Pts',(39.4929579387798,-17.0907609744762,
-100.70908405176));
#172139=CARTESIAN_POINT('Ctrl Pts',(39.4899905322944,-16.8388660825674,
-100.771506934803));
#172140=CARTESIAN_POINT('Ctrl Pts',(39.4872919536633,-16.5874251012425,
-100.828152222157));
#172141=CARTESIAN_POINT('Ctrl Pts',(39.4848610087856,-16.3362741421625,
-100.879107025452));
#172142=CARTESIAN_POINT('Ctrl Pts',(39.4824374819515,-16.0858895718154,
-100.929906339843));
#172143=CARTESIAN_POINT('Ctrl Pts',(39.4802799507959,-15.8357930472734,
-100.975049887297));
#172144=CARTESIAN_POINT('Ctrl Pts',(39.47838954742,-15.5858173398232,-101.014572640927));
#172145=CARTESIAN_POINT('Ctrl Pts',(39.4765129834559,-15.3376716739312,
-101.053806053315));
#172146=CARTESIAN_POINT('Ctrl Pts',(39.4748996443138,-15.0896448639291,
-101.087500689895));
#172147=CARTESIAN_POINT('Ctrl Pts',(39.4735530184565,-14.8415715919254,
-101.115639683381));
#172148=CARTESIAN_POINT('Ctrl Pts',(39.4725996226103,-14.6659385266556,
-101.135561771883));
#172149=CARTESIAN_POINT('Ctrl Pts',(39.4717799652781,-14.490282131345,-101.152698050753));
#172150=CARTESIAN_POINT('Ctrl Pts',(39.4710960421325,-14.3145440204951,
-101.16702673128));
#172151=CARTESIAN_POINT('Ctrl Pts',(39.5365899564018,-19.9017175093585,
-99.7816874458032));
#172152=CARTESIAN_POINT('Ctrl Pts',(39.5215966413189,-19.9028363193258,
-99.8129429095326));
#172153=CARTESIAN_POINT('Ctrl Pts',(39.5051517179811,-19.9040793375384,
-99.8479870711594));
#172154=CARTESIAN_POINT('Ctrl Pts',(39.487486986643,-19.9054569612971,-99.8869339480742));
#172155=CARTESIAN_POINT('Ctrl Pts',(39.4698222553048,-19.9068345850559,
-99.9258808249889));
#172156=CARTESIAN_POINT('Ctrl Pts',(39.4509374704379,-19.9083470628612,
-99.9687309905404));
#172157=CARTESIAN_POINT('Ctrl Pts',(39.4311216183148,-19.9099998322464,
-100.015606617578));
#172158=CARTESIAN_POINT('Ctrl Pts',(39.4149965614371,-19.9113447655945,
-100.053751439585));
#172159=CARTESIAN_POINT('Ctrl Pts',(39.3983441841591,-19.9127752427056,
-100.094348136095));
#172160=CARTESIAN_POINT('Ctrl Pts',(39.3812363475712,-19.9142986868476,
-100.137720804013));
#172161=CARTESIAN_POINT('Ctrl Pts',(39.3649091779095,-19.9157526129972,
-100.179114284955));
#172162=CARTESIAN_POINT('Ctrl Pts',(39.3481669883162,-19.9172913357008,
-100.22303642595));
#172163=CARTESIAN_POINT('Ctrl Pts',(39.3311188505349,-19.9189170716437,
-100.269774993623));
#172164=CARTESIAN_POINT('Ctrl Pts',(39.3221264132096,-19.9197746039303,
-100.294428339687));
#172165=CARTESIAN_POINT('Ctrl Pts',(39.313049662529,-19.9206562638823,-100.319865377738));
#172166=CARTESIAN_POINT('Ctrl Pts',(39.3039104841802,-19.9215616723638,
-100.346128647387));
#172167=CARTESIAN_POINT('Ctrl Pts',(39.2834462149981,-19.9235890453047,
-100.404936846459));
#172168=CARTESIAN_POINT('Ctrl Pts',(39.2651753202424,-19.9255089595866,
-100.460671945153));
#172169=CARTESIAN_POINT('Ctrl Pts',(39.2487802898612,-19.9273067637394,
-100.513176264637));
#172170=CARTESIAN_POINT('Ctrl Pts',(39.232189706142,-19.9291260113782,-100.566306834558));
#172171=CARTESIAN_POINT('Ctrl Pts',(39.2175195190471,-19.9308204611124,
-100.616129564333));
#172172=CARTESIAN_POINT('Ctrl Pts',(39.2044721454028,-19.9323862009587,
-100.662523063451));
#172173=CARTESIAN_POINT('Ctrl Pts',(39.1912503422537,-19.933972873081,-100.709536794295));
#172174=CARTESIAN_POINT('Ctrl Pts',(39.179694640591,-19.9354276023642,-100.753029464758));
#172175=CARTESIAN_POINT('Ctrl Pts',(39.1695341254265,-19.9367542033861,
-100.792910420823));
#172176=CARTESIAN_POINT('Ctrl Pts',(39.167223353613,-19.9370559077977,-100.801980412617));
#172177=CARTESIAN_POINT('Ctrl Pts',(39.1649849144337,-19.9373510088919,
-100.810863723644));
#172178=CARTESIAN_POINT('Ctrl Pts',(39.1628159253519,-19.9376395889075,
-100.819559501765));
#172179=CARTESIAN_POINT('Ctrl Pts',(39.1577463085425,-19.9383140921173,
-100.839884298835));
#172180=CARTESIAN_POINT('Ctrl Pts',(39.1530558607523,-19.9389529548387,
-100.859184461679));
#172181=CARTESIAN_POINT('Ctrl Pts',(39.1487102691849,-19.9395574210345,
-100.877450576426));
#172182=CARTESIAN_POINT('Ctrl Pts',(39.1465374734011,-19.9398596541323,
-100.886583633799));
#172183=CARTESIAN_POINT('Ctrl Pts',(39.1444509506023,-19.9401532929735,
-100.895458192899));
#172184=CARTESIAN_POINT('Ctrl Pts',(39.1424467411147,-19.9404385093095,
-100.904073269843));
#172185=CARTESIAN_POINT('Ctrl Pts',(39.1414446363709,-19.9405811174774,
-100.908380808314));
#172186=CARTESIAN_POINT('Ctrl Pts',(39.1404631136491,-19.9407216203324,
-100.91262347713));
#172187=CARTESIAN_POINT('Ctrl Pts',(39.1395016999041,-19.9408600401499,
-100.916801159935));
#172188=CARTESIAN_POINT('Ctrl Pts',(39.1390209930316,-19.9409292500586,
-100.918890001337));
#172189=CARTESIAN_POINT('Ctrl Pts',(39.1385453136342,-19.9409979392265,
-100.920962596289));
#172190=CARTESIAN_POINT('Ctrl Pts',(39.1380746038964,-19.9410661104793,
-100.923018930895));
#172191=CARTESIAN_POINT('Ctrl Pts',(39.1376038941586,-19.941134281732,-100.925075265502));
#172192=CARTESIAN_POINT('Ctrl Pts',(39.1374930189679,-19.9411502345416,
-100.925556891227));
#172193=CARTESIAN_POINT('Ctrl Pts',(39.1366773267527,-19.9412690733654,
-100.929139140079));
#172194=CARTESIAN_POINT('Ctrl Pts',(39.1161408417601,-19.9442610495997,
-101.019328550293));
#172195=CARTESIAN_POINT('Ctrl Pts',(39.0984087631728,-19.947194301293,-101.107745690636));
#172196=CARTESIAN_POINT('Ctrl Pts',(39.0831681755561,-19.9500376502056,
-101.194177581913));
#172197=CARTESIAN_POINT('Ctrl Pts',(39.0674129017333,-19.9529770211681,
-101.28352834373));
#172198=CARTESIAN_POINT('Ctrl Pts',(39.054319620319,-19.9558204102339,-101.3707575086));
#172199=CARTESIAN_POINT('Ctrl Pts',(39.043541575639,-19.9585528417086,-101.455682826679));
#172200=CARTESIAN_POINT('Ctrl Pts',(39.0325596286468,-19.9613369661491,
-101.542214787635));
#172201=CARTESIAN_POINT('Ctrl Pts',(39.0239807695704,-19.9640060729754,
-101.62635515219));
#172202=CARTESIAN_POINT('Ctrl Pts',(39.017446398052,-19.9665620140938,-101.707963194666));
#172203=CARTESIAN_POINT('Ctrl Pts',(39.0106980132704,-19.9692016672109,
-101.792244057844));
#172204=CARTESIAN_POINT('Ctrl Pts',(39.0061296681829,-19.9717207963296,
-101.873824248984));
#172205=CARTESIAN_POINT('Ctrl Pts',(39.0033639495716,-19.9741374443006,
-101.952600153975));
#172206=CARTESIAN_POINT('Ctrl Pts',(39.0010525559368,-19.9761571091772,
-102.018435530223));
#172207=CARTESIAN_POINT('Ctrl Pts',(39.000000428941,-19.9781055542109,-102.082313347502));
#172208=CARTESIAN_POINT('Ctrl Pts',(39.000000000131,-19.9800000199999,-102.144196959718));
#172209=CARTESIAN_POINT('Ctrl Pts',(39.6286602916726,-19.8949860872698,
-99.5986214172193));
#172210=CARTESIAN_POINT('Ctrl Pts',(39.5391188861498,-20.48000002,-99.5520413536212));
#172211=CARTESIAN_POINT('Ctrl Pts',(40.0657759443213,-20.48000002,-99.8260192271647));
#172212=CARTESIAN_POINT('Ctrl Pts',(39.4043265400278,-19.9104340007096,
-100.024930299828));
#172213=CARTESIAN_POINT('Ctrl Pts',(39.333589588996,-20.48000002,-99.9880739006574));
#172214=CARTESIAN_POINT('Ctrl Pts',(39.8638772323513,-20.48000002,-100.214892381557));
#172215=CARTESIAN_POINT('Ctrl Pts',(39.2415142628292,-19.9258615536628,
-100.468806409009));
#172216=CARTESIAN_POINT('Ctrl Pts',(39.1854308339039,-20.48000002,-100.444304985299));
#172217=CARTESIAN_POINT('Ctrl Pts',(39.7173505054454,-20.48000002,-100.61942636691));
#172218=CARTESIAN_POINT('Ctrl Pts',(39.0318769517979,-19.9564049059902,
-101.38937941419));
#172219=CARTESIAN_POINT('Ctrl Pts',(39.0089042696538,-20.48000002,-101.379934587793));
#172220=CARTESIAN_POINT('Ctrl Pts',(39.5286840449944,-20.48000002,-101.45767138333));
#172221=CARTESIAN_POINT('Ctrl Pts',(38.985661982892,-19.9716359202423,-101.870016772883));
#172222=CARTESIAN_POINT('Ctrl Pts',(38.9771311417734,-20.48000002,-101.863799189494));
#172223=CARTESIAN_POINT('Ctrl Pts',(39.4870938285405,-20.48000002,-101.894962965541));
#172224=CARTESIAN_POINT('Ctrl Pts',(39.0038798675758,-19.9860848632948,
-102.348581386991));
#172225=CARTESIAN_POINT('Ctrl Pts',(39.0098865266841,-20.48000002,-102.348383053508));
#172226=CARTESIAN_POINT('Ctrl Pts',(39.5034933040112,-20.48000002,-102.330021385346));
#172227=CARTESIAN_POINT('',(39.5,-20.48000002,-102.144196959718));
#172228=CARTESIAN_POINT('Origin',(39.5,-19.98000002,-102.144196959718));
#172229=CARTESIAN_POINT('',(39.9829309662066,-20.48000002,-99.9929964369266));
#172230=CARTESIAN_POINT('Origin',(39.9829309662066,-19.98000002,-99.9929964369266));
#172231=CARTESIAN_POINT('Ctrl Pts',(39.5,-20.48000002,-102.144196959718));
#172232=CARTESIAN_POINT('Ctrl Pts',(39.5,-20.48000002,-101.901224059727));
#172233=CARTESIAN_POINT('Ctrl Pts',(39.5178405979396,-20.48000002,-101.658367298417));
#172234=CARTESIAN_POINT('Ctrl Pts',(39.5526223904373,-20.48000002,-101.419269624472));
#172235=CARTESIAN_POINT('Ctrl Pts',(39.5712680114436,-20.48000002,-101.291095534188));
#172236=CARTESIAN_POINT('Ctrl Pts',(39.5947811831661,-20.48000002,-101.164001820978));
#172237=CARTESIAN_POINT('Ctrl Pts',(39.6230172792885,-20.48000002,-101.038548856259));
#172238=CARTESIAN_POINT('Ctrl Pts',(39.6919421332749,-20.48000002,-100.732315755268));
#172239=CARTESIAN_POINT('Ctrl Pts',(39.7887207445095,-20.48000002,-100.433895586519));
#172240=CARTESIAN_POINT('Ctrl Pts',(39.9146180003271,-20.48000002,-100.143643141342));
#172241=CARTESIAN_POINT('Ctrl Pts',(39.93650642588,-20.48000002,-100.093180015704));
#172242=CARTESIAN_POINT('Ctrl Pts',(39.9592751462315,-20.48000002,-100.042963811213));
#172243=CARTESIAN_POINT('Ctrl Pts',(39.9829309662065,-20.48000002,-99.9929964369266));
#172244=CARTESIAN_POINT('Origin',(39.5,-19.98000002,-55.24995));
#172245=CARTESIAN_POINT('',(39.5,-20.48000002,-129.914446011788));
#172246=CARTESIAN_POINT('Origin',(39.5,-19.98000002,-129.914446011788));
#172247=CARTESIAN_POINT('',(39.5,-20.48000002,-55.24995));
#172248=CARTESIAN_POINT('Ctrl Pts',(39.,-19.98000002,-129.914446011788));
#172249=CARTESIAN_POINT('Ctrl Pts',(39.,-20.48000002,-129.914446011788));
#172250=CARTESIAN_POINT('Ctrl Pts',(39.5,-20.48000002,-129.914446011788));
#172251=CARTESIAN_POINT('Ctrl Pts',(39.,-19.9674346440713,-130.324899900514));
#172252=CARTESIAN_POINT('Ctrl Pts',(38.9872746975485,-20.48000002,-130.330124066848));
#172253=CARTESIAN_POINT('Ctrl Pts',(39.5000000028435,-20.48000002,-130.287671434236));
#172254=CARTESIAN_POINT('Ctrl Pts',(39.0456887600695,-19.9546004036482,
-130.727459443406));
#172255=CARTESIAN_POINT('Ctrl Pts',(39.0203709824336,-20.48000002,-130.73585622864));
#172256=CARTESIAN_POINT('Ctrl Pts',(39.5411198836701,-20.48000002,-130.653963774132));
#172257=CARTESIAN_POINT('Ctrl Pts',(39.2244077003248,-19.9284125341257,
-131.517220896748));
#172258=CARTESIAN_POINT('Ctrl Pts',(39.1707024462744,-20.48000002,-131.538360679722));
#172259=CARTESIAN_POINT('Ctrl Pts',(39.7019669306849,-20.48000002,-131.373086703203));
#172260=CARTESIAN_POINT('Ctrl Pts',(39.3590527322559,-19.9149653023259,
-131.906857743156));
#172261=CARTESIAN_POINT('Ctrl Pts',(39.2920635693995,-20.48000002,-131.938092167695));
#172262=CARTESIAN_POINT('Ctrl Pts',(39.8231470367065,-20.48000002,-131.72814043837));
#172263=CARTESIAN_POINT('Ctrl Pts',(39.5365899624517,-19.9017174575869,
-132.27695566545));
#172264=CARTESIAN_POINT('Ctrl Pts',(39.4537365768201,-20.48000002,-132.316180555747));
#172265=CARTESIAN_POINT('Ctrl Pts',(39.9829309662066,-20.48000002,-132.065646534579));
#172266=CARTESIAN_POINT('',(39.9829309662066,-20.48000002,-132.065646534579));
#172267=CARTESIAN_POINT('Origin',(39.9829309662066,-19.98000002,-132.065646534579));
#172268=CARTESIAN_POINT('Ctrl Pts',(39.9829309662066,-20.48000002,-132.065646534579));
#172269=CARTESIAN_POINT('Ctrl Pts',(39.8887941972372,-20.48000002,-131.866804677728));
#172270=CARTESIAN_POINT('Ctrl Pts',(39.8080127216862,-20.48000002,-131.661768384112));
#172271=CARTESIAN_POINT('Ctrl Pts',(39.7410867352565,-20.48000002,-131.453290684188));
#172272=CARTESIAN_POINT('Ctrl Pts',(39.6944643395902,-20.48000002,-131.308059656123));
#172273=CARTESIAN_POINT('Ctrl Pts',(39.6545649019177,-20.48000002,-131.161159371038));
#172274=CARTESIAN_POINT('Ctrl Pts',(39.6215434069806,-20.48000002,-131.013525238711));
#172275=CARTESIAN_POINT('Ctrl Pts',(39.5522800663376,-20.48000002,-130.70385927061));
#172276=CARTESIAN_POINT('Ctrl Pts',(39.5121705688344,-20.48000002,-130.389227115448));
#172277=CARTESIAN_POINT('Ctrl Pts',(39.5023709529579,-20.48000002,-130.069431842247));
#172278=CARTESIAN_POINT('Ctrl Pts',(39.5007919718951,-20.48000002,-130.017904242929));
#172279=CARTESIAN_POINT('Ctrl Pts',(39.5,-20.48000002,-129.966242581154));
#172280=CARTESIAN_POINT('Ctrl Pts',(39.5,-20.48000002,-129.914446011788));
#172281=CARTESIAN_POINT('Ctrl Pts',(58.4402350532158,-20.48000002,-171.237717270032));
#172282=CARTESIAN_POINT('Ctrl Pts',(57.9358462259716,-20.48000002,-171.474604875281));
#172283=CARTESIAN_POINT('Ctrl Pts',(57.9903087491627,-19.9260113903464,
-171.449026400902));
#172284=CARTESIAN_POINT('Ctrl Pts',(52.3041884424236,-20.48000002,-158.172646387016));
#172285=CARTESIAN_POINT('Ctrl Pts',(51.7549262849061,-20.4800000195716,
-158.328906441528));
#172286=CARTESIAN_POINT('Ctrl Pts',(51.8549375290089,-19.9204232153646,
-158.383965825354));
#172287=CARTESIAN_POINT('Ctrl Pts',(46.1592765266851,-20.48000002,-145.111728668187));
#172288=CARTESIAN_POINT('Ctrl Pts',(45.5582765746384,-20.4800000200247,
-145.178124710387));
#172289=CARTESIAN_POINT('Ctrl Pts',(45.7108852546953,-19.9134492574988,
-145.323053305542));
#172290=CARTESIAN_POINT('Ctrl Pts',(39.9829309662066,-20.48000002,-132.065646534579));
#172291=CARTESIAN_POINT('Ctrl Pts',(39.4537365768201,-20.48000002,-132.316180555747));
#172292=CARTESIAN_POINT('Ctrl Pts',(39.5365899624517,-19.9017174575869,
-132.27695566545));
#172293=CARTESIAN_POINT('',(58.4402350532158,-20.48000002,-171.237717270032));
#172294=CARTESIAN_POINT('Origin',(58.4402350532158,-19.98000002,-171.237717270032));
#172295=CARTESIAN_POINT('Ctrl Pts',(58.4402350532158,-20.48000002,-171.237717270032));
#172296=CARTESIAN_POINT('Ctrl Pts',(52.3041884424236,-20.48000002,-158.172646387016));
#172297=CARTESIAN_POINT('Ctrl Pts',(46.1592765266851,-20.48000002,-145.111728668187));
#172298=CARTESIAN_POINT('Ctrl Pts',(39.9829309662066,-20.48000002,-132.065646534579));
#172299=CARTESIAN_POINT('Ctrl Pts',(58.5817791104913,-20.48000002,-171.871644662643));
#172300=CARTESIAN_POINT('Ctrl Pts',(58.0183573349639,-20.48000002,-171.871644662643));
#172301=CARTESIAN_POINT('Ctrl Pts',(58.0853233553177,-19.9205720538986,
-171.871644662643));
#172302=CARTESIAN_POINT('Ctrl Pts',(58.5817790937258,-20.48000002,-171.652759539508));
#172303=CARTESIAN_POINT('Ctrl Pts',(58.018357325283,-20.48000002,-171.735617762033));
#172304=CARTESIAN_POINT('Ctrl Pts',(58.0853233550829,-19.9205720558596,
-171.725723025901));
#172305=CARTESIAN_POINT('Ctrl Pts',(58.5342346140381,-20.48000002,-171.437864213701));
#172306=CARTESIAN_POINT('Ctrl Pts',(57.9913238325147,-20.4800000200031,
-171.602371122267));
#172307=CARTESIAN_POINT('Ctrl Pts',(58.0534084851269,-19.9223906228206,
-171.582455328445));
#172308=CARTESIAN_POINT('Ctrl Pts',(58.4402350532158,-20.48000002,-171.237717270032));
#172309=CARTESIAN_POINT('Ctrl Pts',(57.9358462259716,-20.48000002,-171.474604875281));
#172310=CARTESIAN_POINT('Ctrl Pts',(57.9903087491627,-19.9260113903464,
-171.449026400902));
#172311=CARTESIAN_POINT('',(58.5817791104913,-20.48000002,-171.871644662643));
#172312=CARTESIAN_POINT('Origin',(58.5817791104913,-19.98000002,-171.871644662643));
#172313=CARTESIAN_POINT('Origin',(56.4084014798071,-20.48000002,-172.018072886377));
#172314=CARTESIAN_POINT('Origin',(58.5817791104913,-19.98000002,-179.64995));
#172315=CARTESIAN_POINT('',(58.0853233553177,-19.9205720538986,-179.64995));
#172316=CARTESIAN_POINT('',(58.5817791104913,-20.48000002,-171.871644662643));
#172317=CARTESIAN_POINT('Ctrl Pts',(60.,-20.98000002,-174.500886972636));
#172318=CARTESIAN_POINT('Ctrl Pts',(60.,-20.48000002,-174.500886972636));
#172319=CARTESIAN_POINT('Ctrl Pts',(59.5,-20.48000002,-174.500886972636));
#172320=CARTESIAN_POINT('Ctrl Pts',(60.,-20.9822194010082,-174.791464522024));
#172321=CARTESIAN_POINT('Ctrl Pts',(60.0022242907223,-20.48000002,-174.792108323791));
#172322=CARTESIAN_POINT('Ctrl Pts',(59.4999999934397,-20.48000002,-174.74311983516));
#172323=CARTESIAN_POINT('Ctrl Pts',(59.9586932949262,-20.9843889926879,
-175.075119998302));
#172324=CARTESIAN_POINT('Ctrl Pts',(59.9629392387446,-20.4800000199999,
-175.076359449429));
#172325=CARTESIAN_POINT('Ctrl Pts',(59.4655777479701,-20.48000002,-174.979582459221));
#172326=CARTESIAN_POINT('Ctrl Pts',(59.8360926556437,-20.9875676565265,
-175.49019987132));
#172327=CARTESIAN_POINT('Ctrl Pts',(59.8433264812564,-20.48000002,-175.492827860986));
#172328=CARTESIAN_POINT('Ctrl Pts',(59.3634105452706,-20.48000002,-175.325604118318));
#172329=CARTESIAN_POINT('Ctrl Pts',(59.7847122422101,-20.9886147234176,
-175.626841448369));
#172330=CARTESIAN_POINT('Ctrl Pts',(59.7928073162253,-20.4800000200006,
-175.630213503224));
#172331=CARTESIAN_POINT('Ctrl Pts',(59.3205935345334,-20.48000002,-175.43951222267));
#172332=CARTESIAN_POINT('Ctrl Pts',(59.6645318784846,-20.9906156905346,
-175.887821675912));
#172333=CARTESIAN_POINT('Ctrl Pts',(59.674123349008,-20.4800000199994,-175.892915048025));
#172334=CARTESIAN_POINT('Ctrl Pts',(59.2204432327122,-20.48000002,-175.657072445029));
#172335=CARTESIAN_POINT('Ctrl Pts',(59.5954458739788,-20.9915785299556,
-176.013328010605));
#172336=CARTESIAN_POINT('Ctrl Pts',(59.605650654114,-20.4800000200002,-176.019368430779));
#172337=CARTESIAN_POINT('Ctrl Pts',(59.162871562207,-20.48000002,-175.761697975082));
#172338=CARTESIAN_POINT('Ctrl Pts',(59.4392988603324,-20.9934287142977,
-176.254382360717));
#172339=CARTESIAN_POINT('Ctrl Pts',(59.4504692034509,-20.4800000199998,
-176.262509186853));
#172340=CARTESIAN_POINT('Ctrl Pts',(59.032749049719,-20.48000002,-175.962647558431));
#172341=CARTESIAN_POINT('Ctrl Pts',(59.3514188912717,-20.9943227517297,
-176.370801152158));
#172342=CARTESIAN_POINT('Ctrl Pts',(59.3629214966957,-20.48000002,-176.380037040048));
#172343=CARTESIAN_POINT('Ctrl Pts',(58.9595157418279,-20.48000002,-176.059697515632));
#172344=CARTESIAN_POINT('Ctrl Pts',(59.1611693306144,-20.9959919273243,
-176.588063887092));
#172345=CARTESIAN_POINT('Ctrl Pts',(59.1730156260874,-20.48000002,-176.599598651605));
#172346=CARTESIAN_POINT('Ctrl Pts',(58.800974443077,-20.48000002,-176.240813845549));
#172347=CARTESIAN_POINT('Ctrl Pts',(59.0590996873029,-20.9967669365736,
-176.688892319953));
#172348=CARTESIAN_POINT('Ctrl Pts',(59.0709534896778,-20.4800000200012,
-176.701568343258));
#172349=CARTESIAN_POINT('Ctrl Pts',(58.7159164062094,-20.48000002,-176.324867284949));
#172350=CARTESIAN_POINT('Ctrl Pts',(58.7325172788836,-20.9989167502369,
-176.968486930424));
#172351=CARTESIAN_POINT('Ctrl Pts',(58.7436561080181,-20.4800000199975,
-176.984811315106));
#172352=CARTESIAN_POINT('Ctrl Pts',(58.4437643988224,-20.48000002,-176.557945321316));
#172353=CARTESIAN_POINT('Ctrl Pts',(58.484009011739,-21.0001266369645,-177.125700665905));
#172354=CARTESIAN_POINT('Ctrl Pts',(58.4942266187642,-20.4800000200099,
-177.144085084891));
#172355=CARTESIAN_POINT('Ctrl Pts',(58.2366741051621,-20.48000002,-176.68900326854));
#172356=CARTESIAN_POINT('Ctrl Pts',(58.2221195094937,-21.0010265837306,
-177.24260269584));
#172357=CARTESIAN_POINT('Ctrl Pts',(58.2310611931749,-20.4800000199999,
-177.262627176116));
#172358=CARTESIAN_POINT('Ctrl Pts',(58.0184329245781,-20.48000002,-176.786456163744));
#172359=CARTESIAN_POINT('',(59.5,-20.48000002,-174.500886972636));
#172360=CARTESIAN_POINT('Ctrl Pts',(59.5,-20.48000002,-174.500886972636));
#172361=CARTESIAN_POINT('Ctrl Pts',(59.5,-20.48000002,-174.594133457896));
#172362=CARTESIAN_POINT('Ctrl Pts',(59.4948998873889,-20.48000002,-174.686506499847));
#172363=CARTESIAN_POINT('Ctrl Pts',(59.484743418878,-20.48000002,-174.778024581704));
#172364=CARTESIAN_POINT('Ctrl Pts',(59.4745869503671,-20.48000002,-174.869542663562));
#172365=CARTESIAN_POINT('Ctrl Pts',(59.4593733052792,-20.4800000198432,
-174.96020535248));
#172366=CARTESIAN_POINT('Ctrl Pts',(59.4391579117629,-20.4800000201565,
-175.050010672616));
#172367=CARTESIAN_POINT('Ctrl Pts',(59.4270641008619,-20.4800000203439,
-175.103736490952));
#172368=CARTESIAN_POINT('Ctrl Pts',(59.4131703468088,-20.4800000205099,
-175.157156500734));
#172369=CARTESIAN_POINT('Ctrl Pts',(59.3974877716946,-20.4800000205022,
-175.210269911122));
#172370=CARTESIAN_POINT('Ctrl Pts',(59.3634319732391,-20.4800000204854,
-175.325609361837));
#172371=CARTESIAN_POINT('Ctrl Pts',(59.3206017517199,-20.4800000200584,
-175.43951508737));
#172372=CARTESIAN_POINT('Ctrl Pts',(59.2705225473981,-20.480000020021,-175.548294250575));
#172373=CARTESIAN_POINT('Ctrl Pts',(59.2665668880551,-20.4800000200181,
-175.556886505965));
#172374=CARTESIAN_POINT('Ctrl Pts',(59.2625645131408,-20.4800000200159,
-175.56545285612));
#172375=CARTESIAN_POINT('Ctrl Pts',(59.2585154363462,-20.4800000200145,
-175.573993307709));
#172376=CARTESIAN_POINT('Ctrl Pts',(59.2235121463779,-20.4800000200017,
-175.647823446922));
#172377=CARTESIAN_POINT('Ctrl Pts',(59.1850753506039,-20.4800000200467,
-175.719619366777));
#172378=CARTESIAN_POINT('Ctrl Pts',(59.1431476193817,-20.4800000203096,
-175.789501989863));
#172379=CARTESIAN_POINT('Ctrl Pts',(59.1284714749913,-20.4800000204017,
-175.813963305486));
#172380=CARTESIAN_POINT('Ctrl Pts',(59.1133672159704,-20.4800000205138,
-175.838189938606));
#172381=CARTESIAN_POINT('Ctrl Pts',(59.0978311232235,-20.4800000206151,
-175.862186246726));
#172382=CARTESIAN_POINT('Ctrl Pts',(59.057684395778,-20.4800000208766,-175.924194967805));
#172383=CARTESIAN_POINT('Ctrl Pts',(59.0143956166168,-20.4800000209379,
-175.984944386851));
#172384=CARTESIAN_POINT('Ctrl Pts',(58.9683824813746,-20.4800000205207,
-176.043771514579));
#172385=CARTESIAN_POINT('Ctrl Pts',(58.939956521226,-20.4800000202629,-176.080113693386));
#172386=CARTESIAN_POINT('Ctrl Pts',(58.9105390187326,-20.480000020158,-176.115667750748));
#172387=CARTESIAN_POINT('Ctrl Pts',(58.8802525752657,-20.4800000200989,
-176.150262230718));
#172388=CARTESIAN_POINT('Ctrl Pts',(58.8008883718402,-20.4800000199439,
-176.240915441575));
#172389=CARTESIAN_POINT('Ctrl Pts',(58.7158063838685,-20.4800000199516,
-176.324965650418));
#172390=CARTESIAN_POINT('Ctrl Pts',(58.6252060810682,-20.4800000201162,
-176.402568149682));
#172391=CARTESIAN_POINT('Ctrl Pts',(58.6108845926547,-20.4800000201422,
-176.414835032459));
#172392=CARTESIAN_POINT('Ctrl Pts',(58.5964064444941,-20.4800000201761,
-176.426947791328));
#172393=CARTESIAN_POINT('Ctrl Pts',(58.5817791104913,-20.4800000202216,
-176.438901946458));
#172394=CARTESIAN_POINT('Origin',(59.5,-20.98000002,-174.500886972636));
#172395=CARTESIAN_POINT('Ctrl Pts',(39.9829309662066,-20.48000002,-99.9929964369266));
#172396=CARTESIAN_POINT('Ctrl Pts',(39.4537365768202,-20.48000002,-99.742462415759));
#172397=CARTESIAN_POINT('Ctrl Pts',(39.5365899624517,-19.9017174575869,
-99.7816873060563));
#172398=CARTESIAN_POINT('Ctrl Pts',(46.1212593572987,-20.48000002,-87.0272166609364));
#172399=CARTESIAN_POINT('Ctrl Pts',(45.5211976544485,-20.48000002,-86.9586415917399));
#172400=CARTESIAN_POINT('Ctrl Pts',(45.6728806075319,-19.9133770447829,
-86.815892326284));
#172401=CARTESIAN_POINT('Ctrl Pts',(52.2285110086243,-20.48000002,-74.0467697366574));
#172402=CARTESIAN_POINT('Ctrl Pts',(51.6794916123544,-20.4800000199249,
-73.8897477208158));
#172403=CARTESIAN_POINT('Ctrl Pts',(51.7792721521254,-19.9203329608279,
-73.8354504790526));
#172404=CARTESIAN_POINT('Ctrl Pts',(58.3269264615434,-20.48000002,-61.0621827299711));
#172405=CARTESIAN_POINT('Ctrl Pts',(57.8224346115608,-20.48000002,-60.8252402001721));
#172406=CARTESIAN_POINT('Ctrl Pts',(57.8770125754992,-19.9259080025173,
-60.8508735991007));
#172407=CARTESIAN_POINT('',(57.8770125754992,-19.9259080025173,-60.8508735991007));
#172408=CARTESIAN_POINT('Ctrl Pts',(57.8770125754992,-19.9259080025173,
-60.8508735991007));
#172409=CARTESIAN_POINT('Ctrl Pts',(56.2239580313905,-19.9243966479237,
-64.3709010723032));
#172410=CARTESIAN_POINT('Ctrl Pts',(54.6344108974312,-19.9229079589042,
-67.7535839786999));
#172411=CARTESIAN_POINT('Ctrl Pts',(52.3453693536531,-19.9204384147188,
-72.6215914880863));
#172412=CARTESIAN_POINT('Ctrl Pts',(51.5982350930194,-19.9195813611909,
-74.2099245161803));
#172413=CARTESIAN_POINT('Ctrl Pts',(50.5013522959551,-19.9182610265938,
-76.5409198457692));
#172414=CARTESIAN_POINT('Ctrl Pts',(49.9588655093536,-19.9175926897662,
-77.6935414574256));
#172415=CARTESIAN_POINT('Ctrl Pts',(49.336384233353,-19.9168076573922,-79.0157335780332));
#172416=CARTESIAN_POINT('Ctrl Pts',(48.9864133340098,-19.9163628051879,
-79.7589815597841));
#172417=CARTESIAN_POINT('Ctrl Pts',(48.8137672692214,-19.9161425058677,
-80.1255999074955));
#172418=CARTESIAN_POINT('Ctrl Pts',(48.7263143503862,-19.9160307783446,
-80.3112990142576));
#172419=CARTESIAN_POINT('Ctrl Pts',(48.7241371808068,-19.9160279967759,
-80.3159220498041));
#172420=CARTESIAN_POINT('Ctrl Pts',(45.3540283295419,-19.9117221121947,
-87.4720485631386));
#172421=CARTESIAN_POINT('Ctrl Pts',(42.2926058529678,-19.9069541729552,
-93.9583097862753));
#172422=CARTESIAN_POINT('Ctrl Pts',(39.5365899624517,-19.9017174575869,
-99.7816873060563));
#172423=CARTESIAN_POINT('',(58.3269264615434,-20.48000002,-61.0621827299711));
#172424=CARTESIAN_POINT('Origin',(58.3269264615434,-19.98000002,-61.0621827299711));
#172425=CARTESIAN_POINT('Ctrl Pts',(39.9829309662066,-20.48000002,-99.9929964369266));
#172426=CARTESIAN_POINT('Ctrl Pts',(46.1212593572987,-20.48000002,-87.0272166609364));
#172427=CARTESIAN_POINT('Ctrl Pts',(52.2285110086243,-20.48000002,-74.0467697366574));
#172428=CARTESIAN_POINT('Ctrl Pts',(58.3269264615434,-20.48000002,-61.0621827299711));
#172429=CARTESIAN_POINT('Origin',(59.5,-20.98000002,-55.24995));
#172430=CARTESIAN_POINT('',(59.5,-20.48000002,-58.1336824582564));
#172431=CARTESIAN_POINT('',(59.5,-20.48000002,-174.524030413304));
#172432=CARTESIAN_POINT('',(60.,-20.98000002,-58.1336824582564));
#172433=CARTESIAN_POINT('Origin',(59.5,-20.98000002,-58.1336824582564));
#172434=CARTESIAN_POINT('',(60.,-20.98000002,-58.1134713856835));
#172435=CARTESIAN_POINT('Origin',(60.,-2.55003103885676E-14,0.));
#172436=CARTESIAN_POINT('',(60.,-21.48000002,-58.1532962439713));
#172437=CARTESIAN_POINT('Ctrl Pts',(60.,-20.98000002,-58.1336824582564));
#172438=CARTESIAN_POINT('Ctrl Pts',(60.,-21.1466635001965,-58.1403364979909));
#172439=CARTESIAN_POINT('Ctrl Pts',(60.,-21.3133297017902,-58.1468913732678));
#172440=CARTESIAN_POINT('Ctrl Pts',(60.,-21.48000002,-58.1532962439713));
#172441=CARTESIAN_POINT('',(60.,-21.48000002,-174.45635375974));
#172442=CARTESIAN_POINT('Origin',(59.5,-21.48000002,-55.24995));
#172443=CARTESIAN_POINT('',(59.5,-21.98000002,-58.1532962439713));
#172444=CARTESIAN_POINT('Origin',(59.5,-21.48000002,-58.1532962439713));
#172445=CARTESIAN_POINT('',(59.5,-21.98000002,-174.47822483969));
#172446=CARTESIAN_POINT('',(59.5,-21.98000002,-58.1720074546108));
#172447=CARTESIAN_POINT('Origin',(59.5,-21.48000002,-174.47822483969));
#172448=CARTESIAN_POINT('Ctrl Pts',(59.5,-21.98000002,-174.47822483969));
#172449=CARTESIAN_POINT('Ctrl Pts',(60.,-21.98000002,-174.47822483969));
#172450=CARTESIAN_POINT('Ctrl Pts',(60.,-21.48000002,-174.47822483969));
#172451=CARTESIAN_POINT('Ctrl Pts',(59.4999999932692,-21.98000002,-174.72672222605));
#172452=CARTESIAN_POINT('Ctrl Pts',(59.9977907999382,-21.9800000199965,
-174.775666642734));
#172453=CARTESIAN_POINT('Ctrl Pts',(60.,-21.4822140856788,-174.77632287275));
#172454=CARTESIAN_POINT('Ctrl Pts',(59.4638082272143,-21.98000002,-174.969157756816));
#172455=CARTESIAN_POINT('Ctrl Pts',(59.9524075929633,-21.98000002,-175.065899995449));
#172456=CARTESIAN_POINT('Ctrl Pts',(59.9565698697824,-21.4843793273514,
-175.067148740399));
#172457=CARTESIAN_POINT('Ctrl Pts',(59.3562425753485,-21.98000002,-175.323664095203));
#172458=CARTESIAN_POINT('Ctrl Pts',(59.8205081565721,-21.98000002,-175.489804158754));
#172459=CARTESIAN_POINT('Ctrl Pts',(59.8274910918555,-21.4875521339025,
-175.492414399022));
#172460=CARTESIAN_POINT('Ctrl Pts',(59.3112699374162,-21.98000002,-175.439952697294));
#172461=CARTESIAN_POINT('Ctrl Pts',(59.7657533403762,-21.9800000200007,
-175.628582862653));
#172462=CARTESIAN_POINT('Ctrl Pts',(59.7735239255666,-21.4885940652802,
-175.631914079949));
#172463=CARTESIAN_POINT('Ctrl Pts',(59.2061209187896,-21.98000002,-175.661808757878));
#172464=CARTESIAN_POINT('Ctrl Pts',(59.6382394618755,-21.9800000199994,
-175.893067776338));
#172465=CARTESIAN_POINT('Ctrl Pts',(59.6473451018805,-21.4905837846614,
-175.89805223939));
#172466=CARTESIAN_POINT('Ctrl Pts',(59.1456765053938,-21.98000002,-175.768375282423));
#172467=CARTESIAN_POINT('Ctrl Pts',(59.5651790529315,-21.9800000199994,
-176.020005430174));
#172468=CARTESIAN_POINT('Ctrl Pts',(59.5748118056443,-21.4915405113197,
-176.025889197601));
#172469=CARTESIAN_POINT('Ctrl Pts',(59.0089721749525,-21.98000002,-175.972743369523));
#172470=CARTESIAN_POINT('Ctrl Pts',(59.4003458450454,-21.9800000200006,
-176.263201660659));
#172471=CARTESIAN_POINT('Ctrl Pts',(59.4107666107714,-21.493376849955,-176.271048580335));
#172472=CARTESIAN_POINT('Ctrl Pts',(58.9319928876421,-21.98000002,-176.071220734744));
#172473=CARTESIAN_POINT('Ctrl Pts',(59.3077278616495,-21.9800000199987,
-176.380304393309));
#172474=CARTESIAN_POINT('Ctrl Pts',(59.3183914660909,-21.4942625520954,
-176.389181693558));
#172475=CARTESIAN_POINT('Ctrl Pts',(58.7662605376602,-21.98000002,-176.253552125047));
#172476=CARTESIAN_POINT('Ctrl Pts',(59.1086757415209,-21.9800000200013,
-176.59692321781));
#172477=CARTESIAN_POINT('Ctrl Pts',(59.1195126442718,-21.495903657329,-176.607905725284));
#172478=CARTESIAN_POINT('Ctrl Pts',(58.6773437522104,-21.98000002,-176.337917446619));
#172479=CARTESIAN_POINT('Ctrl Pts',(59.0020443621077,-21.9800000199996,
-176.697095400112));
#172480=CARTESIAN_POINT('Ctrl Pts',(59.012812502338,-21.4966636432885,-176.7091099968));
#172481=CARTESIAN_POINT('Ctrl Pts',(58.3926916168304,-21.98000002,-176.570893328242));
#172482=CARTESIAN_POINT('Ctrl Pts',(58.6613611188049,-21.9800000200008,
-176.973308002926));
#172483=CARTESIAN_POINT('Ctrl Pts',(58.6712299408253,-21.4987636190772,
-176.988586760981));
#172484=CARTESIAN_POINT('Ctrl Pts',(58.1758692424685,-21.98000002,-176.700106570217));
#172485=CARTESIAN_POINT('Ctrl Pts',(58.4021689190212,-21.9800000199881,
-177.126531916838));
#172486=CARTESIAN_POINT('Ctrl Pts',(58.4110432062101,-21.4999301516852,
-177.143590179504));
#172487=CARTESIAN_POINT('Ctrl Pts',(57.9501667771809,-21.98000002,-176.792941619423));
#172488=CARTESIAN_POINT('Ctrl Pts',(58.132621442372,-21.98000002,-177.23652912386));
#172489=CARTESIAN_POINT('Ctrl Pts',(58.140200132617,-21.5007687140674,-177.254954590203));
#172490=CARTESIAN_POINT('Ctrl Pts',(58.2281061322556,-21.9799999688995,
-176.657965001835));
#172491=CARTESIAN_POINT('Ctrl Pts',(58.2763381470521,-21.9799999587489,
-176.630735497029));
#172492=CARTESIAN_POINT('Ctrl Pts',(58.3235842378115,-21.9799999676447,
-176.601941540627));
#172493=CARTESIAN_POINT('Ctrl Pts',(58.3697659029187,-21.9799999836463,
-176.571657891927));
#172494=CARTESIAN_POINT('Ctrl Pts',(58.4333419149384,-21.9800000056749,
-176.529967892025));
#172495=CARTESIAN_POINT('Ctrl Pts',(58.4951281469266,-21.9800000132519,
-176.485368653426));
#172496=CARTESIAN_POINT('Ctrl Pts',(58.5544579572714,-21.9800000168151,
-176.438221543427));
#172497=CARTESIAN_POINT('Ctrl Pts',(58.5638633718754,-21.98000001738,-176.430747423514));
#172498=CARTESIAN_POINT('Ctrl Pts',(58.573207108192,-21.9800000178323,-176.423209364714));
#172499=CARTESIAN_POINT('Ctrl Pts',(58.582486579001,-21.9800000181999,-176.415608906189));
#172500=CARTESIAN_POINT('Ctrl Pts',(58.6422321318881,-21.9800000205672,
-176.366673616007));
#172501=CARTESIAN_POINT('Ctrl Pts',(58.6996264562076,-21.9800000199999,
-176.315076489292));
#172502=CARTESIAN_POINT('Ctrl Pts',(58.7545482746591,-21.9800000199988,
-176.260908374673));
#172503=CARTESIAN_POINT('Ctrl Pts',(58.7869024533102,-21.9800000199981,
-176.228998199318));
#172504=CARTESIAN_POINT('Ctrl Pts',(58.8184303801206,-21.9800000199976,
-176.196159475715));
#172505=CARTESIAN_POINT('Ctrl Pts',(58.8491278703888,-21.9800000199976,
-176.162387482235));
#172506=CARTESIAN_POINT('Ctrl Pts',(58.9319941632242,-21.9800000199974,
-176.071221726439));
#172507=CARTESIAN_POINT('Ctrl Pts',(59.0089727564858,-21.9800000199996,
-175.972743969313));
#172508=CARTESIAN_POINT('Ctrl Pts',(59.0773246245197,-21.9800000199999,
-175.870559516175));
#172509=CARTESIAN_POINT('Ctrl Pts',(59.1060118933486,-21.98000002,-175.82767271642));
#172510=CARTESIAN_POINT('Ctrl Pts',(59.1333062996812,-21.98000002,-175.784013939838));
#172511=CARTESIAN_POINT('Ctrl Pts',(59.1592107352546,-21.98000002,-175.739584721266));
#172512=CARTESIAN_POINT('Ctrl Pts',(59.1950270177852,-21.98000002,-175.678155494582));
#172513=CARTESIAN_POINT('Ctrl Pts',(59.2281939400895,-21.9800000200315,
-175.615256612429));
#172514=CARTESIAN_POINT('Ctrl Pts',(59.2587125449347,-21.9800000196412,
-175.550888840134));
#172515=CARTESIAN_POINT('Ctrl Pts',(59.311304650302,-21.9800000189686,-175.439965137037));
#172516=CARTESIAN_POINT('Ctrl Pts',(59.356300154325,-21.98000001654,-175.32367896183));
#172517=CARTESIAN_POINT('Ctrl Pts',(59.3921466355886,-21.9800000173947,
-175.205510135853));
#172518=CARTESIAN_POINT('Ctrl Pts',(59.3996691193178,-21.9800000175741,
-175.180712079269));
#172519=CARTESIAN_POINT('Ctrl Pts',(59.4067991608448,-21.9800000178929,
-175.15584684927));
#172520=CARTESIAN_POINT('Ctrl Pts',(59.4135356395821,-21.9800000182925,
-175.130914599889));
#172521=CARTESIAN_POINT('Ctrl Pts',(59.4621021364647,-21.9800000211732,
-174.951166090456));
#172522=CARTESIAN_POINT('Ctrl Pts',(59.4903344201338,-21.9800000199997,
-174.767951128808));
#172523=CARTESIAN_POINT('Ctrl Pts',(59.4979153635692,-21.98000002,-174.581221680396));
#172524=CARTESIAN_POINT('Ctrl Pts',(59.499304412066,-21.98000002,-174.547007434923));
#172525=CARTESIAN_POINT('Ctrl Pts',(59.5,-21.98000002,-174.512675235736));
#172526=CARTESIAN_POINT('Ctrl Pts',(59.5,-21.98000002,-174.47822483969));
#172527=CARTESIAN_POINT('Origin',(58.2281061322669,-22.48000002,-179.64995));
#172528=CARTESIAN_POINT('',(58.2281061322669,-21.98000002,-171.871644662643));
#172529=CARTESIAN_POINT('',(58.2281061322669,-21.98000002,-176.848603273909));
#172530=CARTESIAN_POINT('Origin',(58.2281061322669,-22.48000002,-171.871644662643));
#172531=CARTESIAN_POINT('',(57.7346476057223,-22.3993856132206,-179.64995));
#172532=CARTESIAN_POINT('Ctrl Pts',(58.0564197191617,-21.9800000366742,
-171.178790026127));
#172533=CARTESIAN_POINT('Ctrl Pts',(57.6735493970763,-21.9798882430102,
-171.380807602766));
#172534=CARTESIAN_POINT('Ctrl Pts',(57.6186574596683,-22.4082912353334,
-171.40978315061));
#172535=CARTESIAN_POINT('Ctrl Pts',(58.1793335836445,-21.9800000364255,
-171.412176181737));
#172536=CARTESIAN_POINT('Ctrl Pts',(57.7654281245283,-21.9798905214978,
-171.542966774725));
#172537=CARTESIAN_POINT('Ctrl Pts',(57.7016369198821,-22.4019038408433,
-171.565352937794));
#172538=CARTESIAN_POINT('Ctrl Pts',(58.2385448347246,-21.9800000363068,
-171.671295447806));
#172539=CARTESIAN_POINT('Ctrl Pts',(57.8110872810659,-21.9798915951361,
-171.728859197825));
#172540=CARTESIAN_POINT('Ctrl Pts',(57.7416081447113,-22.3988541543228,
-171.738094620076));
#172541=CARTESIAN_POINT('Ctrl Pts',(58.2267633341816,-21.9800000363304,
-171.938197690258));
#172542=CARTESIAN_POINT('Ctrl Pts',(57.8020514502591,-21.9798913838386,
-171.91910344938));
#172543=CARTESIAN_POINT('Ctrl Pts',(57.7336548687769,-22.399461430235,-171.916008414622));
#172544=CARTESIAN_POINT('',(58.085700246061,-21.98000002,-171.237717270032));
#172545=CARTESIAN_POINT('Origin',(56.8433387828479,-21.9799994107774,-171.841912580628));
#172546=CARTESIAN_POINT('Origin',(58.085700246061,-22.48000002,-171.237717270032));
#172547=CARTESIAN_POINT('Ctrl Pts',(40.0320988180411,-21.98000002,-133.252725050377));
#172548=CARTESIAN_POINT('Ctrl Pts',(39.6675936435998,-21.98000002,-133.427429361974));
#172549=CARTESIAN_POINT('Ctrl Pts',(39.5912209089345,-22.3752378108182,
-133.464034181247));
#172550=CARTESIAN_POINT('Ctrl Pts',(46.0913014593244,-21.98000002,-145.894718230889));
#172551=CARTESIAN_POINT('Ctrl Pts',(45.790260298639,-21.98000002,-146.231563592216));
#172552=CARTESIAN_POINT('Ctrl Pts',(45.6468692907591,-22.3902470227078,
-146.106052933848));
#172553=CARTESIAN_POINT('Ctrl Pts',(52.0964117641256,-21.98000002,-158.56249372189));
#172554=CARTESIAN_POINT('Ctrl Pts',(51.7509431131532,-21.9800000203624,
-158.826102375503));
#172555=CARTESIAN_POINT('Ctrl Pts',(51.6504270099243,-22.3994099070849,
-158.773819030963));
#172556=CARTESIAN_POINT('Ctrl Pts',(58.085700246061,-21.98000002,-171.237717270032));
#172557=CARTESIAN_POINT('Ctrl Pts',(57.6956367824858,-21.98000002,-171.422029807066));
#172558=CARTESIAN_POINT('Ctrl Pts',(57.638503474757,-22.4067641070473,-171.449026400902));
#172559=CARTESIAN_POINT('',(40.032098818041,-21.98000002,-133.252725050377));
#172560=CARTESIAN_POINT('Ctrl Pts',(40.0320988180411,-21.98000002,-133.252725050377));
#172561=CARTESIAN_POINT('Ctrl Pts',(46.0913111616059,-21.98000002,-145.894738473846));
#172562=CARTESIAN_POINT('Ctrl Pts',(52.0964027110273,-21.98000002,-158.56247456275));
#172563=CARTESIAN_POINT('Ctrl Pts',(58.085700246061,-21.98000002,-171.237717270032));
#172564=CARTESIAN_POINT('Origin',(40.0320988180411,-22.48000002,-133.252725050377));
#172565=CARTESIAN_POINT('Ctrl Pts',(39.5912209089345,-22.3752378108182,
-133.464034181247));
#172566=CARTESIAN_POINT('Ctrl Pts',(39.6675936435998,-21.98000002,-133.427429361974));
#172567=CARTESIAN_POINT('Ctrl Pts',(40.0320988180411,-21.98000002,-133.252725050377));
#172568=CARTESIAN_POINT('Ctrl Pts',(39.3953798878174,-22.3926947961315,
-133.064083894138));
#172569=CARTESIAN_POINT('Ctrl Pts',(39.4616506489997,-21.98000002,-133.032398833922));
#172570=CARTESIAN_POINT('Ctrl Pts',(39.8558398148562,-21.98000002,-132.884976140755));
#172571=CARTESIAN_POINT('Ctrl Pts',(39.2495325922488,-22.4102623065174,
-132.649599803771));
#172572=CARTESIAN_POINT('Ctrl Pts',(39.306634221246,-21.98000002,-132.626108677501));
#172573=CARTESIAN_POINT('Ctrl Pts',(39.7245793327553,-21.98000002,-132.504273278823));
#172574=CARTESIAN_POINT('Ctrl Pts',(39.0515573542344,-22.4453411404847,
-131.793566113248));
#172575=CARTESIAN_POINT('Ctrl Pts',(39.0825794362701,-21.9800000199999,
-131.782866385322));
#172576=CARTESIAN_POINT('Ctrl Pts',(39.5464016190797,-21.98000002,-131.71886357396));
#172577=CARTESIAN_POINT('Ctrl Pts',(39.,-22.4629715740863,-131.348761468896));
#172578=CARTESIAN_POINT('Ctrl Pts',(39.0167438766121,-21.9800000200007,
-131.341321155374));
#172579=CARTESIAN_POINT('Ctrl Pts',(39.5000000005303,-21.98000002,-131.311180490184));
#172580=CARTESIAN_POINT('Ctrl Pts',(39.,-22.48000002,-130.903539806302));
#172581=CARTESIAN_POINT('Ctrl Pts',(39.,-21.98000002,-130.903539806302));
#172582=CARTESIAN_POINT('Ctrl Pts',(39.5,-21.98000002,-130.903539806302));
#172583=CARTESIAN_POINT('',(39.5,-21.98000002,-130.903539806302));
#172584=CARTESIAN_POINT('Ctrl Pts',(39.5,-21.98000002,-130.903539806302));
#172585=CARTESIAN_POINT('Ctrl Pts',(39.5,-21.98000002,-131.168997483208));
#172586=CARTESIAN_POINT('Ctrl Pts',(39.5196729008546,-21.98000002,-131.434381070388));
#172587=CARTESIAN_POINT('Ctrl Pts',(39.5579798343717,-21.98000002,-131.695636340096));
#172588=CARTESIAN_POINT('Ctrl Pts',(39.5785131750261,-21.98000002,-131.835674786355));
#172589=CARTESIAN_POINT('Ctrl Pts',(39.6044013642074,-21.98000002,-131.974527214016));
#172590=CARTESIAN_POINT('Ctrl Pts',(39.6354904757816,-21.98000002,-132.111568426422));
#172591=CARTESIAN_POINT('Ctrl Pts',(39.7067779603521,-21.98000002,-132.425804595304));
#172592=CARTESIAN_POINT('Ctrl Pts',(39.805057091038,-21.98000002,-132.732328205559));
#172593=CARTESIAN_POINT('Ctrl Pts',(39.9318010945635,-21.98000002,-133.030718310498));
#172594=CARTESIAN_POINT('Ctrl Pts',(39.9634506501669,-21.98000002,-133.105230034564));
#172595=CARTESIAN_POINT('Ctrl Pts',(39.9968754124341,-21.98000002,-133.179234513779));
#172596=CARTESIAN_POINT('Ctrl Pts',(40.032098818041,-21.98000002,-133.252725050377));
#172597=CARTESIAN_POINT('Origin',(39.5,-22.48000002,-130.903539806302));
#172598=CARTESIAN_POINT('Origin',(39.5,-22.48000002,-55.24995));
#172599=CARTESIAN_POINT('',(39.5,-21.98000002,-101.155103165204));
#172600=CARTESIAN_POINT('',(39.5,-21.98000002,-55.24995));
#172601=CARTESIAN_POINT('Origin',(39.5,-22.48000002,-101.155103165204));
#172602=CARTESIAN_POINT('Ctrl Pts',(39.,-22.48000002,-101.155103165204));
#172603=CARTESIAN_POINT('Ctrl Pts',(39.,-21.98000002,-101.155103165204));
#172604=CARTESIAN_POINT('Ctrl Pts',(39.5,-21.98000002,-101.155103165204));
#172605=CARTESIAN_POINT('Ctrl Pts',(39.,-22.4629652077836,-100.709715051444));
#172606=CARTESIAN_POINT('Ctrl Pts',(39.0167494918295,-21.9800000199972,
-100.717175065292));
#172607=CARTESIAN_POINT('Ctrl Pts',(39.5000000028409,-21.98000002,-100.74730649838));
#172608=CARTESIAN_POINT('Ctrl Pts',(39.0503363863868,-22.445662928874,-100.273107244626));
#172609=CARTESIAN_POINT('Ctrl Pts',(39.0810957011176,-21.9800000199993,
-100.283723962358));
#172610=CARTESIAN_POINT('Ctrl Pts',(39.5453027473158,-21.98000002,-100.347142039227));
#172611=CARTESIAN_POINT('Ctrl Pts',(39.2470786821289,-22.4105936079244,
-99.4169535019087));
#172612=CARTESIAN_POINT('Ctrl Pts',(39.3039755059085,-21.9800000200007,
-99.4402934124299));
#172613=CARTESIAN_POINT('Ctrl Pts',(39.7223708143483,-21.98000002,-99.5616325432134));
#172614=CARTESIAN_POINT('Ctrl Pts',(39.3953243387798,-22.392699749305,-98.9946725198791));
#172615=CARTESIAN_POINT('Ctrl Pts',(39.461600153608,-21.98000002,-99.0263409880856));
#172616=CARTESIAN_POINT('Ctrl Pts',(39.8557911961828,-21.98000002,-99.1737682638933));
#172617=CARTESIAN_POINT('Ctrl Pts',(39.5912209089311,-22.3752378108185,
-98.5946087902659));
#172618=CARTESIAN_POINT('Ctrl Pts',(39.6675936435963,-21.98000002,-98.6312136095388));
#172619=CARTESIAN_POINT('Ctrl Pts',(40.032098818038,-21.98000002,-98.8059179211357));
#172620=CARTESIAN_POINT('',(40.032098818038,-21.98000002,-98.8059179211358));
#172621=CARTESIAN_POINT('Ctrl Pts',(40.032098818038,-21.98000002,-98.8059179211358));
#172622=CARTESIAN_POINT('Ctrl Pts',(39.9030508971585,-21.98000002,-99.0751650535137));
#172623=CARTESIAN_POINT('Ctrl Pts',(39.7969528124074,-21.98000002,-99.3552012197209));
#172624=CARTESIAN_POINT('Ctrl Pts',(39.7146317074512,-21.98000002,-99.6400255235404));
#172625=CARTESIAN_POINT('Ctrl Pts',(39.6845025786606,-21.98000002,-99.7442698499136));
#172626=CARTESIAN_POINT('Ctrl Pts',(39.6575579700038,-21.98000002,-99.849155332173));
#172627=CARTESIAN_POINT('Ctrl Pts',(39.6338367806139,-21.98000002,-99.9543872911712));
#172628=CARTESIAN_POINT('Ctrl Pts',(39.561388548558,-21.98000002,-100.275782195106));
#172629=CARTESIAN_POINT('Ctrl Pts',(39.5178914194317,-21.98000002,-100.602110104162));
#172630=CARTESIAN_POINT('Ctrl Pts',(39.5044747449633,-21.98000002,-100.933563458967));
#172631=CARTESIAN_POINT('Ctrl Pts',(39.5014958184563,-21.98000002,-101.007156597624));
#172632=CARTESIAN_POINT('Ctrl Pts',(39.5,-21.98000002,-101.081002444677));
#172633=CARTESIAN_POINT('Ctrl Pts',(39.5,-21.98000002,-101.155103165204));
#172634=CARTESIAN_POINT('',(39.5912209089345,-22.3752378108151,-98.5946087902606));
#172635=CARTESIAN_POINT('Origin',(40.032098818038,-22.4800000199998,-98.8059179211357));
#172636=CARTESIAN_POINT('Ctrl Pts',(39.,-22.48000002,-101.155103165204));
#172637=CARTESIAN_POINT('Ctrl Pts',(39.,-22.4767350571047,-101.069738228568));
#172638=CARTESIAN_POINT('Ctrl Pts',(39.001844810516,-22.4732834802974,-100.980072408275));
#172639=CARTESIAN_POINT('Ctrl Pts',(39.0061450083956,-22.4696426076462,
-100.88622267467));
#172640=CARTESIAN_POINT('Ctrl Pts',(39.0096198368864,-22.4667005551237,
-100.810386227766));
#172641=CARTESIAN_POINT('Ctrl Pts',(39.0146989999904,-22.4636348949715,
-100.73181802585));
#172642=CARTESIAN_POINT('Ctrl Pts',(39.0217284047154,-22.4604441490632,
-100.65058434866));
#172643=CARTESIAN_POINT('Ctrl Pts',(39.026292189657,-22.458372582736,-100.597844031776));
#172644=CARTESIAN_POINT('Ctrl Pts',(39.031678928859,-22.4562481400062,-100.543976489461));
#172645=CARTESIAN_POINT('Ctrl Pts',(39.0379859380183,-22.454071013344,-100.489016010024));
#172646=CARTESIAN_POINT('Ctrl Pts',(39.0484435371741,-22.4504611378278,
-100.39788649858));
#172647=CARTESIAN_POINT('Ctrl Pts',(39.0614304565616,-22.4467066621347,
-100.303758414252));
#172648=CARTESIAN_POINT('Ctrl Pts',(39.0773930576913,-22.4428095278211,
-100.206815225869));
#172649=CARTESIAN_POINT('Ctrl Pts',(39.09274066922,-22.439062538027,-100.113606958396));
#172650=CARTESIAN_POINT('Ctrl Pts',(39.1108399400955,-22.4351837761763,
-100.017799350643));
#172651=CARTESIAN_POINT('Ctrl Pts',(39.1320731933389,-22.4311775089901,
-99.9196156578223));
#172652=CARTESIAN_POINT('Ctrl Pts',(39.1369808481102,-22.4302515380122,
-99.8969224010233));
#172653=CARTESIAN_POINT('Ctrl Pts',(39.1420558181611,-22.4293187663864,
-99.8741024539549));
#172654=CARTESIAN_POINT('Ctrl Pts',(39.1473026139867,-22.4283792645213,
-99.8511589578541));
#172655=CARTESIAN_POINT('Ctrl Pts',(39.1477530888856,-22.4282986015755,
-99.8491890948312));
#172656=CARTESIAN_POINT('Ctrl Pts',(39.1485162523428,-22.4281623691545,
-99.8458628893345));
#172657=CARTESIAN_POINT('Ctrl Pts',(39.1486578411466,-22.4281371266263,
-99.8452466389702));
#172658=CARTESIAN_POINT('Ctrl Pts',(39.1486743781443,-22.4281341784015,
-99.8451746634286));
#172659=CARTESIAN_POINT('Ctrl Pts',(39.1486909425236,-22.4281312255307,
-99.8451025748626));
#172660=CARTESIAN_POINT('Ctrl Pts',(39.148707534297,-22.428128268014,-99.845030373276));
#172661=CARTESIAN_POINT('Ctrl Pts',(39.1518270689057,-22.4275722047527,
-99.8314552513122));
#172662=CARTESIAN_POINT('Ctrl Pts',(39.1559125612838,-22.4268517977281,
-99.8138813002624));
#172663=CARTESIAN_POINT('Ctrl Pts',(39.1610759072736,-22.4259667647546,
-99.7923348463416));
#172664=CARTESIAN_POINT('Ctrl Pts',(39.1662355138054,-22.42508237275,-99.7708039970424));
#172665=CARTESIAN_POINT('Ctrl Pts',(39.1724714900693,-22.4240335791768,
-99.7453061166653));
#172666=CARTESIAN_POINT('Ctrl Pts',(39.1799461680143,-22.4228199948629,
-99.7158789022736));
#172667=CARTESIAN_POINT('Ctrl Pts',(39.1867519047032,-22.4217150194578,
-99.6890852565657));
#172668=CARTESIAN_POINT('Ctrl Pts',(39.1945851963102,-22.4204734171491,
-99.6590340292539));
#172669=CARTESIAN_POINT('Ctrl Pts',(39.2036042917547,-22.4190949885092,
-99.6257653903841));
#172670=CARTESIAN_POINT('Ctrl Pts',(39.2134357504478,-22.4175924027657,
-99.5895001960708));
#172671=CARTESIAN_POINT('Ctrl Pts',(39.2246753006762,-22.415927280686,-99.5494129467876));
#172672=CARTESIAN_POINT('Ctrl Pts',(39.2375704699864,-22.4141000585316,
-99.5055833725206));
#172673=CARTESIAN_POINT('Ctrl Pts',(39.2501483362211,-22.4123177976487,
-99.4628322841872));
#172674=CARTESIAN_POINT('Ctrl Pts',(39.2643018106626,-22.4103812720758,
-99.4165198589484));
#172675=CARTESIAN_POINT('Ctrl Pts',(39.2803005761706,-22.4082917028185,
-99.3667489313563));
#172676=CARTESIAN_POINT('Ctrl Pts',(39.2900736410679,-22.4070152608362,
-99.3363456789858));
#172677=CARTESIAN_POINT('Ctrl Pts',(39.3005360632784,-22.4056817248198,
-99.3046524019425));
#172678=CARTESIAN_POINT('Ctrl Pts',(39.3117561762374,-22.4042915876652,
-99.2716991216448));
#172679=CARTESIAN_POINT('Ctrl Pts',(39.3152146560669,-22.4038630927537,
-99.2615416254019));
#172680=CARTESIAN_POINT('Ctrl Pts',(39.3187451592901,-22.4034292213711,
-99.2512644589312));
#172681=CARTESIAN_POINT('Ctrl Pts',(39.3223498480703,-22.4029895534928,
-99.2408686341921));
#172682=CARTESIAN_POINT('Ctrl Pts',(39.3241521924604,-22.4027697195536,
-99.2356707218225));
#172683=CARTESIAN_POINT('Ctrl Pts',(39.3259731076755,-22.4025482786348,
-99.2304431532566));
#172684=CARTESIAN_POINT('Ctrl Pts',(39.3278127975991,-22.4023256545837,
-99.2251860363515));
#172685=CARTESIAN_POINT('Ctrl Pts',(39.3296524875228,-22.4021030305325,
-99.2199289194463));
#172686=CARTESIAN_POINT('Ctrl Pts',(39.3319414859164,-22.401827635554,-99.2134232135355));
#172687=CARTESIAN_POINT('Ctrl Pts',(39.3333884566463,-22.401654256214,-99.209326170086));
#172688=CARTESIAN_POINT('Ctrl Pts',(39.3571412292357,-22.398808144714,-99.1420710837627));
#172689=CARTESIAN_POINT('Ctrl Pts',(39.3809074316803,-22.3961123131947,
-99.0787019928113));
#172690=CARTESIAN_POINT('Ctrl Pts',(39.4043137429003,-22.3935678599518,
-99.0191392615585));
#172691=CARTESIAN_POINT('Ctrl Pts',(39.4281732527221,-22.3909741403959,
-98.9584232624427));
#172692=CARTESIAN_POINT('Ctrl Pts',(39.4516587935485,-22.3885376879477,
-98.9016618018122));
#172693=CARTESIAN_POINT('Ctrl Pts',(39.4744264125052,-22.3862580561699,
-98.8487497482935));
#172694=CARTESIAN_POINT('Ctrl Pts',(39.4976916026771,-22.3839286045512,
-98.794681336931));
#172695=CARTESIAN_POINT('Ctrl Pts',(39.5202071163624,-22.3817628736423,
-98.7446317833894));
#172696=CARTESIAN_POINT('Ctrl Pts',(39.541659516076,-22.3797591779471,-98.6984773338181));
#172697=CARTESIAN_POINT('Ctrl Pts',(39.5589079809675,-22.378148137909,-98.6613675739008));
#172698=CARTESIAN_POINT('Ctrl Pts',(39.5754702335143,-22.3766418202078,
-98.6267755530437));
#172699=CARTESIAN_POINT('Ctrl Pts',(39.5912077081794,-22.3752389875185,
-98.5946357492765));
#172700=CARTESIAN_POINT('Ctrl Pts',(57.9716987024741,-21.98000002,-61.0621827299711));
#172701=CARTESIAN_POINT('Ctrl Pts',(57.5817506954796,-21.98000002,-60.8779152752782));
#172702=CARTESIAN_POINT('Ctrl Pts',(57.5245249214072,-22.4066238608121,
-60.8508735991008));
#172703=CARTESIAN_POINT('Ctrl Pts',(52.0201596782203,-21.98000002,-73.6568689967289));
#172704=CARTESIAN_POINT('Ctrl Pts',(51.6744341991619,-21.980000020072,-73.3940563428121));
#172705=CARTESIAN_POINT('Ctrl Pts',(51.5741970743562,-22.3992883743679,
-73.4455439799432));
#172706=CARTESIAN_POINT('Ctrl Pts',(46.0528581107812,-21.98000002,-86.2441334050211));
#172707=CARTESIAN_POINT('Ctrl Pts',(45.7509404552383,-21.98000002,-85.9093076925101));
#172708=CARTESIAN_POINT('Ctrl Pts',(45.6084483216386,-22.3901517945239,
-86.0327992211263));
#172709=CARTESIAN_POINT('Ctrl Pts',(40.032098818038,-21.98000002,-98.8059179211357));
#172710=CARTESIAN_POINT('Ctrl Pts',(39.6675936435968,-21.98000002,-98.6312136095384));
#172711=CARTESIAN_POINT('Ctrl Pts',(39.5912209089315,-22.3752378108182,
-98.5946087902654));
#172712=CARTESIAN_POINT('',(57.9716987024741,-21.98000002,-61.0621827299711));
#172713=CARTESIAN_POINT('Ctrl Pts',(57.9716987024741,-21.98000002,-61.0621827299711));
#172714=CARTESIAN_POINT('Ctrl Pts',(52.0201508381868,-21.98000002,-73.6568877040663));
#172715=CARTESIAN_POINT('Ctrl Pts',(46.0528675815424,-21.98000002,-86.2441136451113));
#172716=CARTESIAN_POINT('Ctrl Pts',(40.032098818038,-21.98000002,-98.8059179211357));
#172717=CARTESIAN_POINT('',(57.5245249214072,-22.4066238608121,-60.8508735991007));
#172718=CARTESIAN_POINT('Origin',(57.9716987024741,-22.48000002,-61.0621827299711));
#172719=CARTESIAN_POINT('Ctrl Pts',(39.5912209089345,-22.3752378108151,
-98.5946087902606));
#172720=CARTESIAN_POINT('Ctrl Pts',(40.9473935734796,-22.3785991491226,
-95.763407376981));
#172721=CARTESIAN_POINT('Ctrl Pts',(42.3747096804507,-22.3820178133902,
-92.7761193440102));
#172722=CARTESIAN_POINT('Ctrl Pts',(44.6224781400908,-22.3866023021413,
-88.061057365017));
#172723=CARTESIAN_POINT('Ctrl Pts',(45.389531418281,-22.3880535629714,-86.4503483837631));
#172724=CARTESIAN_POINT('Ctrl Pts',(46.5668026381736,-22.3901600190474,
-83.9757524294981));
#172725=CARTESIAN_POINT('Ctrl Pts',(47.1621109494658,-22.3911969294873,
-82.7238213317696));
#172726=CARTESIAN_POINT('Ctrl Pts',(47.8683124092611,-22.3924015844907,
-81.2376270900431));
#172727=CARTESIAN_POINT('Ctrl Pts',(48.2243315716556,-22.3930065987344,
-80.4881279789192));
#172728=CARTESIAN_POINT('Ctrl Pts',(48.4254131098423,-22.3933482630478,
-80.0647341691511));
#172729=CARTESIAN_POINT('Ctrl Pts',(48.5246188153984,-22.3935169090336,
-79.8558253309021));
#172730=CARTESIAN_POINT('Ctrl Pts',(48.5758868958006,-22.3936041070006,
-79.7478585128181));
#172731=CARTESIAN_POINT('Ctrl Pts',(48.5796195095595,-22.3936104557674,
-79.7399978701883));
#172732=CARTESIAN_POINT('Ctrl Pts',(51.3232477570397,-22.3982772069777,
-73.9620770724378));
#172733=CARTESIAN_POINT('Ctrl Pts',(54.3039844455626,-22.4026536205826,
-67.667581314042));
#172734=CARTESIAN_POINT('Ctrl Pts',(57.5245249214072,-22.4066238608121,
-60.8508735991007));
#172735=CARTESIAN_POINT('Ctrl Pts',(39.7614971661825,-28.0062467616585,
-94.6983380795177));
#172736=CARTESIAN_POINT('Ctrl Pts',(39.,-28.741729147553,-95.6677964063875));
#172737=CARTESIAN_POINT('Ctrl Pts',(39.,-29.6093496431988,-96.8114293882212));
#172738=CARTESIAN_POINT('Ctrl Pts',(39.7437819827477,-27.4973039569491,
-95.1199826758911));
#172739=CARTESIAN_POINT('Ctrl Pts',(39.,-28.2134674407351,-96.0912283932403));
#172740=CARTESIAN_POINT('Ctrl Pts',(39.,-29.0535677480794,-97.2330749436175));
#172741=CARTESIAN_POINT('Ctrl Pts',(39.7262969548998,-26.9800167700376,
-95.5308471039398));
#172742=CARTESIAN_POINT('Ctrl Pts',(39.,-27.6753857963049,-96.504280291422));
#172743=CARTESIAN_POINT('Ctrl Pts',(39.,-28.4877143439141,-97.6439384126816));
#172744=CARTESIAN_POINT('Ctrl Pts',(39.6919956601185,-25.9258412309992,
-96.3274629617598));
#172745=CARTESIAN_POINT('Ctrl Pts',(39.,-26.5774575077333,-97.3050952674327));
#172746=CARTESIAN_POINT('Ctrl Pts',(39.,-27.3325353334211,-98.4405542704251));
#172747=CARTESIAN_POINT('Ctrl Pts',(39.6751334260609,-25.3873798477126,
-96.7142461865699));
#172748=CARTESIAN_POINT('Ctrl Pts',(39.,-26.0159584590169,-97.6939770973016));
#172749=CARTESIAN_POINT('Ctrl Pts',(39.,-26.741479037393,-98.8273374953048));
#172750=CARTESIAN_POINT('Ctrl Pts',(39.6263764589698,-23.7517847228855,
-97.8205111744839));
#172751=CARTESIAN_POINT('Ctrl Pts',(39.,-24.3098005849941,-98.8051808316371));
#172752=CARTESIAN_POINT('Ctrl Pts',(39.,-24.9430461321624,-99.9336024831245));
#172753=CARTESIAN_POINT('Ctrl Pts',(39.5962627317006,-22.634454054442,-98.4870223585708));
#172754=CARTESIAN_POINT('Ctrl Pts',(38.9999999999805,-23.1402109105079,
-99.4757726121153));
#172755=CARTESIAN_POINT('Ctrl Pts',(39.,-23.7104174150638,-100.600117065969));
#172756=CARTESIAN_POINT('Ctrl Pts',(39.5698473334291,-21.4814334314007,
-99.0625227403511));
#172757=CARTESIAN_POINT('Ctrl Pts',(39.,-21.9292338920902,-100.055223222194));
#172758=CARTESIAN_POINT('Ctrl Pts',(39.,-22.4346346021703,-101.175614049055));
#172759=CARTESIAN_POINT('',(39.7602371815487,-27.9700232796676,-94.7283182583424));
#172760=CARTESIAN_POINT('Ctrl Pts',(39.760237187334,-27.9700232996177,-94.7283182916262));
#172761=CARTESIAN_POINT('Ctrl Pts',(39.7447508838319,-27.5244916807806,
-95.096692988375));
#172762=CARTESIAN_POINT('Ctrl Pts',(39.7297644606222,-27.0817800144324,
-95.4491475626341));
#172763=CARTESIAN_POINT('Ctrl Pts',(39.7152783970567,-26.6405416183526,
-95.7865386233445));
#172764=CARTESIAN_POINT('Ctrl Pts',(39.7132243273442,-26.5779756616797,
-95.8343794157002));
#172765=CARTESIAN_POINT('Ctrl Pts',(39.7111803019538,-26.5154393868985,
-95.8819173924144));
#172766=CARTESIAN_POINT('Ctrl Pts',(39.7091463075091,-26.4529290005184,
-95.9291550328498));
#172767=CARTESIAN_POINT('Ctrl Pts',(39.7021598335833,-26.2382149506942,
-96.0914094303885));
#172768=CARTESIAN_POINT('Ctrl Pts',(39.6952842340061,-26.0235489205403,
-96.2502889063942));
#172769=CARTESIAN_POINT('Ctrl Pts',(39.6885330384432,-25.809181245456,-96.4055817431426));
#172770=CARTESIAN_POINT('Ctrl Pts',(39.681431379786,-25.5836854734279,-96.5689360273148));
#172771=CARTESIAN_POINT('Ctrl Pts',(39.6744673646565,-25.3585197762647,
-96.7283219086833));
#172772=CARTESIAN_POINT('Ctrl Pts',(39.6676547428316,-25.1339280420678,
-96.8835265364444));
#172773=CARTESIAN_POINT('Ctrl Pts',(39.6647014284074,-25.0365661122239,
-96.9508087190838));
#172774=CARTESIAN_POINT('Ctrl Pts',(39.6617765415299,-24.939311468461,-97.0173055150268));
#172775=CARTESIAN_POINT('Ctrl Pts',(39.6588811036972,-24.8421814727703,
-97.0830011825413));
#172776=CARTESIAN_POINT('Ctrl Pts',(39.6476505823632,-24.4654438075899,
-97.3378146643689));
#172777=CARTESIAN_POINT('Ctrl Pts',(39.6368573959785,-24.0905821641491,
-97.5807135994866));
#172778=CARTESIAN_POINT('Ctrl Pts',(39.6265067297219,-23.7166730378311,
-97.8120922005714));
#172779=CARTESIAN_POINT('Ctrl Pts',(39.617412986147,-23.3881691878632,-98.0153735753937));
#172780=CARTESIAN_POINT('Ctrl Pts',(39.6086607036092,-23.060400896105,-98.2097630572075));
#172781=CARTESIAN_POINT('Ctrl Pts',(39.6002528798929,-22.7327299685291,
-98.3954874204445));
#172782=CARTESIAN_POINT('Ctrl Pts',(39.597195434678,-22.6135747693504,-98.4630247624282));
#172783=CARTESIAN_POINT('Ctrl Pts',(39.5941835411059,-22.4944322994311,
-98.5294158133307));
#172784=CARTESIAN_POINT('Ctrl Pts',(39.5912173600348,-22.3752713037914,
-98.5946697908291));
#172785=CARTESIAN_POINT('Ctrl Pts',(39.7602371793877,-27.9700232590251,
-94.7283182583078));
#172786=CARTESIAN_POINT('Ctrl Pts',(39.721173342089,-27.9739864535911,-94.8036965512742));
#172787=CARTESIAN_POINT('Ctrl Pts',(39.6812588478966,-27.9782127469329,
-94.8842699537839));
#172788=CARTESIAN_POINT('Ctrl Pts',(39.6410880301102,-27.9827071593153,
-94.9702238054998));
#172789=CARTESIAN_POINT('Ctrl Pts',(39.6256104639824,-27.9844388284395,
-95.0033412897129));
#172790=CARTESIAN_POINT('Ctrl Pts',(39.6100953866432,-27.9862102988464,
-95.0372576699903));
#172791=CARTESIAN_POINT('Ctrl Pts',(39.5945787380208,-27.9880218495183,
-95.0719841268097));
#172792=CARTESIAN_POINT('Ctrl Pts',(39.5666842850881,-27.9912784944409,
-95.1344122669862));
#172793=CARTESIAN_POINT('Ctrl Pts',(39.5387859048961,-27.9946645037012,
-95.1994551025455));
#172794=CARTESIAN_POINT('Ctrl Pts',(39.5111086085599,-27.9981802158359,
-95.2671566087482));
#172795=CARTESIAN_POINT('Ctrl Pts',(39.4972699603918,-27.9999380719032,
-95.3010073618496));
#172796=CARTESIAN_POINT('Ctrl Pts',(39.4834868072858,-28.001728337867,-95.3355225476929));
#172797=CARTESIAN_POINT('Ctrl Pts',(39.4697884556866,-28.0035509529382,
-95.3707060919163));
#172798=CARTESIAN_POINT('Ctrl Pts',(39.462939279887,-28.0044622604738,-95.388297864028));
#172799=CARTESIAN_POINT('Ctrl Pts',(39.456111308277,-28.0053816551031,-95.406056726538));
#172800=CARTESIAN_POINT('Ctrl Pts',(39.449308271849,-28.0063091210918,-95.4239830388244));
#172801=CARTESIAN_POINT('Ctrl Pts',(39.445906753635,-28.0067728540861,-95.4329461949676));
#172802=CARTESIAN_POINT('Ctrl Pts',(39.4425114693047,-28.0072386049083,
-95.441951213587));
#172803=CARTESIAN_POINT('Ctrl Pts',(39.4391228871938,-28.0077063712997,
-95.4509981355552));
#172804=CARTESIAN_POINT('Ctrl Pts',(39.4374285961383,-28.0079402544954,
-95.4555215965394));
#172805=CARTESIAN_POINT('Ctrl Pts',(39.4357359806405,-28.0081746415827,
-95.460055533362));
#172806=CARTESIAN_POINT('Ctrl Pts',(39.4340450994288,-28.0084095322498,
-95.4645999506646));
#172807=CARTESIAN_POINT('Ctrl Pts',(39.433199658823,-28.0085269775834,-95.4668721593159));
#172808=CARTESIAN_POINT('Ctrl Pts',(39.4323546517888,-28.0086445488119,
-95.4691469880873));
#172809=CARTESIAN_POINT('Ctrl Pts',(39.431510085679,-28.0087622458945,-95.4714244375276));
#172810=CARTESIAN_POINT('Ctrl Pts',(39.4306655195692,-28.008879942977,-95.4737018869679));
#172811=CARTESIAN_POINT('Ctrl Pts',(39.4291050611265,-28.0090979116105,
-95.4779201015231));
#172812=CARTESIAN_POINT('Ctrl Pts',(39.4289777174792,-28.0091157146626,
-95.4782646483947));
#172813=CARTESIAN_POINT('Ctrl Pts',(39.426693894066,-28.0094350005327,-95.4844438668219));
#172814=CARTESIAN_POINT('Ctrl Pts',(39.4228824393387,-28.0099686170733,
-95.4947718201092));
#172815=CARTESIAN_POINT('Ctrl Pts',(39.4176054119079,-28.0107171614978,
-95.5092693092406));
#172816=CARTESIAN_POINT('Ctrl Pts',(39.412306317478,-28.0114688361181,-95.5238274226692));
#172817=CARTESIAN_POINT('Ctrl Pts',(39.4055293860221,-28.0124372416699,
-95.5425900228496));
#172818=CARTESIAN_POINT('Ctrl Pts',(39.3973879849454,-28.0136233734704,
-95.5655935175528));
#172819=CARTESIAN_POINT('Ctrl Pts',(39.3891953935039,-28.0148169632648,
-95.5887416504178));
#172820=CARTESIAN_POINT('Ctrl Pts',(39.3796211568778,-28.0162310288329,
-95.6161841886283));
#172821=CARTESIAN_POINT('Ctrl Pts',(39.3688314625449,-28.0178669439296,
-95.6479736028182));
#172822=CARTESIAN_POINT('Ctrl Pts',(39.358671911494,-28.0194073177739,-95.6779064411708));
#172823=CARTESIAN_POINT('Ctrl Pts',(39.3474346778275,-28.0211444822674,
-95.7116951824943));
#172824=CARTESIAN_POINT('Ctrl Pts',(39.3353005090293,-28.0230794904341,
-95.7493891119716));
#172825=CARTESIAN_POINT('Ctrl Pts',(39.3220949453622,-28.025185351492,-95.7904112531542));
#172826=CARTESIAN_POINT('Ctrl Pts',(39.307827638871,-28.0275253887629,-95.8360556009816));
#172827=CARTESIAN_POINT('Ctrl Pts',(39.2927843742968,-28.0301004647007,
-95.8863862017628));
#172828=CARTESIAN_POINT('Ctrl Pts',(39.2775020102043,-28.0327164692158,
-95.9375167633733));
#172829=CARTESIAN_POINT('Ctrl Pts',(39.2614179145521,-28.035575275758,-95.9934882030578));
#172830=CARTESIAN_POINT('Ctrl Pts',(39.2448872805952,-28.0386765911129,
-96.0543562552077));
#172831=CARTESIAN_POINT('Ctrl Pts',(39.2287363134251,-28.0417066771102,
-96.1138263223896));
#172832=CARTESIAN_POINT('Ctrl Pts',(39.2121593315286,-28.0449683682601,
-96.1779727979824));
#172833=CARTESIAN_POINT('Ctrl Pts',(39.1955312387891,-28.0484600623225,
-96.2468332932256));
#172834=CARTESIAN_POINT('Ctrl Pts',(39.1946291423112,-28.048649491439,-96.2505690680494));
#172835=CARTESIAN_POINT('Ctrl Pts',(39.1934506554151,-28.0488980061046,
-96.255470935905));
#172836=CARTESIAN_POINT('Ctrl Pts',(39.1928245891292,-28.0490303797397,
-96.2580822296316));
#172837=CARTESIAN_POINT('Ctrl Pts',(39.1927284851265,-28.0490506996906,
-96.2584830750132));
#172838=CARTESIAN_POINT('Ctrl Pts',(39.1926324279919,-28.0490710181889,
-96.25888387789));
#172839=CARTESIAN_POINT('Ctrl Pts',(39.1925364176938,-28.0490913352319,
-96.2592846382602));
#172840=CARTESIAN_POINT('Ctrl Pts',(39.1705544952503,-28.0537429994074,
-96.3510402473537));
#172841=CARTESIAN_POINT('Ctrl Pts',(39.1510615013283,-28.0583237172308,
-96.4406840483798));
#172842=CARTESIAN_POINT('Ctrl Pts',(39.1337484254094,-28.0627975236857,
-96.528086779579));
#172843=CARTESIAN_POINT('Ctrl Pts',(39.1196099345289,-28.0664509976298,
-96.5994630459213));
#172844=CARTESIAN_POINT('Ctrl Pts',(39.1069256168401,-28.0700332425997,
-96.6693458907162));
#172845=CARTESIAN_POINT('Ctrl Pts',(39.095537681765,-28.0735262649617,-96.7376882535311));
#172846=CARTESIAN_POINT('Ctrl Pts',(39.0802857711333,-28.078204484898,-96.8292194752271));
#172847=CARTESIAN_POINT('Ctrl Pts',(39.0673590162165,-28.0827242117545,
-96.9179853660842));
#172848=CARTESIAN_POINT('Ctrl Pts',(39.0564122238475,-28.0870466384659,
-97.0038380129319));
#172849=CARTESIAN_POINT('Ctrl Pts',(39.0491330840064,-28.0899208638486,
-97.0609262814465));
#172850=CARTESIAN_POINT('Ctrl Pts',(39.0427297849026,-28.0927079320018,
-97.1167275272839));
#172851=CARTESIAN_POINT('Ctrl Pts',(39.0371055462776,-28.0953973309735,
-97.171209960409));
#172852=CARTESIAN_POINT('Ctrl Pts',(39.028325243207,-28.0995958971482,-97.2562654331141));
#172853=CARTESIAN_POINT('Ctrl Pts',(39.0214375200278,-28.1035689840776,
-97.3381388769938));
#172854=CARTESIAN_POINT('Ctrl Pts',(39.0160961336416,-28.1073516111888,
-97.4167589491541));
#172855=CARTESIAN_POINT('Ctrl Pts',(39.0106007252515,-28.1112433125676,
-97.4976460771276));
#172856=CARTESIAN_POINT('Ctrl Pts',(39.0067420005837,-28.1149334424741,
-97.5750899904949));
#172857=CARTESIAN_POINT('Ctrl Pts',(39.0041777909439,-28.1184604696338,
-97.6490565225246));
#172858=CARTESIAN_POINT('Ctrl Pts',(39.0015182173996,-28.1221186682375,
-97.7257738972244));
#172859=CARTESIAN_POINT('Ctrl Pts',(39.0002510559389,-28.1256014236328,
-97.7987508895155));
#172860=CARTESIAN_POINT('Ctrl Pts',(39.000033928547,-28.128951635191,-97.8679882137764));
#172861=CARTESIAN_POINT('Ctrl Pts',(39.0000111867388,-28.1293025345779,
-97.8752400945046));
#172862=CARTESIAN_POINT('Ctrl Pts',(39.,-28.1296519797826,-97.8824509799334));
#172863=CARTESIAN_POINT('Ctrl Pts',(39.,-28.1300000200001,-97.8896208912436));
#172864=CARTESIAN_POINT('Ctrl Pts',(39.7602371906926,-27.9700232578782,
-94.7283182364936));
#172865=CARTESIAN_POINT('Ctrl Pts',(39.5607615517246,-28.6300000199999,
-94.628899882694));
#172866=CARTESIAN_POINT('Ctrl Pts',(40.1842134716234,-28.63000002,-94.9396273673639));
#172867=CARTESIAN_POINT('Ctrl Pts',(39.5060135610296,-27.995815206986,-95.2188728854821));
#172868=CARTESIAN_POINT('Ctrl Pts',(39.3499072921674,-28.63000002,-95.1384098881608));
#172869=CARTESIAN_POINT('Ctrl Pts',(39.9554048343097,-28.63000002,-95.3987151357952));
#172870=CARTESIAN_POINT('Ctrl Pts',(39.3193354149279,-28.0222617282467,
-95.7300059572715));
#172871=CARTESIAN_POINT('Ctrl Pts',(39.1953130903143,-28.63000002,-95.6752490593844));
#172872=CARTESIAN_POINT('Ctrl Pts',(39.7874018733942,-28.63000002,-95.8764151880824));
#172873=CARTESIAN_POINT('Ctrl Pts',(39.0657374218185,-28.0759209337118,
-96.7885633195629));
#172874=CARTESIAN_POINT('Ctrl Pts',(39.0100660589831,-28.63000002,-96.7655348922061));
#172875=CARTESIAN_POINT('Ctrl Pts',(39.5591636796777,-28.63000002,-96.8642956936284));
#172876=CARTESIAN_POINT('Ctrl Pts',(39.,-28.1033206002549,-97.3400031641594));
#172877=CARTESIAN_POINT('Ctrl Pts',(38.9725899744442,-28.63000002,-97.3249520920672));
#172878=CARTESIAN_POINT('Ctrl Pts',(39.500000000016,-28.63000002,-97.3781967454117));
#172879=CARTESIAN_POINT('Ctrl Pts',(39.,-28.13000002,-97.8896208912436));
#172880=CARTESIAN_POINT('Ctrl Pts',(39.,-28.63000002,-97.8896208912435));
#172881=CARTESIAN_POINT('Ctrl Pts',(39.5,-28.63000002,-97.8896208912436));
#172882=CARTESIAN_POINT('',(39.5,-28.63000002,-97.8896208912436));
#172883=CARTESIAN_POINT('Origin',(39.5,-28.13000002,-97.8896208912436));
#172884=CARTESIAN_POINT('',(40.1842134716234,-28.63000002,-94.9396273673639));
#172885=CARTESIAN_POINT('Origin',(40.1842134716234,-28.13000002,-94.9396273673639));
#172886=CARTESIAN_POINT('Ctrl Pts',(39.5,-28.63000002,-97.8896208912436));
#172887=CARTESIAN_POINT('Ctrl Pts',(39.5,-28.63000002,-97.7089321417025));
#172888=CARTESIAN_POINT('Ctrl Pts',(39.50738071193,-28.63000002,-97.5282244682254));
#172889=CARTESIAN_POINT('Ctrl Pts',(39.5219120167722,-28.63000002,-97.3483295034422));
#172890=CARTESIAN_POINT('Ctrl Pts',(39.5366966813149,-28.63000002,-97.1652979907098));
#172891=CARTESIAN_POINT('Ctrl Pts',(39.5588835421168,-28.63000002,-96.9831066045011));
#172892=CARTESIAN_POINT('Ctrl Pts',(39.5882836977189,-28.63000002,-96.8026267328142));
#172893=CARTESIAN_POINT('Ctrl Pts',(39.6119618388167,-28.63000002,-96.6572728127554));
#172894=CARTESIAN_POINT('Ctrl Pts',(39.6403197974462,-28.63000002,-96.5130286888779));
#172895=CARTESIAN_POINT('Ctrl Pts',(39.6732827765156,-28.63000002,-96.3703554408507));
#172896=CARTESIAN_POINT('Ctrl Pts',(39.7499154654027,-28.63000002,-96.0386671366604));
#172897=CARTESIAN_POINT('Ctrl Pts',(39.8508333618868,-28.63000002,-95.7143394136881));
#172898=CARTESIAN_POINT('Ctrl Pts',(39.9781561959403,-28.63000002,-95.3980147135159));
#172899=CARTESIAN_POINT('Ctrl Pts',(40.0404386993088,-28.63000002,-95.2432781782316));
#172900=CARTESIAN_POINT('Ctrl Pts',(40.1090402739364,-28.63000002,-95.0904568779001));
#172901=CARTESIAN_POINT('Ctrl Pts',(40.1842134716234,-28.63000002,-94.9396273673639));
#172902=CARTESIAN_POINT('Origin',(39.5,-28.13000002,-55.24995));
#172903=CARTESIAN_POINT('',(39.5,-28.63000002,-134.169022080262));
#172904=CARTESIAN_POINT('Origin',(39.5,-28.13000002,-134.169022080262));
#172905=CARTESIAN_POINT('',(39.5,-28.63000002,-55.24995));
#172906=CARTESIAN_POINT('Ctrl Pts',(39.,-28.13000002,-134.169022080262));
#172907=CARTESIAN_POINT('Ctrl Pts',(39.,-28.63000002,-134.169022080263));
#172908=CARTESIAN_POINT('Ctrl Pts',(39.5,-28.63000002,-134.169022080262));
#172909=CARTESIAN_POINT('Ctrl Pts',(39.,-28.1032444606982,-134.720208320017));
#172910=CARTESIAN_POINT('Ctrl Pts',(38.9725065924499,-28.63000002,-134.735408648257));
#172911=CARTESIAN_POINT('Ctrl Pts',(39.500000002646,-28.63000002,-134.681913680777));
#172912=CARTESIAN_POINT('Ctrl Pts',(39.0642137165569,-28.076417661445,-135.260142317137));
#172913=CARTESIAN_POINT('Ctrl Pts',(39.0091060618314,-28.6300000199999,
-135.282961361938));
#172914=CARTESIAN_POINT('Ctrl Pts',(39.5577923442835,-28.63000002,-135.185082649765));
#172915=CARTESIAN_POINT('Ctrl Pts',(39.3159560341664,-28.0228058044255,
-136.318039323049));
#172916=CARTESIAN_POINT('Ctrl Pts',(39.1926311399543,-28.63000002,-136.37231025087));
#172917=CARTESIAN_POINT('Ctrl Pts',(39.7843604313674,-28.63000002,-136.172328627912));
#172918=CARTESIAN_POINT('Ctrl Pts',(39.5060247583741,-27.995814073424,-136.839791694484));
#172919=CARTESIAN_POINT('Ctrl Pts',(39.3499007457719,-28.63000002,-136.920217264961));
#172920=CARTESIAN_POINT('Ctrl Pts',(39.9554204749436,-28.63000002,-136.659959223536));
#172921=CARTESIAN_POINT('Ctrl Pts',(39.7602371906926,-27.9700232578782,
-137.330324735012));
#172922=CARTESIAN_POINT('Ctrl Pts',(39.5607615517247,-28.63000002,-137.429743088812));
#172923=CARTESIAN_POINT('Ctrl Pts',(40.1842134716234,-28.63000002,-137.119015604142));
#172924=CARTESIAN_POINT('',(40.1842134716234,-28.63000002,-137.119015604142));
#172925=CARTESIAN_POINT('Ctrl Pts',(40.1842134716234,-28.63000002,-137.119015604142));
#172926=CARTESIAN_POINT('Ctrl Pts',(40.0632593004047,-28.63000002,-136.87632992622));
#172927=CARTESIAN_POINT('Ctrl Pts',(39.9584937855372,-28.63000002,-136.62577590122));
#172928=CARTESIAN_POINT('Ctrl Pts',(39.8698562579301,-28.63000002,-136.370603923319));
#172929=CARTESIAN_POINT('Ctrl Pts',(39.790754739042,-28.63000002,-136.142884450827));
#172930=CARTESIAN_POINT('Ctrl Pts',(39.7244982953545,-28.63000002,-135.91148583538));
#172931=CARTESIAN_POINT('Ctrl Pts',(39.6710763875084,-28.63000002,-135.678705638911));
#172932=CARTESIAN_POINT('Ctrl Pts',(39.5896852679394,-28.63000002,-135.324052621675));
#172933=CARTESIAN_POINT('Ctrl Pts',(39.5369428910349,-28.63000002,-134.964508495217));
#172934=CARTESIAN_POINT('Ctrl Pts',(39.5136924175149,-28.63000002,-134.599929291455));
#172935=CARTESIAN_POINT('Ctrl Pts',(39.5045817727589,-28.63000002,-134.457069766118));
#172936=CARTESIAN_POINT('Ctrl Pts',(39.5,-28.63000002,-134.313437038192));
#172937=CARTESIAN_POINT('Ctrl Pts',(39.5,-28.63000002,-134.169022080262));
#172938=CARTESIAN_POINT('Origin',(40.1842134716235,-28.13000002,-137.119015604142));
#172939=CARTESIAN_POINT('Ctrl Pts',(56.8814116147779,-28.63000002,-171.255207540975));
#172940=CARTESIAN_POINT('Ctrl Pts',(56.3101888392034,-28.6300000199993,
-171.530874113378));
#172941=CARTESIAN_POINT('Ctrl Pts',(56.4435504331081,-28.0132665904809,
-171.466515117848));
#172942=CARTESIAN_POINT('Ctrl Pts',(54.1272610644231,-28.63000002,-165.548193876387));
#172943=CARTESIAN_POINT('Ctrl Pts',(53.5308515392379,-28.6300000202216,
-165.788070495429));
#172944=CARTESIAN_POINT('Ctrl Pts',(53.6908080796597,-28.0079900448831,
-165.759504469858));
#172945=CARTESIAN_POINT('Ctrl Pts',(51.3626815512523,-28.63000002,-159.846279798555));
#172946=CARTESIAN_POINT('Ctrl Pts',(50.7518430064623,-28.63000002,-160.075814652758));
#172947=CARTESIAN_POINT('Ctrl Pts',(50.9279125759463,-28.0020195102152,
-160.05758849772));
#172948=CARTESIAN_POINT('Ctrl Pts',(45.8000159539871,-28.63000002,-148.458842597754));
#172949=CARTESIAN_POINT('Ctrl Pts',(45.1718093453638,-28.63000002,-148.698490742611));
#172950=CARTESIAN_POINT('Ctrl Pts',(45.3696439177297,-27.9879328369328,
-148.670151070157));
#172951=CARTESIAN_POINT('Ctrl Pts',(43.002293156202,-28.63000002,-142.773138192163));
#172952=CARTESIAN_POINT('Ctrl Pts',(42.350918422607,-28.6300000199999,-142.994193600403));
#172953=CARTESIAN_POINT('Ctrl Pts',(42.5746173757444,-27.9798324917395,
-142.984453134689));
#172954=CARTESIAN_POINT('Ctrl Pts',(40.1755504430153,-28.63000002,-137.101634098975));
#172955=CARTESIAN_POINT('Ctrl Pts',(39.552039110073,-28.63000002,-137.412399462834));
#172956=CARTESIAN_POINT('Ctrl Pts',(39.7515900663067,-27.9699781154354,
-137.31294095905));
#172957=CARTESIAN_POINT('',(56.8729709358987,-28.63000002,-171.237717270032));
#172958=CARTESIAN_POINT('Ctrl Pts',(56.8729709358987,-28.63000002,-171.237717270032));
#172959=CARTESIAN_POINT('Ctrl Pts',(54.1216123272523,-28.63000002,-165.536543461238));
#172960=CARTESIAN_POINT('Ctrl Pts',(51.3598402340142,-28.63000002,-159.840463284682));
#172961=CARTESIAN_POINT('Ctrl Pts',(48.5813487526192,-28.63000002,-154.152561198155));
#172962=CARTESIAN_POINT('Ctrl Pts',(45.8028572712242,-28.63000002,-148.464659111628));
#172963=CARTESIAN_POINT('Ctrl Pts',(43.0080103715946,-28.63000002,-142.784757083568));
#172964=CARTESIAN_POINT('Ctrl Pts',(40.1842134716234,-28.63000002,-137.119015604142));
#172965=CARTESIAN_POINT('Origin',(56.8729709358987,-28.13000002,-171.237717270032));
#172966=CARTESIAN_POINT('Ctrl Pts',(57.017028950725,-28.6300000098418,-171.937510237498));
#172967=CARTESIAN_POINT('Ctrl Pts',(56.3674234002834,-28.6301310958619,
-171.9078715334));
#172968=CARTESIAN_POINT('Ctrl Pts',(56.5341822214496,-28.0016231613287,
-171.915549358366));
#172969=CARTESIAN_POINT('Ctrl Pts',(57.0288581213358,-28.6300000098265,
-171.673675468004));
#172970=CARTESIAN_POINT('Ctrl Pts',(56.3722793953451,-28.6301314641988,
-171.762633256231));
#172971=CARTESIAN_POINT('Ctrl Pts',(56.5423215389878,-28.0006714526254,
-171.739685194435));
#172972=CARTESIAN_POINT('Ctrl Pts',(56.9695606031425,-28.6300000099035,
-171.413737441436));
#172973=CARTESIAN_POINT('Ctrl Pts',(56.3485431365402,-28.6301296243106,
-171.621528645649));
#172974=CARTESIAN_POINT('Ctrl Pts',(56.5015214234675,-28.0054385079109,
-171.56638157453));
#172975=CARTESIAN_POINT('Ctrl Pts',(56.8427717751314,-28.6300000100697,
-171.178320644756));
#172976=CARTESIAN_POINT('Ctrl Pts',(56.2873571642799,-28.6301257916421,
-171.477955081174));
#172977=CARTESIAN_POINT('Ctrl Pts',(56.4142663415167,-28.0157208016423,
-171.409463522487));
#172978=CARTESIAN_POINT('',(57.0184057454332,-28.63000002,-171.871644662643));
#172979=CARTESIAN_POINT('Origin',(55.5771425537374,-28.6300004042113,-171.848433761036));
#172980=CARTESIAN_POINT('Origin',(57.0184057454332,-28.13000002,-171.871644662643));
#172981=CARTESIAN_POINT('Origin',(57.0184057454332,-28.13000002,-179.64995));
#172982=CARTESIAN_POINT('',(57.0184057454332,-28.63000002,-171.871644662643));
#172983=CARTESIAN_POINT('',(56.5351989170821,-28.0015042572884,-179.64995));
#172984=CARTESIAN_POINT('Origin',(57.,-29.13000002,-174.34995));
#172985=CARTESIAN_POINT('',(59.5,-28.63000002,-174.34995));
#172986=CARTESIAN_POINT('Origin',(57.,-28.63000002,-174.34995));
#172987=CARTESIAN_POINT('Origin',(59.5,-29.13000002,-174.34995));
#172988=CARTESIAN_POINT('Origin',(59.5,-29.13000002,-55.24995));
#172989=CARTESIAN_POINT('',(59.5,-28.63000002,-58.24995));
#172990=CARTESIAN_POINT('',(59.5,-28.63000002,-174.34995));
#172991=CARTESIAN_POINT('Origin',(59.5,-29.13000002,-58.24995));
#172992=CARTESIAN_POINT('Ctrl Pts',(40.1842134716234,-28.63000002,-94.9396273673639));
#172993=CARTESIAN_POINT('Ctrl Pts',(39.5607615517246,-28.6300000199999,
-94.628899882694));
#172994=CARTESIAN_POINT('Ctrl Pts',(39.7602371906926,-27.9700232578782,
-94.7283182364936));
#172995=CARTESIAN_POINT('Ctrl Pts',(42.9880924510224,-28.63000002,-89.3138497353063));
#172996=CARTESIAN_POINT('Ctrl Pts',(42.3373257946448,-28.63000002,-89.0914456452771));
#172997=CARTESIAN_POINT('Ctrl Pts',(42.5604321400969,-27.9797945689722,
-89.1025347299149));
#172998=CARTESIAN_POINT('Ctrl Pts',(45.7634210292322,-28.63000002,-83.6741003095587));
#172999=CARTESIAN_POINT('Ctrl Pts',(45.1354691768678,-28.630000020022,-83.4336169877673));
#173000=CARTESIAN_POINT('Ctrl Pts',(45.3330806261701,-27.9878402480233,
-83.4627911786917));
#173001=CARTESIAN_POINT('Ctrl Pts',(51.2816902902029,-28.63000002,-72.3787631830378));
#173002=CARTESIAN_POINT('Ctrl Pts',(50.6710028559025,-28.6300000199784,
-72.148355955617));
#173003=CARTESIAN_POINT('Ctrl Pts',(50.8469740031289,-28.0018438144725,
-72.1674540521641));
#173004=CARTESIAN_POINT('Ctrl Pts',(54.0242786911866,-28.63000002,-66.7229996739341));
#173005=CARTESIAN_POINT('Ctrl Pts',(53.4278489247074,-28.6300000200659,
-66.4825194498726));
#173006=CARTESIAN_POINT('Ctrl Pts',(53.5878832423525,-28.0077864042225,
-66.5116884426403));
#173007=CARTESIAN_POINT('Ctrl Pts',(56.7565335485771,-28.63000002,-61.0621827299711));
#173008=CARTESIAN_POINT('Ctrl Pts',(56.1850547298497,-28.63000002,-60.7863522634768));
#173009=CARTESIAN_POINT('Ctrl Pts',(56.3187331343194,-28.0130417005584,
-60.8508735991007));
#173010=CARTESIAN_POINT('',(56.3187331343194,-28.0130417005584,-60.8508735991007));
#173011=CARTESIAN_POINT('Ctrl Pts',(56.3187331343194,-28.0130417005584,
-60.8508735991007));
#173012=CARTESIAN_POINT('Ctrl Pts',(55.4206729151416,-28.0113134574357,
-62.7124744999959));
#173013=CARTESIAN_POINT('Ctrl Pts',(54.5407043741536,-28.0095946269229,
-64.5337352621368));
#173014=CARTESIAN_POINT('Ctrl Pts',(53.6787898395932,-28.0078255152441,
-66.3146356201485));
#173015=CARTESIAN_POINT('Ctrl Pts',(53.1318515029365,-28.0067029039408,
-67.4447275730113));
#173016=CARTESIAN_POINT('Ctrl Pts',(52.5921839629517,-28.0055600958576,
-68.5585681337777));
#173017=CARTESIAN_POINT('Ctrl Pts',(52.0597872155532,-28.0043823157945,
-69.6561569895613));
#173018=CARTESIAN_POINT('Ctrl Pts',(51.3740895455159,-28.0028653999812,
-71.0697909472201));
#173019=CARTESIAN_POINT('Ctrl Pts',(50.7004503528809,-28.0012983267211,
-72.4564656700406));
#173020=CARTESIAN_POINT('Ctrl Pts',(50.0388732398342,-27.9996975550347,
-73.8161848482626));
#173021=CARTESIAN_POINT('Ctrl Pts',(49.7080846833108,-27.9988971691915,
-74.4960444373736));
#173022=CARTESIAN_POINT('Ctrl Pts',(49.3803117753967,-27.9980888638163,
-75.1691652377898));
#173023=CARTESIAN_POINT('Ctrl Pts',(49.055555577712,-27.9972777309138,-75.8355482397257));
#173024=CARTESIAN_POINT('Ctrl Pts',(48.8931774788696,-27.9968721644625,
-76.1687397406936));
#173025=CARTESIAN_POINT('Ctrl Pts',(48.7315535703334,-27.9964658957672,
-76.5002467983552));
#173026=CARTESIAN_POINT('Ctrl Pts',(48.5706840017103,-27.996059781108,-76.8300695637573));
#173027=CARTESIAN_POINT('Ctrl Pts',(48.4902492173988,-27.9958567237784,
-76.9949809464584));
#173028=CARTESIAN_POINT('Ctrl Pts',(48.410003018773,-27.9956537052356,-77.1594712564479));
#173029=CARTESIAN_POINT('Ctrl Pts',(48.3299454270974,-27.9954508395193,
-77.3235405144964));
#173030=CARTESIAN_POINT('Ctrl Pts',(48.2899166312597,-27.9953494066612,
-77.4055751435206));
#173031=CARTESIAN_POINT('Ctrl Pts',(48.2499349872017,-27.9952480120268,
-77.4875045095808));
#173032=CARTESIAN_POINT('Ctrl Pts',(48.210000497641,-27.9951466706255,-77.569328615371));
#173033=CARTESIAN_POINT('Ctrl Pts',(48.1750578192753,-27.9950579968994,
-77.6409247079375));
#173034=CARTESIAN_POINT('Ctrl Pts',(48.1401512435743,-27.9949693639309,
-77.7124402106111));
#173035=CARTESIAN_POINT('Ctrl Pts',(48.1052807723934,-27.994880782046,-77.7838751252387));
#173036=CARTESIAN_POINT('Ctrl Pts',(48.1002992765105,-27.9948681274911,
-77.7940801130427));
#173037=CARTESIAN_POINT('Ctrl Pts',(48.0962023871856,-27.9948577195745,
-77.8024728272216));
#173038=CARTESIAN_POINT('Ctrl Pts',(48.0903384937855,-27.9948428272692,
-77.8144851539887));
#173039=CARTESIAN_POINT('Ctrl Pts',(48.0902347666554,-27.9948425638374,
-77.8146976415112));
#173040=CARTESIAN_POINT('Ctrl Pts',(48.0901310397955,-27.9948423004048,
-77.8149101284225));
#173041=CARTESIAN_POINT('Ctrl Pts',(48.0900273132056,-27.9948420369715,
-77.8151226147225));
#173042=CARTESIAN_POINT('Ctrl Pts',(47.3394787984715,-27.9929358768115,
-79.3526384730988));
#173043=CARTESIAN_POINT('Ctrl Pts',(46.6030922990866,-27.9909910456638,
-80.8581611087631));
#173044=CARTESIAN_POINT('Ctrl Pts',(45.8807954360895,-27.9890047060169,
-82.3316567645428));
#173045=CARTESIAN_POINT('Ctrl Pts',(45.1431757263836,-27.9869762280479,
-83.8364112409215));
#173046=CARTESIAN_POINT('Ctrl Pts',(44.4202500280405,-27.9849044756312,
-85.3077656006454));
#173047=CARTESIAN_POINT('Ctrl Pts',(43.7119916769706,-27.9827892726554,
-86.7457096119736));
#173048=CARTESIAN_POINT('Ctrl Pts',(42.9722991493508,-27.9805801919813,
-88.2474729709351));
#173049=CARTESIAN_POINT('Ctrl Pts',(42.2486049085613,-27.9783237247899,
-89.7127945630624));
#173050=CARTESIAN_POINT('Ctrl Pts',(41.5409305949263,-27.9760225982136,
-91.1416892705798));
#173051=CARTESIAN_POINT('Ctrl Pts',(40.9356314794565,-27.9740543624667,
-92.3638739477615));
#173052=CARTESIAN_POINT('Ctrl Pts',(40.3420535665444,-27.972053512525,-93.5594092747014));
#173053=CARTESIAN_POINT('Ctrl Pts',(39.7602371906927,-27.9700232578782,
-94.7283182364936));
#173054=CARTESIAN_POINT('',(56.7565335485771,-28.63000002,-61.0621827299711));
#173055=CARTESIAN_POINT('Origin',(56.7565335485771,-28.13000002,-61.0621827299711));
#173056=CARTESIAN_POINT('Ctrl Pts',(40.1842134716234,-28.63000002,-94.9396273673639));
#173057=CARTESIAN_POINT('Ctrl Pts',(42.9880935290232,-28.63000002,-89.3138475723767));
#173058=CARTESIAN_POINT('Ctrl Pts',(45.7634210292107,-28.63000002,-83.6741003095903));
#173059=CARTESIAN_POINT('Ctrl Pts',(48.5225556597151,-28.63000002,-78.0264317462971));
#173060=CARTESIAN_POINT('Ctrl Pts',(51.2816902902195,-28.63000002,-72.3787631830038));
#173061=CARTESIAN_POINT('Ctrl Pts',(54.0242783838037,-28.63000002,-66.7230003106817));
#173062=CARTESIAN_POINT('Ctrl Pts',(56.7565335485771,-28.63000002,-61.0621827299711));
#173063=CARTESIAN_POINT('Origin',(57.,-29.13000002,-58.24995));
#173064=CARTESIAN_POINT('',(57.,-28.63000002,-55.74995));
#173065=CARTESIAN_POINT('Origin',(57.,-28.63000002,-58.24995));
#173066=CARTESIAN_POINT('',(57.,-29.13000002,-55.24995));
#173067=CARTESIAN_POINT('Origin',(57.,-29.13000002,-55.74995));
#173068=CARTESIAN_POINT('Origin',(57.,-29.13000002,-58.24995));
#173069=CARTESIAN_POINT('Origin',(57.,-2.42462934179819E-14,-58.24995));
#173070=CARTESIAN_POINT('',(57.,-29.63000002,-55.24995));
#173071=CARTESIAN_POINT('',(57.,28.41999998,-55.24995));
#173072=CARTESIAN_POINT('Origin',(57.,-29.63000002,-58.24995));
#173073=CARTESIAN_POINT('Origin',(57.,-29.63000002,-58.24995));
#173074=CARTESIAN_POINT('',(57.,-30.13000002,-55.74995));
#173075=CARTESIAN_POINT('Origin',(57.,-29.63000002,-55.74995));
#173076=CARTESIAN_POINT('',(59.5,-30.13000002,-58.24995));
#173077=CARTESIAN_POINT('Origin',(57.,-30.13000002,-58.24995));
#173078=CARTESIAN_POINT('Origin',(59.5,-29.63000002,-58.24995));
#173079=CARTESIAN_POINT('Origin',(59.5,-29.63000002,-55.24995));
#173080=CARTESIAN_POINT('',(59.5,-30.13000002,-174.34995));
#173081=CARTESIAN_POINT('',(59.5,-30.13000002,-58.24995));
#173082=CARTESIAN_POINT('Origin',(59.5,-29.63000002,-174.34995));
#173083=CARTESIAN_POINT('Origin',(57.,-29.63000002,-174.34995));
#173084=CARTESIAN_POINT('',(57.,-30.13000002,-176.84995));
#173085=CARTESIAN_POINT('Origin',(57.,-30.13000002,-174.34995));
#173086=CARTESIAN_POINT('Origin',(57.,-29.63000002,-176.84995));
#173087=CARTESIAN_POINT('Origin',(-83.2809572255632,-29.6300000199999,-176.84995));
#173088=CARTESIAN_POINT('',(-83.2809572255632,-30.13000002,-176.84995));
#173089=CARTESIAN_POINT('Origin',(56.294192362543,-30.63000002,-179.64995));
#173090=CARTESIAN_POINT('',(56.294192362543,-30.13000002,-171.871644662643));
#173091=CARTESIAN_POINT('',(56.294192362543,-30.13000002,-176.84995));
#173092=CARTESIAN_POINT('Origin',(56.294192362543,-30.63000002,-171.871644662643));
#173093=CARTESIAN_POINT('',(55.8171229357418,-30.4803178166104,-179.64995));
#173094=CARTESIAN_POINT('Ctrl Pts',(56.1167176003611,-30.13000002714,-171.179145966886));
#173095=CARTESIAN_POINT('Ctrl Pts',(55.7825352402592,-30.1299356988045,
-171.361452749053));
#173096=CARTESIAN_POINT('Ctrl Pts',(55.6935671754689,-30.4968373543263,
-171.410008924779));
#173097=CARTESIAN_POINT('Ctrl Pts',(56.2430624746474,-30.1300000269106,
-171.410992898787));
#173098=CARTESIAN_POINT('Ctrl Pts',(55.8840206261747,-30.1299383387469,
-171.527291609574));
#173099=CARTESIAN_POINT('Ctrl Pts',(55.7814946229066,-30.4850537049709,
-171.564548662911));
#173100=CARTESIAN_POINT('Ctrl Pts',(56.3050537145651,-30.130000026799,-171.670900042786));
#173101=CARTESIAN_POINT('Ctrl Pts',(55.9360241189749,-30.1299395985436,
-171.722483207042));
#173102=CARTESIAN_POINT('Ctrl Pts',(55.8246219322658,-30.4793202225602,
-171.737832654878));
#173103=CARTESIAN_POINT('Ctrl Pts',(56.2927384034373,-30.1300000268212,
-171.93833459815));
#173104=CARTESIAN_POINT('Ctrl Pts',(55.925777764091,-30.1299393505852,-171.921245295793));
#173105=CARTESIAN_POINT('Ctrl Pts',(55.8160539307423,-30.4804600576221,
-171.916099630748));
#173106=CARTESIAN_POINT('',(56.1468816861249,-30.13000002,-171.237717270032));
#173107=CARTESIAN_POINT('Origin',(54.8146431261402,-30.1299997583389,-171.852158294305));
#173108=CARTESIAN_POINT('Origin',(56.146881686125,-30.63000002,-171.237717270032));
#173109=CARTESIAN_POINT('Ctrl Pts',(40.2651432342477,-30.13000002,-139.30435351063));
#173110=CARTESIAN_POINT('Ctrl Pts',(39.9609182162754,-30.1300000199999,
-139.459264328773));
#173111=CARTESIAN_POINT('Ctrl Pts',(39.850159149164,-30.447965242174,-139.5156626415));
#173112=CARTESIAN_POINT('Ctrl Pts',(42.9624569131523,-30.13000002,-144.601532315192));
#173113=CARTESIAN_POINT('Ctrl Pts',(42.6706800009636,-30.13000002,-144.798763083095));
#173114=CARTESIAN_POINT('Ctrl Pts',(42.5429900246349,-30.4581917776324,
-144.812847565038));
#173115=CARTESIAN_POINT('Ctrl Pts',(45.6258101137111,-30.13000002,-149.91560863326));
#173116=CARTESIAN_POINT('Ctrl Pts',(45.3221739986871,-30.1300000200307,
-150.105257848785));
#173117=CARTESIAN_POINT('Ctrl Pts',(45.2030035072277,-30.4667604203174,
-150.126917764117));
#173118=CARTESIAN_POINT('Ctrl Pts',(50.9129382266982,-30.13000002,-160.563437524381));
#173119=CARTESIAN_POINT('Ctrl Pts',(50.5978344679358,-30.1300000199689,
-160.757133407541));
#173120=CARTESIAN_POINT('Ctrl Pts',(50.484627394531,-30.4818027714,-160.774746655264));
#173121=CARTESIAN_POINT('Ctrl Pts',(53.53633422979,-30.13000002,-165.897383514726));
#173122=CARTESIAN_POINT('Ctrl Pts',(53.2127313470812,-30.1300000198871,
-166.08608254617));
#173123=CARTESIAN_POINT('Ctrl Pts',(53.105875183067,-30.4882648083968,-166.108694936931));
#173124=CARTESIAN_POINT('Ctrl Pts',(56.1468816861249,-30.13000002,-171.237717270032));
#173125=CARTESIAN_POINT('Ctrl Pts',(55.8070372118623,-30.13000002,-171.403845487572));
#173126=CARTESIAN_POINT('Ctrl Pts',(55.7146117108563,-30.4940179634924,
-171.449026400902));
#173127=CARTESIAN_POINT('',(40.2651432342477,-30.13000002,-139.30435351063));
#173128=CARTESIAN_POINT('Ctrl Pts',(40.2651432342477,-30.13000002,-139.30435351063));
#173129=CARTESIAN_POINT('Ctrl Pts',(42.96245845912,-30.13000002,-144.601535351275));
#173130=CARTESIAN_POINT('Ctrl Pts',(45.6258101137032,-30.13000002,-149.915608633243));
#173131=CARTESIAN_POINT('Ctrl Pts',(48.2693741701893,-30.13000002,-155.239523078828));
#173132=CARTESIAN_POINT('Ctrl Pts',(50.9129382266755,-30.13000002,-160.563437524412));
#173133=CARTESIAN_POINT('Ctrl Pts',(53.5363337714711,-30.13000002,-165.897382577172));
#173134=CARTESIAN_POINT('Ctrl Pts',(56.1468816861249,-30.13000002,-171.237717270032));
#173135=CARTESIAN_POINT('Origin',(40.2651432342477,-30.63000002,-139.30435351063));
#173136=CARTESIAN_POINT('Ctrl Pts',(39.850159149164,-30.447965242174,-139.5156626415));
#173137=CARTESIAN_POINT('Ctrl Pts',(39.9609182162754,-30.13000002,-139.459264328773));
#173138=CARTESIAN_POINT('Ctrl Pts',(40.2651432342477,-30.13000002,-139.30435351063));
#173139=CARTESIAN_POINT('Ctrl Pts',(39.5639348330521,-30.4769451657213,
-138.978519823589));
#173140=CARTESIAN_POINT('Ctrl Pts',(39.6630612728547,-30.13000002,-138.925676053694));
#173141=CARTESIAN_POINT('Ctrl Pts',(40.0075294671789,-30.13000002,-138.798433034953));
#173142=CARTESIAN_POINT('Ctrl Pts',(39.3557167999464,-30.5068849023477,
-138.41703103581));
#173143=CARTESIAN_POINT('Ctrl Pts',(39.4450625268456,-30.13000002,-138.37488926852));
#173144=CARTESIAN_POINT('Ctrl Pts',(39.8201451200256,-30.13000002,-138.270288236581));
#173145=CARTESIAN_POINT('Ctrl Pts',(39.0729048436467,-30.5680016657979,
-137.252632910085));
#173146=CARTESIAN_POINT('Ctrl Pts',(39.1248051359359,-30.13000002,-137.23047141255));
#173147=CARTESIAN_POINT('Ctrl Pts',(39.5656143592083,-30.13000002,-137.176619865119));
#173148=CARTESIAN_POINT('Ctrl Pts',(39.,-30.5993710675033,-136.645762741564));
#173149=CARTESIAN_POINT('Ctrl Pts',(39.0297176446585,-30.13000002,-136.627803193949));
#173150=CARTESIAN_POINT('Ctrl Pts',(39.5000000014551,-30.13000002,-136.607413315277));
#173151=CARTESIAN_POINT('Ctrl Pts',(39.,-30.63000002,-136.04214564125));
#173152=CARTESIAN_POINT('Ctrl Pts',(39.,-30.13000002,-136.04214564125));
#173153=CARTESIAN_POINT('Ctrl Pts',(39.5,-30.13000002,-136.04214564125));
#173154=CARTESIAN_POINT('',(39.5,-30.13000002,-136.04214564125));
#173155=CARTESIAN_POINT('Ctrl Pts',(39.5,-30.13000002,-136.04214564125));
#173156=CARTESIAN_POINT('Ctrl Pts',(39.5,-30.13000002,-136.325718326755));
#173157=CARTESIAN_POINT('Ctrl Pts',(39.5162728499327,-30.13000002,-136.608122039194));
#173158=CARTESIAN_POINT('Ctrl Pts',(39.5808560770791,-30.13000002,-137.170628022919));
#173159=CARTESIAN_POINT('Ctrl Pts',(39.6292470494507,-30.13000002,-137.450036957971));
#173160=CARTESIAN_POINT('Ctrl Pts',(39.8201451199495,-30.13000002,-138.270288236609));
#173161=CARTESIAN_POINT('Ctrl Pts',(40.0074751366267,-30.13000002,-138.798326348879));
#173162=CARTESIAN_POINT('Ctrl Pts',(40.2651432342477,-30.13000002,-139.30435351063));
#173163=CARTESIAN_POINT('Origin',(39.5,-30.63000002,-136.04214564125));
#173164=CARTESIAN_POINT('Origin',(39.5,-30.63000002,-55.24995));
#173165=CARTESIAN_POINT('',(39.5,-30.13000002,-96.0164973302555));
#173166=CARTESIAN_POINT('',(39.5,-30.13000002,-55.24995));
#173167=CARTESIAN_POINT('Origin',(39.5,-30.63000002,-96.0164973302555));
#173168=CARTESIAN_POINT('Ctrl Pts',(39.,-30.63000002,-96.0164973302555));
#173169=CARTESIAN_POINT('Ctrl Pts',(39.,-30.13000002,-96.0164973302554));
#173170=CARTESIAN_POINT('Ctrl Pts',(39.5,-30.13000002,-96.0164973302555));
#173171=CARTESIAN_POINT('Ctrl Pts',(39.,-30.599243623439,-95.4103686640728));
#173172=CARTESIAN_POINT('Ctrl Pts',(39.0298365376099,-30.1300000199999,
-95.4284967516594));
#173173=CARTESIAN_POINT('Ctrl Pts',(39.5000000024932,-30.13000002,-95.4488679082906));
#173174=CARTESIAN_POINT('Ctrl Pts',(39.0712857711311,-30.5685553796042,
-94.8166771620692));
#173175=CARTESIAN_POINT('Ctrl Pts',(39.1227981005945,-30.13000002,-94.8386739331622));
#173176=CARTESIAN_POINT('Ctrl Pts',(39.5641571932953,-30.13000002,-94.8920319207365));
#173177=CARTESIAN_POINT('Ctrl Pts',(39.3518132725282,-30.5075286049387,
-93.6537603297063));
#173178=CARTESIAN_POINT('Ctrl Pts',(39.4408759042576,-30.13000002,-93.6956127800614));
#173179=CARTESIAN_POINT('Ctrl Pts',(39.8166319459981,-30.13000002,-93.7997753189033));
#173180=CARTESIAN_POINT('Ctrl Pts',(39.5639528617268,-30.4769433431446,
-93.080089311988));
#173181=CARTESIAN_POINT('Ctrl Pts',(39.6631053450898,-30.13000002,-93.1328879562182));
#173182=CARTESIAN_POINT('Ctrl Pts',(40.0075545499357,-30.13000002,-93.260160670532));
#173183=CARTESIAN_POINT('Ctrl Pts',(39.850159149164,-30.447965242174,-92.5429803300057));
#173184=CARTESIAN_POINT('Ctrl Pts',(39.9609182162754,-30.13000002,-92.5993786427328));
#173185=CARTESIAN_POINT('Ctrl Pts',(40.2651432342477,-30.13000002,-92.7542894608761));
#173186=CARTESIAN_POINT('',(40.2651432342477,-30.13000002,-92.754289460876));
#173187=CARTESIAN_POINT('',(39.8501336363284,-30.4479678253472,-92.5430282091296));
#173188=CARTESIAN_POINT('Origin',(40.2651432342477,-30.63000002,-92.754289460876));
#173189=CARTESIAN_POINT('Ctrl Pts',(39.,-30.63000002,-96.0164973302555));
#173190=CARTESIAN_POINT('Ctrl Pts',(39.,-30.6249052535773,-95.9160927210813));
#173191=CARTESIAN_POINT('Ctrl Pts',(39.0019517748916,-30.6195721960509,
-95.8112962237002));
#173192=CARTESIAN_POINT('Ctrl Pts',(39.0064236822507,-30.614000333733,-95.7021746191804));
#173193=CARTESIAN_POINT('Ctrl Pts',(39.0102527558462,-30.6092294229861,
-95.6087391740764));
#173194=CARTESIAN_POINT('Ctrl Pts',(39.0159309893287,-30.6042831282349,
-95.5121269654206));
#173195=CARTESIAN_POINT('Ctrl Pts',(39.0238420499257,-30.5991629267857,
-95.4124159301744));
#173196=CARTESIAN_POINT('Ctrl Pts',(39.0276963700442,-30.5966683313754,
-95.363836066012));
#173197=CARTESIAN_POINT('Ctrl Pts',(39.0320810493253,-30.5941324656576,
-95.3145208290036));
#173198=CARTESIAN_POINT('Ctrl Pts',(39.037041991603,-30.5915556817932,-95.2644827119115));
#173199=CARTESIAN_POINT('Ctrl Pts',(39.041382816096,-30.5893009959119,-95.220699359456));
#173200=CARTESIAN_POINT('Ctrl Pts',(39.0461648739216,-30.5870149782656,
-95.1763624788107));
#173201=CARTESIAN_POINT('Ctrl Pts',(39.0514193421249,-30.5846979430726,
-95.1314819004068));
#173202=CARTESIAN_POINT('Ctrl Pts',(39.0514662876117,-30.5846772417683,
-95.1310809196571));
#173203=CARTESIAN_POINT('Ctrl Pts',(39.0515142285028,-30.5846561156216,
-95.1306717143191));
#173204=CARTESIAN_POINT('Ctrl Pts',(39.0515634188643,-30.5846344546871,
-95.1302521554465));
#173205=CARTESIAN_POINT('Ctrl Pts',(39.0518641291921,-30.5845020371465,
-95.127687309768));
#173206=CARTESIAN_POINT('Ctrl Pts',(39.0522050961516,-30.5843525639836,
-95.1247923237199));
#173207=CARTESIAN_POINT('Ctrl Pts',(39.0525159392357,-30.5842169296647,
-95.1221655723487));
#173208=CARTESIAN_POINT('Ctrl Pts',(39.0526833331722,-30.5841438884304,
-95.1207510250266));
#173209=CARTESIAN_POINT('Ctrl Pts',(39.0528419432779,-30.5840748603693,
-95.1194142571582));
#173210=CARTESIAN_POINT('Ctrl Pts',(39.0529804943758,-30.5840146697563,
-95.1182486665959));
#173211=CARTESIAN_POINT('Ctrl Pts',(39.0530440420663,-30.5839870627975,
-95.1177140581416));
#173212=CARTESIAN_POINT('Ctrl Pts',(39.0531033676915,-30.5839613149507,
-95.117215459505));
#173213=CARTESIAN_POINT('Ctrl Pts',(39.0531573748585,-30.5839378916815,
-95.1167618808849));
#173214=CARTESIAN_POINT('Ctrl Pts',(39.0531858824795,-30.5839255277358,
-95.1165224599322));
#173215=CARTESIAN_POINT('Ctrl Pts',(39.0532129081873,-30.5839138114741,
-95.1162955826442));
#173216=CARTESIAN_POINT('Ctrl Pts',(39.0532382904984,-30.5839028113527,
-95.1160825741236));
#173217=CARTESIAN_POINT('Ctrl Pts',(39.0532602675523,-30.583893286993,-95.1158981425439));
#173218=CARTESIAN_POINT('Ctrl Pts',(39.0532810893944,-30.5838842660806,
-95.1157234607359));
#173219=CARTESIAN_POINT('Ctrl Pts',(39.0533023391604,-30.5838750624374,
-95.1155452413819));
#173220=CARTESIAN_POINT('Ctrl Pts',(39.0592332600412,-30.5813062774663,
-95.0658032871499));
#173221=CARTESIAN_POINT('Ctrl Pts',(39.0662052340743,-30.5784987766604,
-95.011508413269));
#173222=CARTESIAN_POINT('Ctrl Pts',(39.0745203401635,-30.5754521822375,
-94.9526940905704));
#173223=CARTESIAN_POINT('Ctrl Pts',(39.0825579442499,-30.5725072625311,
-94.8958425921788));
#173224=CARTESIAN_POINT('Ctrl Pts',(39.0918507976603,-30.5693389401508,
-94.8347683127649));
#173225=CARTESIAN_POINT('Ctrl Pts',(39.1027173036832,-30.5659470513343,
-94.7695096773549));
#173226=CARTESIAN_POINT('Ctrl Pts',(39.1141365869548,-30.5623826177307,
-94.7009313466487));
#173227=CARTESIAN_POINT('Ctrl Pts',(39.1272940640147,-30.5585711624585,
-94.6277296646441));
#173228=CARTESIAN_POINT('Ctrl Pts',(39.1426044136615,-30.5545146082183,
-94.5499943643404));
#173229=CARTESIAN_POINT('Ctrl Pts',(39.1579147633082,-30.5504580539782,
-94.4722590640368));
#173230=CARTESIAN_POINT('Ctrl Pts',(39.1753792515526,-30.5461561819419,
-94.389986077742));
#173231=CARTESIAN_POINT('Ctrl Pts',(39.1954540957825,-30.5416127257937,
-94.303302840083));
#173232=CARTESIAN_POINT('Ctrl Pts',(39.1991593872304,-30.5407741225639,
-94.2873033804859));
#173233=CARTESIAN_POINT('Ctrl Pts',(39.2027413140868,-30.5399744287283,
-94.2720525195795));
#173234=CARTESIAN_POINT('Ctrl Pts',(39.2066491849319,-30.5391142739385,
-94.2556556609144));
#173235=CARTESIAN_POINT('Ctrl Pts',(39.2082189913868,-30.5387687465158,
-94.2490689809567));
#173236=CARTESIAN_POINT('Ctrl Pts',(39.2098419385736,-30.5384134641158,
-94.2422974725426));
#173237=CARTESIAN_POINT('Ctrl Pts',(39.2115495219815,-30.5380419914382,
-94.2352187459229));
#173238=CARTESIAN_POINT('Ctrl Pts',(39.2116381806325,-30.5380227043765,
-94.2348512146211));
#173239=CARTESIAN_POINT('Ctrl Pts',(39.2117270689434,-30.5380033735724,
-94.2344828534231));
#173240=CARTESIAN_POINT('Ctrl Pts',(39.211816191455,-30.5379839981243,-94.2341136452022));
#173241=CARTESIAN_POINT('Ctrl Pts',(39.2303698501946,-30.533950388163,-94.1572513215619));
#173242=CARTESIAN_POINT('Ctrl Pts',(39.2491858444372,-30.5301075162906,
-94.0846500822156));
#173243=CARTESIAN_POINT('Ctrl Pts',(39.2678896114286,-30.5264770887774,
-94.0162910979177));
#173244=CARTESIAN_POINT('Ctrl Pts',(39.2871262661881,-30.5227432269981,
-93.9459845023932));
#173245=CARTESIAN_POINT('Ctrl Pts',(39.3062439542278,-30.5192340377043,
-93.8801647140279));
#173246=CARTESIAN_POINT('Ctrl Pts',(39.3248813010155,-30.5159694653193,
-93.818780919685));
#173247=CARTESIAN_POINT('Ctrl Pts',(39.3356188989651,-30.5140886361355,
-93.7834156656183));
#173248=CARTESIAN_POINT('Ctrl Pts',(39.3461979255374,-30.5122889392155,
-93.7495223469786));
#173249=CARTESIAN_POINT('Ctrl Pts',(39.3565563938204,-30.5105737630814,
-93.7170880835705));
#173250=CARTESIAN_POINT('Ctrl Pts',(39.3748703165573,-30.5075413067044,
-93.6597438336436));
#173251=CARTESIAN_POINT('Ctrl Pts',(39.3924929457479,-30.5047638464613,
-93.6069649458907));
#173252=CARTESIAN_POINT('Ctrl Pts',(39.4091261367344,-30.5022275366221,
-93.5586840765167));
#173253=CARTESIAN_POINT('Ctrl Pts',(39.4132999564277,-30.5015910923004,
-93.5465688038931));
#173254=CARTESIAN_POINT('Ctrl Pts',(39.4174117270447,-30.5009698324755,
-93.5347367182726));
#173255=CARTESIAN_POINT('Ctrl Pts',(39.4214572463548,-30.500363538649,-93.523186689646));
#173256=CARTESIAN_POINT('Ctrl Pts',(39.4315409550048,-30.4988523135543,
-93.4943975244871));
#173257=CARTESIAN_POINT('Ctrl Pts',(39.4412125697053,-30.4974336004572,
-93.4673609360235));
#173258=CARTESIAN_POINT('Ctrl Pts',(39.4504127978213,-30.4961019998094,
-93.442060190349));
#173259=CARTESIAN_POINT('Ctrl Pts',(39.4550129118793,-30.4954361994855,
-93.4294098175118));
#173260=CARTESIAN_POINT('Ctrl Pts',(39.459495280608,-30.4947922073451,-93.4171934409355));
#173261=CARTESIAN_POINT('Ctrl Pts',(39.4638532593191,-30.4941692342306,
-93.4054090017087));
#173262=CARTESIAN_POINT('Ctrl Pts',(39.4660322486747,-30.4938577476734,
-93.3995167820953));
#173263=CARTESIAN_POINT('Ctrl Pts',(39.4681801470372,-30.493551517769,-93.3937325490637));
#173264=CARTESIAN_POINT('Ctrl Pts',(39.4702961652564,-30.4932504519151,
-93.3880560566882));
#173265=CARTESIAN_POINT('Ctrl Pts',(39.471354174366,-30.4930999189882,-93.3852178105004));
#173266=CARTESIAN_POINT('Ctrl Pts',(39.4724042138444,-30.4929506771965,
-93.3824064996216));
#173267=CARTESIAN_POINT('Ctrl Pts',(39.473446187943,-30.4928027147915,-93.3796220936597));
#173268=CARTESIAN_POINT('Ctrl Pts',(39.4739671749922,-30.492728733589,-93.3782298906788));
#173269=CARTESIAN_POINT('Ctrl Pts',(39.4744861457219,-30.4926550722409,
-93.3768444139362));
#173270=CARTESIAN_POINT('Ctrl Pts',(39.4750030883437,-30.4925817292688,
-93.3754656596573));
#173271=CARTESIAN_POINT('Ctrl Pts',(39.4755200309655,-30.4925083862968,
-93.3740869053783));
#173272=CARTESIAN_POINT('Ctrl Pts',(39.4756022368881,-30.4924967046419,
-93.3738667780565));
#173273=CARTESIAN_POINT('Ctrl Pts',(39.4765478202071,-30.4923626540173,
-93.3713495604645));
#173274=CARTESIAN_POINT('Ctrl Pts',(39.5126025370099,-30.4872513568841,
-93.2753690523553));
#173275=CARTESIAN_POINT('Ctrl Pts',(39.549431291156,-30.4823498708368,-93.1835388191733));
#173276=CARTESIAN_POINT('Ctrl Pts',(39.5866068526539,-30.4776588176486,
-93.095820174658));
#173277=CARTESIAN_POINT('Ctrl Pts',(39.6248843739199,-30.4728287120379,
-93.0055013698956));
#173278=CARTESIAN_POINT('Ctrl Pts',(39.6635293745984,-30.4682216676362,
-92.9195409504136));
#173279=CARTESIAN_POINT('Ctrl Pts',(39.7021109540059,-30.4638355826243,
-92.8378531504812));
#173280=CARTESIAN_POINT('Ctrl Pts',(39.7422060023605,-30.4592774413211,
-92.7529609211173));
#173281=CARTESIAN_POINT('Ctrl Pts',(39.7822322739401,-30.4549579016675,
-92.672682491943));
#173282=CARTESIAN_POINT('Ctrl Pts',(39.8217476739595,-30.4508721484859,
-92.5968843423184));
#173283=CARTESIAN_POINT('Ctrl Pts',(39.8312408753335,-30.4498905849006,
-92.5786745532789));
#173284=CARTESIAN_POINT('Ctrl Pts',(39.8407047841214,-30.4489225049938,
-92.5607232068311));
#173285=CARTESIAN_POINT('Ctrl Pts',(39.8501336363284,-30.4479678253472,
-92.5430282091296));
#173286=CARTESIAN_POINT('Ctrl Pts',(40.2651432342476,-30.13000002,-92.7542894608761));
#173287=CARTESIAN_POINT('Ctrl Pts',(40.149768118957,-30.13000002,-92.9808714190862));
#173288=CARTESIAN_POINT('Ctrl Pts',(40.0478331438219,-30.13000002,-93.2140840893024));
#173289=CARTESIAN_POINT('Ctrl Pts',(39.9590875376241,-30.13000002,-93.45156448926));
#173290=CARTESIAN_POINT('Ctrl Pts',(39.8658509560192,-30.13000002,-93.7010625955762));
#173291=CARTESIAN_POINT('Ctrl Pts',(39.7871721235837,-30.13000002,-93.9552726783295));
#173292=CARTESIAN_POINT('Ctrl Pts',(39.7228113496721,-30.13000002,-94.2114776823655));
#173293=CARTESIAN_POINT('Ctrl Pts',(39.7115691395802,-30.13000002,-94.2562302592369));
#173294=CARTESIAN_POINT('Ctrl Pts',(39.700763918709,-30.13000002,-94.3010437266484));
#173295=CARTESIAN_POINT('Ctrl Pts',(39.6903945692724,-30.13000002,-94.3459036197334));
#173296=CARTESIAN_POINT('Ctrl Pts',(39.6046719082244,-30.13000002,-94.7167571079952));
#173297=CARTESIAN_POINT('Ctrl Pts',(39.5475807634106,-30.13000002,-95.0925075650471));
#173298=CARTESIAN_POINT('Ctrl Pts',(39.5197593574037,-30.13000002,-95.4732641712651));
#173299=CARTESIAN_POINT('Ctrl Pts',(39.5066102516738,-30.13000002,-95.6532194499914));
#173300=CARTESIAN_POINT('Ctrl Pts',(39.5000000000002,-30.13000002,-95.8342931017866));
#173301=CARTESIAN_POINT('Ctrl Pts',(39.5,-30.13000002,-96.0164973302555));
#173302=CARTESIAN_POINT('Ctrl Pts',(56.0289353856639,-30.13000002,-61.0621827299711));
#173303=CARTESIAN_POINT('Ctrl Pts',(55.6892944482707,-30.13000002,-60.8961225062558));
#173304=CARTESIAN_POINT('Ctrl Pts',(55.5967474138374,-30.4937575588533,
-60.8508735991007));
#173305=CARTESIAN_POINT('Ctrl Pts',(53.4376477846732,-30.13000002,-66.3621114555649));
#173306=CARTESIAN_POINT('Ctrl Pts',(53.1140955473737,-30.1300000200305,
-66.1737552088486));
#173307=CARTESIAN_POINT('Ctrl Pts',(53.0072677069205,-30.4880260434848,
-66.1508000801069));
#173308=CARTESIAN_POINT('Ctrl Pts',(50.8336218773704,-30.13000002,-71.655706365272));
#173309=CARTESIAN_POINT('Ctrl Pts',(50.518482898395,-30.13000002,-71.4624685012804));
#173310=CARTESIAN_POINT('Ctrl Pts',(50.405384759569,-30.4815921581836,-71.4443972343972));
#173311=CARTESIAN_POINT('Ctrl Pts',(45.5856873606873,-30.13000002,-82.223056081386));
#173312=CARTESIAN_POINT('Ctrl Pts',(45.2819556815256,-30.13000002,-82.0338364947541));
#173313=CARTESIAN_POINT('Ctrl Pts',(45.1629315870884,-30.4666308723541,
-82.01174695052));
#173314=CARTESIAN_POINT('Ctrl Pts',(42.94214612644,-30.13000002,-87.4969984415611));
#173315=CARTESIAN_POINT('Ctrl Pts',(42.650123001142,-30.13000002,-87.3003867975457));
#173316=CARTESIAN_POINT('Ctrl Pts',(42.5227129344255,-30.4581147715466,
-87.2856833539494));
#173317=CARTESIAN_POINT('Ctrl Pts',(40.2651432342477,-30.13000002,-92.7542894608761));
#173318=CARTESIAN_POINT('Ctrl Pts',(39.9609182162754,-30.13000002,-92.5993786427328));
#173319=CARTESIAN_POINT('Ctrl Pts',(39.850159149164,-30.447965242174,-92.5429803300057));
#173320=CARTESIAN_POINT('',(56.0289353856639,-30.13000002,-61.0621827299711));
#173321=CARTESIAN_POINT('',(55.5967474138374,-30.4937575588533,-60.8508735991007));
#173322=CARTESIAN_POINT('Origin',(56.0289353856639,-30.63000002,-61.0621827299711));
#173323=CARTESIAN_POINT('Ctrl Pts',(39.850159149164,-30.447965242174,-92.5429803300057));
#173324=CARTESIAN_POINT('Ctrl Pts',(40.4919890794513,-30.4504027129368,
-91.2804087139596));
#173325=CARTESIAN_POINT('Ctrl Pts',(41.1472641150672,-30.452803979004,-89.9867515631817));
#173326=CARTESIAN_POINT('Ctrl Pts',(41.8159279844008,-30.4551647590928,
-88.6619683163481));
#173327=CARTESIAN_POINT('Ctrl Pts',(42.4652749676593,-30.4574573391156,
-87.3754564465499));
#173328=CARTESIAN_POINT('Ctrl Pts',(43.1272482893852,-30.4597117299785,
-86.0595906033186));
#173329=CARTESIAN_POINT('Ctrl Pts',(43.8018380914677,-30.461925824762,-84.7143559757826));
#173330=CARTESIAN_POINT('Ctrl Pts',(44.4532739805521,-30.4640639252777,
-83.4152937710014));
#173331=CARTESIAN_POINT('Ctrl Pts',(45.1164743748462,-30.4661644409739,
-82.0888454883916));
#173332=CARTESIAN_POINT('Ctrl Pts',(45.7914697121484,-30.4682272829623,
-80.7350244407743));
#173333=CARTESIAN_POINT('Ctrl Pts',(46.4393888922545,-30.4702073779584,
-79.4355093556948));
#173334=CARTESIAN_POINT('Ctrl Pts',(47.0981756635805,-30.4721527594818,
-78.1107735479491));
#173335=CARTESIAN_POINT('Ctrl Pts',(47.7678960568131,-30.4740650926897,
-76.7608514488592));
#173336=CARTESIAN_POINT('Ctrl Pts',(47.7732963461685,-30.4740805127856,
-76.7499663541003));
#173337=CARTESIAN_POINT('Ctrl Pts',(47.7794480652732,-30.4740980732275,
-76.7375663802255));
#173338=CARTESIAN_POINT('Ctrl Pts',(47.7841581747548,-30.4741115104162,
-76.7280720931668));
#173339=CARTESIAN_POINT('Ctrl Pts',(47.7842851392984,-30.4741118726257,
-76.7278161675185));
#173340=CARTESIAN_POINT('Ctrl Pts',(47.7844110563643,-30.47411223184,-76.727562353186));
#173341=CARTESIAN_POINT('Ctrl Pts',(47.7845358830013,-30.4741125879365,
-76.7273107367533));
#173342=CARTESIAN_POINT('Ctrl Pts',(48.5628078545631,-30.4763327867105,
-75.1585268464595));
#173343=CARTESIAN_POINT('Ctrl Pts',(49.3583939950128,-30.4785153611757,
-73.5505206630954));
#173344=CARTESIAN_POINT('Ctrl Pts',(50.1712495695924,-30.4806565898269,
-71.9032649192444));
#173345=CARTESIAN_POINT('Ctrl Pts',(50.962904574651,-30.4827419718206,-70.2989722318186));
#173346=CARTESIAN_POINT('Ctrl Pts',(51.7709397108168,-30.484788125207,-68.6574505523832));
#173347=CARTESIAN_POINT('Ctrl Pts',(52.5953571041642,-30.4867937041832,
-66.9786972374972));
#173348=CARTESIAN_POINT('Ctrl Pts',(53.3928114301762,-30.4887336894912,
-65.3548485607644));
#173349=CARTESIAN_POINT('Ctrl Pts',(54.2055938276031,-30.4906357043452,
-63.6961637244116));
#173350=CARTESIAN_POINT('Ctrl Pts',(55.033749835842,-30.4925006401861,-62.0026629615056));
#173351=CARTESIAN_POINT('Ctrl Pts',(55.2206323562122,-30.4929214834896,
-61.6205058707253));
#173352=CARTESIAN_POINT('Ctrl Pts',(55.408297930604,-30.4933404476046,-61.2365759484398));
#173353=CARTESIAN_POINT('Ctrl Pts',(55.5967474138374,-30.4937575588533,
-60.8508735991007));
#173354=CARTESIAN_POINT('Ctrl Pts',(56.0289353856639,-30.13000002,-61.0621827299711));
#173355=CARTESIAN_POINT('Ctrl Pts',(53.4376473376604,-30.13000002,-66.3621123698348));
#173356=CARTESIAN_POINT('Ctrl Pts',(50.8336218773754,-30.13000002,-71.6557063652599));
#173357=CARTESIAN_POINT('Ctrl Pts',(48.2096546190284,-30.13000002,-76.9393812233288));
#173358=CARTESIAN_POINT('Ctrl Pts',(45.5856873606815,-30.13000002,-82.2230560813977));
#173359=CARTESIAN_POINT('Ctrl Pts',(42.9421476228591,-30.13000002,-87.4969955027855));
#173360=CARTESIAN_POINT('Ctrl Pts',(40.2651432342477,-30.13000002,-92.754289460876));
#173361=CARTESIAN_POINT('Ctrl Pts',(40.0751063884513,-36.0938884806558,
-86.6376094090262));
#173362=CARTESIAN_POINT('Ctrl Pts',(39.,-37.0899493132599,-87.566881951549));
#173363=CARTESIAN_POINT('Ctrl Pts',(39.,-38.3588510099497,-88.7507007177297));
#173364=CARTESIAN_POINT('Ctrl Pts',(40.0284942066422,-34.9676073874133,
-87.9314164096932));
#173365=CARTESIAN_POINT('Ctrl Pts',(38.9999999999938,-35.9377762186182,
-88.8634929468774));
#173366=CARTESIAN_POINT('Ctrl Pts',(39.,-37.1517824539261,-90.044523203833));
#173367=CARTESIAN_POINT('Ctrl Pts',(39.9811083568879,-33.8078923846355,
-89.2002134624161));
#173368=CARTESIAN_POINT('Ctrl Pts',(39.,-34.7456425298457,-90.138609363953));
#173369=CARTESIAN_POINT('Ctrl Pts',(39.,-35.9043080884012,-91.3133047711639));
#173370=CARTESIAN_POINT('Ctrl Pts',(39.8860349814824,-31.4034505542693,
-91.6586472348866));
#173371=CARTESIAN_POINT('Ctrl Pts',(39.,-32.2660375633753,-92.6092802152048));
#173372=CARTESIAN_POINT('Ctrl Pts',(39.,-33.3065376953223,-93.7717385435459));
#173373=CARTESIAN_POINT('Ctrl Pts',(39.8388209456929,-30.1709967638591,
-92.8359193626927));
#173374=CARTESIAN_POINT('Ctrl Pts',(39.,-30.9915371636578,-93.792984660173));
#173375=CARTESIAN_POINT('Ctrl Pts',(39.,-31.9694828580011,-94.9490286570666));
#173376=CARTESIAN_POINT('Ctrl Pts',(39.7930043023957,-28.8965637205256,
-93.942810661998));
#173377=CARTESIAN_POINT('Ctrl Pts',(39.,-29.6660656545474,-94.9083553778138));
#173378=CARTESIAN_POINT('Ctrl Pts',(39.,-30.5806160716777,-96.0559019707015));
#173379=CARTESIAN_POINT('',(40.0734472026555,-36.0537916247009,-86.6836434020945));
#173380=CARTESIAN_POINT('Ctrl Pts',(40.0734472049734,-36.0537916894494,
-86.683643483585));
#173381=CARTESIAN_POINT('Ctrl Pts',(40.0582294002964,-35.6859715947434,
-87.1056818970377));
#173382=CARTESIAN_POINT('Ctrl Pts',(40.0431653813165,-35.3202583628105,
-87.5185158963228));
#173383=CARTESIAN_POINT('Ctrl Pts',(40.0282656000844,-34.9562785737579,
-87.9223716670628));
#173384=CARTESIAN_POINT('Ctrl Pts',(40.0116226499473,-34.5497157265767,
-88.3734757034434));
#173385=CARTESIAN_POINT('Ctrl Pts',(39.9951846492463,-34.1453161855968,
-88.8133780401699));
#173386=CARTESIAN_POINT('Ctrl Pts',(39.9789600467457,-33.7425726182128,
-89.2424636967788));
#173387=CARTESIAN_POINT('Ctrl Pts',(39.9636394913162,-33.3622702257363,
-89.6476403774287));
#173388=CARTESIAN_POINT('Ctrl Pts',(39.9485091110465,-32.9834450563986,
-90.0431738242611));
#173389=CARTESIAN_POINT('Ctrl Pts',(39.9335716691851,-32.6056714694524,
-90.4294303486514));
#173390=CARTESIAN_POINT('Ctrl Pts',(39.9155227303514,-32.1492069404469,
-90.8961448267766));
#173391=CARTESIAN_POINT('Ctrl Pts',(39.897824098653,-31.6960435093008,-91.347532590367));
#173392=CARTESIAN_POINT('Ctrl Pts',(39.8804902707974,-31.2451213065669,
-91.7842587747131));
#173393=CARTESIAN_POINT('Ctrl Pts',(39.8702497189193,-30.9787235871182,
-92.0422697105862));
#173394=CARTESIAN_POINT('Ctrl Pts',(39.8601363016365,-30.713108867239,-92.2951643300845));
#173395=CARTESIAN_POINT('Ctrl Pts',(39.8501516349846,-30.4480624604452,
-92.5430839616816));
#173396=CARTESIAN_POINT('Ctrl Pts',(40.0734472049734,-36.0537916894494,
-86.683643483585));
#173397=CARTESIAN_POINT('Ctrl Pts',(40.0245584466381,-36.0584545847703,
-86.7694976519593));
#173398=CARTESIAN_POINT('Ctrl Pts',(39.9757226962818,-36.0633262985487,
-86.8593752483436));
#173399=CARTESIAN_POINT('Ctrl Pts',(39.927286973467,-36.0684348005888,-86.9533520768013));
#173400=CARTESIAN_POINT('Ctrl Pts',(39.8951777242464,-36.0718213540584,
-87.0156516612927));
#173401=CARTESIAN_POINT('Ctrl Pts',(39.8632450041024,-36.0753114008984,
-87.0797523342764));
#173402=CARTESIAN_POINT('Ctrl Pts',(39.8315977698661,-36.0789050638006,
-87.1456702267159));
#173403=CARTESIAN_POINT('Ctrl Pts',(39.7919047583749,-36.0834123550793,
-87.2283466351038));
#173404=CARTESIAN_POINT('Ctrl Pts',(39.7526605370814,-36.0880833296136,
-87.3138822668377));
#173405=CARTESIAN_POINT('Ctrl Pts',(39.714092383476,-36.0929016857489,-87.402296181153));
#173406=CARTESIAN_POINT('Ctrl Pts',(39.6948083066732,-36.0953108638166,
-87.4465031383107));
#173407=CARTESIAN_POINT('Ctrl Pts',(39.6756934496369,-36.0977565857494,
-87.4914294306899));
#173408=CARTESIAN_POINT('Ctrl Pts',(39.6567773264731,-36.1002348892133,
-87.5370759143626));
#173409=CARTESIAN_POINT('Ctrl Pts',(39.6473192648912,-36.1014740409452,
-87.559899156199));
#173410=CARTESIAN_POINT('Ctrl Pts',(39.6379108833219,-36.1027213366419,
-87.5829024445171));
#173411=CARTESIAN_POINT('Ctrl Pts',(39.6285559461866,-36.1039761301367,
-87.6060857648908));
#173412=CARTESIAN_POINT('Ctrl Pts',(39.6238784776189,-36.1046035268841,
-87.6176774250777));
#173413=CARTESIAN_POINT('Ctrl Pts',(39.61921436983,-36.1052327979438,-87.6293140931487));
#173414=CARTESIAN_POINT('Ctrl Pts',(39.614564094214,-36.1058638576854,-87.6409957632537));
#173415=CARTESIAN_POINT('Ctrl Pts',(39.612238956406,-36.1061793875562,-87.6468365983062));
#173416=CARTESIAN_POINT('Ctrl Pts',(39.6099172766201,-36.1064953645889,
-87.6526886838591));
#173417=CARTESIAN_POINT('Ctrl Pts',(39.6075991140024,-36.1068117775199,
-87.6585520187252));
#173418=CARTESIAN_POINT('Ctrl Pts',(39.6052809513847,-36.1071281904509,
-87.6644153535913));
#173419=CARTESIAN_POINT('Ctrl Pts',(39.6022185548814,-36.1075476937166,
-87.6721943105456));
#173420=CARTESIAN_POINT('Ctrl Pts',(39.6006552368152,-36.1077623125535,
-87.6761757699178));
#173421=CARTESIAN_POINT('Ctrl Pts',(39.5779632105313,-36.1108775687474,
-87.7339678358275));
#173422=CARTESIAN_POINT('Ctrl Pts',(39.5542205394167,-36.1141975364057,
-87.7964178534076));
#173423=CARTESIAN_POINT('Ctrl Pts',(39.5297328530949,-36.1177665535606,
-87.8636089002945));
#173424=CARTESIAN_POINT('Ctrl Pts',(39.5056031226127,-36.1212833995746,
-87.9298177626136));
#173425=CARTESIAN_POINT('Ctrl Pts',(39.4807501012066,-36.1250425564943,
-88.000630514969));
#173426=CARTESIAN_POINT('Ctrl Pts',(39.4555131835107,-36.1290706613253,
-88.0761190496449));
#173427=CARTESIAN_POINT('Ctrl Pts',(39.4308618377357,-36.1330053020847,
-88.1498560246892));
#173428=CARTESIAN_POINT('Ctrl Pts',(39.4058444701722,-36.1371969955752,
-88.2280547461139));
#173429=CARTESIAN_POINT('Ctrl Pts',(39.3808197403438,-36.141648612017,-88.3107684439465));
#173430=CARTESIAN_POINT('Ctrl Pts',(39.3714871748443,-36.1433087698811,
-88.3416151706854));
#173431=CARTESIAN_POINT('Ctrl Pts',(39.3621539945362,-36.1450048212813,
-88.3730896656766));
#173432=CARTESIAN_POINT('Ctrl Pts',(39.352840229561,-36.1467359139454,-88.4051939925927));
#173433=CARTESIAN_POINT('Ctrl Pts',(39.3385398145363,-36.1493938448261,
-88.4544871839289));
#173434=CARTESIAN_POINT('Ctrl Pts',(39.3242849868855,-36.1521345745536,
-88.5052653310622));
#173435=CARTESIAN_POINT('Ctrl Pts',(39.3101516172692,-36.1549520365536,
-88.5575337102131));
#173436=CARTESIAN_POINT('Ctrl Pts',(39.3030849324611,-36.1563607675536,
-88.5836678997886));
#173437=CARTESIAN_POINT('Ctrl Pts',(39.2960486439358,-36.1577886899918,
-88.6101746554091));
#173438=CARTESIAN_POINT('Ctrl Pts',(39.2890526314425,-36.1592345959982,
-88.6370542948565));
#173439=CARTESIAN_POINT('Ctrl Pts',(39.2855546251958,-36.1599575490013,
-88.6504941145803));
#173440=CARTESIAN_POINT('Ctrl Pts',(39.2820666894481,-36.1606849983143,
-88.6640271556613));
#173441=CARTESIAN_POINT('Ctrl Pts',(39.2785900750634,-36.1614167794284,
-88.6776534472724));
#173442=CARTESIAN_POINT('Ctrl Pts',(39.276851767871,-36.1617826699853,-88.684466593078));
#173443=CARTESIAN_POINT('Ctrl Pts',(39.2751162911093,-36.1621496435148,
-88.6913030515374));
#173444=CARTESIAN_POINT('Ctrl Pts',(39.2733838024279,-36.1625176778282,
-88.6981628250376));
#173445=CARTESIAN_POINT('Ctrl Pts',(39.2725175580872,-36.1627016949849,
-88.7015927117877));
#173446=CARTESIAN_POINT('Ctrl Pts',(39.2716520607718,-36.1628859773388,
-88.7050284272993));
#173447=CARTESIAN_POINT('Ctrl Pts',(39.2707873302702,-36.1630705220061,
-88.7084699717845));
#173448=CARTESIAN_POINT('Ctrl Pts',(39.2699225997686,-36.1632550666735,
-88.7119115162696));
#173449=CARTESIAN_POINT('Ctrl Pts',(39.2693983359119,-36.1633670415458,
-88.713999895811));
#173450=CARTESIAN_POINT('Ctrl Pts',(39.2681954590309,-36.1636249400336,
-88.7188120923488));
#173451=CARTESIAN_POINT('Ctrl Pts',(39.248398147037,-36.167869511449,-88.7980126803225));
#173452=CARTESIAN_POINT('Ctrl Pts',(39.2307677419702,-36.171950025859,-88.8731714624208));
#173453=CARTESIAN_POINT('Ctrl Pts',(39.2149695096784,-36.1758143575034,
-88.9441946157667));
#173454=CARTESIAN_POINT('Ctrl Pts',(39.1988652605947,-36.1797535424828,
-89.0165935102169));
#173455=CARTESIAN_POINT('Ctrl Pts',(39.1846644603266,-36.1834685416629,
-89.0846953678492));
#173456=CARTESIAN_POINT('Ctrl Pts',(39.1720493682215,-36.1869310591102,
-89.1484303377924));
#173457=CARTESIAN_POINT('Ctrl Pts',(39.1591222702079,-36.1904792141329,
-89.2137416487592));
#173458=CARTESIAN_POINT('Ctrl Pts',(39.1478599448633,-36.1937626900379,
-89.2744677490584));
#173459=CARTESIAN_POINT('Ctrl Pts',(39.1379644992164,-36.1967721114012,
-89.3305586607797));
#173460=CARTESIAN_POINT('Ctrl Pts',(39.127964529343,-36.1998133208668,-89.3872420530587));
#173461=CARTESIAN_POINT('Ctrl Pts',(39.1193603137208,-36.2025751137754,
-89.4391922114424));
#173462=CARTESIAN_POINT('Ctrl Pts',(39.11189245695,-36.2050620666782,-89.4863771085259));
#173463=CARTESIAN_POINT('Ctrl Pts',(39.104334359811,-36.2075790715159,-89.5341321802417));
#173464=CARTESIAN_POINT('Ctrl Pts',(39.0979401478849,-36.2098149531853,
-89.5770064754588));
#173465=CARTESIAN_POINT('Ctrl Pts',(39.0924918051001,-36.211782447031,-89.6149810792825));
#173466=CARTESIAN_POINT('Ctrl Pts',(39.089202610369,-36.2129702339684,-89.6379065580461));
#173467=CARTESIAN_POINT('Ctrl Pts',(39.0862591379092,-36.2140603258838,
-89.6590465409137));
#173468=CARTESIAN_POINT('Ctrl Pts',(39.0836224115253,-36.2150560549564,
-89.6783985960165));
#173469=CARTESIAN_POINT('Ctrl Pts',(39.0796481868764,-36.2165568747034,
-89.7075671191007));
#173470=CARTESIAN_POINT('Ctrl Pts',(39.0763692393887,-36.2178434340386,
-89.732673665977));
#173471=CARTESIAN_POINT('Ctrl Pts',(39.0736808720347,-36.2189267619753,
-89.7537135766213));
#173472=CARTESIAN_POINT('Ctrl Pts',(39.0723366883577,-36.2194684259437,
-89.7642335319435));
#173473=CARTESIAN_POINT('Ctrl Pts',(39.0711406879357,-36.2199592627485,
-89.7737368858829));
#173474=CARTESIAN_POINT('Ctrl Pts',(39.0700829940987,-36.2204004509078,
-89.782223326275));
#173475=CARTESIAN_POINT('Ctrl Pts',(39.0695541471802,-36.2206210449875,
-89.7864665464711));
#173476=CARTESIAN_POINT('Ctrl Pts',(39.0690599092086,-36.2208292307969,
-89.790455542088));
#173477=CARTESIAN_POINT('Ctrl Pts',(39.068599245928,-36.221025129606,-89.7941902836961));
#173478=CARTESIAN_POINT('Ctrl Pts',(39.0683689142878,-36.2211230790106,
-89.7960576545002));
#173479=CARTESIAN_POINT('Ctrl Pts',(39.0681469783199,-36.2212179569089,
-89.7978614620406));
#173480=CARTESIAN_POINT('Ctrl Pts',(39.0679333209832,-36.2213097782944,
-89.7996017034629));
#173481=CARTESIAN_POINT('Ctrl Pts',(39.0678264923148,-36.2213556889871,
-89.8004718241741));
#173482=CARTESIAN_POINT('Ctrl Pts',(39.067721733429,-36.2214008355664,-89.8013260533702));
#173483=CARTESIAN_POINT('Ctrl Pts',(39.0676190304694,-36.221445219821,-89.80216439073));
#173484=CARTESIAN_POINT('Ctrl Pts',(39.0675676789896,-36.2214674119482,
-89.8025835594099));
#173485=CARTESIAN_POINT('Ctrl Pts',(39.0675168415914,-36.221489413483,-89.8029987551334));
#173486=CARTESIAN_POINT('Ctrl Pts',(39.067466758021,-36.2215111314003,-89.8034079910735));
#173487=CARTESIAN_POINT('Ctrl Pts',(39.0674166744505,-36.2215328493176,
-89.8038172270136));
#173488=CARTESIAN_POINT('Ctrl Pts',(39.0673667213199,-36.2215544886427,
-89.8042244740143));
#173489=CARTESIAN_POINT('Ctrl Pts',(39.0671690648645,-36.2216404734312,
-89.805843073341));
#173490=CARTESIAN_POINT('Ctrl Pts',(39.0535618414146,-36.2275599068601,
-89.9172719799453));
#173491=CARTESIAN_POINT('Ctrl Pts',(39.0424392254192,-36.2333308081245,
-90.0254583105046));
#173492=CARTESIAN_POINT('Ctrl Pts',(39.0334327685362,-36.2389072191113,
-90.1302828991747));
#173493=CARTESIAN_POINT('Ctrl Pts',(39.0242321778508,-36.2446038294043,
-90.237366977481));
#173494=CARTESIAN_POINT('Ctrl Pts',(39.01723947308,-36.2500978354871,-90.340943088193));
#173495=CARTESIAN_POINT('Ctrl Pts',(39.0120825306864,-36.2553769973198,
-90.4409205822943));
#173496=CARTESIAN_POINT('Ctrl Pts',(39.0067454951592,-36.26084052049,-90.5443895368034));
#173497=CARTESIAN_POINT('Ctrl Pts',(39.0033742127362,-36.266074288559,-90.6440043974332));
#173498=CARTESIAN_POINT('Ctrl Pts',(39.0015855904073,-36.2710982035765,
-90.7396993298735));
#173499=CARTESIAN_POINT('Ctrl Pts',(39.0005031226411,-36.27413865878,-90.7976135569795));
#173500=CARTESIAN_POINT('Ctrl Pts',(39.0000009314936,-36.2771028717565,
-90.8540927106737));
#173501=CARTESIAN_POINT('Ctrl Pts',(39.0000000012937,-36.28000002,-90.9091273827666));
#173502=CARTESIAN_POINT('Origin',(57.,-37.28000002,-174.34995));
#173503=CARTESIAN_POINT('',(57.,-36.78000002,-176.84995));
#173504=CARTESIAN_POINT('Origin',(57.,-37.28000002,-176.84995));
#173505=CARTESIAN_POINT('',(59.5,-36.78000002,-174.34995));
#173506=CARTESIAN_POINT('Origin',(57.,-36.78000002,-174.34995));
#173507=CARTESIAN_POINT('Origin',(59.5,-37.28000002,-174.34995));
#173508=CARTESIAN_POINT('Origin',(59.5,-37.28000002,-55.24995));
#173509=CARTESIAN_POINT('',(59.5,-36.78000002,-58.24995));
#173510=CARTESIAN_POINT('',(59.5,-36.78000002,-174.34995));
#173511=CARTESIAN_POINT('Origin',(59.5,-37.28000002,-58.24995));
#173512=CARTESIAN_POINT('Ctrl Pts',(40.4661024946855,-36.78000002,-86.8949524600738));
#173513=CARTESIAN_POINT('Ctrl Pts',(39.7490326214953,-36.78000002,-86.5090582163831));
#173514=CARTESIAN_POINT('Ctrl Pts',(40.0734472163172,-36.0537915241817,
-86.6836433292035));
#173515=CARTESIAN_POINT('Ctrl Pts',(42.7671781583824,-36.78000002,-82.6190865682492));
#173516=CARTESIAN_POINT('Ctrl Pts',(42.0251435460116,-36.78000002,-82.3205925927599));
#173517=CARTESIAN_POINT('Ctrl Pts',(42.3689613408276,-36.0634493712886,
-82.407773086856));
#173518=CARTESIAN_POINT('Ctrl Pts',(45.0306161020287,-36.78000002,-78.3240684577782));
#173519=CARTESIAN_POINT('Ctrl Pts',(44.3122026972581,-36.7800000199999,
-78.0178858717772));
#173520=CARTESIAN_POINT('Ctrl Pts',(44.6279666698635,-36.0719269202766,
-78.1127593269182));
#173521=CARTESIAN_POINT('Ctrl Pts',(49.5095281828678,-36.78000002,-69.7096607994621));
#173522=CARTESIAN_POINT('Ctrl Pts',(48.8138634148613,-36.78000002,-69.420066134471));
#173523=CARTESIAN_POINT('Ctrl Pts',(49.0993449617391,-36.0872029629615,
-69.4983516685814));
#173524=CARTESIAN_POINT('Ctrl Pts',(51.7247198970815,-36.78000002,-65.3901198450985));
#173525=CARTESIAN_POINT('Ctrl Pts',(51.0452850559209,-36.7800000200001,
-65.0958859597511));
#173526=CARTESIAN_POINT('Ctrl Pts',(51.3114450013405,-36.0939978375791,
-65.1788088209436));
#173527=CARTESIAN_POINT('Ctrl Pts',(53.9233979868778,-36.78000002,-61.0621827299711));
#173528=CARTESIAN_POINT('Ctrl Pts',(53.2738374538033,-36.7800000199999,
-60.7321930665019));
#173529=CARTESIAN_POINT('Ctrl Pts',(53.5074514076768,-36.1001753985996,
-60.8508735991007));
#173530=CARTESIAN_POINT('',(53.5074514076768,-36.1001753985996,-60.8508735991007));
#173531=CARTESIAN_POINT('',(53.9233979868778,-36.78000002,-61.0621827299711));
#173532=CARTESIAN_POINT('Origin',(53.9233979868778,-36.28000002,-61.0621827299711));
#173533=CARTESIAN_POINT('',(40.4661024946855,-36.78000002,-86.8949524600738));
#173534=CARTESIAN_POINT('Ctrl Pts',(40.4661024946855,-36.78000002,-86.8949524600738));
#173535=CARTESIAN_POINT('Ctrl Pts',(42.7668758174593,-36.78000002,-82.6196483790844));
#173536=CARTESIAN_POINT('Ctrl Pts',(45.0302107640621,-36.78000002,-78.3248411901957));
#173537=CARTESIAN_POINT('Ctrl Pts',(47.2696870908413,-36.78000002,-74.0176051177503));
#173538=CARTESIAN_POINT('Ctrl Pts',(49.5091634176204,-36.78000002,-69.7103690453049));
#173539=CARTESIAN_POINT('Ctrl Pts',(51.7244980141576,-36.78000002,-65.3905566052077));
#173540=CARTESIAN_POINT('Ctrl Pts',(53.9233979868778,-36.78000002,-61.0621827299711));
#173541=CARTESIAN_POINT('Origin',(40.4661024946855,-36.28000002,-86.8949524600738));
#173542=CARTESIAN_POINT('Ctrl Pts',(53.5074514076768,-36.1001753985996,
-60.8508735991007));
#173543=CARTESIAN_POINT('Ctrl Pts',(52.7922585244569,-36.0981634975119,
-62.2603906482166));
#173544=CARTESIAN_POINT('Ctrl Pts',(52.087761822413,-36.0961532083163,-63.6445356363279));
#173545=CARTESIAN_POINT('Ctrl Pts',(51.3939147382574,-36.0941045783538,
-65.0032879478635));
#173546=CARTESIAN_POINT('Ctrl Pts',(50.9587608446394,-36.0928197573533,
-65.8554445286564));
#173547=CARTESIAN_POINT('Ctrl Pts',(50.5277967496853,-36.0915198832934,
-66.6976138903416));
#173548=CARTESIAN_POINT('Ctrl Pts',(50.101020147517,-36.0901953772584,-67.5297957986045));
#173549=CARTESIAN_POINT('Ctrl Pts',(49.547387044142,-36.0884771706303,-68.6093382339287));
#173550=CARTESIAN_POINT('Ctrl Pts',(49.0007983189538,-36.0867228439177,
-69.6720723858452));
#173551=CARTESIAN_POINT('Ctrl Pts',(48.461251821417,-36.0849437847744,-70.718001906085));
#173552=CARTESIAN_POINT('Ctrl Pts',(48.1914785726486,-36.0840542552027,
-71.240966666205));
#173553=CARTESIAN_POINT('Ctrl Pts',(47.9234660064517,-36.0831588800052,
-71.7597303678619));
#173554=CARTESIAN_POINT('Ctrl Pts',(47.6572144784549,-36.0822610994337,
-72.2742940187899));
#173555=CARTESIAN_POINT('Ctrl Pts',(47.5240887144565,-36.081812209148,-72.531575844254));
#173556=CARTESIAN_POINT('Ctrl Pts',(47.391403221895,-36.0813627242012,-72.7878076633787));
#173557=CARTESIAN_POINT('Ctrl Pts',(47.2591580668236,-36.0809132157062,
-73.0429896319059));
#173558=CARTESIAN_POINT('Ctrl Pts',(47.193035489288,-36.0806884614586,-73.1705806161696));
#173559=CARTESIAN_POINT('Ctrl Pts',(47.1270229967962,-36.0804637017278,
-73.2979091381477));
#173560=CARTESIAN_POINT('Ctrl Pts',(47.0611206002298,-36.0802390131329,
-73.4249752193029));
#173561=CARTESIAN_POINT('Ctrl Pts',(46.9993371034487,-36.0800283675751,
-73.5440996703859));
#173562=CARTESIAN_POINT('Ctrl Pts',(46.937650370691,-36.0798177845541,-73.6629934606037));
#173563=CARTESIAN_POINT('Ctrl Pts',(46.876060411837,-36.0796073308672,-73.7816566085978));
#173564=CARTESIAN_POINT('Ctrl Pts',(46.8719544145801,-36.0795933006214,
-73.7895674851308));
#173565=CARTESIAN_POINT('Ctrl Pts',(46.8684113527144,-36.0795811932909,
-73.7963936317983));
#173566=CARTESIAN_POINT('Ctrl Pts',(46.8637437084935,-36.0795652467564,
-73.8053861619924));
#173567=CARTESIAN_POINT('Ctrl Pts',(46.8637144102822,-36.079565146662,-73.8054426069651));
#173568=CARTESIAN_POINT('Ctrl Pts',(46.8636851120899,-36.0795650465676,
-73.8054990518909));
#173569=CARTESIAN_POINT('Ctrl Pts',(46.8636558139168,-36.0795649464731,
-73.80555549677));
#173570=CARTESIAN_POINT('Ctrl Pts',(46.2429826651902,-36.0774444738694,
-75.0013235981928));
#173571=CARTESIAN_POINT('Ctrl Pts',(45.6309093168581,-36.0752947306591,
-76.1761119836538));
#173572=CARTESIAN_POINT('Ctrl Pts',(45.0273544360468,-36.0731155201471,
-77.3298876420855));
#173573=CARTESIAN_POINT('Ctrl Pts',(44.4120213549676,-36.0708937829675,
-78.506178901337));
#173574=CARTESIAN_POINT('Ctrl Pts',(43.8055426292206,-36.0686414218454,
-79.6606294077665));
#173575=CARTESIAN_POINT('Ctrl Pts',(43.2078811739115,-36.066359429761,-80.7932300885606));
#173576=CARTESIAN_POINT('Ctrl Pts',(42.5897731390426,-36.0639993685084,
-81.9645781400002));
#173577=CARTESIAN_POINT('Ctrl Pts',(41.9810960802422,-36.0616076169725,
-83.1125558332997));
#173578=CARTESIAN_POINT('Ctrl Pts',(41.3818591117218,-36.0591864926988,
-84.2371795897531));
#173579=CARTESIAN_POINT('Ctrl Pts',(40.9405953429784,-36.0574036347014,
-85.0653256208907));
#173580=CARTESIAN_POINT('Ctrl Pts',(40.5044515400523,-36.0556048756295,
-85.8808085557189));
#173581=CARTESIAN_POINT('Ctrl Pts',(40.0734472163172,-36.0537915241817,
-86.6836433292035));
#173582=CARTESIAN_POINT('Ctrl Pts',(40.1309220332522,-36.0483277296961,
-86.5845687421098));
#173583=CARTESIAN_POINT('Ctrl Pts',(39.7968669198671,-36.7800000199995,
-86.3981771484168));
#173584=CARTESIAN_POINT('Ctrl Pts',(40.5178020946704,-36.78000002,-86.8005666302754));
#173585=CARTESIAN_POINT('Ctrl Pts',(39.7317438420182,-36.0850974253399,
-87.2612325210988));
#173586=CARTESIAN_POINT('Ctrl Pts',(39.4836336651727,-36.7800000200025,
-87.1082114503545));
#173587=CARTESIAN_POINT('Ctrl Pts',(40.1585088632339,-36.78000002,-87.4451185554427));
#173588=CARTESIAN_POINT('Ctrl Pts',(39.4528126178963,-36.1238332542013,
-87.9779440827562));
#173589=CARTESIAN_POINT('Ctrl Pts',(39.2579727974598,-36.7800000200001,
-87.8751206778157));
#173590=CARTESIAN_POINT('Ctrl Pts',(39.9075095278365,-36.78000002,-88.1269484527019));
#173591=CARTESIAN_POINT('Ctrl Pts',(39.0804486566366,-36.2039143776693,
-89.4721907623552));
#173592=CARTESIAN_POINT('Ctrl Pts',(39.0022563977957,-36.78000002,-89.4265019469593));
#173593=CARTESIAN_POINT('Ctrl Pts',(39.572394069454,-36.78000002,-89.5466301924888));
#173594=CARTESIAN_POINT('Ctrl Pts',(38.9910757956325,-36.2453106379154,
-90.2508802901019));
#173595=CARTESIAN_POINT('Ctrl Pts',(38.95517376435,-36.78000002,-90.2192417070188));
#173596=CARTESIAN_POINT('Ctrl Pts',(39.4919635455253,-36.78000002,-90.2855006253694));
#173597=CARTESIAN_POINT('Ctrl Pts',(39.0007023042009,-36.2858508900221,
-91.0217464384246));
#173598=CARTESIAN_POINT('Ctrl Pts',(39.0064880541292,-36.78000002,-91.0217157887641));
#173599=CARTESIAN_POINT('Ctrl Pts',(39.5006328637826,-36.78000002,-91.0158318926359));
#173600=CARTESIAN_POINT('',(39.5,-36.78000002,-90.9091273827666));
#173601=CARTESIAN_POINT('Ctrl Pts',(39.5,-36.78000002,-90.9091273827666));
#173602=CARTESIAN_POINT('Ctrl Pts',(39.5,-36.78000002,-90.7679100061199));
#173603=CARTESIAN_POINT('Ctrl Pts',(39.5033096444594,-36.7800000200224,
-90.6269761431631));
#173604=CARTESIAN_POINT('Ctrl Pts',(39.5098707684965,-36.7800000197587,
-90.486327108651));
#173605=CARTESIAN_POINT('Ctrl Pts',(39.5164908621434,-36.7800000194927,
-90.3444139586241));
#173606=CARTESIAN_POINT('Ctrl Pts',(39.5264211472599,-36.7800000188623,
-90.2027900769916));
#173607=CARTESIAN_POINT('Ctrl Pts',(39.5396544427955,-36.7800000184551,
-90.0614520511831));
#173608=CARTESIAN_POINT('Ctrl Pts',(39.5457621647723,-36.7800000182671,
-89.9962186129912));
#173609=CARTESIAN_POINT('Ctrl Pts',(39.5525742276005,-36.780000018147,-89.9310460673889));
#173610=CARTESIAN_POINT('Ctrl Pts',(39.5600936571067,-36.7800000181768,
-89.8659343821325));
#173611=CARTESIAN_POINT('Ctrl Pts',(39.5772069508045,-36.7800000182445,
-89.7177482209293));
#173612=CARTESIAN_POINT('Ctrl Pts',(39.5980137125872,-36.7800000189104,
-89.569651212335));
#173613=CARTESIAN_POINT('Ctrl Pts',(39.6224903903715,-36.7800000193564,
-89.4222267568301));
#173614=CARTESIAN_POINT('Ctrl Pts',(39.646759527969,-36.7800000197985,-89.276052327955));
#173615=CARTESIAN_POINT('Ctrl Pts',(39.6746364995121,-36.780000019972,-89.1305398192698));
#173616=CARTESIAN_POINT('Ctrl Pts',(39.7060481712977,-36.780000019994,-88.9862487847489));
#173617=CARTESIAN_POINT('Ctrl Pts',(39.7169272984727,-36.7800000200016,
-88.9362749875731));
#173618=CARTESIAN_POINT('Ctrl Pts',(39.7282299820615,-36.78000002,-88.8864475773885));
#173619=CARTESIAN_POINT('Ctrl Pts',(39.7399518035734,-36.78000002,-88.8367893012138));
#173620=CARTESIAN_POINT('Ctrl Pts',(39.8212039955519,-36.78000002,-88.4925728511548));
#173621=CARTESIAN_POINT('Ctrl Pts',(39.9220601466511,-36.78000002,-88.1550003033774));
#173622=CARTESIAN_POINT('Ctrl Pts',(40.0453748819428,-36.78000002,-87.8250390461133));
#173623=CARTESIAN_POINT('Ctrl Pts',(40.16398080735,-36.78000002,-87.5076774577049));
#173624=CARTESIAN_POINT('Ctrl Pts',(40.3033623181985,-36.78000002,-87.1973567576874));
#173625=CARTESIAN_POINT('Ctrl Pts',(40.4661024946855,-36.78000002,-86.8949524600739));
#173626=CARTESIAN_POINT('Origin',(39.5,-36.28000002,-90.9091273827666));
#173627=CARTESIAN_POINT('Origin',(39.5,-36.28000002,-55.24995));
#173628=CARTESIAN_POINT('',(39.5,-36.78000002,-141.149515588739));
#173629=CARTESIAN_POINT('',(39.5,-36.78000002,-55.24995));
#173630=CARTESIAN_POINT('Origin',(39.5,-36.28000002,-141.149515588739));
#173631=CARTESIAN_POINT('Ctrl Pts',(39.,-36.28000002,-141.149515588739));
#173632=CARTESIAN_POINT('Ctrl Pts',(38.9999999999999,-36.78000002,-141.149515588739));
#173633=CARTESIAN_POINT('Ctrl Pts',(39.5,-36.78000002,-141.149515588739));
#173634=CARTESIAN_POINT('Ctrl Pts',(39.,-36.2411525212205,-141.887468602714));
#173635=CARTESIAN_POINT('Ctrl Pts',(38.9595709612524,-36.78000002,-141.917511819575));
#173636=CARTESIAN_POINT('Ctrl Pts',(39.5000000020403,-36.78000002,-141.848776286889));
#173637=CARTESIAN_POINT('Ctrl Pts',(39.0877747262142,-36.202664552653,-142.611197003283));
#173638=CARTESIAN_POINT('Ctrl Pts',(39.0069624314851,-36.78000002,-142.654181226843));
#173639=CARTESIAN_POINT('Ctrl Pts',(39.5789972525929,-36.78000002,-142.535527260215));
#173640=CARTESIAN_POINT('Ctrl Pts',(39.4389223885666,-36.1266531472167,
-144.029685314679));
#173641=CARTESIAN_POINT('Ctrl Pts',(39.2475606867303,-36.78000002,-144.126025522057));
#173642=CARTESIAN_POINT('Ctrl Pts',(39.8950301507098,-36.78000002,-143.883204247708));
#173643=CARTESIAN_POINT('Ctrl Pts',(39.7059668714196,-36.0888399354841,
-144.729666200452));
#173644=CARTESIAN_POINT('Ctrl Pts',(39.4615987310595,-36.78000002,-144.873235586497));
#173645=CARTESIAN_POINT('Ctrl Pts',(40.1353628336737,-36.78000002,-144.549109040068));
#173646=CARTESIAN_POINT('Ctrl Pts',(40.0734472163172,-36.0537915241817,
-145.374999642303));
#173647=CARTESIAN_POINT('Ctrl Pts',(39.7490326214954,-36.78000002,-145.549584755123));
#173648=CARTESIAN_POINT('Ctrl Pts',(40.4661024946855,-36.78000002,-145.163690511432));
#173649=CARTESIAN_POINT('',(40.4661024946856,-36.78000002,-145.163690511432));
#173650=CARTESIAN_POINT('Ctrl Pts',(40.4661024946855,-36.78000002,-145.163690511432));
#173651=CARTESIAN_POINT('Ctrl Pts',(40.4051245273351,-36.78000002,-145.05038106453));
#173652=CARTESIAN_POINT('Ctrl Pts',(40.3473970436746,-36.78000002,-144.935666150371));
#173653=CARTESIAN_POINT('Ctrl Pts',(40.2927291183489,-36.78000002,-144.819632460354));
#173654=CARTESIAN_POINT('Ctrl Pts',(40.2359907375988,-36.78000002,-144.699204190123));
#173655=CARTESIAN_POINT('Ctrl Pts',(40.182547909167,-36.78000002,-144.577354792971));
#173656=CARTESIAN_POINT('Ctrl Pts',(40.1322366185222,-36.78000002,-144.454153170975));
#173657=CARTESIAN_POINT('Ctrl Pts',(40.0991220934988,-36.78000002,-144.373062760806));
#173658=CARTESIAN_POINT('Ctrl Pts',(40.0673652289501,-36.78000002,-144.291385980202));
#173659=CARTESIAN_POINT('Ctrl Pts',(40.0369306905871,-36.78000002,-144.209138150939));
#173660=CARTESIAN_POINT('Ctrl Pts',(39.9567208320406,-36.78000002,-143.99237498955));
#173661=CARTESIAN_POINT('Ctrl Pts',(39.8859370924984,-36.78000002,-143.772269498041));
#173662=CARTESIAN_POINT('Ctrl Pts',(39.8243406671238,-36.78000002,-143.550546349406));
#173663=CARTESIAN_POINT('Ctrl Pts',(39.7928424603809,-36.78000002,-143.437165069032));
#173664=CARTESIAN_POINT('Ctrl Pts',(39.7637458267515,-36.78000002,-143.323361070991));
#173665=CARTESIAN_POINT('Ctrl Pts',(39.737013701299,-36.78000002,-143.209365754044));
#173666=CARTESIAN_POINT('Ctrl Pts',(39.6399004481884,-36.78000002,-142.795240207321));
#173667=CARTESIAN_POINT('Ctrl Pts',(39.5726401857881,-36.78000002,-142.376286688206));
#173668=CARTESIAN_POINT('Ctrl Pts',(39.5352116792707,-36.78000002,-141.952508599874));
#173669=CARTESIAN_POINT('Ctrl Pts',(39.5117389237049,-36.78000002,-141.686742198618));
#173670=CARTESIAN_POINT('Ctrl Pts',(39.5000000000007,-36.78000002,-141.41907812932));
#173671=CARTESIAN_POINT('Ctrl Pts',(39.5,-36.78000002,-141.149515588739));
#173672=CARTESIAN_POINT('Origin',(40.4661024946856,-36.28000002,-145.163690511432));
#173673=CARTESIAN_POINT('Ctrl Pts',(54.061590101286,-36.78000002,-171.268536075449));
#173674=CARTESIAN_POINT('Ctrl Pts',(53.4125141483451,-36.78000002,-171.598146859086));
#173675=CARTESIAN_POINT('Ctrl Pts',(53.6454853125448,-36.1005363232099,
-171.479840562953));
#173676=CARTESIAN_POINT('Ctrl Pts',(51.8377538941353,-36.78000002,-166.889319970653));
#173677=CARTESIAN_POINT('Ctrl Pts',(51.1583704358619,-36.7800000200002,
-167.182444881139));
#173678=CARTESIAN_POINT('Ctrl Pts',(51.4243352023986,-36.0943124607371,
-167.100627882666));
#173679=CARTESIAN_POINT('Ctrl Pts',(49.5972294079553,-36.78000002,-162.518792058211));
#173680=CARTESIAN_POINT('Ctrl Pts',(48.9013482881149,-36.7800000199664,
-162.806967721366));
#173681=CARTESIAN_POINT('Ctrl Pts',(49.1869218186486,-36.0874610318388,
-162.730098242847));
#173682=CARTESIAN_POINT('Ctrl Pts',(45.066960038919,-36.78000002,-153.803374490657));
#173683=CARTESIAN_POINT('Ctrl Pts',(44.348109595875,-36.7800000200345,-154.108244930852));
#173684=CARTESIAN_POINT('Ctrl Pts',(44.6642494092406,-36.072038540157,-154.01468012643));
#173685=CARTESIAN_POINT('Ctrl Pts',(42.777508353219,-36.78000002,-149.458325760535));
#173686=CARTESIAN_POINT('Ctrl Pts',(42.0345588527891,-36.7800000199998,
-149.755027455429));
#173687=CARTESIAN_POINT('Ctrl Pts',(42.3792743432826,-36.0634712454522,
-149.669636259109));
#173688=CARTESIAN_POINT('Ctrl Pts',(40.4497212107858,-36.78000002,-145.133252264122));
#173689=CARTESIAN_POINT('Ctrl Pts',(39.7324960674638,-36.78000002,-145.519268764292));
#173690=CARTESIAN_POINT('Ctrl Pts',(40.0571172805695,-36.0536964873408,
-145.34455504538));
#173691=CARTESIAN_POINT('',(54.0459394689003,-36.78000002,-171.237717270032));
#173692=CARTESIAN_POINT('Ctrl Pts',(54.0459394689003,-36.78000002,-171.237717270032));
#173693=CARTESIAN_POINT('Ctrl Pts',(51.8272412193298,-36.78000002,-166.868813514854));
#173694=CARTESIAN_POINT('Ctrl Pts',(49.5919157423625,-36.78000002,-162.508569528244));
#173695=CARTESIAN_POINT('Ctrl Pts',(47.3320947234338,-36.78000002,-158.161083274436));
#173696=CARTESIAN_POINT('Ctrl Pts',(45.0722737045051,-36.78000002,-153.813597020627));
#173697=CARTESIAN_POINT('Ctrl Pts',(42.7882516015473,-36.78000002,-149.478715140467));
#173698=CARTESIAN_POINT('Ctrl Pts',(40.4661024946855,-36.78000002,-145.163690511432));
#173699=CARTESIAN_POINT('Origin',(54.0459394689003,-36.28000002,-171.237717270032));
#173700=CARTESIAN_POINT('Ctrl Pts',(54.1985583159464,-36.7800000191852,
-171.906167818556));
#173701=CARTESIAN_POINT('Ctrl Pts',(53.439506223589,-36.7800433691512,-171.887030357476));
#173702=CARTESIAN_POINT('Ctrl Pts',(53.7393383808297,-36.082487169742,-171.894658379215));
#173703=CARTESIAN_POINT('Ctrl Pts',(54.2046305452548,-36.7800000191843,
-171.662933242572));
#173704=CARTESIAN_POINT('Ctrl Pts',(53.4406325939144,-36.7800434674344,
-171.77861312897));
#173705=CARTESIAN_POINT('Ctrl Pts',(53.7436938429465,-36.0817727411105,
-171.732515491476));
#173706=CARTESIAN_POINT('Ctrl Pts',(54.1464425180027,-36.7800000191923,
-171.423436673455));
#173707=CARTESIAN_POINT('Ctrl Pts',(53.4304080193293,-36.7800425499783,
-171.672542976743));
#173708=CARTESIAN_POINT('Ctrl Pts',(53.7019584052344,-36.0886165914289,
-171.572834421448));
#173709=CARTESIAN_POINT('Ctrl Pts',(54.0297882222771,-36.7800000192084,
-171.206777509126));
#173710=CARTESIAN_POINT('Ctrl Pts',(53.3916114660656,-36.7800408062075,
-171.550460731129));
#173711=CARTESIAN_POINT('Ctrl Pts',(53.6182347475101,-36.1024349685033,
-171.42841039456));
#173712=CARTESIAN_POINT('',(54.1989607257493,-36.78000002,-171.871644662643));
#173713=CARTESIAN_POINT('Origin',(52.6055188870422,-36.7800000520242,-171.864725026498));
#173714=CARTESIAN_POINT('Origin',(54.1989607257493,-36.28000002,-171.871644662643));
#173715=CARTESIAN_POINT('Origin',(54.1989607257493,-36.28000002,-179.64995));
#173716=CARTESIAN_POINT('',(54.1989607257493,-36.78000002,-171.871644662643));
#173717=CARTESIAN_POINT('',(53.7396474992599,-36.0824364606782,-179.64995));
#173718=CARTESIAN_POINT('Origin',(60.,-37.28000002,-176.84995));
#173719=CARTESIAN_POINT('',(-83.2809572255632,-36.78000002,-176.84995));
#173720=CARTESIAN_POINT('Origin',(57.,-37.28000002,-58.24995));
#173721=CARTESIAN_POINT('',(57.,-36.78000002,-55.74995));
#173722=CARTESIAN_POINT('Origin',(57.,-36.78000002,-58.24995));
#173723=CARTESIAN_POINT('',(57.,-37.28000002,-55.24995));
#173724=CARTESIAN_POINT('Origin',(57.,-37.28000002,-55.74995));
#173725=CARTESIAN_POINT('Origin',(57.,-37.28000002,-58.24995));
#173726=CARTESIAN_POINT('Origin',(57.,-2.42462934179819E-14,-58.24995));
#173727=CARTESIAN_POINT('',(57.,-37.78000002,-55.24995));
#173728=CARTESIAN_POINT('',(57.,28.41999998,-55.24995));
#173729=CARTESIAN_POINT('Origin',(57.,-37.78000002,-58.24995));
#173730=CARTESIAN_POINT('Origin',(57.,-37.78000002,-58.24995));
#173731=CARTESIAN_POINT('',(57.,-38.28000002,-55.74995));
#173732=CARTESIAN_POINT('Origin',(57.,-37.78000002,-55.74995));
#173733=CARTESIAN_POINT('Origin',(57.,-38.28000002,-58.24995));
#173734=CARTESIAN_POINT('Origin',(57.,11.61999998,-58.24995));
#173735=CARTESIAN_POINT('',(57.,12.11999998,-55.74995));
#173736=CARTESIAN_POINT('Origin',(57.,12.11999998,-58.24995));
#173737=CARTESIAN_POINT('',(57.,11.61999998,-55.24995));
#173738=CARTESIAN_POINT('Origin',(57.,11.61999998,-55.74995));
#173739=CARTESIAN_POINT('Origin',(57.,11.61999998,-58.24995));
#173740=CARTESIAN_POINT('Origin',(57.,-2.42462934179819E-14,-58.24995));
#173741=CARTESIAN_POINT('',(57.,11.11999998,-55.24995));
#173742=CARTESIAN_POINT('',(57.,28.41999998,-55.24995));
#173743=CARTESIAN_POINT('Origin',(57.,11.11999998,-58.24995));
#173744=CARTESIAN_POINT('Origin',(57.,11.11999998,-58.24995));
#173745=CARTESIAN_POINT('',(57.,10.61999998,-55.74995));
#173746=CARTESIAN_POINT('Origin',(57.,11.11999998,-55.74995));
#173747=CARTESIAN_POINT('Origin',(57.,10.61999998,-58.24995));
#173748=CARTESIAN_POINT('Ctrl Pts',(5.,45.5214348882082,-61.0621827299711));
#173749=CARTESIAN_POINT('Ctrl Pts',(5.,45.1055585268383,-60.8674008824013));
#173750=CARTESIAN_POINT('Ctrl Pts',(5.45757488824865,45.0702713246265,-60.8508735991007));
#173751=CARTESIAN_POINT('Ctrl Pts',(5.,40.8246742459034,-71.0901794372786));
#173752=CARTESIAN_POINT('Ctrl Pts',(5.00000000013405,40.426315064797,-70.8653394730463));
#173753=CARTESIAN_POINT('Ctrl Pts',(5.45419794131935,40.3738290579191,-70.8788685457756));
#173754=CARTESIAN_POINT('Ctrl Pts',(5.,36.1242566254946,-81.1164625478583));
#173755=CARTESIAN_POINT('Ctrl Pts',(5.00000000003379,35.7394456595583,-80.8717315350143));
#173756=CARTESIAN_POINT('Ctrl Pts',(5.4500940393161,35.6738220550387,-80.9051511012611));
#173757=CARTESIAN_POINT('Ctrl Pts',(5.,31.4150905187971,-91.1386408691297));
#173758=CARTESIAN_POINT('Ctrl Pts',(4.99999999999999,31.0104747491644,-90.9485222334823));
#173759=CARTESIAN_POINT('Ctrl Pts',(5.44427033638569,30.9653765476951,-90.9273317382593));
#173760=CARTESIAN_POINT('',(5.,45.5214348882082,-61.062182729971));
#173761=CARTESIAN_POINT('',(5.45757488824865,45.0702713246265,-60.8508735991007));
#173762=CARTESIAN_POINT('Origin',(5.5,45.5214348882082,-61.062182729971));
#173763=CARTESIAN_POINT('',(5.44427033638568,30.9653765476951,-90.9273317382593));
#173764=CARTESIAN_POINT('Ctrl Pts',(5.44427033638568,30.9653765476951,-90.9273317382593));
#173765=CARTESIAN_POINT('Ctrl Pts',(5.44561970702987,32.0563384739202,-88.6051603388755));
#173766=CARTESIAN_POINT('Ctrl Pts',(5.44696375827399,33.1898917997868,-86.1910626080188));
#173767=CARTESIAN_POINT('Ctrl Pts',(5.44885264917258,34.9541150607098,-82.4320265145244));
#173768=CARTESIAN_POINT('Ctrl Pts',(5.44976896906513,35.8521997505521,-80.5180360934748));
#173769=CARTESIAN_POINT('Ctrl Pts',(5.45080151723396,36.927917076703,-78.2247206138878));
#173770=CARTESIAN_POINT('Ctrl Pts',(5.45131315589655,37.4727634355675,-77.062981210337));
#173771=CARTESIAN_POINT('Ctrl Pts',(5.45160037064691,37.7812047612991,-76.4052610779079));
#173772=CARTESIAN_POINT('Ctrl Pts',(5.45174164230917,37.9336020084846,-76.0802730329389));
#173773=CARTESIAN_POINT('Ctrl Pts',(5.45181457454894,38.0124146208361,-75.9122006235131));
#173774=CARTESIAN_POINT('Ctrl Pts',(5.45181971490317,38.0179701347131,-75.9003531509149));
#173775=CARTESIAN_POINT('Ctrl Pts',(5.45385962122421,40.2228504311467,-71.1983046079137));
#173776=CARTESIAN_POINT('Ctrl Pts',(5.45577865562035,42.5721856437188,-66.1848666861869));
#173777=CARTESIAN_POINT('Ctrl Pts',(5.45757488824865,45.0702713246265,-60.8508735991007));
#173778=CARTESIAN_POINT('',(5.,31.415090518797,-91.1386408691297));
#173779=CARTESIAN_POINT('Origin',(5.5,31.415090518797,-91.1386408691297));
#173780=CARTESIAN_POINT('Ctrl Pts',(5.,45.5214348882082,-61.0621827299711));
#173781=CARTESIAN_POINT('Ctrl Pts',(5.,40.8246742459034,-71.0901794372786));
#173782=CARTESIAN_POINT('Ctrl Pts',(5.,36.1242566254946,-81.1164625478583));
#173783=CARTESIAN_POINT('Ctrl Pts',(5.,31.4150905187971,-91.1386408691297));
#173784=CARTESIAN_POINT('Ctrl Pts',(12.,30.2507177004773,-91.1386408691297));
#173785=CARTESIAN_POINT('Ctrl Pts',(12.,29.679733250215,-90.8631216114043));
#173786=CARTESIAN_POINT('Ctrl Pts',(11.3834743397155,29.812801930373,-90.9273317382593));
#173787=CARTESIAN_POINT('Ctrl Pts',(12.,35.0807977947169,-81.1288119730547));
#173788=CARTESIAN_POINT('Ctrl Pts',(11.9999999998861,34.4484178829812,-81.0174669870403));
#173789=CARTESIAN_POINT('Ctrl Pts',(11.3956361798112,34.6396513996494,-80.9174913671817));
#173790=CARTESIAN_POINT('Ctrl Pts',(12.,39.8700921493796,-71.0994291820815));
#173791=CARTESIAN_POINT('Ctrl Pts',(11.9999999999222,39.2806183751482,-70.92559601425));
#173792=CARTESIAN_POINT('Ctrl Pts',(11.4042255504145,39.4271199662976,-70.8881122426161));
#173793=CARTESIAN_POINT('Ctrl Pts',(12.,44.6428767076058,-61.062182729971));
#173794=CARTESIAN_POINT('Ctrl Pts',(12.,44.102645384174,-60.8052987597771));
#173795=CARTESIAN_POINT('Ctrl Pts',(11.4112929481563,44.1984900402045,-60.8508735991007));
#173796=CARTESIAN_POINT('',(11.4112929481563,44.1984900402045,-60.8508735991007));
#173797=CARTESIAN_POINT('',(12.,44.6428767076058,-61.062182729971));
#173798=CARTESIAN_POINT('Origin',(11.5,44.6428767076058,-61.062182729971));
#173799=CARTESIAN_POINT('',(12.,30.2507177004773,-91.1386408691297));
#173800=CARTESIAN_POINT('Ctrl Pts',(12.,30.2507177004773,-91.1386408691297));
#173801=CARTESIAN_POINT('Ctrl Pts',(12.,35.0808027196733,-81.1288017666047));
#173802=CARTESIAN_POINT('Ctrl Pts',(12.,39.8700874953717,-71.0994389691951));
#173803=CARTESIAN_POINT('Ctrl Pts',(12.,44.6428767076058,-61.062182729971));
#173804=CARTESIAN_POINT('',(11.3834743397155,29.812801930373,-90.9273317382593));
#173805=CARTESIAN_POINT('Origin',(11.5,30.2507177004773,-91.1386408691297));
#173806=CARTESIAN_POINT('Ctrl Pts',(11.4112929481563,44.1984900402045,-60.8508735991007));
#173807=CARTESIAN_POINT('Ctrl Pts',(11.4094109984326,42.9279405506231,-63.5236506500919));
#173808=CARTESIAN_POINT('Ctrl Pts',(11.4075038463216,41.6949692901581,-66.1140437492198));
#173809=CARTESIAN_POINT('Ctrl Pts',(11.4044750232958,39.9018903158517,-69.876057470117));
#173810=CARTESIAN_POINT('Ctrl Pts',(11.4029232381826,39.0194448925056,-71.7261703486169));
#173811=CARTESIAN_POINT('Ctrl Pts',(11.4010679295011,38.0145870304699,-73.8305709051232));
#173812=CARTESIAN_POINT('Ctrl Pts',(11.4001352611225,37.5183227466879,-74.8692550662738));
#173813=CARTESIAN_POINT('Ctrl Pts',(11.3996102114504,37.2409077632026,-75.4497134989859));
#173814=CARTESIAN_POINT('Ctrl Pts',(11.3993518934088,37.1049529011707,-75.7341278491348));
#173815=CARTESIAN_POINT('Ctrl Pts',(11.3992186208999,37.0349202316132,-75.8806206533949));
#173816=CARTESIAN_POINT('Ctrl Pts',(11.3992115364803,37.0311977944665,-75.8884071252557));
#173817=CARTESIAN_POINT('Ctrl Pts',(11.3943001013229,34.4508453562602,-81.2858634887265));
#173818=CARTESIAN_POINT('Ctrl Pts',(11.3891021666564,32.0464009004938,-86.2953312405831));
#173819=CARTESIAN_POINT('Ctrl Pts',(11.3834743397155,29.812801930373,-90.9273317382593));
#173820=CARTESIAN_POINT('Ctrl Pts',(13.5,29.5462485400348,-91.058247935017));
#173821=CARTESIAN_POINT('Ctrl Pts',(13.5,29.2108963546553,-90.8936099040706));
#173822=CARTESIAN_POINT('Ctrl Pts',(13.8582614853459,29.115831713372,-90.8469388041467));
#173823=CARTESIAN_POINT('Ctrl Pts',(13.5,29.5320844445084,-91.0870988658315));
#173824=CARTESIAN_POINT('Ctrl Pts',(13.5,29.1946688455411,-90.923776404174));
#173825=CARTESIAN_POINT('Ctrl Pts',(13.8598257678503,29.1000938294036,-90.8779461296248));
#173826=CARTESIAN_POINT('Ctrl Pts',(13.5,29.518158585283,-91.1160643410222));
#173827=CARTESIAN_POINT('Ctrl Pts',(13.4999999999997,29.1787031940904,-90.9540383533105));
#173828=CARTESIAN_POINT('Ctrl Pts',(13.8613943096149,29.0846206527093,-90.9090791787867));
#173829=CARTESIAN_POINT('Ctrl Pts',(13.5,29.5044693674792,-91.1451435916293));
#173830=CARTESIAN_POINT('Ctrl Pts',(13.5,29.1629965026825,-90.9843933533492));
#173831=CARTESIAN_POINT('Ctrl Pts',(13.8629670146618,29.0694104105324,-90.9403371832586));
#173832=CARTESIAN_POINT('',(13.5,29.5462485400348,-91.058247935017));
#173833=CARTESIAN_POINT('',(13.8582614743845,29.1158316800856,-90.8469387878052));
#173834=CARTESIAN_POINT('Origin',(14.,29.5462485400348,-91.058247935017));
#173835=CARTESIAN_POINT('',(13.8629628324617,29.0693971421497,-90.9403366624458));
#173836=CARTESIAN_POINT('Origin',(13.9259921622961,31.8088924073546,-92.6508709683574));
#173837=CARTESIAN_POINT('',(13.5,29.5044693674792,-91.1451435916293));
#173838=CARTESIAN_POINT('Origin',(14.,29.5044693674792,-91.1451435916293));
#173839=CARTESIAN_POINT('Ctrl Pts',(13.5,29.5462485400348,-91.058247935017));
#173840=CARTESIAN_POINT('Ctrl Pts',(13.5,29.5320849211775,-91.0870978945881));
#173841=CARTESIAN_POINT('Ctrl Pts',(13.5,29.5181581265359,-91.1160653155133));
#173842=CARTESIAN_POINT('Ctrl Pts',(13.5,29.5044693674792,-91.1451435916293));
#173843=CARTESIAN_POINT('Ctrl Pts',(13.5,44.086908282047,-61.0621827299711));
#173844=CARTESIAN_POINT('Ctrl Pts',(13.5,43.724980245498,-60.8884062566336));
#173845=CARTESIAN_POINT('Ctrl Pts',(13.8920088064511,43.6468101642065,-60.8508735991007));
#173846=CARTESIAN_POINT('Ctrl Pts',(13.5,39.2774015744131,-71.0790468430123));
#173847=CARTESIAN_POINT('Ctrl Pts',(13.5,38.9561333124887,-70.8371780085667));
#173848=CARTESIAN_POINT('Ctrl Pts',(13.883422492558,38.8394158858892,-70.8677262129548));
#173849=CARTESIAN_POINT('Ctrl Pts',(13.5,34.4430593692808,-81.0839048048873));
#173850=CARTESIAN_POINT('Ctrl Pts',(13.5000000000877,34.1527775267561,-80.7999951426717));
#173851=CARTESIAN_POINT('Ctrl Pts',(13.8729900235566,34.0078012896411,-80.8725774805421));
#173852=CARTESIAN_POINT('Ctrl Pts',(13.5,29.5462485400348,-91.058247935017));
#173853=CARTESIAN_POINT('Ctrl Pts',(13.5,29.2108963546553,-90.8936099040706));
#173854=CARTESIAN_POINT('Ctrl Pts',(13.8582614853459,29.115831713372,-90.8469388041467));
#173855=CARTESIAN_POINT('',(13.5,44.086908282047,-61.0621827299711));
#173856=CARTESIAN_POINT('',(13.8920088064511,43.6468101642065,-60.8508735991007));
#173857=CARTESIAN_POINT('Origin',(14.,44.086908282047,-61.0621827299711));
#173858=CARTESIAN_POINT('Ctrl Pts',(13.8582614853459,29.115831713372,-90.8469388041467));
#173859=CARTESIAN_POINT('Ctrl Pts',(13.8606694674642,29.9156242721724,-89.2162213924719));
#173860=CARTESIAN_POINT('Ctrl Pts',(13.8630372008162,30.7386522803969,-87.534015044631));
#173861=CARTESIAN_POINT('Ctrl Pts',(13.8653554193648,31.584799169861,-85.8002497556502));
#173862=CARTESIAN_POINT('Ctrl Pts',(13.8675774780501,32.3958478287453,-84.1384011688891));
#173863=CARTESIAN_POINT('Ctrl Pts',(13.8697540270431,33.2281369500207,-82.4291821376903));
#173864=CARTESIAN_POINT('Ctrl Pts',(13.8718797439041,34.0816065397358,-80.6725529454259));
#173865=CARTESIAN_POINT('Ctrl Pts',(13.8738910205824,34.8891287045455,-79.0104937166035));
#173866=CARTESIAN_POINT('Ctrl Pts',(13.8758567874135,35.7156127493098,-77.3059903174534));
#173867=CARTESIAN_POINT('Ctrl Pts',(13.8777752709462,36.5610466523927,-75.5590348924101));
#173868=CARTESIAN_POINT('Ctrl Pts',(13.8796481768889,37.3863955043561,-73.8535820483342));
#173869=CARTESIAN_POINT('Ctrl Pts',(13.8814760018982,38.2298035907086,-72.1076716166056));
#173870=CARTESIAN_POINT('Ctrl Pts',(13.8832599520145,39.0913013121694,-70.3213206281249));
#173871=CARTESIAN_POINT('Ctrl Pts',(13.8849797115563,39.9218003901471,-68.5992466029468));
#173872=CARTESIAN_POINT('Ctrl Pts',(13.8866586900895,40.7691106156835,-66.8395898988203));
#173873=CARTESIAN_POINT('Ctrl Pts',(13.8883008096956,41.6333016406227,-65.042387541687));
#173874=CARTESIAN_POINT('Ctrl Pts',(13.8895573392646,42.2945699015106,-63.6671905738076));
#173875=CARTESIAN_POINT('Ctrl Pts',(13.8907923409499,42.965722872781,-62.2700105827591));
#173876=CARTESIAN_POINT('Ctrl Pts',(13.8920088064511,43.6468101642066,-60.8508735991007));
#173877=CARTESIAN_POINT('Ctrl Pts',(13.5,44.086908282047,-61.0621827299711));
#173878=CARTESIAN_POINT('Ctrl Pts',(13.5,39.2774232822218,-71.079001631676));
#173879=CARTESIAN_POINT('Ctrl Pts',(13.5,34.4431166252676,-81.0837881795346));
#173880=CARTESIAN_POINT('Ctrl Pts',(13.5,29.5462485400348,-91.058247935017));
#173881=CARTESIAN_POINT('Ctrl Pts',(20.5,29.726759920701,-85.9392854774869));
#173882=CARTESIAN_POINT('Ctrl Pts',(20.5,29.0600890554149,-85.5959926642051));
#173883=CARTESIAN_POINT('Ctrl Pts',(19.8077680666402,29.3163999141123,-85.7279763466165));
#173884=CARTESIAN_POINT('Ctrl Pts',(20.5,33.9784532599698,-77.6825438045949));
#173885=CARTESIAN_POINT('Ctrl Pts',(20.5000000001728,33.2278557603418,-77.5610859264982));
#173886=CARTESIAN_POINT('Ctrl Pts',(19.8234665452012,33.5607487699413,-77.4712163753771));
#173887=CARTESIAN_POINT('Ctrl Pts',(20.5,38.1440461521965,-69.3822166533219));
#173888=CARTESIAN_POINT('Ctrl Pts',(20.5000000002289,37.4529027206824,-69.1923113693162));
#173889=CARTESIAN_POINT('Ctrl Pts',(19.8355385600285,37.7216554195719,-69.1708971047811));
#173890=CARTESIAN_POINT('Ctrl Pts',(20.5,42.270218132516,-61.0621827299711));
#173891=CARTESIAN_POINT('Ctrl Pts',(20.5,41.6540022187559,-60.7565814715328));
#173892=CARTESIAN_POINT('Ctrl Pts',(19.8457268663587,41.8441333387867,-60.8508735991007));
#173893=CARTESIAN_POINT('',(19.8457268663587,41.8441333387867,-60.8508735991007));
#173894=CARTESIAN_POINT('',(20.5,42.270218132516,-61.0621827299711));
#173895=CARTESIAN_POINT('Origin',(20.,42.270218132516,-61.0621827299711));
#173896=CARTESIAN_POINT('',(20.5,29.726759920701,-85.9392854774869));
#173897=CARTESIAN_POINT('Ctrl Pts',(20.5,29.726759920701,-85.9392854774869));
#173898=CARTESIAN_POINT('Ctrl Pts',(20.5,33.9784770268254,-77.682497649623));
#173899=CARTESIAN_POINT('Ctrl Pts',(20.5,38.1440239783714,-69.3822613645965));
#173900=CARTESIAN_POINT('Ctrl Pts',(20.5,42.270218132516,-61.0621827299711));
#173901=CARTESIAN_POINT('',(19.8077681423597,29.3163998849126,-85.7279763868962));
#173902=CARTESIAN_POINT('Origin',(20.,29.726759920701,-85.9392854774869));
#173903=CARTESIAN_POINT('Ctrl Pts',(19.8457268663587,41.8441333387867,-60.8508735991007));
#173904=CARTESIAN_POINT('Ctrl Pts',(19.8438917319593,41.101585869444,-62.3494898488539));
#173905=CARTESIAN_POINT('Ctrl Pts',(19.8420266925439,40.3704767068203,-63.8218555336744));
#173906=CARTESIAN_POINT('Ctrl Pts',(19.8401287326225,39.6506919358387,-65.2679151976064));
#173907=CARTESIAN_POINT('Ctrl Pts',(19.8381885441163,38.9148923418786,-66.7461489092091));
#173908=CARTESIAN_POINT('Ctrl Pts',(19.8362139596767,38.1909268139742,-68.1968930645251));
#173909=CARTESIAN_POINT('Ctrl Pts',(19.8342035897005,37.4787222386946,-69.620114247757));
#173910=CARTESIAN_POINT('Ctrl Pts',(19.832114429525,36.73860501991,-71.0991141593137));
#173911=CARTESIAN_POINT('Ctrl Pts',(19.8299866260592,36.0111887347363,-72.5483914937309));
#173912=CARTESIAN_POINT('Ctrl Pts',(19.8278205210925,35.2964419024826,-73.9679356449112));
#173913=CARTESIAN_POINT('Ctrl Pts',(19.8256028260814,34.5646719704813,-75.4212890283832));
#173914=CARTESIAN_POINT('Ctrl Pts',(19.8233449918063,33.8461823850751,-76.8434761657068));
#173915=CARTESIAN_POINT('Ctrl Pts',(19.8210492509101,33.1409891728991,-78.2345121767389));
#173916=CARTESIAN_POINT('Ctrl Pts',(19.8186535378293,32.4050870483357,-79.6861233638405));
#173917=CARTESIAN_POINT('Ctrl Pts',(19.8162165495322,31.6836646490343,-81.1038113445808));
#173918=CARTESIAN_POINT('Ctrl Pts',(19.8137427373434,30.9767915267581,-82.4876206314048));
#173919=CARTESIAN_POINT('Ctrl Pts',(19.8117734698976,30.414088248637,-83.5891960025022));
#173920=CARTESIAN_POINT('Ctrl Pts',(19.8097809087695,29.860605784483,-84.6693034148617));
#173921=CARTESIAN_POINT('Ctrl Pts',(19.8077680666402,29.3163999141123,-85.7279763466165));
#173922=CARTESIAN_POINT('Ctrl Pts',(19.8077680666402,29.3163999141123,-85.7279763466166));
#173923=CARTESIAN_POINT('Ctrl Pts',(20.5,29.060089055415,-85.5959926642051));
#173924=CARTESIAN_POINT('Ctrl Pts',(20.5,29.7267599207011,-85.9392854774869));
#173925=CARTESIAN_POINT('Ctrl Pts',(19.8381616888784,29.0132146764574,-86.2891090855032));
#173926=CARTESIAN_POINT('Ctrl Pts',(20.5000000000088,28.8159639706074,-86.1813743808706));
#173927=CARTESIAN_POINT('Ctrl Pts',(20.5,29.4538783950287,-86.4692184100357));
#173928=CARTESIAN_POINT('Ctrl Pts',(19.8696882890952,28.7939665404343,-86.8767409776521));
#173929=CARTESIAN_POINT('Ctrl Pts',(20.5,28.6378348142226,-86.8034965148886));
#173930=CARTESIAN_POINT('Ctrl Pts',(20.5,29.2565698845367,-87.023482728964));
#173931=CARTESIAN_POINT('Ctrl Pts',(19.9342607161865,28.4963466916806,-88.096087277311));
#173932=CARTESIAN_POINT('Ctrl Pts',(20.5,28.4280256078311,-88.0643854695474));
#173933=CARTESIAN_POINT('Ctrl Pts',(20.5,28.9887120203667,-88.1720534995035));
#173934=CARTESIAN_POINT('Ctrl Pts',(19.9674881255149,28.4199999800001,-88.7314889737132));
#173935=CARTESIAN_POINT('Ctrl Pts',(20.5,28.3863947724214,-88.7102571696975));
#173936=CARTESIAN_POINT('Ctrl Pts',(20.5,28.9199999814054,-88.7697908796757));
#173937=CARTESIAN_POINT('Ctrl Pts',(20.,28.4199999800001,-89.3628471840451));
#173938=CARTESIAN_POINT('Ctrl Pts',(20.5,28.41999998,-89.3628471840451));
#173939=CARTESIAN_POINT('Ctrl Pts',(20.5,28.9199999800001,-89.3628471840451));
#173940=CARTESIAN_POINT('',(20.5,28.9199999800001,-89.3628471840452));
#173941=CARTESIAN_POINT('Ctrl Pts',(20.5,28.9199999800001,-89.3628471840452));
#173942=CARTESIAN_POINT('Ctrl Pts',(20.5,28.9199999800001,-89.0651820878934));
#173943=CARTESIAN_POINT('Ctrl Pts',(20.5,28.93706429112,-88.7687961767652));
#173944=CARTESIAN_POINT('Ctrl Pts',(20.5,29.004819730958,-88.1785451079783));
#173945=CARTESIAN_POINT('Ctrl Pts',(20.5,29.0556764864843,-87.8849108068938));
#173946=CARTESIAN_POINT('Ctrl Pts',(20.5,29.2565698843866,-87.0234827289138));
#173947=CARTESIAN_POINT('Ctrl Pts',(20.5,29.453814841029,-86.4693418183145));
#173948=CARTESIAN_POINT('Ctrl Pts',(20.5,29.726759920701,-85.9392854774869));
#173949=CARTESIAN_POINT('',(20.,28.4199999800001,-89.3628471840451));
#173950=CARTESIAN_POINT('Origin',(20.,28.9199999800001,-89.3628471840452));
#173951=CARTESIAN_POINT('Ctrl Pts',(19.8077680691566,29.3163998890102,-85.7279763930753));
#173952=CARTESIAN_POINT('Ctrl Pts',(19.8138059530845,29.2561708716977,-85.8394477061454));
#173953=CARTESIAN_POINT('Ctrl Pts',(19.8202703692203,29.1954402850721,-85.9590140875865));
#173954=CARTESIAN_POINT('Ctrl Pts',(19.8271724235496,29.1354166241997,-86.0869929818154));
#173955=CARTESIAN_POINT('Ctrl Pts',(19.8278791125124,29.1292709092249,-86.100096511245));
#173956=CARTESIAN_POINT('Ctrl Pts',(19.8285903887909,29.1231326473758,-86.1132882440816));
#173957=CARTESIAN_POINT('Ctrl Pts',(19.8293062638353,29.1170031622791,-86.1265685285763));
#173958=CARTESIAN_POINT('Ctrl Pts',(19.8344373255712,29.0730698436299,-86.2217554751544));
#173959=CARTESIAN_POINT('Ctrl Pts',(19.8398044093972,29.0295900163094,-86.3214872821633));
#173960=CARTESIAN_POINT('Ctrl Pts',(19.8454079188031,28.9870783305874,-86.4258270644159));
#173961=CARTESIAN_POINT('Ctrl Pts',(19.8477324609691,28.9694429169824,-86.4691110505534));
#173962=CARTESIAN_POINT('Ctrl Pts',(19.8500976503827,28.9519743036303,-86.5131873880211));
#173963=CARTESIAN_POINT('Ctrl Pts',(19.8525033305116,28.9347097768219,-86.5580575288924));
#173964=CARTESIAN_POINT('Ctrl Pts',(19.8526348911436,28.9337656230121,-86.5605113647213));
#173965=CARTESIAN_POINT('Ctrl Pts',(19.8527665728447,28.9328220795741,-86.5629675741412));
#173966=CARTESIAN_POINT('Ctrl Pts',(19.8528983755796,28.9318791526062,-86.5654261572288));
#173967=CARTESIAN_POINT('Ctrl Pts',(19.8529637620926,28.9314113724307,-86.5666458449325));
#173968=CARTESIAN_POINT('Ctrl Pts',(19.8530291783932,28.930943743974,-86.567866116817));
#173969=CARTESIAN_POINT('Ctrl Pts',(19.8530946244768,28.9304762679801,-86.5690869728917));
#173970=CARTESIAN_POINT('Ctrl Pts',(19.8531272591149,28.9302431614438,-86.5696957518119));
#173971=CARTESIAN_POINT('Ctrl Pts',(19.8531599011586,28.9300100928176,-86.5703046759916));
#173972=CARTESIAN_POINT('Ctrl Pts',(19.8531925506074,28.9297770621936,-86.5709137454318));
#173973=CARTESIAN_POINT('Ctrl Pts',(19.8532109379793,28.9296458250397,-86.5712567584595));
#173974=CARTESIAN_POINT('Ctrl Pts',(19.8532294228268,28.9295139204569,-86.5716015920954));
#173975=CARTESIAN_POINT('Ctrl Pts',(19.8532484967547,28.9293778437378,-86.5719574174513));
#173976=CARTESIAN_POINT('Ctrl Pts',(19.8533833936122,28.9284154660929,-86.5744739270359));
#173977=CARTESIAN_POINT('Ctrl Pts',(19.8535396018,28.927302884498,-86.5773881447066));
#173978=CARTESIAN_POINT('Ctrl Pts',(19.8536815320461,28.926293817902,-86.5800361364514));
#173979=CARTESIAN_POINT('Ctrl Pts',(19.8538223534622,28.9252926346389,-86.5826634407606));
#173980=CARTESIAN_POINT('Ctrl Pts',(19.8539491178474,28.9243932488445,-86.5850286292047));
#173981=CARTESIAN_POINT('Ctrl Pts',(19.8540270312009,28.9238408419878,-86.5864823782079));
#173982=CARTESIAN_POINT('Ctrl Pts',(19.8540350253345,28.9237841634593,-86.5866315370267));
#173983=CARTESIAN_POINT('Ctrl Pts',(19.8540429572621,28.9237279313574,-86.5867795355964));
#173984=CARTESIAN_POINT('Ctrl Pts',(19.854050924075,28.9236714573129,-86.5869281854998));
#173985=CARTESIAN_POINT('Ctrl Pts',(19.8563700093498,28.9072322454547,-86.6301991655269));
#173986=CARTESIAN_POINT('Ctrl Pts',(19.8589484826522,28.8894066613016,-86.6783454040105));
#173987=CARTESIAN_POINT('Ctrl Pts',(19.861789010759,28.8704970519722,-86.7314446547894));
#173988=CARTESIAN_POINT('Ctrl Pts',(19.8645532478657,28.8520953175712,-86.7831177640904));
#173989=CARTESIAN_POINT('Ctrl Pts',(19.8675656622532,28.8326675258354,-86.839481569511));
#173990=CARTESIAN_POINT('Ctrl Pts',(19.8708290798645,28.8125353830987,-86.9006211059241));
#173991=CARTESIAN_POINT('Ctrl Pts',(19.8742516216661,28.7914215974065,-86.9647418051478));
#173992=CARTESIAN_POINT('Ctrl Pts',(19.8779505890201,28.7695315696661,-87.0341217459319));
#173993=CARTESIAN_POINT('Ctrl Pts',(19.881927060228,28.7472934410884,-87.108826435092));
#173994=CARTESIAN_POINT('Ctrl Pts',(19.8858361123418,28.7254323489346,-87.1822645433543));
#173995=CARTESIAN_POINT('Ctrl Pts',(19.8900135681237,28.7032345847988,-87.2608526848623));
#173996=CARTESIAN_POINT('Ctrl Pts',(19.8944591271272,28.6811431666031,-87.3446366822712));
#173997=CARTESIAN_POINT('Ctrl Pts',(19.8955745229581,28.6756004045488,-87.3656581829045));
#173998=CARTESIAN_POINT('Ctrl Pts',(19.8967067865892,28.6700644898885,-87.3870066305516));
#173999=CARTESIAN_POINT('Ctrl Pts',(19.8978558878223,28.6645427205203,-87.4086823557021));
#174000=CARTESIAN_POINT('Ctrl Pts',(19.89887720476,28.6596349922718,-87.4279476602687));
#174001=CARTESIAN_POINT('Ctrl Pts',(19.8998752459103,28.6549099612437,-87.446781111282));
#174002=CARTESIAN_POINT('Ctrl Pts',(19.9009366140947,28.6499659548319,-87.4668174126734));
#174003=CARTESIAN_POINT('Ctrl Pts',(19.9012200059135,28.6486458747789,-87.4721672281063));
#174004=CARTESIAN_POINT('Ctrl Pts',(19.9015079153701,28.6473104524095,-87.4776028816474));
#174005=CARTESIAN_POINT('Ctrl Pts',(19.9018019975683,28.6459526530311,-87.4831556819491));
#174006=CARTESIAN_POINT('Ctrl Pts',(19.9018595593474,28.6456868860161,-87.4842425517656));
#174007=CARTESIAN_POINT('Ctrl Pts',(19.9019170864846,28.6454215357657,-87.4853286991829));
#174008=CARTESIAN_POINT('Ctrl Pts',(19.9019745789215,28.6451566012051,-87.4864141240178));
#174009=CARTESIAN_POINT('Ctrl Pts',(19.9059518365993,28.6268287467454,-87.5615025094597));
#174010=CARTESIAN_POINT('Ctrl Pts',(19.9097655725751,28.6105182419633,-87.6331851842344));
#174011=CARTESIAN_POINT('Ctrl Pts',(19.913394524837,28.5959092357283,-87.7013592376738));
#174012=CARTESIAN_POINT('Ctrl Pts',(19.9171523881801,28.5807812745294,-87.7719550344457));
#174013=CARTESIAN_POINT('Ctrl Pts',(19.9207121251527,28.5674776275295,-87.8387888721745));
#174014=CARTESIAN_POINT('Ctrl Pts',(19.9240526752648,28.5556847412826,-87.9017892292155));
#174015=CARTESIAN_POINT('Ctrl Pts',(19.9264836775809,28.5471027614233,-87.947636173206));
#174016=CARTESIAN_POINT('Ctrl Pts',(19.9287986577477,28.5393216422585,-87.9914538920984));
#174017=CARTESIAN_POINT('Ctrl Pts',(19.9309902059722,28.5322331361077,-88.0332265793131));
#174018=CARTESIAN_POINT('Ctrl Pts',(19.9341130131768,28.5221324968288,-88.0927498182434));
#174019=CARTESIAN_POINT('Ctrl Pts',(19.9369954702788,28.5134356307963,-88.1481148204475));
#174020=CARTESIAN_POINT('Ctrl Pts',(19.9396491505859,28.5058659354445,-88.1992828513666));
#174021=CARTESIAN_POINT('Ctrl Pts',(19.9404596972027,28.5035538291438,-88.214911740137));
#174022=CARTESIAN_POINT('Ctrl Pts',(19.9412489070806,28.5013471920599,-88.2301492763028));
#174023=CARTESIAN_POINT('Ctrl Pts',(19.9420171267609,28.4992389562131,-88.244994858652));
#174024=CARTESIAN_POINT('Ctrl Pts',(19.943658788847,28.4947337203449,-88.2767194165039));
#174025=CARTESIAN_POINT('Ctrl Pts',(19.945205054462,28.4906773451103,-88.3066533814086));
#174026=CARTESIAN_POINT('Ctrl Pts',(19.9466613325595,28.48700670808,-88.3347914894808));
#174027=CARTESIAN_POINT('Ctrl Pts',(19.9473894716083,28.4851713895648,-88.3488605435169));
#174028=CARTESIAN_POINT('Ctrl Pts',(19.9480951270559,28.4834326321617,-88.3624806487063));
#174029=CARTESIAN_POINT('Ctrl Pts',(19.948779043131,28.4817832803921,-88.3756513708551));
#174030=CARTESIAN_POINT('Ctrl Pts',(19.9491210011685,28.4809586045074,-88.3822367319295));
#174031=CARTESIAN_POINT('Ctrl Pts',(19.9494575252137,28.4801562877716,-88.388709748227));
#174032=CARTESIAN_POINT('Ctrl Pts',(19.9497887098329,28.479375482198,-88.3950703715738));
#174033=CARTESIAN_POINT('Ctrl Pts',(19.9499543021425,28.4789850794112,-88.3982506832472));
#174034=CARTESIAN_POINT('Ctrl Pts',(19.9501185596432,28.4786000548937,-88.401402896738));
#174035=CARTESIAN_POINT('Ctrl Pts',(19.9502814943068,28.478220305484,-88.4045270067001));
#174036=CARTESIAN_POINT('Ctrl Pts',(19.9503629616386,28.4780304307791,-88.4060890616811));
#174037=CARTESIAN_POINT('Ctrl Pts',(19.9504440982641,28.4778418748811,-88.4076440907833));
#174038=CARTESIAN_POINT('Ctrl Pts',(19.9505249056845,28.4776546250721,-88.4091920933774));
#174039=CARTESIAN_POINT('Ctrl Pts',(19.950605713105,28.4774673752631,-88.4107400959714));
#174040=CARTESIAN_POINT('Ctrl Pts',(19.9506232874581,28.477426349047,-88.4110771956486));
#174041=CARTESIAN_POINT('Ctrl Pts',(19.9507663418393,28.4770967813136,-88.4138150210238));
#174042=CARTESIAN_POINT('Ctrl Pts',(19.9561774440553,28.4646307199664,-88.5173746102378));
#174043=CARTESIAN_POINT('Ctrl Pts',(19.9614261063647,28.4545670612358,-88.6180628114536));
#174044=CARTESIAN_POINT('Ctrl Pts',(19.9665083066635,28.4465583754429,-88.7157667717928));
#174045=CARTESIAN_POINT('Ctrl Pts',(19.9717269590573,28.4383346642888,-88.8160939876713));
#174046=CARTESIAN_POINT('Ctrl Pts',(19.97677011187,28.4322776514497,-88.9132749359466));
#174047=CARTESIAN_POINT('Ctrl Pts',(19.9816359372707,28.4280374234223,-89.0072367202588));
#174048=CARTESIAN_POINT('Ctrl Pts',(19.9866936397869,28.4236299878492,-89.1049037579766));
#174049=CARTESIAN_POINT('Ctrl Pts',(19.9915597727704,28.4211852765213,-89.1990930646804));
#174050=CARTESIAN_POINT('Ctrl Pts',(19.9962346717654,28.4203405465593,-89.289770015951));
#174051=CARTESIAN_POINT('Ctrl Pts',(19.9975038532053,28.4201112120666,-89.314387767843));
#174052=CARTESIAN_POINT('Ctrl Pts',(19.998758951749,28.4199999800001,-89.338746881695));
#174053=CARTESIAN_POINT('Ctrl Pts',(20.,28.4199999800001,-89.3628471840451));
#174054=CARTESIAN_POINT('Origin',(20.,28.9199999800001,-55.24995));
#174055=CARTESIAN_POINT('',(20.5,28.9199999800001,-91.34995));
#174056=CARTESIAN_POINT('',(20.5,28.9199999800001,-88.9338641536579));
#174057=CARTESIAN_POINT('',(20.,28.4199999800001,-91.34995));
#174058=CARTESIAN_POINT('Origin',(20.,28.9199999800001,-91.34995));
#174059=CARTESIAN_POINT('',(20.,28.4199999800001,-91.34995));
#174060=CARTESIAN_POINT('Origin',(21.,43.91999998,-58.24995));
#174061=CARTESIAN_POINT('',(21.,46.91999998,-58.24995));
#174062=CARTESIAN_POINT('',(20.5,46.41999998,-58.24995));
#174063=CARTESIAN_POINT('Origin',(21.,46.41999998,-58.24995));
#174064=CARTESIAN_POINT('',(20.5,43.91999998,-55.74995));
#174065=CARTESIAN_POINT('Origin',(20.5,43.91999998,-58.24995));
#174066=CARTESIAN_POINT('',(21.,43.91999998,-55.24995));
#174067=CARTESIAN_POINT('Origin',(21.,43.91999998,-55.74995));
#174068=CARTESIAN_POINT('Origin',(21.,43.91999998,-58.24995));
#174069=CARTESIAN_POINT('Origin',(0.,43.91999998,-58.24995));
#174070=CARTESIAN_POINT('',(21.5,46.91999998,-58.24995));
#174071=CARTESIAN_POINT('',(-39.,46.91999998,-58.24995));
#174072=CARTESIAN_POINT('',(21.5,43.91999998,-55.24995));
#174073=CARTESIAN_POINT('',(0.,43.91999998,-55.24995));
#174074=CARTESIAN_POINT('Origin',(21.5,43.91999998,-58.24995));
#174075=CARTESIAN_POINT('Origin',(21.5,43.91999998,-58.24995));
#174076=CARTESIAN_POINT('',(22.,43.91999998,-55.74995));
#174077=CARTESIAN_POINT('Origin',(21.5,43.91999998,-55.74995));
#174078=CARTESIAN_POINT('',(22.,46.41999998,-58.24995));
#174079=CARTESIAN_POINT('Origin',(22.,43.91999998,-58.24995));
#174080=CARTESIAN_POINT('Origin',(21.5,46.41999998,-58.24995));
#174081=CARTESIAN_POINT('Origin',(22.5,28.9199999800001,-55.24995));
#174082=CARTESIAN_POINT('',(22.,28.9199999800001,-87.1305533863517));
#174083=CARTESIAN_POINT('Origin',(22.5,28.91999998,-87.1305533863517));
#174084=CARTESIAN_POINT('',(22.5,28.4199999800001,-91.34995));
#174085=CARTESIAN_POINT('',(22.5,28.4199999800001,-87.5942752792638));
#174086=CARTESIAN_POINT('',(22.,28.9199999800001,-91.34995));
#174087=CARTESIAN_POINT('Origin',(22.5,28.9199999800001,-91.34995));
#174088=CARTESIAN_POINT('',(22.,28.9199999800001,-91.34995));
#174089=CARTESIAN_POINT('Ctrl Pts',(22.5,28.41999998,-87.1305533863517));
#174090=CARTESIAN_POINT('Ctrl Pts',(22.,28.41999998,-87.1305533863516));
#174091=CARTESIAN_POINT('Ctrl Pts',(22.,28.91999998,-87.1305533863517));
#174092=CARTESIAN_POINT('Ctrl Pts',(22.4639153689348,28.41999998,-86.4410479992692));
#174093=CARTESIAN_POINT('Ctrl Pts',(22.0000000000044,28.4548243482677,-86.4651291551651));
#174094=CARTESIAN_POINT('Ctrl Pts',(22.,28.9199999821681,-86.4796041157695));
#174095=CARTESIAN_POINT('Ctrl Pts',(22.4281188150557,28.5015955861724,-85.7652097651195));
#174096=CARTESIAN_POINT('Ctrl Pts',(22.,28.5601858706255,-85.7927489918333));
#174097=CARTESIAN_POINT('Ctrl Pts',(22.,28.9934360246446,-85.840664401161));
#174098=CARTESIAN_POINT('Ctrl Pts',(22.3573227200049,28.8261151186122,-84.4410318437717));
#174099=CARTESIAN_POINT('Ctrl Pts',(22.,28.9249341693522,-84.4905989888491));
#174100=CARTESIAN_POINT('Ctrl Pts',(22.,29.2855036056616,-84.5872260208873));
#174101=CARTESIAN_POINT('Ctrl Pts',(22.3220283366802,29.072521775155,-83.7873824528849));
#174102=CARTESIAN_POINT('Ctrl Pts',(22.,29.1803706436616,-83.8479871870358));
#174103=CARTESIAN_POINT('Ctrl Pts',(22.,29.5072644006254,-83.9676830002751));
#174104=CARTESIAN_POINT('Ctrl Pts',(22.2890532034791,29.4093902975657,-83.1809305852948));
#174105=CARTESIAN_POINT('Ctrl Pts',(22.,29.5283900973743,-83.2436286443491));
#174106=CARTESIAN_POINT('Ctrl Pts',(22.,29.8104512658091,-83.3922397161652));
#174107=CARTESIAN_POINT('',(22.,29.8104512658091,-83.3922397161652));
#174108=CARTESIAN_POINT('Origin',(22.5,29.8104512658091,-83.3922397161652));
#174109=CARTESIAN_POINT('Ctrl Pts',(22.,29.8104512658091,-83.3922397161652));
#174110=CARTESIAN_POINT('Ctrl Pts',(22.,29.7130107699212,-83.5771800425296));
#174111=CARTESIAN_POINT('Ctrl Pts',(22.,29.6241027734271,-83.7664339874128));
#174112=CARTESIAN_POINT('Ctrl Pts',(22.,29.5434345930966,-83.9588738468728));
#174113=CARTESIAN_POINT('Ctrl Pts',(22.,29.4578017187799,-84.1631573478909));
#174114=CARTESIAN_POINT('Ctrl Pts',(22.,29.3814538044554,-84.3710319263881));
#174115=CARTESIAN_POINT('Ctrl Pts',(22.,29.3140928258488,-84.5811807101608));
#174116=CARTESIAN_POINT('Ctrl Pts',(22.,29.2470690502148,-84.7902775081099));
#174117=CARTESIAN_POINT('Ctrl Pts',(22.,29.188942707981,-85.0016271465759));
#174118=CARTESIAN_POINT('Ctrl Pts',(22.,29.1394698146751,-85.2139452109128));
#174119=CARTESIAN_POINT('Ctrl Pts',(22.,29.0466872110912,-85.6121313989588));
#174120=CARTESIAN_POINT('Ctrl Pts',(22.,28.9832164657711,-86.0152044949698));
#174121=CARTESIAN_POINT('Ctrl Pts',(22.,28.9492578229235,-86.4231979120729));
#174122=CARTESIAN_POINT('Ctrl Pts',(22.,28.9297677681887,-86.6573596265579));
#174123=CARTESIAN_POINT('Ctrl Pts',(22.,28.9199999800002,-86.8931422598655));
#174124=CARTESIAN_POINT('Ctrl Pts',(22.,28.91999998,-87.1305533863517));
#174125=CARTESIAN_POINT('Ctrl Pts',(22.,41.1098595241823,-61.4386408691296));
#174126=CARTESIAN_POINT('Ctrl Pts',(22.,40.7995210108967,-61.2819013639433));
#174127=CARTESIAN_POINT('Ctrl Pts',(22.3259225534138,40.6914751389564,-61.2273317382593));
#174128=CARTESIAN_POINT('Ctrl Pts',(22.,37.3993732891074,-68.7852685139811));
#174129=CARTESIAN_POINT('Ctrl Pts',(22.,37.1246521940256,-68.5757439011997));
#174130=CARTESIAN_POINT('Ctrl Pts',(22.3157409333924,36.9852292354808,-68.5739513464269));
#174131=CARTESIAN_POINT('Ctrl Pts',(22.,33.6470169072337,-76.1105064350252));
#174132=CARTESIAN_POINT('Ctrl Pts',(22.,33.3938486289533,-75.8821367178777));
#174133=CARTESIAN_POINT('Ctrl Pts',(22.3038724392466,33.2381690210168,-75.8991829107314));
#174134=CARTESIAN_POINT('Ctrl Pts',(22.,29.8104512658091,-83.3922397161652));
#174135=CARTESIAN_POINT('Ctrl Pts',(22.,29.5283900973743,-83.243628644349));
#174136=CARTESIAN_POINT('Ctrl Pts',(22.2890532034791,29.4093902975657,-83.1809305852948));
#174137=CARTESIAN_POINT('',(22.,41.1098595241823,-61.4386408691296));
#174138=CARTESIAN_POINT('',(22.3259225534138,40.6914751389564,-61.2273317382593));
#174139=CARTESIAN_POINT('Origin',(22.5,41.1098595241823,-61.4386408691296));
#174140=CARTESIAN_POINT('Ctrl Pts',(22.2890532034791,29.4093902975657,-83.1809305852948));
#174141=CARTESIAN_POINT('Ctrl Pts',(22.2915992865075,30.0672102202902,-81.9298583665631));
#174142=CARTESIAN_POINT('Ctrl Pts',(22.2941161314434,30.7375917756893,-80.6490156487439));
#174143=CARTESIAN_POINT('Ctrl Pts',(22.2965989022532,31.4204400512108,-79.3383406087535));
#174144=CARTESIAN_POINT('Ctrl Pts',(22.2990071415531,32.0827895707544,-78.067011363099));
#174145=CARTESIAN_POINT('Ctrl Pts',(22.3013833157878,32.7568683731644,-76.7676139152288));
#174146=CARTESIAN_POINT('Ctrl Pts',(22.3037242761676,33.4426330710029,-75.4401153073922));
#174147=CARTESIAN_POINT('Ctrl Pts',(22.3059739143508,34.101645697684,-74.164403175777));
#174148=CARTESIAN_POINT('Ctrl Pts',(22.308191030053,34.7714501903432,-72.8627395683749));
#174149=CARTESIAN_POINT('Ctrl Pts',(22.310374071687,35.4520502432749,-71.5351181260537));
#174150=CARTESIAN_POINT('Ctrl Pts',(22.3125129104872,36.1188693171654,-70.2343787317024));
#174151=CARTESIAN_POINT('Ctrl Pts',(22.3146190356274,36.7960510223641,-68.908721970169));
#174152=CARTESIAN_POINT('Ctrl Pts',(22.3166922686174,37.4836420872136,-67.5581653122663));
#174153=CARTESIAN_POINT('Ctrl Pts',(22.318707401592,38.1519641882275,-66.2454564809706));
#174154=CARTESIAN_POINT('Ctrl Pts',(22.320691457232,38.8301203169625,-64.9092237355817));
#174155=CARTESIAN_POINT('Ctrl Pts',(22.3226455520959,39.5181964415169,-63.5495064562538));
#174156=CARTESIAN_POINT('Ctrl Pts',(22.3237472546366,39.9061280760574,-62.782909087359));
#174157=CARTESIAN_POINT('Ctrl Pts',(22.3248394573525,40.2972136823501,-62.0088473266159));
#174158=CARTESIAN_POINT('Ctrl Pts',(22.3259225534138,40.6914751389564,-61.2273317382593));
#174159=CARTESIAN_POINT('Ctrl Pts',(22.,41.1098595241823,-61.4386408691296));
#174160=CARTESIAN_POINT('Ctrl Pts',(22.,37.3993520818416,-68.7853105030709));
#174161=CARTESIAN_POINT('Ctrl Pts',(22.,33.6470396305176,-76.1104633065809));
#174162=CARTESIAN_POINT('Ctrl Pts',(22.,29.8104512658091,-83.3922397161652));
#174163=CARTESIAN_POINT('Ctrl Pts',(28.4933647440612,38.6927858841382,-60.650327573148));
#174164=CARTESIAN_POINT('Ctrl Pts',(29.,38.6926240909195,-60.6436056187277));
#174165=CARTESIAN_POINT('Ctrl Pts',(29.,38.7048160259599,-61.150138786574));
#174166=CARTESIAN_POINT('Ctrl Pts',(28.4508217728044,38.5151017970219,-60.6551690977179));
#174167=CARTESIAN_POINT('Ctrl Pts',(29.,38.5056874437974,-60.6032547660267));
#174168=CARTESIAN_POINT('Ctrl Pts',(29.,38.6042425482601,-61.1525595652015));
#174169=CARTESIAN_POINT('Ctrl Pts',(28.4075947879363,38.335472514688,-60.707925961796));
#174170=CARTESIAN_POINT('Ctrl Pts',(29.,38.2987442898004,-60.603134659432));
#174171=CARTESIAN_POINT('Ctrl Pts',(29.,38.5024684382473,-61.1789379706814));
#174172=CARTESIAN_POINT('Ctrl Pts',(28.3514280416523,38.1029959208976,-60.8540715547449));
#174173=CARTESIAN_POINT('Ctrl Pts',(29.0000000000001,37.990375163389,-60.6863576421133));
#174174=CARTESIAN_POINT('Ctrl Pts',(29.,38.3706532052714,-61.2520107824808));
#174175=CARTESIAN_POINT('Ctrl Pts',(28.3338483525148,38.0303960306507,-60.9145171861254));
#174176=CARTESIAN_POINT('Ctrl Pts',(29.,37.8822359354345,-60.7316627868476));
#174177=CARTESIAN_POINT('Ctrl Pts',(29.,38.3294709783247,-61.2822335925436));
#174178=CARTESIAN_POINT('Ctrl Pts',(28.302912455342,37.9028346914031,-61.0569005178125));
#174179=CARTESIAN_POINT('Ctrl Pts',(29.,37.6732261500514,-60.8640556435108));
#174180=CARTESIAN_POINT('Ctrl Pts',(29.,38.2570904307121,-61.3534252594253));
#174181=CARTESIAN_POINT('Ctrl Pts',(28.28982523324,37.8489775515987,-61.1370349799883));
#174182=CARTESIAN_POINT('Ctrl Pts',(29.,37.5759010011862,-60.9505556565881));
#174183=CARTESIAN_POINT('Ctrl Pts',(29.,38.2265217687548,-61.3934878926125));
#174184=CARTESIAN_POINT('Ctrl Pts',(28.2795019009908,37.8065307949999,-61.2273317382593));
#174185=CARTESIAN_POINT('Ctrl Pts',(29.,37.4942143736512,-61.0606306836509));
#174186=CARTESIAN_POINT('Ctrl Pts',(29.,38.2024209812184,-61.4386408691297));
#174187=CARTESIAN_POINT('',(28.49336474298,38.692785884125,-60.6503274733137));
#174188=CARTESIAN_POINT('',(29.,38.7048160259599,-61.150138786574));
#174189=CARTESIAN_POINT('Origin',(28.5,38.7048160259599,-61.150138786574));
#174190=CARTESIAN_POINT('Ctrl Pts',(29.,38.2024209812184,-61.4386408691297));
#174191=CARTESIAN_POINT('Ctrl Pts',(29.,38.2265260808242,-61.3934796764616));
#174192=CARTESIAN_POINT('Ctrl Pts',(29.,38.2570947542809,-61.3534209131338));
#174193=CARTESIAN_POINT('Ctrl Pts',(29.,38.293280667393,-61.3178293882391));
#174194=CARTESIAN_POINT('Ctrl Pts',(29.,38.3294709547425,-61.2822335609581));
#174195=CARTESIAN_POINT('Ctrl Pts',(29.,38.3706505444737,-61.2520122466304));
#174196=CARTESIAN_POINT('Ctrl Pts',(29.,38.4145916132166,-61.2276531730517));
#174197=CARTESIAN_POINT('Ctrl Pts',(29.,38.4390337855644,-61.2141034645061));
#174198=CARTESIAN_POINT('Ctrl Pts',(29.,38.4644512947928,-61.2023317240159));
#174199=CARTESIAN_POINT('Ctrl Pts',(29.,38.490593259323,-61.1923093713145));
#174200=CARTESIAN_POINT('Ctrl Pts',(29.,38.5172131854938,-61.1821037768321));
#174201=CARTESIAN_POINT('Ctrl Pts',(29.,38.5445857496398,-61.1737118246007));
#174202=CARTESIAN_POINT('Ctrl Pts',(29.,38.5724697430453,-61.1671525783509));
#174203=CARTESIAN_POINT('Ctrl Pts',(29.,38.5996144829857,-61.1607672291985));
#174204=CARTESIAN_POINT('Ctrl Pts',(29.,38.6272453201521,-61.1561187181941));
#174205=CARTESIAN_POINT('Ctrl Pts',(29.,38.6551404973774,-61.1532723608215));
#174206=CARTESIAN_POINT('Ctrl Pts',(29.,38.6716230181358,-61.1515905237032));
#174207=CARTESIAN_POINT('Ctrl Pts',(29.,38.688197742811,-61.1505387782063));
#174208=CARTESIAN_POINT('Ctrl Pts',(29.,38.7048160259599,-61.150138786574));
#174209=CARTESIAN_POINT('Ctrl Pts',(28.4933647440612,38.6927858841382,-60.650327573148));
#174210=CARTESIAN_POINT('Ctrl Pts',(28.4866112948369,38.6645795682284,-60.6510961370265));
#174211=CARTESIAN_POINT('Ctrl Pts',(28.4800601957753,38.6372412590608,-60.6530442725806));
#174212=CARTESIAN_POINT('Ctrl Pts',(28.4737238128436,38.6108170677176,-60.6559437523982));
#174213=CARTESIAN_POINT('Ctrl Pts',(28.4670685534825,38.5830630874591,-60.6589891476034));
#174214=CARTESIAN_POINT('Ctrl Pts',(28.4606500721898,38.5563171621938,-60.6630840224132));
#174215=CARTESIAN_POINT('Ctrl Pts',(28.4544730160308,38.5305935477136,-60.6680036899134));
#174216=CARTESIAN_POINT('Ctrl Pts',(28.4538555252183,38.5280220807886,-60.6684954855849));
#174217=CARTESIAN_POINT('Ctrl Pts',(28.4532404400623,38.525460801933,-60.6689955548281));
#174218=CARTESIAN_POINT('Ctrl Pts',(28.4526277607726,38.522909707497,-60.6695036937783));
#174219=CARTESIAN_POINT('Ctrl Pts',(28.4435667341815,38.485181103132,-60.6770186540817));
#174220=CARTESIAN_POINT('Ctrl Pts',(28.4350378093247,38.4497043204397,-60.6862892049898));
#174221=CARTESIAN_POINT('Ctrl Pts',(28.4270696258733,38.4165855517814,-60.6966603137934));
#174222=CARTESIAN_POINT('Ctrl Pts',(28.4242404806142,38.4048265595461,-60.7003426302813));
#174223=CARTESIAN_POINT('Ctrl Pts',(28.4214820436404,38.3933649319099,-60.7041640893731));
#174224=CARTESIAN_POINT('Ctrl Pts',(28.4187957564384,38.3822061546877,-60.7080959629319));
#174225=CARTESIAN_POINT('Ctrl Pts',(28.4157769158789,38.3696659582232,-60.7125145892669));
#174226=CARTESIAN_POINT('Ctrl Pts',(28.4128472428645,38.357500126538,-60.7170753249694));
#174227=CARTESIAN_POINT('Ctrl Pts',(28.4100050480235,38.3457010004413,-60.7217450693001));
#174228=CARTESIAN_POINT('Ctrl Pts',(28.4038012283365,38.3199463795004,-60.7319379847875));
#174229=CARTESIAN_POINT('Ctrl Pts',(28.3980168462861,38.2959498502083,-60.7426442520555));
#174230=CARTESIAN_POINT('Ctrl Pts',(28.3926401637082,38.2736568809467,-60.7535341130708));
#174231=CARTESIAN_POINT('Ctrl Pts',(28.3876929931094,38.2531447676696,-60.7635540462657));
#174232=CARTESIAN_POINT('Ctrl Pts',(28.3830906731624,38.234073632809,-60.7737303004237));
#174233=CARTESIAN_POINT('Ctrl Pts',(28.3788195853896,38.2163832003577,-60.7838358975799));
#174234=CARTESIAN_POINT('Ctrl Pts',(28.3762732387338,38.2058364787947,-60.7898606750819));
#174235=CARTESIAN_POINT('Ctrl Pts',(28.3738445066921,38.1957800356412,-60.7958609581478));
#174236=CARTESIAN_POINT('Ctrl Pts',(28.3715298746371,38.1861985984285,-60.8017935811565));
#174237=CARTESIAN_POINT('Ctrl Pts',(28.3710654296699,38.1842760249112,-60.8029839979626));
#174238=CARTESIAN_POINT('Ctrl Pts',(28.3706055595698,38.1823724975692,-60.8041717490278));
#174239=CARTESIAN_POINT('Ctrl Pts',(28.3701502904136,38.1804881188278,-60.8053563570953));
#174240=CARTESIAN_POINT('Ctrl Pts',(28.3697831735728,38.1789686063346,-60.8063115932792));
#174241=CARTESIAN_POINT('Ctrl Pts',(28.3694189788947,38.1774612515492,-60.8072648797398));
#174242=CARTESIAN_POINT('Ctrl Pts',(28.3690577461341,38.1759662158436,-60.8082158932158));
#174243=CARTESIAN_POINT('Ctrl Pts',(28.3687139645852,38.1745434055486,-60.8091209630808));
#174244=CARTESIAN_POINT('Ctrl Pts',(28.3685506475493,38.1738674773002,-60.8095518784965));
#174245=CARTESIAN_POINT('Ctrl Pts',(28.3681154374745,38.1720662519997,-60.8107093564416));
#174246=CARTESIAN_POINT('Ctrl Pts',(28.3680374556281,38.1717435047037,-60.8109167557474));
#174247=CARTESIAN_POINT('Ctrl Pts',(28.3679507553739,38.1713846756153,-60.8111475922255));
#174248=CARTESIAN_POINT('Ctrl Pts',(28.3678527542032,38.1709790791434,-60.8114089693127));
#174249=CARTESIAN_POINT('Ctrl Pts',(28.3607255558591,38.1414818141342,-60.8304177865576));
#174250=CARTESIAN_POINT('Ctrl Pts',(28.3539183117575,38.113332878083,-60.850746794587));
#174251=CARTESIAN_POINT('Ctrl Pts',(28.3474565546205,38.0866307902112,-60.8721473077096));
#174252=CARTESIAN_POINT('Ctrl Pts',(28.3407512736884,38.0589223825975,-60.8943543404928));
#174253=CARTESIAN_POINT('Ctrl Pts',(28.334417972381,38.032771774352,-60.9177151428445));
#174254=CARTESIAN_POINT('Ctrl Pts',(28.3284731047364,38.008240394159,-60.9419785882647));
#174255=CARTESIAN_POINT('Ctrl Pts',(28.32497451288,37.9938035232142,-60.9562577779171));
#174256=CARTESIAN_POINT('Ctrl Pts',(28.3216102278411,37.9799265561799,-60.970850091482));
#174257=CARTESIAN_POINT('Ctrl Pts',(28.3183818526901,37.9666149649566,-60.9857084492844));
#174258=CARTESIAN_POINT('Ctrl Pts',(28.3093491455501,37.9293703141764,-61.0272808156703));
#174259=CARTESIAN_POINT('Ctrl Pts',(28.3014724081544,37.8969287820801,-61.0703254314474));
#174260=CARTESIAN_POINT('Ctrl Pts',(28.2946292360272,37.8687619975003,-61.1144056260449));
#174261=CARTESIAN_POINT('Ctrl Pts',(28.2888847384778,37.8451174037381,-61.1514087241892));
#174262=CARTESIAN_POINT('Ctrl Pts',(28.2838681852101,37.8244837283527,-61.1891405466858));
#174263=CARTESIAN_POINT('Ctrl Pts',(28.2795019009908,37.8065307949998,-61.2273317382593));
#174264=CARTESIAN_POINT('Ctrl Pts',(22.3259225534138,40.6914751389564,-61.2273317382593));
#174265=CARTESIAN_POINT('Ctrl Pts',(22.,40.7995210108967,-61.2819013639433));
#174266=CARTESIAN_POINT('Ctrl Pts',(22.,41.1098595241823,-61.4386408691297));
#174267=CARTESIAN_POINT('Ctrl Pts',(22.3307532272019,40.7164963923335,-61.1738110360374));
#174268=CARTESIAN_POINT('Ctrl Pts',(22.,40.8194184511061,-61.2339961299344));
#174269=CARTESIAN_POINT('Ctrl Pts',(22.,41.1233751604146,-61.4118804447591));
#174270=CARTESIAN_POINT('Ctrl Pts',(22.3364246839863,40.745888690896,-61.1232259520736));
#174271=CARTESIAN_POINT('Ctrl Pts',(22.,40.8429002807173,-61.1881281443964));
#174272=CARTESIAN_POINT('Ctrl Pts',(22.,41.1392509618672,-61.3865876948747));
#174273=CARTESIAN_POINT('Ctrl Pts',(22.3428990418276,40.7794755973204,-61.0754935261973));
#174274=CARTESIAN_POINT('Ctrl Pts',(22.,40.8698280768405,-61.1441646043172));
#174275=CARTESIAN_POINT('Ctrl Pts',(22.,41.1573899115079,-61.3627217630986));
#174276=CARTESIAN_POINT('',(22.,41.1573899115079,-61.3627217630986));
#174277=CARTESIAN_POINT('',(22.3428990418278,40.7794755973209,-61.0754935261978));
#174278=CARTESIAN_POINT('Origin',(22.5,41.1573899115079,-61.3627217630986));
#174279=CARTESIAN_POINT('Origin',(22.4949966047551,41.5721884749956,-61.6542986908816));
#174280=CARTESIAN_POINT('Origin',(22.,41.5483105744962,-61.6603021206194));
#174281=CARTESIAN_POINT('Origin',(0.,-12.9675000200281,-60.64995));
#174282=CARTESIAN_POINT('Origin',(0.,-12.9675000200281,-61.2273317382593));
#174283=CARTESIAN_POINT('Origin',(24.2,-70.08000002,-58.24995));
#174284=CARTESIAN_POINT('',(24.2,-70.08000002,-55.24995));
#174285=CARTESIAN_POINT('',(23.7,-70.08000002,-55.74995));
#174286=CARTESIAN_POINT('Origin',(24.2,-70.08000002,-55.74995));
#174287=CARTESIAN_POINT('',(23.7,-72.58000002,-58.24995));
#174288=CARTESIAN_POINT('Origin',(23.7,-70.08000002,-58.24995));
#174289=CARTESIAN_POINT('Origin',(24.2,-72.58000002,-58.24995));
#174290=CARTESIAN_POINT('Origin',(24.2,-70.08000002,-58.24995));
#174291=CARTESIAN_POINT('Origin',(24.2,-72.58000002,-55.24995));
#174292=CARTESIAN_POINT('',(23.7,-72.58000002,-174.34995));
#174293=CARTESIAN_POINT('',(23.7,-72.58000002,-58.24995));
#174294=CARTESIAN_POINT('Origin',(24.2,-72.58000002,-174.34995));
#174295=CARTESIAN_POINT('Origin',(24.2,-70.08000002,-174.34995));
#174296=CARTESIAN_POINT('',(23.7,-70.08000002,-176.84995));
#174297=CARTESIAN_POINT('Origin',(23.7,-70.08000002,-174.34995));
#174298=CARTESIAN_POINT('Origin',(24.2,-70.08000002,-176.84995));
#174299=CARTESIAN_POINT('Ctrl Pts',(23.7,-55.9902808012637,-149.835491960129));
#174300=CARTESIAN_POINT('Ctrl Pts',(23.6999999999999,-55.2903249255959,
-150.206318626088));
#174301=CARTESIAN_POINT('Ctrl Pts',(22.9849163103247,-55.591423110293,-150.046801090999));
#174302=CARTESIAN_POINT('Ctrl Pts',(23.7,-59.7506418899787,-156.933381838169));
#174303=CARTESIAN_POINT('Ctrl Pts',(23.7,-58.9786022357095,-157.10917403496));
#174304=CARTESIAN_POINT('Ctrl Pts',(22.9994804181366,-59.343937645489,-157.144704426787));
#174305=CARTESIAN_POINT('Ctrl Pts',(23.7,-63.4274104915032,-164.074673486974));
#174306=CARTESIAN_POINT('Ctrl Pts',(23.7000000002973,-62.707250125371,-164.298966961939));
#174307=CARTESIAN_POINT('Ctrl Pts',(23.0112491123844,-63.0152939322715,
-164.285990110815));
#174308=CARTESIAN_POINT('Ctrl Pts',(23.7,-67.0618271655313,-171.237717270032));
#174309=CARTESIAN_POINT('Ctrl Pts',(23.7,-66.413901371901,-171.56646471025));
#174310=CARTESIAN_POINT('Ctrl Pts',(23.0213852109847,-66.6453596297547,
-171.449026400902));
#174311=CARTESIAN_POINT('',(23.0213852109847,-66.6453596297547,-171.449026400902));
#174312=CARTESIAN_POINT('',(23.7,-67.0618271655313,-171.237717270032));
#174313=CARTESIAN_POINT('Origin',(23.2,-67.0618271655313,-171.237717270032));
#174314=CARTESIAN_POINT('',(23.7,-55.9902808012637,-149.835491960129));
#174315=CARTESIAN_POINT('Ctrl Pts',(23.7,-55.9902808012637,-149.835491960129));
#174316=CARTESIAN_POINT('Ctrl Pts',(23.7,-59.7506641394806,-156.933423835337));
#174317=CARTESIAN_POINT('Ctrl Pts',(23.7,-63.4273897219659,-164.074632552453));
#174318=CARTESIAN_POINT('Ctrl Pts',(23.7,-67.0618271655313,-171.237717270032));
#174319=CARTESIAN_POINT('Origin',(23.2,-55.9902808012637,-149.835491960129));
#174320=CARTESIAN_POINT('Ctrl Pts',(23.0213852109847,-66.6453596297547,
-171.449026400902));
#174321=CARTESIAN_POINT('Ctrl Pts',(23.0194522730378,-65.9531118514689,
-170.083046727027));
#174322=CARTESIAN_POINT('Ctrl Pts',(23.0174911199861,-65.2705560001936,
-168.739955519058));
#174323=CARTESIAN_POINT('Ctrl Pts',(23.0155001081443,-64.5975812226656,
-167.419805386397));
#174324=CARTESIAN_POINT('Ctrl Pts',(23.0134670373099,-63.9103902357703,
-166.071767833125));
#174325=CARTESIAN_POINT('Ctrl Pts',(23.0114028370452,-63.2331895248465,
-164.747650752542));
#174326=CARTESIAN_POINT('Ctrl Pts',(23.009307102834,-62.5659090224749,-163.447484054915));
#174327=CARTESIAN_POINT('Ctrl Pts',(23.0071368764899,-61.8749102701637,
-162.101103390916));
#174328=CARTESIAN_POINT('Ctrl Pts',(23.0049328366384,-61.1945495374443,
-160.780405954722));
#174329=CARTESIAN_POINT('Ctrl Pts',(23.0026959184795,-60.5247985662132,
-159.485397982963));
#174330=CARTESIAN_POINT('Ctrl Pts',(23.0004093438121,-59.8401800439888,
-158.16164261421));
#174331=CARTESIAN_POINT('Ctrl Pts',(22.9980884208888,-59.1666477519959,
-156.864729804607));
#174332=CARTESIAN_POINT('Ctrl Pts',(22.9957355042192,-58.5042202747206,
-155.594639653445));
#174333=CARTESIAN_POINT('Ctrl Pts',(22.9932955694915,-57.8172942024143,
-154.277577682221));
#174334=CARTESIAN_POINT('Ctrl Pts',(22.990821234914,-57.1423096389527,-152.989358956594));
#174335=CARTESIAN_POINT('Ctrl Pts',(22.9883164942772,-56.4793368434331,
-151.729934291109));
#174336=CARTESIAN_POINT('Ctrl Pts',(22.9871890935365,-56.1809282937553,
-151.163058711302));
#174337=CARTESIAN_POINT('Ctrl Pts',(22.9860555502485,-55.8849539210098,
-150.602016347596));
#174338=CARTESIAN_POINT('Ctrl Pts',(22.9849163103247,-55.591423110293,-150.046801090999));
#174339=CARTESIAN_POINT('Ctrl Pts',(22.9849163103247,-55.591423110293,-150.046801090999));
#174340=CARTESIAN_POINT('Ctrl Pts',(23.7,-55.2903249255959,-150.206318626088));
#174341=CARTESIAN_POINT('Ctrl Pts',(23.7,-55.9902808012637,-149.835491960129));
#174342=CARTESIAN_POINT('Ctrl Pts',(23.0185164903604,-55.2457834197403,
-149.428587397877));
#174343=CARTESIAN_POINT('Ctrl Pts',(23.6999999999934,-55.0174267883622,
-149.559543666635));
#174344=CARTESIAN_POINT('Ctrl Pts',(23.7,-55.679180688293,-149.248273246943));
#174345=CARTESIAN_POINT('Ctrl Pts',(23.0536516940073,-54.9992937875436,
-148.778013896122));
#174346=CARTESIAN_POINT('Ctrl Pts',(23.6999999999976,-54.8189393966138,
-148.866857423336));
#174347=CARTESIAN_POINT('Ctrl Pts',(23.7,-55.4573644110639,-148.631050162126));
#174348=CARTESIAN_POINT('Ctrl Pts',(23.1260141051261,-54.6648889616571,
-147.425793812224));
#174349=CARTESIAN_POINT('Ctrl Pts',(23.7000000000022,-54.5876251483541,
-147.465034950376));
#174350=CARTESIAN_POINT('Ctrl Pts',(23.7,-55.1564000672167,-147.34971633988));
#174351=CARTESIAN_POINT('Ctrl Pts',(23.1633521516227,-54.58000002,-146.721873935393));
#174352=CARTESIAN_POINT('Ctrl Pts',(23.7,-54.5419546351293,-146.748518174438));
#174353=CARTESIAN_POINT('Ctrl Pts',(23.7,-55.0800000213654,-146.683510743886));
#174354=CARTESIAN_POINT('Ctrl Pts',(23.2,-54.58000002,-146.023178055809));
#174355=CARTESIAN_POINT('Ctrl Pts',(23.7,-54.58000002,-146.023178055809));
#174356=CARTESIAN_POINT('Ctrl Pts',(23.7,-55.08000002,-146.023178055809));
#174357=CARTESIAN_POINT('',(23.7,-55.08000002,-146.023178055809));
#174358=CARTESIAN_POINT('Ctrl Pts',(23.7,-55.08000002,-146.023178055809));
#174359=CARTESIAN_POINT('Ctrl Pts',(23.7,-55.08000002,-146.158053606653));
#174360=CARTESIAN_POINT('Ctrl Pts',(23.7000000000707,-55.0831707493112,
-146.292669951121));
#174361=CARTESIAN_POINT('Ctrl Pts',(23.6999999992499,-55.0894565008803,
-146.427026468199));
#174362=CARTESIAN_POINT('Ctrl Pts',(23.6999999984213,-55.0958009827677,
-146.562638332538));
#174363=CARTESIAN_POINT('Ctrl Pts',(23.6999999964552,-55.1053189899911,
-146.697986218053));
#174364=CARTESIAN_POINT('Ctrl Pts',(23.6999999951529,-55.118005919724,-146.833072917224));
#174365=CARTESIAN_POINT('Ctrl Pts',(23.6999999945721,-55.1236634789143,
-146.893312944755));
#174366=CARTESIAN_POINT('Ctrl Pts',(23.6999999941814,-55.1299519000527,
-146.953501011813));
#174367=CARTESIAN_POINT('Ctrl Pts',(23.6999999942164,-55.1368740952971,
-147.013636993293));
#174368=CARTESIAN_POINT('Ctrl Pts',(23.6999999943017,-55.1537261451256,
-147.160037740544));
#174369=CARTESIAN_POINT('Ctrl Pts',(23.6999999965898,-55.1743560689037,
-147.306288458158));
#174370=CARTESIAN_POINT('Ctrl Pts',(23.6999999980531,-55.1987232126618,
-147.451788749128));
#174371=CARTESIAN_POINT('Ctrl Pts',(23.6999999995039,-55.2228814172676,
-147.596041429475));
#174372=CARTESIAN_POINT('Ctrl Pts',(23.699999999956,-55.2507128773888,-147.739555725363));
#174373=CARTESIAN_POINT('Ctrl Pts',(23.6999999999927,-55.2821282400243,
-147.881757850271));
#174374=CARTESIAN_POINT('Ctrl Pts',(23.700000000002,-55.2901469859137,-147.918054827575));
#174375=CARTESIAN_POINT('Ctrl Pts',(23.7,-55.298398982964,-147.954266404713));
#174376=CARTESIAN_POINT('Ctrl Pts',(23.7,-55.3068822390434,-147.990383251025));
#174377=CARTESIAN_POINT('Ctrl Pts',(23.7,-55.3875157587036,-148.333674601652));
#174378=CARTESIAN_POINT('Ctrl Pts',(23.7,-55.4886143891028,-148.670181748626));
#174379=CARTESIAN_POINT('Ctrl Pts',(23.7,-55.6129610034793,-148.998982220304));
#174380=CARTESIAN_POINT('Ctrl Pts',(23.7,-55.7206760510301,-149.283805081137));
#174381=CARTESIAN_POINT('Ctrl Pts',(23.7,-55.8458362712953,-149.562844907636));
#174382=CARTESIAN_POINT('Ctrl Pts',(23.7,-55.9902808012637,-149.835491960129));
#174383=CARTESIAN_POINT('Origin',(23.2,-55.08000002,-146.023178055809));
#174384=CARTESIAN_POINT('Origin',(23.2,-55.08000002,-55.24995));
#174385=CARTESIAN_POINT('',(23.7,-55.08000002,-86.035464915697));
#174386=CARTESIAN_POINT('',(23.7,-55.08000002,-146.505061715151));
#174387=CARTESIAN_POINT('Origin',(23.2,-55.08000002,-86.035464915697));
#174388=CARTESIAN_POINT('Ctrl Pts',(23.2,-54.58000002,-86.035464915697));
#174389=CARTESIAN_POINT('Ctrl Pts',(23.7,-54.58000002,-86.0354649156969));
#174390=CARTESIAN_POINT('Ctrl Pts',(23.7,-55.08000002,-86.035464915697));
#174391=CARTESIAN_POINT('Ctrl Pts',(23.163155884673,-54.58000002,-85.3330272043393));
#174392=CARTESIAN_POINT('Ctrl Pts',(23.7,-54.5417374496194,-85.3059841364058));
#174393=CARTESIAN_POINT('Ctrl Pts',(23.7,-55.0800000221098,-85.3715851430748));
#174394=CARTESIAN_POINT('Ctrl Pts',(23.1266268844869,-54.6631759768986,
-84.6443771511225));
#174395=CARTESIAN_POINT('Ctrl Pts',(23.6999999999999,-54.5866204760292,
-84.6055144627376));
#174396=CARTESIAN_POINT('Ctrl Pts',(23.7,-55.1548583802702,-84.7198400663338));
#174397=CARTESIAN_POINT('Ctrl Pts',(23.054421382878,-54.9946392637262,-83.2949364184621));
#174398=CARTESIAN_POINT('Ctrl Pts',(23.7,-54.8153941542428,-83.2070098309739));
#174399=CARTESIAN_POINT('Ctrl Pts',(23.7,-55.4531753402921,-83.4411601721359));
#174400=CARTESIAN_POINT('Ctrl Pts',(23.0184485767712,-55.2464820601011,
-82.6288059779555));
#174401=CARTESIAN_POINT('Ctrl Pts',(23.7000000000021,-55.01791265188,-82.4979478032362));
#174402=CARTESIAN_POINT('Ctrl Pts',(23.7,-55.6798282904624,-82.8091473369244));
#174403=CARTESIAN_POINT('Ctrl Pts',(22.9849163103247,-55.591423110293,-82.011841880507));
#174404=CARTESIAN_POINT('Ctrl Pts',(23.7,-55.290324925596,-81.8523243454179));
#174405=CARTESIAN_POINT('Ctrl Pts',(23.7,-55.9902808012637,-82.2231510113773));
#174406=CARTESIAN_POINT('',(23.7,-55.9902808012638,-82.2231510113773));
#174407=CARTESIAN_POINT('Ctrl Pts',(23.7,-55.9902808012637,-82.2231510113773));
#174408=CARTESIAN_POINT('Ctrl Pts',(23.7,-55.895308966207,-82.4024156114538));
#174409=CARTESIAN_POINT('Ctrl Pts',(23.7,-55.8083129339555,-82.5857246305521));
#174410=CARTESIAN_POINT('Ctrl Pts',(23.7,-55.7290034297555,-82.7720704820173));
#174411=CARTESIAN_POINT('Ctrl Pts',(23.7,-55.6467059711239,-82.9654368402717));
#174412=CARTESIAN_POINT('Ctrl Pts',(23.7,-55.5726850268913,-83.1620740930086));
#174413=CARTESIAN_POINT('Ctrl Pts',(23.7,-55.5066653875376,-83.3608873091128));
#174414=CARTESIAN_POINT('Ctrl Pts',(23.7,-55.4379479535128,-83.5678247325011));
#174415=CARTESIAN_POINT('Ctrl Pts',(23.7,-55.3778989830437,-83.77712082886));
#174416=CARTESIAN_POINT('Ctrl Pts',(23.7,-55.3262609792119,-83.9875567996252));
#174417=CARTESIAN_POINT('Ctrl Pts',(23.7,-55.3186643927325,-84.018514523233));
#174418=CARTESIAN_POINT('Ctrl Pts',(23.7,-55.3112499282573,-84.049496922863));
#174419=CARTESIAN_POINT('Ctrl Pts',(23.7,-55.304016859788,-84.0805001191198));
#174420=CARTESIAN_POINT('Ctrl Pts',(23.7,-55.21004869831,-84.4832770822505));
#174421=CARTESIAN_POINT('Ctrl Pts',(23.7,-55.1455757138287,-84.8909305418253));
#174422=CARTESIAN_POINT('Ctrl Pts',(23.7,-55.1107223807412,-85.3034811063192));
#174423=CARTESIAN_POINT('Ctrl Pts',(23.7,-55.090251973458,-85.5457844194318));
#174424=CARTESIAN_POINT('Ctrl Pts',(23.7,-55.0800000200001,-85.7897771817885));
#174425=CARTESIAN_POINT('Ctrl Pts',(23.7,-55.08000002,-86.035464915697));
#174426=CARTESIAN_POINT('',(22.9849163801915,-55.5914230811224,-82.0118419126005));
#174427=CARTESIAN_POINT('Origin',(23.2,-55.9902808012638,-82.2231510113773));
#174428=CARTESIAN_POINT('Ctrl Pts',(23.2,-54.58000002,-86.035464915697));
#174429=CARTESIAN_POINT('Ctrl Pts',(23.1920402965293,-54.5800017017972,
-85.8837121586465));
#174430=CARTESIAN_POINT('Ctrl Pts',(23.1835403629471,-54.5839598123894,
-85.7206407633663));
#174431=CARTESIAN_POINT('Ctrl Pts',(23.1697796176188,-54.5986644019983,
-85.4593001058024));
#174432=CARTESIAN_POINT('Ctrl Pts',(23.165027521493,-54.6050321375862,-85.3694015520161));
#174433=CARTESIAN_POINT('Ctrl Pts',(23.1576641956209,-54.6171785178051,
-85.2304493091738));
#174434=CARTESIAN_POINT('Ctrl Pts',(23.1539241950504,-54.6239008049671,
-85.1599475867037));
#174435=CARTESIAN_POINT('Ctrl Pts',(23.1494668404016,-54.6329698265421,
-85.0759224813336));
#174436=CARTESIAN_POINT('Ctrl Pts',(23.1472161062405,-54.6378224902552,
-85.033469831222));
#174437=CARTESIAN_POINT('Ctrl Pts',(23.1460854202932,-54.6403298113479,
-85.0121338935036));
#174438=CARTESIAN_POINT('Ctrl Pts',(23.1455997231209,-54.6414218885205,
-85.0029664772816));
#174439=CARTESIAN_POINT('Ctrl Pts',(23.1452756792326,-54.6421538486887,
-84.9968496620711));
#174440=CARTESIAN_POINT('Ctrl Pts',(23.1450102786686,-54.6427571616886,
-84.991839171787));
#174441=CARTESIAN_POINT('Ctrl Pts',(23.1411745835637,-54.651500893296,-84.9194207908848));
#174442=CARTESIAN_POINT('Ctrl Pts',(23.1350026391964,-54.6665568729644,
-84.7980543962098));
#174443=CARTESIAN_POINT('Ctrl Pts',(23.1214040625537,-54.7085737971116,
-84.5416144084218));
#174444=CARTESIAN_POINT('Ctrl Pts',(23.116147164529,-54.7259043978822,-84.4437479506998));
#174445=CARTESIAN_POINT('Ctrl Pts',(23.1072156913328,-54.7588787344353,
-84.2786960342647));
#174446=CARTESIAN_POINT('Ctrl Pts',(23.1040658786267,-54.7710385863112,
-84.2206390915918));
#174447=CARTESIAN_POINT('Ctrl Pts',(23.0991086491905,-54.791325856885,-84.1290624366227));
#174448=CARTESIAN_POINT('Ctrl Pts',(23.0965721813468,-54.8019818279521,
-84.0821516295463));
#174449=CARTESIAN_POINT('Ctrl Pts',(23.0935208041597,-54.8153795734307,
-84.0254767767619));
#174450=CARTESIAN_POINT('Ctrl Pts',(23.0921945341807,-54.8213361128053,
-84.0007729266273));
#174451=CARTESIAN_POINT('Ctrl Pts',(23.0913063774615,-54.8253557005597,
-83.9842118158473));
#174452=CARTESIAN_POINT('Ctrl Pts',(23.0907645078269,-54.8278300533453,
-83.9740948772035));
#174453=CARTESIAN_POINT('Ctrl Pts',(23.0791426045535,-54.8812408887612,
-83.7568936655029));
#174454=CARTESIAN_POINT('Ctrl Pts',(23.0688848562799,-54.9361530157815,
-83.5685045958181));
#174455=CARTESIAN_POINT('Ctrl Pts',(23.0554633667156,-55.0166580274008,
-83.3187294874312));
#174456=CARTESIAN_POINT('Ctrl Pts',(23.051304010892,-55.043196963619,-83.2409289274376));
#174457=CARTESIAN_POINT('Ctrl Pts',(23.0455019800433,-55.0818833389378,
-83.1322819992919));
#174458=CARTESIAN_POINT('Ctrl Pts',(23.0427094889204,-55.1009475486401,
-83.0799715449524));
#174459=CARTESIAN_POINT('Ctrl Pts',(23.0396275793895,-55.1225688432194,
-83.0224327427873));
#174460=CARTESIAN_POINT('Ctrl Pts',(23.0381285275456,-55.1332091208129,
-82.9945316065666));
#174461=CARTESIAN_POINT('Ctrl Pts',(23.0374948273548,-55.1377311211599,
-82.9827595784604));
#174462=CARTESIAN_POINT('Ctrl Pts',(23.0370742789371,-55.1407371415232,
-82.974952753697));
#174463=CARTESIAN_POINT('Ctrl Pts',(23.0369652251154,-55.1415168257422,
-82.9729283381724));
#174464=CARTESIAN_POINT('Ctrl Pts',(23.0169042607352,-55.2853799515071,
-82.6010865135727));
#174465=CARTESIAN_POINT('Ctrl Pts',(22.9996766784886,-55.4395892989142,
-82.2834139753259));
#174466=CARTESIAN_POINT('Ctrl Pts',(22.9849163124813,-55.5914230881085,
-82.0118419201865));
#174467=CARTESIAN_POINT('Ctrl Pts',(23.7,-66.9393955463102,-61.0621827299711));
#174468=CARTESIAN_POINT('Ctrl Pts',(23.6999999999999,-66.2910081673095,
-60.7330850354506));
#174469=CARTESIAN_POINT('Ctrl Pts',(23.0210431649761,-66.5230748737403,
-60.8508735991007));
#174470=CARTESIAN_POINT('Ctrl Pts',(23.7,-63.3447762129971,-68.1442919238122));
#174471=CARTESIAN_POINT('Ctrl Pts',(23.7000000000839,-62.6252669058498,
-67.9176543808627));
#174472=CARTESIAN_POINT('Ctrl Pts',(23.0109831737233,-62.9327835325611,
-67.9329755599233));
#174473=CARTESIAN_POINT('Ctrl Pts',(23.7,-59.7084208561779,-75.2049556739983));
#174474=CARTESIAN_POINT('Ctrl Pts',(23.7000000000403,-58.9382045046749,
-75.0250759674623));
#174475=CARTESIAN_POINT('Ctrl Pts',(22.9993168926453,-59.3018045077389,
-74.9936336228867));
#174476=CARTESIAN_POINT('Ctrl Pts',(23.7,-55.9902808012637,-82.2231510113773));
#174477=CARTESIAN_POINT('Ctrl Pts',(23.7,-55.290324925596,-81.8523243454179));
#174478=CARTESIAN_POINT('Ctrl Pts',(22.9849163103247,-55.591423110293,-82.011841880507));
#174479=CARTESIAN_POINT('',(23.7,-66.9393955463102,-61.0621827299711));
#174480=CARTESIAN_POINT('Ctrl Pts',(23.7,-66.9393955463102,-61.0621827299711));
#174481=CARTESIAN_POINT('Ctrl Pts',(23.7,-63.3447563953728,-68.1443309684329));
#174482=CARTESIAN_POINT('Ctrl Pts',(23.7,-59.7084420726901,-75.2049156266561));
#174483=CARTESIAN_POINT('Ctrl Pts',(23.7,-55.9902808012637,-82.2231510113772));
#174484=CARTESIAN_POINT('',(23.0210431649761,-66.5230748737403,-60.8508735991007));
#174485=CARTESIAN_POINT('Origin',(23.2,-66.9393955463102,-61.0621827299711));
#174486=CARTESIAN_POINT('Ctrl Pts',(22.9849163103247,-55.591423110293,-82.011841880507));
#174487=CARTESIAN_POINT('Ctrl Pts',(22.9874520115223,-56.2447590890542,
-80.7760530302538));
#174488=CARTESIAN_POINT('Ctrl Pts',(22.9899593093536,-56.9101806270537,
-79.5114224368043));
#174489=CARTESIAN_POINT('Ctrl Pts',(22.9924336508059,-57.5875975912162,
-78.2178899897237));
#174490=CARTESIAN_POINT('Ctrl Pts',(22.9948354544934,-58.2451554076757,
-76.9622787245506));
#174491=CARTESIAN_POINT('Ctrl Pts',(22.9972062002304,-58.9140154656596,
-75.679435243296));
#174492=CARTESIAN_POINT('Ctrl Pts',(22.9995429153294,-59.5941386568059,
-74.3693281841293));
#174493=CARTESIAN_POINT('Ctrl Pts',(23.0017912304752,-60.2485321994087,
-73.1087836080915));
#174494=CARTESIAN_POINT('Ctrl Pts',(23.0040080387239,-60.9133527386916,
-71.8229992084517));
#174495=CARTESIAN_POINT('Ctrl Pts',(23.0061918653351,-61.5886078011582,
-70.5119701265815));
#174496=CARTESIAN_POINT('Ctrl Pts',(23.0083322086256,-62.2504175048093,
-69.2270456345218));
#174497=CARTESIAN_POINT('Ctrl Pts',(23.010440865525,-62.9222501651157,-67.9178716804198));
#174498=CARTESIAN_POINT('Ctrl Pts',(23.0125176561367,-63.6041562644662,
-66.5844673204324));
#174499=CARTESIAN_POINT('Ctrl Pts',(23.0145386178111,-64.2677311499829,
-65.2869079550462));
#174500=CARTESIAN_POINT('Ctrl Pts',(23.0165294006075,-64.9408450698268,
-63.9664033639007));
#174501=CARTESIAN_POINT('Ctrl Pts',(23.018491050079,-65.6235878475027,-62.6229946789642));
#174502=CARTESIAN_POINT('Ctrl Pts',(23.019347233991,-65.9215785899104,-62.0366488918377));
#174503=CARTESIAN_POINT('Ctrl Pts',(23.0201978841437,-66.2214041884932,
-61.4459402241975));
#174504=CARTESIAN_POINT('Ctrl Pts',(23.0210431649761,-66.5230748737403,
-60.8508735991007));
#174505=CARTESIAN_POINT('Ctrl Pts',(25.1782904241482,-54.58000002,-84.0816077695088));
#174506=CARTESIAN_POINT('Ctrl Pts',(23.9800920467566,-54.58000002,-82.9059773201362));
#174507=CARTESIAN_POINT('Ctrl Pts',(23.0246352694011,-55.592944139339,-81.9685164608053));
#174508=CARTESIAN_POINT('Ctrl Pts',(23.9841110090257,-54.58000002,-85.2987111873827));
#174509=CARTESIAN_POINT('Ctrl Pts',(22.8383173576728,-54.5800000199764,
-84.1257656115248));
#174510=CARTESIAN_POINT('Ctrl Pts',(21.9095359072908,-55.5502317234241,
-83.1856130754768));
#174511=CARTESIAN_POINT('Ctrl Pts',(22.7486109694941,-54.58000002,-86.4914322348344));
#174512=CARTESIAN_POINT('Ctrl Pts',(21.6556870958782,-54.5800000200059,
-85.3242347169187));
#174513=CARTESIAN_POINT('Ctrl Pts',(20.7596485158525,-55.5069863868931,
-84.3783409260868));
#174514=CARTESIAN_POINT('Ctrl Pts',(20.1853568720873,-54.58000002,-88.7908549573443));
#174515=CARTESIAN_POINT('Ctrl Pts',(19.2046498564035,-54.580000019994,-87.6346041928195));
#174516=CARTESIAN_POINT('Ctrl Pts',(18.3831304802005,-55.4209867081881,
-86.677763648685));
#174517=CARTESIAN_POINT('Ctrl Pts',(18.8674767865624,-54.58000002,-89.8890267533221));
#174518=CARTESIAN_POINT('Ctrl Pts',(17.9458952665738,-54.5800000199822,
-88.738506470326));
#174519=CARTESIAN_POINT('Ctrl Pts',(17.1656615705366,-55.378552771758,-87.7759223265742));
#174520=CARTESIAN_POINT('Ctrl Pts',(17.501426021519,-54.58000002,-90.9187660074097));
#174521=CARTESIAN_POINT('Ctrl Pts',(16.6397068497462,-54.58000002,-89.7756104658071));
#174522=CARTESIAN_POINT('Ctrl Pts',(15.908562035693,-55.3376387148139,-88.8056746987062));
#174523=CARTESIAN_POINT('',(17.3782102443508,-55.3867109640818,-87.5561378285247));
#174524=CARTESIAN_POINT('Ctrl Pts',(17.3782874561047,-55.3867051039103,
-87.556225265873));
#174525=CARTESIAN_POINT('Ctrl Pts',(18.0129714837723,-55.4084038769681,
-86.9972203403477));
#174526=CARTESIAN_POINT('Ctrl Pts',(18.6500362552073,-55.4308164859441,
-86.4112422645402));
#174527=CARTESIAN_POINT('Ctrl Pts',(19.2925057736155,-55.4539248269632,
-85.7964162320036));
#174528=CARTESIAN_POINT('Ctrl Pts',(19.3853509908652,-55.4572642833587,
-85.7075658586768));
#174529=CARTESIAN_POINT('Ctrl Pts',(19.4783091534519,-55.4606182248066,
-85.6181130637534));
#174530=CARTESIAN_POINT('Ctrl Pts',(19.5713894980265,-55.4639865475406,
-85.5280522873859));
#174531=CARTESIAN_POINT('Ctrl Pts',(19.9333948730858,-55.4770865305736,
-85.1777905293742));
#174532=CARTESIAN_POINT('Ctrl Pts',(20.296400295736,-55.4903745638692,-84.8191217954611));
#174533=CARTESIAN_POINT('Ctrl Pts',(20.6606795729677,-55.5038451834361,
-84.4518497844382));
#174534=CARTESIAN_POINT('Ctrl Pts',(21.0070859618513,-55.5166548845963,
-84.1025974963494));
#174535=CARTESIAN_POINT('Ctrl Pts',(21.3546440024347,-55.5296297142268,
-83.7455647941717));
#174536=CARTESIAN_POINT('Ctrl Pts',(21.7035673985787,-55.542761750743,-83.3806236068663));
#174537=CARTESIAN_POINT('Ctrl Pts',(22.0308691120961,-55.5550800363645,
-83.0382966741983));
#174538=CARTESIAN_POINT('Ctrl Pts',(22.3593719626064,-55.5675366547334,
-82.6890106640993));
#174539=CARTESIAN_POINT('Ctrl Pts',(22.6892363727748,-55.580122001814,-82.3327033186524));
#174540=CARTESIAN_POINT('Ctrl Pts',(22.7876738992419,-55.5838776977853,
-82.2263747404044));
#174541=CARTESIAN_POINT('Ctrl Pts',(22.886232576619,-55.5876448353322,-82.1194212171195));
#174542=CARTESIAN_POINT('Ctrl Pts',(22.9849164160517,-55.5914231002813,
-82.0118419843783));
#174543=CARTESIAN_POINT('Ctrl Pts',(17.3782124086123,-55.3866898704104,
-87.5561779776695));
#174544=CARTESIAN_POINT('Ctrl Pts',(17.3842286240988,-55.3280540017891,
-87.6677848839424));
#174545=CARTESIAN_POINT('Ctrl Pts',(17.3906321444487,-55.2684282622658,
-87.7889551607595));
#174546=CARTESIAN_POINT('Ctrl Pts',(17.4010617540412,-55.1796759858784,
-87.9857741968713));
#174547=CARTESIAN_POINT('Ctrl Pts',(17.4046735378182,-55.1502087677355,
-88.053893722921));
#174548=CARTESIAN_POINT('Ctrl Pts',(17.4102842569604,-55.1064962524215,
-88.15988362143));
#174549=CARTESIAN_POINT('Ctrl Pts',(17.4131375697184,-55.0847624375805,
-88.213830936193));
#174550=CARTESIAN_POINT('Ctrl Pts',(17.4165447907984,-55.059691963569,-88.2784434090018));
#174551=CARTESIAN_POINT('Ctrl Pts',(17.4182670115253,-55.0472373150833,
-88.3111687633467));
#174552=CARTESIAN_POINT('Ctrl Pts',(17.4191326431444,-55.0410312913305,
-88.3276362900039));
#174553=CARTESIAN_POINT('Ctrl Pts',(17.4195045820392,-55.0383762555384,
-88.3347162758178));
#174554=CARTESIAN_POINT('Ctrl Pts',(17.4197527515741,-55.0366072874539,
-88.3394412613556));
#174555=CARTESIAN_POINT('Ctrl Pts',(17.4199359858737,-55.0353036730375,
-88.3429308972497));
#174556=CARTESIAN_POINT('Ctrl Pts',(17.4241772216026,-55.0051590733497,
-88.4237156579429));
#174557=CARTESIAN_POINT('Ctrl Pts',(17.4296648760824,-54.9665842581938,
-88.5311376661661));
#174558=CARTESIAN_POINT('Ctrl Pts',(17.4403028769676,-54.901358367034,-88.7357239344459));
#174559=CARTESIAN_POINT('Ctrl Pts',(17.4442474101977,-54.8784231995579,
-88.811164929113));
#174560=CARTESIAN_POINT('Ctrl Pts',(17.4507497336677,-54.8432876528706,
-88.9353776653523));
#174561=CARTESIAN_POINT('Ctrl Pts',(17.4541462110081,-54.8255399335536,
-89.0002461963404));
#174562=CARTESIAN_POINT('Ctrl Pts',(17.4577462028239,-54.8077493096576,
-89.0692833205201));
#174563=CARTESIAN_POINT('Ctrl Pts',(17.4601887667519,-54.7959065114956,
-89.1162363644095));
#174564=CARTESIAN_POINT('Ctrl Pts',(17.4615109836412,-54.7896224138083,
-89.1417160608586));
#174565=CARTESIAN_POINT('Ctrl Pts',(17.4816184041917,-54.6958051164707,
-89.5304494018354));
#174566=CARTESIAN_POINT('Ctrl Pts',(17.4976217601376,-54.6506607776598,
-89.8378333642392));
#174567=CARTESIAN_POINT('Ctrl Pts',(17.5128265027635,-54.6172691760158,
-90.1417732814389));
#174568=CARTESIAN_POINT('Ctrl Pts',(17.5156576011187,-54.611790867425,-90.198591549364));
#174569=CARTESIAN_POINT('Ctrl Pts',(17.5189723296823,-54.6060867273699,
-90.2646304500862));
#174570=CARTESIAN_POINT('Ctrl Pts',(17.5196241069914,-54.6050032951348,
-90.2775891192987));
#174571=CARTESIAN_POINT('Ctrl Pts',(17.5205858356443,-54.6034581849455,
-90.296653285516));
#174572=CARTESIAN_POINT('Ctrl Pts',(17.5209033418797,-54.6029538192376,
-90.3029333388735));
#174573=CARTESIAN_POINT('Ctrl Pts',(17.5218721007445,-54.6014589661519,
-90.3220976255049));
#174574=CARTESIAN_POINT('Ctrl Pts',(17.5242872361714,-54.5978262790508,
-90.3698821869256));
#174575=CARTESIAN_POINT('Ctrl Pts',(17.526667856459,-54.5947081383125,-90.4170335494899));
#174576=CARTESIAN_POINT('Ctrl Pts',(17.5360744592059,-54.5837858480397,
-90.6035864662938));
#174577=CARTESIAN_POINT('Ctrl Pts',(17.5432187572949,-54.5800000268131,
-90.7462467549563));
#174578=CARTESIAN_POINT('Ctrl Pts',(17.55,-54.58000002,-90.8821060618472));
#174579=CARTESIAN_POINT('Origin',(16.55,-70.08000002,-174.34995));
#174580=CARTESIAN_POINT('',(17.05,-70.08000002,-176.84995));
#174581=CARTESIAN_POINT('Origin',(16.55,-70.08000002,-176.84995));
#174582=CARTESIAN_POINT('',(17.05,-72.58000002,-174.34995));
#174583=CARTESIAN_POINT('Origin',(17.05,-70.08000002,-174.34995));
#174584=CARTESIAN_POINT('Origin',(16.55,-72.58000002,-174.34995));
#174585=CARTESIAN_POINT('Origin',(16.55,-72.58000002,-55.24995));
#174586=CARTESIAN_POINT('',(17.05,-72.58000002,-58.24995));
#174587=CARTESIAN_POINT('',(17.05,-72.58000002,-174.34995));
#174588=CARTESIAN_POINT('Origin',(16.55,-72.58000002,-58.24995));
#174589=CARTESIAN_POINT('Ctrl Pts',(17.3782102443508,-55.3867109640818,
-87.5561378285247));
#174590=CARTESIAN_POINT('Ctrl Pts',(17.0499999999999,-55.4939415516614,
-87.6101736986065));
#174591=CARTESIAN_POINT('Ctrl Pts',(17.05,-55.8060398696737,-87.7674469593951));
#174592=CARTESIAN_POINT('Ctrl Pts',(17.4056693808345,-55.1158123847072,
-88.0713943440392));
#174593=CARTESIAN_POINT('Ctrl Pts',(17.05,-55.2114257865401,-88.1214372575005));
#174594=CARTESIAN_POINT('Ctrl Pts',(17.05,-55.5622216475024,-88.2512880043934));
#174595=CARTESIAN_POINT('Ctrl Pts',(17.4339593787444,-54.9179776170691,
-88.6091505606876));
#174596=CARTESIAN_POINT('Ctrl Pts',(17.05,-55.0036171481024,-88.6486574682591));
#174597=CARTESIAN_POINT('Ctrl Pts',(17.05,-55.3841798573999,-88.7556128927223));
#174598=CARTESIAN_POINT('Ctrl Pts',(17.4916046269366,-54.6493515142325,
-89.7235249939138));
#174599=CARTESIAN_POINT('Ctrl Pts',(17.0499999999999,-54.6987064687868,
-89.7439019899564));
#174600=CARTESIAN_POINT('Ctrl Pts',(17.05,-55.1424163647715,-89.7992759203947));
#174601=CARTESIAN_POINT('Ctrl Pts',(17.5211522384036,-54.58000002,-90.3041534556916));
#174602=CARTESIAN_POINT('Ctrl Pts',(17.0500000000018,-54.6080382399387,
-90.3203722819605));
#174603=CARTESIAN_POINT('Ctrl Pts',(17.05,-55.0800000196891,-90.3423386098486));
#174604=CARTESIAN_POINT('Ctrl Pts',(17.55,-54.58000002,-90.8821060618472));
#174605=CARTESIAN_POINT('Ctrl Pts',(17.0499999999999,-54.58000002,-90.8821060618472));
#174606=CARTESIAN_POINT('Ctrl Pts',(17.05,-55.08000002,-90.8821060618472));
#174607=CARTESIAN_POINT('',(17.05,-55.08000002,-90.8821060618472));
#174608=CARTESIAN_POINT('Origin',(17.55,-55.08000002,-90.8821060618472));
#174609=CARTESIAN_POINT('',(17.05,-55.8060398696737,-87.7674469593951));
#174610=CARTESIAN_POINT('Origin',(17.55,-55.8060398696737,-87.7674469593951));
#174611=CARTESIAN_POINT('Ctrl Pts',(17.05,-55.08000002,-90.8821060618472));
#174612=CARTESIAN_POINT('Ctrl Pts',(17.05,-55.0800000198976,-90.7044011282776));
#174613=CARTESIAN_POINT('Ctrl Pts',(17.05,-55.0867609195445,-90.5266735432509));
#174614=CARTESIAN_POINT('Ctrl Pts',(17.05,-55.1000918811982,-90.3496297314756));
#174615=CARTESIAN_POINT('Ctrl Pts',(17.05,-55.1137303582782,-90.1685019155117));
#174616=CARTESIAN_POINT('Ctrl Pts',(17.05,-55.1342455055614,-89.988088644052));
#174617=CARTESIAN_POINT('Ctrl Pts',(17.05,-55.1614876321833,-89.8091398363491));
#174618=CARTESIAN_POINT('Ctrl Pts',(17.05,-55.1887297588052,-89.6301910286463));
#174619=CARTESIAN_POINT('Ctrl Pts',(17.05,-55.2226990580678,-89.4527054855482));
#174620=CARTESIAN_POINT('Ctrl Pts',(17.05,-55.2632981110657,-89.2774444065538));
#174621=CARTESIAN_POINT('Ctrl Pts',(17.05,-55.3408916382099,-88.942482768631));
#174622=CARTESIAN_POINT('Ctrl Pts',(17.05,-55.4420234811562,-88.6147745215355));
#174623=CARTESIAN_POINT('Ctrl Pts',(17.05,-55.5689958159258,-88.2950290565852));
#174624=CARTESIAN_POINT('Ctrl Pts',(17.05,-55.6398317020634,-88.1166480463494));
#174625=CARTESIAN_POINT('Ctrl Pts',(17.05,-55.7187108542584,-87.9407455779152));
#174626=CARTESIAN_POINT('Ctrl Pts',(17.05,-55.8060398696737,-87.7674469593951));
#174627=CARTESIAN_POINT('Origin',(17.55,-55.08000002,-55.24995));
#174628=CARTESIAN_POINT('',(17.05,-55.08000002,-141.176536909659));
#174629=CARTESIAN_POINT('Origin',(17.55,-55.08000002,-141.176536909659));
#174630=CARTESIAN_POINT('',(17.05,-55.08000002,-91.2551956845905));
#174631=CARTESIAN_POINT('Ctrl Pts',(17.55,-54.58000002,-141.176536909659));
#174632=CARTESIAN_POINT('Ctrl Pts',(17.0499999999999,-54.5800000199999,
-141.176536909659));
#174633=CARTESIAN_POINT('Ctrl Pts',(17.05,-55.08000002,-141.176536909659));
#174634=CARTESIAN_POINT('Ctrl Pts',(17.5210482604771,-54.58000002,-141.756572644947));
#174635=CARTESIAN_POINT('Ctrl Pts',(17.05,-54.6081354389567,-141.740217950908));
#174636=CARTESIAN_POINT('Ctrl Pts',(17.05,-55.0800000225241,-141.718258289701));
#174637=CARTESIAN_POINT('Ctrl Pts',(17.4921321192376,-54.6477817704653,
-142.324800749723));
#174638=CARTESIAN_POINT('Ctrl Pts',(17.05,-54.6967583223106,-142.304574247435));
#174639=CARTESIAN_POINT('Ctrl Pts',(17.05,-55.1410035947335,-142.249713786832));
#174640=CARTESIAN_POINT('Ctrl Pts',(17.4345568574947,-54.9143222027725,
-143.438059836182));
#174641=CARTESIAN_POINT('Ctrl Pts',(17.05,-54.9996847823657,-143.398819151438));
#174642=CARTESIAN_POINT('Ctrl Pts',(17.05,-55.3808899851806,-143.292313830226));
#174643=CARTESIAN_POINT('Ctrl Pts',(17.4056704634348,-55.1158017299176,
-143.987228363879));
#174644=CARTESIAN_POINT('Ctrl Pts',(17.05,-55.2114362483487,-143.937224655552));
#174645=CARTESIAN_POINT('Ctrl Pts',(17.05,-55.5622193543528,-143.807350422822));
#174646=CARTESIAN_POINT('Ctrl Pts',(17.3782102443502,-55.3867109640874,
-144.502505142992));
#174647=CARTESIAN_POINT('Ctrl Pts',(17.05,-55.4939415516672,-144.44846927291));
#174648=CARTESIAN_POINT('Ctrl Pts',(17.05,-55.8060398696787,-144.291196012121));
#174649=CARTESIAN_POINT('',(17.05,-55.8060398696787,-144.291196012121));
#174650=CARTESIAN_POINT('Origin',(17.55,-55.8060398696787,-144.291196012121));
#174651=CARTESIAN_POINT('Ctrl Pts',(17.05,-55.8060398696787,-144.291196012121));
#174652=CARTESIAN_POINT('Ctrl Pts',(17.05,-55.6831540655492,-144.047337313039));
#174653=CARTESIAN_POINT('Ctrl Pts',(17.05,-55.5762002500364,-143.795681932959));
#174654=CARTESIAN_POINT('Ctrl Pts',(17.05,-55.4849662480682,-143.539333784846));
#174655=CARTESIAN_POINT('Ctrl Pts',(17.05,-55.3950897214922,-143.286799853971));
#174656=CARTESIAN_POINT('Ctrl Pts',(17.05,-55.3204688827065,-143.029710172846));
#174657=CARTESIAN_POINT('Ctrl Pts',(17.05,-55.2609467896032,-142.77101380861));
#174658=CARTESIAN_POINT('Ctrl Pts',(17.05,-55.1772261529212,-142.407145147547));
#174659=CARTESIAN_POINT('Ctrl Pts',(17.05,-55.1222258452557,-142.038367265712));
#174660=CARTESIAN_POINT('Ctrl Pts',(17.05,-55.0966366319611,-141.66456206908));
#174661=CARTESIAN_POINT('Ctrl Pts',(17.05,-55.085565206749,-141.50283156839));
#174662=CARTESIAN_POINT('Ctrl Pts',(17.05,-55.0800000200001,-141.340159872026));
#174663=CARTESIAN_POINT('Ctrl Pts',(17.05,-55.08000002,-141.176536909659));
#174664=CARTESIAN_POINT('Ctrl Pts',(17.05,-69.1496478013716,-171.237717270032));
#174665=CARTESIAN_POINT('Ctrl Pts',(17.0499999999999,-68.809126121555,-171.404072041895));
#174666=CARTESIAN_POINT('Ctrl Pts',(17.4148840712406,-68.7171063154928,
-171.449026400902));
#174667=CARTESIAN_POINT('Ctrl Pts',(17.05,-64.7499600097223,-162.23172927942));
#174668=CARTESIAN_POINT('Ctrl Pts',(17.05,-64.4501495263081,-162.463595694272));
#174669=CARTESIAN_POINT('Ctrl Pts',(17.4052437025222,-64.32043537753,-162.443049517833));
#174670=CARTESIAN_POINT('Ctrl Pts',(17.05,-60.3166713897233,-153.242244037967));
#174671=CARTESIAN_POINT('Ctrl Pts',(17.0500000000351,-60.0450216003573,
-153.507379856866));
#174672=CARTESIAN_POINT('Ctrl Pts',(17.393699089013,-59.8910064308848,-153.453571789302));
#174673=CARTESIAN_POINT('Ctrl Pts',(17.05,-55.8060398696787,-144.291196012121));
#174674=CARTESIAN_POINT('Ctrl Pts',(17.05,-55.4939415516665,-144.448469272909));
#174675=CARTESIAN_POINT('Ctrl Pts',(17.3782102443508,-55.3867109640869,
-144.502505142991));
#174676=CARTESIAN_POINT('',(17.05,-69.1496478013716,-171.237717270032));
#174677=CARTESIAN_POINT('',(17.4148840712406,-68.7171063154928,-171.449026400902));
#174678=CARTESIAN_POINT('Origin',(17.55,-69.1496478013716,-171.237717270032));
#174679=CARTESIAN_POINT('Ctrl Pts',(17.3782102443508,-55.3867109640869,
-144.502505142991));
#174680=CARTESIAN_POINT('Ctrl Pts',(17.380720868236,-56.1168229918889,-145.953404949254));
#174681=CARTESIAN_POINT('Ctrl Pts',(17.3831954450421,-56.8646679860372,
-147.444471578493));
#174682=CARTESIAN_POINT('Ctrl Pts',(17.3856269123549,-57.6301346747941,
-148.975776438915));
#174683=CARTESIAN_POINT('Ctrl Pts',(17.3879710060604,-58.3680946866318,
-150.452054596438));
#174684=CARTESIAN_POINT('Ctrl Pts',(17.390275021825,-59.122432474325,-151.965731174827));
#174685=CARTESIAN_POINT('Ctrl Pts',(17.3925346451406,-59.8930912343523,
-153.516847722935));
#174686=CARTESIAN_POINT('Ctrl Pts',(17.3946832424879,-60.6258838887878,
-154.99175058732));
#174687=CARTESIAN_POINT('Ctrl Pts',(17.3967917011905,-61.3734335506627,
-156.500505714666));
#174688=CARTESIAN_POINT('Ctrl Pts',(17.3988582507656,-62.1357307859902,
-158.043123599146));
#174689=CARTESIAN_POINT('Ctrl Pts',(17.4008823945055,-62.8823855943037,
-159.554086787072));
#174690=CARTESIAN_POINT('Ctrl Pts',(17.4028663182098,-63.6431878049361,
-161.097535507723));
#174691=CARTESIAN_POINT('Ctrl Pts',(17.4048103792945,-64.4181692783863,
-162.673452998055));
#174692=CARTESIAN_POINT('Ctrl Pts',(17.406689765421,-65.1673686945184,-164.196942918881));
#174693=CARTESIAN_POINT('Ctrl Pts',(17.4085318928252,-65.9298195526288,
-165.750777247564));
#174694=CARTESIAN_POINT('Ctrl Pts',(17.4103390985595,-66.7055930840024,
-167.33491867873));
#174695=CARTESIAN_POINT('Ctrl Pts',(17.4118784989981,-67.3664066769433,
-168.684310155134));
#174696=CARTESIAN_POINT('Ctrl Pts',(17.4133925883603,-68.0368875784479,
-170.055691692052));
#174697=CARTESIAN_POINT('Ctrl Pts',(17.4148840712406,-68.7171063154928,
-171.449026400902));
#174698=CARTESIAN_POINT('Ctrl Pts',(17.05,-69.1496478013716,-171.237717270032));
#174699=CARTESIAN_POINT('Ctrl Pts',(17.05,-64.7499424271364,-162.231693289135));
#174700=CARTESIAN_POINT('Ctrl Pts',(17.05,-60.3166901832211,-153.242281332923));
#174701=CARTESIAN_POINT('Ctrl Pts',(17.05,-55.8060398696787,-144.291196012121));
#174702=CARTESIAN_POINT('Ctrl Pts',(17.05,-55.8060398696737,-87.7674469593951));
#174703=CARTESIAN_POINT('Ctrl Pts',(17.0499999999999,-55.4939415516614,
-87.6101736986065));
#174704=CARTESIAN_POINT('Ctrl Pts',(17.3782102443508,-55.3867109640818,
-87.5561378285247));
#174705=CARTESIAN_POINT('Ctrl Pts',(17.05,-60.2763921316847,-78.8963304394585));
#174706=CARTESIAN_POINT('Ctrl Pts',(17.0499999998605,-60.0039146247672,
-78.6330864204663));
#174707=CARTESIAN_POINT('Ctrl Pts',(17.3935607753682,-59.8507835488919,
-78.6850032603101));
#174708=CARTESIAN_POINT('Ctrl Pts',(17.05,-64.6707170319981,-69.9874285386638));
#174709=CARTESIAN_POINT('Ctrl Pts',(17.0499999999316,-64.3705933782976,
-69.756601957739));
#174710=CARTESIAN_POINT('Ctrl Pts',(17.4050347595683,-64.2412639062053,
-69.7761086016325));
#174711=CARTESIAN_POINT('Ctrl Pts',(17.05,-69.0317756926871,-61.0621827299711));
#174712=CARTESIAN_POINT('Ctrl Pts',(17.05,-68.6914563568371,-60.8958957033858));
#174713=CARTESIAN_POINT('Ctrl Pts',(17.4146253252297,-68.5993151180197,
-60.8508735991007));
#174714=CARTESIAN_POINT('',(17.4146253252297,-68.5993151180197,-60.8508735991007));
#174715=CARTESIAN_POINT('Ctrl Pts',(17.4146253252297,-68.5993151180197,
-60.8508735991007));
#174716=CARTESIAN_POINT('Ctrl Pts',(17.4128776238819,-67.8051417363082,
-62.4773308663589));
#174717=CARTESIAN_POINT('Ctrl Pts',(17.4110988447299,-67.0242728470718,
-64.0737822849279));
#174718=CARTESIAN_POINT('Ctrl Pts',(17.4092848745463,-66.2565999860111,
-65.6401711202791));
#174719=CARTESIAN_POINT('Ctrl Pts',(17.407428178194,-65.4708453943339,-67.2434546048986));
#174720=CARTESIAN_POINT('Ctrl Pts',(17.4055346211606,-64.6989159435754,
-68.8152427226574));
#174721=CARTESIAN_POINT('Ctrl Pts',(17.4036021153684,-63.9407442116168,
-70.3555001505591));
#174722=CARTESIAN_POINT('Ctrl Pts',(17.4015949038351,-63.1532634957471,
-71.9552999990896));
#174723=CARTESIAN_POINT('Ctrl Pts',(17.3995456779925,-62.3806248102645,
-73.521084285121));
#174724=CARTESIAN_POINT('Ctrl Pts',(17.3974544925988,-61.6228031213183,
-75.0528398018804));
#174725=CARTESIAN_POINT('Ctrl Pts',(17.3953146083248,-60.8473335146984,
-76.6202663685062));
#174726=CARTESIAN_POINT('Ctrl Pts',(17.3931308036726,-60.0873807420183,
-78.1520580110134));
#174727=CARTESIAN_POINT('Ctrl Pts',(17.3909054532109,-59.3429628661628,
-79.6482351286049));
#174728=CARTESIAN_POINT('Ctrl Pts',(17.3885629111999,-58.5593424081476,
-81.2232040219992));
#174729=CARTESIAN_POINT('Ctrl Pts',(17.3861743366006,-57.7929361965902,
-82.7587086075468));
#174730=CARTESIAN_POINT('Ctrl Pts',(17.3837449346187,-57.0438170021005,
-84.2547997688877));
#174731=CARTESIAN_POINT('Ctrl Pts',(17.3819219752636,-56.481697660022,-85.3774272298958));
#174732=CARTESIAN_POINT('Ctrl Pts',(17.380076081124,-55.9293130928866,-86.4778631342493));
#174733=CARTESIAN_POINT('Ctrl Pts',(17.3782102443508,-55.3867109640818,
-87.5561378285247));
#174734=CARTESIAN_POINT('',(17.05,-69.0317756926871,-61.0621827299711));
#174735=CARTESIAN_POINT('Origin',(17.55,-69.0317756926871,-61.0621827299711));
#174736=CARTESIAN_POINT('Ctrl Pts',(17.05,-55.8060398696737,-87.7674469593951));
#174737=CARTESIAN_POINT('Ctrl Pts',(17.05,-60.2764102501238,-78.896294484622));
#174738=CARTESIAN_POINT('Ctrl Pts',(17.05,-64.6707000732441,-69.9874632456984));
#174739=CARTESIAN_POINT('Ctrl Pts',(17.05,-69.0317756926871,-61.0621827299711));
#174740=CARTESIAN_POINT('Origin',(16.55,-70.08000002,-58.24995));
#174741=CARTESIAN_POINT('',(17.05,-70.08000002,-55.74995));
#174742=CARTESIAN_POINT('Origin',(17.05,-70.08000002,-58.24995));
#174743=CARTESIAN_POINT('',(16.55,-70.08000002,-55.24995));
#174744=CARTESIAN_POINT('Origin',(16.55,-70.08000002,-55.74995));
#174745=CARTESIAN_POINT('Origin',(16.55,-70.08000002,-58.24995));
#174746=CARTESIAN_POINT('Origin',(-3.3975957231091E-14,-70.08000002,-58.24995));
#174747=CARTESIAN_POINT('',(16.05,-70.08000002,-55.24995));
#174748=CARTESIAN_POINT('',(41.5,-70.08000002,-55.24995));
#174749=CARTESIAN_POINT('Origin',(16.05,-70.08000002,-58.24995));
#174750=CARTESIAN_POINT('Origin',(16.05,-70.08000002,-58.24995));
#174751=CARTESIAN_POINT('',(15.55,-70.08000002,-55.74995));
#174752=CARTESIAN_POINT('Origin',(16.05,-70.08000002,-55.74995));
#174753=CARTESIAN_POINT('',(15.55,-72.58000002,-58.24995));
#174754=CARTESIAN_POINT('Origin',(15.55,-70.08000002,-58.24995));
#174755=CARTESIAN_POINT('Origin',(16.05,-72.58000002,-58.24995));
#174756=CARTESIAN_POINT('Origin',(16.05,-72.58000002,-55.24995));
#174757=CARTESIAN_POINT('',(15.55,-72.58000002,-174.34995));
#174758=CARTESIAN_POINT('',(15.55,-72.58000002,-58.24995));
#174759=CARTESIAN_POINT('Origin',(16.05,-72.58000002,-174.34995));
#174760=CARTESIAN_POINT('Origin',(16.05,-70.08000002,-174.34995));
#174761=CARTESIAN_POINT('',(15.55,-70.08000002,-176.84995));
#174762=CARTESIAN_POINT('Origin',(15.55,-70.08000002,-174.34995));
#174763=CARTESIAN_POINT('Origin',(16.05,-70.08000002,-176.84995));
#174764=CARTESIAN_POINT('Ctrl Pts',(15.55,-55.7328910677637,-142.237228854888));
#174765=CARTESIAN_POINT('Ctrl Pts',(15.55,-55.1214867472491,-142.539470838321));
#174766=CARTESIAN_POINT('Ctrl Pts',(14.8995694550282,-55.3054345175152,
-142.448537985759));
#174767=CARTESIAN_POINT('Ctrl Pts',(15.55,-60.4987241912205,-151.878017105041));
#174768=CARTESIAN_POINT('Ctrl Pts',(15.5500000000182,-59.8063638088321,
-151.967058554268));
#174769=CARTESIAN_POINT('Ctrl Pts',(14.9144862578123,-60.0660270491051,
-152.089344301479));
#174770=CARTESIAN_POINT('Ctrl Pts',(15.55,-65.1981673386922,-161.551271258869));
#174771=CARTESIAN_POINT('Ctrl Pts',(15.549999999915,-64.5626692295555,-161.718722395353));
#174772=CARTESIAN_POINT('Ctrl Pts',(14.9252396269456,-64.7624344426112,
-161.762591659591));
#174773=CARTESIAN_POINT('Ctrl Pts',(15.55,-69.870344670579,-171.237717270032));
#174774=CARTESIAN_POINT('Ctrl Pts',(15.5499999999999,-69.3001099534342,
-171.51276528209));
#174775=CARTESIAN_POINT('Ctrl Pts',(14.9341313545396,-69.4322546019743,
-171.449026400902));
#174776=CARTESIAN_POINT('',(14.9341313545396,-69.4322546019744,-171.449026400902));
#174777=CARTESIAN_POINT('',(15.55,-69.870344670579,-171.237717270032));
#174778=CARTESIAN_POINT('Origin',(15.05,-69.870344670579,-171.237717270032));
#174779=CARTESIAN_POINT('',(15.55,-55.7328910677637,-142.237228854888));
#174780=CARTESIAN_POINT('Ctrl Pts',(15.55,-55.7328910677637,-142.237228854888));
#174781=CARTESIAN_POINT('Ctrl Pts',(15.55,-60.4987378575172,-151.878044750548));
#174782=CARTESIAN_POINT('Ctrl Pts',(15.55,-65.1981545194713,-161.551244681819));
#174783=CARTESIAN_POINT('Ctrl Pts',(15.55,-69.870344670579,-171.237717270032));
#174784=CARTESIAN_POINT('Origin',(15.05,-55.7328910677637,-142.237228854888));
#174785=CARTESIAN_POINT('Ctrl Pts',(14.9341313545396,-69.4322546019743,
-171.449026400902));
#174786=CARTESIAN_POINT('Ctrl Pts',(14.9325246708401,-68.5884451336383,
-169.698743719727));
#174787=CARTESIAN_POINT('Ctrl Pts',(14.9310233213259,-67.7597775482042,
-167.982185348246));
#174788=CARTESIAN_POINT('Ctrl Pts',(14.9295360070345,-66.9461670298033,
-166.299394335229));
#174789=CARTESIAN_POINT('Ctrl Pts',(14.9279426283007,-66.0745357241675,
-164.496598901032));
#174790=CARTESIAN_POINT('Ctrl Pts',(14.9263653852153,-65.2201851979954,
-162.732558509485));
#174791=CARTESIAN_POINT('Ctrl Pts',(14.9246943502029,-64.3830706161263,
-161.007300204738));
#174792=CARTESIAN_POINT('Ctrl Pts',(14.9230233151905,-63.5459560342572,
-159.282041899991));
#174793=CARTESIAN_POINT('Ctrl Pts',(14.9212584740815,-62.7260779904469,
-157.59556600155));
#174794=CARTESIAN_POINT('Ctrl Pts',(14.9192919729217,-61.923445829236,-155.947872412608));
#174795=CARTESIAN_POINT('Ctrl Pts',(14.9171604680817,-61.0534670205351,
-154.161925406137));
#174796=CARTESIAN_POINT('Ctrl Pts',(14.9147932490124,-60.2037518026807,
-152.421545017592));
#174797=CARTESIAN_POINT('Ctrl Pts',(14.9123287456633,-59.3742952696168,
-150.726717945526));
#174798=CARTESIAN_POINT('Ctrl Pts',(14.9096915492495,-58.4867169284227,
-148.91313068535));
#174799=CARTESIAN_POINT('Ctrl Pts',(14.9069430335476,-57.6223358513715,
-147.151703764968));
#174800=CARTESIAN_POINT('Ctrl Pts',(14.904257075721,-56.7812024435093,-145.4423974361));
#174801=CARTESIAN_POINT('Ctrl Pts',(14.902659968314,-56.2810529688437,-144.426020420951));
#174802=CARTESIAN_POINT('Ctrl Pts',(14.901085044351,-55.789124173773,-143.428071155623));
#174803=CARTESIAN_POINT('Ctrl Pts',(14.8995694550282,-55.3054345175152,
-142.448537985759));
#174804=CARTESIAN_POINT('Ctrl Pts',(14.8995694550282,-55.3054345175152,
-142.448537985759));
#174805=CARTESIAN_POINT('Ctrl Pts',(15.55,-55.1214867472491,-142.539470838321));
#174806=CARTESIAN_POINT('Ctrl Pts',(15.55,-55.7328910677637,-142.237228854888));
#174807=CARTESIAN_POINT('Ctrl Pts',(14.923902352475,-55.0632436795865,-141.975933471946));
#174808=CARTESIAN_POINT('Ctrl Pts',(15.55,-54.9185275760486,-142.049333574245));
#174809=CARTESIAN_POINT('Ctrl Pts',(15.55,-55.5149133573324,-141.796282446699));
#174810=CARTESIAN_POINT('Ctrl Pts',(14.9487965116602,-54.8849324628699,
-141.484081280379));
#174811=CARTESIAN_POINT('Ctrl Pts',(15.5499999999978,-54.7697596388846,
-141.534069766353));
#174812=CARTESIAN_POINT('Ctrl Pts',(15.55,-55.354439218511,-141.337957116977));
#174813=CARTESIAN_POINT('Ctrl Pts',(14.999232255606,-54.6427941514753,-140.466078071863));
#174814=CARTESIAN_POINT('Ctrl Pts',(15.550000000002,-54.5906769405451,-140.486936595447));
#174815=CARTESIAN_POINT('Ctrl Pts',(15.55,-55.1365147383997,-140.390621931638));
#174816=CARTESIAN_POINT('Ctrl Pts',(15.0249522987129,-54.58000002,-139.93601039575));
#174817=CARTESIAN_POINT('Ctrl Pts',(15.55,-54.554309680371,-139.949574386333));
#174818=CARTESIAN_POINT('Ctrl Pts',(15.55,-55.0800000201344,-139.897989788153));
#174819=CARTESIAN_POINT('Ctrl Pts',(15.05,-54.58000002,-139.407335470919));
#174820=CARTESIAN_POINT('Ctrl Pts',(15.55,-54.58000002,-139.407335470919));
#174821=CARTESIAN_POINT('Ctrl Pts',(15.55,-55.08000002,-139.407335470919));
#174822=CARTESIAN_POINT('',(15.55,-55.08000002,-139.407335470919));
#174823=CARTESIAN_POINT('Ctrl Pts',(15.55,-55.08000002,-139.407335470919));
#174824=CARTESIAN_POINT('Ctrl Pts',(15.55,-55.08000002,-139.590838222559));
#174825=CARTESIAN_POINT('Ctrl Pts',(15.55,-55.0879005396307,-139.774357162876));
#174826=CARTESIAN_POINT('Ctrl Pts',(15.55,-55.1034481519508,-139.956947178508));
#174827=CARTESIAN_POINT('Ctrl Pts',(15.55,-55.1192595423608,-140.142634984629));
#174828=CARTESIAN_POINT('Ctrl Pts',(15.55,-55.1429798052589,-140.327363292653));
#174829=CARTESIAN_POINT('Ctrl Pts',(15.55,-55.1743956555213,-140.510141133097));
#174830=CARTESIAN_POINT('Ctrl Pts',(15.55,-55.1948438531099,-140.629109022394));
#174831=CARTESIAN_POINT('Ctrl Pts',(15.55,-55.2185534084261,-140.747250607223));
#174832=CARTESIAN_POINT('Ctrl Pts',(15.55,-55.2454769784189,-140.864289524316));
#174833=CARTESIAN_POINT('Ctrl Pts',(15.55,-55.3211274089255,-141.193148010263));
#174834=CARTESIAN_POINT('Ctrl Pts',(15.55,-55.4215956233221,-141.51457580258));
#174835=CARTESIAN_POINT('Ctrl Pts',(15.55,-55.5489107707194,-141.827965375909));
#174836=CARTESIAN_POINT('Ctrl Pts',(15.55,-55.6049725527737,-141.965962922291));
#174837=CARTESIAN_POINT('Ctrl Pts',(15.55,-55.666240524004,-142.102401687741));
#174838=CARTESIAN_POINT('Ctrl Pts',(15.55,-55.7328910677637,-142.237228854888));
#174839=CARTESIAN_POINT('Origin',(15.05,-55.08000002,-139.407335470919));
#174840=CARTESIAN_POINT('Origin',(15.05,-55.08000002,-55.24995));
#174841=CARTESIAN_POINT('',(15.55,-55.08000002,-92.6513075005872));
#174842=CARTESIAN_POINT('',(15.55,-55.08000002,-139.74173251362));
#174843=CARTESIAN_POINT('Origin',(15.05,-55.08000002,-92.6513075005872));
#174844=CARTESIAN_POINT('Ctrl Pts',(15.05,-54.58000002,-92.6513075005872));
#174845=CARTESIAN_POINT('Ctrl Pts',(15.55,-54.5800000199999,-92.6513075005872));
#174846=CARTESIAN_POINT('Ctrl Pts',(15.55,-55.08000002,-92.6513075005872));
#174847=CARTESIAN_POINT('Ctrl Pts',(15.024892260188,-54.58000002,-92.1213653817264));
#174848=CARTESIAN_POINT('Ctrl Pts',(15.5499999999999,-54.5542439251598,
-92.1076806752376));
#174849=CARTESIAN_POINT('Ctrl Pts',(15.55,-55.0800000226551,-92.1594703795246));
#174850=CARTESIAN_POINT('Ctrl Pts',(14.9996997961174,-54.6413287797427,
-91.6021394176417));
#174851=CARTESIAN_POINT('Ctrl Pts',(15.5499999999983,-54.5897383680245,
-91.5814692358521));
#174852=CARTESIAN_POINT('Ctrl Pts',(15.55,-55.1351959031758,-91.676922782688));
#174853=CARTESIAN_POINT('Ctrl Pts',(14.9493011640063,-54.8817452975266,
-90.5846126995011));
#174854=CARTESIAN_POINT('Ctrl Pts',(15.5500000000017,-54.7672056222625,
-90.5350573580561));
#174855=CARTESIAN_POINT('Ctrl Pts',(15.55,-55.3515707703666,-90.7300471126767));
#174856=CARTESIAN_POINT('Ctrl Pts',(14.923904192,-55.0632253929174,-90.0827451820487));
#174857=CARTESIAN_POINT('Ctrl Pts',(15.5499999999938,-54.9184989239094,
-90.0093785901182));
#174858=CARTESIAN_POINT('Ctrl Pts',(15.55,-55.5149014993407,-90.2623845064693));
#174859=CARTESIAN_POINT('Ctrl Pts',(14.8995694550282,-55.3054345175152,
-89.6101049857472));
#174860=CARTESIAN_POINT('Ctrl Pts',(15.55,-55.121486747249,-89.5191721331851));
#174861=CARTESIAN_POINT('Ctrl Pts',(15.55,-55.7328910677637,-89.8214141166176));
#174862=CARTESIAN_POINT('',(15.55,-55.7328910677637,-89.8214141166176));
#174863=CARTESIAN_POINT('Ctrl Pts',(15.55,-55.7328910677637,-89.8214141166176));
#174864=CARTESIAN_POINT('Ctrl Pts',(15.55,-55.6023063246612,-90.0855735666696));
#174865=CARTESIAN_POINT('Ctrl Pts',(15.55,-55.4913767816605,-90.3592181628643));
#174866=CARTESIAN_POINT('Ctrl Pts',(15.55,-55.4001499318864,-90.6379301891953));
#174867=CARTESIAN_POINT('Ctrl Pts',(15.55,-55.3390449811745,-90.8246151911869));
#174868=CARTESIAN_POINT('Ctrl Pts',(15.55,-55.2867806294651,-91.0135745317669));
#174869=CARTESIAN_POINT('Ctrl Pts',(15.55,-55.2433833364682,-91.2034849476131));
#174870=CARTESIAN_POINT('Ctrl Pts',(15.55,-55.1636960311289,-91.5522036867227));
#174871=CARTESIAN_POINT('Ctrl Pts',(15.55,-55.1127619110557,-91.9058298381009));
#174872=CARTESIAN_POINT('Ctrl Pts',(15.55,-55.0914526404123,-92.2645121879628));
#174873=CARTESIAN_POINT('Ctrl Pts',(15.55,-55.0838313896102,-92.3927947647028));
#174874=CARTESIAN_POINT('Ctrl Pts',(15.55,-55.08000002,-92.5217241762766));
#174875=CARTESIAN_POINT('Ctrl Pts',(15.55,-55.08000002,-92.6513075005872));
#174876=CARTESIAN_POINT('',(14.8995695466442,-55.3054345064313,-89.6101050856063));
#174877=CARTESIAN_POINT('Origin',(15.05,-55.7328910677637,-89.8214141166176));
#174878=CARTESIAN_POINT('Ctrl Pts',(15.05,-54.5800000213444,-92.6513075005872));
#174879=CARTESIAN_POINT('Ctrl Pts',(15.0458933768937,-54.5800017521292,
-92.5646301382912));
#174880=CARTESIAN_POINT('Ctrl Pts',(15.0416395067651,-54.5816724036173,
-92.4748619271837));
#174881=CARTESIAN_POINT('Ctrl Pts',(15.0372157372707,-54.5853737320494,
-92.3820625728329));
#174882=CARTESIAN_POINT('Ctrl Pts',(15.0355328910543,-54.5867817544511,
-92.3467607691209));
#174883=CARTESIAN_POINT('Ctrl Pts',(15.0338256891318,-54.5884839168519,
-92.3110207073987));
#174884=CARTESIAN_POINT('Ctrl Pts',(15.0320938066638,-54.5905011024224,
-92.2748471742631));
#174885=CARTESIAN_POINT('Ctrl Pts',(15.0289515288417,-54.594161026002,-92.2092149543954));
#174886=CARTESIAN_POINT('Ctrl Pts',(15.0257275985235,-54.5988577289582,
-92.1421551536645));
#174887=CARTESIAN_POINT('Ctrl Pts',(15.0224251368449,-54.6047198056994,
-92.0737042390075));
#174888=CARTESIAN_POINT('Ctrl Pts',(15.0207739060056,-54.6076508440699,
-92.0394787816791));
#174889=CARTESIAN_POINT('Ctrl Pts',(15.0191030478259,-54.6108733196573,
-92.004905554086));
#174890=CARTESIAN_POINT('Ctrl Pts',(15.0174137469137,-54.614403682952,-91.9699903181173));
#174891=CARTESIAN_POINT('Ctrl Pts',(15.0165690964576,-54.6161688645993,
-91.952532700133));
#174892=CARTESIAN_POINT('Ctrl Pts',(15.0157198355364,-54.6180110230736,
-91.9349895803821));
#174893=CARTESIAN_POINT('Ctrl Pts',(15.0148661413604,-54.6199322383161,
-91.9173617205731));
#174894=CARTESIAN_POINT('Ctrl Pts',(15.0144392942724,-54.6208928459373,
-91.9085477906686));
#174895=CARTESIAN_POINT('Ctrl Pts',(15.0140113388933,-54.6218732180572,
-91.8997126757832));
#174896=CARTESIAN_POINT('Ctrl Pts',(15.0135823003155,-54.6228736158331,
-91.8908564754731));
#174897=CARTESIAN_POINT('Ctrl Pts',(15.0133677810267,-54.623373814721,-91.8864283753181));
#174898=CARTESIAN_POINT('Ctrl Pts',(15.0131529909395,-54.6238790200414,
-91.881995003809));
#174899=CARTESIAN_POINT('Ctrl Pts',(15.0129379333912,-54.6243892645035,
-91.877556373683));
#174900=CARTESIAN_POINT('Ctrl Pts',(15.0127228758429,-54.6248995089657,
-91.8731177435571));
#174901=CARTESIAN_POINT('Ctrl Pts',(15.0124491667809,-54.6255557109238,
-91.8674689771974));
#174902=CARTESIAN_POINT('Ctrl Pts',(15.0122919617645,-54.6259351480827,
-91.8642247202862));
#174903=CARTESIAN_POINT('Ctrl Pts',(15.0095085000646,-54.6326534375083,
-91.8067821203983));
#174904=CARTESIAN_POINT('Ctrl Pts',(15.0065479524336,-54.640561215979,-91.7454833205905));
#174905=CARTESIAN_POINT('Ctrl Pts',(15.0033879091281,-54.6499830230815,
-91.6803729622894));
#174906=CARTESIAN_POINT('Ctrl Pts',(15.0003178326951,-54.6591365900248,
-91.6171163049481));
#174907=CARTESIAN_POINT('Ctrl Pts',(14.9970591152687,-54.6697195336152,
-91.5502616453185));
#174908=CARTESIAN_POINT('Ctrl Pts',(14.9936054921246,-54.6820664342457,
-91.4798778723979));
#174909=CARTESIAN_POINT('Ctrl Pts',(14.9909769599697,-54.6914635873127,
-91.426309198983));
#174910=CARTESIAN_POINT('Ctrl Pts',(14.988235755913,-54.701883324779,-91.3706967310606));
#174911=CARTESIAN_POINT('Ctrl Pts',(14.9853868715498,-54.713486216082,-91.3130843738657));
#174912=CARTESIAN_POINT('Ctrl Pts',(14.9836460612115,-54.7205761609719,
-91.2778803521415));
#174913=CARTESIAN_POINT('Ctrl Pts',(14.9818651855333,-54.7281080902031,
-91.2419298484048));
#174914=CARTESIAN_POINT('Ctrl Pts',(14.9800469402429,-54.7361204910152,
-91.2052454222553));
#174915=CARTESIAN_POINT('Ctrl Pts',(14.9791378175977,-54.7401266914212,
-91.1869032091805));
#174916=CARTESIAN_POINT('Ctrl Pts',(14.978219356738,-54.7442530383326,-91.1683775216247));
#174917=CARTESIAN_POINT('Ctrl Pts',(14.9772920391227,-54.7485044521196,
-91.1496701581355));
#174918=CARTESIAN_POINT('Ctrl Pts',(14.976828380315,-54.7506301590131,-91.1403164763909));
#174919=CARTESIAN_POINT('Ctrl Pts',(14.9763625075567,-54.7527871343342,
-91.1309173760119));
#174920=CARTESIAN_POINT('Ctrl Pts',(14.9758944868423,-54.7549760012729,
-91.1214730904895));
#174921=CARTESIAN_POINT('Ctrl Pts',(14.9756604764851,-54.7560704347422,
-91.1167509477282));
#174922=CARTESIAN_POINT('Ctrl Pts',(14.9754259291553,-54.7571728412223,
-91.1120175087052));
#174923=CARTESIAN_POINT('Ctrl Pts',(14.9751908536412,-54.7582832990244,
-91.1072728034403));
#174924=CARTESIAN_POINT('Ctrl Pts',(14.9750733158841,-54.7588385279254,
-91.1049004508078));
#174925=CARTESIAN_POINT('Ctrl Pts',(14.974955646082,-54.7593957696634,-91.1025252816164));
#174926=CARTESIAN_POINT('Ctrl Pts',(14.9748378453696,-54.7599550340516,
-91.1001472996742));
#174927=CARTESIAN_POINT('Ctrl Pts',(14.9747200446573,-54.7605142984398,
-91.097769317732));
#174928=CARTESIAN_POINT('Ctrl Pts',(14.9746589234672,-54.7608045194713,
-91.0965354989367));
#174929=CARTESIAN_POINT('Ctrl Pts',(14.9744840516501,-54.761638905001,-91.0930049194237));
#174930=CARTESIAN_POINT('Ctrl Pts',(14.9712879276385,-54.7768889302514,
-91.0284766830101));
#174931=CARTESIAN_POINT('Ctrl Pts',(14.9682575247718,-54.7921574606343,
-90.9681333553976));
#174932=CARTESIAN_POINT('Ctrl Pts',(14.9654248623909,-54.8071025510312,
-90.9119403256999));
#174933=CARTESIAN_POINT('Ctrl Pts',(14.962559488986,-54.8222202243711,-90.855098390028));
#174934=CARTESIAN_POINT('Ctrl Pts',(14.9598960678549,-54.8370067435763,
-90.8025026027613));
#174935=CARTESIAN_POINT('Ctrl Pts',(14.957449120201,-54.8511563261295,-90.754103022306));
#174936=CARTESIAN_POINT('Ctrl Pts',(14.9549597206588,-54.8655513885955,
-90.7048637616166));
#174937=CARTESIAN_POINT('Ctrl Pts',(14.9526940092514,-54.8792870587007,
-90.6599670468528));
#174938=CARTESIAN_POINT('Ctrl Pts',(14.9506537885868,-54.8920937467772,
-90.619354020203));
#174939=CARTESIAN_POINT('Ctrl Pts',(14.94861546294,-54.9048885396201,-90.5787787161429));
#174940=CARTESIAN_POINT('Ctrl Pts',(14.9468018624224,-54.9167561342402,
-90.542478692155));
#174941=CARTESIAN_POINT('Ctrl Pts',(14.9452068624669,-54.9274800524862,
-90.5103964667988));
#174942=CARTESIAN_POINT('Ctrl Pts',(14.9436064679013,-54.9382402411767,
-90.4782057329156));
#174943=CARTESIAN_POINT('Ctrl Pts',(14.9422258779312,-54.9478490573687,
-90.4502610146561));
#174944=CARTESIAN_POINT('Ctrl Pts',(14.9410556150303,-54.9561397422719,
-90.4265116055838));
#174945=CARTESIAN_POINT('Ctrl Pts',(14.9398899886193,-54.9643975801323,
-90.4028562898062));
#174946=CARTESIAN_POINT('Ctrl Pts',(14.9389328214154,-54.9713478278598,
-90.3833628560987));
#174947=CARTESIAN_POINT('Ctrl Pts',(14.9381751005125,-54.9768757304564,
-90.3679930506267));
#174948=CARTESIAN_POINT('Ctrl Pts',(14.937852325165,-54.9792305165991,-90.3614457925467));
#174949=CARTESIAN_POINT('Ctrl Pts',(14.9375657634153,-54.9813278138561,
-90.3556469787911));
#174950=CARTESIAN_POINT('Ctrl Pts',(14.9373148566348,-54.9831614508253,
-90.3505944556927));
#174951=CARTESIAN_POINT('Ctrl Pts',(14.9371894032445,-54.9840782693099,
-90.3480681941436));
#174952=CARTESIAN_POINT('Ctrl Pts',(14.9370728694485,-54.9849291965647,
-90.3457285136322));
#174953=CARTESIAN_POINT('Ctrl Pts',(14.936965191492,-54.9857136121027,-90.3435751934635));
#174954=CARTESIAN_POINT('Ctrl Pts',(14.9369113525138,-54.9861058198717,
-90.3424985333791));
#174955=CARTESIAN_POINT('Ctrl Pts',(14.9368597278605,-54.9864814012052,
-90.341468463903));
#174956=CARTESIAN_POINT('Ctrl Pts',(14.9368103110741,-54.9868402876361,
-90.3404849606904));
#174957=CARTESIAN_POINT('Ctrl Pts',(14.9367856026809,-54.9870197308516,
-90.3399932090841));
#174958=CARTESIAN_POINT('Ctrl Pts',(14.9367614463196,-54.9871950008638,
-90.3395130992309));
#174959=CARTESIAN_POINT('Ctrl Pts',(14.9367381141154,-54.9873639714566,
-90.3390504377747));
#174960=CARTESIAN_POINT('Ctrl Pts',(14.9367147819112,-54.9875329420495,
-90.3385877763185));
#174961=CARTESIAN_POINT('Ctrl Pts',(14.936691690197,-54.9876994699089,-90.3381308072005));
#174962=CARTESIAN_POINT('Ctrl Pts',(14.9365793719496,-54.9885126937962,
-90.3359077490858));
#174963=CARTESIAN_POINT('Ctrl Pts',(14.932320345283,-55.0193495551381,-90.2516109940237));
#174964=CARTESIAN_POINT('Ctrl Pts',(14.9282177537613,-55.0507709943322,
-90.1710764495536));
#174965=CARTESIAN_POINT('Ctrl Pts',(14.9243031313811,-55.0823649839917,
-90.0942965928955));
#174966=CARTESIAN_POINT('Ctrl Pts',(14.9203172922909,-55.114533746843,-90.0161199198253));
#174967=CARTESIAN_POINT('Ctrl Pts',(14.9165260129442,-55.1468809599686,
-89.9418352830905));
#174968=CARTESIAN_POINT('Ctrl Pts',(14.9129329981448,-55.1790051991007,
-89.8714032691796));
#174969=CARTESIAN_POINT('Ctrl Pts',(14.9092446511795,-55.2119817790847,
-89.7991025080434));
#174970=CARTESIAN_POINT('Ctrl Pts',(14.9057648845781,-55.2447230132529,
-89.7308609781904));
#174971=CARTESIAN_POINT('Ctrl Pts',(14.9024718238562,-55.2768360660964,
-89.6666112571839));
#174972=CARTESIAN_POINT('Ctrl Pts',(14.9014882245471,-55.2864278651114,
-89.6474206055301));
#174973=CARTESIAN_POINT('Ctrl Pts',(14.9005211306358,-55.2959639152063,
-89.6285859491188));
#174974=CARTESIAN_POINT('Ctrl Pts',(14.8995696009239,-55.3054345059065,
-89.6101051906852));
#174975=CARTESIAN_POINT('Ctrl Pts',(15.55,-69.753968537624,-61.0621827299711));
#174976=CARTESIAN_POINT('Ctrl Pts',(15.55,-69.1834807533182,-60.7869757488078));
#174977=CARTESIAN_POINT('Ctrl Pts',(14.9339094669349,-69.3159372152924,
-60.8508735991008));
#174978=CARTESIAN_POINT('Ctrl Pts',(15.55,-65.1200769667078,-70.6679657074144));
#174979=CARTESIAN_POINT('Ctrl Pts',(15.5499999999812,-64.4850428243905,
-70.4989618700373));
#174980=CARTESIAN_POINT('Ctrl Pts',(14.9250579803326,-64.6843968356381,
-70.4566455899725));
#174981=CARTESIAN_POINT('Ctrl Pts',(15.55,-60.4591562379615,-80.2606677496439));
#174982=CARTESIAN_POINT('Ctrl Pts',(15.5500000001812,-59.7682625842489,
-80.1682572157014));
#174983=CARTESIAN_POINT('Ctrl Pts',(14.9143624117001,-60.0265024281888,
-80.0493410623047));
#174984=CARTESIAN_POINT('Ctrl Pts',(15.55,-55.7328910677637,-89.8214141166175));
#174985=CARTESIAN_POINT('Ctrl Pts',(15.55,-55.1214867472491,-89.519172133185));
#174986=CARTESIAN_POINT('Ctrl Pts',(14.8995694550282,-55.3054345175152,
-89.6101049857472));
#174987=CARTESIAN_POINT('',(15.55,-69.7539685376239,-61.0621827299711));
#174988=CARTESIAN_POINT('Ctrl Pts',(15.55,-69.7539685376239,-61.0621827299711));
#174989=CARTESIAN_POINT('Ctrl Pts',(15.55,-65.1200645664474,-70.6679914124205));
#174990=CARTESIAN_POINT('Ctrl Pts',(15.55,-60.459169452046,-80.2606410189155));
#174991=CARTESIAN_POINT('Ctrl Pts',(15.55,-55.7328910677637,-89.8214141166175));
#174992=CARTESIAN_POINT('',(14.9339094669349,-69.3159372152925,-60.8508735991008));
#174993=CARTESIAN_POINT('Origin',(15.05,-69.753968537624,-61.0621827299711));
#174994=CARTESIAN_POINT('Ctrl Pts',(14.8995694550282,-55.3054345175152,
-89.6101049857472));
#174995=CARTESIAN_POINT('Ctrl Pts',(14.9021428471819,-56.126714494731,-87.9469084112056));
#174996=CARTESIAN_POINT('Ctrl Pts',(14.9048838536198,-56.9717170086061,
-86.2306729016001));
#174997=CARTESIAN_POINT('Ctrl Pts',(14.9076126716805,-57.8403614223101,
-84.4613461791733));
#174998=CARTESIAN_POINT('Ctrl Pts',(14.9101550205963,-58.6496484961364,
-82.8129233916143));
#174999=CARTESIAN_POINT('Ctrl Pts',(14.9126867965068,-59.4794565058462,
-81.1184174199939));
#175000=CARTESIAN_POINT('Ctrl Pts',(14.9150655785119,-60.329761996796,-79.3778019676598));
#175001=CARTESIAN_POINT('Ctrl Pts',(14.9164835292938,-60.8366143830631,
-78.3402512226876));
#175002=CARTESIAN_POINT('Ctrl Pts',(14.917847170542,-61.3507506625969,-77.2863173579256));
#175003=CARTESIAN_POINT('Ctrl Pts',(14.9191269994737,-61.8721739455428,
-76.2159986380771));
#175004=CARTESIAN_POINT('Ctrl Pts',(14.9210339184465,-62.6490839890544,
-74.6212456026722));
#175005=CARTESIAN_POINT('Ctrl Pts',(14.9227536565489,-63.4421679559353,
-72.9901189526708));
#175006=CARTESIAN_POINT('Ctrl Pts',(14.9243835901195,-64.2514169346386,
-71.3226182784319));
#175007=CARTESIAN_POINT('Ctrl Pts',(14.9260180885611,-65.0629323353103,
-69.6504475208691));
#175008=CARTESIAN_POINT('Ctrl Pts',(14.9275622911326,-65.8907028888218,
-67.9416989707886));
#175009=CARTESIAN_POINT('Ctrl Pts',(14.9291162534416,-66.7347676310078,
-66.1963964579937));
#175010=CARTESIAN_POINT('Ctrl Pts',(14.9306702157506,-67.5788323731938,
-64.4510939451989));
#175011=CARTESIAN_POINT('Ctrl Pts',(14.9322338889336,-68.4391910232791,
-62.6692371075657));
#175012=CARTESIAN_POINT('Ctrl Pts',(14.9339094669349,-69.3159372152924,
-60.8508735991008));
#175013=CARTESIAN_POINT('Ctrl Pts',(16.4431419066885,-54.58000002,-91.6952124319348));
#175014=CARTESIAN_POINT('Ctrl Pts',(15.6303319911964,-54.58000002,-90.5558876551412));
#175015=CARTESIAN_POINT('Ctrl Pts',(14.9356335973474,-55.3065630170304,
-89.5821211232313));
#175016=CARTESIAN_POINT('Ctrl Pts',(15.339723951503,-54.58000002,-92.4824059293848));
#175017=CARTESIAN_POINT('Ctrl Pts',(14.580009345269,-54.5800000199812,-91.3456221401381));
#175018=CARTESIAN_POINT('Ctrl Pts',(13.9221964884044,-55.2748268726715,
-90.3693030445756));
#175019=CARTESIAN_POINT('Ctrl Pts',(14.2000751633255,-54.58000002,-93.2257513219804));
#175020=CARTESIAN_POINT('Ctrl Pts',(13.4941774039103,-54.58000002,-92.0929943757894));
#175021=CARTESIAN_POINT('Ctrl Pts',(12.878461314285,-55.2441424314898,-91.1126600131971));
#175022=CARTESIAN_POINT('Ctrl Pts',(11.824167023199,-54.58000002,-94.5957116711942));
#175023=CARTESIAN_POINT('Ctrl Pts',(11.232462400793,-54.58000002,-93.4698992380895));
#175024=CARTESIAN_POINT('Ctrl Pts',(10.7089431339248,-55.1865276043544,
-92.4826203625704));
#175025=CARTESIAN_POINT('Ctrl Pts',(10.607529289827,-54.58000002,-95.2106503240539));
#175026=CARTESIAN_POINT('Ctrl Pts',(10.0749231938442,-54.5800000200141,
-94.0883976981553));
#175027=CARTESIAN_POINT('Ctrl Pts',(9.60108129664725,-55.1600911541447,
-93.0975581705506));
#175028=CARTESIAN_POINT('Ctrl Pts',(9.35547542469517,-54.58000002,-95.7390202399778));
#175029=CARTESIAN_POINT('Ctrl Pts',(8.88330761013172,-54.58000002,-94.6201459052405));
#175030=CARTESIAN_POINT('Ctrl Pts',(8.4637455188182,-55.1370659786207,-93.6259289312743));
#175031=CARTESIAN_POINT('',(9.30242220787995,-55.1547652726018,-93.2181494891395));
#175032=CARTESIAN_POINT('Ctrl Pts',(9.30244148822568,-55.1547632761147,
-93.2181873809143));
#175033=CARTESIAN_POINT('Ctrl Pts',(9.61839909982102,-55.1616974672035,
-93.0577850773918));
#175034=CARTESIAN_POINT('Ctrl Pts',(9.93432541699597,-55.1689288990669,
-92.8897556011866));
#175035=CARTESIAN_POINT('Ctrl Pts',(10.2507660919963,-55.1764563648516,
-92.7139149924441));
#175036=CARTESIAN_POINT('Ctrl Pts',(10.5909200390141,-55.1845479200782,
-92.5248973286759));
#175037=CARTESIAN_POINT('Ctrl Pts',(10.9316681646333,-55.1929815934896,
-92.3268537703324));
#175038=CARTESIAN_POINT('Ctrl Pts',(11.2736708069581,-55.2017567532371,
-92.1194964152936));
#175039=CARTESIAN_POINT('Ctrl Pts',(11.4466658104287,-55.2061954873377,
-92.0146089614693));
#175040=CARTESIAN_POINT('Ctrl Pts',(11.6199815475503,-55.2107216033676,
-91.9073375579729));
#175041=CARTESIAN_POINT('Ctrl Pts',(11.7937022241049,-55.2153350179221,
-91.7976401878838));
#175042=CARTESIAN_POINT('Ctrl Pts',(12.2295670546593,-55.2269100658263,
-91.5224097053964));
#175043=CARTESIAN_POINT('Ctrl Pts',(12.6650898659555,-55.2389551468803,
-91.2337939943317));
#175044=CARTESIAN_POINT('Ctrl Pts',(13.1016107174846,-55.2514743713384,
-90.9311140181789));
#175045=CARTESIAN_POINT('Ctrl Pts',(13.5853543625944,-55.2653479245766,
-90.5956901444901));
#175046=CARTESIAN_POINT('Ctrl Pts',(14.0703195878936,-55.2798042384788,
-90.242989300559));
#175047=CARTESIAN_POINT('Ctrl Pts',(14.5583239929663,-55.294841368818,-89.8720620734263));
#175048=CARTESIAN_POINT('Ctrl Pts',(14.6718999929854,-55.2983410444314,
-89.7857341011416));
#175049=CARTESIAN_POINT('Ctrl Pts',(14.7856407595719,-55.301872131609,-89.6984190004166));
#175050=CARTESIAN_POINT('Ctrl Pts',(14.8995696009239,-55.3054345059065,
-89.6101051906852));
#175051=CARTESIAN_POINT('Ctrl Pts',(9.30244004339758,-55.1547632444057,
-93.2181881144106));
#175052=CARTESIAN_POINT('Ctrl Pts',(9.30427433941287,-55.1332939358577,
-93.2623011656816));
#175053=CARTESIAN_POINT('Ctrl Pts',(9.30624352124608,-55.1107681190608,
-93.3100497844399));
#175054=CARTESIAN_POINT('Ctrl Pts',(9.30836251838502,-55.0874709846995,
-93.3615546812591));
#175055=CARTESIAN_POINT('Ctrl Pts',(9.30992763140037,-55.0702634823677,
-93.3995967261891));
#175056=CARTESIAN_POINT('Ctrl Pts',(9.31157437985831,-55.0526361927093,
-93.439688104872));
#175057=CARTESIAN_POINT('Ctrl Pts',(9.31330526457061,-55.0347219445586,
-93.481875686768));
#175058=CARTESIAN_POINT('Ctrl Pts',(9.31534242415013,-55.0136378238366,
-93.5315282349621));
#175059=CARTESIAN_POINT('Ctrl Pts',(9.3174964869314,-54.9921554559608,-93.5840849551193));
#175060=CARTESIAN_POINT('Ctrl Pts',(9.31976404326403,-54.9705191678377,
-93.6396151789178));
#175061=CARTESIAN_POINT('Ctrl Pts',(9.32089782143035,-54.9597010237762,
-93.6673802908171));
#175062=CARTESIAN_POINT('Ctrl Pts',(9.32205983145287,-54.9488448734871,
-93.6958886290157));
#175063=CARTESIAN_POINT('Ctrl Pts',(9.3232486734891,-54.9379841011688,-93.7251477030176));
#175064=CARTESIAN_POINT('Ctrl Pts',(9.32384309450721,-54.9325537150096,
-93.7397772400185));
#175065=CARTESIAN_POINT('Ctrl Pts',(9.32444422673949,-54.9271221929293,
-93.754594468051));
#175066=CARTESIAN_POINT('Ctrl Pts',(9.32505180826187,-54.9216938962469,
-93.7696002084956));
#175067=CARTESIAN_POINT('Ctrl Pts',(9.32535559902306,-54.9189797479057,
-93.777103078718));
#175068=CARTESIAN_POINT('Ctrl Pts',(9.32566100229853,-54.9162664070469,
-93.7846530774654));
#175069=CARTESIAN_POINT('Ctrl Pts',(9.32596798310117,-54.9135544280597,
-93.7922503045262));
#175070=CARTESIAN_POINT('Ctrl Pts',(9.32612147350249,-54.9121984385661,
-93.7960489180566));
#175071=CARTESIAN_POINT('Ctrl Pts',(9.3262753582968,-54.9108427896114,-93.7998593386901));
#175072=CARTESIAN_POINT('Ctrl Pts',(9.32642963280402,-54.9094875511762,
-93.8036815784753));
#175073=CARTESIAN_POINT('Ctrl Pts',(9.32650677005764,-54.9088099319586,
-93.8055926983679));
#175074=CARTESIAN_POINT('Ctrl Pts',(9.32658400474017,-54.9081324153753,
-93.80750677305));
#175075=CARTESIAN_POINT('Ctrl Pts',(9.32666133624566,-54.9074550102173,
-93.809423803998));
#175076=CARTESIAN_POINT('Ctrl Pts',(9.32673866775115,-54.9067776050594,
-93.8113408349459));
#175077=CARTESIAN_POINT('Ctrl Pts',(9.32677113000359,-54.9064930880799,
-93.8121454682918));
#175078=CARTESIAN_POINT('Ctrl Pts',(9.32689362062015,-54.9054231378333,
-93.8151837671098));
#175079=CARTESIAN_POINT('Ctrl Pts',(9.32907568700704,-54.8863628821635,
-93.8693084822138));
#175080=CARTESIAN_POINT('Ctrl Pts',(9.33113370306065,-54.8693839288859,
-93.9201129178801));
#175081=CARTESIAN_POINT('Ctrl Pts',(9.3330474098387,-54.8541913521633,-93.9674628293226));
#175082=CARTESIAN_POINT('Ctrl Pts',(9.33498196023909,-54.8388333016414,
-94.0153284643247));
#175083=CARTESIAN_POINT('Ctrl Pts',(9.33676931245704,-54.8253003429326,
-94.0596643643792));
#175084=CARTESIAN_POINT('Ctrl Pts',(9.33840041440837,-54.8133245098168,
-94.1003684347088));
#175085=CARTESIAN_POINT('Ctrl Pts',(9.34004917218116,-54.8012190446009,
-94.1415131052091));
#175086=CARTESIAN_POINT('Ctrl Pts',(9.34153852943323,-54.7907042806318,
-94.1789473298604));
#175087=CARTESIAN_POINT('Ctrl Pts',(9.34286722215193,-54.7815462682086,
-94.2125960809697));
#175088=CARTESIAN_POINT('Ctrl Pts',(9.34420075570395,-54.7723548903496,
-94.2463674247548));
#175089=CARTESIAN_POINT('Ctrl Pts',(9.34537267165175,-54.7645299865231,
-94.2763260722162));
#175090=CARTESIAN_POINT('Ctrl Pts',(9.34638621535443,-54.7578816051877,
-94.3024201830284));
#175091=CARTESIAN_POINT('Ctrl Pts',(9.34740282266097,-54.7512131280176,
-94.3285931676167));
#175092=CARTESIAN_POINT('Ctrl Pts',(9.34826027114869,-54.745728182414,-94.3508785485639));
#175093=CARTESIAN_POINT('Ctrl Pts',(9.34896342191889,-54.7412840483787,
-94.3692425251512));
#175094=CARTESIAN_POINT('Ctrl Pts',(9.34916988110587,-54.7399791613777,
-94.3746345574672));
#175095=CARTESIAN_POINT('Ctrl Pts',(9.34936303935837,-54.738764331903,-94.3796886188088));
#175096=CARTESIAN_POINT('Ctrl Pts',(9.3495430157132,-54.7376367641466,-94.3844040976793));
#175097=CARTESIAN_POINT('Ctrl Pts',(9.35007821311692,-54.7342837051501,
-94.3984265621923));
#175098=CARTESIAN_POINT('Ctrl Pts',(9.35049691873413,-54.7317001298129,
-94.4094544485823));
#175099=CARTESIAN_POINT('Ctrl Pts',(9.35080171450003,-54.729832066066,-94.417476557166));
#175100=CARTESIAN_POINT('Ctrl Pts',(9.35095411238298,-54.7288980341925,
-94.4214876114579));
#175101=CARTESIAN_POINT('Ctrl Pts',(9.35107801732042,-54.7281433382731,
-94.4247473300645));
#175102=CARTESIAN_POINT('Ctrl Pts',(9.35117363515788,-54.7275639869044,
-94.4272549215081));
#175103=CARTESIAN_POINT('Ctrl Pts',(9.35122144407661,-54.7272743112201,
-94.4285087172299));
#175104=CARTESIAN_POINT('Ctrl Pts',(9.35126218405767,-54.727028499904,-94.429574487568));
#175105=CARTESIAN_POINT('Ctrl Pts',(9.35129586718252,-54.7268262272475,
-94.4304521681997));
#175106=CARTESIAN_POINT('Ctrl Pts',(9.35131270874495,-54.7267250909192,
-94.4308910085156));
#175107=CARTESIAN_POINT('Ctrl Pts',(9.35132778627098,-54.7266348410177,
-94.431282826806));
#175108=CARTESIAN_POINT('Ctrl Pts',(9.3513411014339,-54.7265554475381,-94.4316276172239));
#175109=CARTESIAN_POINT('Ctrl Pts',(9.35134775901537,-54.7265157507983,
-94.4318000124328));
#175110=CARTESIAN_POINT('Ctrl Pts',(9.35135397600869,-54.7264787684293,
-94.4319606507287));
#175111=CARTESIAN_POINT('Ctrl Pts',(9.35135953256314,-54.7264458494721,
-94.4321036520747));
#175112=CARTESIAN_POINT('Ctrl Pts',(9.35136508911759,-54.726412930515,-94.4322466534208));
#175113=CARTESIAN_POINT('Ctrl Pts',(9.35137044371634,-54.7263810282556,
-94.4323837104159));
#175114=CARTESIAN_POINT('Ctrl Pts',(9.35144642391555,-54.7259337110089,
-94.4343302656795));
#175115=CARTESIAN_POINT('Ctrl Pts',(9.35496709525164,-54.7052065080629,
-94.5245272037296));
#175116=CARTESIAN_POINT('Ctrl Pts',(9.35842399639266,-54.6872251950304,
-94.6127481737394));
#175117=CARTESIAN_POINT('Ctrl Pts',(9.36177567320373,-54.671666092566,-94.6987859198705));
#175118=CARTESIAN_POINT('Ctrl Pts',(9.3652001974941,-54.6557688186553,-94.7866936651941));
#175119=CARTESIAN_POINT('Ctrl Pts',(9.36851502920089,-54.6423995879464,
-94.8723223801593));
#175120=CARTESIAN_POINT('Ctrl Pts',(9.37169866947417,-54.6312146453525,
-94.955500484486));
#175121=CARTESIAN_POINT('Ctrl Pts',(9.37499207965511,-54.619644052996,-95.0415465173622));
#175122=CARTESIAN_POINT('Ctrl Pts',(9.37814525879686,-54.6104103700865,
-95.1249701790108));
#175123=CARTESIAN_POINT('Ctrl Pts',(9.38115604701931,-54.6031440314951,
-95.2056319574495));
#175124=CARTESIAN_POINT('Ctrl Pts',(9.38422794052159,-54.5957302193453,
-95.2879308023903));
#175125=CARTESIAN_POINT('Ctrl Pts',(9.38715185380867,-54.5903639102433,
-95.3673548787892));
#175126=CARTESIAN_POINT('Ctrl Pts',(9.38994437245913,-54.5866723986661,
-95.4438035593695));
#175127=CARTESIAN_POINT('Ctrl Pts',(9.39281977434526,-54.5828713213305,
-95.5225212718889));
#175128=CARTESIAN_POINT('Ctrl Pts',(9.39555612076478,-54.58084546469,-95.5980847279305));
#175129=CARTESIAN_POINT('Ctrl Pts',(9.39818746661894,-54.5802163907876,
-95.6704283316989));
#175130=CARTESIAN_POINT('Ctrl Pts',(9.39879705050409,-54.5800706580201,
-95.6871876242796));
#175131=CARTESIAN_POINT('Ctrl Pts',(9.39940105561197,-54.5800000205198,
-95.7037742834776));
#175132=CARTESIAN_POINT('Ctrl Pts',(9.4,-54.58000002,-95.7201877838351));
#175133=CARTESIAN_POINT('Ctrl Pts',(9.30242220787995,-55.1547652726018,
-93.2181494891395));
#175134=CARTESIAN_POINT('Ctrl Pts',(8.89999999999997,-55.2270244231188,
-93.2526539147005));
#175135=CARTESIAN_POINT('Ctrl Pts',(8.9,-55.5972887473416,-93.4294586200098));
#175136=CARTESIAN_POINT('Ctrl Pts',(9.31868748160984,-54.9644104418147,
-93.609279542603));
#175137=CARTESIAN_POINT('Ctrl Pts',(8.90000000000102,-55.0269773455407,
-93.6389456903403));
#175138=CARTESIAN_POINT('Ctrl Pts',(8.9,-55.4259676862915,-93.7882391070165));
#175139=CARTESIAN_POINT('Ctrl Pts',(9.33504644279423,-54.8225599750811,
-94.0144115846847));
#175140=CARTESIAN_POINT('Ctrl Pts',(8.90000000000064,-54.8762991189121,
-94.036294307786));
#175141=CARTESIAN_POINT('Ctrl Pts',(8.9,-55.2983039792949,-94.15951472994));
#175142=CARTESIAN_POINT('Ctrl Pts',(9.36771205478627,-54.6300877991462,
-94.8508246266895));
#175143=CARTESIAN_POINT('Ctrl Pts',(8.89999999999928,-54.6591463230926,
-94.8606734038326));
#175144=CARTESIAN_POINT('Ctrl Pts',(8.9,-55.1250790215096,-94.9253056568412));
#175145=CARTESIAN_POINT('Ctrl Pts',(9.38412882836456,-54.58000002,-95.28525344501));
#175146=CARTESIAN_POINT('Ctrl Pts',(8.89999999999998,-54.5956237519515,
-95.2920343273126));
#175147=CARTESIAN_POINT('Ctrl Pts',(8.9,-55.0800000205144,-95.3226944715878));
#175148=CARTESIAN_POINT('Ctrl Pts',(9.4,-54.58000002,-95.7201877838351));
#175149=CARTESIAN_POINT('Ctrl Pts',(8.89999999999996,-54.58000002,-95.720187783835));
#175150=CARTESIAN_POINT('Ctrl Pts',(8.9,-55.08000002,-95.7201877838351));
#175151=CARTESIAN_POINT('',(8.9,-55.08000002,-95.7201877838351));
#175152=CARTESIAN_POINT('Origin',(9.4,-55.08000002,-95.7201877838351));
#175153=CARTESIAN_POINT('',(8.9,-55.5972887473416,-93.4294586200098));
#175154=CARTESIAN_POINT('Origin',(9.4,-55.5972887473416,-93.4294586200098));
#175155=CARTESIAN_POINT('Ctrl Pts',(8.9,-55.08000002,-95.7201877838351));
#175156=CARTESIAN_POINT('Ctrl Pts',(8.9,-55.08000002,-95.3987883664614));
#175157=CARTESIAN_POINT('Ctrl Pts',(8.9,-55.1094672114476,-95.0775170947052));
#175158=CARTESIAN_POINT('Ctrl Pts',(8.9,-55.1665218943283,-94.7639046607854));
#175159=CARTESIAN_POINT('Ctrl Pts',(8.9,-55.1800381380326,-94.6896099338406));
#175160=CARTESIAN_POINT('Ctrl Pts',(8.9,-55.1951028648123,-94.6157450445103));
#175161=CARTESIAN_POINT('Ctrl Pts',(8.9,-55.2116915002618,-94.5424101933588));
#175162=CARTESIAN_POINT('Ctrl Pts',(8.9,-55.2822535699003,-94.2304701974735));
#175163=CARTESIAN_POINT('Ctrl Pts',(8.9,-55.3800515517671,-93.9262693258917));
#175164=CARTESIAN_POINT('Ctrl Pts',(8.9,-55.5065195348801,-93.6302150670226));
#175165=CARTESIAN_POINT('Ctrl Pts',(8.9,-55.5352865894012,-93.5628730505181));
#175166=CARTESIAN_POINT('Ctrl Pts',(8.9,-55.5655372445695,-93.4959526010179));
#175167=CARTESIAN_POINT('Ctrl Pts',(8.9,-55.5972887473416,-93.4294586200098));
#175168=CARTESIAN_POINT('Origin',(9.4,-55.08000002,-55.24995));
#175169=CARTESIAN_POINT('',(8.9,-55.08000002,-136.338455187671));
#175170=CARTESIAN_POINT('Origin',(9.4,-55.08000002,-136.338455187671));
#175171=CARTESIAN_POINT('',(8.9,-55.08000002,-95.926725859984));
#175172=CARTESIAN_POINT('Ctrl Pts',(9.4,-54.58000002,-136.338455187671));
#175173=CARTESIAN_POINT('Ctrl Pts',(8.89999999999996,-54.58000002,-136.338455187671));
#175174=CARTESIAN_POINT('Ctrl Pts',(8.9,-55.08000002,-136.338455187671));
#175175=CARTESIAN_POINT('Ctrl Pts',(9.38412562712359,-54.58000002,-136.773477252872));
#175176=CARTESIAN_POINT('Ctrl Pts',(8.90000000000676,-54.5956263749734,
-136.766680459455));
#175177=CARTESIAN_POINT('Ctrl Pts',(8.9,-55.0800000228167,-136.736031631193));
#175178=CARTESIAN_POINT('Ctrl Pts',(9.36801042327471,-54.6289055341263,
-137.200007658363));
#175179=CARTESIAN_POINT('Ctrl Pts',(8.90000000000101,-54.6577176624563,
-137.1902362241));
#175180=CARTESIAN_POINT('Ctrl Pts',(8.9,-55.1240149822832,-137.126190519306));
#175181=CARTESIAN_POINT('Ctrl Pts',(9.33535293620398,-54.8201888415935,
-138.036551263121));
#175182=CARTESIAN_POINT('Ctrl Pts',(8.89999999999897,-54.8737336732754,
-138.014810226815));
#175183=CARTESIAN_POINT('Ctrl Pts',(8.9,-55.2961699598647,-137.892092266279));
#175184=CARTESIAN_POINT('Ctrl Pts',(9.31869380983081,-54.964336399011,-138.449211290729));
#175185=CARTESIAN_POINT('Ctrl Pts',(8.89999999999893,-55.0269063853653,
-138.419560264108));
#175186=CARTESIAN_POINT('Ctrl Pts',(8.9,-55.4259022184636,-138.270266767248));
#175187=CARTESIAN_POINT('Ctrl Pts',(9.30242220788036,-55.154765272597,-138.840493482357));
#175188=CARTESIAN_POINT('Ctrl Pts',(8.89999999999998,-55.2270244231137,
-138.805989056796));
#175189=CARTESIAN_POINT('Ctrl Pts',(8.9,-55.5972887473373,-138.629184351487));
#175190=CARTESIAN_POINT('',(8.9,-55.5972887473373,-138.629184351487));
#175191=CARTESIAN_POINT('Origin',(9.4,-55.5972887473373,-138.629184351487));
#175192=CARTESIAN_POINT('Ctrl Pts',(8.9,-55.5972887473373,-138.629184351487));
#175193=CARTESIAN_POINT('Ctrl Pts',(8.9,-55.4856871847872,-138.395468415773));
#175194=CARTESIAN_POINT('Ctrl Pts',(8.9,-55.3917128230548,-138.153503053547));
#175195=CARTESIAN_POINT('Ctrl Pts',(8.9,-55.3159696737911,-137.907364658634));
#175196=CARTESIAN_POINT('Ctrl Pts',(8.9,-55.2754252840371,-137.775609759164));
#175197=CARTESIAN_POINT('Ctrl Pts',(8.9,-55.2401039344703,-137.642659649433));
#175198=CARTESIAN_POINT('Ctrl Pts',(8.9,-55.2100924708571,-137.509141392841));
#175199=CARTESIAN_POINT('Ctrl Pts',(8.9,-55.1385732376582,-137.190958865905));
#175200=CARTESIAN_POINT('Ctrl Pts',(8.9,-55.0960936141186,-136.867828326609));
#175201=CARTESIAN_POINT('Ctrl Pts',(8.9,-55.0837682332358,-136.539559845945));
#175202=CARTESIAN_POINT('Ctrl Pts',(8.9,-55.0812593131245,-136.472738430779));
#175203=CARTESIAN_POINT('Ctrl Pts',(8.9,-55.08000002,-136.40570409352));
#175204=CARTESIAN_POINT('Ctrl Pts',(8.9,-55.08000002,-136.338455187671));
#175205=CARTESIAN_POINT('Ctrl Pts',(8.9,-71.0715121820529,-171.237717270032));
#175206=CARTESIAN_POINT('Ctrl Pts',(8.89999999999996,-70.6807353060531,
-171.422308714525));
#175207=CARTESIAN_POINT('Ctrl Pts',(9.3276302147955,-70.6241744288951,-171.449026400902));
#175208=CARTESIAN_POINT('Ctrl Pts',(8.9,-65.932751045448,-160.359049360718));
#175209=CARTESIAN_POINT('Ctrl Pts',(8.89999999999997,-65.5751008964372,
-160.600947379136));
#175210=CARTESIAN_POINT('Ctrl Pts',(9.32139302491482,-65.48642588992,-160.570366012028));
#175211=CARTESIAN_POINT('Ctrl Pts',(8.9,-60.7816272203214,-149.486223352848));
#175212=CARTESIAN_POINT('Ctrl Pts',(8.89999999996837,-60.4515277778623,
-149.769759336176));
#175213=CARTESIAN_POINT('Ctrl Pts',(9.31373872503275,-60.3366136221522,
-149.697543381378));
#175214=CARTESIAN_POINT('Ctrl Pts',(8.9,-55.5972887473373,-138.629184351487));
#175215=CARTESIAN_POINT('Ctrl Pts',(8.89999999999998,-55.2270244231145,
-138.805989056796));
#175216=CARTESIAN_POINT('Ctrl Pts',(9.30242220787994,-55.1547652725975,
-138.840493482357));
#175217=CARTESIAN_POINT('',(8.9,-71.0715121820529,-171.237717270032));
#175218=CARTESIAN_POINT('',(9.3276302147955,-70.6241744288951,-171.449026400902));
#175219=CARTESIAN_POINT('Origin',(9.4,-71.0715121820529,-171.237717270032));
#175220=CARTESIAN_POINT('Ctrl Pts',(9.30242220787652,-55.1547652726017,
-138.840493482365));
#175221=CARTESIAN_POINT('Ctrl Pts',(9.30502066599635,-56.3446027211807,
-141.333450373329));
#175222=CARTESIAN_POINT('Ctrl Pts',(9.30762015406821,-57.5854232432311,
-143.937974471921));
#175223=CARTESIAN_POINT('Ctrl Pts',(9.31122614649335,-59.523163084648,-148.012111431249));
#175224=CARTESIAN_POINT('Ctrl Pts',(9.31238561873438,-60.1818270656114,
-149.398048886265));
#175225=CARTESIAN_POINT('Ctrl Pts',(9.31408147943844,-61.1889472073688,
-151.518792771649));
#175226=CARTESIAN_POINT('Ctrl Pts',(9.31491917086314,-61.6972882651846,
-152.589624140057));
#175227=CARTESIAN_POINT('Ctrl Pts',(9.31588935336845,-62.2987186132309,
-153.8572313982));
#175228=CARTESIAN_POINT('Ctrl Pts',(9.3163744849145,-62.6015250786792,-154.495611026022));
#175229=CARTESIAN_POINT('Ctrl Pts',(9.31664331763924,-62.7697289037899,
-154.850266319648));
#175230=CARTESIAN_POINT('Ctrl Pts',(9.31677352444865,-62.8512928935264,
-155.0222567554));
#175231=CARTESIAN_POINT('Ctrl Pts',(9.31684300904555,-62.8948372533087,
-155.114080321108));
#175232=CARTESIAN_POINT('Ctrl Pts',(9.31685291467516,-62.90104528335,-155.127171497753));
#175233=CARTESIAN_POINT('Ctrl Pts',(9.32068386750567,-65.3020872796149,
-160.190390144699));
#175234=CARTESIAN_POINT('Ctrl Pts',(9.32429261610782,-67.874900615077,-165.627718505107));
#175235=CARTESIAN_POINT('Ctrl Pts',(9.3276302147955,-70.6241744288951,-171.449026400902));
#175236=CARTESIAN_POINT('Ctrl Pts',(8.9,-71.0715121820529,-171.237717270032));
#175237=CARTESIAN_POINT('Ctrl Pts',(8.9,-65.932751045448,-160.359049360718));
#175238=CARTESIAN_POINT('Ctrl Pts',(8.9,-60.7816272203214,-149.486223352848));
#175239=CARTESIAN_POINT('Ctrl Pts',(8.9,-55.5972887473373,-138.629184351487));
#175240=CARTESIAN_POINT('Ctrl Pts',(8.9,-55.5972887473416,-93.4294586200098));
#175241=CARTESIAN_POINT('Ctrl Pts',(8.89999999999997,-55.2270244231188,
-93.2526539147005));
#175242=CARTESIAN_POINT('Ctrl Pts',(9.30242220787995,-55.1547652726018,
-93.2181494891395));
#175243=CARTESIAN_POINT('Ctrl Pts',(8.9,-60.7433024895534,-82.6526792495127));
#175244=CARTESIAN_POINT('Ctrl Pts',(8.89999999981176,-60.4125449242165,
-82.3706902717217));
#175245=CARTESIAN_POINT('Ctrl Pts',(9.31365506854171,-60.298307210959,-82.4413594877101));
#175246=CARTESIAN_POINT('Ctrl Pts',(8.9,-65.8565639782118,-71.8603324984455));
#175247=CARTESIAN_POINT('Ctrl Pts',(8.89999999999997,-65.4986935712713,
-71.6191417519029));
#175248=CARTESIAN_POINT('Ctrl Pts',(9.32127686740287,-65.4102595335587,
-71.6490160146723));
#175249=CARTESIAN_POINT('Ctrl Pts',(8.9,-70.9575466375288,-61.0621827299711));
#175250=CARTESIAN_POINT('Ctrl Pts',(8.89999999999996,-70.5668839574465,
-60.8776359696917));
#175251=CARTESIAN_POINT('Ctrl Pts',(9.32749162718857,-70.5102313269446,
-60.8508735991008));
#175252=CARTESIAN_POINT('',(9.32749162718857,-70.5102313269446,-60.8508735991008));
#175253=CARTESIAN_POINT('Ctrl Pts',(9.32749162718857,-70.5102313269446,
-60.8508735991008));
#175254=CARTESIAN_POINT('Ctrl Pts',(9.32582952826763,-69.1462755360622,
-63.7387697434672));
#175255=CARTESIAN_POINT('Ctrl Pts',(9.32415588545215,-67.8258212790612,
-66.5319899948945));
#175256=CARTESIAN_POINT('Ctrl Pts',(9.32147279007466,-65.91040469489,-70.579806532627));
#175257=CARTESIAN_POINT('Ctrl Pts',(9.32055305784016,-65.2828097278533,
-71.9054097386364));
#175258=CARTESIAN_POINT('Ctrl Pts',(9.31914659172631,-64.3577321272153,
-73.8583110877983));
#175259=CARTESIAN_POINT('Ctrl Pts',(9.31843696007727,-63.8992720094891,
-74.8258858974162));
#175260=CARTESIAN_POINT('Ctrl Pts',(9.31760366459636,-63.3715390091911,
-75.9391904116184));
#175261=CARTESIAN_POINT('Ctrl Pts',(9.31713451737182,-63.0766964068097,
-76.5610556110707));
#175262=CARTESIAN_POINT('Ctrl Pts',(9.31690371853256,-62.9322529809882,
-76.8656644741659));
#175263=CARTESIAN_POINT('Ctrl Pts',(9.31678465495306,-62.8578608284992,
-77.0225352384175));
#175264=CARTESIAN_POINT('Ctrl Pts',(9.31677841983388,-62.8539654033096,
-77.0307494927582));
#175265=CARTESIAN_POINT('Ctrl Pts',(9.31234247770848,-60.0829432119856,
-82.8739514734244));
#175266=CARTESIAN_POINT('Ctrl Pts',(9.30758397812651,-57.5183467731809,
-88.265954719794));
#175267=CARTESIAN_POINT('Ctrl Pts',(9.30242220787995,-55.1547652726018,
-93.2181494891395));
#175268=CARTESIAN_POINT('',(8.9,-70.9575466375288,-61.0621827299711));
#175269=CARTESIAN_POINT('Origin',(9.4,-70.9575466375288,-61.0621827299711));
#175270=CARTESIAN_POINT('Ctrl Pts',(8.9,-55.5972887473416,-93.4294586200098));
#175271=CARTESIAN_POINT('Ctrl Pts',(8.9,-60.7433024895534,-82.6526792495127));
#175272=CARTESIAN_POINT('Ctrl Pts',(8.9,-65.8565639782118,-71.8603324984455));
#175273=CARTESIAN_POINT('Ctrl Pts',(8.9,-70.9575466375288,-61.0621827299711));
#175274=CARTESIAN_POINT('Origin',(8.4,-72.58000002,-55.24995));
#175275=CARTESIAN_POINT('',(8.4,-73.08000002,-174.451268889151));
#175276=CARTESIAN_POINT('',(8.9,-72.58000002,-174.451268889151));
#175277=CARTESIAN_POINT('Origin',(8.4,-72.58000002,-174.451268889151));
#175278=CARTESIAN_POINT('',(8.9,-72.58000002,-58.1763194612681));
#175279=CARTESIAN_POINT('',(8.9,-72.58000002,-174.432329119515));
#175280=CARTESIAN_POINT('',(8.4,-73.08000002,-58.1763194612681));
#175281=CARTESIAN_POINT('Origin',(8.4,-72.58000002,-58.1763194612681));
#175282=CARTESIAN_POINT('',(8.4,-73.08000002,-58.1922197332626));
#175283=CARTESIAN_POINT('Origin',(-3.54807775957937E-14,-73.08000002,3.11172719585489E-30));
#175284=CARTESIAN_POINT('',(7.9,-73.08000002,-58.1594740865074));
#175285=CARTESIAN_POINT('Ctrl Pts',(8.4,-73.08000002,-58.1763194612681));
#175286=CARTESIAN_POINT('Ctrl Pts',(8.23332974561635,-73.08000002,-58.1708448514923));
#175287=CARTESIAN_POINT('Ctrl Pts',(8.06666350196851,-73.08000002,-58.1652131587787));
#175288=CARTESIAN_POINT('Ctrl Pts',(7.9,-73.08000002,-58.1594740865074));
#175289=CARTESIAN_POINT('',(7.9,-73.08000002,-174.471034982976));
#175290=CARTESIAN_POINT('',(7.9,-73.08000002,-174.491325336599));
#175291=CARTESIAN_POINT('Ctrl Pts',(7.9,-73.08000002,-174.471034982976));
#175292=CARTESIAN_POINT('Ctrl Pts',(8.06666381945983,-73.08000002,-174.464342510025));
#175293=CARTESIAN_POINT('Ctrl Pts',(8.23333002609749,-73.08000002,-174.457737044943));
#175294=CARTESIAN_POINT('Ctrl Pts',(8.4,-73.08000002,-174.451268889151));
#175295=CARTESIAN_POINT('Origin',(7.9,-72.58000002,-55.24995));
#175296=CARTESIAN_POINT('',(7.4,-72.58000002,-58.1594740865074));
#175297=CARTESIAN_POINT('Origin',(7.9,-72.58000002,-58.1594740865074));
#175298=CARTESIAN_POINT('',(7.4,-72.58000002,-174.471034982976));
#175299=CARTESIAN_POINT('',(7.4,-72.58000002,-58.1419820049528));
#175300=CARTESIAN_POINT('Origin',(7.9,-72.58000002,-174.471034982976));
#175301=CARTESIAN_POINT('Ctrl Pts',(7.4,-55.5541151520872,-137.531452880088));
#175302=CARTESIAN_POINT('Ctrl Pts',(7.39999999999997,-55.0309624818203,
-137.77858424555));
#175303=CARTESIAN_POINT('Ctrl Pts',(6.82752390105444,-55.106794611208,-137.742762010959));
#175304=CARTESIAN_POINT('Ctrl Pts',(7.4,-60.858236996045,-148.759754479668));
#175305=CARTESIAN_POINT('Ctrl Pts',(7.39999999999996,-60.2903951615484,
-148.888188464867));
#175306=CARTESIAN_POINT('Ctrl Pts',(6.83631982946675,-60.4094944461354,
-148.971070239217));
#175307=CARTESIAN_POINT('Ctrl Pts',(7.4,-66.1431501582269,-159.997106821727));
#175308=CARTESIAN_POINT('Ctrl Pts',(7.40000000024359,-65.6065688428949,
-160.175729571892));
#175309=CARTESIAN_POINT('Ctrl Pts',(6.84214680798085,-65.6936814170396,
-160.208420694715));
#175310=CARTESIAN_POINT('Ctrl Pts',(7.4,-71.4211246238516,-171.237717270032));
#175311=CARTESIAN_POINT('Ctrl Pts',(7.39999999999995,-70.9175980522951,
-171.474145745141));
#175312=CARTESIAN_POINT('Ctrl Pts',(6.84687749809456,-70.9710952348089,
-171.449026400902));
#175313=CARTESIAN_POINT('',(6.84687749809456,-70.9710952348089,-171.449026400902));
#175314=CARTESIAN_POINT('',(7.4,-71.4211246238516,-171.237717270032));
#175315=CARTESIAN_POINT('Origin',(6.9,-71.4211246238516,-171.237717270032));
#175316=CARTESIAN_POINT('',(7.4,-55.5541151520872,-137.531452880088));
#175317=CARTESIAN_POINT('Ctrl Pts',(7.4,-55.5541151520872,-137.531452880088));
#175318=CARTESIAN_POINT('Ctrl Pts',(7.4,-60.858236996045,-148.759754479668));
#175319=CARTESIAN_POINT('Ctrl Pts',(7.4,-66.1431501582269,-159.997106821727));
#175320=CARTESIAN_POINT('Ctrl Pts',(7.4,-71.4211246238516,-171.237717270032));
#175321=CARTESIAN_POINT('Origin',(6.9,-55.5541151520872,-137.531452880088));
#175322=CARTESIAN_POINT('Ctrl Pts',(6.84687749809456,-70.9710952348089,
-171.449026400902));
#175323=CARTESIAN_POINT('Ctrl Pts',(6.84560962234199,-69.5566916474712,
-168.436423337422));
#175324=CARTESIAN_POINT('Ctrl Pts',(6.84434141864909,-68.1892497014956,
-165.525328844702));
#175325=CARTESIAN_POINT('Ctrl Pts',(6.84229651062739,-66.2085386323005,
-161.310949961766));
#175326=CARTESIAN_POINT('Ctrl Pts',(6.84124275267032,-65.2357958436729,
-159.241826234334));
#175327=CARTESIAN_POINT('Ctrl Pts',(6.83997337454142,-64.1317508737894,
-156.894463551891));
#175328=CARTESIAN_POINT('Ctrl Pts',(6.83933395326739,-63.5874334599924,
-155.73743596056));
#175329=CARTESIAN_POINT('Ctrl Pts',(6.83897379504999,-63.2834219089447,
-155.091291807594));
#175330=CARTESIAN_POINT('Ctrl Pts',(6.83879657177648,-63.134517564385,-154.774836350161));
#175331=CARTESIAN_POINT('Ctrl Pts',(6.83870513850053,-63.0578356875946,
-154.611876236652));
#175332=CARTESIAN_POINT('Ctrl Pts',(6.83870038730762,-63.0538514139574,
-154.603409094398));
#175333=CARTESIAN_POINT('Ctrl Pts',(6.83527484268849,-60.1816612512713,
-148.499619545533));
#175334=CARTESIAN_POINT('Ctrl Pts',(6.83155090300906,-57.5345067998195,
-142.883369926133));
#175335=CARTESIAN_POINT('Ctrl Pts',(6.82752390105444,-55.106794611208,-137.742762010959));
#175336=CARTESIAN_POINT('Ctrl Pts',(6.82155174273623,-55.1933079511192,
-137.915802602945));
#175337=CARTESIAN_POINT('Ctrl Pts',(7.40000000000079,-55.1116820355855,
-137.95800482368));
#175338=CARTESIAN_POINT('Ctrl Pts',(7.4,-55.6319612289116,-137.689008690545));
#175339=CARTESIAN_POINT('Ctrl Pts',(6.83574484367583,-54.9750692399274,
-137.49783139603));
#175340=CARTESIAN_POINT('Ctrl Pts',(7.39999999999827,-54.9102656072896,
-137.531225757498));
#175341=CARTESIAN_POINT('Ctrl Pts',(7.4,-55.4355479201386,-137.308418641867));
#175342=CARTESIAN_POINT('Ctrl Pts',(6.84992613641256,-54.8164562186196,
-137.062923068212));
#175343=CARTESIAN_POINT('Ctrl Pts',(7.39999999999997,-54.7649351562061,
-137.085189013788));
#175344=CARTESIAN_POINT('Ctrl Pts',(7.4,-55.2927998688587,-136.91270337825));
#175345=CARTESIAN_POINT('Ctrl Pts',(6.87803385475026,-54.6118666660822,
-136.161406076667));
#175346=CARTESIAN_POINT('Ctrl Pts',(7.39999999999997,-54.5904817529938,
-136.169973106407));
#175347=CARTESIAN_POINT('Ctrl Pts',(7.4,-55.1086754192619,-136.09302879305));
#175348=CARTESIAN_POINT('Ctrl Pts',(6.89206539026919,-54.566470030062,-135.690989882161));
#175349=CARTESIAN_POINT('Ctrl Pts',(7.40000000000168,-54.5583847259971,
-135.696616305969));
#175350=CARTESIAN_POINT('Ctrl Pts',(7.4,-55.0678212801175,-135.665613736665));
#175351=CARTESIAN_POINT('Ctrl Pts',(6.90540919710522,-54.5834976982804,
-135.222393609581));
#175352=CARTESIAN_POINT('Ctrl Pts',(7.39999999999918,-54.5888446965326,
-135.222564106606));
#175353=CARTESIAN_POINT('Ctrl Pts',(7.4,-55.0831491250257,-135.24013604883));
#175354=CARTESIAN_POINT('',(7.4,-55.08000002,-135.415380765739));
#175355=CARTESIAN_POINT('Ctrl Pts',(7.4,-55.08000002,-135.415380765739));
#175356=CARTESIAN_POINT('Ctrl Pts',(7.4,-55.08000002,-135.642528198471));
#175357=CARTESIAN_POINT('Ctrl Pts',(7.4,-55.0958102967117,-135.869567477776));
#175358=CARTESIAN_POINT('Ctrl Pts',(7.4,-55.1266901212397,-136.093433076221));
#175359=CARTESIAN_POINT('Ctrl Pts',(7.4,-55.1457148268955,-136.231354103363));
#175360=CARTESIAN_POINT('Ctrl Pts',(7.4,-55.1704583130128,-136.368070310451));
#175361=CARTESIAN_POINT('Ctrl Pts',(7.4,-55.2007376448274,-136.502866089854));
#175362=CARTESIAN_POINT('Ctrl Pts',(7.4,-55.2691608068209,-136.807468367956));
#175363=CARTESIAN_POINT('Ctrl Pts',(7.4,-55.3655723350795,-137.104245532169));
#175364=CARTESIAN_POINT('Ctrl Pts',(7.4,-55.4912205286075,-137.392848584246));
#175365=CARTESIAN_POINT('Ctrl Pts',(7.4,-55.5114273685592,-137.439261950958));
#175366=CARTESIAN_POINT('Ctrl Pts',(7.4,-55.5323904712439,-137.485463878358));
#175367=CARTESIAN_POINT('Ctrl Pts',(7.4,-55.5541151520872,-137.531452880088));
#175368=CARTESIAN_POINT('Origin',(6.9,-55.08000002,-135.415380765739));
#175369=CARTESIAN_POINT('Origin',(6.9,-55.08000002,-55.24995));
#175370=CARTESIAN_POINT('',(7.4,-55.08000002,-96.6432622057672));
#175371=CARTESIAN_POINT('',(7.4,-55.08000002,-135.57795249279));
#175372=CARTESIAN_POINT('Origin',(6.9,-55.08000002,-96.6432622057672));
#175373=CARTESIAN_POINT('Ctrl Pts',(6.9,-54.58000002,-96.6432622057672));
#175374=CARTESIAN_POINT('Ctrl Pts',(7.39999999999996,-54.58000002,-96.6432622057672));
#175375=CARTESIAN_POINT('Ctrl Pts',(7.4,-55.08000002,-96.6432622057672));
#175376=CARTESIAN_POINT('Ctrl Pts',(6.8883412776675,-54.58000002,-96.2390470799649));
#175377=CARTESIAN_POINT('Ctrl Pts',(7.39999999999997,-54.5682037738145,
-96.2342789461818));
#175378=CARTESIAN_POINT('Ctrl Pts',(7.4,-55.0800000228223,-96.276173584436));
#175379=CARTESIAN_POINT('Ctrl Pts',(6.87644795534686,-54.6248256750472,
-95.842546745885));
#175380=CARTESIAN_POINT('Ctrl Pts',(7.39999999999997,-54.6014014206736,
-95.8348803330818));
#175381=CARTESIAN_POINT('Ctrl Pts',(7.4,-55.1203431091477,-95.9158883524807));
#175382=CARTESIAN_POINT('Ctrl Pts',(6.85220551019199,-54.8002766424245,
-95.064563743706));
#175383=CARTESIAN_POINT('Ctrl Pts',(7.39999999999995,-54.7508604913788,
-95.0452270964761));
#175384=CARTESIAN_POINT('Ctrl Pts',(7.4,-55.2782489805768,-95.2085406483778));
#175385=CARTESIAN_POINT('Ctrl Pts',(6.83977061757738,-54.9324757245047,
-94.6806963574476));
#175386=CARTESIAN_POINT('Ctrl Pts',(7.39999999999369,-54.8709621105524,
-94.6521767160421));
#175387=CARTESIAN_POINT('Ctrl Pts',(7.4,-55.3972278356279,-94.8593050327909));
#175388=CARTESIAN_POINT('Ctrl Pts',(6.82752390105444,-55.106794611208,-94.3158809605474));
#175389=CARTESIAN_POINT('Ctrl Pts',(7.39999999999997,-55.0309624818203,
-94.2800587259558));
#175390=CARTESIAN_POINT('Ctrl Pts',(7.4,-55.5541151520872,-94.5271900914177));
#175391=CARTESIAN_POINT('',(7.4,-55.5541151520872,-94.5271900914178));
#175392=CARTESIAN_POINT('Ctrl Pts',(7.4,-55.5541151520872,-94.5271900914178));
#175393=CARTESIAN_POINT('Ctrl Pts',(7.4,-55.4646684466496,-94.7165399244866));
#175394=CARTESIAN_POINT('Ctrl Pts',(7.4,-55.3874966670403,-94.9115657139011));
#175395=CARTESIAN_POINT('Ctrl Pts',(7.4,-55.3230550301972,-95.1098279144973));
#175396=CARTESIAN_POINT('Ctrl Pts',(7.4,-55.2745243397298,-95.2591382355855));
#175397=CARTESIAN_POINT('Ctrl Pts',(7.4,-55.2332126733291,-95.4102831677243));
#175398=CARTESIAN_POINT('Ctrl Pts',(7.4,-55.199296044664,-95.5622145003849));
#175399=CARTESIAN_POINT('Ctrl Pts',(7.4,-55.1306219000107,-95.8698439649617));
#175400=CARTESIAN_POINT('Ctrl Pts',(7.4,-55.0911602505336,-96.1824496092641));
#175401=CARTESIAN_POINT('Ctrl Pts',(7.4,-55.0820478268106,-96.5002250748419));
#175402=CARTESIAN_POINT('Ctrl Pts',(7.4,-55.0806839263479,-96.5477880633181));
#175403=CARTESIAN_POINT('Ctrl Pts',(7.4,-55.08000002,-96.5954668848809));
#175404=CARTESIAN_POINT('Ctrl Pts',(7.4,-55.08000002,-96.6432622057672));
#175405=CARTESIAN_POINT('',(6.82752390124981,-55.1067946109655,-94.3158809609937));
#175406=CARTESIAN_POINT('Origin',(6.9,-55.5541151520872,-94.5271900914178));
#175407=CARTESIAN_POINT('Ctrl Pts',(6.9,-54.58000002,-96.6432622057672));
#175408=CARTESIAN_POINT('Ctrl Pts',(6.89747516029584,-54.58000002,-96.5557244490382));
#175409=CARTESIAN_POINT('Ctrl Pts',(6.89483138514496,-54.5820978077061,
-96.4637717709372));
#175410=CARTESIAN_POINT('Ctrl Pts',(6.89203565904072,-54.5869879127523,
-96.3675661682017));
#175411=CARTESIAN_POINT('Ctrl Pts',(6.88947633569459,-54.5914645172348,
-96.2794955790493));
#175412=CARTESIAN_POINT('Ctrl Pts',(6.88678966447231,-54.5982820020438,
-96.1878610154668));
#175413=CARTESIAN_POINT('Ctrl Pts',(6.88394936679525,-54.6080107494815,
-96.0927938740058));
#175414=CARTESIAN_POINT('Ctrl Pts',(6.88097789104612,-54.6181888154334,
-95.9933360926358));
#175415=CARTESIAN_POINT('Ctrl Pts',(6.87784445989682,-54.6315541980301,
-95.890142050635));
#175416=CARTESIAN_POINT('Ctrl Pts',(6.87456401227554,-54.6487592943821,
-95.7835116338186));
#175417=CARTESIAN_POINT('Ctrl Pts',(6.8729237884649,-54.6573618425582,-95.7301964254104));
#175418=CARTESIAN_POINT('Ctrl Pts',(6.87124734708462,-54.6669241215913,
-95.6760238582546));
#175419=CARTESIAN_POINT('Ctrl Pts',(6.86953990780671,-54.6775244017527,
-95.6210418063674));
#175420=CARTESIAN_POINT('Ctrl Pts',(6.86868618816775,-54.6828245418335,
-95.5935507804238));
#175421=CARTESIAN_POINT('Ctrl Pts',(6.86782471473417,-54.6883841572439,
-95.5658573703005));
#175422=CARTESIAN_POINT('Ctrl Pts',(6.86695640095496,-54.6942126277729,
-95.5379683292162));
#175423=CARTESIAN_POINT('Ctrl Pts',(6.86652224406536,-54.6971268630374,
-95.524023808674));
#175424=CARTESIAN_POINT('Ctrl Pts',(6.86608637653929,-54.7001083092455,
-95.510030378775));
#175425=CARTESIAN_POINT('Ctrl Pts',(6.86564891907798,-54.7031581143021,
-95.4959889008478));
#175426=CARTESIAN_POINT('Ctrl Pts',(6.86543019034733,-54.7046830168303,
-95.4889681618842));
#175427=CARTESIAN_POINT('Ctrl Pts',(6.86521106409204,-54.7062250088754,
-95.4819354107944));
#175428=CARTESIAN_POINT('Ctrl Pts',(6.86499155622248,-54.7077842319553,
-95.4748907575898));
#175429=CARTESIAN_POINT('Ctrl Pts',(6.86488180228771,-54.7085638434952,
-95.4713684309875));
#175430=CARTESIAN_POINT('Ctrl Pts',(6.86477195294651,-54.7093477627807,
-95.4678431288482));
#175431=CARTESIAN_POINT('Ctrl Pts',(6.8646620102436,-54.7101360073698,-95.4643148650801));
#175432=CARTESIAN_POINT('Ctrl Pts',(6.86455206754068,-54.7109242519588,
-95.460786601312));
#175433=CARTESIAN_POINT('Ctrl Pts',(6.86438870235264,-54.7121027263867,
-95.4555439545126));
#175434=CARTESIAN_POINT('Ctrl Pts',(6.86433190484278,-54.7125137344833,
-95.453721202814));
#175435=CARTESIAN_POINT('Ctrl Pts',(6.86433018162012,-54.7125262043691,
-95.4536659009699));
#175436=CARTESIAN_POINT('Ctrl Pts',(6.86432845787219,-54.7125386791002,
-95.453610581626));
#175437=CARTESIAN_POINT('Ctrl Pts',(6.86432673359892,-54.712551158678,-95.4535552447826));
#175438=CARTESIAN_POINT('Ctrl Pts',(6.86351930135692,-54.7183950198008,
-95.4276424428322));
#175439=CARTESIAN_POINT('Ctrl Pts',(6.86259629795188,-54.7253045249752,
-95.3978804668901));
#175440=CARTESIAN_POINT('Ctrl Pts',(6.86155176392851,-54.7334765966147,
-95.3643212878303));
#175441=CARTESIAN_POINT('Ctrl Pts',(6.86051181961651,-54.7416127599454,
-95.3309095687308));
#175442=CARTESIAN_POINT('Ctrl Pts',(6.85935139548513,-54.7510005850816,
-95.2937335050213));
#175443=CARTESIAN_POINT('Ctrl Pts',(6.85806469255273,-54.7618822044733,
-95.2528636616271));
#175444=CARTESIAN_POINT('Ctrl Pts',(6.8577356277149,-54.7646650988231,-95.2424114989327));
#175445=CARTESIAN_POINT('Ctrl Pts',(6.85739830478949,-54.7675459309099,
-95.2317178653169));
#175446=CARTESIAN_POINT('Ctrl Pts',(6.85705262961774,-54.7705292349977,
-95.2207842021938));
#175447=CARTESIAN_POINT('Ctrl Pts',(6.85571293772219,-54.7820912696329,
-95.1784099124803));
#175448=CARTESIAN_POINT('Ctrl Pts',(6.85424828974271,-54.7951888263501,
-95.1324292778536));
#175449=CARTESIAN_POINT('Ctrl Pts',(6.85266114233615,-54.8101095220533,
-95.0829520905385));
#175450=CARTESIAN_POINT('Ctrl Pts',(6.85243695912735,-54.8122170575137,
-95.0759634803005));
#175451=CARTESIAN_POINT('Ctrl Pts',(6.8522103329922,-54.8143610336592,-95.0689051620074));
#175452=CARTESIAN_POINT('Ctrl Pts',(6.85198127202152,-54.8165423261462,
-95.0617774993062));
#175453=CARTESIAN_POINT('Ctrl Pts',(6.85105590131421,-54.8253544086477,
-95.0329828501979));
#175454=CARTESIAN_POINT('Ctrl Pts',(6.85009096050149,-54.8347751397566,
-95.0030562681139));
#175455=CARTESIAN_POINT('Ctrl Pts',(6.84908838500605,-54.8448644132515,
-94.9720250304464));
#175456=CARTESIAN_POINT('Ctrl Pts',(6.84858709725833,-54.8499090499989,
-94.9565094116127));
#175457=CARTESIAN_POINT('Ctrl Pts',(6.84807640877095,-54.8551208983739,
-94.940717653009));
#175458=CARTESIAN_POINT('Ctrl Pts',(6.84755689936396,-54.8605077376624,
-94.9246536948557));
#175459=CARTESIAN_POINT('Ctrl Pts',(6.847151051795,-54.8647160072338,-94.9121043198558));
#175460=CARTESIAN_POINT('Ctrl Pts',(6.84671716909453,-54.8692741665164,
-94.8986776066087));
#175461=CARTESIAN_POINT('Ctrl Pts',(6.84630851886264,-54.8736171201975,
-94.8860425593514));
#175462=CARTESIAN_POINT('Ctrl Pts',(6.84619407210966,-54.8748334096018,
-94.88250398279));
#175463=CARTESIAN_POINT('Ctrl Pts',(6.84608160495438,-54.8760325092529,
-94.8790274153598));
#175464=CARTESIAN_POINT('Ctrl Pts',(6.84597228850087,-54.8772013065748,
-94.8756493244326));
#175465=CARTESIAN_POINT('Ctrl Pts',(6.84397369594434,-54.8985699985937,
-94.8138889291219));
#175466=CARTESIAN_POINT('Ctrl Pts',(6.84208965831291,-54.9198341771577,
-94.7560365588245));
#175467=CARTESIAN_POINT('Ctrl Pts',(6.84032134685682,-54.9406229360708,
-94.7020029951088));
#175468=CARTESIAN_POINT('Ctrl Pts',(6.83855714785133,-54.9613633478765,
-94.6480950938497));
#175469=CARTESIAN_POINT('Ctrl Pts',(6.8369081109529,-54.9816307635276,-94.5979875534939));
#175470=CARTESIAN_POINT('Ctrl Pts',(6.83537425787087,-55.001110405453,-94.551575598675));
#175471=CARTESIAN_POINT('Ctrl Pts',(6.83381061644668,-55.0209683536487,
-94.5042622959978));
#175472=CARTESIAN_POINT('Ctrl Pts',(6.83236665529882,-55.0400076472729,
-94.4607889078687));
#175473=CARTESIAN_POINT('Ctrl Pts',(6.83104156414129,-55.0579490545743,
-94.4210374968657));
#175474=CARTESIAN_POINT('Ctrl Pts',(6.82975787054648,-55.0753299490915,
-94.3825279713894));
#175475=CARTESIAN_POINT('Ctrl Pts',(6.82858571520043,-55.0916808891523,
-94.347511028551));
#175476=CARTESIAN_POINT('Ctrl Pts',(6.82752390106997,-55.106794610987,-94.31588096101));
#175477=CARTESIAN_POINT('Ctrl Pts',(7.4,-71.3078420373655,-61.0621827299711));
#175478=CARTESIAN_POINT('Ctrl Pts',(7.39999999999997,-70.8042142666047,
-60.8257004209668));
#175479=CARTESIAN_POINT('Ctrl Pts',(6.84677576889373,-70.8578246683297,
-60.8508735991007));
#175480=CARTESIAN_POINT('Ctrl Pts',(7.4,-66.0675133276181,-72.2223201517098));
#175481=CARTESIAN_POINT('Ctrl Pts',(7.39999999999996,-65.5311408351844,
-72.0430210271706));
#175482=CARTESIAN_POINT('Ctrl Pts',(6.84206094040904,-65.61805576689,-72.0110063808198));
#175483=CARTESIAN_POINT('Ctrl Pts',(7.4,-60.8202894597531,-83.3792196747323));
#175484=CARTESIAN_POINT('Ctrl Pts',(7.39999999995234,-60.2531402990131,
-83.2491486934777));
#175485=CARTESIAN_POINT('Ctrl Pts',(6.83625690025051,-60.3715570323219,
-83.1679040708394));
#175486=CARTESIAN_POINT('Ctrl Pts',(7.4,-55.5541151520872,-94.5271900914177));
#175487=CARTESIAN_POINT('Ctrl Pts',(7.39999999999997,-55.0309624818203,
-94.2800587259558));
#175488=CARTESIAN_POINT('Ctrl Pts',(6.82752390105444,-55.106794611208,-94.3158809605474));
#175489=CARTESIAN_POINT('',(7.4,-71.3078420373655,-61.0621827299711));
#175490=CARTESIAN_POINT('Ctrl Pts',(7.4,-71.3078420373655,-61.0621827299711));
#175491=CARTESIAN_POINT('Ctrl Pts',(7.4,-66.0675133276181,-72.2223201517098));
#175492=CARTESIAN_POINT('Ctrl Pts',(7.4,-60.8202894597531,-83.3792196747323));
#175493=CARTESIAN_POINT('Ctrl Pts',(7.4,-55.5541151520872,-94.5271900914177));
#175494=CARTESIAN_POINT('',(6.84677576889373,-70.8578246683297,-60.8508735991007));
#175495=CARTESIAN_POINT('Origin',(6.9,-71.3078420373655,-61.0621827299711));
#175496=CARTESIAN_POINT('Ctrl Pts',(6.82752390105444,-55.106794611208,-94.3158809605474));
#175497=CARTESIAN_POINT('Ctrl Pts',(6.82952415560735,-56.3126649847602,
-91.7624865276987));
#175498=CARTESIAN_POINT('Ctrl Pts',(6.8315454834894,-57.5727256222142,-89.0918089072798));
#175499=CARTESIAN_POINT('Ctrl Pts',(6.83340376219997,-58.8869041773412,
-86.3038079768894));
#175500=CARTESIAN_POINT('Ctrl Pts',(6.83433290155526,-59.5439934549047,
-84.9098075116943));
#175501=CARTESIAN_POINT('Ctrl Pts',(6.83522669847064,-60.2146122398928,
-83.4864764706228));
#175502=CARTESIAN_POINT('Ctrl Pts',(6.83609469396308,-60.8987533307654,
-82.0338119093995));
#175503=CARTESIAN_POINT('Ctrl Pts',(6.83652869170931,-61.2408238762017,
-81.3074796287878));
#175504=CARTESIAN_POINT('Ctrl Pts',(6.83695657838775,-61.5862750307562,
-80.5738139942268));
#175505=CARTESIAN_POINT('Ctrl Pts',(6.83738159482193,-61.9351061371133,
-79.8328148104165));
#175506=CARTESIAN_POINT('Ctrl Pts',(6.83759410303902,-62.1095216902918,
-79.4623152185113));
#175507=CARTESIAN_POINT('Ctrl Pts',(6.83780589456058,-62.284782236783,-79.0899822418052));
#175508=CARTESIAN_POINT('Ctrl Pts',(6.83801780376435,-62.4608876783509,
-78.7158158549579));
#175509=CARTESIAN_POINT('Ctrl Pts',(6.83812375836623,-62.5489403991348,
-78.5287326615342));
#175510=CARTESIAN_POINT('Ctrl Pts',(6.83823079828926,-62.6372042208913,
-78.3411910683908));
#175511=CARTESIAN_POINT('Ctrl Pts',(6.83833751782365,-62.7256793104055,
-78.1531911415523));
#175512=CARTESIAN_POINT('Ctrl Pts',(6.83839254508357,-62.7712992784363,
-78.0562536792761));
#175513=CARTESIAN_POINT('Ctrl Pts',(6.83844748719141,-62.8169754159942,
-77.9591943601788));
#175514=CARTESIAN_POINT('Ctrl Pts',(6.83850234420444,-62.8627077234333,
-77.8620131846426));
#175515=CARTESIAN_POINT('Ctrl Pts',(6.83852934414054,-62.885216593501,-77.8141818248084));
#175516=CARTESIAN_POINT('Ctrl Pts',(6.83855632346278,-62.9077390706416,
-77.7663209454311));
#175517=CARTESIAN_POINT('Ctrl Pts',(6.83858328217936,-62.9302751549059,
-77.7184305465605));
#175518=CARTESIAN_POINT('Ctrl Pts',(6.83859665623016,-62.941455165459,-77.6946724189958));
#175519=CARTESIAN_POINT('Ctrl Pts',(6.83861002520974,-62.9526385248478,
-77.6709070264179));
#175520=CARTESIAN_POINT('Ctrl Pts',(6.83862338911918,-62.9638252330791,
-77.6471343688332));
#175521=CARTESIAN_POINT('Ctrl Pts',(6.83862671704584,-62.9666109856172,
-77.6412144199229));
#175522=CARTESIAN_POINT('Ctrl Pts',(6.83863004465809,-62.969396945826,-77.6352940204902));
#175523=CARTESIAN_POINT('Ctrl Pts',(6.83863337195595,-62.9721831137055,
-77.629373170535));
#175524=CARTESIAN_POINT('Ctrl Pts',(6.83863417442051,-62.9728550706734,
-77.6279452033216));
#175525=CARTESIAN_POINT('Ctrl Pts',(6.83863497686678,-62.9735270397206,
-77.6265172099031));
#175526=CARTESIAN_POINT('Ctrl Pts',(6.83863577929477,-62.9741990208472,
-77.6250891902796));
#175527=CARTESIAN_POINT('Ctrl Pts',(6.83863645562837,-62.9747654061459,
-77.6238855711764));
#175528=CARTESIAN_POINT('Ctrl Pts',(6.83863712970764,-62.9753299227988,
-77.6226859227363));
#175529=CARTESIAN_POINT('Ctrl Pts',(6.83863781492277,-62.9759037853613,
-77.6214664130097));
#175530=CARTESIAN_POINT('Ctrl Pts',(6.83864118100574,-62.9787228547662,
-77.6154756361513));
#175531=CARTESIAN_POINT('Ctrl Pts',(6.83864475015493,-62.9817125075398,
-77.609122344141));
#175532=CARTESIAN_POINT('Ctrl Pts',(6.83864816330869,-62.984572000546,-77.6030456438992));
#175533=CARTESIAN_POINT('Ctrl Pts',(6.83864986821899,-62.9860003508123,
-77.6000102609171));
#175534=CARTESIAN_POINT('Ctrl Pts',(6.83865153421473,-62.987396224711,-77.5970438909131));
#175535=CARTESIAN_POINT('Ctrl Pts',(6.83865311659043,-62.9887221396635,
-77.5942261885717));
#175536=CARTESIAN_POINT('Ctrl Pts',(6.83865381739304,-62.9893093609242,
-77.5929782844598));
#175537=CARTESIAN_POINT('Ctrl Pts',(6.83865450179456,-62.9898828602488,
-77.5917595404295));
#175538=CARTESIAN_POINT('Ctrl Pts',(6.83865516591314,-62.990439381622,-77.5905768759047));
#175539=CARTESIAN_POINT('Ctrl Pts',(6.83865566961575,-62.9908614768272,
-77.5896798806604));
#175540=CARTESIAN_POINT('Ctrl Pts',(6.83865616165061,-62.9912738054544,
-77.5888036401762));
#175541=CARTESIAN_POINT('Ctrl Pts',(6.83865664032437,-62.9916749469045,
-77.5879511734013));
#175542=CARTESIAN_POINT('Ctrl Pts',(6.83865696846394,-62.9919499366577,
-77.5873667919368));
#175543=CARTESIAN_POINT('Ctrl Pts',(6.83865729477323,-62.992223397155,-77.5867856602091));
#175544=CARTESIAN_POINT('Ctrl Pts',(6.83865762193763,-62.9924975788079,
-77.5862029958628));
#175545=CARTESIAN_POINT('Ctrl Pts',(6.84001201799662,-64.1275555370883,
-75.1740875375366));
#175546=CARTESIAN_POINT('Ctrl Pts',(6.84132064847969,-65.3028889469105,
-72.6748470242097));
#175547=CARTESIAN_POINT('Ctrl Pts',(6.84258533113874,-66.5185108777293,
-70.0884870713488));
#175548=CARTESIAN_POINT('Ctrl Pts',(6.84378902860916,-67.6755134132239,
-67.6268458757626));
#175549=CARTESIAN_POINT('Ctrl Pts',(6.84495288483861,-68.8690124037817,
-65.08628466818));
#175550=CARTESIAN_POINT('Ctrl Pts',(6.84608524591606,-70.0990616765064,
-62.4668293203369));
#175551=CARTESIAN_POINT('Ctrl Pts',(6.84631667458969,-70.3504555802412,
-61.9314726316618));
#175552=CARTESIAN_POINT('Ctrl Pts',(6.84654681219227,-70.6033763429088,
-61.3928206107334));
#175553=CARTESIAN_POINT('Ctrl Pts',(6.84677576889373,-70.8578246683297,
-60.8508735991007));
#175554=CARTESIAN_POINT('Ctrl Pts',(7.58857520038279,-54.58000002,-96.4164960598359));
#175555=CARTESIAN_POINT('Ctrl Pts',(7.2042299691157,-54.58000002,-95.3011321772634));
#175556=CARTESIAN_POINT('Ctrl Pts',(6.8604212943599,-55.1073456615429,-94.3034047511324));
#175557=CARTESIAN_POINT('Ctrl Pts',(6.56867789944001,-54.58000002,-96.7679442920248));
#175558=CARTESIAN_POINT('Ctrl Pts',(6.23607825680947,-54.580000019985,-95.6541184528592));
#175559=CARTESIAN_POINT('Ctrl Pts',(5.93585888223459,-55.0918247516195,
-94.6548535475511));
#175560=CARTESIAN_POINT('Ctrl Pts',(5.52653095835546,-54.58000002,-97.0582339217052));
#175561=CARTESIAN_POINT('Ctrl Pts',(5.24614565799262,-54.58000002,-95.9461039187036));
#175562=CARTESIAN_POINT('Ctrl Pts',(4.99263467931988,-55.0788453329258,
-94.9451426129372));
#175563=CARTESIAN_POINT('Ctrl Pts',(3.38973164031852,-54.58000002,-97.4945129415963));
#175564=CARTESIAN_POINT('Ctrl Pts',(3.21753929952213,-54.58000002,-96.3846721597723));
#175565=CARTESIAN_POINT('Ctrl Pts',(3.06075099962147,-55.0592467101081,
-95.3814216329573));
#175566=CARTESIAN_POINT('Ctrl Pts',(2.28937244057036,-54.58000002,-97.638711952094));
#175567=CARTESIAN_POINT('Ctrl Pts',(2.17279343333145,-54.5800000200112,
-96.5297363078781));
#175568=CARTESIAN_POINT('Ctrl Pts',(2.0669285329079,-55.052711592208,-95.5256220795631));
#175569=CARTESIAN_POINT('Ctrl Pts',(1.21149627184771,-54.58000002,-97.6987697451473));
#175570=CARTESIAN_POINT('Ctrl Pts',(1.14972373305894,-54.5800000199999,
-96.5901184946094));
#175571=CARTESIAN_POINT('Ctrl Pts',(1.09375770007614,-55.0499908864773,
-95.5856784364438));
#175572=CARTESIAN_POINT('',(1.23668893160606,-55.0504165218159,-95.5762821576559));
#175573=CARTESIAN_POINT('Ctrl Pts',(1.23668893165476,-55.0504165218147,
-95.5762821576554));
#175574=CARTESIAN_POINT('Ctrl Pts',(1.71088764457684,-55.0519150062272,
-95.543198672456));
#175575=CARTESIAN_POINT('Ctrl Pts',(2.18480270652532,-55.0542599488238,
-95.4911648085245));
#175576=CARTESIAN_POINT('Ctrl Pts',(2.8961822350534,-55.0590678993593,-95.3846884445288));
#175577=CARTESIAN_POINT('Ctrl Pts',(3.25199862731268,-55.0617933172342,
-95.3243438705064));
#175578=CARTESIAN_POINT('Ctrl Pts',(3.6675418607141,-55.0655275836122,-95.2415056814372));
#175579=CARTESIAN_POINT('Ctrl Pts',(3.8754446803529,-55.0675314608682,-95.1969775403918));
#175580=CARTESIAN_POINT('Ctrl Pts',(3.96457669660492,-55.0684193417625,
-95.1772278271201));
#175581=CARTESIAN_POINT('Ctrl Pts',(4.0240051857539,-55.0690176961945,-95.1639133017718));
#175582=CARTESIAN_POINT('Ctrl Pts',(4.0549182561813,-55.069332380045,-95.1569083381592));
#175583=CARTESIAN_POINT('Ctrl Pts',(4.996285678452,-55.0790115168945,-94.941364334101));
#175584=CARTESIAN_POINT('Ctrl Pts',(5.90958570151961,-55.0914523430888,
-94.6631990870593));
#175585=CARTESIAN_POINT('Ctrl Pts',(6.82752390105444,-55.106794611208,-94.3158809605474));
#175586=CARTESIAN_POINT('Origin',(1.23481659430174,-62.0604750000681,-98.242868717055));
#175587=CARTESIAN_POINT('Ctrl Pts',(1.23668893165476,-55.0504165218147,
-95.5762821576554));
#175588=CARTESIAN_POINT('Ctrl Pts',(0.749999999999967,-55.0621625368995,
-95.5817617789931));
#175589=CARTESIAN_POINT('Ctrl Pts',(0.749999999999973,-55.5033748716332,
-95.7875912885257));
#175590=CARTESIAN_POINT('Ctrl Pts',(1.24124884403065,-54.7408920390033,
-96.2394858776278));
#175591=CARTESIAN_POINT('Ctrl Pts',(0.750000000004129,-54.7481304442385,
-96.2443585547261));
#175592=CARTESIAN_POINT('Ctrl Pts',(0.749999999999973,-55.2248025687359,
-96.3847337445855));
#175593=CARTESIAN_POINT('Ctrl Pts',(1.24576233955167,-54.58000002,-96.9572624945429));
#175594=CARTESIAN_POINT('Ctrl Pts',(0.750000000006829,-54.5842199033567,
-96.9603643458105));
#175595=CARTESIAN_POINT('Ctrl Pts',(0.749999999999973,-55.0800000216326,
-97.0309759697293));
#175596=CARTESIAN_POINT('Ctrl Pts',(1.25,-54.58000002,-97.6965903014517));
#175597=CARTESIAN_POINT('Ctrl Pts',(0.749999999999965,-54.5800000199999,
-97.6965903014516));
#175598=CARTESIAN_POINT('Ctrl Pts',(0.749999999999973,-55.08000002,-97.6965903014517));
#175599=CARTESIAN_POINT('',(0.749999999999973,-55.08000002,-97.6965903014517));
#175600=CARTESIAN_POINT('Origin',(1.24999999999997,-55.08000002,-97.6965903014517));
#175601=CARTESIAN_POINT('',(0.749999999999973,-55.5033748716332,-95.7875912885257));
#175602=CARTESIAN_POINT('Origin',(1.24999999999997,-55.5033748716332,-95.7875912885257));
#175603=CARTESIAN_POINT('Origin',(0.749999999999973,-61.7707294447932,-98.1780034241954));
#175604=CARTESIAN_POINT('Origin',(1.24999999999997,-55.08000002,-55.24995));
#175605=CARTESIAN_POINT('',(0.749999999999973,-55.08000002,-134.362052670054));
#175606=CARTESIAN_POINT('Origin',(1.24999999999997,-55.08000002,-134.362052670054));
#175607=CARTESIAN_POINT('',(0.749999999999973,-55.08000002,-97.7195882395211));
#175608=CARTESIAN_POINT('Ctrl Pts',(1.24999999999997,-54.58000002,-134.362052670054));
#175609=CARTESIAN_POINT('Ctrl Pts',(0.749999999999966,-54.5800000199999,
-134.362052670054));
#175610=CARTESIAN_POINT('Ctrl Pts',(0.749999999999973,-55.08000002,-134.362052670054));
#175611=CARTESIAN_POINT('Ctrl Pts',(1.24580493030994,-54.58000002,-135.093949837831));
#175612=CARTESIAN_POINT('Ctrl Pts',(0.750000000006796,-54.5841777042435,
-135.09091556402));
#175613=CARTESIAN_POINT('Ctrl Pts',(0.749999999999973,-55.0800000255278,
-135.020977206459));
#175614=CARTESIAN_POINT('Ctrl Pts',(1.24129514745974,-54.7377489917927,
-135.812422632741));
#175615=CARTESIAN_POINT('Ctrl Pts',(0.749999999993926,-54.7449249516581,
-135.807520949259));
#175616=CARTESIAN_POINT('Ctrl Pts',(0.749999999999973,-55.2219738253108,
-135.667845593964));
#175617=CARTESIAN_POINT('Ctrl Pts',(1.23668893165479,-55.0504165218146,
-136.482360813851));
#175618=CARTESIAN_POINT('Ctrl Pts',(0.74999999999998,-55.0621625368994,
-136.476881192513));
#175619=CARTESIAN_POINT('Ctrl Pts',(0.749999999999973,-55.5033748716332,
-136.27105168298));
#175620=CARTESIAN_POINT('',(0.749999999999973,-55.5033748716332,-136.27105168298));
#175621=CARTESIAN_POINT('Origin',(1.24999999999997,-55.5033748716332,-136.27105168298));
#175622=CARTESIAN_POINT('Origin',(0.749999999999973,-61.7710312681108,-133.877753475455));
#175623=CARTESIAN_POINT('Ctrl Pts',(0.749999999999965,-71.813687061541,
-171.237717270032));
#175624=CARTESIAN_POINT('Ctrl Pts',(0.749999999999976,-71.3691907154172,
-171.445036077089));
#175625=CARTESIAN_POINT('Ctrl Pts',(1.24037635835043,-71.360635368318,-171.449026400902));
#175626=CARTESIAN_POINT('Ctrl Pts',(0.749999999999967,-66.3773023734559,
-159.58198200727));
#175627=CARTESIAN_POINT('Ctrl Pts',(0.749999999778459,-65.9383759687714,
-159.799181671811));
#175628=CARTESIAN_POINT('Ctrl Pts',(1.23948769887611,-65.9242696435089,
-159.793291324051));
#175629=CARTESIAN_POINT('Ctrl Pts',(0.74999999999997,-60.9406796476674,
-147.926357767621));
#175630=CARTESIAN_POINT('Ctrl Pts',(0.749999999843541,-60.5069208340151,
-148.152089356292));
#175631=CARTESIAN_POINT('Ctrl Pts',(1.23838899982829,-60.4876714538986,
-148.137667147083));
#175632=CARTESIAN_POINT('Ctrl Pts',(0.749999999999973,-55.5033748716332,
-136.27105168298));
#175633=CARTESIAN_POINT('Ctrl Pts',(0.749999999999973,-55.0621625368995,
-136.476881192513));
#175634=CARTESIAN_POINT('Ctrl Pts',(1.23668893165476,-55.0504165218146,
-136.482360813851));
#175635=CARTESIAN_POINT('',(0.749999999999965,-71.813687061541,-171.237717270032));
#175636=CARTESIAN_POINT('',(1.24037635835043,-71.360635368318,-171.449026400902));
#175637=CARTESIAN_POINT('Origin',(1.24999999999996,-71.813687061541,-171.237717270032));
#175638=CARTESIAN_POINT('Ctrl Pts',(1.23668893165476,-55.0504165218146,
-136.482360813851));
#175639=CARTESIAN_POINT('Ctrl Pts',(1.23673299366641,-55.1913381585796,
-136.784440607054));
#175640=CARTESIAN_POINT('Ctrl Pts',(1.23677661819369,-55.3322593149882,
-137.08652062441));
#175641=CARTESIAN_POINT('Ctrl Pts',(1.23699261729668,-56.0368627647092,
-138.596921799561));
#175642=CARTESIAN_POINT('Ctrl Pts',(1.23715863033152,-56.6005380707885,
-139.805246217854));
#175643=CARTESIAN_POINT('Ctrl Pts',(1.23731859936897,-57.1642067307399,
-141.01357373723));
#175644=CARTESIAN_POINT('Ctrl Pts',(1.23795847551899,-59.4188813711729,
-145.84688381608));
#175645=CARTESIAN_POINT('Ctrl Pts',(1.23850317159002,-61.6734513223852,
-150.68024274455));
#175646=CARTESIAN_POINT('Ctrl Pts',(1.23898586311735,-63.927952799307,-155.513633616344));
#175647=CARTESIAN_POINT('Ctrl Pts',(1.23951632777425,-66.4055876545563,
-160.825396689281));
#175648=CARTESIAN_POINT('Ctrl Pts',(1.23997137264739,-68.8831392394364,
-166.137198611174));
#175649=CARTESIAN_POINT('Ctrl Pts',(1.24037635835043,-71.360635368318,-171.449026400902));
#175650=CARTESIAN_POINT('Ctrl Pts',(0.749999999999965,-71.813687061541,
-171.237717270032));
#175651=CARTESIAN_POINT('Ctrl Pts',(0.749999999999967,-66.3773023734559,
-159.58198200727));
#175652=CARTESIAN_POINT('Ctrl Pts',(0.74999999999997,-60.9406796476674,
-147.926357767621));
#175653=CARTESIAN_POINT('Ctrl Pts',(0.749999999999973,-55.5033748716332,
-136.27105168298));
#175654=CARTESIAN_POINT('Ctrl Pts',(0.749999999999971,-55.5033748716332,
-95.7875912885257));
#175655=CARTESIAN_POINT('Ctrl Pts',(0.749999999999964,-55.0621625368994,
-95.581761778993));
#175656=CARTESIAN_POINT('Ctrl Pts',(1.23668893165476,-55.0504165218147,
-95.5762821576554));
#175657=CARTESIAN_POINT('Ctrl Pts',(0.749999999999969,-60.9031648374056,
-84.2127012585751));
#175658=CARTESIAN_POINT('Ctrl Pts',(0.750000000106769,-60.4692939396047,
-83.9872370540609));
#175659=CARTESIAN_POINT('Ctrl Pts',(1.23837727019305,-60.4501569855996,
-84.0013918846235));
#175660=CARTESIAN_POINT('Ctrl Pts',(0.749999999999967,-66.3022815738571,
-72.6374971882577));
#175661=CARTESIAN_POINT('Ctrl Pts',(0.749999999981978,-65.8633206076967,
-72.4204079747872));
#175662=CARTESIAN_POINT('Ctrl Pts',(1.23947201783252,-65.8492492116834,
-72.4261878753526));
#175663=CARTESIAN_POINT('Ctrl Pts',(0.749999999999965,-71.701161634982,
-61.062182729971));
#175664=CARTESIAN_POINT('Ctrl Pts',(0.749999999999965,-71.2566817467536,
-60.8548714197835));
#175665=CARTESIAN_POINT('Ctrl Pts',(1.24035792914739,-71.2481103336038,
-60.8508735991007));
#175666=CARTESIAN_POINT('',(1.24035792914739,-71.2481103336038,-60.8508735991007));
#175667=CARTESIAN_POINT('Ctrl Pts',(1.24035792914739,-71.2481103336038,
-60.8508735991007));
#175668=CARTESIAN_POINT('Ctrl Pts',(1.24033480878609,-71.1072117831156,
-61.1529641634137));
#175669=CARTESIAN_POINT('Ctrl Pts',(1.24031152212174,-70.9663130484708,
-61.4550546418214));
#175670=CARTESIAN_POINT('Ctrl Pts',(1.24019423907957,-70.2618184344542,
-62.9655065950025));
#175671=CARTESIAN_POINT('Ctrl Pts',(1.2400976958218,-69.6982197351968,-64.1738667543558));
#175672=CARTESIAN_POINT('Ctrl Pts',(1.23999818500278,-69.1346177525067,
-65.3822253820002));
#175673=CARTESIAN_POINT('Ctrl Pts',(1.23960014172664,-66.8802098214716,
-70.2156598931668));
#175674=CARTESIAN_POINT('Ctrl Pts',(1.23915545083688,-64.6257502610154,
-75.0490703206921));
#175675=CARTESIAN_POINT('Ctrl Pts',(1.23864216610312,-62.3712150282457,
-79.8824454429464));
#175676=CARTESIAN_POINT('Ctrl Pts',(1.23808662039688,-59.9310540692955,
-85.1137734354556));
#175677=CARTESIAN_POINT('Ctrl Pts',(1.23745196892516,-57.4908058054248,
-90.3450606997508));
#175678=CARTESIAN_POINT('Ctrl Pts',(1.23668893165476,-55.0504165218147,
-95.5762821576554));
#175679=CARTESIAN_POINT('',(0.749999999999965,-71.701161634982,-61.0621827299711));
#175680=CARTESIAN_POINT('Origin',(1.24999999999996,-71.701161634982,-61.0621827299711));
#175681=CARTESIAN_POINT('Ctrl Pts',(0.749999999999971,-55.5033748716332,
-95.7875912885257));
#175682=CARTESIAN_POINT('Ctrl Pts',(0.749999999999969,-60.9031648374056,
-84.2127012585751));
#175683=CARTESIAN_POINT('Ctrl Pts',(0.749999999999967,-66.3022815738571,
-72.6374971882577));
#175684=CARTESIAN_POINT('Ctrl Pts',(0.749999999999965,-71.701161634982,
-61.062182729971));
#175685=CARTESIAN_POINT('Origin',(41.5,-73.08000002,-177.34995));
#175686=CARTESIAN_POINT('',(24.2,-66.7760495265873,-177.34995));
#175687=CARTESIAN_POINT('',(24.2,-73.08000002,-177.34995));
#175688=CARTESIAN_POINT('',(24.7,-66.5483734731532,-177.34995));
#175689=CARTESIAN_POINT('Origin',(0.,-12.9675000200281,-177.34995));
#175690=CARTESIAN_POINT('',(24.7,-73.08000002,-177.34995));
#175691=CARTESIAN_POINT('Origin',(24.7,-73.08000002,-176.84995));
#175692=CARTESIAN_POINT('',(25.0407404589729,-66.228934721057,-177.2158679411));
#175693=CARTESIAN_POINT('Ctrl Pts',(24.7,-66.5483734731532,-177.34995));
#175694=CARTESIAN_POINT('Ctrl Pts',(24.7151484196587,-66.5344070727695,
-177.34995));
#175695=CARTESIAN_POINT('Ctrl Pts',(24.7294276217104,-66.5212071123009,
-177.349259041047));
#175696=CARTESIAN_POINT('Ctrl Pts',(24.7428260025297,-66.5087976049832,
-177.348101171356));
#175697=CARTESIAN_POINT('Ctrl Pts',(24.7495926258282,-66.5025303953502,
-177.347516409053));
#175698=CARTESIAN_POINT('Ctrl Pts',(24.7561350473995,-66.4964643177492,
-177.346811961198));
#175699=CARTESIAN_POINT('Ctrl Pts',(24.7624541748984,-66.4905999359657,
-177.346013195118));
#175700=CARTESIAN_POINT('Ctrl Pts',(24.7782079605574,-66.4759798458257,
-177.3440218459));
#175701=CARTESIAN_POINT('Ctrl Pts',(24.7925691181153,-66.4626181429203,
-177.341448439213));
#175702=CARTESIAN_POINT('Ctrl Pts',(24.805519745065,-66.4505491735357,-177.338647136582));
#175703=CARTESIAN_POINT('Ctrl Pts',(24.8080497717743,-66.4481913869192,
-177.338099875781));
#175704=CARTESIAN_POINT('Ctrl Pts',(24.8105259039867,-66.4458829797902,
-177.337543769072));
#175705=CARTESIAN_POINT('Ctrl Pts',(24.812948010595,-66.4436241853332,-177.336981231575));
#175706=CARTESIAN_POINT('Ctrl Pts',(24.8245684958003,-66.4327872190828,
-177.334282358356));
#175707=CARTESIAN_POINT('Ctrl Pts',(24.8349638344589,-66.4230751742553,
-177.3314348709));
#175708=CARTESIAN_POINT('Ctrl Pts',(24.8441561790726,-66.4144557330666,
-177.3286658351));
#175709=CARTESIAN_POINT('Ctrl Pts',(24.8466873935909,-66.4120822738902,
-177.327903350238));
#175710=CARTESIAN_POINT('Ctrl Pts',(24.8491274673187,-66.4097915816494,
-177.327146526476));
#175711=CARTESIAN_POINT('Ctrl Pts',(24.8514769953736,-66.407582837082,-177.326399450407));
#175712=CARTESIAN_POINT('Ctrl Pts',(24.8569180259311,-66.4024678325347,
-177.324669373718));
#175713=CARTESIAN_POINT('Ctrl Pts',(24.8618700924437,-66.3977843689127,
-177.322993320373));
#175714=CARTESIAN_POINT('Ctrl Pts',(24.8663521453577,-66.3935491356442,
-177.321412257989));
#175715=CARTESIAN_POINT('Ctrl Pts',(24.8685931718147,-66.39143151901,-177.320621726797));
#175716=CARTESIAN_POINT('Ctrl Pts',(24.8707166368713,-66.3894259510714,
-177.319854809349));
#175717=CARTESIAN_POINT('Ctrl Pts',(24.8727240319675,-66.3875324318892,
-177.319116074401));
#175718=CARTESIAN_POINT('Ctrl Pts',(24.8737277295157,-66.3865856722982,
-177.318746706927));
#175719=CARTESIAN_POINT('Ctrl Pts',(24.8747024069947,-66.3856669248983,
-177.318384377616));
#175720=CARTESIAN_POINT('Ctrl Pts',(24.8756482370288,-66.3847761897005,
-177.318029612383));
#175721=CARTESIAN_POINT('Ctrl Pts',(24.8761211520459,-66.3843308221016,
-177.317852229766));
#175722=CARTESIAN_POINT('Ctrl Pts',(24.8762952359649,-66.3841660105406,
-177.317786544152));
#175723=CARTESIAN_POINT('Ctrl Pts',(24.8766081401647,-66.3838714254534,
-177.317668448636));
#175724=CARTESIAN_POINT('Ctrl Pts',(24.8769210443645,-66.3835768403661,
-177.31755035312));
#175725=CARTESIAN_POINT('Ctrl Pts',(24.8773729678627,-66.3831524816923,
-177.31738036387));
#175726=CARTESIAN_POINT('Ctrl Pts',(24.8783993497236,-66.3821880207246,
-177.316988504263));
#175727=CARTESIAN_POINT('Ctrl Pts',(24.8948214594981,-66.3667566452422,
-177.310718750545));
#175728=CARTESIAN_POINT('Ctrl Pts',(24.9105266151752,-66.351990337037,-177.303734637161));
#175729=CARTESIAN_POINT('Ctrl Pts',(24.9255112984692,-66.3378890967839,
-177.296168963569));
#175730=CARTESIAN_POINT('Ctrl Pts',(24.9431116330293,-66.3213264146572,
-177.287282663888));
#175731=CARTESIAN_POINT('Ctrl Pts',(24.959731749144,-66.3056662947302,-177.277584719044));
#175732=CARTESIAN_POINT('Ctrl Pts',(24.9753358287529,-66.2909341784927,
-177.267297394451));
#175733=CARTESIAN_POINT('Ctrl Pts',(24.9914404771145,-66.2757294655218,
-177.256680059157));
#175734=CARTESIAN_POINT('Ctrl Pts',(25.0064629606483,-66.2615131607872,
-177.245435170344));
#175735=CARTESIAN_POINT('Ctrl Pts',(25.0204053672138,-66.2482764016167,
-177.233798655926));
#175736=CARTESIAN_POINT('Ctrl Pts',(25.0274581624319,-66.241580559594,-177.227912301023));
#175737=CARTESIAN_POINT('Ctrl Pts',(25.0342352192367,-66.2351348025665,
-177.221925578959));
#175738=CARTESIAN_POINT('Ctrl Pts',(25.0407404589728,-66.228934721057,-177.2158679411));
#175739=CARTESIAN_POINT('',(25.2,-66.1031295107182,-176.84995));
#175740=CARTESIAN_POINT('Ctrl Pts',(25.0407404589729,-66.228934721057,-177.2158679411));
#175741=CARTESIAN_POINT('Ctrl Pts',(25.0847395070529,-66.1869996509441,
-177.174896307427));
#175742=CARTESIAN_POINT('Ctrl Pts',(25.1244954390544,-66.1555483483594,
-177.12286866857));
#175743=CARTESIAN_POINT('Ctrl Pts',(25.1822082377855,-66.1136132782465,
-176.998799564474));
#175744=CARTESIAN_POINT('Ctrl Pts',(25.2,-66.1031295107183,-176.926663869319));
#175745=CARTESIAN_POINT('Ctrl Pts',(25.2,-66.1031295107182,-176.84995));
#175746=CARTESIAN_POINT('',(25.2,67.7009572055632,-176.84995));
#175747=CARTESIAN_POINT('Ctrl Pts',(26.2379083085631,-65.1635541261514,
-171.346593949865));
#175748=CARTESIAN_POINT('Ctrl Pts',(26.188244627337,-65.494631983645,-171.628250848894));
#175749=CARTESIAN_POINT('Ctrl Pts',(26.0510006858591,-65.5133697788369,
-172.043246117731));
#175750=CARTESIAN_POINT('Ctrl Pts',(25.9971706168399,-65.2375572433357,
-171.303343061545));
#175751=CARTESIAN_POINT('Ctrl Pts',(25.9737737091347,-65.5150103099346,
-171.582081143282));
#175752=CARTESIAN_POINT('Ctrl Pts',(25.8585042848855,-65.5396766827938,
-171.956814849412));
#175753=CARTESIAN_POINT('Ctrl Pts',(25.7542731404381,-65.3249121430513,
-171.265064732433));
#175754=CARTESIAN_POINT('Ctrl Pts',(25.7517856586292,-65.5594176286463,
-171.534269559735));
#175755=CARTESIAN_POINT('Ctrl Pts',(25.6686777183217,-65.5842439051372,
-171.880177321686));
#175756=CARTESIAN_POINT('Ctrl Pts',(25.5048932192108,-65.4282717079069,
-171.24324485235));
#175757=CARTESIAN_POINT('Ctrl Pts',(25.5297574101185,-65.6321545000982,
-171.506780891573));
#175758=CARTESIAN_POINT('Ctrl Pts',(25.4789337502923,-65.6496774707413,
-171.836549850108));
#175759=CARTESIAN_POINT('Ctrl Pts',(26.0394480946395,-65.5149709682656,
-172.038055421481));
#175760=CARTESIAN_POINT('Ctrl Pts',(25.9934781597493,-65.5214316212864,
-172.017499691038));
#175761=CARTESIAN_POINT('Ctrl Pts',(25.9500895256781,-65.5286146559866,
-171.9986631729));
#175762=CARTESIAN_POINT('Ctrl Pts',(25.8888633443777,-65.5399834876779,
-171.97298721415));
#175763=CARTESIAN_POINT('Ctrl Pts',(25.8592138997392,-65.5458173722782,
-171.960793939389));
#175764=CARTESIAN_POINT('Ctrl Pts',(25.8310028817436,-65.5517918933206,
-171.94956772155));
#175765=CARTESIAN_POINT('Ctrl Pts',(25.8125141728673,-65.5557974424197,
-171.942298477862));
#175766=CARTESIAN_POINT('Ctrl Pts',(25.8054251757784,-65.557359537272,-171.93953600361));
#175767=CARTESIAN_POINT('Ctrl Pts',(25.7071248585263,-65.5796157721532,
-171.901876249447));
#175768=CARTESIAN_POINT('Ctrl Pts',(25.6251638390528,-65.6022780898996,
-171.874763931484));
#175769=CARTESIAN_POINT('Ctrl Pts',(25.5486065204936,-65.6266003779646,
-171.854014632593));
#175770=CARTESIAN_POINT('Ctrl Pts',(25.54864668864,-65.6265809455192,-176.826359947228));
#175771=CARTESIAN_POINT('Ctrl Pts',(25.1997818129229,-65.7371542671639,
-176.835443989308));
#175772=CARTESIAN_POINT('Ctrl Pts',(25.1998556150807,-66.1032295031672,
-176.838160112216));
#175773=CARTESIAN_POINT('Ctrl Pts',(25.5529523483652,-65.6253023760353,
-176.972546990942));
#175774=CARTESIAN_POINT('Ctrl Pts',(25.2023635504854,-65.7357920520888,
-176.925322463907));
#175775=CARTESIAN_POINT('Ctrl Pts',(25.2016488868717,-66.1021639228633,
-176.911221791747));
#175776=CARTESIAN_POINT('Ctrl Pts',(25.5170441055793,-65.6358444287873,
-177.121198634883));
#175777=CARTESIAN_POINT('Ctrl Pts',(25.1809363031095,-65.747065159673,-177.017221417402));
#175778=CARTESIAN_POINT('Ctrl Pts',(25.1866937732675,-66.1109497354307,
-176.985515400943));
#175779=CARTESIAN_POINT('Ctrl Pts',(25.3765977400936,-65.6860676120866,
-177.38644456451));
#175780=CARTESIAN_POINT('Ctrl Pts',(25.0919963386827,-65.7962596108139,
-177.18144271446));
#175781=CARTESIAN_POINT('Ctrl Pts',(25.1281992647199,-66.1528013266155,
-177.118080932736));
#175782=CARTESIAN_POINT('Ctrl Pts',(25.2719907766206,-65.7262135374441,
-177.504397480335));
#175783=CARTESIAN_POINT('Ctrl Pts',(25.0235400714211,-65.8346526306424,
-177.25498331877));
#175784=CARTESIAN_POINT('Ctrl Pts',(25.0846190279164,-66.1862656195983,
-177.177043188278));
#175785=CARTESIAN_POINT('Ctrl Pts',(25.1465824121021,-65.7870908289106,
-177.597292784559));
#175786=CARTESIAN_POINT('Ctrl Pts',(24.9378206840703,-65.8881436940036,
-177.307601476654));
#175787=CARTESIAN_POINT('Ctrl Pts',(25.0323995999485,-66.2369758560726,
-177.223456543475));
#175788=CARTESIAN_POINT('',(25.166383622031,-65.7775666303703,-177.581785882201));
#175789=CARTESIAN_POINT('Origin',(25.3814809179458,-66.228934721057,-177.581785882201));
#175790=CARTESIAN_POINT('',(25.548606520496,-65.6266003779638,-176.84995));
#175791=CARTESIAN_POINT('Ctrl Pts',(25.548606520496,-65.6266003779638,-176.84995));
#175792=CARTESIAN_POINT('Ctrl Pts',(25.5483880050666,-65.6266698003955,
-176.923301524269));
#175793=CARTESIAN_POINT('Ctrl Pts',(25.5391662663674,-65.6295529063921,
-176.994603239542));
#175794=CARTESIAN_POINT('Ctrl Pts',(25.5119555175164,-65.6384880995831,
-177.098481098957));
#175795=CARTESIAN_POINT('Ctrl Pts',(25.5006581261773,-65.6422428632939,
-177.132594599846));
#175796=CARTESIAN_POINT('Ctrl Pts',(25.4804126501714,-65.6491589363909,
-177.182996172806));
#175797=CARTESIAN_POINT('Ctrl Pts',(25.4731144514682,-65.6516787676171,
-177.199668584064));
#175798=CARTESIAN_POINT('Ctrl Pts',(25.4574280034951,-65.6571730351468,
-177.232757180455));
#175799=CARTESIAN_POINT('Ctrl Pts',(25.4484827026432,-65.6603481655915,
-177.250189665967));
#175800=CARTESIAN_POINT('Ctrl Pts',(25.3731469612502,-65.6874900466836,
-177.387635611196));
#175801=CARTESIAN_POINT('Ctrl Pts',(25.2806998533548,-65.7230897793383,
-177.49307709271));
#175802=CARTESIAN_POINT('Ctrl Pts',(25.166383622031,-65.7775666303703,-177.581785882201));
#175803=CARTESIAN_POINT('Origin',(25.7,-66.1031295107182,-176.84995));
#175804=CARTESIAN_POINT('Origin',(25.7,-66.1031295107182,-179.64995));
#175805=CARTESIAN_POINT('',(25.548606520496,-65.6266003779638,-179.64995));
#175806=CARTESIAN_POINT('',(25.2,-66.1031295107182,-171.799329694116));
#175807=CARTESIAN_POINT('Ctrl Pts',(0.749999999999965,-71.9542570083556,
-171.871644662643));
#175808=CARTESIAN_POINT('Ctrl Pts',(0.749999999999965,-71.4647403528508,
-171.871644662643));
#175809=CARTESIAN_POINT('Ctrl Pts',(1.23940677966098,-71.4543692372681,
-171.871644662643));
#175810=CARTESIAN_POINT('Ctrl Pts',(0.749999999999965,-71.9542569918424,
-171.652832243085));
#175811=CARTESIAN_POINT('Ctrl Pts',(0.75,-71.4647403416089,-171.724250912112));
#175812=CARTESIAN_POINT('Ctrl Pts',(1.23940678000784,-71.4543692372607,
-171.725769781663));
#175813=CARTESIAN_POINT('Ctrl Pts',(0.749999999999965,-71.9071171402653,
-171.43803354201));
#175814=CARTESIAN_POINT('Ctrl Pts',(0.749999999994888,-71.4326041940841,
-171.579497326419));
#175815=CARTESIAN_POINT('Ctrl Pts',(1.23973038817724,-71.4229357713421,
-171.582570495172));
#175816=CARTESIAN_POINT('Ctrl Pts',(0.749999999999965,-71.813687061541,
-171.237717270032));
#175817=CARTESIAN_POINT('Ctrl Pts',(0.749999999999965,-71.3691907154173,
-171.445036077089));
#175818=CARTESIAN_POINT('Ctrl Pts',(1.24037635835043,-71.360635368318,-171.449026400902));
#175819=CARTESIAN_POINT('',(0.749999999999965,-71.9542570083556,-171.871644662643));
#175820=CARTESIAN_POINT('',(1.23940677966098,-71.4543692372681,-171.871644662643));
#175821=CARTESIAN_POINT('Origin',(1.24999999999996,-71.9542570083556,-171.871644662643));
#175822=CARTESIAN_POINT('Origin',(1.25479963396822,-69.9697011186647,-171.979266830671));
#175823=CARTESIAN_POINT('Origin',(0.749999999999965,-69.7273331732481,-172.033160909053));
#175824=CARTESIAN_POINT('Origin',(0.,-12.9675000200281,-171.64995));
#175825=CARTESIAN_POINT('Origin',(0.,-12.9675000200281,-171.449026400902));
#175826=CARTESIAN_POINT('Ctrl Pts',(7.4,-71.4211246238516,-171.237717270032));
#175827=CARTESIAN_POINT('Ctrl Pts',(7.39999999999995,-70.9175980522952,
-171.474145745141));
#175828=CARTESIAN_POINT('Ctrl Pts',(6.84687749809456,-70.9710952348089,
-171.449026400902));
#175829=CARTESIAN_POINT('Ctrl Pts',(7.4,-71.5141496698322,-171.435834655863));
#175830=CARTESIAN_POINT('Ctrl Pts',(7.40000000000424,-70.9726288200743,
-171.600718024433));
#175831=CARTESIAN_POINT('Ctrl Pts',(6.84335093752903,-71.0335272731666,
-171.581102626116));
#175832=CARTESIAN_POINT('Ctrl Pts',(7.4,-71.5626363329153,-171.650517772678));
#175833=CARTESIAN_POINT('Ctrl Pts',(7.39999999999997,-71.0003029730699,
-171.734045906264));
#175834=CARTESIAN_POINT('Ctrl Pts',(6.84152542419482,-71.0660673850682,
-171.724228262147));
#175835=CARTESIAN_POINT('Ctrl Pts',(7.4,-71.5626363369615,-171.871644662643));
#175836=CARTESIAN_POINT('Ctrl Pts',(7.39999999999996,-71.0003029749948,
-171.871644662643));
#175837=CARTESIAN_POINT('Ctrl Pts',(6.84152542372878,-71.066067385123,-171.871644662643));
#175838=CARTESIAN_POINT('',(6.84152542372877,-71.066067385123,-171.871644662643));
#175839=CARTESIAN_POINT('',(7.4,-71.5626363369615,-171.871644662643));
#175840=CARTESIAN_POINT('Origin',(6.9,-71.5626363369615,-171.871644662643));
#175841=CARTESIAN_POINT('Origin',(7.4,-69.3873379576789,-172.017654079519));
#175842=CARTESIAN_POINT('Origin',(6.92387916107346,-69.6079656440742,-171.968783295101));
#175843=CARTESIAN_POINT('Ctrl Pts',(7.4,-72.58000002,-174.471034982976));
#175844=CARTESIAN_POINT('Ctrl Pts',(7.39999999999995,-73.0800000199999,
-174.471034982977));
#175845=CARTESIAN_POINT('Ctrl Pts',(7.9,-73.08000002,-174.471034982976));
#175846=CARTESIAN_POINT('Ctrl Pts',(7.4,-72.5800000132661,-174.719615315523));
#175847=CARTESIAN_POINT('Ctrl Pts',(7.39999999999984,-73.081997137201,-174.769844466954));
#175848=CARTESIAN_POINT('Ctrl Pts',(7.90199316078775,-73.08000002,-174.769251346187));
#175849=CARTESIAN_POINT('Ctrl Pts',(7.4,-72.5437711321103,-174.962127460747));
#175850=CARTESIAN_POINT('Ctrl Pts',(7.39999999999996,-73.040326257465,-175.061328113453));
#175851=CARTESIAN_POINT('Ctrl Pts',(7.90394076068631,-73.0365253516511,
-175.060187649793));
#175852=CARTESIAN_POINT('Ctrl Pts',(7.4,-72.4360935067573,-175.316738645421));
#175853=CARTESIAN_POINT('Ctrl Pts',(7.39999999999996,-72.9137734508192,
-175.488022550208));
#175854=CARTESIAN_POINT('Ctrl Pts',(7.90679252703161,-72.9073122055494,
-175.485606387024));
#175855=CARTESIAN_POINT('Ctrl Pts',(7.4,-72.3910774582401,-175.433049854657));
#175856=CARTESIAN_POINT('Ctrl Pts',(7.39999999999998,-72.8605108035235,
-175.628237972001));
#175857=CARTESIAN_POINT('Ctrl Pts',(7.90772857701081,-72.8532929465542,
-175.625142180141));
#175858=CARTESIAN_POINT('Ctrl Pts',(7.4,-72.2858284501893,-175.654944429739));
#175859=CARTESIAN_POINT('Ctrl Pts',(7.39999999999997,-72.7355139213092,
-175.896009980972));
#175860=CARTESIAN_POINT('Ctrl Pts',(7.90951546143904,-72.7269941355612,
-175.891343758978));
#175861=CARTESIAN_POINT('Ctrl Pts',(7.4,-72.2253270246874,-175.761526340889));
#175862=CARTESIAN_POINT('Ctrl Pts',(7.39999999999901,-72.6634371311262,
-176.024735407069));
#175863=CARTESIAN_POINT('Ctrl Pts',(7.9103743244834,-72.6543924247951,-176.019207476496));
#175864=CARTESIAN_POINT('Ctrl Pts',(7.4,-72.0884932351423,-175.96591668417));
#175865=CARTESIAN_POINT('Ctrl Pts',(7.40000000000093,-72.5000420015558,
-176.271831635453));
#175866=CARTESIAN_POINT('Ctrl Pts',(7.9120222658245,-72.4901918790006,-176.264409528534));
#175867=CARTESIAN_POINT('Ctrl Pts',(7.4,-72.0114432535103,-176.064396375895));
#175868=CARTESIAN_POINT('Ctrl Pts',(7.39999999999755,-72.4078441030974,
-176.390977561524));
#175869=CARTESIAN_POINT('Ctrl Pts',(7.91281676658892,-72.3977319011293,
-176.382553154925));
#175870=CARTESIAN_POINT('Ctrl Pts',(7.4,-71.8455797798041,-176.246702589259));
#175871=CARTESIAN_POINT('Ctrl Pts',(7.40000000000237,-72.2090331198025,
-176.611745838634));
#175872=CARTESIAN_POINT('Ctrl Pts',(7.91428825612723,-72.198695730848,-176.6012613201));
#175873=CARTESIAN_POINT('Ctrl Pts',(7.4,-71.7565932593015,-176.331051292497));
#175874=CARTESIAN_POINT('Ctrl Pts',(7.40000000000137,-72.1022117673413,
-176.713954380549));
#175875=CARTESIAN_POINT('Ctrl Pts',(7.91496944868021,-72.0919119068452,
-176.702452310058));
#175876=CARTESIAN_POINT('Ctrl Pts',(7.4,-71.4717169212771,-176.56396241752));
#175877=CARTESIAN_POINT('Ctrl Pts',(7.39999999999722,-71.7595719221786,
-176.996603847265));
#175878=CARTESIAN_POINT('Ctrl Pts',(7.91685114292327,-71.7500603021656,
-176.981869807169));
#175879=CARTESIAN_POINT('Ctrl Pts',(7.4,-71.2547332556153,-176.693097313134));
#175880=CARTESIAN_POINT('Ctrl Pts',(7.39999999999668,-71.4982684775377,
-177.153312936568));
#175881=CARTESIAN_POINT('Ctrl Pts',(7.91789548135802,-71.4896799957509,
-177.136789521634));
#175882=CARTESIAN_POINT('Ctrl Pts',(7.4,-71.028920068719,-176.785817298486));
#175883=CARTESIAN_POINT('Ctrl Pts',(7.39999999999996,-71.2260554869631,
-177.265927135801));
#175884=CARTESIAN_POINT('Ctrl Pts',(7.91864558019502,-71.2187040784628,
-177.248023282853));
#175885=CARTESIAN_POINT('',(7.40000000143918,-71.5626363369614,-176.485569595296));
#175886=CARTESIAN_POINT('Ctrl Pts',(7.40000000575672,-71.5626363369612,
-176.485569595296));
#175887=CARTESIAN_POINT('Ctrl Pts',(7.39999999964314,-71.5963334703268,
-176.460729295267));
#175888=CARTESIAN_POINT('Ctrl Pts',(7.40000000050213,-71.6293602055438,
-176.435105116127));
#175889=CARTESIAN_POINT('Ctrl Pts',(7.40000000080687,-71.6616524595397,
-176.408710325206));
#175890=CARTESIAN_POINT('Ctrl Pts',(7.40000000085713,-71.6669782225453,
-176.404357194544));
#175891=CARTESIAN_POINT('Ctrl Pts',(7.40000000093686,-71.6722864874059,
-176.399982537289));
#175892=CARTESIAN_POINT('Ctrl Pts',(7.40000000105475,-71.6775773354997,
-176.395586157876));
#175893=CARTESIAN_POINT('Ctrl Pts',(7.40000000288459,-71.759704119665,-176.327343695265));
#175894=CARTESIAN_POINT('Ctrl Pts',(7.40000000086288,-71.8372393620171,
-176.253983607117));
#175895=CARTESIAN_POINT('Ctrl Pts',(7.40000000055521,-71.9102228395816,
-176.175469994321));
#175896=CARTESIAN_POINT('Ctrl Pts',(7.40000000052935,-71.9163567428985,
-176.168871310263));
#175897=CARTESIAN_POINT('Ctrl Pts',(7.40000000051231,-71.9224585008204,
-176.162236193809));
#175898=CARTESIAN_POINT('Ctrl Pts',(7.40000000050508,-71.9285281400417,
-176.15556460665));
#175899=CARTESIAN_POINT('Ctrl Pts',(7.40000000048088,-71.9488281698803,
-176.133251349886));
#175900=CARTESIAN_POINT('Ctrl Pts',(7.4000000005302,-71.9687792955913,-176.110498872159));
#175901=CARTESIAN_POINT('Ctrl Pts',(7.40000000090086,-71.9883433756989,
-176.087359845977));
#175902=CARTESIAN_POINT('Ctrl Pts',(7.40000000204431,-72.0486965657351,
-176.01597831223));
#175903=CARTESIAN_POINT('Ctrl Pts',(7.40000000174205,-72.1052822109679,
-175.940916275219));
#175904=CARTESIAN_POINT('Ctrl Pts',(7.40000000104438,-72.1569369843104,
-175.863739490819));
#175905=CARTESIAN_POINT('Ctrl Pts',(7.40000000027758,-72.2137093550038,
-175.778916564894));
#175906=CARTESIAN_POINT('Ctrl Pts',(7.39999999999849,-72.2650200455803,
-175.691076839899));
#175907=CARTESIAN_POINT('Ctrl Pts',(7.40000000003311,-72.3109220293856,
-175.600232860702));
#175908=CARTESIAN_POINT('Ctrl Pts',(7.4000000000402,-72.3203292671906,-175.5816151269));
#175909=CARTESIAN_POINT('Ctrl Pts',(7.40000000005342,-72.3295088745487,
-175.562871130851));
#175910=CARTESIAN_POINT('Ctrl Pts',(7.40000000007737,-72.3384609015072,
-175.544000911756));
#175911=CARTESIAN_POINT('Ctrl Pts',(7.40000000021819,-72.3910932309574,
-175.433055804823));
#175912=CARTESIAN_POINT('Ctrl Pts',(7.4000000012263,-72.436127459958,-175.316747505601));
#175913=CARTESIAN_POINT('Ctrl Pts',(7.40000000110901,-72.4720179137164,
-175.198544593051));
#175914=CARTESIAN_POINT('Ctrl Pts',(7.40000000106034,-72.4869106518372,
-175.14949631315));
#175915=CARTESIAN_POINT('Ctrl Pts',(7.40000000071105,-72.5002693294562,
-175.100185099317));
#175916=CARTESIAN_POINT('Ctrl Pts',(7.4000000003472,-72.5120857612517,-175.050611983827));
#175917=CARTESIAN_POINT('Ctrl Pts',(7.39999999965227,-72.534654114155,-174.955931662031));
#175918=CARTESIAN_POINT('Ctrl Pts',(7.4,-72.5516373021817,-174.860293425931));
#175919=CARTESIAN_POINT('Ctrl Pts',(7.4,-72.5629735391251,-174.763699740561));
#175920=CARTESIAN_POINT('Ctrl Pts',(7.4,-72.5743097760684,-174.667106055192));
#175921=CARTESIAN_POINT('Ctrl Pts',(7.4,-72.58000002,-174.569557605373));
#175922=CARTESIAN_POINT('Ctrl Pts',(7.4,-72.58000002,-174.471034982976));
#175923=CARTESIAN_POINT('',(7.91859121655489,-71.2381488508947,-177.239961484012));
#175924=CARTESIAN_POINT('Ctrl Pts',(7.4,-71.5626363369615,-176.485569595297));
#175925=CARTESIAN_POINT('Ctrl Pts',(7.4,-71.5506036695784,-176.519632609605));
#175926=CARTESIAN_POINT('Ctrl Pts',(7.40124182377961,-71.5387437345536,
-176.553192135052));
#175927=CARTESIAN_POINT('Ctrl Pts',(7.40377535877835,-71.5271166640425,
-176.586019648744));
#175928=CARTESIAN_POINT('Ctrl Pts',(7.40622177366248,-71.5158894110653,
-176.617718329893));
#175929=CARTESIAN_POINT('Ctrl Pts',(7.40987259906279,-71.5048792758311,
-176.648734213767));
#175930=CARTESIAN_POINT('Ctrl Pts',(7.41473087025355,-71.494133681817,-176.678884073483));
#175931=CARTESIAN_POINT('Ctrl Pts',(7.41866902349833,-71.4854232178944,
-176.703323789425));
#175932=CARTESIAN_POINT('Ctrl Pts',(7.42339982845854,-71.4768864593179,
-176.727194803422));
#175933=CARTESIAN_POINT('Ctrl Pts',(7.42890359949814,-71.4685453034926,
-176.75041264347));
#175934=CARTESIAN_POINT('Ctrl Pts',(7.43039440453314,-71.4662859367761,
-176.756701653787));
#175935=CARTESIAN_POINT('Ctrl Pts',(7.43194146136298,-71.4640414204283,
-176.762941376912));
#175936=CARTESIAN_POINT('Ctrl Pts',(7.43354440994792,-71.4618116713854,
-176.769131638689));
#175937=CARTESIAN_POINT('Ctrl Pts',(7.4377989840509,-71.4558934325703,-176.785561939508));
#175938=CARTESIAN_POINT('Ctrl Pts',(7.44244689889008,-71.4500853619215,
-176.801621162751));
#175939=CARTESIAN_POINT('Ctrl Pts',(7.44746558592961,-71.4443873125637,
-176.817288504605));
#175940=CARTESIAN_POINT('Ctrl Pts',(7.45592268298431,-71.4347854075113,
-176.843689878032));
#175941=CARTESIAN_POINT('Ctrl Pts',(7.46543034530173,-71.4255017180002,
-176.868960780972));
#175942=CARTESIAN_POINT('Ctrl Pts',(7.47583467172322,-71.4165597639218,
-176.892953826141));
#175943=CARTESIAN_POINT('Ctrl Pts',(7.48331456949562,-71.4101311976041,
-176.91020295096));
#175944=CARTESIAN_POINT('Ctrl Pts',(7.49125715404826,-71.4038792424485,
-176.926792127842));
#175945=CARTESIAN_POINT('Ctrl Pts',(7.49959455240465,-71.3978116293706,
-176.942679207561));
#175946=CARTESIAN_POINT('Ctrl Pts',(7.50169522409967,-71.3962828475487,
-176.946682079591));
#175947=CARTESIAN_POINT('Ctrl Pts',(7.50382092027666,-71.3947657561162,
-176.950640434758));
#175948=CARTESIAN_POINT('Ctrl Pts',(7.50596959979478,-71.3932574848628,
-176.954554085486));
#175949=CARTESIAN_POINT('Ctrl Pts',(7.50734971529259,-71.39228870915,-176.957067857306));
#175950=CARTESIAN_POINT('Ctrl Pts',(7.50849831293203,-71.391492060449,-176.95913101286));
#175951=CARTESIAN_POINT('Ctrl Pts',(7.50987883023994,-71.3905463578264,
-176.96157741569));
#175952=CARTESIAN_POINT('Ctrl Pts',(7.5106476180218,-71.3900197113169,-176.962939777896));
#175953=CARTESIAN_POINT('Ctrl Pts',(7.51148881635629,-71.3894469329875,
-176.964420536038));
#175954=CARTESIAN_POINT('Ctrl Pts',(7.51248752482203,-71.3887735212086,
-176.966158828872));
#175955=CARTESIAN_POINT('Ctrl Pts',(7.52040526868911,-71.3834347239867,
-176.979939985129));
#175956=CARTESIAN_POINT('Ctrl Pts',(7.528724573393,-71.3781777648363,-176.993315121));
#175957=CARTESIAN_POINT('Ctrl Pts',(7.53742401159906,-71.3730105085842,
-177.006241431523));
#175958=CARTESIAN_POINT('Ctrl Pts',(7.55157063114754,-71.3646077581333,
-177.027261593147));
#175959=CARTESIAN_POINT('Ctrl Pts',(7.56677045080576,-71.3564218411025,
-177.047118964408));
#175960=CARTESIAN_POINT('Ctrl Pts',(7.58280101197635,-71.3485013029008,
-177.065623012365));
#175961=CARTESIAN_POINT('Ctrl Pts',(7.58472281489058,-71.3475517595108,
-177.067841346016));
#175962=CARTESIAN_POINT('Ctrl Pts',(7.58665653135238,-71.3466060208685,
-177.070040284832));
#175963=CARTESIAN_POINT('Ctrl Pts',(7.5886017583046,-71.3456641628206,-177.072219547107));
#175964=CARTESIAN_POINT('Ctrl Pts',(7.60267640683548,-71.338849368806,-177.087987553275));
#175965=CARTESIAN_POINT('Ctrl Pts',(7.61736717206938,-71.3322314016754,
-177.102738989088));
#175966=CARTESIAN_POINT('Ctrl Pts',(7.63254357701316,-71.3258225700846,
-177.11639818297));
#175967=CARTESIAN_POINT('Ctrl Pts',(7.64013177948506,-71.3226181542892,
-177.12322777991));
#175968=CARTESIAN_POINT('Ctrl Pts',(7.64784173532136,-71.3194674390364,
-177.129784166108));
#175969=CARTESIAN_POINT('Ctrl Pts',(7.6556568499062,-71.3163736401622,-177.13605865242));
#175970=CARTESIAN_POINT('Ctrl Pts',(7.65935939288764,-71.3149079005133,
-177.139031296646));
#175971=CARTESIAN_POINT('Ctrl Pts',(7.6628170835859,-71.3135596068012,-177.141730715413));
#175972=CARTESIAN_POINT('Ctrl Pts',(7.66640603380969,-71.3121789599471,
-177.144461325117));
#175973=CARTESIAN_POINT('Ctrl Pts',(7.66983434317808,-71.3108601106321,
-177.147069713154));
#175974=CARTESIAN_POINT('Ctrl Pts',(7.67338251641711,-71.309511712934,-177.149706742547));
#175975=CARTESIAN_POINT('Ctrl Pts',(7.67739913373759,-71.308009866984,-177.152597143897));
#175976=CARTESIAN_POINT('Ctrl Pts',(7.67805299354838,-71.307765383472,-177.153067668503));
#175977=CARTESIAN_POINT('Ctrl Pts',(7.67871931450839,-71.3075168498756,
-177.153544807822));
#175978=CARTESIAN_POINT('Ctrl Pts',(7.67939965845519,-71.3072637521496,
-177.154029406282));
#175979=CARTESIAN_POINT('Ctrl Pts',(7.68837037659409,-71.3039265160767,
-177.160419109932));
#175980=CARTESIAN_POINT('Ctrl Pts',(7.69748767629138,-71.3006476354715,
-177.166472905463));
#175981=CARTESIAN_POINT('Ctrl Pts',(7.70673174046216,-71.297430665461,-177.172175429854));
#175982=CARTESIAN_POINT('Ctrl Pts',(7.72768672414405,-71.2901382502603,
-177.185102244658));
#175983=CARTESIAN_POINT('Ctrl Pts',(7.74939099709486,-71.2831283244239,
-177.196256748911));
#175984=CARTESIAN_POINT('Ctrl Pts',(7.77148013541325,-71.2764641353456,
-177.205563508786));
#175985=CARTESIAN_POINT('Ctrl Pts',(7.79294215838971,-71.2699891440147,
-177.214606047767));
#175986=CARTESIAN_POINT('Ctrl Pts',(7.81476661214664,-71.2638406432925,
-177.221904234036));
#175987=CARTESIAN_POINT('Ctrl Pts',(7.83662991855142,-71.2580661408856,
-177.227435014853));
#175988=CARTESIAN_POINT('Ctrl Pts',(7.85770145362575,-71.2525007598884,
-177.232765500545));
#175989=CARTESIAN_POINT('Ctrl Pts',(7.8788084897248,-71.247282821352,-177.236454389783));
#175990=CARTESIAN_POINT('Ctrl Pts',(7.89968194537098,-71.2424439309288,
-177.238523807616));
#175991=CARTESIAN_POINT('Ctrl Pts',(7.90600864332505,-71.24097727401,-177.239151043555));
#175992=CARTESIAN_POINT('Ctrl Pts',(7.91231406191567,-71.2395453591647,
-177.239629801061));
#175993=CARTESIAN_POINT('Ctrl Pts',(7.91859121655422,-71.2381488509314,
-177.239961484007));
#175994=CARTESIAN_POINT('Ctrl Pts',(7.9,-73.08000002,-174.471034982976));
#175995=CARTESIAN_POINT('Ctrl Pts',(7.90029399716905,-73.080000019775,-174.515022787248));
#175996=CARTESIAN_POINT('Ctrl Pts',(7.90085674855018,-73.0803883548312,
-174.607717845982));
#175997=CARTESIAN_POINT('Ctrl Pts',(7.90228899981587,-73.0600424381335,
-174.824207987439));
#175998=CARTESIAN_POINT('Ctrl Pts',(7.90286592665474,-73.0495149637409,
-174.909313799419));
#175999=CARTESIAN_POINT('Ctrl Pts',(7.9038762253622,-73.0228545180863,-175.056228893897));
#176000=CARTESIAN_POINT('Ctrl Pts',(7.9042367222111,-73.0121368256507,-175.108399370711));
#176001=CARTESIAN_POINT('Ctrl Pts',(7.90480656268785,-72.9924911650618,
-175.191284311026));
#176002=CARTESIAN_POINT('Ctrl Pts',(7.90509867676605,-72.9817743855232,
-175.233882088622));
#176003=CARTESIAN_POINT('Ctrl Pts',(7.90544965740232,-72.967510881305,-175.285539712882));
#176004=CARTESIAN_POINT('Ctrl Pts',(7.90562730551323,-72.959913400428,-175.311848730422));
#176005=CARTESIAN_POINT('Ctrl Pts',(7.90570385869998,-72.9565547804075,
-175.323225805126));
#176006=CARTESIAN_POINT('Ctrl Pts',(7.90575498195503,-72.9542926010636,
-175.330833008964));
#176007=CARTESIAN_POINT('Ctrl Pts',(7.90578862396314,-72.9527882461173,
-175.335846745901));
#176008=CARTESIAN_POINT('Ctrl Pts',(7.90693329510708,-72.9012674128257,
-175.506610298774));
#176009=CARTESIAN_POINT('Ctrl Pts',(7.90796841236697,-72.839623599414,-175.657481499327));
#176010=CARTESIAN_POINT('Ctrl Pts',(7.90929927756806,-72.7426206144854,
-175.855928107122));
#176011=CARTESIAN_POINT('Ctrl Pts',(7.9097081812878,-72.7095177001685,-175.917489253729));
#176012=CARTESIAN_POINT('Ctrl Pts',(7.91027517352814,-72.6599954134491,
-176.003103640448));
#176013=CARTESIAN_POINT('Ctrl Pts',(7.91054721380992,-72.6352646259782,
-176.044232319737));
#176014=CARTESIAN_POINT('Ctrl Pts',(7.91084698606837,-72.6067161650734,
-176.089341310574));
#176015=CARTESIAN_POINT('Ctrl Pts',(7.91099284326656,-72.5925469657504,
-176.111186720346));
#176016=CARTESIAN_POINT('Ctrl Pts',(7.91105453093491,-72.5865000065411,
-176.120398132595));
#176017=CARTESIAN_POINT('Ctrl Pts',(7.91109547794238,-72.5824747114477,
-176.126505658783));
#176018=CARTESIAN_POINT('Ctrl Pts',(7.91110782189276,-72.5812598872988,
-176.128346248943));
#176019=CARTESIAN_POINT('Ctrl Pts',(7.91294980900864,-72.3991760858112,
-176.402443010638));
#176020=CARTESIAN_POINT('Ctrl Pts',(7.91462251977688,-72.1818766937441,
-176.633078403434));
#176021=CARTESIAN_POINT('Ctrl Pts',(7.91709744842058,-71.7199235074033,
-177.001812138227));
#176022=CARTESIAN_POINT('Ctrl Pts',(7.9179199571433,-71.4758859239583,-177.140416596742));
#176023=CARTESIAN_POINT('Ctrl Pts',(7.91859121655449,-71.2381488509313,
-177.239961484006));
#176024=CARTESIAN_POINT('Ctrl Pts',(8.40355780430818,-73.08000002,-174.451130838212));
#176025=CARTESIAN_POINT('Ctrl Pts',(8.48384574056985,-73.0800000199999,
-176.520599502442));
#176026=CARTESIAN_POINT('Ctrl Pts',(8.51230691249381,-71.1434663357064,
-177.254202907715));
#176027=CARTESIAN_POINT('Ctrl Pts',(8.20353011255175,-73.08000002,-174.458891192924));
#176028=CARTESIAN_POINT('Ctrl Pts',(8.28507376820399,-73.0800000200062,
-176.507651386999));
#176029=CARTESIAN_POINT('Ctrl Pts',(8.31384446654333,-71.1696907801609,
-177.251953160255));
#176030=CARTESIAN_POINT('Ctrl Pts',(8.00350691066062,-73.08000002,-174.46684979476));
#176031=CARTESIAN_POINT('Ctrl Pts',(8.08524840860192,-73.0800000200062,
-176.495676023668));
#176032=CARTESIAN_POINT('Ctrl Pts',(8.11484675268685,-71.1950080123696,
-177.249844108498));
#176033=CARTESIAN_POINT('Ctrl Pts',(7.80348623696872,-73.08000002,-174.474919939778));
#176034=CARTESIAN_POINT('Ctrl Pts',(7.88456937757999,-73.0800000199999,
-176.484587012089));
#176035=CARTESIAN_POINT('Ctrl Pts',(7.91536503462485,-71.2194103886423,
-177.247865511993));
#176036=CARTESIAN_POINT('',(8.41817820009134,-71.1781942230057,-177.244433726518));
#176037=CARTESIAN_POINT('Origin',(0.060185797981942,-4.47315859110275,-188.387285563199));
#176038=CARTESIAN_POINT('Ctrl Pts',(8.4181782717274,-71.1781985203566,-177.244444626904));
#176039=CARTESIAN_POINT('Ctrl Pts',(8.41754848274224,-71.4223190079251,
-177.148366085912));
#176040=CARTESIAN_POINT('Ctrl Pts',(8.41677076479328,-71.673624968976,-177.012030245796));
#176041=CARTESIAN_POINT('Ctrl Pts',(8.41497352559848,-72.0310711490723,
-176.73626320784));
#176042=CARTESIAN_POINT('Ctrl Pts',(8.41427511117919,-72.1468008645235,
-176.632607910667));
#176043=CARTESIAN_POINT('Ctrl Pts',(8.4131024423523,-72.3104942873253,-176.460057862085));
#176044=CARTESIAN_POINT('Ctrl Pts',(8.41269135999703,-72.3634047131022,
-176.399713077921));
#176045=CARTESIAN_POINT('Ctrl Pts',(8.4120536281718,-72.4396864660478,-176.305177352398));
#176046=CARTESIAN_POINT('Ctrl Pts',(8.41172955234536,-72.4770565412457,
-176.256906560854));
#176047=CARTESIAN_POINT('Ctrl Pts',(8.41134506529128,-72.5191777814738,
-176.198902525325));
#176048=CARTESIAN_POINT('Ctrl Pts',(8.41115161467346,-72.5398534996524,
-176.169488201525));
#176049=CARTESIAN_POINT('Ctrl Pts',(8.41106849187588,-72.548630387431,-176.156794784155));
#176050=CARTESIAN_POINT('Ctrl Pts',(8.41101303376165,-72.5544627669252,
-176.148313233444));
#176051=CARTESIAN_POINT('Ctrl Pts',(8.41097732083378,-72.5582002437319,
-176.142841345939));
#176052=CARTESIAN_POINT('Ctrl Pts',(8.41032368769178,-72.6263945170234,
-176.042570516628));
#176053=CARTESIAN_POINT('Ctrl Pts',(8.40959647252647,-72.6963293373607,
-175.927578445735));
#176054=CARTESIAN_POINT('Ctrl Pts',(8.40828842764586,-72.7968914105421,
-175.726319312506));
#176055=CARTESIAN_POINT('Ctrl Pts',(8.40781726081728,-72.8296531002271,
-175.654464109059));
#176056=CARTESIAN_POINT('Ctrl Pts',(8.40706213181642,-72.8761394871332,
-175.539615438644));
#176057=CARTESIAN_POINT('Ctrl Pts',(8.40680248104364,-72.8911907824282,
-175.500158002453));
#176058=CARTESIAN_POINT('Ctrl Pts',(8.4064028588357,-72.9129021099126,-175.439252056873));
#176059=CARTESIAN_POINT('Ctrl Pts',(8.40620052494692,-72.9235412990844,
-175.408369486283));
#176060=CARTESIAN_POINT('Ctrl Pts',(8.40596059062688,-72.9355307482792,
-175.371601060581));
#176061=CARTESIAN_POINT('Ctrl Pts',(8.40583973271934,-72.9414142108593,
-175.353034085953));
#176062=CARTESIAN_POINT('Ctrl Pts',(8.40578775433374,-72.9439112614011,
-175.345037862003));
#176063=CARTESIAN_POINT('Ctrl Pts',(8.40575306260396,-72.9455704663852,
-175.339698415293));
#176064=CARTESIAN_POINT('Ctrl Pts',(8.40574305179098,-72.9460486900454,
-175.338157470166));
#176065=CARTESIAN_POINT('Ctrl Pts',(8.40413497651592,-73.0222745409279,
-175.090414177992));
#176066=CARTESIAN_POINT('Ctrl Pts',(8.40277568211103,-73.0511183020758,
-174.892229744757));
#176067=CARTESIAN_POINT('Ctrl Pts',(8.40089353347954,-73.0800350040009,
-174.598255016089));
#176068=CARTESIAN_POINT('Ctrl Pts',(8.40032278615858,-73.08000002,-174.501236406862));
#176069=CARTESIAN_POINT('Ctrl Pts',(8.4,-73.08000002,-174.451268889151));
#176070=CARTESIAN_POINT('Ctrl Pts',(8.4,-73.08000002,-174.451268889151));
#176071=CARTESIAN_POINT('Ctrl Pts',(8.89999999999996,-73.0800000199999,
-174.45126888915));
#176072=CARTESIAN_POINT('Ctrl Pts',(8.9,-72.58000002,-174.451268889151));
#176073=CARTESIAN_POINT('Ctrl Pts',(8.40197484549326,-73.08000002,-174.75697631869));
#176074=CARTESIAN_POINT('Ctrl Pts',(8.89999999999997,-73.0780290434905,
-174.756376067791));
#176075=CARTESIAN_POINT('Ctrl Pts',(8.9,-72.58000001309,-174.70608894667));
#176076=CARTESIAN_POINT('Ctrl Pts',(8.40390532350201,-73.0343597586633,
-175.055047332367));
#176077=CARTESIAN_POINT('Ctrl Pts',(8.89999999999997,-73.0306532835766,
-175.053905133681));
#176078=CARTESIAN_POINT('Ctrl Pts',(8.9,-72.5419664714886,-174.954543971783));
#176079=CARTESIAN_POINT('Ctrl Pts',(8.40673247093662,-72.8985137923177,
-175.490582060873));
#176080=CARTESIAN_POINT('Ctrl Pts',(8.89999999999997,-72.892300013639,-175.488192872161));
#176081=CARTESIAN_POINT('Ctrl Pts',(8.9,-72.4287614956301,-175.317581230789));
#176082=CARTESIAN_POINT('Ctrl Pts',(8.40765712457444,-72.8418854248583,
-175.632858253021));
#176083=CARTESIAN_POINT('Ctrl Pts',(8.89999999999996,-72.8349801887897,
-175.629812439872));
#176084=CARTESIAN_POINT('Ctrl Pts',(8.9,-72.3815711902508,-175.436174718935));
#176085=CARTESIAN_POINT('Ctrl Pts',(8.40942187655549,-72.7094695330285,
-175.904119271778));
#176086=CARTESIAN_POINT('Ctrl Pts',(8.89999999999995,-72.7014018648635,
-175.899567338683));
#176087=CARTESIAN_POINT('Ctrl Pts',(8.9,-72.2712246146549,-175.662282844729));
#176088=CARTESIAN_POINT('Ctrl Pts',(8.41026946333178,-72.6333495611344,
-176.034257895752));
#176089=CARTESIAN_POINT('Ctrl Pts',(8.90000000000094,-72.6248303464193,
-176.028888062411));
#176090=CARTESIAN_POINT('Ctrl Pts',(8.9,-72.2077913051056,-175.770759223));
#176091=CARTESIAN_POINT('Ctrl Pts',(8.41189381664575,-72.4610685811814,
-176.283431179031));
#176092=CARTESIAN_POINT('Ctrl Pts',(8.89999999999898,-72.4518932717193,
-176.276278393733));
#176093=CARTESIAN_POINT('Ctrl Pts',(8.9,-72.0642238201576,-175.978456398961));
#176094=CARTESIAN_POINT('Ctrl Pts',(8.41267385193151,-72.3642066660697,
-176.402964676645));
#176095=CARTESIAN_POINT('Ctrl Pts',(8.89999999999997,-72.354843766023,-176.394881486481));
#176096=CARTESIAN_POINT('Ctrl Pts',(8.9,-71.9835055577593,-176.078093003191));
#176097=CARTESIAN_POINT('Ctrl Pts',(8.41411048564612,-72.15640796091,-176.622941542856));
#176098=CARTESIAN_POINT('Ctrl Pts',(8.89999999999996,-72.1469580486365,
-176.612968031678));
#176099=CARTESIAN_POINT('Ctrl Pts',(8.9,-71.8103399713904,-176.261453778625));
#176100=CARTESIAN_POINT('Ctrl Pts',(8.41477368991416,-72.0449155064423,
-176.724399172119));
#176101=CARTESIAN_POINT('Ctrl Pts',(8.89999999999996,-72.0355638390553,
-176.713502881279));
#176102=CARTESIAN_POINT('Ctrl Pts',(8.9,-71.7174295924368,-176.34602338026));
#176103=CARTESIAN_POINT('Ctrl Pts',(8.4165979801388,-71.6877682388606,-177.003302608065));
#176104=CARTESIAN_POINT('Ctrl Pts',(8.89999999999996,-71.6793465425378,
-176.989505620533));
#176105=CARTESIAN_POINT('Ctrl Pts',(8.9,-71.4198068682475,-176.578502281526));
#176106=CARTESIAN_POINT('Ctrl Pts',(8.41759316850175,-71.4163525958445,
-177.155190995531));
#176107=CARTESIAN_POINT('Ctrl Pts',(8.90000000001297,-71.4089014982389,
-177.139847092069));
#176108=CARTESIAN_POINT('Ctrl Pts',(8.9,-71.1936270830052,-176.705108386635));
#176109=CARTESIAN_POINT('Ctrl Pts',(8.41828452049191,-71.1360889256296,
-177.260652939026));
#176110=CARTESIAN_POINT('Ctrl Pts',(8.89999999999996,-71.1298793121603,
-177.244155204947));
#176111=CARTESIAN_POINT('Ctrl Pts',(8.9,-70.9600741080247,-176.793015835821));
#176112=CARTESIAN_POINT('',(8.89999997275898,-71.2138732976769,-176.681036188727));
#176113=CARTESIAN_POINT('Ctrl Pts',(8.41817820009134,-71.1781942230057,
-177.244433726518));
#176114=CARTESIAN_POINT('Ctrl Pts',(8.4375676815764,-71.1735772869606,-177.245495661848));
#176115=CARTESIAN_POINT('Ctrl Pts',(8.45706991645918,-71.1692642601874,
-177.245202134556));
#176116=CARTESIAN_POINT('Ctrl Pts',(8.47646911593593,-71.1652585866833,
-177.243540741873));
#176117=CARTESIAN_POINT('Ctrl Pts',(8.49577878075638,-71.1612714008803,
-177.241887017147));
#176118=CARTESIAN_POINT('Ctrl Pts',(8.51498522998455,-71.1575887387568,
-177.23887793747));
#176119=CARTESIAN_POINT('Ctrl Pts',(8.53387350322163,-71.1542229400008,
-177.234551943534));
#176120=CARTESIAN_POINT('Ctrl Pts',(8.55275572222947,-71.1508582200793,
-177.230227336202));
#176121=CARTESIAN_POINT('Ctrl Pts',(8.57131886615291,-71.1478102320468,
-177.224586951484));
#176122=CARTESIAN_POINT('Ctrl Pts',(8.58936291095303,-71.1450997228584,
-177.217718454791));
#176123=CARTESIAN_POINT('Ctrl Pts',(8.60132827930681,-71.1433023298002,
-177.213163816743));
#176124=CARTESIAN_POINT('Ctrl Pts',(8.61306573561802,-71.1416535136919,
-177.208070186524));
#176125=CARTESIAN_POINT('Ctrl Pts',(8.62452390663931,-71.1401610362592,
-177.202473579344));
#176126=CARTESIAN_POINT('Ctrl Pts',(8.64195785660902,-71.1378901871993,
-177.193958174102));
#176127=CARTESIAN_POINT('Ctrl Pts',(8.65874305599649,-71.1359810973278,
-177.184277184033));
#176128=CARTESIAN_POINT('Ctrl Pts',(8.6747322821397,-71.1344654177415,-177.173585916584));
#176129=CARTESIAN_POINT('Ctrl Pts',(8.68781013665856,-71.1332257181495,
-177.164841350771));
#176130=CARTESIAN_POINT('Ctrl Pts',(8.70035618379775,-71.1322493563043,
-177.155421846894));
#176131=CARTESIAN_POINT('Ctrl Pts',(8.71231337647849,-71.1315550709588,
-177.145423344239));
#176132=CARTESIAN_POINT('Ctrl Pts',(8.72071844212296,-71.1310670371819,
-177.13839509995));
#176133=CARTESIAN_POINT('Ctrl Pts',(8.72898238026593,-71.1307390133705,
-177.130939053363));
#176134=CARTESIAN_POINT('Ctrl Pts',(8.73693891047363,-71.1305519295886,
-177.123212241614));
#176135=CARTESIAN_POINT('Ctrl Pts',(8.74495542280103,-71.1303634354328,
-177.11542717953));
#176136=CARTESIAN_POINT('Ctrl Pts',(8.75265932972759,-71.1303181328619,
-177.107367856751));
#176137=CARTESIAN_POINT('Ctrl Pts',(8.75991760607799,-71.1304134424502,
-177.099229163266));
#176138=CARTESIAN_POINT('Ctrl Pts',(8.7674395027199,-71.1305122136788,-177.090794872777));
#176139=CARTESIAN_POINT('Ctrl Pts',(8.77448249260797,-71.1307621917784,
-177.082276150992));
#176140=CARTESIAN_POINT('Ctrl Pts',(8.78094542604629,-71.1311763041073,
-177.073915789783));
#176141=CARTESIAN_POINT('Ctrl Pts',(8.78162793702423,-71.1312200359843,
-177.073032903032));
#176142=CARTESIAN_POINT('Ctrl Pts',(8.78230402224777,-71.1312656104982,
-177.072151798275));
#176143=CARTESIAN_POINT('Ctrl Pts',(8.78297359262185,-71.1313130510302,
-177.071272771358));
#176144=CARTESIAN_POINT('Ctrl Pts',(8.79600518416733,-71.1322363679208,
-177.054164607398));
#176145=CARTESIAN_POINT('Ctrl Pts',(8.80812287853332,-71.1338142536925,
-177.035862021369));
#176146=CARTESIAN_POINT('Ctrl Pts',(8.81918777435556,-71.1360315585211,
-177.016532094964));
#176147=CARTESIAN_POINT('Ctrl Pts',(8.83018794089226,-71.1382358921875,
-176.997315248008));
#176148=CARTESIAN_POINT('Ctrl Pts',(8.84014710779646,-71.1410722089947,
-176.977084017575));
#176149=CARTESIAN_POINT('Ctrl Pts',(8.84897550413698,-71.1445316150493,
-176.956023186274));
#176150=CARTESIAN_POINT('Ctrl Pts',(8.85781148218762,-71.1479939919961,
-176.93494426821));
#176151=CARTESIAN_POINT('Ctrl Pts',(8.86551459101941,-71.152080615517,-176.913035370358));
#176152=CARTESIAN_POINT('Ctrl Pts',(8.8720466382876,-71.1567877685274,-176.890487227023));
#176153=CARTESIAN_POINT('Ctrl Pts',(8.87859517279702,-71.161506802647,-176.867882170952));
#176154=CARTESIAN_POINT('Ctrl Pts',(8.8839669332145,-71.1668496494419,-176.844635638253));
#176155=CARTESIAN_POINT('Ctrl Pts',(8.88817509862186,-71.1728160217048,
-176.820929774949));
#176156=CARTESIAN_POINT('Ctrl Pts',(8.89243798486614,-71.1788599776299,
-176.796915652689));
#176157=CARTESIAN_POINT('Ctrl Pts',(8.89550727603177,-71.1855439770296,
-176.772431064185));
#176158=CARTESIAN_POINT('Ctrl Pts',(8.89744466027399,-71.1928686565381,
-176.747640578285));
#176159=CARTESIAN_POINT('Ctrl Pts',(8.89916327906971,-71.1993662482918,
-176.725649383098));
#176160=CARTESIAN_POINT('Ctrl Pts',(8.89999223003091,-71.2063681174939,
-176.703417350348));
#176161=CARTESIAN_POINT('Ctrl Pts',(8.89999994551797,-71.2138732976722,
-176.681036188718));
#176162=CARTESIAN_POINT('Ctrl Pts',(8.9,-72.58000002,-174.451268889151));
#176163=CARTESIAN_POINT('Ctrl Pts',(8.9,-72.58000002,-174.643662890546));
#176164=CARTESIAN_POINT('Ctrl Pts',(8.90000000018189,-72.5583230934325,
-174.832372832558));
#176165=CARTESIAN_POINT('Ctrl Pts',(8.89999999981754,-72.5152520259331,
-175.017431778835));
#176166=CARTESIAN_POINT('Ctrl Pts',(8.89999999974366,-72.5065182586995,
-175.0549572421));
#176167=CARTESIAN_POINT('Ctrl Pts',(8.89999999963417,-72.4969046367659,
-175.092332595982));
#176168=CARTESIAN_POINT('Ctrl Pts',(8.89999999944856,-72.4864132528963,
-175.129558133433));
#176169=CARTESIAN_POINT('Ctrl Pts',(8.89999999933697,-72.4801056624026,
-175.151938731556));
#176170=CARTESIAN_POINT('Ctrl Pts',(8.89999999923514,-72.4734752856604,
-175.174281489137));
#176171=CARTESIAN_POINT('Ctrl Pts',(8.8999999991621,-72.4665241218154,-175.196577428232));
#176172=CARTESIAN_POINT('Ctrl Pts',(8.89999999896656,-72.4479148757583,
-175.256266801975));
#176173=CARTESIAN_POINT('Ctrl Pts',(8.89999999902277,-72.4269795805928,
-175.315421893865));
#176174=CARTESIAN_POINT('Ctrl Pts',(8.89999999928889,-72.403958991798,-175.373505006317));
#176175=CARTESIAN_POINT('Ctrl Pts',(8.89999999941373,-72.3931602367393,
-175.400751281815));
#176176=CARTESIAN_POINT('Ctrl Pts',(8.8999999995758,-72.3819033245034,-175.427761928545));
#176177=CARTESIAN_POINT('Ctrl Pts',(8.89999999971899,-72.3702165277834,
-175.454483443826));
#176178=CARTESIAN_POINT('Ctrl Pts',(8.89999999989012,-72.356250141463,-175.486417173351));
#176179=CARTESIAN_POINT('Ctrl Pts',(8.89999999994017,-72.3416346359546,
-175.518026103028));
#176180=CARTESIAN_POINT('Ctrl Pts',(8.89999999996783,-72.3264029998066,
-175.549231269472));
#176181=CARTESIAN_POINT('Ctrl Pts',(8.90000000003108,-72.2915692635033,
-175.620595404528));
#176182=CARTESIAN_POINT('Ctrl Pts',(8.90000000000045,-72.2533993434511,
-175.690229109067));
#176183=CARTESIAN_POINT('Ctrl Pts',(8.89999999999886,-72.2119321367876,
-175.757979856507));
#176184=CARTESIAN_POINT('Ctrl Pts',(8.89999999999793,-72.1877543610133,
-175.797482454149));
#176185=CARTESIAN_POINT('Ctrl Pts',(8.89999999999706,-72.1624481423419,
-175.836359594911));
#176186=CARTESIAN_POINT('Ctrl Pts',(8.89999999999683,-72.1360090283531,
-175.874608824138));
#176187=CARTESIAN_POINT('Ctrl Pts',(8.8999999999962,-72.0642253375692,-175.978457646179));
#176188=CARTESIAN_POINT('Ctrl Pts',(8.89999999999926,-71.983506448042,-176.078093573446));
#176189=CARTESIAN_POINT('Ctrl Pts',(8.8999999999998,-71.8969230956059,-176.169773703533));
#176190=CARTESIAN_POINT('Ctrl Pts',(8.90000000000003,-71.8581752387953,
-176.210802474689));
#176191=CARTESIAN_POINT('Ctrl Pts',(8.9,-71.8181601276395,-176.250407223135));
#176192=CARTESIAN_POINT('Ctrl Pts',(8.9,-71.7768804944358,-176.288591148433));
#176193=CARTESIAN_POINT('Ctrl Pts',(8.9,-71.7350069729775,-176.327324424174));
#176194=CARTESIAN_POINT('Ctrl Pts',(8.9,-71.691683332544,-176.364727207912));
#176195=CARTESIAN_POINT('Ctrl Pts',(8.9,-71.6470438920772,-176.40066126947));
#176196=CARTESIAN_POINT('Ctrl Pts',(8.9,-71.6374948625339,-176.408348091075));
#176197=CARTESIAN_POINT('Ctrl Pts',(8.9,-71.6278871345229,-176.415966736531));
#176198=CARTESIAN_POINT('Ctrl Pts',(8.9,-71.6182220181434,-176.423516347907));
#176199=CARTESIAN_POINT('Ctrl Pts',(8.9,-71.5940005454252,-176.442436213824));
#176200=CARTESIAN_POINT('Ctrl Pts',(8.9,-71.5693801206575,-176.460921216669));
#176201=CARTESIAN_POINT('Ctrl Pts',(8.9,-71.5444197215458,-176.478940580039));
#176202=CARTESIAN_POINT('Ctrl Pts',(8.9,-71.4920391665984,-176.516755049627));
#176203=CARTESIAN_POINT('Ctrl Pts',(8.89999999451621,-71.4381757456861,
-176.552638667358));
#176204=CARTESIAN_POINT('Ctrl Pts',(8.89999997064356,-71.3830164241513,
-176.586384312661));
#176205=CARTESIAN_POINT('Ctrl Pts',(8.89999995870723,-71.355436763384,-176.603257135313));
#176206=CARTESIAN_POINT('Ctrl Pts',(8.89999994562374,-71.3275333910231,
-176.61959527903));
#176207=CARTESIAN_POINT('Ctrl Pts',(8.89999993949196,-71.2993337292249,
-176.635377629733));
#176208=CARTESIAN_POINT('Ctrl Pts',(8.89999993336017,-71.2711340674268,
-176.651159980436));
#176209=CARTESIAN_POINT('Ctrl Pts',(8.89999993496575,-71.242638116192,-176.666386538126));
#176210=CARTESIAN_POINT('Ctrl Pts',(8.89999994551797,-71.2138732976722,
-176.681036188718));
#176211=CARTESIAN_POINT('Ctrl Pts',(8.9,-71.2138732976838,-171.871644662643));
#176212=CARTESIAN_POINT('Ctrl Pts',(8.89999999999996,-70.7880957152448,
-171.871644662643));
#176213=CARTESIAN_POINT('Ctrl Pts',(9.32033898305081,-70.7202599648223,
-171.871644662643));
#176214=CARTESIAN_POINT('Ctrl Pts',(8.9,-71.2138732807092,-171.652697712588));
#176215=CARTESIAN_POINT('Ctrl Pts',(8.89999999999997,-70.7880957023883,
-171.715624308049));
#176216=CARTESIAN_POINT('Ctrl Pts',(9.32033898569755,-70.7202599643952,
-171.725683074261));
#176217=CARTESIAN_POINT('Ctrl Pts',(8.9,-71.16598797688,-171.437720890984));
#176218=CARTESIAN_POINT('Ctrl Pts',(8.90000000000455,-70.7514100828351,
-171.561941332422));
#176219=CARTESIAN_POINT('Ctrl Pts',(9.32278024510803,-70.6879410017649,
-171.582358093922));
#176220=CARTESIAN_POINT('Ctrl Pts',(8.9,-71.0715121820529,-171.237717270032));
#176221=CARTESIAN_POINT('Ctrl Pts',(8.89999999999997,-70.680735306053,-171.422308714525));
#176222=CARTESIAN_POINT('Ctrl Pts',(9.3276302147955,-70.6241744288951,-171.449026400902));
#176223=CARTESIAN_POINT('',(8.9,-71.2138732976838,-171.871644662643));
#176224=CARTESIAN_POINT('',(9.32033898305081,-70.7202599648223,-171.871644662643));
#176225=CARTESIAN_POINT('Origin',(9.4,-71.2138732976838,-171.871644662643));
#176226=CARTESIAN_POINT('Origin',(9.42941145485511,-69.2860804967121,-171.96074458416));
#176227=CARTESIAN_POINT('Origin',(8.9,-69.0831852719725,-172.006057477089));
#176228=CARTESIAN_POINT('Origin',(0.,-12.9675000200281,-171.64995));
#176229=CARTESIAN_POINT('Origin',(0.,-12.9675000200281,-171.449026400902));
#176230=CARTESIAN_POINT('Ctrl Pts',(15.5499999899231,-69.8405291599117,
-171.179005018994));
#176231=CARTESIAN_POINT('Ctrl Pts',(15.5501264775731,-69.2858420378445,
-171.477695372047));
#176232=CARTESIAN_POINT('Ctrl Pts',(14.9365391746094,-69.4116829512028,
-171.409919376296));
#176233=CARTESIAN_POINT('Ctrl Pts',(15.5499999897578,-69.9655161046422,
-171.411462758814));
#176234=CARTESIAN_POINT('Ctrl Pts',(15.5501302527646,-69.3463988305637,
-171.619616090566));
#176235=CARTESIAN_POINT('Ctrl Pts',(14.9264726997877,-69.4976592258842,
-171.564867666237));
#176236=CARTESIAN_POINT('Ctrl Pts',(15.5499999896779,-70.0263968022397,
-171.67105498688));
#176237=CARTESIAN_POINT('Ctrl Pts',(15.5501321305782,-69.3710444733645,
-171.760987815194));
#176238=CARTESIAN_POINT('Ctrl Pts',(14.9216112388798,-69.5395284795157,
-171.737936502975));
#176239=CARTESIAN_POINT('Ctrl Pts',(15.5499999896938,-70.014294651194,-171.938280796929));
#176240=CARTESIAN_POINT('Ctrl Pts',(15.5501317589361,-69.3660274114058,
-171.908368448016));
#176241=CARTESIAN_POINT('Ctrl Pts',(14.9225783333433,-69.5312053406244,
-171.916063466645));
#176242=CARTESIAN_POINT('',(14.9224576271186,-69.5322439721301,-171.871644662643));
#176243=CARTESIAN_POINT('',(15.55,-70.015703322148,-171.871644662643));
#176244=CARTESIAN_POINT('Origin',(15.05,-70.015703322148,-171.871644662643));
#176245=CARTESIAN_POINT('Origin',(15.5500003878737,-68.575584871424,-171.847853238404));
#176246=CARTESIAN_POINT('Origin',(15.0818693592772,-68.1696517950468,-171.933679697753));
#176247=CARTESIAN_POINT('Origin',(16.05,67.7009572055632,-176.84995));
#176248=CARTESIAN_POINT('',(15.55,-70.015703322148,-176.84995));
#176249=CARTESIAN_POINT('',(15.55,67.7009572055632,-176.84995));
#176250=CARTESIAN_POINT('',(16.05,-69.7424724991055,-177.34995));
#176251=CARTESIAN_POINT('Ctrl Pts',(15.55,-70.015703322148,-176.84995));
#176252=CARTESIAN_POINT('Ctrl Pts',(15.55,-70.015703322148,-176.91494123845));
#176253=CARTESIAN_POINT('Ctrl Pts',(15.5628555543669,-70.0086459123549,
-176.981685962264));
#176254=CARTESIAN_POINT('Ctrl Pts',(15.6027343713053,-69.9874736829755,
-177.076046165501));
#176255=CARTESIAN_POINT('Ctrl Pts',(15.6194250432354,-69.9786519207341,
-177.106520258027));
#176256=CARTESIAN_POINT('Ctrl Pts',(15.6493572717207,-69.9627727486995,
-177.149601759466));
#176257=CARTESIAN_POINT('Ctrl Pts',(15.665543236393,-69.9541715305142,-177.170484481011));
#176258=CARTESIAN_POINT('Ctrl Pts',(15.6864714438853,-69.9429789196704,
-177.193440465358));
#176259=CARTESIAN_POINT('Ctrl Pts',(15.695866056015,-69.9379339743885,-177.202950082533));
#176260=CARTESIAN_POINT('Ctrl Pts',(15.7022221563807,-69.93451554152,-177.20921380285));
#176261=CARTESIAN_POINT('Ctrl Pts',(15.7065958386429,-69.9321588011156,
-177.213380882268));
#176262=CARTESIAN_POINT('Ctrl Pts',(15.742655916585,-69.9127040608674,-177.24705982817));
#176263=CARTESIAN_POINT('Ctrl Pts',(15.7871759484761,-69.8878370635255,
-177.279883700671));
#176264=CARTESIAN_POINT('Ctrl Pts',(15.9012930184395,-69.8249897616838,
-177.331412046965));
#176265=CARTESIAN_POINT('Ctrl Pts',(15.9712278950399,-69.7870094571841,
-177.34995));
#176266=CARTESIAN_POINT('Ctrl Pts',(16.05,-69.7424724991055,-177.34995));
#176267=CARTESIAN_POINT('',(16.05,-73.08000002,-177.34995));
#176268=CARTESIAN_POINT('Origin',(41.5,-73.08000002,-177.34995));
#176269=CARTESIAN_POINT('',(16.55,-69.5987413979107,-177.34995));
#176270=CARTESIAN_POINT('Origin',(0.,-12.9675000200281,-177.34995));
#176271=CARTESIAN_POINT('',(16.55,-73.08000002,-177.34995));
#176272=CARTESIAN_POINT('Origin',(16.55,-73.08000002,-176.84995));
#176273=CARTESIAN_POINT('',(17.05,-69.2968662511513,-176.84995));
#176274=CARTESIAN_POINT('Ctrl Pts',(16.55,-69.5987413979107,-177.34995));
#176275=CARTESIAN_POINT('Ctrl Pts',(16.6373149037964,-69.5477073176868,
-177.34995));
#176276=CARTESIAN_POINT('Ctrl Pts',(16.7108961971465,-69.505235927113,-177.327452298007));
#176277=CARTESIAN_POINT('Ctrl Pts',(16.7952352006602,-69.4543728757275,
-177.286795171739));
#176278=CARTESIAN_POINT('Ctrl Pts',(16.8192471597269,-69.4395591976782,
-177.272004751375));
#176279=CARTESIAN_POINT('Ctrl Pts',(16.849797428493,-69.420549689223,-177.250296803926));
#176280=CARTESIAN_POINT('Ctrl Pts',(16.85907485883,-69.4147483545077,-177.243132320069));
#176281=CARTESIAN_POINT('Ctrl Pts',(16.8717470097012,-69.4068491045895,
-177.232714631389));
#176282=CARTESIAN_POINT('Ctrl Pts',(16.8777722497188,-69.4031001676691,
-177.227587343521));
#176283=CARTESIAN_POINT('Ctrl Pts',(16.8842838194923,-69.3990776119963,
-177.221789622403));
#176284=CARTESIAN_POINT('Ctrl Pts',(16.8869663155695,-69.3974289175796,
-177.219348341421));
#176285=CARTESIAN_POINT('Ctrl Pts',(16.8887309156035,-69.3963465119717,
-177.217730912076));
#176286=CARTESIAN_POINT('Ctrl Pts',(16.8887814612853,-69.3963144313396,
-177.217689547856));
#176287=CARTESIAN_POINT('Ctrl Pts',(16.9978912643005,-69.3296738982238,
-177.116243128376));
#176288=CARTESIAN_POINT('Ctrl Pts',(17.05,-69.2968662511514,-176.977183756916));
#176289=CARTESIAN_POINT('Ctrl Pts',(17.05,-69.2968662511513,-176.84995));
#176290=CARTESIAN_POINT('',(17.05,67.7009572055632,-176.84995));
#176291=CARTESIAN_POINT('Ctrl Pts',(17.0500000069342,-69.2954487057977,
-171.937551171933));
#176292=CARTESIAN_POINT('Ctrl Pts',(17.0499387022882,-68.9277121722468,
-171.920632758432));
#176293=CARTESIAN_POINT('Ctrl Pts',(17.4014093021639,-68.8184551193695,
-171.915576738158));
#176294=CARTESIAN_POINT('Ctrl Pts',(17.0500000069124,-69.3074655181351,
-171.673561286109));
#176295=CARTESIAN_POINT('Ctrl Pts',(17.0499389461697,-68.9377102872281,
-171.724562885898));
#176296=CARTESIAN_POINT('Ctrl Pts',(17.4003036470898,-68.8268112548536,
-171.739609324912));
#176297=CARTESIAN_POINT('Ctrl Pts',(17.0500000070217,-69.2471945003534,
-171.413338787174));
#176298=CARTESIAN_POINT('Ctrl Pts',(17.0499377162343,-68.887140708855,-171.529148195035));
#176299=CARTESIAN_POINT('Ctrl Pts',(17.4058449755969,-68.7849016359872,
-171.566109516219));
#176300=CARTESIAN_POINT('Ctrl Pts',(17.050000007256,-69.1191208280442,-171.178440426026));
#176301=CARTESIAN_POINT('Ctrl Pts',(17.049935034885,-68.784349448281,-171.361182926232));
#176302=CARTESIAN_POINT('Ctrl Pts',(17.4177209010562,-68.6958205805999,
-171.409539580699));
#176303=CARTESIAN_POINT('',(17.05,-69.2968662511513,-171.871644662643));
#176304=CARTESIAN_POINT('',(17.4012711864406,-68.8194987407181,-171.871644662643));
#176305=CARTESIAN_POINT('Origin',(17.55,-69.2968662511513,-171.871644662643));
#176306=CARTESIAN_POINT('Origin',(17.5775564056945,-67.4962149130001,-171.919974670304));
#176307=CARTESIAN_POINT('Origin',(17.0499997303006,-67.819556247646,-171.852380931002));
#176308=CARTESIAN_POINT('Origin',(0.,-12.9675000200281,-171.64995));
#176309=CARTESIAN_POINT('Origin',(0.,-12.9675000200281,-171.449026400902));
#176310=CARTESIAN_POINT('Ctrl Pts',(23.6999999991623,-67.0454033354271,
-171.20624326692));
#176311=CARTESIAN_POINT('Ctrl Pts',(23.7000418723672,-66.4085345904086,
-171.54923960952));
#176312=CARTESIAN_POINT('Ctrl Pts',(23.0233258551592,-66.6335614679979,
-171.428053802022));
#176313=CARTESIAN_POINT('Ctrl Pts',(23.6999999991454,-67.1609416565798,
-171.420795636131));
#176314=CARTESIAN_POINT('Ctrl Pts',(23.7000436385783,-66.4472919682882,
-171.670421709918));
#176315=CARTESIAN_POINT('Ctrl Pts',(23.0096928629965,-66.7164302706426,
-171.571078901793));
#176316=CARTESIAN_POINT('Ctrl Pts',(23.6999999991368,-67.2206799332608,
-171.660715193498));
#176317=CARTESIAN_POINT('Ctrl Pts',(23.7000445959749,-66.4581897882971,
-171.777275420467));
#176318=CARTESIAN_POINT('Ctrl Pts',(23.0026938228069,-66.7592463230828,
-171.731032985114));
#176319=CARTESIAN_POINT('Ctrl Pts',(23.6999999991377,-67.2142749444978,
-171.907589194386));
#176320=CARTESIAN_POINT('Ctrl Pts',(23.7000444926391,-66.4569597257247,
-171.887725483324));
#176321=CARTESIAN_POINT('Ctrl Pts',(23.0034444927494,-66.7546555329274,
-171.895606459213));
#176322=CARTESIAN_POINT('',(23.0033898305084,-66.7549897951204,-171.871644662643));
#176323=CARTESIAN_POINT('',(23.7,-67.2147119299503,-171.871644662643));
#176324=CARTESIAN_POINT('Origin',(23.2,-67.2147119299503,-171.871644662643));
#176325=CARTESIAN_POINT('Origin',(23.7000000319861,-65.6225360749325,-171.86419456266));
#176326=CARTESIAN_POINT('Origin',(23.2065639509939,-65.5194270282055,-171.885488297765));
#176327=CARTESIAN_POINT('Origin',(24.2,67.7009572055632,-176.84995));
#176328=CARTESIAN_POINT('',(23.7,-67.2147119299503,-176.84995));
#176329=CARTESIAN_POINT('',(23.7,67.7009572055632,-176.84995));
#176330=CARTESIAN_POINT('Ctrl Pts',(23.7,-67.2147119299503,-176.84995));
#176331=CARTESIAN_POINT('Ctrl Pts',(23.7,-67.2147119285726,-176.870692031375));
#176332=CARTESIAN_POINT('Ctrl Pts',(23.7012797601937,-67.2135616384388,
-176.891634364146));
#176333=CARTESIAN_POINT('Ctrl Pts',(23.7039194454134,-67.2112230997102,
-176.912596783915));
#176334=CARTESIAN_POINT('Ctrl Pts',(23.7066095392776,-67.2088399031692,
-176.933959511703));
#176335=CARTESIAN_POINT('Ctrl Pts',(23.7107117632145,-67.2052226460133,
-176.955342815323));
#176336=CARTESIAN_POINT('Ctrl Pts',(23.7162692188089,-67.2003662942674,
-176.976554114755));
#176337=CARTESIAN_POINT('Ctrl Pts',(23.7220047923845,-67.1953542951115,
-176.998445242172));
#176338=CARTESIAN_POINT('Ctrl Pts',(23.7292901618176,-67.1890225112425,
-177.020152969052));
#176339=CARTESIAN_POINT('Ctrl Pts',(23.7381319919838,-67.1814025218832,
-177.041467487942));
#176340=CARTESIAN_POINT('Ctrl Pts',(23.7391976331291,-67.1804841402771,
-177.044036371069));
#176341=CARTESIAN_POINT('Ctrl Pts',(23.7402858382315,-67.1795470891622,
-177.046599546418));
#176342=CARTESIAN_POINT('Ctrl Pts',(23.7413965830518,-67.1785914583024,
-177.04915664994));
#176343=CARTESIAN_POINT('Ctrl Pts',(23.741870080286,-67.1781840842947,-177.050246712593));
#176344=CARTESIAN_POINT('Ctrl Pts',(23.7423474960057,-67.1777734819474,
-177.051335172668));
#176345=CARTESIAN_POINT('Ctrl Pts',(23.7428288211218,-67.1773596636845,
-177.05242200224));
#176346=CARTESIAN_POINT('Ctrl Pts',(23.7517852561296,-67.169659387399,-177.072645585206));
#176347=CARTESIAN_POINT('Ctrl Pts',(23.7621641594692,-67.1607728029265,
-177.09245347496));
#176348=CARTESIAN_POINT('Ctrl Pts',(23.7739445340405,-67.1506901238837,
-177.111633175902));
#176349=CARTESIAN_POINT('Ctrl Pts',(23.7812121202196,-67.1444698854341,
-177.123465578059));
#176350=CARTESIAN_POINT('Ctrl Pts',(23.789012306361,-67.1377950491387,-177.135058645404));
#176351=CARTESIAN_POINT('Ctrl Pts',(23.7973324888522,-67.1306693301689,
-177.146360830239));
#176352=CARTESIAN_POINT('Ctrl Pts',(23.8082358689858,-67.121331263037,-177.161172045945));
#176353=CARTESIAN_POINT('Ctrl Pts',(23.8200331807256,-67.1112150240728,
-177.175484411367));
#176354=CARTESIAN_POINT('Ctrl Pts',(23.8326843101586,-67.1003206129902,
-177.189182955555));
#176355=CARTESIAN_POINT('Ctrl Pts',(23.839009874875,-67.0948734074488,-177.196032227649));
#176356=CARTESIAN_POINT('Ctrl Pts',(23.8455486735696,-67.089231658847,-177.202728037883));
#176357=CARTESIAN_POINT('Ctrl Pts',(23.8522943595325,-67.0833953671697,
-177.209255974639));
#176358=CARTESIAN_POINT('Ctrl Pts',(23.8531068061667,-67.0826924474732,
-177.210042195681));
#176359=CARTESIAN_POINT('Ctrl Pts',(23.853922355455,-67.0819866047119,-177.210826081485));
#176360=CARTESIAN_POINT('Ctrl Pts',(23.8547411191067,-67.0812777232316,
-177.211607719321));
#176361=CARTESIAN_POINT('Ctrl Pts',(23.8573214233073,-67.0790437087423,
-177.214071022849));
#176362=CARTESIAN_POINT('Ctrl Pts',(23.8599283666054,-67.0767840894236,
-177.21650808797));
#176363=CARTESIAN_POINT('Ctrl Pts',(23.8625657042021,-67.0744950225944,
-177.218921760132));
#176364=CARTESIAN_POINT('Ctrl Pts',(23.8643028035408,-67.0729873140326,
-177.220511540796));
#176365=CARTESIAN_POINT('Ctrl Pts',(23.8660524525317,-67.0714674465852,
-177.222090569041));
#176366=CARTESIAN_POINT('Ctrl Pts',(23.8678145807482,-67.0699354202555,
-177.223658583861));
#176367=CARTESIAN_POINT('Ctrl Pts',(23.8691222662937,-67.0687984946517,
-177.224822216732));
#176368=CARTESIAN_POINT('Ctrl Pts',(23.8708574224727,-67.0672886464112,
-177.226347875915));
#176369=CARTESIAN_POINT('Ctrl Pts',(23.8720842239918,-67.0662206684884,
-177.227414994998));
#176370=CARTESIAN_POINT('Ctrl Pts',(23.8725105581066,-67.0658495282385,
-177.227785836786));
#176371=CARTESIAN_POINT('Ctrl Pts',(23.8728752241867,-67.0655320043267,
-177.228101752667));
#176372=CARTESIAN_POINT('Ctrl Pts',(23.8731383243725,-67.0653028646134,
-177.228329329561));
#176373=CARTESIAN_POINT('Ctrl Pts',(23.887766197763,-67.0525631293517,-177.240982175007));
#176374=CARTESIAN_POINT('Ctrl Pts',(23.9043961020168,-67.0378486429253,
-177.25389505309));
#176375=CARTESIAN_POINT('Ctrl Pts',(23.9232187485375,-67.0211404256529,
-177.266409258693));
#176376=CARTESIAN_POINT('Ctrl Pts',(23.9397950230927,-67.0064262356728,
-177.277429967587));
#176377=CARTESIAN_POINT('Ctrl Pts',(23.9580728621069,-66.990165285662,-177.288140814983));
#176378=CARTESIAN_POINT('Ctrl Pts',(23.9781590017411,-66.9723643726518,
-177.298066162563));
#176379=CARTESIAN_POINT('Ctrl Pts',(23.9861671400254,-66.9652673308325,
-177.302023297055));
#176380=CARTESIAN_POINT('Ctrl Pts',(23.9944623545837,-66.9579257812752,
-177.305855307432));
#176381=CARTESIAN_POINT('Ctrl Pts',(24.0030496089252,-66.9503413947625,
-177.30953097987));
#176382=CARTESIAN_POINT('Ctrl Pts',(24.0072023560129,-66.9466736288213,
-177.311308514039));
#176383=CARTESIAN_POINT('Ctrl Pts',(24.0114211643624,-66.942952280217,-177.313048623161));
#176384=CARTESIAN_POINT('Ctrl Pts',(24.0157157303611,-66.9391675502872,
-177.314751315045));
#176385=CARTESIAN_POINT('Ctrl Pts',(24.0184771087475,-66.9367339932224,
-177.315846135003));
#176386=CARTESIAN_POINT('Ctrl Pts',(24.021264601256,-66.9342788232166,-177.316923432121));
#176387=CARTESIAN_POINT('Ctrl Pts',(24.0240806672581,-66.9317995439269,
-177.317982914177));
#176388=CARTESIAN_POINT('Ctrl Pts',(24.0418552938833,-66.9161506693476,
-177.324670221204));
#176389=CARTESIAN_POINT('Ctrl Pts',(24.0607501496559,-66.8995614641303,
-177.330637276664));
#176390=CARTESIAN_POINT('Ctrl Pts',(24.0806754375043,-66.8820258797966,
-177.335543884029));
#176391=CARTESIAN_POINT('Ctrl Pts',(24.08898231696,-66.8747152709686,-177.337589455276));
#176392=CARTESIAN_POINT('Ctrl Pts',(24.0974678845696,-66.8672405112961,
-177.339451006893));
#176393=CARTESIAN_POINT('Ctrl Pts',(24.1061239179331,-66.8596026636562,
-177.341105388679));
#176394=CARTESIAN_POINT('Ctrl Pts',(24.1276333471999,-66.8406233302057,
-177.34521637191));
#176395=CARTESIAN_POINT('Ctrl Pts',(24.1501943609476,-66.8206347276726,
-177.348045999505));
#176396=CARTESIAN_POINT('Ctrl Pts',(24.17369751107,-66.7996305028337,-177.349268224205));
#176397=CARTESIAN_POINT('Ctrl Pts',(24.1823400263588,-66.7919068856439,
-177.349717657391));
#176398=CARTESIAN_POINT('Ctrl Pts',(24.1911096430966,-66.7840462719998,
-177.34995));
#176399=CARTESIAN_POINT('Ctrl Pts',(24.2,-66.7760495265873,-177.34995));
#176400=CARTESIAN_POINT('Origin',(0.,-12.9675000200281,-171.64995));
#176401=CARTESIAN_POINT('',(42.,30.4123236926243,-171.64995));
#176402=CARTESIAN_POINT('Origin',(44.5079524583208,31.5404524382925,-171.64995));
#176403=CARTESIAN_POINT('',(42.,28.91999998,-171.64995));
#176404=CARTESIAN_POINT('Origin',(0.,-12.9675000200281,-171.64995));
#176405=CARTESIAN_POINT('',(42.,32.6685811839606,-171.64995));
#176406=CARTESIAN_POINT('',(42.,28.91999998,-171.64995));
#176407=CARTESIAN_POINT('Origin',(44.5079524583208,31.5404524382925,-171.64995));
#176408=CARTESIAN_POINT('Ctrl Pts',(45.342056117244,28.41999998,-171.14995));
#176409=CARTESIAN_POINT('Ctrl Pts',(45.342056117244,28.41999998,-171.649955087908));
#176410=CARTESIAN_POINT('Ctrl Pts',(45.342056117244,28.9200050678815,-171.649949999974));
#176411=CARTESIAN_POINT('Ctrl Pts',(45.2032855852167,28.41999998,-171.149950027441));
#176412=CARTESIAN_POINT('Ctrl Pts',(45.2207546457863,28.4199999799926,-171.611343620546));
#176413=CARTESIAN_POINT('Ctrl Pts',(45.2161093325492,28.8799153348106,-171.649950408626));
#176414=CARTESIAN_POINT('Ctrl Pts',(45.0642313709306,28.41999998,-171.155055788632));
#176415=CARTESIAN_POINT('Ctrl Pts',(45.0814092233328,28.4199999800032,-171.586474354512));
#176416=CARTESIAN_POINT('Ctrl Pts',(45.0809055449373,28.8470468727513,-171.649950690988));
#176417=CARTESIAN_POINT('Ctrl Pts',(44.7862672310248,28.41999998,-171.163656910012));
#176418=CARTESIAN_POINT('Ctrl Pts',(44.7998786663722,28.4199999799969,-171.556875075933));
#176419=CARTESIAN_POINT('Ctrl Pts',(44.7999542633241,28.8023061531436,-171.649951053492));
#176420=CARTESIAN_POINT('Ctrl Pts',(44.6472721153249,28.41999998,-171.16702013224));
#176421=CARTESIAN_POINT('Ctrl Pts',(44.652744176702,28.4199999799986,-171.550586180072));
#176422=CARTESIAN_POINT('Ctrl Pts',(44.6541596767004,28.7904721518725,-171.64995113455));
#176423=CARTESIAN_POINT('Ctrl Pts',(44.3691883762669,28.41999998,-171.167028040093));
#176424=CARTESIAN_POINT('Ctrl Pts',(44.3637416796286,28.4199999800014,-171.550568959217));
#176425=CARTESIAN_POINT('Ctrl Pts',(44.36232828092,28.7904412154044,-171.649951134795));
#176426=CARTESIAN_POINT('Ctrl Pts',(44.2300913879779,28.41999998,-171.163669856825));
#176427=CARTESIAN_POINT('Ctrl Pts',(44.2164931090597,28.4199999799986,-171.556843793952));
#176428=CARTESIAN_POINT('Ctrl Pts',(44.2164190292983,28.802252604719,-171.649951053893));
#176429=CARTESIAN_POINT('Ctrl Pts',(43.9520032655911,28.41999998,-171.15506708045));
#176430=CARTESIAN_POINT('Ctrl Pts',(43.9348222136901,28.4199999800015,-171.586421593668));
#176431=CARTESIAN_POINT('Ctrl Pts',(43.9353228646307,28.846974377406,-171.649950691605));
#176432=CARTESIAN_POINT('Ctrl Pts',(43.8129594627921,28.41999998,-171.149950027533));
#176433=CARTESIAN_POINT('Ctrl Pts',(43.7954409326623,28.41999998,-171.611251100138));
#176434=CARTESIAN_POINT('Ctrl Pts',(43.8001087095933,28.8798156647999,-171.649950409642));
#176435=CARTESIAN_POINT('Ctrl Pts',(43.6738487993976,28.41999998,-171.14995));
#176436=CARTESIAN_POINT('Ctrl Pts',(43.6738487993976,28.41999998,-171.649955087908));
#176437=CARTESIAN_POINT('Ctrl Pts',(43.6738487993977,28.9200050678815,-171.649949999974));
#176438=CARTESIAN_POINT('',(44.5079524583208,28.7904524382925,-171.649949999924));
#176439=CARTESIAN_POINT('Ctrl Pts',(45.342056117244,28.91999998,-171.64995));
#176440=CARTESIAN_POINT('Ctrl Pts',(45.2444206001237,28.8889220866335,-171.64995));
#176441=CARTESIAN_POINT('Ctrl Pts',(45.1451244228621,28.8633251672671,-171.649944548206));
#176442=CARTESIAN_POINT('Ctrl Pts',(44.9394280113021,28.8223952301246,-171.649950242377));
#176443=CARTESIAN_POINT('Ctrl Pts',(44.8330889161033,28.8076347675278,-171.649941035199));
#176444=CARTESIAN_POINT('Ctrl Pts',(44.6535686799005,28.7933450738466,-171.649939911887));
#176445=CARTESIAN_POINT('Ctrl Pts',(44.5807764535826,28.7904525215287,-171.649950037471));
#176446=CARTESIAN_POINT('Ctrl Pts',(44.5079556015787,28.7904524382943,-171.649949999926));
#176447=CARTESIAN_POINT('Ctrl Pts',(44.5079524583208,28.7904524382925,-171.649949999924));
#176448=CARTESIAN_POINT('Ctrl Pts',(44.4351590053695,28.7904524382925,-171.649949961984));
#176449=CARTESIAN_POINT('Ctrl Pts',(44.3623973025111,28.7933425641162,-171.649939477443));
#176450=CARTESIAN_POINT('Ctrl Pts',(44.1829231968703,28.8076227744787,-171.649940712955));
#176451=CARTESIAN_POINT('Ctrl Pts',(44.0766026663103,28.8223760301809,-171.649950205467));
#176452=CARTESIAN_POINT('Ctrl Pts',(43.8708751019518,28.8633007826367,-171.649945186571));
#176453=CARTESIAN_POINT('Ctrl Pts',(43.771530849245,28.8889072750242,-171.64995));
#176454=CARTESIAN_POINT('Ctrl Pts',(43.6738487993977,28.91999998,-171.64995));
#176455=CARTESIAN_POINT('Ctrl Pts',(45.342056117244,28.41999998,-171.14995));
#176456=CARTESIAN_POINT('Ctrl Pts',(45.222494788141,28.41999998,-171.149950023642));
#176457=CARTESIAN_POINT('Ctrl Pts',(45.102890712293,28.41999998,-171.153734801587));
#176458=CARTESIAN_POINT('Ctrl Pts',(44.9833706553288,28.41999998,-171.157527071728));
#176459=CARTESIAN_POINT('Ctrl Pts',(44.9639944908896,28.41999998,-171.158141861008));
#176460=CARTESIAN_POINT('Ctrl Pts',(44.9446205282342,28.41999998,-171.158756957286));
#176461=CARTESIAN_POINT('Ctrl Pts',(44.9252493015934,28.41999998,-171.15935636922));
#176462=CARTESIAN_POINT('Ctrl Pts',(44.7862513546676,28.41999998,-171.163657440581));
#176463=CARTESIAN_POINT('Ctrl Pts',(44.6473090850418,28.41999998,-171.167020207454));
#176464=CARTESIAN_POINT('Ctrl Pts',(44.5082302458003,28.41999998,-171.167024238765));
#176465=CARTESIAN_POINT('Ctrl Pts',(44.5082032664897,28.41999998,-171.167024239547));
#176466=CARTESIAN_POINT('Ctrl Pts',(44.5081762871737,28.41999998,-171.167024240203));
#176467=CARTESIAN_POINT('Ctrl Pts',(44.5081493078523,28.41999998,-171.167024240732));
#176468=CARTESIAN_POINT('Ctrl Pts',(44.3691292618367,28.41999998,-171.16702696589));
#176469=CARTESIAN_POINT('Ctrl Pts',(44.2300667116137,28.41999998,-171.163669289098));
#176470=CARTESIAN_POINT('Ctrl Pts',(44.0910473224682,28.41999998,-171.159368608161));
#176471=CARTESIAN_POINT('Ctrl Pts',(43.9520204566156,28.41999998,-171.155067695926));
#176472=CARTESIAN_POINT('Ctrl Pts',(43.8129841111527,28.41999998,-171.149950027538));
#176473=CARTESIAN_POINT('Ctrl Pts',(43.6738487993976,28.41999998,-171.14995));
#176474=CARTESIAN_POINT('Origin',(0.,-12.9675000200281,-171.64995));
#176475=CARTESIAN_POINT('Origin',(44.5079524583208,-57.4754524783487,-171.64995));
#176476=CARTESIAN_POINT('Ctrl Pts',(43.1572831724514,-54.58000002,-171.14995));
#176477=CARTESIAN_POINT('Ctrl Pts',(43.1572831724515,-54.58000002,-171.650098123446));
#176478=CARTESIAN_POINT('Ctrl Pts',(43.1572831724514,-55.0801481215052,
-171.649949978066));
#176479=CARTESIAN_POINT('Ctrl Pts',(43.3817682803707,-54.58000002,-171.149950056136));
#176480=CARTESIAN_POINT('Ctrl Pts',(43.3143913613983,-54.5800000199971,
-171.561466059479));
#176481=CARTESIAN_POINT('Ctrl Pts',(43.3271185292342,-54.98437233152,-171.649978738968));
#176482=CARTESIAN_POINT('Ctrl Pts',(43.6059648750607,-54.58000002,-171.185915645006));
#176483=CARTESIAN_POINT('Ctrl Pts',(43.5407821982003,-54.5800000200016,
-171.520211742113));
#176484=CARTESIAN_POINT('Ctrl Pts',(43.529947173783,-54.8943395876962,-171.649995064611));
#176485=CARTESIAN_POINT('Ctrl Pts',(44.0540062919344,-54.58000002,-171.260373422648));
#176486=CARTESIAN_POINT('Ctrl Pts',(44.0046317151096,-54.5800000199985,
-171.495876387334));
#176487=CARTESIAN_POINT('Ctrl Pts',(43.9881565230544,-54.764616113508,-171.65000835312));
#176488=CARTESIAN_POINT('Ctrl Pts',(44.2780419706102,-54.58000002,-171.296906912307));
#176489=CARTESIAN_POINT('Ctrl Pts',(44.2580491347888,-54.58000002,-171.503655116484));
#176490=CARTESIAN_POINT('Ctrl Pts',(44.2440095987557,-54.7260645641698,
-171.650006647718));
#176491=CARTESIAN_POINT('Ctrl Pts',(44.7276655629966,-54.58000002,-171.297869301671));
#176492=CARTESIAN_POINT('Ctrl Pts',(44.7466180387422,-54.58000002,-171.503788967852));
#176493=CARTESIAN_POINT('Ctrl Pts',(44.7601884828714,-54.724965517749,-171.65000663285));
#176494=CARTESIAN_POINT('Ctrl Pts',(44.9532637149971,-54.58000002,-171.261822611311));
#176495=CARTESIAN_POINT('Ctrl Pts',(45.0021140860299,-54.58000002,-171.495868847089));
#176496=CARTESIAN_POINT('Ctrl Pts',(45.0183788445838,-54.7626525929473,
-171.650008425802));
#176497=CARTESIAN_POINT('Ctrl Pts',(45.4045230317323,-54.58000002,-171.186802156157));
#176498=CARTESIAN_POINT('Ctrl Pts',(45.4698465063651,-54.58000002,-171.51943524171));
#176499=CARTESIAN_POINT('Ctrl Pts',(45.4809398893321,-54.8922510295818,
-171.649995402787));
#176500=CARTESIAN_POINT('Ctrl Pts',(45.6299507757146,-54.58000002,-171.149950055386));
#176501=CARTESIAN_POINT('Ctrl Pts',(45.6987517183233,-54.5800000199883,
-171.559908009068));
#176502=CARTESIAN_POINT('Ctrl Pts',(45.6855420836464,-54.9825427397822,
-171.649979290157));
#176503=CARTESIAN_POINT('Ctrl Pts',(45.8586217441902,-54.58000002,-171.14995));
#176504=CARTESIAN_POINT('Ctrl Pts',(45.8586217441902,-54.58000002,-171.650098123446));
#176505=CARTESIAN_POINT('Ctrl Pts',(45.8586217441902,-55.0801481215052,
-171.649949978066));
#176506=CARTESIAN_POINT('Ctrl Pts',(43.1572831724514,-55.08000002,-171.64995));
#176507=CARTESIAN_POINT('Ctrl Pts',(43.2591939625018,-55.0225379010838,
-171.64995));
#176508=CARTESIAN_POINT('Ctrl Pts',(43.3646678477779,-54.9716377963967,
-171.649923799797));
#176509=CARTESIAN_POINT('Ctrl Pts',(43.5936897926191,-54.8786129298122,
-171.649916554972));
#176510=CARTESIAN_POINT('Ctrl Pts',(43.7176454367752,-54.838244085283,-171.650015979223));
#176511=CARTESIAN_POINT('Ctrl Pts',(43.9338902925313,-54.7844427443934,
-171.649835982333));
#176512=CARTESIAN_POINT('Ctrl Pts',(44.0248533307643,-54.7666339585907,
-171.649693211769));
#176513=CARTESIAN_POINT('Ctrl Pts',(44.1415243890184,-54.7498576856655,
-171.649668212268));
#176514=CARTESIAN_POINT('Ctrl Pts',(44.1665445877735,-54.7466107515317,
-171.649670743825));
#176515=CARTESIAN_POINT('Ctrl Pts',(44.2185163631217,-54.7405922226087,
-171.6496923846));
#176516=CARTESIAN_POINT('Ctrl Pts',(44.2454709099305,-54.7378737484813,
-171.649712753147));
#176517=CARTESIAN_POINT('Ctrl Pts',(44.3345799964015,-54.7302149256914,
-171.649800202596));
#176518=CARTESIAN_POINT('Ctrl Pts',(44.3968571027421,-54.7269903094681,
-171.649898655));
#176519=CARTESIAN_POINT('Ctrl Pts',(44.4753229318754,-54.7255987179305,
-171.649945978707));
#176520=CARTESIAN_POINT('Ctrl Pts',(44.4914595253056,-54.7254545924529,
-171.649951370195));
#176521=CARTESIAN_POINT('Ctrl Pts',(44.5716245853701,-54.7254442044783,
-171.649943153781));
#176522=CARTESIAN_POINT('Ctrl Pts',(44.63563633795,-54.7276720035778,-171.649830605824));
#176523=CARTESIAN_POINT('Ctrl Pts',(44.8100535271275,-54.7398514986523,
-171.649607168589));
#176524=CARTESIAN_POINT('Ctrl Pts',(44.9200103914804,-54.754242207499,-171.649613940458));
#176525=CARTESIAN_POINT('Ctrl Pts',(45.1075048885201,-54.7904085846999,
-171.649838422852));
#176526=CARTESIAN_POINT('Ctrl Pts',(45.1854986877315,-54.809021075728,-171.649951780061));
#176527=CARTESIAN_POINT('Ctrl Pts',(45.3711482014372,-54.8619988092884,
-171.649947090133));
#176528=CARTESIAN_POINT('Ctrl Pts',(45.4777060174367,-54.8996370242685,
-171.649926384802));
#176529=CARTESIAN_POINT('Ctrl Pts',(45.6764516340787,-54.9839240727134,
-171.649937563492));
#176530=CARTESIAN_POINT('Ctrl Pts',(45.7689217186597,-55.0294229071028,
-171.64995));
#176531=CARTESIAN_POINT('Ctrl Pts',(45.8586217441902,-55.08000002,-171.64995));
#176532=CARTESIAN_POINT('Ctrl Pts',(43.1572831724514,-54.58000002,-171.14995));
#176533=CARTESIAN_POINT('Ctrl Pts',(43.2795244112609,-54.58000002,-171.149950030568));
#176534=CARTESIAN_POINT('Ctrl Pts',(43.4015975649155,-54.58000002,-171.160610139865));
#176535=CARTESIAN_POINT('Ctrl Pts',(43.5235528170182,-54.58000002,-171.176313109178));
#176536=CARTESIAN_POINT('Ctrl Pts',(43.6257700730182,-54.5800000200001,
-171.189474612324));
#176537=CARTESIAN_POINT('Ctrl Pts',(43.7279044984682,-54.5800000200001,
-171.20618048842));
#176538=CARTESIAN_POINT('Ctrl Pts',(43.829985527596,-54.5800000200001,-171.223144870208));
#176539=CARTESIAN_POINT('Ctrl Pts',(43.9984923413722,-54.5800000200002,
-171.251148250928));
#176540=CARTESIAN_POINT('Ctrl Pts',(44.1669616089357,-54.5800000200002,
-171.278751491315));
#176541=CARTESIAN_POINT('Ctrl Pts',(44.3358012503099,-54.5800000200001,
-171.290923113046));
#176542=CARTESIAN_POINT('Ctrl Pts',(44.3914319971457,-54.5800000200001,
-171.294933524354));
#176543=CARTESIAN_POINT('Ctrl Pts',(44.4471029574805,-54.5800000200001,
-171.297268373358));
#176544=CARTESIAN_POINT('Ctrl Pts',(44.5028287572163,-54.58000002,-171.297388261734));
#176545=CARTESIAN_POINT('Ctrl Pts',(44.5028370935956,-54.58000002,-171.297388279669));
#176546=CARTESIAN_POINT('Ctrl Pts',(44.5028454299759,-54.58000002,-171.297388297554));
#176547=CARTESIAN_POINT('Ctrl Pts',(44.5028537663573,-54.58000002,-171.29738831539));
#176548=CARTESIAN_POINT('Ctrl Pts',(44.7276220562719,-54.58000002,-171.297869208197));
#176549=CARTESIAN_POINT('Ctrl Pts',(44.9531763212381,-54.5800000200004,
-171.261837296445));
#176550=CARTESIAN_POINT('Ctrl Pts',(45.1787623634369,-54.5800000200001,
-171.22433455003));
#176551=CARTESIAN_POINT('Ctrl Pts',(45.1788060542272,-54.5800000200001,
-171.224327286617));
#176552=CARTESIAN_POINT('Ctrl Pts',(45.178849745033,-54.5800000200001,-171.224320023146));
#176553=CARTESIAN_POINT('Ctrl Pts',(45.1788934358544,-54.5800000200001,
-171.224312759618));
#176554=CARTESIAN_POINT('Ctrl Pts',(45.294603484892,-54.58000002,-171.205076152327));
#176555=CARTESIAN_POINT('Ctrl Pts',(45.4103612459223,-54.58000002,-171.185995253716));
#176556=CARTESIAN_POINT('Ctrl Pts',(45.526508841826,-54.58000002,-171.171982248345));
#176557=CARTESIAN_POINT('Ctrl Pts',(45.6241378685054,-54.58000002,-171.160203476132));
#176558=CARTESIAN_POINT('Ctrl Pts',(45.722042620539,-54.58000002,-171.152008348194));
#176559=CARTESIAN_POINT('Ctrl Pts',(45.8204240164971,-54.58000002,-171.150287040904));
#176560=CARTESIAN_POINT('Ctrl Pts',(45.8331484827202,-54.58000002,-171.150064410231));
#176561=CARTESIAN_POINT('Ctrl Pts',(45.8458809158954,-54.58000002,-171.149950003086));
#176562=CARTESIAN_POINT('Ctrl Pts',(45.8586217441902,-54.58000002,-171.14995));
#176563=CARTESIAN_POINT('Origin',(0.,-12.9675000200281,-171.64995));
#176564=CARTESIAN_POINT('',(44.5079524583208,-60.2254524783487,-171.64995));
#176565=CARTESIAN_POINT('Origin',(44.5079524583208,-57.4754524783487,-171.64995));
#176566=CARTESIAN_POINT('Origin',(44.5079524583208,-57.4754524783487,-171.64995));
#176567=CARTESIAN_POINT('Ctrl Pts',(41.5,-58.6035812240168,-171.14995));
#176568=CARTESIAN_POINT('Ctrl Pts',(41.5,-58.6035812240167,-171.650011780221));
#176569=CARTESIAN_POINT('Ctrl Pts',(42.0000617764046,-58.6035812240168,
-171.649949996184));
#176570=CARTESIAN_POINT('Ctrl Pts',(41.5,-58.415688549198,-171.149950044589));
#176571=CARTESIAN_POINT('Ctrl Pts',(41.5,-58.4568531764745,-171.58399675791));
#176572=CARTESIAN_POINT('Ctrl Pts',(41.9298643117037,-58.4475344566842,
-171.649958724212));
#176573=CARTESIAN_POINT('Ctrl Pts',(41.5,-58.227785502943,-171.167360442076));
#176574=CARTESIAN_POINT('Ctrl Pts',(41.5,-58.2676804549564,-171.547558090573));
#176575=CARTESIAN_POINT('Ctrl Pts',(41.8681695534326,-58.2705723212599,
-171.649964230513));
#176576=CARTESIAN_POINT('Ctrl Pts',(41.5,-57.8520667952971,-171.199054581264));
#176577=CARTESIAN_POINT('Ctrl Pts',(41.5,-57.8827900893765,-171.511616746682));
#176578=CARTESIAN_POINT('Ctrl Pts',(41.7820591277973,-57.8880263314597,
-171.649970496006));
#176579=CARTESIAN_POINT('Ctrl Pts',(41.5,-57.6641810084405,-171.212413163406));
#176580=CARTESIAN_POINT('Ctrl Pts',(41.4999999999974,-57.6764631965623,
-171.507283264427));
#176581=CARTESIAN_POINT('Ctrl Pts',(41.7580490411455,-57.6823964313123,
-171.649971475853));
#176582=CARTESIAN_POINT('Ctrl Pts',(41.5,-57.2881262594105,-171.212471328128));
#176583=CARTESIAN_POINT('Ctrl Pts',(41.5000000000026,-57.275950831087,-171.507256427632));
#176584=CARTESIAN_POINT('Ctrl Pts',(41.7579337455091,-57.2700461805852,
-171.649971481651));
#176585=CARTESIAN_POINT('Ctrl Pts',(41.5,-57.0999570266663,-171.199145438258));
#176586=CARTESIAN_POINT('Ctrl Pts',(41.5,-57.0692704467351,-171.511552982749));
#176587=CARTESIAN_POINT('Ctrl Pts',(41.7818539242554,-57.0640562802561,
-171.649970508384));
#176588=CARTESIAN_POINT('Ctrl Pts',(41.5,-56.7235644715492,-171.167401493624));
#176589=CARTESIAN_POINT('Ctrl Pts',(41.5,-56.6836417097802,-171.547472271891));
#176590=CARTESIAN_POINT('Ctrl Pts',(41.8680165447745,-56.6807474451005,
-171.649964244171));
#176591=CARTESIAN_POINT('Ctrl Pts',(41.5,-56.5353526996975,-171.149950046396));
#176592=CARTESIAN_POINT('Ctrl Pts',(41.4999999999999,-56.494149705945,-171.583952704407));
#176593=CARTESIAN_POINT('Ctrl Pts',(41.929815802996,-56.5034783375505,-171.649958730482));
#176594=CARTESIAN_POINT('Ctrl Pts',(41.5,-56.3473237326807,-171.14995));
#176595=CARTESIAN_POINT('Ctrl Pts',(41.5,-56.3473237326807,-171.650011780221));
#176596=CARTESIAN_POINT('Ctrl Pts',(42.0000617764046,-56.3473237326807,
-171.649949996184));
#176597=CARTESIAN_POINT('Ctrl Pts',(42.,-58.6035812240168,-171.64995));
#176598=CARTESIAN_POINT('Ctrl Pts',(41.9586127577212,-58.5115728992447,
-171.64995));
#176599=CARTESIAN_POINT('Ctrl Pts',(41.9223200866005,-58.4173567491321,
-171.649936040447));
#176600=CARTESIAN_POINT('Ctrl Pts',(41.8579031946499,-58.2180944893019,
-171.649932806722));
#176601=CARTESIAN_POINT('Ctrl Pts',(41.8306620008006,-58.1129431414185,
-171.649968769067));
#176602=CARTESIAN_POINT('Ctrl Pts',(41.7951274186659,-57.9323775711288,
-171.649917110529));
#176603=CARTESIAN_POINT('Ctrl Pts',(41.7836058362706,-57.8577298063977,
-171.649879920008));
#176604=CARTESIAN_POINT('Ctrl Pts',(41.7636999883713,-57.6806798505214,
-171.649872834512));
#176605=CARTESIAN_POINT('Ctrl Pts',(41.7579524619681,-57.5781054625682,
-171.649950538122));
#176606=CARTESIAN_POINT('Ctrl Pts',(41.7579524619681,-57.3728595819387,
-171.649949462193));
#176607=CARTESIAN_POINT('Ctrl Pts',(41.7636932451378,-57.2703453579385,
-171.649869923244));
#176608=CARTESIAN_POINT('Ctrl Pts',(41.7835828980498,-57.0933348984401,
-171.649877908044));
#176609=CARTESIAN_POINT('Ctrl Pts',(41.7951032511141,-57.0186677636545,
-171.649916441382));
#176610=CARTESIAN_POINT('Ctrl Pts',(41.8306429216695,-56.8380335332052,
-171.649969369358));
#176611=CARTESIAN_POINT('Ctrl Pts',(41.857894634129,-56.7328337987611,-171.64993233013));
#176612=CARTESIAN_POINT('Ctrl Pts',(41.9223259722371,-56.5335329279263,
-171.649935735269));
#176613=CARTESIAN_POINT('Ctrl Pts',(41.9586161144825,-56.4393245950086,
-171.64995));
#176614=CARTESIAN_POINT('Ctrl Pts',(42.,-56.3473237326807,-171.64995));
#176615=CARTESIAN_POINT('Ctrl Pts',(41.5,-58.6035812240168,-171.14995));
#176616=CARTESIAN_POINT('Ctrl Pts',(41.5,-58.4156574039305,-171.149950044596));
#176617=CARTESIAN_POINT('Ctrl Pts',(41.4999999999992,-58.2278101348557,
-171.167358426711));
#176618=CARTESIAN_POINT('Ctrl Pts',(41.5000000000009,-58.0399262281501,
-171.183208448531));
#176619=CARTESIAN_POINT('Ctrl Pts',(41.5000000000009,-58.0397839854562,
-171.183220448228));
#176620=CARTESIAN_POINT('Ctrl Pts',(41.5000000000009,-58.039641742701,-171.183232446501));
#176621=CARTESIAN_POINT('Ctrl Pts',(41.5000000000009,-58.0394994998845,
-171.183244443348));
#176622=CARTESIAN_POINT('Ctrl Pts',(41.5000000000023,-57.8789705149695,
-171.196783556844));
#176623=CARTESIAN_POINT('Ctrl Pts',(41.4999999999993,-57.7184422672226,
-171.208492413787));
#176624=CARTESIAN_POINT('Ctrl Pts',(41.500000000002,-57.5579169091166,-171.211623701819));
#176625=CARTESIAN_POINT('Ctrl Pts',(41.5000000000025,-57.5306624002125,
-171.21215534192));
#176626=CARTESIAN_POINT('Ctrl Pts',(41.5000000000032,-57.5034079726048,
-171.212439843791));
#176627=CARTESIAN_POINT('Ctrl Pts',(41.5000000000045,-57.4761536342535,
-171.212444366368));
#176628=CARTESIAN_POINT('Ctrl Pts',(41.5000000000045,-57.4759114394356,
-171.212444406558));
#176629=CARTESIAN_POINT('Ctrl Pts',(41.5000000000045,-57.4756692446243,
-171.212444424596));
#176630=CARTESIAN_POINT('Ctrl Pts',(41.5000000000045,-57.4754270498201,
-171.212444420506));
#176631=CARTESIAN_POINT('Ctrl Pts',(41.5000000000123,-57.3141767266989,
-171.21244169735));
#176632=CARTESIAN_POINT('Ctrl Pts',(41.5000000000007,-57.1529297994966,
-171.202628065339));
#176633=CARTESIAN_POINT('Ctrl Pts',(41.5000000000001,-56.991684015905,-171.189830777414));
#176634=CARTESIAN_POINT('Ctrl Pts',(41.5,-56.9650429029001,-171.187716402786));
#176635=CARTESIAN_POINT('Ctrl Pts',(41.5,-56.9384018139027,-171.185520466728));
#176636=CARTESIAN_POINT('Ctrl Pts',(41.5,-56.9117607329797,-171.183273657174));
#176637=CARTESIAN_POINT('Ctrl Pts',(41.5,-56.9116320467988,-171.18326280426));
#176638=CARTESIAN_POINT('Ctrl Pts',(41.5,-56.9115033606235,-171.183251950612));
#176639=CARTESIAN_POINT('Ctrl Pts',(41.5,-56.9113746744539,-171.183241096235));
#176640=CARTESIAN_POINT('Ctrl Pts',(41.5000000000001,-56.7724125203339,
-171.171519963662));
#176641=CARTESIAN_POINT('Ctrl Pts',(41.5,-56.6334506983205,-171.158942972401));
#176642=CARTESIAN_POINT('Ctrl Pts',(41.5,-56.494486471781,-171.153174108112));
#176643=CARTESIAN_POINT('Ctrl Pts',(41.5,-56.4454325541955,-171.151137717881));
#176644=CARTESIAN_POINT('Ctrl Pts',(41.5,-56.3963783401914,-171.149950012104));
#176645=CARTESIAN_POINT('Ctrl Pts',(41.5,-56.3473237326807,-171.14995));
#176646=CARTESIAN_POINT('Origin',(45.5612236321975,-62.7713643393447,-171.64995));
#176647=CARTESIAN_POINT('',(26.0394480946395,-65.5149709682656,-179.39995));
#176648=CARTESIAN_POINT('',(26.0394480946395,-65.5149709682656,-171.64995));
#176649=CARTESIAN_POINT('',(44.628608857647,-62.9024347982158,-179.39995));
#176650=CARTESIAN_POINT('',(44.628608857647,-62.9024347982158,-179.39995));
#176651=CARTESIAN_POINT('',(44.628608857647,-62.9024347982158,-171.64995));
#176652=CARTESIAN_POINT('Origin',(44.2110895547669,-59.9316305919911,-171.64995));
#176653=CARTESIAN_POINT('',(46.2674193015002,-62.1160087581289,-179.39995));
#176654=CARTESIAN_POINT('Origin',(44.2110895547669,-59.9316305919911,-179.39995));
#176655=CARTESIAN_POINT('',(46.2674193015002,-62.1160087581289,-171.64995));
#176656=CARTESIAN_POINT('Origin',(0.,-12.9675000200281,-171.64995));
#176657=CARTESIAN_POINT('',(49.148508738101,-59.2349193215281,-179.39995));
#176658=CARTESIAN_POINT('Origin',(0.,-12.9675000200281,-179.39995));
#176659=CARTESIAN_POINT('',(49.148508738101,-59.2349193215281,-171.64995));
#176660=CARTESIAN_POINT('Origin',(46.9641305719631,-57.1785895747948,-171.64995));
#176661=CARTESIAN_POINT('',(49.9349347781878,-57.596108877675,-179.39995));
#176662=CARTESIAN_POINT('Origin',(46.9641305719631,-57.1785895747948,-179.39995));
#176663=CARTESIAN_POINT('',(49.9349347781878,-57.596108877675,-171.64995));
#176664=CARTESIAN_POINT('Origin',(52.6124803109501,-38.5443824635529,-171.64995));
#176665=CARTESIAN_POINT('',(52.5050296388285,-39.3089337226171,-179.39995));
#176666=CARTESIAN_POINT('',(52.5050296388285,-39.3089337226171,-179.39995));
#176667=CARTESIAN_POINT('',(52.5050296388285,-39.3089337226171,-171.64995));
#176668=CARTESIAN_POINT('Origin',(57.4563699825363,-40.0047992274175,-179.64995));
#176669=CARTESIAN_POINT('',(52.9322463618642,-37.8758780299853,-179.39995));
#176670=CARTESIAN_POINT('',(52.9322463618642,-37.8758780299853,-179.64995));
#176671=CARTESIAN_POINT('Origin',(57.4563699825363,-40.0047992274175,-179.39995));
#176672=CARTESIAN_POINT('Origin',(0.,-12.9675000200281,-179.64995));
#176673=CARTESIAN_POINT('',(52.9322463618642,11.9408779899289,-179.39995));
#176674=CARTESIAN_POINT('',(52.9322463618642,11.9408779899289,-179.64995));
#176675=CARTESIAN_POINT('Origin',(0.,-12.9675000200281,-179.39995));
#176676=CARTESIAN_POINT('Origin',(57.4563699825364,14.0697991873612,-179.64995));
#176677=CARTESIAN_POINT('',(52.5050296388285,13.3739336825608,-179.39995));
#176678=CARTESIAN_POINT('Origin',(57.4563699825364,14.0697991873612,-179.39995));
#176679=CARTESIAN_POINT('',(52.5050296388285,13.3739336825608,-171.64995));
#176680=CARTESIAN_POINT('Origin',(52.6124803109502,12.6093824234965,-171.64995));
#176681=CARTESIAN_POINT('',(49.9349347781878,31.6611088376188,-179.39995));
#176682=CARTESIAN_POINT('',(49.9349347781878,31.6611088376188,-179.39995));
#176683=CARTESIAN_POINT('',(49.9349347781878,31.6611088376188,-171.64995));
#176684=CARTESIAN_POINT('Origin',(46.9641305719631,31.2435895347386,-171.64995));
#176685=CARTESIAN_POINT('',(49.1485087381009,33.2999192814719,-179.39995));
#176686=CARTESIAN_POINT('Origin',(46.9641305719631,31.2435895347386,-179.39995));
#176687=CARTESIAN_POINT('',(49.1485087381009,33.2999192814719,-171.64995));
#176688=CARTESIAN_POINT('Origin',(0.,-12.9675000200281,-171.64995));
#176689=CARTESIAN_POINT('',(46.2674193015002,36.1810087180727,-179.39995));
#176690=CARTESIAN_POINT('Origin',(0.,-12.9675000200281,-179.39995));
#176691=CARTESIAN_POINT('',(46.2674193015002,36.1810087180727,-171.64995));
#176692=CARTESIAN_POINT('Origin',(44.2110895547669,33.9966305519348,-171.64995));
#176693=CARTESIAN_POINT('',(44.628608857647,36.9674347581595,-179.39995));
#176694=CARTESIAN_POINT('Origin',(44.2110895547669,33.9966305519348,-179.39995));
#176695=CARTESIAN_POINT('',(44.628608857647,36.9674347581595,-171.64995));
#176696=CARTESIAN_POINT('Origin',(45.5612236321975,36.8363642992885,-171.64995));
#176697=CARTESIAN_POINT('',(26.3414337025898,39.5375296188,-179.39995));
#176698=CARTESIAN_POINT('',(26.3414337025898,39.5375296188,-177.84995));
#176699=CARTESIAN_POINT('',(26.3414337025898,39.5375296188,-171.64995));
#176700=CARTESIAN_POINT('',(38.43041344952,37.8385343144662,-177.84995));
#176701=CARTESIAN_POINT('',(45.5612236321975,36.8363642992885,-177.84995));
#176702=CARTESIAN_POINT('',(41.93041344952,37.3466413930079,-174.34995));
#176703=CARTESIAN_POINT('Ctrl Pts',(38.43041344952,37.8385343144662,-177.84995));
#176704=CARTESIAN_POINT('Ctrl Pts',(38.8886449769195,37.7741340731185,-177.849949999987));
#176705=CARTESIAN_POINT('Ctrl Pts',(39.3465310504406,37.7097823821472,-177.758854365991));
#176706=CARTESIAN_POINT('Ctrl Pts',(39.7698054627978,37.6502950429264,-177.58352836379));
#176707=CARTESIAN_POINT('Ctrl Pts',(40.193079875155,37.5908077037056,-177.408202361589));
#176708=CARTESIAN_POINT('Ctrl Pts',(40.5813269737971,37.5362431323916,-177.148783944032));
#176709=CARTESIAN_POINT('Ctrl Pts',(40.9052871836729,37.4907134940853,-176.824823734153));
#176710=CARTESIAN_POINT('Ctrl Pts',(41.2292473935486,37.445183855779,-176.500863524274));
#176711=CARTESIAN_POINT('Ctrl Pts',(41.4886658111382,37.4087249748338,-176.112616425556));
#176712=CARTESIAN_POINT('Ctrl Pts',(41.6639918133095,37.3840845121436,-175.689342013278));
#176713=CARTESIAN_POINT('Ctrl Pts',(41.8393178154807,37.3594440494534,-175.266067601));
#176714=CARTESIAN_POINT('Ctrl Pts',(41.9304134495165,37.3466413930083,-174.808181527339));
#176715=CARTESIAN_POINT('Ctrl Pts',(41.93041344952,37.3466413930079,-174.34995));
#176716=CARTESIAN_POINT('',(41.93041344952,37.3466413930079,-171.64995));
#176717=CARTESIAN_POINT('',(26.3414337025898,39.5375296188,-179.39995));
#176718=CARTESIAN_POINT('Ctrl Pts',(41.5,37.8417754273786,-174.34995));
#176719=CARTESIAN_POINT('Ctrl Pts',(41.5,37.4071320584705,-174.34995));
#176720=CARTESIAN_POINT('Ctrl Pts',(41.93041344952,37.3466413930079,-174.34995));
#176721=CARTESIAN_POINT('Ctrl Pts',(41.5,37.8417754273818,-174.742719880575));
#176722=CARTESIAN_POINT('Ctrl Pts',(41.4999999999921,37.4071320584705,-174.750729116851));
#176723=CARTESIAN_POINT('Ctrl Pts',(41.9304134495165,37.3466413930083,-174.808181527339));
#176724=CARTESIAN_POINT('Ctrl Pts',(41.4219180279654,37.8545780838243,-175.135193658002));
#176725=CARTESIAN_POINT('Ctrl Pts',(41.418170761701,37.4186324079233,-175.152286591264));
#176726=CARTESIAN_POINT('Ctrl Pts',(41.8393178154807,37.3594440494534,-175.266067601));
#176727=CARTESIAN_POINT('Ctrl Pts',(41.1213591671024,37.9038590092046,-175.860806936189));
#176728=CARTESIAN_POINT('Ctrl Pts',(41.1060831277358,37.4624934645027,-175.889590467068));
#176729=CARTESIAN_POINT('Ctrl Pts',(41.4886658111382,37.4087249748338,-176.112616425556));
#176730=CARTESIAN_POINT('Ctrl Pts',(40.8990005234543,37.9403178901501,-176.193590163665));
#176731=CARTESIAN_POINT('Ctrl Pts',(40.8743194488686,37.4950657253844,-176.226515658809));
#176732=CARTESIAN_POINT('Ctrl Pts',(41.2292473935486,37.445183855779,-176.500863524274));
#176733=CARTESIAN_POINT('Ctrl Pts',(40.343640163665,38.0313771667621,-176.748950523454));
#176734=CARTESIAN_POINT('Ctrl Pts',(40.3016108905592,37.5755546642088,-176.782638117262));
#176735=CARTESIAN_POINT('Ctrl Pts',(40.5813269737971,37.5362431323916,-177.148783944032));
#176736=CARTESIAN_POINT('Ctrl Pts',(40.0108569362568,38.0859417380754,-176.971309167074));
#176737=CARTESIAN_POINT('Ctrl Pts',(39.9585494594759,37.6237688040866,-177.001555340038));
#176738=CARTESIAN_POINT('Ctrl Pts',(40.193079875155,37.5908077037056,-177.408202361589));
#176739=CARTESIAN_POINT('Ctrl Pts',(39.2852436579338,38.204916416519,-177.271868027993));
#176740=CARTESIAN_POINT('Ctrl Pts',(39.218856185771,37.7277259142,-177.290648705564));
#176741=CARTESIAN_POINT('Ctrl Pts',(39.3465310504406,37.7097823821472,-177.758854365991));
#176742=CARTESIAN_POINT('Ctrl Pts',(38.8927698806272,38.2692681074913,-177.34995));
#176743=CARTESIAN_POINT('Ctrl Pts',(38.8208550398785,37.7836613274466,-177.358977353131));
#176744=CARTESIAN_POINT('Ctrl Pts',(38.8886449769195,37.7741340731185,-177.849949999987));
#176745=CARTESIAN_POINT('Ctrl Pts',(38.5,38.333668348837,-177.34995));
#176746=CARTESIAN_POINT('Ctrl Pts',(38.43041344952,37.8385343144661,-177.34995));
#176747=CARTESIAN_POINT('Ctrl Pts',(38.43041344952,37.8385343144662,-177.84995));
#176748=CARTESIAN_POINT('',(41.5,37.8417754273786,-174.34995));
#176749=CARTESIAN_POINT('Origin',(42.,37.8417754273786,-174.34995));
#176750=CARTESIAN_POINT('',(38.5,38.333668348837,-177.34995));
#176751=CARTESIAN_POINT('Origin',(38.5,38.333668348837,-177.84995));
#176752=CARTESIAN_POINT('Ctrl Pts',(41.5,37.8417754273786,-174.34995));
#176753=CARTESIAN_POINT('Ctrl Pts',(41.5,37.8417754273786,-174.476353976316));
#176754=CARTESIAN_POINT('Ctrl Pts',(41.4919114500808,37.8431014152902,-174.603274421342));
#176755=CARTESIAN_POINT('Ctrl Pts',(41.4757304211612,37.8457540208828,-174.729690050826));
#176756=CARTESIAN_POINT('Ctrl Pts',(41.4680748448541,37.8470090229366,-174.789499875202));
#176757=CARTESIAN_POINT('Ctrl Pts',(41.4586080657167,37.8485609393631,-174.849195979142));
#176758=CARTESIAN_POINT('Ctrl Pts',(41.4473309666377,37.8504096236584,-174.908666369613));
#176759=CARTESIAN_POINT('Ctrl Pts',(41.4297746293963,37.85328767986,-175.001250661341));
#176760=CARTESIAN_POINT('Ctrl Pts',(41.4078298483949,37.8568852355436,-175.093293139518));
#176761=CARTESIAN_POINT('Ctrl Pts',(41.3814995882027,37.8612023039407,-175.184367198324));
#176762=CARTESIAN_POINT('Ctrl Pts',(41.371452626058,37.862849588185,-175.219118758487));
#176763=CARTESIAN_POINT('Ctrl Pts',(41.360858123554,37.8645866920548,-175.253429957384));
#176764=CARTESIAN_POINT('Ctrl Pts',(41.3496247022485,37.8664286294454,-175.28762251975));
#176765=CARTESIAN_POINT('Ctrl Pts',(41.3385105141439,37.8682510162392,-175.321452157185));
#176766=CARTESIAN_POINT('Ctrl Pts',(41.3267707930063,37.8701760402071,-175.355165937406));
#176767=CARTESIAN_POINT('Ctrl Pts',(41.3142698257931,37.8722259837527,-175.389059282268));
#176768=CARTESIAN_POINT('Ctrl Pts',(41.306292887867,37.8735340643305,-175.410686817439));
#176769=CARTESIAN_POINT('Ctrl Pts',(41.2980050551031,37.8748931622609,-175.432387137017));
#176770=CARTESIAN_POINT('Ctrl Pts',(41.2893609525011,37.8763107253537,-175.454232639964));
#176771=CARTESIAN_POINT('Ctrl Pts',(41.2835806796571,37.8772586434694,-175.468840630321));
#176772=CARTESIAN_POINT('Ctrl Pts',(41.2776735291647,37.8782273521849,-175.48343068445));
#176773=CARTESIAN_POINT('Ctrl Pts',(41.2716385658268,37.8792170058608,-175.498000373649));
#176774=CARTESIAN_POINT('Ctrl Pts',(41.236613156753,37.8849607068411,-175.582559184651));
#176775=CARTESIAN_POINT('Ctrl Pts',(41.1972870501281,37.8914091716528,-175.666416279207));
#176776=CARTESIAN_POINT('Ctrl Pts',(41.153627526666,37.8985679655939,-175.749123315229));
#176777=CARTESIAN_POINT('Ctrl Pts',(41.1114124456556,37.905489916229,-175.829094051255));
#176778=CARTESIAN_POINT('Ctrl Pts',(41.06514597395,37.9130759664727,-175.907989464207));
#176779=CARTESIAN_POINT('Ctrl Pts',(41.0148201132632,37.9213276113521,-175.985363378084));
#176780=CARTESIAN_POINT('Ctrl Pts',(40.9626287142217,37.9298851379354,-176.06560547945));
#176781=CARTESIAN_POINT('Ctrl Pts',(40.9060697862906,37.9391587833669,-176.144214115591));
#176782=CARTESIAN_POINT('Ctrl Pts',(40.8451545165363,37.9491467133671,-176.220648295229));
#176783=CARTESIAN_POINT('Ctrl Pts',(40.7909989817862,37.9580262881009,-176.288600614708));
#176784=CARTESIAN_POINT('Ctrl Pts',(40.7333998072024,37.9674704968541,-176.354834221104));
#176785=CARTESIAN_POINT('Ctrl Pts',(40.6723886669702,37.9774741461908,-176.418927468631));
#176786=CARTESIAN_POINT('Ctrl Pts',(40.6647732100798,37.9787228093034,-176.426927636496));
#176787=CARTESIAN_POINT('Ctrl Pts',(40.6571046345291,37.9799801819804,-176.434894399285));
#176788=CARTESIAN_POINT('Ctrl Pts',(40.6493830370906,37.9812462483545,-176.442826888852));
#176789=CARTESIAN_POINT('Ctrl Pts',(40.6433862987247,37.9822294994059,-176.448987410026));
#176790=CARTESIAN_POINT('Ctrl Pts',(40.6368004697369,37.9833093402939,-176.455693039846));
#176791=CARTESIAN_POINT('Ctrl Pts',(40.6307040241344,37.9843089345486,-176.461844450969));
#176792=CARTESIAN_POINT('Ctrl Pts',(40.6273684653236,37.9848558442795,-176.46521008316));
#176793=CARTESIAN_POINT('Ctrl Pts',(40.624180151531,37.9853786095184,-176.468410535592));
#176794=CARTESIAN_POINT('Ctrl Pts',(40.6213203422155,37.9858475093267,-176.471270344904));
#176795=CARTESIAN_POINT('Ctrl Pts',(40.5709024849344,37.9941141176937,-176.521688202121));
#176796=CARTESIAN_POINT('Ctrl Pts',(40.5175232725426,38.0028663790502,-176.571427643008));
#176797=CARTESIAN_POINT('Ctrl Pts',(40.4611036304162,38.012117202431,-176.620119132926));
#176798=CARTESIAN_POINT('Ctrl Pts',(40.4062711116874,38.0211077937777,-176.667440897692));
#176799=CARTESIAN_POINT('Ctrl Pts',(40.348566681604,38.0305693139387,-176.713772847727));
#176800=CARTESIAN_POINT('Ctrl Pts',(40.2879492542279,38.0405084467926,-176.758738723489));
#176801=CARTESIAN_POINT('Ctrl Pts',(40.2508731893274,38.0465876215562,-176.786241667778));
#176802=CARTESIAN_POINT('Ctrl Pts',(40.2127079839217,38.0528453708976,-176.813232834678));
#176803=CARTESIAN_POINT('Ctrl Pts',(40.1734506493455,38.059282172562,-176.839618952926));
#176804=CARTESIAN_POINT('Ctrl Pts',(40.1114897149355,38.0694415542431,-176.881264891444));
#176805=CARTESIAN_POINT('Ctrl Pts',(40.0468039828495,38.0800477054872,-176.921407207624));
#176806=CARTESIAN_POINT('Ctrl Pts',(39.9794042488894,38.0910988561683,-176.959651363111));
#176807=CARTESIAN_POINT('Ctrl Pts',(39.9127899593656,38.1020212219966,-176.997449839404));
#176808=CARTESIAN_POINT('Ctrl Pts',(39.8435235796991,38.1133784359477,-177.033394563102));
#176809=CARTESIAN_POINT('Ctrl Pts',(39.7716539135189,38.1251624959684,-177.067065073469));
#176810=CARTESIAN_POINT('Ctrl Pts',(39.7312690241559,38.1317841763723,-177.085985153501));
#176811=CARTESIAN_POINT('Ctrl Pts',(39.6900628025815,38.1385405259433,-177.104186447972));
#176812=CARTESIAN_POINT('Ctrl Pts',(39.6480502970953,38.1454290772972,-177.121588597534));
#176813=CARTESIAN_POINT('Ctrl Pts',(39.6400227671394,38.1467453056846,-177.124913709314));
#176814=CARTESIAN_POINT('Ctrl Pts',(39.6319659013663,38.1480663440989,-177.128209611011));
#176815=CARTESIAN_POINT('Ctrl Pts',(39.6238797774804,38.1493921797995,-177.131475878803));
#176816=CARTESIAN_POINT('Ctrl Pts',(39.6206230494417,38.1499261669559,-177.132791384978));
#176817=CARTESIAN_POINT('Ctrl Pts',(39.6173615800294,38.1504609315351,-177.134102082276));
#176818=CARTESIAN_POINT('Ctrl Pts',(39.6140953721306,38.1509963995422,-177.135407943764));
#176819=CARTESIAN_POINT('Ctrl Pts',(39.6108291642318,38.1515318675494,-177.136713805253));
#176820=CARTESIAN_POINT('Ctrl Pts',(39.6061167246918,38.1523044534494,-177.138585218931));
#176821=CARTESIAN_POINT('Ctrl Pts',(39.6042825755168,38.152605166686,-177.139310978034));
#176822=CARTESIAN_POINT('Ctrl Pts',(39.5690593443383,38.1583801014609,-177.153248547029));
#176823=CARTESIAN_POINT('Ctrl Pts',(39.530961535174,38.1646266368639,-177.167548422363));
#176824=CARTESIAN_POINT('Ctrl Pts',(39.4899041451713,38.1713585854016,-177.181880372341));
#176825=CARTESIAN_POINT('Ctrl Pts',(39.4495809627956,38.177970150058,-177.195956031625));
#176826=CARTESIAN_POINT('Ctrl Pts',(39.4064025243435,38.1850500171143,-177.210062601644));
#176827=CARTESIAN_POINT('Ctrl Pts',(39.3603028130147,38.1926088913928,-177.223839844921));
#176828=CARTESIAN_POINT('Ctrl Pts',(39.3156809756124,38.1999254417415,-177.237175414528));
#176829=CARTESIAN_POINT('Ctrl Pts',(39.26832167597,38.2076908595149,-177.250202308661));
#176830=CARTESIAN_POINT('Ctrl Pts',(39.2181864360695,38.2159113437581,-177.262550300708));
#176831=CARTESIAN_POINT('Ctrl Pts',(39.1970979178763,38.2193691477272,-177.267744269171));
#176832=CARTESIAN_POINT('Ctrl Pts',(39.1755185545334,38.2229074170752,-177.272817588752));
#176833=CARTESIAN_POINT('Ctrl Pts',(39.1534469930419,38.2265263653629,-177.277740366434));
#176834=CARTESIAN_POINT('Ctrl Pts',(39.1037587962994,38.2346734561155,-177.288822679123));
#176835=CARTESIAN_POINT('Ctrl Pts',(39.0515724039289,38.2432301617833,-177.299144914683));
#176836=CARTESIAN_POINT('Ctrl Pts',(38.9968918500243,38.2521958209189,-177.308339389731));
#176837=CARTESIAN_POINT('Ctrl Pts',(38.9435492322889,38.2609421062775,-177.317308892283));
#176838=CARTESIAN_POINT('Ctrl Pts',(38.8878326440064,38.2700776380719,-177.325205101624));
#176839=CARTESIAN_POINT('Ctrl Pts',(38.8297783760627,38.2795964658924,-177.331651494106));
#176840=CARTESIAN_POINT('Ctrl Pts',(38.7739147618162,38.2887561046972,-177.337854634644));
#176841=CARTESIAN_POINT('Ctrl Pts',(38.7158863278997,38.2982706966594,-177.342715195092));
#176842=CARTESIAN_POINT('Ctrl Pts',(38.6557601433083,38.3081292448576,-177.345865997974));
#176843=CARTESIAN_POINT('Ctrl Pts',(38.6052967544591,38.3164034394467,-177.348510439695));
#176844=CARTESIAN_POINT('Ctrl Pts',(38.5533561382533,38.3249198465959,-177.34995));
#176845=CARTESIAN_POINT('Ctrl Pts',(38.5,38.333668348837,-177.34995));
#176846=CARTESIAN_POINT('Origin',(42.,37.8417754273786,-171.64995));
#176847=CARTESIAN_POINT('',(41.5,37.8417754273786,-172.64995));
#176848=CARTESIAN_POINT('Origin',(42.,37.8417754273786,-172.64995));
#176849=CARTESIAN_POINT('',(41.5,37.8417754273786,-92.34995));
#176850=CARTESIAN_POINT('Ctrl Pts',(41.5,36.3270340686007,-171.14995));
#176851=CARTESIAN_POINT('Ctrl Pts',(41.5,36.3270340686007,-171.64995));
#176852=CARTESIAN_POINT('Ctrl Pts',(42.,36.3270340686007,-171.64995));
#176853=CARTESIAN_POINT('Ctrl Pts',(41.5,36.5253489879757,-171.149950000016));
#176854=CARTESIAN_POINT('Ctrl Pts',(41.5,36.4592824973649,-171.640924254979));
#176855=CARTESIAN_POINT('Ctrl Pts',(41.9908895000013,36.460524412126,-171.64995));
#176856=CARTESIAN_POINT('Ctrl Pts',(41.5,36.7235144279567,-171.18899099047));
#176857=CARTESIAN_POINT('Ctrl Pts',(41.5,36.5965520755147,-171.658003579003));
#176858=CARTESIAN_POINT('Ctrl Pts',(41.9817858670191,36.5939141376228,-171.675977326981));
#176859=CARTESIAN_POINT('Ctrl Pts',(41.5,37.0898865538897,-171.339270411997));
#176860=CARTESIAN_POINT('Ctrl Pts',(41.5,36.8549873364184,-171.746711574348));
#176861=CARTESIAN_POINT('Ctrl Pts',(41.9649548930127,36.840527660716,-171.776163607997));
#176862=CARTESIAN_POINT('Ctrl Pts',(41.5,37.2579134125323,-171.450449746589));
#176863=CARTESIAN_POINT('Ctrl Pts',(41.4999999999986,36.9765510525756,-171.817687494207));
#176864=CARTESIAN_POINT('Ctrl Pts',(41.9572358131754,36.9536304124011,-171.850283164392));
#176865=CARTESIAN_POINT('Ctrl Pts',(41.5,37.5383224977403,-171.728129909852));
#176866=CARTESIAN_POINT('Ctrl Pts',(41.5000000000014,37.1809962719461,-172.003556970024));
#176867=CARTESIAN_POINT('Ctrl Pts',(41.9443539433771,37.1423802312719,-172.035403273234));
#176868=CARTESIAN_POINT('Ctrl Pts',(41.5,37.6505944553831,-171.894521542842));
#176869=CARTESIAN_POINT('Ctrl Pts',(41.5,37.2645653642152,-172.118296873734));
#176870=CARTESIAN_POINT('Ctrl Pts',(41.9391962191204,37.2179530739059,-172.146331028561));
#176871=CARTESIAN_POINT('Ctrl Pts',(41.5,37.8023507586648,-172.257328160063));
#176872=CARTESIAN_POINT('Ctrl Pts',(41.5,37.3773763733446,-172.371853931892));
#176873=CARTESIAN_POINT('Ctrl Pts',(41.9322246014265,37.3201037397322,-172.388202106709));
#176874=CARTESIAN_POINT('Ctrl Pts',(41.5,37.8417754273637,-172.453565067926));
#176875=CARTESIAN_POINT('Ctrl Pts',(41.5,37.4071320584576,-172.511015867074));
#176876=CARTESIAN_POINT('Ctrl Pts',(41.9304134495219,37.3466413930076,-172.51902671195));
#176877=CARTESIAN_POINT('Ctrl Pts',(41.5,37.8417754273786,-172.64995));
#176878=CARTESIAN_POINT('Ctrl Pts',(41.5,37.4071320584705,-172.64995));
#176879=CARTESIAN_POINT('Ctrl Pts',(41.93041344952,37.3466413930079,-172.64995));
#176880=CARTESIAN_POINT('',(41.5,36.3270340686007,-171.14995));
#176881=CARTESIAN_POINT('Origin',(42.,36.3270340686007,-171.14995));
#176882=CARTESIAN_POINT('Ctrl Pts',(41.5,36.3270340686007,-171.14995));
#176883=CARTESIAN_POINT('Ctrl Pts',(41.5,36.5253489879757,-171.149950000016));
#176884=CARTESIAN_POINT('Ctrl Pts',(41.5,36.7235144279567,-171.18899099047));
#176885=CARTESIAN_POINT('Ctrl Pts',(41.5,37.0898865538897,-171.339270411997));
#176886=CARTESIAN_POINT('Ctrl Pts',(41.5,37.2579134125323,-171.450449746589));
#176887=CARTESIAN_POINT('Ctrl Pts',(41.5,37.5383224977403,-171.728129909852));
#176888=CARTESIAN_POINT('Ctrl Pts',(41.5,37.6505944553831,-171.894521542842));
#176889=CARTESIAN_POINT('Ctrl Pts',(41.5,37.8023507586648,-172.257328160063));
#176890=CARTESIAN_POINT('Ctrl Pts',(41.5,37.8417754273637,-172.453565067926));
#176891=CARTESIAN_POINT('Ctrl Pts',(41.5,37.8417754273786,-172.64995));
#176892=CARTESIAN_POINT('Origin',(42.,58.91999998,-171.14995));
#176893=CARTESIAN_POINT('',(41.5,32.6685811839606,-171.14995));
#176894=CARTESIAN_POINT('Origin',(42.,32.6685811839606,-171.14995));
#176895=CARTESIAN_POINT('',(41.5,36.3973044859519,-171.14995));
#176896=CARTESIAN_POINT('Ctrl Pts',(41.5,30.4123236926243,-171.14995));
#176897=CARTESIAN_POINT('Ctrl Pts',(41.5,30.4123236926244,-171.650011780222));
#176898=CARTESIAN_POINT('Ctrl Pts',(42.0000617764046,30.4123236926243,-171.649949996184));
#176899=CARTESIAN_POINT('Ctrl Pts',(41.5,30.6002163674433,-171.149950044589));
#176900=CARTESIAN_POINT('Ctrl Pts',(41.5,30.5590517401679,-171.583996757915));
#176901=CARTESIAN_POINT('Ctrl Pts',(41.929864311704,30.5683704599569,-171.649958724212));
#176902=CARTESIAN_POINT('Ctrl Pts',(41.5,30.7881194136978,-171.167360442076));
#176903=CARTESIAN_POINT('Ctrl Pts',(41.5,30.7482244616852,-171.547558090571));
#176904=CARTESIAN_POINT('Ctrl Pts',(41.8681695534321,30.7453325953812,-171.649964230513));
#176905=CARTESIAN_POINT('Ctrl Pts',(41.5,31.1638381213445,-171.199054581264));
#176906=CARTESIAN_POINT('Ctrl Pts',(41.5,31.1331148272644,-171.511616746684));
#176907=CARTESIAN_POINT('Ctrl Pts',(41.782059127798,31.1278785851814,-171.649970496006));
#176908=CARTESIAN_POINT('Ctrl Pts',(41.5,31.3517239082014,-171.212413163406));
#176909=CARTESIAN_POINT('Ctrl Pts',(41.5000000000007,31.3394417200798,-171.507283264433));
#176910=CARTESIAN_POINT('Ctrl Pts',(41.7580490411456,31.3335084853296,-171.649971475853));
#176911=CARTESIAN_POINT('Ctrl Pts',(41.5,31.72777865723,-171.212471328128));
#176912=CARTESIAN_POINT('Ctrl Pts',(41.4999999999994,31.739954085554,-171.507256427626));
#176913=CARTESIAN_POINT('Ctrl Pts',(41.7579337455091,31.7458587360553,-171.649971481651));
#176914=CARTESIAN_POINT('Ctrl Pts',(41.5,31.9159478899749,-171.199145438258));
#176915=CARTESIAN_POINT('Ctrl Pts',(41.5000000000001,31.9466344699074,-171.511552982749));
#176916=CARTESIAN_POINT('Ctrl Pts',(41.7818539242555,31.9518486363857,-171.649970508384));
#176917=CARTESIAN_POINT('Ctrl Pts',(41.5,32.2923404450921,-171.167401493624));
#176918=CARTESIAN_POINT('Ctrl Pts',(41.5,32.3322632068598,-171.547472271891));
#176919=CARTESIAN_POINT('Ctrl Pts',(41.8680165447745,32.3351574715402,-171.649964244171));
#176920=CARTESIAN_POINT('Ctrl Pts',(41.5,32.4805522169437,-171.149950046396));
#176921=CARTESIAN_POINT('Ctrl Pts',(41.5,32.5217552106974,-171.583952704406));
#176922=CARTESIAN_POINT('Ctrl Pts',(41.9298158029953,32.5124265790917,-171.649958730482));
#176923=CARTESIAN_POINT('Ctrl Pts',(41.5,32.6685811839606,-171.14995));
#176924=CARTESIAN_POINT('Ctrl Pts',(41.5,32.6685811839606,-171.650011780222));
#176925=CARTESIAN_POINT('Ctrl Pts',(42.0000617764046,32.6685811839606,-171.649949996184));
#176926=CARTESIAN_POINT('',(41.5,30.4123236926243,-171.14995));
#176927=CARTESIAN_POINT('Origin',(42.,30.4123236926243,-171.14995));
#176928=CARTESIAN_POINT('Ctrl Pts',(42.,30.4123236926244,-171.64995));
#176929=CARTESIAN_POINT('Ctrl Pts',(41.9586127577213,30.5043320173964,-171.64995));
#176930=CARTESIAN_POINT('Ctrl Pts',(41.9223200866006,30.5985481675088,-171.649936040447));
#176931=CARTESIAN_POINT('Ctrl Pts',(41.8579031946499,30.7978104273391,-171.649932806722));
#176932=CARTESIAN_POINT('Ctrl Pts',(41.8306620008007,30.9029617752221,-171.649968769066));
#176933=CARTESIAN_POINT('Ctrl Pts',(41.7951274186661,31.0835273455115,-171.649917110529));
#176934=CARTESIAN_POINT('Ctrl Pts',(41.7836058362707,31.1581751102427,-171.649879920008));
#176935=CARTESIAN_POINT('Ctrl Pts',(41.7636999883716,31.3352250661168,-171.649872834512));
#176936=CARTESIAN_POINT('Ctrl Pts',(41.7579524619681,31.4377994540704,-171.649950538122));
#176937=CARTESIAN_POINT('Ctrl Pts',(41.7579524619681,31.6430453346997,-171.649949462193));
#176938=CARTESIAN_POINT('Ctrl Pts',(41.7636932451375,31.7455595586994,-171.649869923244));
#176939=CARTESIAN_POINT('Ctrl Pts',(41.7835828980497,31.9225700182006,-171.649877908044));
#176940=CARTESIAN_POINT('Ctrl Pts',(41.795103251114,31.9972371529861,-171.649916441382));
#176941=CARTESIAN_POINT('Ctrl Pts',(41.8306429216694,32.1778713834354,-171.649969369358));
#176942=CARTESIAN_POINT('Ctrl Pts',(41.8578946341289,32.2830711178797,-171.64993233013));
#176943=CARTESIAN_POINT('Ctrl Pts',(41.922325972237,32.4823719887145,-171.649935735269));
#176944=CARTESIAN_POINT('Ctrl Pts',(41.9586161144823,32.5765803216321,-171.64995));
#176945=CARTESIAN_POINT('Ctrl Pts',(42.,32.6685811839606,-171.64995));
#176946=CARTESIAN_POINT('Ctrl Pts',(41.5,30.4123236926243,-171.14995));
#176947=CARTESIAN_POINT('Ctrl Pts',(41.5,30.6002475127106,-171.149950044596));
#176948=CARTESIAN_POINT('Ctrl Pts',(41.4999999999992,30.7880947817855,-171.167358426711));
#176949=CARTESIAN_POINT('Ctrl Pts',(41.5000000000009,30.9759786884911,-171.183208448531));
#176950=CARTESIAN_POINT('Ctrl Pts',(41.5000000000009,30.976120931185,-171.183220448228));
#176951=CARTESIAN_POINT('Ctrl Pts',(41.5000000000009,30.9762631739402,-171.183232446501));
#176952=CARTESIAN_POINT('Ctrl Pts',(41.5000000000009,30.9764054167567,-171.183244443348));
#176953=CARTESIAN_POINT('Ctrl Pts',(41.5000000000023,31.1369344018913,-171.196783556862));
#176954=CARTESIAN_POINT('Ctrl Pts',(41.4999999999993,31.2974626498578,-171.208492413819));
#176955=CARTESIAN_POINT('Ctrl Pts',(41.500000000002,31.4579880081833,-171.211623701832));
#176956=CARTESIAN_POINT('Ctrl Pts',(41.5000000000025,31.4852425168678,-171.212155341924));
#176957=CARTESIAN_POINT('Ctrl Pts',(41.5000000000032,31.512496944256,-171.212439843791));
#176958=CARTESIAN_POINT('Ctrl Pts',(41.5000000000045,31.5397512823877,-171.212444366369));
#176959=CARTESIAN_POINT('Ctrl Pts',(41.5000000000045,31.5399934772056,-171.212444406558));
#176960=CARTESIAN_POINT('Ctrl Pts',(41.5000000000045,31.5402356720169,-171.212444424596));
#176961=CARTESIAN_POINT('Ctrl Pts',(41.5000000000045,31.5404778668211,-171.212444420506));
#176962=CARTESIAN_POINT('Ctrl Pts',(41.5000000000123,31.7017281895742,-171.21244169735));
#176963=CARTESIAN_POINT('Ctrl Pts',(41.5000000000007,31.8629751164084,-171.202628065384));
#176964=CARTESIAN_POINT('Ctrl Pts',(41.5000000000001,32.0242208996319,-171.189830777502));
#176965=CARTESIAN_POINT('Ctrl Pts',(41.5,32.0508620130049,-171.187716402846));
#176966=CARTESIAN_POINT('Ctrl Pts',(41.5,32.0775031023704,-171.185520466759));
#176967=CARTESIAN_POINT('Ctrl Pts',(41.5,32.1041441836616,-171.183273657174));
#176968=CARTESIAN_POINT('Ctrl Pts',(41.5,32.1042728698425,-171.18326280426));
#176969=CARTESIAN_POINT('Ctrl Pts',(41.5,32.1044015560177,-171.183251950612));
#176970=CARTESIAN_POINT('Ctrl Pts',(41.5,32.1045302421874,-171.183241096235));
#176971=CARTESIAN_POINT('Ctrl Pts',(41.5000000000001,32.2434923963672,-171.171519963657));
#176972=CARTESIAN_POINT('Ctrl Pts',(41.5,32.3824542184406,-171.15894297239));
#176973=CARTESIAN_POINT('Ctrl Pts',(41.5,32.5214184450399,-171.153174108105));
#176974=CARTESIAN_POINT('Ctrl Pts',(41.5,32.5704723625655,-171.151137717878));
#176975=CARTESIAN_POINT('Ctrl Pts',(41.5,32.6195265765098,-171.149950012104));
#176976=CARTESIAN_POINT('Ctrl Pts',(41.5,32.6685811839606,-171.14995));
#176977=CARTESIAN_POINT('Origin',(42.,58.91999998,-171.14995));
#176978=CARTESIAN_POINT('',(41.5,36.3973044859519,-171.14995));
#176979=CARTESIAN_POINT('Origin',(42.,28.91999998,-92.34995));
#176980=CARTESIAN_POINT('',(42.,28.41999998,-95.34995));
#176981=CARTESIAN_POINT('',(42.,28.41999998,-95.34995));
#176982=CARTESIAN_POINT('',(41.5,28.91999998,-95.34995));
#176983=CARTESIAN_POINT('',(41.5,28.91999998,-171.64995));
#176984=CARTESIAN_POINT('Origin',(42.,28.91999998,-95.34995));
#176985=CARTESIAN_POINT('Ctrl Pts',(37.,28.41999998,-91.34995));
#176986=CARTESIAN_POINT('Ctrl Pts',(37.,28.41999998,-92.34995));
#176987=CARTESIAN_POINT('Ctrl Pts',(37.,29.41999998,-92.34995));
#176988=CARTESIAN_POINT('Ctrl Pts',(37.5,28.41999998,-91.34995));
#176989=CARTESIAN_POINT('Ctrl Pts',(37.5,28.41999998,-92.34995));
#176990=CARTESIAN_POINT('Ctrl Pts',(37.5,29.41999998,-92.34995));
#176991=CARTESIAN_POINT('Ctrl Pts',(37.5,28.91999998,-91.34995));
#176992=CARTESIAN_POINT('Ctrl Pts',(37.5,28.91999998,-91.84995));
#176993=CARTESIAN_POINT('Ctrl Pts',(37.5,29.41999998,-91.84995));
#176994=CARTESIAN_POINT('',(37.5,29.41999998,-91.84995));
#176995=CARTESIAN_POINT('Origin',(37.5,29.41999998,-91.34995));
#176996=CARTESIAN_POINT('',(37.,29.41999998,-92.34995));
#176997=CARTESIAN_POINT('Origin',(37.,29.41999998,-91.84995));
#176998=CARTESIAN_POINT('Origin',(37.,29.41999998,-91.34995));
#176999=CARTESIAN_POINT('Origin',(60.,28.41999998,-55.24995));
#177000=CARTESIAN_POINT('',(30.5,28.41999998,-91.34995));
#177001=CARTESIAN_POINT('Ctrl Pts',(31.,29.41999998,-92.34995));
#177002=CARTESIAN_POINT('Ctrl Pts',(31.,28.41999998,-92.34995));
#177003=CARTESIAN_POINT('Ctrl Pts',(31.,28.41999998,-91.34995));
#177004=CARTESIAN_POINT('Ctrl Pts',(30.5,29.41999998,-92.34995));
#177005=CARTESIAN_POINT('Ctrl Pts',(30.5,28.41999998,-92.34995));
#177006=CARTESIAN_POINT('Ctrl Pts',(30.5,28.41999998,-91.34995));
#177007=CARTESIAN_POINT('Ctrl Pts',(30.5,29.41999998,-91.84995));
#177008=CARTESIAN_POINT('Ctrl Pts',(30.5,28.91999998,-91.84995));
#177009=CARTESIAN_POINT('Ctrl Pts',(30.5,28.91999998,-91.34995));
#177010=CARTESIAN_POINT('',(31.,29.41999998,-92.34995));
#177011=CARTESIAN_POINT('Origin',(31.,29.41999998,-91.34995));
#177012=CARTESIAN_POINT('',(30.5,29.41999998,-91.84995));
#177013=CARTESIAN_POINT('Origin',(31.,29.41999998,-91.84995));
#177014=CARTESIAN_POINT('Origin',(30.5,29.41999998,-91.34995));
#177015=CARTESIAN_POINT('Origin',(30.,46.41999998,-92.34995));
#177016=CARTESIAN_POINT('',(30.5,46.41999998,-91.84995));
#177017=CARTESIAN_POINT('',(30.5,46.41999998,-58.24995));
#177018=CARTESIAN_POINT('',(30.,46.91999998,-91.84995));
#177019=CARTESIAN_POINT('Origin',(30.,46.41999998,-91.84995));
#177020=CARTESIAN_POINT('',(30.,46.91999998,-92.34995));
#177021=CARTESIAN_POINT('Origin',(-39.,46.91999998,-129.34995));
#177022=CARTESIAN_POINT('',(29.5,46.91999998,-91.84995));
#177023=CARTESIAN_POINT('',(-39.,46.91999998,-91.84995));
#177024=CARTESIAN_POINT('',(29.5,46.91999998,-58.24995));
#177025=CARTESIAN_POINT('Origin',(29.5,46.41999998,-92.34995));
#177026=CARTESIAN_POINT('',(29.,46.41999998,-91.84995));
#177027=CARTESIAN_POINT('Origin',(29.5,46.41999998,-91.84995));
#177028=CARTESIAN_POINT('',(29.,46.41999998,-92.34995));
#177029=CARTESIAN_POINT('Ctrl Pts',(28.5,28.41999998,-91.34995));
#177030=CARTESIAN_POINT('Ctrl Pts',(28.5,28.41999998,-92.34995));
#177031=CARTESIAN_POINT('Ctrl Pts',(28.5,29.41999998,-92.34995));
#177032=CARTESIAN_POINT('Ctrl Pts',(29.,28.41999998,-91.34995));
#177033=CARTESIAN_POINT('Ctrl Pts',(29.,28.41999998,-92.34995));
#177034=CARTESIAN_POINT('Ctrl Pts',(29.,29.41999998,-92.34995));
#177035=CARTESIAN_POINT('Ctrl Pts',(29.,28.91999998,-91.34995));
#177036=CARTESIAN_POINT('Ctrl Pts',(29.,28.91999998,-91.84995));
#177037=CARTESIAN_POINT('Ctrl Pts',(29.,29.41999998,-91.84995));
#177038=CARTESIAN_POINT('',(29.,29.41999998,-91.84995));
#177039=CARTESIAN_POINT('Origin',(29.,29.41999998,-91.34995));
#177040=CARTESIAN_POINT('',(28.5,29.41999998,-92.34995));
#177041=CARTESIAN_POINT('Origin',(28.5,29.41999998,-91.84995));
#177042=CARTESIAN_POINT('Origin',(28.5,29.41999998,-91.34995));
#177043=CARTESIAN_POINT('Origin',(60.,28.41999998,-55.24995));
#177044=CARTESIAN_POINT('',(22.,28.4199999800001,-91.34995));
#177045=CARTESIAN_POINT('Ctrl Pts',(22.5,29.41999998,-92.34995));
#177046=CARTESIAN_POINT('Ctrl Pts',(22.5,28.41999998,-92.34995));
#177047=CARTESIAN_POINT('Ctrl Pts',(22.5,28.41999998,-91.34995));
#177048=CARTESIAN_POINT('Ctrl Pts',(22.,29.41999998,-92.34995));
#177049=CARTESIAN_POINT('Ctrl Pts',(22.,28.41999998,-92.34995));
#177050=CARTESIAN_POINT('Ctrl Pts',(22.,28.41999998,-91.34995));
#177051=CARTESIAN_POINT('Ctrl Pts',(22.,29.41999998,-91.84995));
#177052=CARTESIAN_POINT('Ctrl Pts',(22.,28.91999998,-91.84995));
#177053=CARTESIAN_POINT('Ctrl Pts',(22.,28.91999998,-91.34995));
#177054=CARTESIAN_POINT('',(22.5,29.41999998,-92.34995));
#177055=CARTESIAN_POINT('Origin',(22.5,29.41999998,-91.34995));
#177056=CARTESIAN_POINT('',(22.,29.41999998,-91.84995));
#177057=CARTESIAN_POINT('Origin',(22.5,29.41999998,-91.84995));
#177058=CARTESIAN_POINT('Origin',(22.,29.41999998,-91.34995));
#177059=CARTESIAN_POINT('Origin',(21.5,46.41999998,-92.34995));
#177060=CARTESIAN_POINT('',(22.,46.41999998,-91.84995));
#177061=CARTESIAN_POINT('',(22.,46.41999998,-58.24995));
#177062=CARTESIAN_POINT('',(21.5,46.91999998,-91.84995));
#177063=CARTESIAN_POINT('Origin',(21.5,46.41999998,-91.84995));
#177064=CARTESIAN_POINT('',(21.5,46.91999998,-92.34995));
#177065=CARTESIAN_POINT('Origin',(-39.,46.91999998,-129.34995));
#177066=CARTESIAN_POINT('',(21.,46.91999998,-91.84995));
#177067=CARTESIAN_POINT('',(-39.,46.91999998,-91.84995));
#177068=CARTESIAN_POINT('',(21.,46.91999998,-58.24995));
#177069=CARTESIAN_POINT('Origin',(21.,46.41999998,-92.34995));
#177070=CARTESIAN_POINT('',(20.5,46.41999998,-91.84995));
#177071=CARTESIAN_POINT('Origin',(21.,46.41999998,-91.84995));
#177072=CARTESIAN_POINT('',(20.5,46.41999998,-92.34995));
#177073=CARTESIAN_POINT('Ctrl Pts',(20.,28.41999998,-91.34995));
#177074=CARTESIAN_POINT('Ctrl Pts',(20.,28.41999998,-92.34995));
#177075=CARTESIAN_POINT('Ctrl Pts',(20.,29.41999998,-92.34995));
#177076=CARTESIAN_POINT('Ctrl Pts',(20.5,28.41999998,-91.34995));
#177077=CARTESIAN_POINT('Ctrl Pts',(20.5,28.41999998,-92.34995));
#177078=CARTESIAN_POINT('Ctrl Pts',(20.5,29.41999998,-92.34995));
#177079=CARTESIAN_POINT('Ctrl Pts',(20.5,28.91999998,-91.34995));
#177080=CARTESIAN_POINT('Ctrl Pts',(20.5,28.91999998,-91.84995));
#177081=CARTESIAN_POINT('Ctrl Pts',(20.5,29.41999998,-91.84995));
#177082=CARTESIAN_POINT('',(20.5,29.41999998,-91.84995));
#177083=CARTESIAN_POINT('Origin',(20.5,29.41999998,-91.34995));
#177084=CARTESIAN_POINT('',(20.,29.41999998,-92.34995));
#177085=CARTESIAN_POINT('Origin',(20.,29.41999998,-91.84995));
#177086=CARTESIAN_POINT('Origin',(20.,29.41999998,-91.34995));
#177087=CARTESIAN_POINT('Origin',(60.,28.41999998,-55.24995));
#177088=CARTESIAN_POINT('',(17.5283474636331,28.4199999800081,-91.3499485560103));
#177089=CARTESIAN_POINT('Origin',(20.088871062793,28.4200000295341,-83.1773333825974));
#177090=CARTESIAN_POINT('',(16.1621051845127,28.4199999800001,-91.34995));
#177091=CARTESIAN_POINT('Ctrl Pts',(19.8416434885933,29.3176415862829,-85.6947270505041));
#177092=CARTESIAN_POINT('Ctrl Pts',(20.7092106783515,28.41999998,-86.6470800003654));
#177093=CARTESIAN_POINT('Ctrl Pts',(21.7666112105514,28.41999998,-87.8078183592076));
#177094=CARTESIAN_POINT('Ctrl Pts',(18.8896716409139,29.2827357288726,-86.6297133466452));
#177095=CARTESIAN_POINT('Ctrl Pts',(19.7296405475881,28.4199999799976,-87.5847244149314));
#177096=CARTESIAN_POINT('Ctrl Pts',(20.7402388551495,28.41999998,-88.7428151801658));
#177097=CARTESIAN_POINT('Ctrl Pts',(17.9119477871191,29.2478866829953,-87.5391531932496));
#177098=CARTESIAN_POINT('Ctrl Pts',(18.7197222668567,28.4199999800025,-88.4987039616193));
#177099=CARTESIAN_POINT('Ctrl Pts',(19.6830654074503,28.4199999800001,-89.6522445020127));
#177100=CARTESIAN_POINT('Ctrl Pts',(15.8876250911483,29.1791411788287,-89.290529750932));
#177101=CARTESIAN_POINT('Ctrl Pts',(16.6238286994528,28.4199999799976,-90.2586559409325));
#177102=CARTESIAN_POINT('Ctrl Pts',(17.4871574021565,28.4199999800001,-91.4036210595759));
#177103=CARTESIAN_POINT('Ctrl Pts',(14.8453850851454,29.1454134093176,-90.1279271408305));
#177104=CARTESIAN_POINT('Ctrl Pts',(15.5423832476573,28.4199999800097,-91.1005048403699));
#177105=CARTESIAN_POINT('Ctrl Pts',(16.353131902533,28.4199999800001,-92.2410073071712));
#177106=CARTESIAN_POINT('Ctrl Pts',(13.781556827362,29.1135284095041,-90.9029551205337));
#177107=CARTESIAN_POINT('Ctrl Pts',(14.4341913591531,28.41999998,-91.8807658383619));
#177108=CARTESIAN_POINT('Ctrl Pts',(15.1919283151595,28.4199999800001,-93.0160464292372));
#177109=CARTESIAN_POINT('Ctrl Pts',(17.5283474636331,28.4199999800081,-91.3499485560103));
#177110=CARTESIAN_POINT('Ctrl Pts',(17.4449670690501,28.4200000828332,-91.3407525162259));
#177111=CARTESIAN_POINT('Ctrl Pts',(17.3556350906279,28.4209780981964,-91.3309072709742));
#177112=CARTESIAN_POINT('Ctrl Pts',(17.2604628566404,28.4233820658963,-91.3204025719688));
#177113=CARTESIAN_POINT('Ctrl Pts',(17.209353748992,28.4246730374203,-91.3147613700153));
#177114=CARTESIAN_POINT('Ctrl Pts',(17.1565605798997,28.4263761331184,-91.3089299869687));
#177115=CARTESIAN_POINT('Ctrl Pts',(17.1021019331091,28.4285667561178,-91.3029068081637));
#177116=CARTESIAN_POINT('Ctrl Pts',(17.0241651859755,28.4317017960211,-91.29428692884));
#177117=CARTESIAN_POINT('Ctrl Pts',(16.9428200887949,28.435834974118,-91.2852725602857));
#177118=CARTESIAN_POINT('Ctrl Pts',(16.8581470738689,28.4411979043932,-91.2758758511481));
#177119=CARTESIAN_POINT('Ctrl Pts',(16.8158105664059,28.4438793695307,-91.2711774965793));
#177120=CARTESIAN_POINT('Ctrl Pts',(16.7726423863633,28.4468684484924,-91.2663838155556));
#177121=CARTESIAN_POINT('Ctrl Pts',(16.72865452465,28.4501948590961,-91.2614980219493));
#177122=CARTESIAN_POINT('Ctrl Pts',(16.7066605937934,28.451858064398,-91.2590551251462));
#177123=CARTESIAN_POINT('Ctrl Pts',(16.6844617436482,28.4536056114285,-91.256589201598));
#177124=CARTESIAN_POINT('Ctrl Pts',(16.662059622183,28.4554412241898,-91.2541008944022));
#177125=CARTESIAN_POINT('Ctrl Pts',(16.6508585614504,28.4563590305704,-91.2528567408044));
#177126=CARTESIAN_POINT('Ctrl Pts',(16.63960667785,28.4572987847638,-91.2516076963612));
#177127=CARTESIAN_POINT('Ctrl Pts',(16.6283041889963,28.4582610451365,-91.2503528794858));
#177128=CARTESIAN_POINT('Ctrl Pts',(16.6170017001427,28.4592233055093,-91.2490980626103));
#177129=CARTESIAN_POINT('Ctrl Pts',(16.6040146503638,28.4603524696449,-91.247656024132));
#177130=CARTESIAN_POINT('Ctrl Pts',(16.5942451218782,28.4612158251874,-91.2465711301194));
#177131=CARTESIAN_POINT('Ctrl Pts',(16.4255035637327,28.4761279020287,-91.2278325895262));
#177132=CARTESIAN_POINT('Ctrl Pts',(16.2577107764323,28.495018036401,-91.2091649348818));
#177133=CARTESIAN_POINT('Ctrl Pts',(16.0911292123908,28.517718159937,-91.190598973341));
#177134=CARTESIAN_POINT('Ctrl Pts',(15.9587321256393,28.5357599537114,-91.1758429633655));
#177135=CARTESIAN_POINT('Ctrl Pts',(15.8270995738065,28.5562073684433,-91.1611511371293));
#177136=CARTESIAN_POINT('Ctrl Pts',(15.6963501489323,28.5789561723598,-91.1465376691438));
#177137=CARTESIAN_POINT('Ctrl Pts',(15.6873039166932,28.5805301063453,-91.1455265991116));
#177138=CARTESIAN_POINT('Ctrl Pts',(15.6799762942362,28.5818126045997,-91.1447075451513));
#177139=CARTESIAN_POINT('Ctrl Pts',(15.669481806099,28.5836615901236,-91.1435525932031));
#177140=CARTESIAN_POINT('Ctrl Pts',(15.6689270297337,28.5837593341446,-91.1434915382916));
#177141=CARTESIAN_POINT('Ctrl Pts',(15.6683634058881,28.5838586733159,-91.1434295448885));
#177142=CARTESIAN_POINT('Ctrl Pts',(15.6677902137525,28.583959738813,-91.1433665350773));
#177143=CARTESIAN_POINT('Ctrl Pts',(15.6460612240955,28.5877910041168,-91.1409779127442));
#177144=CARTESIAN_POINT('Ctrl Pts',(15.6244513449189,28.5916691515427,-91.1385998012044));
#177145=CARTESIAN_POINT('Ctrl Pts',(15.602960062943,28.5955921284231,-91.1362322410147));
#177146=CARTESIAN_POINT('Ctrl Pts',(15.3794960512604,28.6363828151961,-91.1116146077591));
#177147=CARTESIAN_POINT('Ctrl Pts',(15.1688312125338,28.6819952998695,-91.0881339378895));
#177148=CARTESIAN_POINT('Ctrl Pts',(14.9704909007038,28.7307074200043,-91.0658565029333));
#177149=CARTESIAN_POINT('Ctrl Pts',(14.8672115437093,28.7560726944608,-91.0542562430741));
#177150=CARTESIAN_POINT('Ctrl Pts',(14.7672740628269,28.7822789906839,-91.0429824470375));
#177151=CARTESIAN_POINT('Ctrl Pts',(14.6706121874534,28.8090890708133,-91.0320453163648));
#177152=CARTESIAN_POINT('Ctrl Pts',(14.5146056345302,28.85235895533,-91.0143934339808));
#177153=CARTESIAN_POINT('Ctrl Pts',(14.367125110666,28.8972010263637,-90.9976177986137));
#177154=CARTESIAN_POINT('Ctrl Pts',(14.2279053139402,28.9426415327345,-90.9817809628304));
#177155=CARTESIAN_POINT('Ctrl Pts',(14.0992751073288,28.9846256604266,-90.9671487373368));
#177156=CARTESIAN_POINT('Ctrl Pts',(13.9776966559743,29.027120305016,-90.9533180092168));
#177157=CARTESIAN_POINT('Ctrl Pts',(13.8629628324617,29.0693971421497,-90.9403366624458));
#177158=CARTESIAN_POINT('Ctrl Pts',(19.8077681778583,29.3163999071086,-85.7279764688716));
#177159=CARTESIAN_POINT('Ctrl Pts',(19.4082493848523,29.3017607914722,-86.1198602027121));
#177160=CARTESIAN_POINT('Ctrl Pts',(19.0112633927749,29.2873923085991,-86.5002814539897));
#177161=CARTESIAN_POINT('Ctrl Pts',(18.6159839225994,29.273296094587,-86.8698151354957));
#177162=CARTESIAN_POINT('Ctrl Pts',(18.0851775960533,29.2543668049513,-87.3660483851714));
#177163=CARTESIAN_POINT('Ctrl Pts',(17.5574499676151,29.2359287990193,-87.842649941049));
#177164=CARTESIAN_POINT('Ctrl Pts',(17.0308778298195,29.2179724993612,-88.3010753210071));
#177165=CARTESIAN_POINT('Ctrl Pts',(16.9871738817249,29.2164821789817,-88.3391232874164));
#177166=CARTESIAN_POINT('Ctrl Pts',(16.9434779139457,29.2149951697386,-88.37704606025));
#177167=CARTESIAN_POINT('Ctrl Pts',(16.8997888344922,29.2135114625125,-88.4148444754352));
#177168=CARTESIAN_POINT('Ctrl Pts',(16.6124645154597,29.2037537570695,-88.6634284245469));
#177169=CARTESIAN_POINT('Ctrl Pts',(16.3257931544452,29.1941526893015,-88.9062649282737));
#177170=CARTESIAN_POINT('Ctrl Pts',(16.0398114822454,29.1847211178926,-89.1432707978858));
#177171=CARTESIAN_POINT('Ctrl Pts',(15.7410191195434,29.174867054576,-89.3908934626912));
#177172=CARTESIAN_POINT('Ctrl Pts',(15.4429795241797,29.1651979819656,-89.6321521383054));
#177173=CARTESIAN_POINT('Ctrl Pts',(15.1456858692503,29.1557258311974,-89.8669852373506));
#177174=CARTESIAN_POINT('Ctrl Pts',(14.8277972288318,29.1455974982188,-90.118086373695));
#177175=CARTESIAN_POINT('Ctrl Pts',(14.510761504061,29.1356942810336,-90.3618417424226));
#177176=CARTESIAN_POINT('Ctrl Pts',(14.1945159768074,29.1260282160452,-90.5982005175673));
#177177=CARTESIAN_POINT('Ctrl Pts',(14.082333602721,29.1225993545277,-90.682044512966));
#177178=CARTESIAN_POINT('Ctrl Pts',(13.9702501885868,29.119200315509,-90.7649579036228));
#177179=CARTESIAN_POINT('Ctrl Pts',(13.8582614415001,29.1158315802267,-90.8469387387806));
#177180=CARTESIAN_POINT('Ctrl Pts',(13.9704776589254,29.793296457161,-92.3317099697086));
#177181=CARTESIAN_POINT('Ctrl Pts',(13.5,29.798334383687,-92.3043420473087));
#177182=CARTESIAN_POINT('Ctrl Pts',(13.5,29.8836583509376,-91.8408299848543));
#177183=CARTESIAN_POINT('Ctrl Pts',(13.9485824763266,29.6507732526529,-92.3041572803908));
#177184=CARTESIAN_POINT('Ctrl Pts',(13.5,29.6658016093476,-92.2593052595342));
#177185=CARTESIAN_POINT('Ctrl Pts',(13.5,29.8088158028921,-91.8270528245268));
#177186=CARTESIAN_POINT('Ctrl Pts',(13.9277414892694,29.5120300570818,-92.2444171371624));
#177187=CARTESIAN_POINT('Ctrl Pts',(13.5,29.5406281722262,-92.1878683704653));
#177188=CARTESIAN_POINT('Ctrl Pts',(13.5,29.7360856593875,-91.7971835648529));
#177189=CARTESIAN_POINT('Ctrl Pts',(13.8924131672203,29.2732201982241,-92.0703719609639));
#177190=CARTESIAN_POINT('Ctrl Pts',(13.5,29.3333704157687,-92.0065554596633));
#177191=CARTESIAN_POINT('Ctrl Pts',(13.5,29.6110266364568,-91.7101609842055));
#177192=CARTESIAN_POINT('Ctrl Pts',(13.8776710606793,29.1715523493698,-91.9547463954628));
#177193=CARTESIAN_POINT('Ctrl Pts',(13.4999999999999,29.2476129207544,-91.895386283959));
#177194=CARTESIAN_POINT('Ctrl Pts',(13.5,29.5578590401594,-91.6523482016898));
#177195=CARTESIAN_POINT('Ctrl Pts',(13.8571693529918,29.0291974882966,-91.6899374203782));
#177196=CARTESIAN_POINT('Ctrl Pts',(13.5000000000001,29.1302566914018,-91.6522607622863));
#177197=CARTESIAN_POINT('Ctrl Pts',(13.5,29.4834479217461,-91.5199437062307));
#177198=CARTESIAN_POINT('Ctrl Pts',(13.851254772454,28.9875557647693,-91.5391474846049));
#177199=CARTESIAN_POINT('Ctrl Pts',(13.5000000000001,29.0962692564556,-91.5174684103174));
#177200=CARTESIAN_POINT('Ctrl Pts',(13.5,29.4617011701904,-91.4445487431295));
#177201=CARTESIAN_POINT('Ctrl Pts',(13.8496827900737,28.9765232161018,-91.2324126084916));
#177202=CARTESIAN_POINT('Ctrl Pts',(13.4999999999999,29.0873381907095,-91.2460073456115));
#177203=CARTESIAN_POINT('Ctrl Pts',(13.5,29.4559384360516,-91.2911813034188));
#177204=CARTESIAN_POINT('Ctrl Pts',(13.8539744318671,29.0067940350096,-91.0793665022882));
#177205=CARTESIAN_POINT('Ctrl Pts',(13.4999999999996,29.1119956223332,-91.1098405101534));
#177206=CARTESIAN_POINT('Ctrl Pts',(13.5,29.4717444256829,-91.2146593048585));
#177207=CARTESIAN_POINT('Ctrl Pts',(13.8629670146647,29.0694104105324,-90.9403371832566));
#177208=CARTESIAN_POINT('Ctrl Pts',(13.5,29.162996502681,-90.984393353347));
#177209=CARTESIAN_POINT('Ctrl Pts',(13.5,29.5044693674792,-91.1451435916293));
#177210=CARTESIAN_POINT('',(13.9704776589253,29.7932964571609,-92.3317099697081));
#177211=CARTESIAN_POINT('Ctrl Pts',(13.9704776589253,29.7932964571608,-92.3317099697086));
#177212=CARTESIAN_POINT('Ctrl Pts',(13.9660719436602,29.7646181560608,-92.3261658597216));
#177213=CARTESIAN_POINT('Ctrl Pts',(13.9618386370306,29.7371021221773,-92.3195123058631));
#177214=CARTESIAN_POINT('Ctrl Pts',(13.9578073956371,29.7108795338756,-92.3120680988498));
#177215=CARTESIAN_POINT('Ctrl Pts',(13.9545099890295,29.6894304249052,-92.3059790123879));
#177216=CARTESIAN_POINT('Ctrl Pts',(13.951347604472,29.6688456216843,-92.2993607697152));
#177217=CARTESIAN_POINT('Ctrl Pts',(13.9483326909375,29.6491723257345,-92.2923807044248));
#177218=CARTESIAN_POINT('Ctrl Pts',(13.9449822942959,29.6273098928904,-92.2846239356023));
#177219=CARTESIAN_POINT('Ctrl Pts',(13.9418154271827,29.6065821601135,-92.2764227184054));
#177220=CARTESIAN_POINT('Ctrl Pts',(13.9388506916509,29.5870682923812,-92.2680191239684));
#177221=CARTESIAN_POINT('Ctrl Pts',(13.937368323885,29.577311358515,-92.2638173267498));
#177222=CARTESIAN_POINT('Ctrl Pts',(13.9359364614834,29.5678578067295,-92.2595650702609));
#177223=CARTESIAN_POINT('Ctrl Pts',(13.9345572256012,29.5587169031431,-92.2552934382594));
#177224=CARTESIAN_POINT('Ctrl Pts',(13.9331779897191,29.5495759995568,-92.251021806258));
#177225=CARTESIAN_POINT('Ctrl Pts',(13.9318513808664,29.5407477463153,-92.2467308038121));
#177226=CARTESIAN_POINT('Ctrl Pts',(13.9305793585068,29.5322409034925,-92.2424520252128));
#177227=CARTESIAN_POINT('Ctrl Pts',(13.9274618297608,29.5113919562722,-92.2319654050833));
#177228=CARTESIAN_POINT('Ctrl Pts',(13.9246529340422,29.4924097351835,-92.2215211793986));
#177229=CARTESIAN_POINT('Ctrl Pts',(13.9221331430184,29.4752674918061,-92.2114767008387));
#177230=CARTESIAN_POINT('Ctrl Pts',(13.9205404067363,29.4644320404825,-92.2051276801119));
#177231=CARTESIAN_POINT('Ctrl Pts',(13.9190630962149,29.4543309529263,-92.1989375124784));
#177232=CARTESIAN_POINT('Ctrl Pts',(13.9176958195654,29.4449523900882,-92.1929871167551));
#177233=CARTESIAN_POINT('Ctrl Pts',(13.9159306301178,29.4328444233788,-92.1853050022808));
#177234=CARTESIAN_POINT('Ctrl Pts',(13.9143475548871,29.4219382408964,-92.1780218851911));
#177235=CARTESIAN_POINT('Ctrl Pts',(13.9129299430038,29.4121931549255,-92.1712831761532));
#177236=CARTESIAN_POINT('Ctrl Pts',(13.9122211370622,29.40732061194,-92.1679138216343));
#177237=CARTESIAN_POINT('Ctrl Pts',(13.9115536689625,29.4027382131008,-92.1646801183343));
#177238=CARTESIAN_POINT('Ctrl Pts',(13.9109253948871,29.3984404244484,-92.1615974984745));
#177239=CARTESIAN_POINT('Ctrl Pts',(13.9106330619778,29.3964406840335,-92.1601631702616));
#177240=CARTESIAN_POINT('Ctrl Pts',(13.9103492096096,29.3945025216351,-92.1587614975373));
#177241=CARTESIAN_POINT('Ctrl Pts',(13.9100736461926,29.3926255121625,-92.1573939964895));
#177242=CARTESIAN_POINT('Ctrl Pts',(13.9100530928442,29.3924855123394,-92.157291999186));
#177243=CARTESIAN_POINT('Ctrl Pts',(13.9100325852604,29.3923458505292,-92.1571901901387));
#177244=CARTESIAN_POINT('Ctrl Pts',(13.9100121233666,29.3922065265855,-92.1570885699965));
#177245=CARTESIAN_POINT('Ctrl Pts',(13.9098647237869,29.3912028907114,-92.1563565377456));
#177246=CARTESIAN_POINT('Ctrl Pts',(13.9097197094941,29.3902168737225,-92.1556343722458));
#177247=CARTESIAN_POINT('Ctrl Pts',(13.9095770470687,29.3892483865609,-92.1549222874115));
#177248=CARTESIAN_POINT('Ctrl Pts',(13.909505715856,29.3887641429801,-92.1545662449943));
#177249=CARTESIAN_POINT('Ctrl Pts',(13.9094751716244,29.3885555991234,-92.1544125945762));
#177250=CARTESIAN_POINT('Ctrl Pts',(13.9094250101062,29.3882155492447,-92.1541618662424));
#177251=CARTESIAN_POINT('Ctrl Pts',(13.9093748485881,29.3878754993659,-92.1539111379085));
#177252=CARTESIAN_POINT('Ctrl Pts',(13.9093050857272,29.3874037424048,-92.1535636138701));
#177253=CARTESIAN_POINT('Ctrl Pts',(13.9091560094093,29.3863954359885,-92.152816470617));
#177254=CARTESIAN_POINT('Ctrl Pts',(13.9048390217758,29.3571966578547,-92.1311805177665));
#177255=CARTESIAN_POINT('Ctrl Pts',(13.9007550483884,29.329522680952,-92.1081500266596));
#177256=CARTESIAN_POINT('Ctrl Pts',(13.8969256320677,29.303496130266,-92.0840897594474));
#177257=CARTESIAN_POINT('Ctrl Pts',(13.8931589395588,29.2778958807006,-92.0604235866737));
#177258=CARTESIAN_POINT('Ctrl Pts',(13.8896385152793,29.2538895184042,-92.0357614245562));
#177259=CARTESIAN_POINT('Ctrl Pts',(13.8863779446049,29.2315457150798,-92.0104355370998));
#177260=CARTESIAN_POINT('Ctrl Pts',(13.8856272645384,29.2264015089148,-92.0046047667294));
#177261=CARTESIAN_POINT('Ctrl Pts',(13.8848903295692,29.221345225095,-91.9987387408664));
#177262=CARTESIAN_POINT('Ctrl Pts',(13.8841672543394,29.2163773369429,-91.9928413741767));
#177263=CARTESIAN_POINT('Ctrl Pts',(13.8809865167897,29.1945240805472,-91.9668994321714));
#177264=CARTESIAN_POINT('Ctrl Pts',(13.8780714941699,29.1743821555997,-91.9403489716015));
#177265=CARTESIAN_POINT('Ctrl Pts',(13.8754145679604,29.1559578661073,-91.9134942881761));
#177266=CARTESIAN_POINT('Ctrl Pts',(13.8751241956756,29.1539442975643,-91.9105593719722));
#177267=CARTESIAN_POINT('Ctrl Pts',(13.874836900671,29.1519512003806,-91.9076207966203));
#177268=CARTESIAN_POINT('Ctrl Pts',(13.8745526690139,29.1499785504107,-91.9046789404017));
#177269=CARTESIAN_POINT('Ctrl Pts',(13.8731101836618,29.1399672845464,-91.8897489197756));
#177270=CARTESIAN_POINT('Ctrl Pts',(13.8717464644608,29.1304829683556,-91.8747345104047));
#177271=CARTESIAN_POINT('Ctrl Pts',(13.8704584257147,29.1215200363874,-91.8596831904024));
#177272=CARTESIAN_POINT('Ctrl Pts',(13.8698849070136,29.1175291555882,-91.8529813628963));
#177273=CARTESIAN_POINT('Ctrl Pts',(13.869356255753,29.1138487597176,-91.8466285500808));
#177274=CARTESIAN_POINT('Ctrl Pts',(13.868831041355,29.1101938494189,-91.840157299871));
#177275=CARTESIAN_POINT('Ctrl Pts',(13.8683658756017,29.1069568111566,-91.8344259185726));
#177276=CARTESIAN_POINT('Ctrl Pts',(13.8679034723206,29.103740197726,-91.8286012287684));
#177277=CARTESIAN_POINT('Ctrl Pts',(13.8674193485158,29.1003751246054,-91.8223417922768));
#177278=CARTESIAN_POINT('Ctrl Pts',(13.8672224644036,29.099006612198,-91.8197961963281));
#177279=CARTESIAN_POINT('Ctrl Pts',(13.867021980309,29.0976135305897,-91.8171779274437));
#177280=CARTESIAN_POINT('Ctrl Pts',(13.8668164546783,29.0961859184677,-91.8144631545686));
#177281=CARTESIAN_POINT('Ctrl Pts',(13.8642275697956,29.0782031324296,-91.7802667653671));
#177282=CARTESIAN_POINT('Ctrl Pts',(13.8619343749943,29.0622384906243,-91.7449845405102));
#177283=CARTESIAN_POINT('Ctrl Pts',(13.8599486096495,29.0483917564659,-91.709006233217));
#177284=CARTESIAN_POINT('Ctrl Pts',(13.8579976218432,29.0347875259502,-91.673658029057));
#177285=CARTESIAN_POINT('Ctrl Pts',(13.8563434001964,29.0232278025212,-91.6376388186669));
#177286=CARTESIAN_POINT('Ctrl Pts',(13.8549901949726,29.0137586069535,-91.6013194042953));
#177287=CARTESIAN_POINT('Ctrl Pts',(13.853656462459,29.0044256737189,-91.5655226286316));
#177288=CARTESIAN_POINT('Ctrl Pts',(13.8526151487513,28.9971236073399,-91.5294349801731));
#177289=CARTESIAN_POINT('Ctrl Pts',(13.8518634700335,28.9918473079284,-91.4934004105108));
#177290=CARTESIAN_POINT('Ctrl Pts',(13.8511117913156,28.9865710085169,-91.4573658408485));
#177291=CARTESIAN_POINT('Ctrl Pts',(13.8506497573169,28.9833205884546,-91.4213850311442));
#177292=CARTESIAN_POINT('Ctrl Pts',(13.8504675584972,28.9820398733893,-91.3857800321588));
#177293=CARTESIAN_POINT('Ctrl Pts',(13.850459871782,28.9819858417989,-91.3842779066858));
#177294=CARTESIAN_POINT('Ctrl Pts',(13.8504526772006,28.9819352758935,-91.3827767240698));
#177295=CARTESIAN_POINT('Ctrl Pts',(13.8504459726624,28.981888160148,-91.3812765043687));
#177296=CARTESIAN_POINT('Ctrl Pts',(13.8503108157195,28.9809383527283,-91.3510335402089));
#177297=CARTESIAN_POINT('Ctrl Pts',(13.8503713034644,28.9813677928989,-91.3203201309666));
#177298=CARTESIAN_POINT('Ctrl Pts',(13.8506407953683,28.9832638958992,-91.2893816972864));
#177299=CARTESIAN_POINT('Ctrl Pts',(13.8509127119446,28.9851770585159,-91.258164904357));
#177300=CARTESIAN_POINT('Ctrl Pts',(13.8513974319433,28.9885835117664,-91.2267196122043));
#177301=CARTESIAN_POINT('Ctrl Pts',(13.8521014903619,28.9935216895577,-91.1953097078188));
#177302=CARTESIAN_POINT('Ctrl Pts',(13.85280750844,28.9984736121552,-91.163812377855));
#177303=CARTESIAN_POINT('Ctrl Pts',(13.8537340898665,29.0049657742317,-91.1323513226142));
#177304=CARTESIAN_POINT('Ctrl Pts',(13.8548804607771,29.0129848879013,-91.1011947079472));
#177305=CARTESIAN_POINT('Ctrl Pts',(13.8560254849809,29.020994581064,-91.0700746947195));
#177306=CARTESIAN_POINT('Ctrl Pts',(13.8573897688233,29.0305275024821,-91.0392591235628));
#177307=CARTESIAN_POINT('Ctrl Pts',(13.858965299919,29.0415198349271,-91.009006688265));
#177308=CARTESIAN_POINT('Ctrl Pts',(13.8601766023979,29.04997097853,-90.9857479598451));
#177309=CARTESIAN_POINT('Ctrl Pts',(13.8615126204926,29.0592837088275,-90.9628220098879));
#177310=CARTESIAN_POINT('Ctrl Pts',(13.8629668992758,29.0694096071188,-90.9403389671137));
#177311=CARTESIAN_POINT('',(13.5,29.8836583509375,-91.8408299848543));
#177312=CARTESIAN_POINT('Origin',(14.,29.8836583509375,-91.8408299848543));
#177313=CARTESIAN_POINT('Ctrl Pts',(13.5,29.5044693674792,-91.1451435916293));
#177314=CARTESIAN_POINT('Ctrl Pts',(13.5,29.4871798972865,-91.1818706195726));
#177315=CARTESIAN_POINT('Ctrl Pts',(13.5,29.4746493543107,-91.2204653406996));
#177316=CARTESIAN_POINT('Ctrl Pts',(13.5,29.4670724885977,-91.259957519387));
#177317=CARTESIAN_POINT('Ctrl Pts',(13.5,29.4602667842095,-91.2954302470261));
#177318=CARTESIAN_POINT('Ctrl Pts',(13.5,29.4574580326191,-91.3316285116295));
#177319=CARTESIAN_POINT('Ctrl Pts',(13.5000000000001,29.4588194335385,-91.3678650371612));
#177320=CARTESIAN_POINT('Ctrl Pts',(13.5000000000001,29.4588222728777,-91.367940612098));
#177321=CARTESIAN_POINT('Ctrl Pts',(13.5000000000001,29.4588251305407,-91.3680161857943));
#177322=CARTESIAN_POINT('Ctrl Pts',(13.5000000000001,29.4588280065244,-91.3680917582431));
#177323=CARTESIAN_POINT('Ctrl Pts',(13.5000000000004,29.4617431600592,-91.4446934778138));
#177324=CARTESIAN_POINT('Ctrl Pts',(13.4999999999999,29.483485076552,-91.5200098118263));
#177325=CARTESIAN_POINT('Ctrl Pts',(13.5000000000001,29.5206532241076,-91.5861460983069));
#177326=CARTESIAN_POINT('Ctrl Pts',(13.5000000000001,29.5206776694618,-91.5861895958997));
#177327=CARTESIAN_POINT('Ctrl Pts',(13.5000000000001,29.5207021217052,-91.5862330898687));
#177328=CARTESIAN_POINT('Ctrl Pts',(13.5000000000001,29.5207265808359,-91.5862765802124));
#177329=CARTESIAN_POINT('Ctrl Pts',(13.5000000000003,29.5579279046594,-91.6524235901087));
#177330=CARTESIAN_POINT('Ctrl Pts',(13.5,29.6110672833213,-91.710189265371));
#177331=CARTESIAN_POINT('Ctrl Pts',(13.5,29.6735560708361,-91.7536723853085));
#177332=CARTESIAN_POINT('Ctrl Pts',(13.5,29.6735766131945,-91.7536866798063));
#177333=CARTESIAN_POINT('Ctrl Pts',(13.5,29.6735971566538,-91.7537009728318));
#177334=CARTESIAN_POINT('Ctrl Pts',(13.5,29.6736177012137,-91.753715264385));
#177335=CARTESIAN_POINT('Ctrl Pts',(13.5,29.6935761704139,-91.7675991112376));
#177336=CARTESIAN_POINT('Ctrl Pts',(13.5,29.7144903240443,-91.7800410703758));
#177337=CARTESIAN_POINT('Ctrl Pts',(13.5,29.7361680987988,-91.7910278638482));
#177338=CARTESIAN_POINT('Ctrl Pts',(13.5,29.7580697930565,-91.8021281448608));
#177339=CARTESIAN_POINT('Ctrl Pts',(13.5,29.78075231092,-91.8117435399085));
#177340=CARTESIAN_POINT('Ctrl Pts',(13.5,29.8040427282678,-91.8198138783841));
#177341=CARTESIAN_POINT('Ctrl Pts',(13.5,29.8266838607853,-91.8276592338434));
#177342=CARTESIAN_POINT('Ctrl Pts',(13.5,29.8499007708166,-91.8340446948146));
#177343=CARTESIAN_POINT('Ctrl Pts',(13.5,29.8735386060567,-91.8388665069538));
#177344=CARTESIAN_POINT('Ctrl Pts',(13.5,29.8769034909812,-91.8395528998832));
#177345=CARTESIAN_POINT('Ctrl Pts',(13.5,29.8802768936902,-91.8402075213397));
#177346=CARTESIAN_POINT('Ctrl Pts',(13.5,29.8836583509375,-91.8408299848543));
#177347=CARTESIAN_POINT('Ctrl Pts',(14.,29.9836543272765,-92.34995));
#177348=CARTESIAN_POINT('Ctrl Pts',(13.5,29.9836543272765,-92.34995));
#177349=CARTESIAN_POINT('Ctrl Pts',(13.5,29.9836543272765,-91.84995));
#177350=CARTESIAN_POINT('Ctrl Pts',(13.9900288285115,29.9192223045234,-92.34995));
#177351=CARTESIAN_POINT('Ctrl Pts',(13.5,29.9198591164476,-92.340077310875));
#177352=CARTESIAN_POINT('Ctrl Pts',(13.5,29.9498130224307,-91.8499499813658));
#177353=CARTESIAN_POINT('Ctrl Pts',(13.9801870069313,29.8557668849998,-92.3437935523175));
#177354=CARTESIAN_POINT('Ctrl Pts',(13.4999999999992,29.8581345500688,-92.3247747757233));
#177355=CARTESIAN_POINT('Ctrl Pts',(13.5,29.9164799575816,-91.8468718299503));
#177356=CARTESIAN_POINT('Ctrl Pts',(13.9704776589253,29.7932964571608,-92.3317099697086));
#177357=CARTESIAN_POINT('Ctrl Pts',(13.5,29.7983343836869,-92.3043420473086));
#177358=CARTESIAN_POINT('Ctrl Pts',(13.5,29.8836583509375,-91.8408299848543));
#177359=CARTESIAN_POINT('',(14.,29.9836543272765,-92.34995));
#177360=CARTESIAN_POINT('',(13.5,29.9836543272765,-91.84995));
#177361=CARTESIAN_POINT('Origin',(14.,29.9836543272765,-91.84995));
#177362=CARTESIAN_POINT('Origin',(13.5,29.9835150560362,-91.2987164399481));
#177363=CARTESIAN_POINT('Origin',(14.0082677506659,29.9821486511294,-91.3259572338972));
#177364=CARTESIAN_POINT('Origin',(13.,46.41999998,-92.34995));
#177365=CARTESIAN_POINT('',(13.5,46.41999998,-91.84995));
#177366=CARTESIAN_POINT('',(13.5,46.41999998,-58.2497627936531));
#177367=CARTESIAN_POINT('',(13.5,46.41999998,-58.24995));
#177368=CARTESIAN_POINT('',(13.,46.91999998,-91.84995));
#177369=CARTESIAN_POINT('Origin',(13.,46.41999998,-91.84995));
#177370=CARTESIAN_POINT('',(13.,46.91999998,-58.2497627936531));
#177371=CARTESIAN_POINT('',(13.,46.91999998,-92.34995));
#177372=CARTESIAN_POINT('Origin',(13.,46.41999998,-58.2497627936531));
#177373=CARTESIAN_POINT('Origin',(-39.,46.91999998,-129.34995));
#177374=CARTESIAN_POINT('',(12.5,46.91999998,-91.84995));
#177375=CARTESIAN_POINT('',(-39.,46.91999998,-91.84995));
#177376=CARTESIAN_POINT('',(12.5,46.91999998,-58.2465463958495));
#177377=CARTESIAN_POINT('',(12.5,46.91999998,-58.2396719107252));
#177378=CARTESIAN_POINT('Origin',(13.1654225534,46.91999998,6.33069708304167));
#177379=CARTESIAN_POINT('Origin',(12.5,46.41999998,-92.34995));
#177380=CARTESIAN_POINT('',(12.,46.41999998,-91.84995));
#177381=CARTESIAN_POINT('Origin',(12.5,46.41999998,-91.84995));
#177382=CARTESIAN_POINT('',(12.,46.41999998,-58.2465463958495));
#177383=CARTESIAN_POINT('',(12.,46.41999998,-92.34995));
#177384=CARTESIAN_POINT('Origin',(12.5,46.41999998,-58.2465463958495));
#177385=CARTESIAN_POINT('Ctrl Pts',(11.3828490268763,29.8129372786953,-90.9273970483904));
#177386=CARTESIAN_POINT('Ctrl Pts',(12.,29.6789774176902,-90.8627568967152));
#177387=CARTESIAN_POINT('Ctrl Pts',(12.,30.2507177004773,-91.1386408691297));
#177388=CARTESIAN_POINT('Ctrl Pts',(11.3736122815127,29.7418362505901,-91.0798688801893));
#177389=CARTESIAN_POINT('Ctrl Pts',(11.9999999999987,29.5823965713538,-91.0340021334692));
#177390=CARTESIAN_POINT('Ctrl Pts',(12.,30.2139234693476,-91.2148931255634));
#177391=CARTESIAN_POINT('Ctrl Pts',(11.3694271586094,29.7097409287485,-91.2531177376593));
#177392=CARTESIAN_POINT('Ctrl Pts',(11.9999999999999,29.5374187137922,-91.2360706889224));
#177393=CARTESIAN_POINT('Ctrl Pts',(12.,30.1973151560885,-91.3015254072135));
#177394=CARTESIAN_POINT('Ctrl Pts',(11.3717857023911,29.7278584436048,-91.5056751034728));
#177395=CARTESIAN_POINT('Ctrl Pts',(12.0000000000001,29.5627300607015,-91.5325373605759));
#177396=CARTESIAN_POINT('Ctrl Pts',(12.,30.2066913195442,-91.427825927492));
#177397=CARTESIAN_POINT('Ctrl Pts',(11.3740091557864,29.7449360486904,-91.59034805389));
#177398=CARTESIAN_POINT('Ctrl Pts',(11.9999999999998,29.5864519111761,-91.6308853388652));
#177399=CARTESIAN_POINT('Ctrl Pts',(12.,30.2155293203062,-91.4701692696895));
#177400=CARTESIAN_POINT('Ctrl Pts',(11.3810283772274,29.7989166519369,-91.7500080967778));
#177401=CARTESIAN_POINT('Ctrl Pts',(12.0000000000001,29.6601524162645,-91.8125032590501));
#177402=CARTESIAN_POINT('Ctrl Pts',(12.,30.2434629903521,-91.5500105484349));
#177403=CARTESIAN_POINT('Ctrl Pts',(11.3858517899463,29.8360332465147,-91.8263697865188));
#177404=CARTESIAN_POINT('Ctrl Pts',(11.9999999999999,29.7099192942087,-91.8968680856685));
#177405=CARTESIAN_POINT('Ctrl Pts',(12.,30.2626690028682,-91.5881956385046));
#177406=CARTESIAN_POINT('Ctrl Pts',(11.4037918623192,29.9743449793193,-92.038010246663));
#177407=CARTESIAN_POINT('Ctrl Pts',(12.0000000000002,29.8889381806538,-92.1200651023362));
#177408=CARTESIAN_POINT('Ctrl Pts',(12.,30.3342288077533,-91.6940226905849));
#177409=CARTESIAN_POINT('Ctrl Pts',(11.4201987017183,30.1011425197784,-92.1530192095865));
#177410=CARTESIAN_POINT('Ctrl Pts',(11.9999999999989,30.044850112339,-92.2289441977774));
#177411=CARTESIAN_POINT('Ctrl Pts',(12.,30.3998197343385,-91.7515247512526));
#177412=CARTESIAN_POINT('Ctrl Pts',(11.4619399583253,30.4256124104741,-92.3272312824867));
#177413=CARTESIAN_POINT('Ctrl Pts',(12.0000000000013,30.4142697832356,-92.3669482747856));
#177414=CARTESIAN_POINT('Ctrl Pts',(12.,30.5676008328764,-91.8386125685596));
#177415=CARTESIAN_POINT('Ctrl Pts',(11.4887517849116,30.6352262411195,-92.3673064106212));
#177416=CARTESIAN_POINT('Ctrl Pts',(11.9999999999994,30.6346409292876,-92.3781417391106));
#177417=CARTESIAN_POINT('Ctrl Pts',(12.,30.675950734103,-91.8586341550587));
#177418=CARTESIAN_POINT('Ctrl Pts',(11.5140711352129,30.8347410688585,-92.3430217069376));
#177419=CARTESIAN_POINT('Ctrl Pts',(12.0000000000002,30.8328497940556,-92.3295276769414));
#177420=CARTESIAN_POINT('Ctrl Pts',(12.,30.7790312201287,-91.8464778288845));
#177421=CARTESIAN_POINT('',(12.,30.7194735506599,-91.84995));
#177422=CARTESIAN_POINT('Ctrl Pts',(12.,30.7194735506598,-91.84995));
#177423=CARTESIAN_POINT('Ctrl Pts',(12.,30.6947425199752,-91.84995));
#177424=CARTESIAN_POINT('Ctrl Pts',(12.,30.6701386971986,-91.8481899526742));
#177425=CARTESIAN_POINT('Ctrl Pts',(12.,30.6458464406133,-91.8447815200538));
#177426=CARTESIAN_POINT('Ctrl Pts',(12.,30.6209700785576,-91.841291131929));
#177427=CARTESIAN_POINT('Ctrl Pts',(12.,30.5964191072392,-91.8360720015142));
#177428=CARTESIAN_POINT('Ctrl Pts',(12.,30.5723817191876,-91.8291895987897));
#177429=CARTESIAN_POINT('Ctrl Pts',(12.,30.548553583565,-91.8223671093755));
#177430=CARTESIAN_POINT('Ctrl Pts',(12.,30.5252287940054,-91.8139098291041));
#177431=CARTESIAN_POINT('Ctrl Pts',(12.,30.5026013041075,-91.8038327530222));
#177432=CARTESIAN_POINT('Ctrl Pts',(12.,30.4932234054494,-91.7996563375783));
#177433=CARTESIAN_POINT('Ctrl Pts',(12.,30.4839655197029,-91.7952011432061));
#177434=CARTESIAN_POINT('Ctrl Pts',(12.,30.4748428234451,-91.7904659511164));
#177435=CARTESIAN_POINT('Ctrl Pts',(12.,30.3998197342529,-91.7515247512294));
#177436=CARTESIAN_POINT('Ctrl Pts',(12.,30.3342288071963,-91.6940226895201));
#177437=CARTESIAN_POINT('Ctrl Pts',(12.,30.2865222597932,-91.6234713302197));
#177438=CARTESIAN_POINT('Ctrl Pts',(12.,30.2626689858469,-91.5881956502074));
#177439=CARTESIAN_POINT('Ctrl Pts',(12.,30.2434629741256,-91.5500105562497));
#177440=CARTESIAN_POINT('Ctrl Pts',(12.,30.2294961429083,-91.5100899134078));
#177441=CARTESIAN_POINT('Ctrl Pts',(12.,30.2155293119778,-91.4701692713854));
#177442=CARTESIAN_POINT('Ctrl Pts',(12.,30.2066913177853,-91.427825927269));
#177443=CARTESIAN_POINT('Ctrl Pts',(12.,30.20356593057,-91.3857257541517));
#177444=CARTESIAN_POINT('Ctrl Pts',(12.,30.2016706004035,-91.3601949246491));
#177445=CARTESIAN_POINT('Ctrl Pts',(12.,30.2018789661756,-91.3345298932578));
#177446=CARTESIAN_POINT('Ctrl Pts',(12.,30.2040942316499,-91.3090051705625));
#177447=CARTESIAN_POINT('Ctrl Pts',(12.,30.2063233672373,-91.2833206337077));
#177448=CARTESIAN_POINT('Ctrl Pts',(12.,30.2105848815976,-91.2577766407644));
#177449=CARTESIAN_POINT('Ctrl Pts',(12.,30.2168325161081,-91.2326549802759));
#177450=CARTESIAN_POINT('Ctrl Pts',(12.,30.2228393598883,-91.2085015363124));
#177451=CARTESIAN_POINT('Ctrl Pts',(12.,30.2306827015454,-91.1847372739709));
#177452=CARTESIAN_POINT('Ctrl Pts',(12.,30.2403633283688,-91.1616344702769));
#177453=CARTESIAN_POINT('Ctrl Pts',(12.,30.2436077578597,-91.1538916433923));
#177454=CARTESIAN_POINT('Ctrl Pts',(12.,30.2470588833974,-91.1462233796091));
#177455=CARTESIAN_POINT('Ctrl Pts',(12.,30.2507177004773,-91.1386408691297));
#177456=CARTESIAN_POINT('',(11.5,30.7194735506599,-92.34995));
#177457=CARTESIAN_POINT('Origin',(11.5,30.7194735506599,-91.84995));
#177458=CARTESIAN_POINT('',(11.3712933400037,29.7190889970661,-91.34995));
#177459=CARTESIAN_POINT('Ctrl Pts',(11.3712933400037,29.7190889970661,-91.34995));
#177460=CARTESIAN_POINT('Ctrl Pts',(11.3712933400037,29.7190889970661,-91.4733567786907));
#177461=CARTESIAN_POINT('Ctrl Pts',(11.3741527847607,29.7422826479407,-91.6008386596925));
#177462=CARTESIAN_POINT('Ctrl Pts',(11.3836657034065,29.8155581996794,-91.783323087588));
#177463=CARTESIAN_POINT('Ctrl Pts',(11.3876915067885,29.8463423612377,-91.842649921852));
#177464=CARTESIAN_POINT('Ctrl Pts',(11.394957471004,29.9019098608904,-91.9272311993885));
#177465=CARTESIAN_POINT('Ctrl Pts',(11.3975826489861,29.9219927335249,-91.9546886186485));
#177466=CARTESIAN_POINT('Ctrl Pts',(11.4018054333812,29.9543927938362,-91.9944916815559));
#177467=CARTESIAN_POINT('Ctrl Pts',(11.4039879398925,29.9711612553143,-92.0140473917535));
#177468=CARTESIAN_POINT('Ctrl Pts',(11.4066528137211,29.9916995580463,-92.0361959839154));
#177469=CARTESIAN_POINT('Ctrl Pts',(11.4078195966584,30.0007081718305,-92.0455388832796));
#177470=CARTESIAN_POINT('Ctrl Pts',(11.4086028563942,30.0067595156802,-92.0517335659694));
#177471=CARTESIAN_POINT('Ctrl Pts',(11.4091488014936,30.0109808652905,-92.05598374434));
#177472=CARTESIAN_POINT('Ctrl Pts',(11.4172463075705,30.0736231630541,-92.1184615112787));
#177473=CARTESIAN_POINT('Ctrl Pts',(11.427711960877,30.1586873759409,-92.1882507670382));
#177474=CARTESIAN_POINT('Ctrl Pts',(11.4577433109396,30.3931008233118,-92.3041894616728));
#177475=CARTESIAN_POINT('Ctrl Pts',(11.4776449981906,30.5437415320498,-92.34995));
#177476=CARTESIAN_POINT('Ctrl Pts',(11.5,30.7194735506599,-92.34995));
#177477=CARTESIAN_POINT('Origin',(11.4700666481164,30.4797619500454,-91.297907126496));
#177478=CARTESIAN_POINT('Ctrl Pts',(5.5,31.8716754827171,-92.34995));
#177479=CARTESIAN_POINT('Ctrl Pts',(4.99900616154848,31.8716754827171,-92.34995));
#177480=CARTESIAN_POINT('Ctrl Pts',(5.00000098575356,31.8716754827171,-91.8489571492614));
#177481=CARTESIAN_POINT('Ctrl Pts',(5.48989377680063,31.7056523166615,-92.34995));
#177482=CARTESIAN_POINT('Ctrl Pts',(4.99903601393591,31.7072113826353,-92.3399186475543));
#177483=CARTESIAN_POINT('Ctrl Pts',(5.00000096584847,31.7882063435843,-91.84896712888));
#177484=CARTESIAN_POINT('Ctrl Pts',(5.47963373781052,31.538103809625,-92.3071746231476));
#177485=CARTESIAN_POINT('Ctrl Pts',(4.99906555653679,31.5446619586649,-92.2883582792096));
#177486=CARTESIAN_POINT('Ctrl Pts',(5.0000009456393,31.7039607739187,-91.827630757647));
#177487=CARTESIAN_POINT('Ctrl Pts',(5.46619042199875,31.3196047327668,-92.1878686007335));
#177488=CARTESIAN_POINT('Ctrl Pts',(4.99910325428495,31.3370094182925,-92.161272810455));
#177489=CARTESIAN_POINT('Ctrl Pts',(5.00000091915851,31.5940866659351,-91.7681041344854));
#177490=CARTESIAN_POINT('Ctrl Pts',(5.46194839019336,31.2508398250121,-92.1383294170381));
#177491=CARTESIAN_POINT('Ctrl Pts',(4.99911492812254,31.2726858878275,-92.1103972204605));
#177492=CARTESIAN_POINT('Ctrl Pts',(5.00000091080218,31.5595055375377,-91.7433851154792));
#177493=CARTESIAN_POINT('Ctrl Pts',(5.45439667136824,31.1286541135227,-92.0244078521253));
#177494=CARTESIAN_POINT('Ctrl Pts',(4.99913545432273,31.1595480268539,-91.9961676804233));
#177495=CARTESIAN_POINT('Ctrl Pts',(5.00000089592572,31.4980571027827,-91.6865378587347));
#177496=CARTESIAN_POINT('Ctrl Pts',(5.45108997919633,31.0752759499814,-91.9605552262364));
#177497=CARTESIAN_POINT('Ctrl Pts',(4.99914433728197,31.1105664451878,-91.9333048742067));
#177498=CARTESIAN_POINT('Ctrl Pts',(5.00000088941156,31.4712115049494,-91.6546739801719));
#177499=CARTESIAN_POINT('Ctrl Pts',(5.44262999595016,30.938884482232,-91.7477840212027));
#177500=CARTESIAN_POINT('Ctrl Pts',(4.99916680129804,30.9866628751626,-91.7272955383522));
#177501=CARTESIAN_POINT('Ctrl Pts',(5.00000087274503,31.4026135113348,-91.548492809174));
#177502=CARTESIAN_POINT('Ctrl Pts',(5.43928039898085,30.8851161679224,-91.5835323055617));
#177503=CARTESIAN_POINT('Ctrl Pts',(4.99917557416918,30.9382275273278,-91.5708670061702));
#177504=CARTESIAN_POINT('Ctrl Pts',(5.00000086614598,31.3755689941209,-91.4665221319675));
#177505=CARTESIAN_POINT('Ctrl Pts',(5.43788833142316,30.8627516985332,-91.2503023235849));
#177506=CARTESIAN_POINT('Ctrl Pts',(4.99917920690125,30.918174361902,-91.2558237036598));
#177507=CARTESIAN_POINT('Ctrl Pts',(5.00000086340344,31.3643200540035,-91.3002194649784));
#177508=CARTESIAN_POINT('Ctrl Pts',(5.4398728408893,30.894582824155,-91.0791566847487));
#177509=CARTESIAN_POINT('Ctrl Pts',(4.99917405374089,30.9467642298381,-91.0936720204705));
#177510=CARTESIAN_POINT('Ctrl Pts',(5.00000086731322,31.3803302826741,-91.2148086838993));
#177511=CARTESIAN_POINT('Ctrl Pts',(5.44427033638568,30.9653765476951,-90.9273317382594));
#177512=CARTESIAN_POINT('Ctrl Pts',(4.99916246706145,31.0105597677356,-90.9485621815415));
#177513=CARTESIAN_POINT('Ctrl Pts',(5.0000008759766,31.4159376038041,-91.1390388927805));
#177514=CARTESIAN_POINT('',(5.43844464087133,30.8716892291687,-91.3499500006361));
#177515=CARTESIAN_POINT('Origin',(5.48568341414045,31.6321344502636,-91.297904512692));
#177516=CARTESIAN_POINT('',(5.5,31.8716754827171,-92.34995));
#177517=CARTESIAN_POINT('Ctrl Pts',(5.49999999999999,31.8716754827171,-92.34995));
#177518=CARTESIAN_POINT('Ctrl Pts',(5.4978815673594,31.8368742625198,-92.34995));
#177519=CARTESIAN_POINT('Ctrl Pts',(5.49579787553642,31.8029594634244,-92.348133240981));
#177520=CARTESIAN_POINT('Ctrl Pts',(5.493769479706,31.7700915140547,-92.3447767183816));
#177521=CARTESIAN_POINT('Ctrl Pts',(5.49169197795832,31.7364278566788,-92.3413389369279));
#177522=CARTESIAN_POINT('Ctrl Pts',(5.48967245804065,31.7038621275029,-92.3362865275642));
#177523=CARTESIAN_POINT('Ctrl Pts',(5.48772616666163,31.6725108730827,-92.3299137899354));
#177524=CARTESIAN_POINT('Ctrl Pts',(5.48573075716194,31.6403684140593,-92.3233802249508));
#177525=CARTESIAN_POINT('Ctrl Pts',(5.48381228263233,31.609502182019,-92.3154593937791));
#177526=CARTESIAN_POINT('Ctrl Pts',(5.48198053529549,31.5799839743614,-92.3064561998247));
#177527=CARTESIAN_POINT('Ctrl Pts',(5.48001777371976,31.548354500902,-92.2968090597431));
#177528=CARTESIAN_POINT('Ctrl Pts',(5.47815458294883,31.5182727007077,-92.2859199157918));
#177529=CARTESIAN_POINT('Ctrl Pts',(5.47639575095647,31.4897685177843,-92.2741396830177));
#177530=CARTESIAN_POINT('Ctrl Pts',(5.47464127727594,31.4613349670296,-92.2623886411658));
#177531=CARTESIAN_POINT('Ctrl Pts',(5.47299054949597,31.4344704273083,-92.2497512170054));
#177532=CARTESIAN_POINT('Ctrl Pts',(5.47144226944925,31.4091563595002,-92.2365449915221));
#177533=CARTESIAN_POINT('Ctrl Pts',(5.46982926682253,31.3827840905079,-92.2227867076515));
#177534=CARTESIAN_POINT('Ctrl Pts',(5.46832739057934,31.3580940820943,-92.2084115017261));
#177535=CARTESIAN_POINT('Ctrl Pts',(5.46692979196242,31.3350228801632,-92.1937391327595));
#177536=CARTESIAN_POINT('Ctrl Pts',(5.46563435464848,31.3136381309962,-92.1801392808328));
#177537=CARTESIAN_POINT('Ctrl Pts',(5.46442839146343,31.2936432479195,-92.1662837176707));
#177538=CARTESIAN_POINT('Ctrl Pts',(5.46330338345437,31.2749638086464,-92.1523952289126));
#177539=CARTESIAN_POINT('Ctrl Pts',(5.46199291939706,31.2532050890809,-92.1362172415728));
#177540=CARTESIAN_POINT('Ctrl Pts',(5.46079227751257,31.2332310339142,-92.1199956745703));
#177541=CARTESIAN_POINT('Ctrl Pts',(5.45968468767403,31.2148987829739,-92.1040310703102));
#177542=CARTESIAN_POINT('Ctrl Pts',(5.45913089275476,31.2057326575037,-92.0960487681802));
#177543=CARTESIAN_POINT('Ctrl Pts',(5.45860031611243,31.1969766464014,-92.0881298511603));
#177544=CARTESIAN_POINT('Ctrl Pts',(5.4580906611324,31.1886114184243,-92.080306896806));
#177545=CARTESIAN_POINT('Ctrl Pts',(5.45783583364236,31.1844288044357,-92.0763954196288));
#177546=CARTESIAN_POINT('Ctrl Pts',(5.4575862390359,31.1803439061936,-92.072507911857));
#177547=CARTESIAN_POINT('Ctrl Pts',(5.4573415784771,31.1763542226034,-92.0686481149132));
#177548=CARTESIAN_POINT('Ctrl Pts',(5.45721924819772,31.1743593808083,-92.0667182164412));
#177549=CARTESIAN_POINT('Ctrl Pts',(5.45709815159589,31.1723883440164,-92.0647952442053));
#177550=CARTESIAN_POINT('Ctrl Pts',(5.45697825169214,31.1704408029121,-92.0628796526239));
#177551=CARTESIAN_POINT('Ctrl Pts',(5.45689074900465,31.1690194916743,-92.061481658078));
#177552=CARTESIAN_POINT('Ctrl Pts',(5.45684243353217,31.1682316144817,-92.0607031835794));
#177553=CARTESIAN_POINT('Ctrl Pts',(5.45674878977622,31.1667167878402,-92.0591974721066));
#177554=CARTESIAN_POINT('Ctrl Pts',(5.45671411887524,31.1661559345943,-92.0586399936838));
#177555=CARTESIAN_POINT('Ctrl Pts',(5.45667326412361,31.1654956759037,-92.057982576319));
#177556=CARTESIAN_POINT('Ctrl Pts',(5.45662210535926,31.164668359648,-92.0571554655836));
#177557=CARTESIAN_POINT('Ctrl Pts',(5.45476221172077,31.1345910061276,-92.0270855838199));
#177558=CARTESIAN_POINT('Ctrl Pts',(5.45302521158081,31.1066918096424,-91.9953506844654));
#177559=CARTESIAN_POINT('Ctrl Pts',(5.45142749767532,31.0810905033727,-91.9622939859181));
#177560=CARTESIAN_POINT('Ctrl Pts',(5.44981011830393,31.0551740833559,-91.9288304089078));
#177561=CARTESIAN_POINT('Ctrl Pts',(5.44833546364656,31.0316123470578,-91.8940128061608));
#177562=CARTESIAN_POINT('Ctrl Pts',(5.44701370805013,31.0104761931718,-91.8581941654681));
#177563=CARTESIAN_POINT('Ctrl Pts',(5.44567535131068,30.9890745709085,-91.8219256455554));
#177564=CARTESIAN_POINT('Ctrl Pts',(5.44449373720189,30.9701596493975,-91.7846312698169));
#177565=CARTESIAN_POINT('Ctrl Pts',(5.44347271632439,30.9537531147354,-91.7466667565915));
#177566=CARTESIAN_POINT('Ctrl Pts',(5.44243190076202,30.9370285041252,-91.7079662196546));
#177567=CARTESIAN_POINT('Ctrl Pts',(5.44155794121925,30.9229102693208,-91.6685697880071));
#177568=CARTESIAN_POINT('Ctrl Pts',(5.44084832463001,30.911370814837,-91.6288357624295));
#177569=CARTESIAN_POINT('Ctrl Pts',(5.44013077807845,30.8997024069992,-91.5886577092878));
#177570=CARTESIAN_POINT('Ctrl Pts',(5.43958122565515,30.8906703898251,-91.5481348790471));
#177571=CARTESIAN_POINT('Ctrl Pts',(5.43919091728486,30.8841994180308,-91.5076122570601));
#177572=CARTESIAN_POINT('Ctrl Pts',(5.4387941168249,30.8776208130615,-91.4664156129009));
#177573=CARTESIAN_POINT('Ctrl Pts',(5.43856185618865,30.8736887906221,-91.4252195592088));
#177574=CARTESIAN_POINT('Ctrl Pts',(5.43847928442791,30.8722814764636,-91.3843544127705));
#177575=CARTESIAN_POINT('Ctrl Pts',(5.43845605490473,30.8718855634231,-91.3728580142727));
#177576=CARTESIAN_POINT('Ctrl Pts',(5.43844464087176,30.871689229176,-91.3613875941317));
#177577=CARTESIAN_POINT('Ctrl Pts',(5.43844464087133,30.8716892291687,-91.3499500006361));
#177578=CARTESIAN_POINT('',(5.,31.8716754827171,-91.84995));
#177579=CARTESIAN_POINT('Origin',(5.5,31.8716754827171,-91.84995));
#177580=CARTESIAN_POINT('Ctrl Pts',(5.,31.415090518797,-91.1386408691297));
#177581=CARTESIAN_POINT('Ctrl Pts',(5.,31.3430615709327,-91.2919348798756));
#177582=CARTESIAN_POINT('Ctrl Pts',(5.,31.355929990322,-91.4779432828738));
#177583=CARTESIAN_POINT('Ctrl Pts',(5.,31.5391820921123,-91.7616382083514));
#177584=CARTESIAN_POINT('Ctrl Pts',(5.,31.7023337675853,-91.84995));
#177585=CARTESIAN_POINT('Ctrl Pts',(5.,31.8716754827171,-91.84995));
#177586=CARTESIAN_POINT('Origin',(4.5,46.41999998,-92.34995));
#177587=CARTESIAN_POINT('',(5.,46.41999998,-91.84995));
#177588=CARTESIAN_POINT('',(5.,46.41999998,-57.9428177527387));
#177589=CARTESIAN_POINT('',(5.,46.41999998,-57.9628508566217));
#177590=CARTESIAN_POINT('',(4.5,46.91999998,-91.84995));
#177591=CARTESIAN_POINT('Origin',(4.5,46.41999998,-91.84995));
#177592=CARTESIAN_POINT('',(4.5,46.91999998,-57.9428177527387));
#177593=CARTESIAN_POINT('',(4.5,46.91999998,-92.34995));
#177594=CARTESIAN_POINT('Origin',(4.5,46.41999998,-57.9428177527387));
#177595=CARTESIAN_POINT('Origin',(-39.,46.91999998,-129.34995));
#177596=CARTESIAN_POINT('',(4.,46.91999998,-91.84995));
#177597=CARTESIAN_POINT('',(-39.,46.91999998,-91.84995));
#177598=CARTESIAN_POINT('',(4.,46.91999998,-57.9242045702762));
#177599=CARTESIAN_POINT('',(4.,46.91999998,-57.9072287192657));
#177600=CARTESIAN_POINT('Ctrl Pts',(4.,46.91999998,-57.9242045702762));
#177601=CARTESIAN_POINT('Ctrl Pts',(4.16667353124555,46.91999998,-57.9301478976981));
#177602=CARTESIAN_POINT('Ctrl Pts',(4.33333987978916,46.91999998,-57.9363643903873));
#177603=CARTESIAN_POINT('Ctrl Pts',(4.5,46.91999998,-57.9428177527387));
#177604=CARTESIAN_POINT('Origin',(4.,46.41999998,-92.34995));
#177605=CARTESIAN_POINT('',(3.5,46.41999998,-91.84995));
#177606=CARTESIAN_POINT('Origin',(4.,46.41999998,-91.84995));
#177607=CARTESIAN_POINT('',(3.5,46.41999998,-57.9242045702762));
#177608=CARTESIAN_POINT('',(3.5,46.41999998,-92.34995));
#177609=CARTESIAN_POINT('Origin',(4.,46.41999998,-57.9242045702762));
#177610=CARTESIAN_POINT('Ctrl Pts',(41.0540572871253,28.7076050220164,-93.3976987687948));
#177611=CARTESIAN_POINT('Ctrl Pts',(40.9209666515892,28.8387123238495,-93.5739383154377));
#177612=CARTESIAN_POINT('Ctrl Pts',(40.9899542848408,29.0638025010082,-93.6765918018241));
#177613=CARTESIAN_POINT('Ctrl Pts',(40.8263518506557,28.931917162897,-93.0559775318146));
#177614=CARTESIAN_POINT('Ctrl Pts',(40.6946394065552,29.0602110175707,-93.2636650794047));
#177615=CARTESIAN_POINT('Ctrl Pts',(40.7930602005308,29.2900891143653,-93.3836137237161));
#177616=CARTESIAN_POINT('Ctrl Pts',(40.5620537232219,29.1885351995273,-92.7839978150636));
#177617=CARTESIAN_POINT('Ctrl Pts',(40.4345448959912,29.3109818121476,-93.0268336432776));
#177618=CARTESIAN_POINT('Ctrl Pts',(40.5646325235533,29.548843193136,-93.1505624120075));
#177619=CARTESIAN_POINT('Ctrl Pts',(39.979050150362,29.7418321774292,-92.3381410201203));
#177620=CARTESIAN_POINT('Ctrl Pts',(39.8699190705461,29.8439046252157,-92.6499647524336));
#177621=CARTESIAN_POINT('Ctrl Pts',(40.0606440851126,30.1068692044787,-92.7683994467215));
#177622=CARTESIAN_POINT('Ctrl Pts',(39.6579655806366,30.0405777253273,-92.1665648604216));
#177623=CARTESIAN_POINT('Ctrl Pts',(39.5589873293178,30.1314683688792,-92.5153277294035));
#177624=CARTESIAN_POINT('Ctrl Pts',(39.7830757934441,30.4081688522969,-92.6213339269874));
#177625=CARTESIAN_POINT('Ctrl Pts',(39.3277310924369,30.3404619167909,-92.0491293459315));
#177626=CARTESIAN_POINT('Ctrl Pts',(39.2532568247562,30.4080916052286,-92.4345203712043));
#177627=CARTESIAN_POINT('Ctrl Pts',(39.4975990396159,30.7106154376184,-92.5206751536556));
#177628=CARTESIAN_POINT('',(39.4975990396159,30.7106154376184,-92.5206751536556));
#177629=CARTESIAN_POINT('Origin',(39.6638655462185,30.7106154376184,-92.0491293459315));
#177630=CARTESIAN_POINT('',(40.9899542848408,29.0638025010082,-93.6765918018241));
#177631=CARTESIAN_POINT('Origin',(41.4049466656476,29.0638025010082,-93.3976987687947));
#177632=CARTESIAN_POINT('Ctrl Pts',(39.4975990396159,30.7106154376184,-92.5206751536556));
#177633=CARTESIAN_POINT('Ctrl Pts',(39.5502437311338,30.6548413440315,-92.5392376110171));
#177634=CARTESIAN_POINT('Ctrl Pts',(39.6012366148037,30.6005720208656,-92.5588889597982));
#177635=CARTESIAN_POINT('Ctrl Pts',(39.6505780614367,30.5478567214463,-92.5794001703044));
#177636=CARTESIAN_POINT('Ctrl Pts',(39.7019051901957,30.4930199635987,-92.6007368277089));
#177637=CARTESIAN_POINT('Ctrl Pts',(39.7514455416351,30.4398645312726,-92.6230039260027));
#177638=CARTESIAN_POINT('Ctrl Pts',(39.799227420812,30.3884074698674,-92.6459761157129));
#177639=CARTESIAN_POINT('Ctrl Pts',(39.8509326004218,30.332725344175,-92.6708345184267));
#177640=CARTESIAN_POINT('Ctrl Pts',(39.900578831291,30.2790318107528,-92.6965182934803));
#177641=CARTESIAN_POINT('Ctrl Pts',(39.9482309785535,30.2273074761566,-92.7227817257198));
#177642=CARTESIAN_POINT('Ctrl Pts',(39.9787063007134,30.194227838598,-92.7395781683673));
#177643=CARTESIAN_POINT('Ctrl Pts',(40.0083613832834,30.161958444705,-92.7566098271306));
#177644=CARTESIAN_POINT('Ctrl Pts',(40.0372057906019,30.1305006022898,-92.7738119274539));
#177645=CARTESIAN_POINT('Ctrl Pts',(40.0970075868769,30.0652804900306,-92.8094762587635));
#177646=CARTESIAN_POINT('Ctrl Pts',(40.1533265445702,30.0035479209865,-92.8458721381057));
#177647=CARTESIAN_POINT('Ctrl Pts',(40.2062866145755,29.945258258757,-92.8824715547153));
#177648=CARTESIAN_POINT('Ctrl Pts',(40.2376516594108,29.9107368189424,-92.9041471745321));
#177649=CARTESIAN_POINT('Ctrl Pts',(40.2678386038127,29.877422603041,-92.925894814687));
#177650=CARTESIAN_POINT('Ctrl Pts',(40.2968760309461,29.8453006562658,-92.9476110057979));
#177651=CARTESIAN_POINT('Ctrl Pts',(40.2997081664554,29.8421676753142,-92.9497290721021));
#177652=CARTESIAN_POINT('Ctrl Pts',(40.3015941680139,29.8400809906412,-92.9511431029648));
#177653=CARTESIAN_POINT('Ctrl Pts',(40.3049675683909,29.8363475009641,-92.953683917945));
#177654=CARTESIAN_POINT('Ctrl Pts',(40.3054835593242,29.8357764312398,-92.9540725576991));
#177655=CARTESIAN_POINT('Ctrl Pts',(40.306034306853,29.8351668697406,-92.95448763497));
#177656=CARTESIAN_POINT('Ctrl Pts',(40.3066284628192,29.8345092283034,-92.9549358002383));
#177657=CARTESIAN_POINT('Ctrl Pts',(40.3086347740026,29.8322885430872,-92.9564491385554));
#177658=CARTESIAN_POINT('Ctrl Pts',(40.3106380437744,29.8300708433843,-92.9579641773452));
#177659=CARTESIAN_POINT('Ctrl Pts',(40.3126382671633,29.8278561371225,-92.9594809011795));
#177660=CARTESIAN_POINT('Ctrl Pts',(40.3644584567136,29.7704792966522,-92.9987749705472));
#177661=CARTESIAN_POINT('Ctrl Pts',(40.4143172745278,29.7150280799745,-93.0391169254633));
#177662=CARTESIAN_POINT('Ctrl Pts',(40.4622134803595,29.6615579422969,-93.0804043143038));
#177663=CARTESIAN_POINT('Ctrl Pts',(40.5106606856377,29.6074726824868,-93.122166674554));
#177664=CARTESIAN_POINT('Ctrl Pts',(40.5570999020178,29.5554143181597,-93.164896282026));
#177665=CARTESIAN_POINT('Ctrl Pts',(40.6015490772091,29.5054130210184,-93.2084453489337));
#177666=CARTESIAN_POINT('Ctrl Pts',(40.6471301804922,29.4541384072719,-93.2531034220713));
#177667=CARTESIAN_POINT('Ctrl Pts',(40.690618621974,29.4050269608719,-93.2986231900119));
#177668=CARTESIAN_POINT('Ctrl Pts',(40.7320534431439,29.3580828825712,-93.3448022074815));
#177669=CARTESIAN_POINT('Ctrl Pts',(40.774314355202,29.310202874677,-93.3919019014374));
#177670=CARTESIAN_POINT('Ctrl Pts',(40.8144390257268,29.264577440295,-93.4396872428883));
#177671=CARTESIAN_POINT('Ctrl Pts',(40.8524882640605,29.2211825760875,-93.4879006275346));
#177672=CARTESIAN_POINT('Ctrl Pts',(40.8920154539822,29.1761021194406,-93.5379867710458));
#177673=CARTESIAN_POINT('Ctrl Pts',(40.929302926327,29.1334288224211,-93.588534721447));
#177674=CARTESIAN_POINT('Ctrl Pts',(40.964438429471,29.0931062913192,-93.6392119293362));
#177675=CARTESIAN_POINT('Ctrl Pts',(40.9730731090496,29.0831968804752,-93.6516660402185));
#177676=CARTESIAN_POINT('Ctrl Pts',(40.9815779064276,29.0734293123152,-93.664127764331));
#177677=CARTESIAN_POINT('Ctrl Pts',(40.9899542848408,29.0638025010082,-93.6765918018241));
#177678=CARTESIAN_POINT('Ctrl Pts',(39.3571428571429,31.080768958446,-92.4750054575003));
#177679=CARTESIAN_POINT('Ctrl Pts',(39.,31.080768958446,-92.3685260300003));
#177680=CARTESIAN_POINT('Ctrl Pts',(39.,31.080768958446,-91.9958480337503));
#177681=CARTESIAN_POINT('Ctrl Pts',(39.3571429430277,30.9391538899445,-92.4750054831062));
#177682=CARTESIAN_POINT('Ctrl Pts',(39.0000001561187,30.8288322275033,-92.3685260646169));
#177683=CARTESIAN_POINT('Ctrl Pts',(39.,30.7973529986378,-91.9958480635187));
#177684=CARTESIAN_POINT('Ctrl Pts',(39.410274588038,30.8031308123719,-92.4898846529936));
#177685=CARTESIAN_POINT('Ctrl Pts',(39.0995023767794,30.5843250255347,-92.3886066067861));
#177686=CARTESIAN_POINT('Ctrl Pts',(39.1237015311635,30.5257400818631,-92.0131591004063));
#177687=CARTESIAN_POINT('Ctrl Pts',(39.4975990396159,30.7106154376184,-92.5206751536556));
#177688=CARTESIAN_POINT('Ctrl Pts',(39.2532568247562,30.4080916052285,-92.4345203712043));
#177689=CARTESIAN_POINT('Ctrl Pts',(39.3277310924369,30.3404619167909,-92.0491293459315));
#177690=CARTESIAN_POINT('',(39.3571428571429,31.080768958446,-92.4750054575003));
#177691=CARTESIAN_POINT('Origin',(39.5,31.080768958446,-91.9958480337503));
#177692=CARTESIAN_POINT('Ctrl Pts',(39.3571428571429,31.080768958446,-92.4750054575003));
#177693=CARTESIAN_POINT('Ctrl Pts',(39.3571428624528,31.0720133575057,-92.4750054590834));
#177694=CARTESIAN_POINT('Ctrl Pts',(39.3573458482566,31.0633092009137,-92.4750623091666));
#177695=CARTESIAN_POINT('Ctrl Pts',(39.3577390766937,31.0546580420142,-92.475173820379));
#177696=CARTESIAN_POINT('Ctrl Pts',(39.3586243755247,31.0351811676592,-92.4754248722785));
#177697=CARTESIAN_POINT('Ctrl Pts',(39.3604436448217,31.0159715870608,-92.4759439815933));
#177698=CARTESIAN_POINT('Ctrl Pts',(39.3631916882095,30.9970230542622,-92.476746763375));
#177699=CARTESIAN_POINT('Ctrl Pts',(39.3641054890546,30.9907221401785,-92.4770137106414));
#177700=CARTESIAN_POINT('Ctrl Pts',(39.3651223182342,30.9844503546779,-92.4773121194727));
#177701=CARTESIAN_POINT('Ctrl Pts',(39.3662428843127,30.9782083090249,-92.4776428409703));
#177702=CARTESIAN_POINT('Ctrl Pts',(39.3683883585622,30.9662570743143,-92.4782760516934));
#177703=CARTESIAN_POINT('Ctrl Pts',(39.3708845217043,30.9545679259021,-92.4790189420789));
#177704=CARTESIAN_POINT('Ctrl Pts',(39.3737461808994,30.9429694337232,-92.4798801534962));
#177705=CARTESIAN_POINT('Ctrl Pts',(39.3765700228016,30.9315242175094,-92.4807299838641));
#177706=CARTESIAN_POINT('Ctrl Pts',(39.3797500540198,30.9201667541774,-92.481695025529));
#177707=CARTESIAN_POINT('Ctrl Pts',(39.3833449200573,30.9087492309475,-92.482798172154));
#177708=CARTESIAN_POINT('Ctrl Pts',(39.3862733107318,30.8994484758694,-92.4836967993228));
#177709=CARTESIAN_POINT('Ctrl Pts',(39.3894777725275,30.8901079961926,-92.4846873039166));
#177710=CARTESIAN_POINT('Ctrl Pts',(39.3930110105606,30.8806604192302,-92.4857896691593));
#177711=CARTESIAN_POINT('Ctrl Pts',(39.3991440441352,30.8642612108655,-92.4877031669144));
#177712=CARTESIAN_POINT('Ctrl Pts',(39.4059290901326,30.8484191983756,-92.4898483081196));
#177713=CARTESIAN_POINT('Ctrl Pts',(39.4133615041905,30.833134388963,-92.492236979355));
#177714=CARTESIAN_POINT('Ctrl Pts',(39.418935814734,30.8216707819036,-92.4940284827816));
#177715=CARTESIAN_POINT('Ctrl Pts',(39.4248742687166,30.8105206008932,-92.495956985567));
#177716=CARTESIAN_POINT('Ctrl Pts',(39.4311748370853,30.7996838446308,-92.4980279306107));
#177717=CARTESIAN_POINT('Ctrl Pts',(39.4406256896384,30.7834287102371,-92.5011343481761));
#177718=CARTESIAN_POINT('Ctrl Pts',(39.4508913265187,30.7678787816064,-92.5045611481668));
#177719=CARTESIAN_POINT('Ctrl Pts',(39.4619645235623,30.753034049853,-92.5083285582182));
#177720=CARTESIAN_POINT('Ctrl Pts',(39.4675011220841,30.7456116839763,-92.5102122632439));
#177721=CARTESIAN_POINT('Ctrl Pts',(39.4732396026272,30.7383656171964,-92.5121811573189));
#177722=CARTESIAN_POINT('Ctrl Pts',(39.4791790118521,30.7312958485624,-92.5142379855905));
#177723=CARTESIAN_POINT('Ctrl Pts',(39.485118421077,30.7242260799284,-92.516294813862));
#177724=CARTESIAN_POINT('Ctrl Pts',(39.4912587585353,30.7173326092718,-92.5184395778772));
#177725=CARTESIAN_POINT('Ctrl Pts',(39.4975990396159,30.7106154376184,-92.5206751536556));
#177726=CARTESIAN_POINT('Origin',(39.5,58.91999998,-91.9958480337503));
#177727=CARTESIAN_POINT('',(39.3571428571429,46.41999998,-92.4750054575003));
#177728=CARTESIAN_POINT('Origin',(39.5,46.41999998,-91.9958480337503));
#177729=CARTESIAN_POINT('',(39.,46.41999998,-91.9958480337503));
#177730=CARTESIAN_POINT('',(39.3571428571429,58.91999998,-92.4750054575003));
#177731=CARTESIAN_POINT('Origin',(38.5,28.91999998,-95.34995));
#177732=CARTESIAN_POINT('',(41.2907166092886,28.91999998,-94.2490863360338));
#177733=CARTESIAN_POINT('Origin',(41.75583604417,28.91999998,-94.0656090587062));
#177734=CARTESIAN_POINT('Origin',(38.5,28.41999998,-95.34995));
#177735=CARTESIAN_POINT('Origin',(38.5,28.91999998,-95.34995));
#177736=CARTESIAN_POINT('Ctrl Pts',(40.9899542848408,29.0638025010082,-93.6765918018241));
#177737=CARTESIAN_POINT('Ctrl Pts',(40.9209666515892,28.8387123238495,-93.5739383154377));
#177738=CARTESIAN_POINT('Ctrl Pts',(41.0540572871253,28.7076050220164,-93.3976987687948));
#177739=CARTESIAN_POINT('Ctrl Pts',(41.0445777715999,29.0010249744694,-93.7578714615268));
#177740=CARTESIAN_POINT('Ctrl Pts',(40.9927653037546,28.7197223139655,-93.6733291751567));
#177741=CARTESIAN_POINT('Ctrl Pts',(41.181465342889,28.5820956174237,-93.4924903917862));
#177742=CARTESIAN_POINT('Ctrl Pts',(41.1012013116007,28.9670983124193,-93.8513385014916));
#177743=CARTESIAN_POINT('Ctrl Pts',(41.064373682842,28.640994986895,-93.7860557549848));
#177744=CARTESIAN_POINT('Ctrl Pts',(41.3136336664734,28.5141965951637,-93.601569918277));
#177745=CARTESIAN_POINT('Ctrl Pts',(41.203906529354,28.9262911739198,-94.0457359962981));
#177746=CARTESIAN_POINT('Ctrl Pts',(41.1909352247283,28.5106646509549,-94.0164009875504));
#177747=CARTESIAN_POINT('Ctrl Pts',(41.5532792074141,28.4325824175145,-93.828366995811));
#177748=CARTESIAN_POINT('Ctrl Pts',(41.2500626594833,28.9199999557335,-94.1460275680244));
#177749=CARTESIAN_POINT('Ctrl Pts',(41.245616944193,28.4623003387481,-94.1347575623882));
#177750=CARTESIAN_POINT('Ctrl Pts',(41.6609761593771,28.4199999800001,-93.9453729847263));
#177751=CARTESIAN_POINT('Ctrl Pts',(41.2907166092886,28.91999998,-94.2490863360339));
#177752=CARTESIAN_POINT('Ctrl Pts',(41.2907166092886,28.4199999800001,-94.2490863360339));
#177753=CARTESIAN_POINT('Ctrl Pts',(41.7558360441699,28.41999998,-94.0656090587062));
#177754=CARTESIAN_POINT('Ctrl Pts',(40.9899542848408,29.0638025010082,-93.6765918018241));
#177755=CARTESIAN_POINT('Ctrl Pts',(41.0017693811953,29.0502236370209,-93.6941726460364));
#177756=CARTESIAN_POINT('Ctrl Pts',(41.0140708376759,29.0375478614379,-93.7129059904779));
#177757=CARTESIAN_POINT('Ctrl Pts',(41.0268202538681,29.0258419966797,-93.7328567862257));
#177758=CARTESIAN_POINT('Ctrl Pts',(41.0391013343248,29.0145661339467,-93.7520747115062));
#177759=CARTESIAN_POINT('Ctrl Pts',(41.0517974761858,29.0041919373727,-93.7724211552444));
#177760=CARTESIAN_POINT('Ctrl Pts',(41.0648448407171,28.9947506178104,-93.7939356517422));
#177761=CARTESIAN_POINT('Ctrl Pts',(41.0769698659622,28.9859767203872,-93.8139292537102));
#177762=CARTESIAN_POINT('Ctrl Pts',(41.0893969827306,28.978009516043,-93.8349292598603));
#177763=CARTESIAN_POINT('Ctrl Pts',(41.1020540344261,28.970836888857,-93.8569624977988));
#177764=CARTESIAN_POINT('Ctrl Pts',(41.114660062725,28.9636931761299,-93.8789069148439));
#177765=CARTESIAN_POINT('Ctrl Pts',(41.1274932261777,28.9573390332433,-93.9018734002197));
#177766=CARTESIAN_POINT('Ctrl Pts',(41.1404601253197,28.9517165675485,-93.9258935221142));
#177767=CARTESIAN_POINT('Ctrl Pts',(41.1426479037218,28.9507679437581,-93.9299462029689));
#177768=CARTESIAN_POINT('Ctrl Pts',(41.1451435660091,28.949712012454,-93.9345963342413));
#177769=CARTESIAN_POINT('Ctrl Pts',(41.1473963625423,28.9487825885311,-93.938820756772));
#177770=CARTESIAN_POINT('Ctrl Pts',(41.1488876270705,28.9481673456952,-93.9416171617641));
#177771=CARTESIAN_POINT('Ctrl Pts',(41.1502729027338,28.9476061534381,-93.9442266086178));
#177772=CARTESIAN_POINT('Ctrl Pts',(41.1513966516507,28.9471554910944,-93.9463491184234));
#177773=CARTESIAN_POINT('Ctrl Pts',(41.151782175637,28.9470008825865,-93.947077286815));
#177774=CARTESIAN_POINT('Ctrl Pts',(41.1521678999204,28.9468468449385,-93.9478066003647));
#177775=CARTESIAN_POINT('Ctrl Pts',(41.152553818993,28.9466933775795,-93.9485370568041));
#177776=CARTESIAN_POINT('Ctrl Pts',(41.1650174545953,28.9417369984439,-93.972127865167));
#177777=CARTESIAN_POINT('Ctrl Pts',(41.177689249371,28.937413983186,-93.996873043816));
#177778=CARTESIAN_POINT('Ctrl Pts',(41.1904798430551,28.9337971267814,-94.0228026361174));
#177779=CARTESIAN_POINT('Ctrl Pts',(41.2027935565744,28.9303151200265,-94.0477654782778));
#177780=CARTESIAN_POINT('Ctrl Pts',(41.2152173467937,28.9274879657075,-94.0738260971387));
#177781=CARTESIAN_POINT('Ctrl Pts',(41.2276649958569,28.9253345395707,-94.1010116186227));
#177782=CARTESIAN_POINT('Ctrl Pts',(41.239510966971,28.92328520289,-94.1268830824301));
#177783=CARTESIAN_POINT('Ctrl Pts',(41.2513785111291,28.9218461913099,-94.153773355429));
#177784=CARTESIAN_POINT('Ctrl Pts',(41.2631878035387,28.9209877361867,-94.181705677918));
#177785=CARTESIAN_POINT('Ctrl Pts',(41.2724131953157,28.9203171130402,-94.2035263433116));
#177786=CARTESIAN_POINT('Ctrl Pts',(41.2816029331176,28.91999997456,-94.2259829415861));
#177787=CARTESIAN_POINT('Ctrl Pts',(41.2907166092885,28.91999998,-94.2490863360338));
#177788=CARTESIAN_POINT('Ctrl Pts',(38.9935757799223,46.3414635373644,-91.9917603781375));
#177789=CARTESIAN_POINT('Ctrl Pts',(38.9900733339343,46.3237628848257,-92.3673479459613));
#177790=CARTESIAN_POINT('Ctrl Pts',(39.3465508854728,46.2628551564744,-92.471625094235));
#177791=CARTESIAN_POINT('Ctrl Pts',(39.0086597700523,46.4322161067703,-92.0014907415683));
#177792=CARTESIAN_POINT('Ctrl Pts',(39.0135957341955,46.4340914316513,-92.3710345401694));
#177793=CARTESIAN_POINT('Ctrl Pts',(39.372415088039,46.4444445610447,-92.4799718784786));
#177794=CARTESIAN_POINT('Ctrl Pts',(38.9968525252245,46.5274603514191,-91.9931823769061));
#177795=CARTESIAN_POINT('Ctrl Pts',(38.9935526885049,46.5545728778829,-92.3674784092348));
#177796=CARTESIAN_POINT('Ctrl Pts',(39.352171245683,46.6350158585226,-92.472845419099));
#177797=CARTESIAN_POINT('Ctrl Pts',(38.9364433009268,46.6726027208644,-91.9601428292582));
#177798=CARTESIAN_POINT('Ctrl Pts',(38.911047638376,46.7195613858442,-92.3581836088519));
#177799=CARTESIAN_POINT('Ctrl Pts',(39.248577561246,46.9254427981845,-92.4445007012883));
#177800=CARTESIAN_POINT('Ctrl Pts',(38.8992979918264,46.7278476911263,-91.9409870962964));
#177801=CARTESIAN_POINT('Ctrl Pts',(38.8613543660254,46.7770521061531,-92.3536048202297));
#177802=CARTESIAN_POINT('Ctrl Pts',(39.1848780116966,47.0359893155312,-92.4280665419693));
#177803=CARTESIAN_POINT('Ctrl Pts',(38.8075082704007,46.819559441354,-91.903134346114));
#177804=CARTESIAN_POINT('Ctrl Pts',(38.7552065584773,46.8601509227914,-92.3483332716903));
#177805=CARTESIAN_POINT('Ctrl Pts',(39.0274561372425,47.2195137681446,-92.3955887391387));
#177806=CARTESIAN_POINT('Ctrl Pts',(38.7519713842669,46.8567503512399,-91.884306817494));
#177807=CARTESIAN_POINT('Ctrl Pts',(38.698339541767,46.8858041857146,-92.3478246517919));
#177808=CARTESIAN_POINT('Ctrl Pts',(38.9322034872781,47.2939415269622,-92.3794330966327));
#177809=CARTESIAN_POINT('Ctrl Pts',(38.6076467465342,46.9167126634347,-91.8524730691734));
#177810=CARTESIAN_POINT('Ctrl Pts',(38.5727409105641,46.9214414682097,-92.3493758984604));
#177811=CARTESIAN_POINT('Ctrl Pts',(38.6846545006084,47.4139412866979,-92.3521157644398));
#177812=CARTESIAN_POINT('Ctrl Pts',(38.5109178162184,46.9287522863742,-91.8445567093303));
#177813=CARTESIAN_POINT('Ctrl Pts',(38.5081212350499,46.9220589191625,-92.3516898082073));
#177814=CARTESIAN_POINT('Ctrl Pts',(38.5187272696553,47.4380404247362,-92.345320843866));
#177815=CARTESIAN_POINT('Ctrl Pts',(38.4229506706146,46.9135241055511,-91.8538609392359));
#177816=CARTESIAN_POINT('Ctrl Pts',(38.4459457313602,46.9181397812628,-92.3496852111588));
#177817=CARTESIAN_POINT('Ctrl Pts',(38.3678334725473,47.4075618803718,-92.353306306564));
#177818=CARTESIAN_POINT('',(38.5,47.41999998,-92.34995));
#177819=CARTESIAN_POINT('Origin',(38.5,47.41999998,-91.84995));
#177820=CARTESIAN_POINT('Ctrl Pts',(38.5,47.41999998,-92.34995));
#177821=CARTESIAN_POINT('Ctrl Pts',(38.6219812275058,47.41999998,-92.34995));
#177822=CARTESIAN_POINT('Ctrl Pts',(38.7465335263591,47.3872258650965,-92.3582058121698));
#177823=CARTESIAN_POINT('Ctrl Pts',(38.904967841915,47.3039420525654,-92.3769331713773));
#177824=CARTESIAN_POINT('Ctrl Pts',(38.9543966496893,47.2707466454047,-92.3841945628516));
#177825=CARTESIAN_POINT('Ctrl Pts',(39.0234767926682,47.2128023301881,-92.395882049767));
#177826=CARTESIAN_POINT('Ctrl Pts',(39.0456603010004,47.19212902437,-92.3999114754588));
#177827=CARTESIAN_POINT('Ctrl Pts',(39.0883490971152,47.1480653445753,-92.408127809539));
#177828=CARTESIAN_POINT('Ctrl Pts',(39.1098053189841,47.1234786494394,-92.4125184625557));
#177829=CARTESIAN_POINT('Ctrl Pts',(39.1659681949264,47.0528208887496,-92.4245521432492));
#177830=CARTESIAN_POINT('Ctrl Pts',(39.1988865967866,47.0026358634964,-92.4323449540457));
#177831=CARTESIAN_POINT('Ctrl Pts',(39.2558436333345,46.8961061100704,-92.446579186395));
#177832=CARTESIAN_POINT('Ctrl Pts',(39.280342254491,46.8383758180937,-92.4531476926319));
#177833=CARTESIAN_POINT('Ctrl Pts',(39.3380013103976,46.6642587706065,-92.4690917299284));
#177834=CARTESIAN_POINT('Ctrl Pts',(39.3570864259713,46.5441464965183,-92.4749886329755));
#177835=CARTESIAN_POINT('Ctrl Pts',(39.3571428571429,46.41999998,-92.4750054575003));
#177836=CARTESIAN_POINT('Origin',(-39.,46.91999998,-129.34995));
#177837=CARTESIAN_POINT('',(38.,46.91999998,-91.84995));
#177838=CARTESIAN_POINT('',(-39.,46.91999998,-91.84995));
#177839=CARTESIAN_POINT('',(38.,46.91999998,-58.24995));
#177840=CARTESIAN_POINT('Origin',(38.,46.41999998,-92.34995));
#177841=CARTESIAN_POINT('',(37.5,46.41999998,-91.84995));
#177842=CARTESIAN_POINT('Origin',(38.,46.41999998,-91.84995));
#177843=CARTESIAN_POINT('',(37.5,46.41999998,-92.34995));
#177844=CARTESIAN_POINT('Origin',(24.7,-70.08000002,-58.24995));
#177845=CARTESIAN_POINT('',(25.2,-70.08000002,-55.74995));
#177846=CARTESIAN_POINT('Origin',(25.2,-70.08000002,-58.24995));
#177847=CARTESIAN_POINT('',(24.7,-70.08000002,-55.24995));
#177848=CARTESIAN_POINT('Origin',(24.7,-70.08000002,-55.74995));
#177849=CARTESIAN_POINT('Origin',(24.7,-70.08000002,-58.24995));
#177850=CARTESIAN_POINT('Origin',(-3.3975957231091E-14,-70.08000002,-58.24995));
#177851=CARTESIAN_POINT('',(41.5,-70.08000002,-55.24995));
#177852=CARTESIAN_POINT('Origin',(-1.8445455022812E-14,-55.08000002,-61.14995));
#177853=CARTESIAN_POINT('',(50.4435446592566,-54.58000002,-61.14995));
#177854=CARTESIAN_POINT('',(60.,-54.58000002,-61.14995));
#177855=CARTESIAN_POINT('',(50.4435446592566,-55.08000002,-60.64995));
#177856=CARTESIAN_POINT('Origin',(50.4435446592566,-55.08000002,-61.14995));
#177857=CARTESIAN_POINT('',(-1.8445455022812E-14,-55.08000002,-60.64995));
#177858=CARTESIAN_POINT('Origin',(44.5079524583206,-57.4754524783489,-52.64995));
#177859=CARTESIAN_POINT('',(44.5079524583206,-60.2254524783489,-55.24995));
#177860=CARTESIAN_POINT('Origin',(44.5079524583206,-57.4754524783489,-55.24995));
#177861=CARTESIAN_POINT('',(44.5079524583206,-60.2254524783489,-60.64995));
#177862=CARTESIAN_POINT('',(44.5079524583206,-60.2254524783489,-52.64995));
#177863=CARTESIAN_POINT('Origin',(44.5079524583206,-57.4754524783489,-60.64995));
#177864=CARTESIAN_POINT('Origin',(44.5079524583206,-57.4754524783489,-60.64995));
#177865=CARTESIAN_POINT('Origin',(0.,45.41999998,-55.24995));
#177866=CARTESIAN_POINT('',(44.5079524583206,-59.475452478349,-55.24995));
#177867=CARTESIAN_POINT('Origin',(44.5079524583206,-57.4754524783489,-55.24995));
#177868=CARTESIAN_POINT('Origin',(44.5079524583206,-57.475452478349,235.35105));
#177869=CARTESIAN_POINT('',(44.5079524583206,-59.475452478349,-52.64995));
#177870=CARTESIAN_POINT('Origin',(44.5079524583206,-57.4754524783489,-52.64995));
#177871=CARTESIAN_POINT('',(44.5079524583206,-59.475452478349,235.35105));
#177872=CARTESIAN_POINT('Origin',(42.,-12.9675000200281,-61.14995));
#177873=CARTESIAN_POINT('',(42.,-63.4208871539288,-60.64995));
#177874=CARTESIAN_POINT('',(41.5,-63.4208871539288,-61.14995));
#177875=CARTESIAN_POINT('Origin',(42.,-63.4208871539288,-61.14995));
#177876=CARTESIAN_POINT('',(41.5,-73.08000002,-61.14995));
#177877=CARTESIAN_POINT('',(42.,-12.9675000200281,-60.64995));
#177878=CARTESIAN_POINT('Origin',(39.5,46.91999998,-61.14995));
#177879=CARTESIAN_POINT('',(39.5,31.080768958446,-60.64995));
#177880=CARTESIAN_POINT('Origin',(39.5,31.080768958446,-61.14995));
#177881=CARTESIAN_POINT('',(39.,37.7046087726872,-61.14995));
#177882=CARTESIAN_POINT('',(39.,31.080768958446,-61.14995));
#177883=CARTESIAN_POINT('',(39.5,37.7046087726872,-60.64995));
#177884=CARTESIAN_POINT('Origin',(39.5,37.7046087726872,-61.14995));
#177885=CARTESIAN_POINT('',(39.5,37.7483531044501,-60.64995));
#177886=CARTESIAN_POINT('Ctrl Pts',(39.6638655462185,30.7106154376184,-60.64995));
#177887=CARTESIAN_POINT('Ctrl Pts',(39.5,30.859420873127,-60.64995));
#177888=CARTESIAN_POINT('Ctrl Pts',(39.5,31.080768958446,-60.64995));
#177889=CARTESIAN_POINT('Ctrl Pts',(39.327731092437,30.3404619167909,-60.64995));
#177890=CARTESIAN_POINT('Ctrl Pts',(39.,30.638072787808,-60.64995));
#177891=CARTESIAN_POINT('Ctrl Pts',(39.,31.080768958446,-60.64995));
#177892=CARTESIAN_POINT('Ctrl Pts',(39.327731092437,30.3404619167909,-61.14995));
#177893=CARTESIAN_POINT('Ctrl Pts',(39.,30.638072787808,-61.14995));
#177894=CARTESIAN_POINT('Ctrl Pts',(39.,31.080768958446,-61.14995));
#177895=CARTESIAN_POINT('',(39.6638655462185,30.7106154376184,-60.64995));
#177896=CARTESIAN_POINT('Origin',(39.6638655462185,30.7106154376184,-61.14995));
#177897=CARTESIAN_POINT('Origin',(40.,31.080768958446,-60.64995));
#177898=CARTESIAN_POINT('Origin',(0.,-12.9675000200281,-61.14995));
#177899=CARTESIAN_POINT('',(41.4049466656476,29.0638025010082,-60.64995));
#177900=CARTESIAN_POINT('Origin',(41.4049466656476,29.0638025010082,-61.14995));
#177901=CARTESIAN_POINT('Origin',(0.,-12.9675000200281,-60.64995));
#177902=CARTESIAN_POINT('Ctrl Pts',(41.7558360441701,28.91999998,-60.64995));
#177903=CARTESIAN_POINT('Ctrl Pts',(41.5509245680609,28.91999998,-60.64995));
#177904=CARTESIAN_POINT('Ctrl Pts',(41.4049466656477,29.0638025010082,-60.64995));
#177905=CARTESIAN_POINT('Ctrl Pts',(41.7558360441701,28.41999998,-60.64995));
#177906=CARTESIAN_POINT('Ctrl Pts',(41.3460130919516,28.41999998,-60.64995));
#177907=CARTESIAN_POINT('Ctrl Pts',(41.0540572871252,28.7076050220163,-60.64995));
#177908=CARTESIAN_POINT('Ctrl Pts',(41.7558360441701,28.41999998,-61.14995));
#177909=CARTESIAN_POINT('Ctrl Pts',(41.3460130919516,28.41999998,-61.14995));
#177910=CARTESIAN_POINT('Ctrl Pts',(41.0540572871252,28.7076050220163,-61.14995));
#177911=CARTESIAN_POINT('',(41.7558360441701,28.91999998,-60.64995));
#177912=CARTESIAN_POINT('Origin',(41.7558360441701,28.91999998,-61.14995));
#177913=CARTESIAN_POINT('Origin',(41.7558360441701,29.41999998,-60.64995));
#177914=CARTESIAN_POINT('Origin',(1.8346904061005E-14,28.9199999800001,
-61.14995));
#177915=CARTESIAN_POINT('',(60.,28.41999998,-61.14995));
#177916=CARTESIAN_POINT('',(1.8346904061005E-14,28.9199999800001,-60.64995));
#177917=CARTESIAN_POINT('Origin',(44.5079524583208,31.5404524382925,-52.64995));
#177918=CARTESIAN_POINT('',(44.5079524583208,28.7904524382925,-55.24995));
#177919=CARTESIAN_POINT('Origin',(44.5079524583208,31.5404524382925,-55.24995));
#177920=CARTESIAN_POINT('',(44.5079524583208,28.7904524382925,-52.64995));
#177921=CARTESIAN_POINT('Origin',(44.5079524583208,31.5404524382925,-60.64995));
#177922=CARTESIAN_POINT('Origin',(0.,45.41999998,-55.24995));
#177923=CARTESIAN_POINT('',(44.5079524583208,29.5404524382925,-55.24995));
#177924=CARTESIAN_POINT('Origin',(44.5079524583208,31.5404524382925,-55.24995));
#177925=CARTESIAN_POINT('Origin',(44.5079524583208,31.5404524382925,235.35105));
#177926=CARTESIAN_POINT('',(44.5079524583208,29.5404524382925,-52.64995));
#177927=CARTESIAN_POINT('Origin',(44.5079524583208,31.5404524382925,-52.64995));
#177928=CARTESIAN_POINT('',(44.5079524583208,29.5404524382925,235.35105));
#177929=CARTESIAN_POINT('Origin',(1.8346904061005E-14,28.9199999800001,
-61.14995));
#177930=CARTESIAN_POINT('',(50.4632296085449,28.91999998,-60.64995));
#177931=CARTESIAN_POINT('',(1.8346904061005E-14,28.9199999800001,-60.64995));
#177932=CARTESIAN_POINT('',(50.4632296085449,28.41999998,-61.14995));
#177933=CARTESIAN_POINT('Origin',(50.4632296085449,28.91999998,-61.14995));
#177934=CARTESIAN_POINT('',(60.,28.41999998,-61.14995));
#177935=CARTESIAN_POINT('Origin',(0.,-12.9675000200281,-60.64995));
#177936=CARTESIAN_POINT('',(51.6244217512083,-41.5825130958571,-60.64995));
#177937=CARTESIAN_POINT('',(53.7167487055513,-17.6671065732338,-60.64995));
#177938=CARTESIAN_POINT('Origin',(0.,-12.9675000200281,-60.64995));
#177939=CARTESIAN_POINT('Origin',(-83.2809572255632,-44.93000002,-55.2499500000007));
#177940=CARTESIAN_POINT('',(52.8810286821225,-44.93000002,-59.64995));
#177941=CARTESIAN_POINT('Ctrl Pts',(51.3752989258075,-44.93000002,-61.14995));
#177942=CARTESIAN_POINT('Ctrl Pts',(51.5724340164545,-44.93000002,-61.149949999985));
#177943=CARTESIAN_POINT('Ctrl Pts',(51.7694205173407,-44.93000002,-61.1109090094727));
#177944=CARTESIAN_POINT('Ctrl Pts',(52.1336129969961,-44.93000002,-60.9606295880612));
#177945=CARTESIAN_POINT('Ctrl Pts',(52.3006402190038,-44.93000002,-60.8494502533521));
#177946=CARTESIAN_POINT('Ctrl Pts',(52.5793810752606,-44.93000002,-60.5717700902076));
#177947=CARTESIAN_POINT('Ctrl Pts',(52.6909850969965,-44.93000002,-60.4053784571342));
#177948=CARTESIAN_POINT('Ctrl Pts',(52.8418385613238,-44.93000002,-60.0425718399611));
#177949=CARTESIAN_POINT('Ctrl Pts',(52.8810286821055,-44.93000002,-59.8463349320562));
#177950=CARTESIAN_POINT('Ctrl Pts',(52.8810286821225,-44.93000002,-59.64995));
#177951=CARTESIAN_POINT('',(52.8810286821225,-44.93000002,-55.74995));
#177952=CARTESIAN_POINT('',(52.8810286821225,-44.93000002,-55.2499500000007));
#177953=CARTESIAN_POINT('',(-83.2809572255632,-44.93000002,-55.74995));
#177954=CARTESIAN_POINT('Ctrl Pts',(51.375172246442,-44.93000002,-61.1499499946262));
#177955=CARTESIAN_POINT('Ctrl Pts',(51.3752141318477,-44.93000002,-60.6498941830801));
#177956=CARTESIAN_POINT('Ctrl Pts',(51.3752141521426,-44.4299442087041,
-60.6499499995188));
#177957=CARTESIAN_POINT('Ctrl Pts',(51.5723496265306,-44.93000002,-61.1499667235334));
#177958=CARTESIAN_POINT('Ctrl Pts',(51.5079545643181,-44.9300000200007,
-60.6441634129642));
#177959=CARTESIAN_POINT('Ctrl Pts',(51.5071649062657,-44.424237291042,-60.6499618311935));
#177960=CARTESIAN_POINT('Ctrl Pts',(51.7693815122227,-44.93000002,-61.1109251044414));
#177961=CARTESIAN_POINT('Ctrl Pts',(51.637293275499,-44.9300000200007,-60.6119868070537));
#177962=CARTESIAN_POINT('Ctrl Pts',(51.6390186853523,-44.4185345954033,
-60.6239348042612));
#177963=CARTESIAN_POINT('Ctrl Pts',(52.1336129969961,-44.93000002,-60.9606295880612));
#177964=CARTESIAN_POINT('Ctrl Pts',(51.8725693108456,-44.9300000199993,
-60.5030970594193));
#177965=CARTESIAN_POINT('Ctrl Pts',(51.8827629060799,-44.4079926660298,
-60.5237387895065));
#177966=CARTESIAN_POINT('Ctrl Pts',(52.3006402190038,-44.93000002,-60.8494502533521));
#177967=CARTESIAN_POINT('Ctrl Pts',(51.977992200991,-44.93000002,-60.4261477374103));
#177968=CARTESIAN_POINT('Ctrl Pts',(51.9945380358051,-44.4031584192941,
-60.4496195485704));
#177969=CARTESIAN_POINT('Ctrl Pts',(52.5793810752606,-44.93000002,-60.5717700902076));
#177970=CARTESIAN_POINT('Ctrl Pts',(52.1520057930301,-44.93000002,-60.2406358789575));
#177971=CARTESIAN_POINT('Ctrl Pts',(52.1810724759249,-44.3950908753576,
-60.2644994621534));
#177972=CARTESIAN_POINT('Ctrl Pts',(52.6909850969965,-44.93000002,-60.4053784571342));
#177973=CARTESIAN_POINT('Ctrl Pts',(52.2200668721359,-44.9300000199999,
-60.1321953438309));
#177974=CARTESIAN_POINT('Ctrl Pts',(52.2557584885118,-44.3918607474242,
-60.153571413262));
#177975=CARTESIAN_POINT('Ctrl Pts',(52.8418547177727,-44.93000002,-60.0425329832694));
#177976=CARTESIAN_POINT('Ctrl Pts',(52.3118976785816,-44.93000002,-59.8989282761455));
#177977=CARTESIAN_POINT('Ctrl Pts',(52.3567212630826,-44.387494169614,-59.9116734379891));
#177978=CARTESIAN_POINT('Ctrl Pts',(52.8810454695352,-44.93000002,-59.8462508632613));
#177979=CARTESIAN_POINT('Ctrl Pts',(52.3353165341951,-44.9300000200007,
-59.7745406636052));
#177980=CARTESIAN_POINT('Ctrl Pts',(52.3829479761289,-44.3863598840851,
-59.7808179550118));
#177981=CARTESIAN_POINT('Ctrl Pts',(52.8810286767281,-44.93000002,-59.6498238026878));
#177982=CARTESIAN_POINT('Ctrl Pts',(52.3353064873126,-44.93000002,-59.6498699040777));
#177983=CARTESIAN_POINT('Ctrl Pts',(52.3829367382961,-44.3863603697065,
-59.6498658680002));
#177984=CARTESIAN_POINT('',(52.3829313330767,-44.3864221486262,-59.64995));
#177985=CARTESIAN_POINT('Ctrl Pts',(52.3829313330767,-44.3864221486262,
-59.64995));
#177986=CARTESIAN_POINT('Ctrl Pts',(52.3829313330767,-44.3864221486262,
-59.6909167350341));
#177987=CARTESIAN_POINT('Ctrl Pts',(52.3803897263674,-44.3865523180115,
-59.7322798285798));
#177988=CARTESIAN_POINT('Ctrl Pts',(52.3751806262637,-44.3868016431244,
-59.7737125482639));
#177989=CARTESIAN_POINT('Ctrl Pts',(52.3700397112217,-44.3870477046701,
-59.8146029300225));
#177990=CARTESIAN_POINT('Ctrl Pts',(52.3623003085474,-44.38740979058,-59.8555607844284));
#177991=CARTESIAN_POINT('Ctrl Pts',(52.3518818373882,-44.3878808509431,
-59.8962415307623));
#177992=CARTESIAN_POINT('Ctrl Pts',(52.3416571248465,-44.3883431507112,
-59.9361657126203));
#177993=CARTESIAN_POINT('Ctrl Pts',(52.3288517987115,-44.3889103859351,
-59.975822586086));
#177994=CARTESIAN_POINT('Ctrl Pts',(52.3134335070198,-44.3895797261845,
-60.0148624568469));
#177995=CARTESIAN_POINT('Ctrl Pts',(52.2981820855851,-44.3902418222476,
-60.0534798039331));
#177996=CARTESIAN_POINT('Ctrl Pts',(52.2803736880321,-44.3910038020508,
-60.0914930062));
#177997=CARTESIAN_POINT('Ctrl Pts',(52.2600242856205,-44.3918670628984,
-60.1285460469148));
#177998=CARTESIAN_POINT('Ctrl Pts',(52.2399875641714,-44.3927170592173,
-60.1650297450909));
#177999=CARTESIAN_POINT('Ctrl Pts',(52.2174871679696,-44.3936652341685,
-60.2005820954543));
#178000=CARTESIAN_POINT('Ctrl Pts',(52.192587492136,-44.3947172215951,-60.2348527378331));
#178001=CARTESIAN_POINT('Ctrl Pts',(52.1812851570981,-44.3951947344121,
-60.2504086946543));
#178002=CARTESIAN_POINT('Ctrl Pts',(52.1694891682159,-44.3956936970622,
-60.2657004677395));
#178003=CARTESIAN_POINT('Ctrl Pts',(52.1572090867896,-44.3962149460507,
-60.2806949718618));
#178004=CARTESIAN_POINT('Ctrl Pts',(52.146382848985,-44.3966744841684,-60.2939142708023));
#178005=CARTESIAN_POINT('Ctrl Pts',(52.1351803878862,-44.3971513466985,
-60.3069025151132));
#178006=CARTESIAN_POINT('Ctrl Pts',(52.1236097339139,-44.3976462362116,
-60.319637030479));
#178007=CARTESIAN_POINT('Ctrl Pts',(52.1184044198055,-44.3978688731837,
-60.3253659333271));
#178008=CARTESIAN_POINT('Ctrl Pts',(52.1128462456499,-44.3981087671614,
-60.3313432771974));
#178009=CARTESIAN_POINT('Ctrl Pts',(52.1073053941287,-44.3983470728172,
-60.3371563979184));
#178010=CARTESIAN_POINT('Ctrl Pts',(52.1015839317946,-44.3985931463364,
-60.3431590043988));
#178011=CARTESIAN_POINT('Ctrl Pts',(52.0958811206976,-44.3988375421255,
-60.3489863692236));
#178012=CARTESIAN_POINT('Ctrl Pts',(52.090645706994,-44.3990631132714,-60.3542239167039));
#178013=CARTESIAN_POINT('Ctrl Pts',(52.0896810715817,-44.3991046752047,
-60.3551889452689));
#178014=CARTESIAN_POINT('Ctrl Pts',(52.0887324034389,-44.3991456067858,
-60.3561340538162));
#178015=CARTESIAN_POINT('Ctrl Pts',(52.0878026339309,-44.3991858116419,
-60.3570567811866));
#178016=CARTESIAN_POINT('Ctrl Pts',(52.0656716302681,-44.400142794861,-60.3790201631155));
#178017=CARTESIAN_POINT('Ctrl Pts',(52.0418506706569,-44.4011805791872,
-60.4006133594539));
#178018=CARTESIAN_POINT('Ctrl Pts',(52.0162710562994,-44.4022931542543,
-60.4215416038383));
#178019=CARTESIAN_POINT('Ctrl Pts',(51.9913941546727,-44.4033751651131,
-60.4418949160304));
#178020=CARTESIAN_POINT('Ctrl Pts',(51.9648534607165,-44.4045278757317,
-60.4616189818122));
#178021=CARTESIAN_POINT('Ctrl Pts',(51.9366235653637,-44.4057490631047,
-60.4804121740066));
#178022=CARTESIAN_POINT('Ctrl Pts',(51.9083936700108,-44.4069702504778,
-60.499205366201));
#178023=CARTESIAN_POINT('Ctrl Pts',(51.8784739585051,-44.4082598608211,
-60.5170673748192));
#178024=CARTESIAN_POINT('Ctrl Pts',(51.8468854021593,-44.4096197288869,
-60.5336701569294));
#178025=CARTESIAN_POINT('Ctrl Pts',(51.8309424071766,-44.4103060650876,
-60.5420497127719));
#178026=CARTESIAN_POINT('Ctrl Pts',(51.8145750983105,-44.4110103672594,
-60.5501081144062));
#178027=CARTESIAN_POINT('Ctrl Pts',(51.7977914535884,-44.4117333333892,
-60.5578010744768));
#178028=CARTESIAN_POINT('Ctrl Pts',(51.7893996312274,-44.4120948164541,
-60.561647554512));
#178029=CARTESIAN_POINT('Ctrl Pts',(51.78090372741,-44.4124609657279,-60.5654026797756));
#178030=CARTESIAN_POINT('Ctrl Pts',(51.7723051681535,-44.4128319059709,
-60.5690607764376));
#178031=CARTESIAN_POINT('Ctrl Pts',(51.7680058885252,-44.4130173760924,
-60.5708898247687));
#178032=CARTESIAN_POINT('Ctrl Pts',(51.7636809453568,-44.4132040439841,
-60.572694616651));
#178033=CARTESIAN_POINT('Ctrl Pts',(51.7593305321249,-44.4133919265732,
-60.5744744411433));
#178034=CARTESIAN_POINT('Ctrl Pts',(51.7566892401513,-44.4135059968346,
-60.5755550364558));
#178035=CARTESIAN_POINT('Ctrl Pts',(51.7533267700704,-44.4136516104333,
-60.5769130552734));
#178036=CARTESIAN_POINT('Ctrl Pts',(51.7505384799174,-44.4137720333314,
-60.5780234113453));
#178037=CARTESIAN_POINT('Ctrl Pts',(51.7487342394082,-44.413849956309,-60.5787418980503));
#178038=CARTESIAN_POINT('Ctrl Pts',(51.747170962424,-44.4139173797181,-60.5793580291754));
#178039=CARTESIAN_POINT('Ctrl Pts',(51.7462030841064,-44.4139592360934,
-60.5797383010624));
#178040=CARTESIAN_POINT('Ctrl Pts',(51.730823640736,-44.4146243277082,-60.5857807651258));
#178041=CARTESIAN_POINT('Ctrl Pts',(51.7138127700712,-44.4153695794285,
-60.59203299983));
#178042=CARTESIAN_POINT('Ctrl Pts',(51.6951076439614,-44.4161894945035,
-60.5982457370374));
#178043=CARTESIAN_POINT('Ctrl Pts',(51.6768144165372,-44.4169913545309,
-60.6043216658492));
#178044=CARTESIAN_POINT('Ctrl Pts',(51.6568999668665,-44.4178645591487,
-60.6103597074779));
#178045=CARTESIAN_POINT('Ctrl Pts',(51.6353215996103,-44.4188053729988,
-60.6160795516463));
#178046=CARTESIAN_POINT('Ctrl Pts',(51.6145837107182,-44.4197095421076,
-60.62157660763));
#178047=CARTESIAN_POINT('Ctrl Pts',(51.5923083534765,-44.4206760997577,
-60.6267794477222));
#178048=CARTESIAN_POINT('Ctrl Pts',(51.5684827119301,-44.4217039246985,
-60.6313985671859));
#178049=CARTESIAN_POINT('Ctrl Pts',(51.5452580328485,-44.4227058244523,
-60.6359011769886));
#178050=CARTESIAN_POINT('Ctrl Pts',(51.5205596402882,-44.4237658829128,
-60.6398488190514));
#178051=CARTESIAN_POINT('Ctrl Pts',(51.4944094354873,-44.4248860161899,
-60.6429384344745));
#178052=CARTESIAN_POINT('Ctrl Pts',(51.4692420222068,-44.4259640519961,
-60.6459119342548));
#178053=CARTESIAN_POINT('Ctrl Pts',(51.4427294002456,-44.4270976906941,
-60.6480902258672));
#178054=CARTESIAN_POINT('Ctrl Pts',(51.4149307233305,-44.4282921075643,
-60.6491761922995));
#178055=CARTESIAN_POINT('Ctrl Pts',(51.4019948308487,-44.4288479199239,
-60.6496815381132));
#178056=CARTESIAN_POINT('Ctrl Pts',(51.3887810672911,-44.4294169472215,
-60.64995));
#178057=CARTESIAN_POINT('Ctrl Pts',(51.3752989258075,-44.43000002,-60.64995));
#178058=CARTESIAN_POINT('',(52.3810286821225,-44.43000002,-59.64995));
#178059=CARTESIAN_POINT('Origin',(52.8810286821225,-44.43000002,-59.64995));
#178060=CARTESIAN_POINT('Origin',(52.8810286821225,-44.43000002,-59.64995));
#178061=CARTESIAN_POINT('Origin',(-83.2809572255632,-45.4300000199999,-55.74995));
#178062=CARTESIAN_POINT('',(52.7935400185966,-45.43000002,-55.24995));
#178063=CARTESIAN_POINT('Ctrl Pts',(52.8810286821225,-44.93000002,-55.74995));
#178064=CARTESIAN_POINT('Ctrl Pts',(52.8810286821214,-44.93000002,-55.7240274876136));
#178065=CARTESIAN_POINT('Ctrl Pts',(52.8806555354494,-44.9321038000435,
-55.6978059976788));
#178066=CARTESIAN_POINT('Ctrl Pts',(52.8799059022337,-44.9363531599825,
-55.6716073783532));
#178067=CARTESIAN_POINT('Ctrl Pts',(52.8791497351538,-44.9406395576885,
-55.6451804097294));
#178068=CARTESIAN_POINT('Ctrl Pts',(52.8780104850152,-44.9471091347783,
-55.6187767695886));
#178069=CARTESIAN_POINT('Ctrl Pts',(52.8764897360373,-44.9557761309555,
-55.5927712416137));
#178070=CARTESIAN_POINT('Ctrl Pts',(52.8759205170078,-44.9590202029387,
-55.5830373265427));
#178071=CARTESIAN_POINT('Ctrl Pts',(52.8752978996289,-44.9625718489931,
-55.5733596261139));
#178072=CARTESIAN_POINT('Ctrl Pts',(52.8746221467745,-44.9664307842404,
-55.5637593428073));
#178073=CARTESIAN_POINT('Ctrl Pts',(52.8728440766865,-44.9765845812825,
-55.5384986628543));
#178074=CARTESIAN_POINT('Ctrl Pts',(52.8706960694052,-44.9888727751743,
-55.5137551369759));
#178075=CARTESIAN_POINT('Ctrl Pts',(52.8681778191489,-45.0032950405858,
-55.489926848577));
#178076=CARTESIAN_POINT('Ctrl Pts',(52.867671674228,-45.0061937820303,-55.485137583842));
#178077=CARTESIAN_POINT('Ctrl Pts',(52.8671505801727,-45.0091786900675,
-55.4803854542241));
#178078=CARTESIAN_POINT('Ctrl Pts',(52.8666145463196,-45.0122496941479,
-55.4756739401742));
#178079=CARTESIAN_POINT('Ctrl Pts',(52.8650130502525,-45.0214248627082,
-55.4615974575482));
#178080=CARTESIAN_POINT('Ctrl Pts',(52.8632780871792,-45.0313686933034,
-55.4478834520303));
#178081=CARTESIAN_POINT('Ctrl Pts',(52.8614096369564,-45.0420727511099,
-55.4346345056539));
#178082=CARTESIAN_POINT('Ctrl Pts',(52.8604754118449,-45.0474247800131,
-55.4280100324658));
#178083=CARTESIAN_POINT('Ctrl Pts',(52.8595078154648,-45.052966812139,-55.4215019155655));
#178084=CARTESIAN_POINT('Ctrl Pts',(52.8585068493069,-45.0586966555504,
-55.4151241748974));
#178085=CARTESIAN_POINT('Ctrl Pts',(52.858006366228,-45.0615615772561,-55.4119353045634));
#178086=CARTESIAN_POINT('Ctrl Pts',(52.8574975407611,-45.0644734423857,
-55.4087790343541));
#178087=CARTESIAN_POINT('Ctrl Pts',(52.8569803733541,-45.0674318984956,
-55.4056571673493));
#178088=CARTESIAN_POINT('Ctrl Pts',(52.8566794288446,-45.069153451538,-55.4038405239921));
#178089=CARTESIAN_POINT('Ctrl Pts',(52.8563126508256,-45.071250909713,-55.4016627141456));
#178090=CARTESIAN_POINT('Ctrl Pts',(52.8559894746429,-45.0730986811608,
-55.399777933153));
#178091=CARTESIAN_POINT('Ctrl Pts',(52.8557572787116,-45.0744262697484,
-55.3984237539124));
#178092=CARTESIAN_POINT('Ctrl Pts',(52.855547825501,-45.0756236244489,-55.3972196143699));
#178093=CARTESIAN_POINT('Ctrl Pts',(52.8554038192003,-45.0764466282408,
-55.3963966105726));
#178094=CARTESIAN_POINT('Ctrl Pts',(52.8536925773759,-45.0862264677528,
-55.3866167709961));
#178095=CARTESIAN_POINT('Ctrl Pts',(52.851754330019,-45.0971430353417,-55.3765446164713));
#178096=CARTESIAN_POINT('Ctrl Pts',(52.8495832355115,-45.109325146193,-55.3664154208622));
#178097=CARTESIAN_POINT('Ctrl Pts',(52.8475054116275,-45.1209839112987,
-55.3567213773785));
#178098=CARTESIAN_POINT('Ctrl Pts',(52.8452141961207,-45.1338025296426,
-55.3469750519385));
#178099=CARTESIAN_POINT('Ctrl Pts',(52.8427082950591,-45.1478716582866,
-55.3374234994891));
#178100=CARTESIAN_POINT('Ctrl Pts',(52.8403472166539,-45.1611276947396,
-55.3284239565424));
#178101=CARTESIAN_POINT('Ctrl Pts',(52.8377954759301,-45.1754943248228,
-55.3195974072008));
#178102=CARTESIAN_POINT('Ctrl Pts',(52.8350568009413,-45.1910192354886,
-55.3111870421648));
#178103=CARTESIAN_POINT('Ctrl Pts',(52.8339582620473,-45.1972465966259,
-55.3078134716817));
#178104=CARTESIAN_POINT('Ctrl Pts',(52.8328297081496,-45.2036599569019,
-55.3045072862908));
#178105=CARTESIAN_POINT('Ctrl Pts',(52.8316716567513,-45.2102607648964,
-55.3012859403148));
#178106=CARTESIAN_POINT('Ctrl Pts',(52.828999083875,-45.2254942341827,-55.2938516572656));
#178107=CARTESIAN_POINT('Ctrl Pts',(52.826174751091,-45.2417391406544,-55.2868619638522));
#178108=CARTESIAN_POINT('Ctrl Pts',(52.8231873524218,-45.2589873547265,
-55.2805581078704));
#178109=CARTESIAN_POINT('Ctrl Pts',(52.8202817251599,-45.275763448773,-55.2744268017326));
#178110=CARTESIAN_POINT('Ctrl Pts',(52.8172217775644,-45.2934889899389,
-55.2689442786239));
#178111=CARTESIAN_POINT('Ctrl Pts',(52.8140036335369,-45.3121198505846,
-55.264362018836));
#178112=CARTESIAN_POINT('Ctrl Pts',(52.8108844970282,-45.3301775251725,
-55.259920734147));
#178113=CARTESIAN_POINT('Ctrl Pts',(52.8076167059087,-45.3490858911464,
-55.256325174742));
#178114=CARTESIAN_POINT('Ctrl Pts',(52.8042036732994,-45.3687660560856,
-55.2538325278146));
#178115=CARTESIAN_POINT('Ctrl Pts',(52.8007906406901,-45.3884462210248,
-55.2513398808872));
#178116=CARTESIAN_POINT('Ctrl Pts',(52.7972322905145,-45.4088985894293,
-55.24995));
#178117=CARTESIAN_POINT('Ctrl Pts',(52.7935400185966,-45.43000002,-55.24995));
#178118=CARTESIAN_POINT('',(60.,-45.43000002,-55.24995));
#178119=CARTESIAN_POINT('Origin',(60.,28.41999998,-55.24995));
#178120=CARTESIAN_POINT('',(52.7497956868337,-45.93000002,-55.24995));
#178121=CARTESIAN_POINT('',(59.2602401389193,28.4847205815761,-55.24995));
#178122=CARTESIAN_POINT('',(60.,-45.93000002,-55.24995));
#178123=CARTESIAN_POINT('Origin',(60.,-45.93000002,-55.74995));
#178124=CARTESIAN_POINT('',(52.6623070233078,-46.43000002,-55.74995));
#178125=CARTESIAN_POINT('Ctrl Pts',(52.7497956868337,-45.93000002,-55.24995));
#178126=CARTESIAN_POINT('Ctrl Pts',(52.7460187925163,-45.9515850697951,
-55.24995));
#178127=CARTESIAN_POINT('Ctrl Pts',(52.7423610411603,-45.9724892144497,
-55.2514041468224));
#178128=CARTESIAN_POINT('Ctrl Pts',(52.7388452120446,-45.9925822697903,
-55.2540052053732));
#178129=CARTESIAN_POINT('Ctrl Pts',(52.7353551265784,-46.0125281995008,
-55.2565872184194));
#178130=CARTESIAN_POINT('Ctrl Pts',(52.7320048008033,-46.0316753989214,
-55.260299617229));
#178131=CARTESIAN_POINT('Ctrl Pts',(52.7288082793926,-46.0499436023777,
-55.2648742466987));
#178132=CARTESIAN_POINT('Ctrl Pts',(52.7254663302596,-46.0690429290696,
-55.2696570017705));
#178133=CARTESIAN_POINT('Ctrl Pts',(52.7222924665376,-46.0871816432422,
-55.2753821626626));
#178134=CARTESIAN_POINT('Ctrl Pts',(52.7192945613869,-46.1043147495782,
-55.2817780783569));
#178135=CARTESIAN_POINT('Ctrl Pts',(52.716494116128,-46.1203193674686,-55.2877527209429));
#178136=CARTESIAN_POINT('Ctrl Pts',(52.7138470746185,-46.1354472789192,
-55.2943131224857));
#178137=CARTESIAN_POINT('Ctrl Pts',(52.7113543626339,-46.1496931930989,
-55.3012636512206));
#178138=CARTESIAN_POINT('Ctrl Pts',(52.7084584871895,-46.166243196994,-55.3093383367891));
#178139=CARTESIAN_POINT('Ctrl Pts',(52.7057691575151,-46.1816127864123,
-55.3179437621966));
#178140=CARTESIAN_POINT('Ctrl Pts',(52.7032802093755,-46.1958371901192,
-55.3268178701236));
#178141=CARTESIAN_POINT('Ctrl Pts',(52.7006035647027,-46.2111342844216,
-55.3363611921922));
#178142=CARTESIAN_POINT('Ctrl Pts',(52.6981585023978,-46.2251078794353,
-55.3462154234316));
#178143=CARTESIAN_POINT('Ctrl Pts',(52.695930445538,-46.237841282656,-55.3561026478091));
#178144=CARTESIAN_POINT('Ctrl Pts',(52.6936636080107,-46.2507963184048,
-55.3661619652632));
#178145=CARTESIAN_POINT('Ctrl Pts',(52.6916213571538,-46.2624678354595,
-55.3762552362856));
#178146=CARTESIAN_POINT('Ctrl Pts',(52.6897832999643,-46.272972380365,-55.3861352293988));
#178147=CARTESIAN_POINT('Ctrl Pts',(52.6895145215425,-46.2745084560746,
-55.3875799771312));
#178148=CARTESIAN_POINT('Ctrl Pts',(52.6892501028258,-46.2760196159558,
-55.3890202396049));
#178149=CARTESIAN_POINT('Ctrl Pts',(52.6889899717987,-46.2775062715784,
-55.3904553319095));
#178150=CARTESIAN_POINT('Ctrl Pts',(52.6887686497785,-46.2787711327118,
-55.3916763224679));
#178151=CARTESIAN_POINT('Ctrl Pts',(52.6886223994534,-46.2796069571358,
-55.3924916493942));
#178152=CARTESIAN_POINT('Ctrl Pts',(52.6884184363187,-46.2807725552524,
-55.3936383710037));
#178153=CARTESIAN_POINT('Ctrl Pts',(52.6882898108671,-46.2815076174213,
-55.3943615290642));
#178154=CARTESIAN_POINT('Ctrl Pts',(52.6881382781733,-46.2823735725975,
-55.3952167714233));
#178155=CARTESIAN_POINT('Ctrl Pts',(52.687931817023,-46.2835534087318,-55.3963966075452));
#178156=CARTESIAN_POINT('Ctrl Pts',(52.6843315421343,-46.3041274218082,
-55.416970620405));
#178157=CARTESIAN_POINT('Ctrl Pts',(52.6811035150388,-46.3225747482756,
-55.439163047915));
#178158=CARTESIAN_POINT('Ctrl Pts',(52.6782552198821,-46.338852377289,-55.4624843710585));
#178159=CARTESIAN_POINT('Ctrl Pts',(52.6754034087636,-46.3551500995569,
-55.4858344822573));
#178160=CARTESIAN_POINT('Ctrl Pts',(52.6729322643169,-46.3692727837042,
-55.5103162635779));
#178161=CARTESIAN_POINT('Ctrl Pts',(52.670845226173,-46.3812005423344,-55.5354850657357));
#178162=CARTESIAN_POINT('Ctrl Pts',(52.6687546255404,-46.3931486611603,
-55.5606968300082));
#178163=CARTESIAN_POINT('Ctrl Pts',(52.6670494390977,-46.402894380944,-55.5865979625005));
#178164=CARTESIAN_POINT('Ctrl Pts',(52.6657290991159,-46.4104407221667,
-55.6127884619271));
#178165=CARTESIAN_POINT('Ctrl Pts',(52.6644028119805,-46.4180210540667,
-55.6390969301531));
#178166=CARTESIAN_POINT('Ctrl Pts',(52.6634648417048,-46.4233821745086,
-55.6656973742807));
#178167=CARTESIAN_POINT('Ctrl Pts',(52.6629106187229,-46.4265499748194,
-55.6922317372147));
#178168=CARTESIAN_POINT('Ctrl Pts',(52.6625072019682,-46.4288558043545,
-55.7115459968728));
#178169=CARTESIAN_POINT('Ctrl Pts',(52.6623070233078,-46.43000002,-55.7308262353414));
#178170=CARTESIAN_POINT('Ctrl Pts',(52.6623070233078,-46.43000002,-55.74995));
#178171=CARTESIAN_POINT('',(-83.2809572255632,-46.4300000199999,-55.74995));
#178172=CARTESIAN_POINT('Origin',(-83.2809572255632,-46.4300000199999,-55.2499500000008));
#178173=CARTESIAN_POINT('',(52.6623070233077,-46.43000002,-59.64995));
#178174=CARTESIAN_POINT('',(52.6623070233078,-46.43000002,-55.2499500000008));
#178175=CARTESIAN_POINT('Ctrl Pts',(52.6623070233077,-46.43000002,-59.64995));
#178176=CARTESIAN_POINT('Ctrl Pts',(52.6623070232906,-46.43000002,-59.8463349320562));
#178177=CARTESIAN_POINT('Ctrl Pts',(52.623116902509,-46.43000002,-60.0425718399611));
#178178=CARTESIAN_POINT('Ctrl Pts',(52.5476901703453,-46.43000002,-60.2239751485476));
#178179=CARTESIAN_POINT('Ctrl Pts',(52.4722634381816,-46.43000002,-60.4053784571342));
#178180=CARTESIAN_POINT('Ctrl Pts',(52.3606594164458,-46.43000002,-60.5717700902076));
#178181=CARTESIAN_POINT('Ctrl Pts',(52.2212889883174,-46.43000002,-60.7106101717798));
#178182=CARTESIAN_POINT('Ctrl Pts',(52.0819185601891,-46.43000002,-60.8494502533521));
#178183=CARTESIAN_POINT('Ctrl Pts',(51.9148913381812,-46.43000002,-60.9606295880612));
#178184=CARTESIAN_POINT('Ctrl Pts',(51.7327950983536,-46.43000002,-61.0357692987669));
#178185=CARTESIAN_POINT('Ctrl Pts',(51.550698858526,-46.43000002,-61.1109090094727));
#178186=CARTESIAN_POINT('Ctrl Pts',(51.3537123576397,-46.43000002,-61.149949999985));
#178187=CARTESIAN_POINT('Ctrl Pts',(51.1565772669927,-46.43000002,-61.14995));
#178188=CARTESIAN_POINT('Ctrl Pts',(52.6623070233078,-46.43000002,-59.64995));
#178189=CARTESIAN_POINT('Ctrl Pts',(52.2041414362991,-46.43000002,-59.64995));
#178190=CARTESIAN_POINT('Ctrl Pts',(52.1642096742619,-46.8864221486262,
-59.64995));
#178191=CARTESIAN_POINT('Ctrl Pts',(52.6623070232907,-46.43000002,-59.8463349320562));
#178192=CARTESIAN_POINT('Ctrl Pts',(52.2041414362827,-46.4300000200027,
-59.7861314645));
#178193=CARTESIAN_POINT('Ctrl Pts',(52.1642096742618,-46.8864221486274,
-59.7808732880376));
#178194=CARTESIAN_POINT('Ctrl Pts',(52.6231169025091,-46.43000002,-60.0425718399611));
#178195=CARTESIAN_POINT('Ctrl Pts',(52.175748088412,-46.43000002,-59.9224177216061));
#178196=CARTESIAN_POINT('Ctrl Pts',(52.1379836960638,-46.8875563641358,
-59.9116978933072));
#178197=CARTESIAN_POINT('Ctrl Pts',(52.4722634381817,-46.43000002,-60.4053784571342));
#178198=CARTESIAN_POINT('Ctrl Pts',(52.0676362723124,-46.43000002,-60.1718710142644));
#178199=CARTESIAN_POINT('Ctrl Pts',(52.0370327526638,-46.8919222689988,
-60.153568971423));
#178200=CARTESIAN_POINT('Ctrl Pts',(52.3606594164458,-46.43000002,-60.5717700902076));
#178201=CARTESIAN_POINT('Ctrl Pts',(51.9876181407653,-46.43000002,-60.2852157712123));
#178202=CARTESIAN_POINT('Ctrl Pts',(51.9623474855296,-46.8951522414972,
-60.264496726805));
#178203=CARTESIAN_POINT('Ctrl Pts',(52.0819185601891,-46.43000002,-60.8494502533521));
#178204=CARTESIAN_POINT('Ctrl Pts',(51.7906875266988,-46.43000002,-60.4706504746462));
#178205=CARTESIAN_POINT('Ctrl Pts',(51.7758144647026,-46.9032193817865,
-60.4496168355682));
#178206=CARTESIAN_POINT('Ctrl Pts',(51.9148913381812,-46.43000002,-60.9606295880612));
#178207=CARTESIAN_POINT('Ctrl Pts',(51.6733804433437,-46.4300000200007,
-60.5426326522478));
#178208=CARTESIAN_POINT('Ctrl Pts',(51.6640400635624,-46.9080533772402,
-60.5237363920407));
#178209=CARTESIAN_POINT('Ctrl Pts',(51.550698858526,-46.43000002,-61.1109090094727));
#178210=CARTESIAN_POINT('Ctrl Pts',(51.4220052245013,-46.4300000199993,
-60.6353187454025));
#178211=CARTESIAN_POINT('Ctrl Pts',(51.4203229267752,-46.9185936039748,
-60.6239226729819));
#178212=CARTESIAN_POINT('Ctrl Pts',(51.3537123576397,-46.43000002,-61.149949999985));
#178213=CARTESIAN_POINT('Ctrl Pts',(51.2877237368248,-46.4300000199999,
-60.6556217969811));
#178214=CARTESIAN_POINT('Ctrl Pts',(51.288499814922,-46.9242946617933,-60.64995));
#178215=CARTESIAN_POINT('Ctrl Pts',(51.1565772669927,-46.43000002,-61.14995));
#178216=CARTESIAN_POINT('Ctrl Pts',(51.1565772669928,-46.43000002,-60.64995));
#178217=CARTESIAN_POINT('Ctrl Pts',(51.1565772669927,-46.93000002,-60.64995));
#178218=CARTESIAN_POINT('',(52.1642096742619,-46.8864221486262,-59.64995));
#178219=CARTESIAN_POINT('Origin',(52.6623070233077,-46.93000002,-59.64995));
#178220=CARTESIAN_POINT('Ctrl Pts',(51.1565772669927,-46.93000002,-60.64995));
#178221=CARTESIAN_POINT('Ctrl Pts',(51.1847702648877,-46.928780735242,-60.64995));
#178222=CARTESIAN_POINT('Ctrl Pts',(51.2117854385287,-46.927612388776,-60.6487640562879));
#178223=CARTESIAN_POINT('Ctrl Pts',(51.2375495222804,-46.9264981491786,
-60.6466905423627));
#178224=CARTESIAN_POINT('Ctrl Pts',(51.264653008408,-46.9253259833931,-60.6445092322705));
#178225=CARTESIAN_POINT('Ctrl Pts',(51.2903722894732,-46.9242136814127,
-60.6413458429197));
#178226=CARTESIAN_POINT('Ctrl Pts',(51.314667764435,-46.923162955895,-60.6375094924141));
#178227=CARTESIAN_POINT('Ctrl Pts',(51.3362491645544,-46.922229608107,-60.6341017049398));
#178228=CARTESIAN_POINT('Ctrl Pts',(51.3567080746573,-46.9213448055277,
-60.6301623057541));
#178229=CARTESIAN_POINT('Ctrl Pts',(51.3760406982618,-46.9205087123465,
-60.6258833728634));
#178230=CARTESIAN_POINT('Ctrl Pts',(51.3993088743585,-46.9195024152309,
-60.6207333753234));
#178231=CARTESIAN_POINT('Ctrl Pts',(51.4209463563881,-46.9185666420243,
-60.6150923634367));
#178232=CARTESIAN_POINT('Ctrl Pts',(51.4409781638996,-46.9177003106867,
-60.6092528148882));
#178233=CARTESIAN_POINT('Ctrl Pts',(51.461841288257,-46.9167980267356,-60.6031709259978));
#178234=CARTESIAN_POINT('Ctrl Pts',(51.4809635757311,-46.9159710301266,
-60.59687378199));
#178235=CARTESIAN_POINT('Ctrl Pts',(51.4983982409252,-46.9152170194459,
-60.590641719777));
#178236=CARTESIAN_POINT('Ctrl Pts',(51.5058957306206,-46.9148927696111,
-60.587961724394));
#178237=CARTESIAN_POINT('Ctrl Pts',(51.5130813113975,-46.9145820091467,
-60.5852931620018));
#178238=CARTESIAN_POINT('Ctrl Pts',(51.5199602052477,-46.9142845122131,
-60.5826554871348));
#178239=CARTESIAN_POINT('Ctrl Pts',(51.5217040730788,-46.9142090937892,
-60.5819868103897));
#178240=CARTESIAN_POINT('Ctrl Pts',(51.5225209356732,-46.9141737217426,
-60.5816714634958));
#178241=CARTESIAN_POINT('Ctrl Pts',(51.5242736665976,-46.9140978936724,
-60.5809901111742));
#178242=CARTESIAN_POINT('Ctrl Pts',(51.5250828151279,-46.9140628876308,
-60.5806755647587));
#178243=CARTESIAN_POINT('Ctrl Pts',(51.5260912919896,-46.9140192649611,
-60.5802826897577));
#178244=CARTESIAN_POINT('Ctrl Pts',(51.5274809097942,-46.9139591688407,
-60.5797369933149));
#178245=CARTESIAN_POINT('Ctrl Pts',(51.5324129413637,-46.9137458756876,
-60.5778002074776));
#178246=CARTESIAN_POINT('Ctrl Pts',(51.5373132446684,-46.9135339542674,
-60.5758307565194));
#178247=CARTESIAN_POINT('Ctrl Pts',(51.5421814960853,-46.9133234186079,
-60.5738295347324));
#178248=CARTESIAN_POINT('Ctrl Pts',(51.575230464493,-46.9118941607979,-60.5602438938215));
#178249=CARTESIAN_POINT('Ctrl Pts',(51.6067903400481,-46.9105292839638,
-60.5452002162122));
#178250=CARTESIAN_POINT('Ctrl Pts',(51.6368130930596,-46.9092308751016,
-60.5290286703019));
#178251=CARTESIAN_POINT('Ctrl Pts',(51.665490560407,-46.9079906464745,-60.5135817531047));
#178252=CARTESIAN_POINT('Ctrl Pts',(51.6927660898016,-46.9068110401859,
-60.4971053444812));
#178253=CARTESIAN_POINT('Ctrl Pts',(51.7186284446323,-46.9056925505819,
-60.479855118547));
#178254=CARTESIAN_POINT('Ctrl Pts',(51.7476702048669,-46.9044365587312,
-60.4604842248734));
#178255=CARTESIAN_POINT('Ctrl Pts',(51.7749307436447,-46.9032576007661,
-60.4401373907221));
#178256=CARTESIAN_POINT('Ctrl Pts',(51.8004335247133,-46.9021546619314,
-60.4191325964794));
#178257=CARTESIAN_POINT('Ctrl Pts',(51.8124227509342,-46.9016361544336,
-60.4092579389186));
#178258=CARTESIAN_POINT('Ctrl Pts',(51.8240239907144,-46.9011344264906,
-60.3992372748785));
#178259=CARTESIAN_POINT('Ctrl Pts',(51.8352421085066,-46.9006492677257,
-60.3891007236107));
#178260=CARTESIAN_POINT('Ctrl Pts',(51.8406826553793,-46.9004139761152,
-60.3841847133385));
#178261=CARTESIAN_POINT('Ctrl Pts',(51.8457127685635,-46.9001964348515,
-60.3795368119428));
#178262=CARTESIAN_POINT('Ctrl Pts',(51.8507857721989,-46.8999770320173,
-60.3747537947662));
#178263=CARTESIAN_POINT('Ctrl Pts',(51.855707981935,-46.8997641508833,-60.3701129517062));
#178264=CARTESIAN_POINT('Ctrl Pts',(51.8606707216413,-46.8995495106536,
-60.3653448266592));
#178265=CARTESIAN_POINT('Ctrl Pts',(51.8660550406273,-46.899316625737,-60.3600469434816));
#178266=CARTESIAN_POINT('Ctrl Pts',(51.8670486809789,-46.8992736483705,
-60.3590692542852));
#178267=CARTESIAN_POINT('Ctrl Pts',(51.8680565774982,-46.899230054037,-60.3580734246752));
#178268=CARTESIAN_POINT('Ctrl Pts',(51.8690809779991,-46.8991857454855,
-60.3570567840805));
#178269=CARTESIAN_POINT('Ctrl Pts',(51.9031359181947,-46.8977127619508,
-60.3232598124644));
#178270=CARTESIAN_POINT('Ctrl Pts',(51.9344045600307,-46.8963604150637,
-60.2873222677668));
#178271=CARTESIAN_POINT('Ctrl Pts',(51.9627607287964,-46.8951340888708,
-60.2497596517395));
#178272=CARTESIAN_POINT('Ctrl Pts',(51.9915444077599,-46.8938892740394,
-60.2116307250254));
#178273=CARTESIAN_POINT('Ctrl Pts',(52.0173271644005,-46.8927743070765,
-60.1718273241926));
#178274=CARTESIAN_POINT('Ctrl Pts',(52.0400037418449,-46.8917936658769,
-60.1308415624652));
#178275=CARTESIAN_POINT('Ctrl Pts',(52.0577545058505,-46.8910260398738,
-60.0987587410695));
#178276=CARTESIAN_POINT('Ctrl Pts',(52.0736025244311,-46.8903406975554,
-60.0659504745663));
#178277=CARTESIAN_POINT('Ctrl Pts',(52.0875082244596,-46.8897393152827,
-60.032633432405));
#178278=CARTESIAN_POINT('Ctrl Pts',(52.0888900686388,-46.8896795544227,
-60.0293226346255));
#178279=CARTESIAN_POINT('Ctrl Pts',(52.0902527105013,-46.8896206236163,
-60.0260068882407));
#178280=CARTESIAN_POINT('Ctrl Pts',(52.0915961909269,-46.8895625210615,
-60.0226864258008));
#178281=CARTESIAN_POINT('Ctrl Pts',(52.1091485881571,-46.8888034187308,
-59.979305015382));
#178282=CARTESIAN_POINT('Ctrl Pts',(52.123429659647,-46.8881857939979,-59.9351228136313));
#178283=CARTESIAN_POINT('Ctrl Pts',(52.1345334358967,-46.8877055802516,
-59.8906338459064));
#178284=CARTESIAN_POINT('Ctrl Pts',(52.1457717122319,-46.8872195496743,
-59.8456059831406));
#178285=CARTESIAN_POINT('Ctrl Pts',(52.1537552706727,-46.8868742784422,
-59.800263845221));
#178286=CARTESIAN_POINT('Ctrl Pts',(52.158589917584,-46.886665190664,-59.7550665496285));
#178287=CARTESIAN_POINT('Ctrl Pts',(52.1623541733489,-46.8865023949338,
-59.7198759382737));
#178288=CARTESIAN_POINT('Ctrl Pts',(52.1642096742619,-46.8864221486262,
-59.6847720495211));
#178289=CARTESIAN_POINT('Ctrl Pts',(52.1642096742619,-46.8864221486262,
-59.64995));
#178290=CARTESIAN_POINT('Origin',(0.,-12.9675000200281,-60.64995));
#178291=CARTESIAN_POINT('',(53.7167487055513,-17.6671065732338,-60.64995));
#178292=CARTESIAN_POINT('Ctrl Pts',(50.6621396387151,-53.08000002,-61.1499499946262));
#178293=CARTESIAN_POINT('Ctrl Pts',(50.6621815241177,-53.0800000199999,
-60.6498941830841));
#178294=CARTESIAN_POINT('Ctrl Pts',(50.6621815444126,-52.5799442087081,
-60.6499499995188));
#178295=CARTESIAN_POINT('Ctrl Pts',(50.8593170188006,-53.08000002,-61.1499667235322));
#178296=CARTESIAN_POINT('Ctrl Pts',(50.7949219565861,-53.08000002,-60.6441634129678));
#178297=CARTESIAN_POINT('Ctrl Pts',(50.7941322985337,-52.5742372910461,
-60.6499618311926));
#178298=CARTESIAN_POINT('Ctrl Pts',(51.0563489044894,-53.08000002,-61.1109251044403));
#178299=CARTESIAN_POINT('Ctrl Pts',(50.9242606677665,-53.08000002,-60.6119868070572));
#178300=CARTESIAN_POINT('Ctrl Pts',(50.925986077618,-52.5685345954075,-60.6239348042603));
#178301=CARTESIAN_POINT('Ctrl Pts',(51.4205803892599,-53.08000002,-60.9606295880612));
#178302=CARTESIAN_POINT('Ctrl Pts',(51.1595367031111,-53.08000002,-60.5030970594232));
#178303=CARTESIAN_POINT('Ctrl Pts',(51.1697302983437,-52.5579926660341,
-60.5237387895063));
#178304=CARTESIAN_POINT('Ctrl Pts',(51.5876076112677,-53.08000002,-60.8494502533514));
#178305=CARTESIAN_POINT('Ctrl Pts',(51.2649595932576,-53.0800000200007,
-60.4261477374134));
#178306=CARTESIAN_POINT('Ctrl Pts',(51.2815054280689,-52.5531584192985,
-60.4496195485702));
#178307=CARTESIAN_POINT('Ctrl Pts',(51.8663484675245,-53.08000002,-60.5717700902082));
#178308=CARTESIAN_POINT('Ctrl Pts',(51.4389731852977,-53.0800000199992,
-60.2406358789611));
#178309=CARTESIAN_POINT('Ctrl Pts',(51.4680398681885,-52.545090875362,-60.2644994621532));
#178310=CARTESIAN_POINT('Ctrl Pts',(51.9779524892604,-53.08000002,-60.4053784571342));
#178311=CARTESIAN_POINT('Ctrl Pts',(51.507034264404,-53.08000002,-60.1321953438333));
#178312=CARTESIAN_POINT('Ctrl Pts',(51.5427258807753,-52.5418607474287,
-60.1535714132618));
#178313=CARTESIAN_POINT('Ctrl Pts',(52.1288221100354,-53.08000002,-60.0425329832722));
#178314=CARTESIAN_POINT('Ctrl Pts',(51.5988650708495,-53.08000002,-59.8989282761487));
#178315=CARTESIAN_POINT('Ctrl Pts',(51.6436886553452,-52.5374941696185,
-59.9116734379909));
#178316=CARTESIAN_POINT('Ctrl Pts',(52.1680128617978,-53.08000002,-59.8462508632673));
#178317=CARTESIAN_POINT('Ctrl Pts',(51.6222839264631,-53.0800000200021,
-59.7745406636097));
#178318=CARTESIAN_POINT('Ctrl Pts',(51.6699153683916,-52.5363598840896,
-59.7808179550158));
#178319=CARTESIAN_POINT('Ctrl Pts',(52.167996068992,-53.08000002,-59.6498238026969));
#178320=CARTESIAN_POINT('Ctrl Pts',(51.6222738795813,-53.08000002,-59.6498699040835));
#178321=CARTESIAN_POINT('Ctrl Pts',(51.6699041305595,-52.536360369711,-59.6498658680063));
#178322=CARTESIAN_POINT('',(51.6698987253405,-52.5364221486262,-59.64995));
#178323=CARTESIAN_POINT('',(52.1679960743864,-53.08000002,-59.64995));
#178324=CARTESIAN_POINT('Origin',(52.1679960743864,-52.58000002,-59.64995));
#178325=CARTESIAN_POINT('Ctrl Pts',(50.6622663180714,-53.08000002,-61.14995));
#178326=CARTESIAN_POINT('Ctrl Pts',(50.8594014087184,-53.08000002,-61.149949999985));
#178327=CARTESIAN_POINT('Ctrl Pts',(51.0563879096046,-53.08000002,-61.1109090094727));
#178328=CARTESIAN_POINT('Ctrl Pts',(51.4205803892599,-53.08000002,-60.9606295880612));
#178329=CARTESIAN_POINT('Ctrl Pts',(51.5876076112677,-53.08000002,-60.8494502533514));
#178330=CARTESIAN_POINT('Ctrl Pts',(51.8663484675245,-53.08000002,-60.5717700902082));
#178331=CARTESIAN_POINT('Ctrl Pts',(51.9779524892604,-53.08000002,-60.4053784571342));
#178332=CARTESIAN_POINT('Ctrl Pts',(52.1288059535877,-53.08000002,-60.0425718399611));
#178333=CARTESIAN_POINT('Ctrl Pts',(52.1679960743694,-53.08000002,-59.8463349320561));
#178334=CARTESIAN_POINT('Ctrl Pts',(52.1679960743864,-53.08000002,-59.64995));
#178335=CARTESIAN_POINT('Ctrl Pts',(51.6698987253405,-52.5364221486262,
-59.64995));
#178336=CARTESIAN_POINT('Ctrl Pts',(51.6698987253405,-52.5364221486262,
-59.6909727319776));
#178337=CARTESIAN_POINT('Ctrl Pts',(51.6673501566751,-52.5365526733191,
-59.7323929144446));
#178338=CARTESIAN_POINT('Ctrl Pts',(51.6621266428239,-52.5368026661919,
-59.7738824503071));
#178339=CARTESIAN_POINT('Ctrl Pts',(51.6570039945927,-52.537047831723,-59.8145708266674));
#178340=CARTESIAN_POINT('Ctrl Pts',(51.6493083876707,-52.5374078679653,
-59.855325534387));
#178341=CARTESIAN_POINT('Ctrl Pts',(51.638960382346,-52.5378758248444,-59.8958071079189));
#178342=CARTESIAN_POINT('Ctrl Pts',(51.6287267706847,-52.53833860862,-59.935841171486));
#178343=CARTESIAN_POINT('Ctrl Pts',(51.6158987551754,-52.5389069118211,
-59.9756077249091));
#178344=CARTESIAN_POINT('Ctrl Pts',(51.6004436152177,-52.5395778717659,
-60.014754279517));
#178345=CARTESIAN_POINT('Ctrl Pts',(51.5852405811232,-52.5402378869418,
-60.0532622714225));
#178346=CARTESIAN_POINT('Ctrl Pts',(51.5674952125664,-52.5409972179362,
-60.0911698875945));
#178347=CARTESIAN_POINT('Ctrl Pts',(51.5472232272244,-52.5418572398676,
-60.1281241911634));
#178348=CARTESIAN_POINT('Ctrl Pts',(51.5340632031642,-52.5424155428221,
-60.1521139245758));
#178349=CARTESIAN_POINT('Ctrl Pts',(51.5198393596716,-52.5430163636053,
-60.1757015641967));
#178350=CARTESIAN_POINT('Ctrl Pts',(51.5045674653046,-52.5436610817872,
-60.1987879161313));
#178351=CARTESIAN_POINT('Ctrl Pts',(51.4859751882522,-52.5444459732205,
-60.2268936534408));
#178352=CARTESIAN_POINT('Ctrl Pts',(51.465828954641,-52.5452958698133,-60.2542563740088));
#178353=CARTESIAN_POINT('Ctrl Pts',(51.4441764790361,-52.5462149460492,
-60.2806949718832));
#178354=CARTESIAN_POINT('Ctrl Pts',(51.4333502412336,-52.5466744841671,
-60.2939142708204));
#178355=CARTESIAN_POINT('Ctrl Pts',(51.4221477801373,-52.5471513466974,
-60.3069025151278));
#178356=CARTESIAN_POINT('Ctrl Pts',(51.4105771261679,-52.5476462362108,
-60.31963703049));
#178357=CARTESIAN_POINT('Ctrl Pts',(51.4053718121764,-52.547868873178,-60.3253659332093));
#178358=CARTESIAN_POINT('Ctrl Pts',(51.3998136381294,-52.5481087671514,
-60.3313432769659));
#178359=CARTESIAN_POINT('Ctrl Pts',(51.3942727867154,-52.5483470728028,
-60.3371563975798));
#178360=CARTESIAN_POINT('Ctrl Pts',(51.3885513244787,-52.5485931463181,
-60.3431590039636));
#178361=CARTESIAN_POINT('Ctrl Pts',(51.3828485134777,-52.5488375421032,
-60.348986368698));
#178362=CARTESIAN_POINT('Ctrl Pts',(51.3776130998802,-52.5490631132445,
-60.3542239160814));
#178363=CARTESIAN_POINT('Ctrl Pts',(51.3766484642515,-52.5491046751872,
-60.3551889448644));
#178364=CARTESIAN_POINT('Ctrl Pts',(51.3756997959006,-52.5491456067773,
-60.35613405362));
#178365=CARTESIAN_POINT('Ctrl Pts',(51.3747700261947,-52.5491858116419,
-60.3570567811866));
#178366=CARTESIAN_POINT('Ctrl Pts',(51.3526390232836,-52.5501427948295,
-60.3790201623695));
#178367=CARTESIAN_POINT('Ctrl Pts',(51.3288180644561,-52.5511805791252,
-60.4006133580694));
#178368=CARTESIAN_POINT('Ctrl Pts',(51.303238450899,-52.5522931541618,-60.4215416019267));
#178369=CARTESIAN_POINT('Ctrl Pts',(51.2783615492186,-52.5533751650271,
-60.441894914287));
#178370=CARTESIAN_POINT('Ctrl Pts',(51.251820855113,-52.5545278756568,-60.4616189803006));
#178371=CARTESIAN_POINT('Ctrl Pts',(51.2235909594968,-52.5557490630439,
-60.480412172761));
#178372=CARTESIAN_POINT('Ctrl Pts',(51.1953610638806,-52.5569702504311,
-60.4992053652214));
#178373=CARTESIAN_POINT('Ctrl Pts',(51.1654413519975,-52.5582598607915,
-60.5170673741396));
#178374=CARTESIAN_POINT('Ctrl Pts',(51.1338527951471,-52.5596197288762,
-60.533670156548));
#178375=CARTESIAN_POINT('Ctrl Pts',(51.1179098000908,-52.5603060650788,
-60.5420497124458));
#178376=CARTESIAN_POINT('Ctrl Pts',(51.1015424911284,-52.5610103672524,
-60.550108114142));
#178377=CARTESIAN_POINT('Ctrl Pts',(51.084758846286,-52.561733333384,-60.5578010742774));
#178378=CARTESIAN_POINT('Ctrl Pts',(51.0763670238648,-52.5620948164497,
-60.5616475543451));
#178379=CARTESIAN_POINT('Ctrl Pts',(51.0678711199813,-52.5624609657244,
-60.5654026796418));
#178380=CARTESIAN_POINT('Ctrl Pts',(51.0592725606525,-52.5628319059683,
-60.5690607763373));
#178381=CARTESIAN_POINT('Ctrl Pts',(51.0549732809881,-52.5630173760902,
-60.570889824685));
#178382=CARTESIAN_POINT('Ctrl Pts',(51.050648337782,-52.5632040439824,-60.5726946165842));
#178383=CARTESIAN_POINT('Ctrl Pts',(51.0462979245109,-52.5633919265719,
-60.5744744410932));
#178384=CARTESIAN_POINT('Ctrl Pts',(51.0436566325577,-52.5635059968317,
-60.5755550363978));
#178385=CARTESIAN_POINT('Ctrl Pts',(51.0402941624751,-52.5636516104294,
-60.5769130552168));
#178386=CARTESIAN_POINT('Ctrl Pts',(51.0375058723162,-52.5637720333269,
-60.5780234112916));
#178387=CARTESIAN_POINT('Ctrl Pts',(51.0357016317266,-52.5638499563074,
-60.5787418980289));
#178388=CARTESIAN_POINT('Ctrl Pts',(51.0341383546808,-52.5639173797187,
-60.5793580291782));
#178389=CARTESIAN_POINT('Ctrl Pts',(51.0331704763702,-52.5639592360933,
-60.5797383010625));
#178390=CARTESIAN_POINT('Ctrl Pts',(51.0177910339138,-52.5646243276637,
-60.5857807647669));
#178391=CARTESIAN_POINT('Ctrl Pts',(51.0007801641594,-52.5653695793414,
-60.5920329991653));
#178392=CARTESIAN_POINT('Ctrl Pts',(50.9820750389557,-52.5661894943757,
-60.5982457361307));
#178393=CARTESIAN_POINT('Ctrl Pts',(50.9637818123841,-52.5669913543647,
-60.6043216647171));
#178394=CARTESIAN_POINT('Ctrl Pts',(50.9438673635558,-52.5678645589462,
-60.6103597061813));
#178395=CARTESIAN_POINT('Ctrl Pts',(50.922288997128,-52.5688053727616,-60.6160795502538));
#178396=CARTESIAN_POINT('Ctrl Pts',(50.9015511090088,-52.5697095418381,
-60.6215766061516));
#178397=CARTESIAN_POINT('Ctrl Pts',(50.8792757525235,-52.5706760994577,
-60.6267794462207));
#178398=CARTESIAN_POINT('Ctrl Pts',(50.8554501117109,-52.571703924369,-60.6313985657287));
#178399=CARTESIAN_POINT('Ctrl Pts',(50.8322254333362,-52.5727058240945,
-60.6359011755762));
#178400=CARTESIAN_POINT('Ctrl Pts',(50.8075270414602,-52.5737658825278,
-60.6398488177474));
#178401=CARTESIAN_POINT('Ctrl Pts',(50.7813768373136,-52.5748860157782,
-60.6429384333447));
#178402=CARTESIAN_POINT('Ctrl Pts',(50.7562094246909,-52.5759640515575,
-60.6459119332894));
#178403=CARTESIAN_POINT('Ctrl Pts',(50.7296968033627,-52.5770976902288,
-60.6480902251289));
#178404=CARTESIAN_POINT('Ctrl Pts',(50.701898127047,-52.5782921070719,-60.6491761918521));
#178405=CARTESIAN_POINT('Ctrl Pts',(50.6889622309209,-52.5788479195876,
-60.6496815379545));
#178406=CARTESIAN_POINT('Ctrl Pts',(50.6757484635432,-52.579416947049,-60.64995));
#178407=CARTESIAN_POINT('Ctrl Pts',(50.6622663180714,-52.58000002,-60.64995));
#178408=CARTESIAN_POINT('Origin',(-83.2809572255632,-53.0800000199999,-55.2499500000008));
#178409=CARTESIAN_POINT('',(52.1679960743864,-53.08000002,-55.74995));
#178410=CARTESIAN_POINT('',(52.1679960743864,-53.08000002,-55.2499500000008));
#178411=CARTESIAN_POINT('',(-83.2809572255632,-53.0800000199999,-55.74995));
#178412=CARTESIAN_POINT('Origin',(-83.2809572255632,-53.5800000199999,-55.74995));
#178413=CARTESIAN_POINT('',(52.0805074108605,-53.58000002,-55.24995));
#178414=CARTESIAN_POINT('Ctrl Pts',(52.1679960743864,-53.08000002,-55.74995));
#178415=CARTESIAN_POINT('Ctrl Pts',(52.1679960743853,-53.08000002,-55.7240274879025));
#178416=CARTESIAN_POINT('Ctrl Pts',(52.1676229277195,-53.0821037999966,
-55.6978059982456));
#178417=CARTESIAN_POINT('Ctrl Pts',(52.1668732945162,-53.0863531598489,
-55.6716073791772));
#178418=CARTESIAN_POINT('Ctrl Pts',(52.1661171274503,-53.0906395574591,
-55.6451804108644));
#178419=CARTESIAN_POINT('Ctrl Pts',(52.1649778773335,-53.097109134404,-55.6187767710135));
#178420=CARTESIAN_POINT('Ctrl Pts',(52.1634571283852,-53.1057761303949,
-55.5927712432962));
#178421=CARTESIAN_POINT('Ctrl Pts',(52.162887909333,-53.1090202025008,-55.5830373277441));
#178422=CARTESIAN_POINT('Ctrl Pts',(52.1622652919261,-53.1125718487088,
-55.5733596268362));
#178423=CARTESIAN_POINT('Ctrl Pts',(52.1615895390385,-53.1164307841406,
-55.5637593430561));
#178424=CARTESIAN_POINT('Ctrl Pts',(52.1598114689721,-53.1265845810459,
-55.5384986634051));
#178425=CARTESIAN_POINT('Ctrl Pts',(52.1576634617214,-53.138872774755,-55.5137551378007));
#178426=CARTESIAN_POINT('Ctrl Pts',(52.1551452115047,-53.1532950399446,
-55.4899268496365));
#178427=CARTESIAN_POINT('Ctrl Pts',(52.154639066555,-53.1561937815553,-55.4851375846006));
#178428=CARTESIAN_POINT('Ctrl Pts',(52.1541179724691,-53.1591786897697,
-55.4803854546854));
#178429=CARTESIAN_POINT('Ctrl Pts',(52.1535819385834,-53.1622496940383,
-55.4756739403427));
#178430=CARTESIAN_POINT('Ctrl Pts',(52.1519804425163,-53.171424862605,-55.4615974576943));
#178431=CARTESIAN_POINT('Ctrl Pts',(52.1502454794431,-53.1813686932119,
-55.4478834521503));
#178432=CARTESIAN_POINT('Ctrl Pts',(52.1483770292202,-53.1920727510362,
-55.4346345057453));
#178433=CARTESIAN_POINT('Ctrl Pts',(52.1474428041087,-53.1974247799484,
-55.4280100325428));
#178434=CARTESIAN_POINT('Ctrl Pts',(52.1464752077285,-53.2029668120848,
-55.4215019156276));
#178435=CARTESIAN_POINT('Ctrl Pts',(52.1454742415707,-53.2086966555084,
-55.4151241749442));
#178436=CARTESIAN_POINT('Ctrl Pts',(52.1449737584918,-53.2115615772202,
-55.4119353046026));
#178437=CARTESIAN_POINT('Ctrl Pts',(52.1444649330249,-53.2144734423564,
-55.4087790343855));
#178438=CARTESIAN_POINT('Ctrl Pts',(52.1439477656179,-53.2174318984733,
-55.4056571673729));
#178439=CARTESIAN_POINT('Ctrl Pts',(52.1436468211098,-53.2191534515113,
-55.4038405240201));
#178440=CARTESIAN_POINT('Ctrl Pts',(52.143280043092,-53.221250909685,-55.4016627141745));
#178441=CARTESIAN_POINT('Ctrl Pts',(52.14295686691,-53.2230986811324,-55.399777933182));
#178442=CARTESIAN_POINT('Ctrl Pts',(52.1427246709765,-53.2244262697353,
-55.3984237539257));
#178443=CARTESIAN_POINT('Ctrl Pts',(52.142515217764,-53.2256236244485,-55.3972196143704));
#178444=CARTESIAN_POINT('Ctrl Pts',(52.1423712114632,-53.2264466282408,
-55.3963966105727));
#178445=CARTESIAN_POINT('Ctrl Pts',(52.1406599696547,-53.2362264676637,
-55.3866167710853));
#178446=CARTESIAN_POINT('Ctrl Pts',(52.1387217223152,-53.2471430351613,
-55.3765446166362));
#178447=CARTESIAN_POINT('Ctrl Pts',(52.1365506278256,-53.2593251459205,
-55.3664154210889));
#178448=CARTESIAN_POINT('Ctrl Pts',(52.1344728039586,-53.2709839109385,
-55.3567213776639));
#178449=CARTESIAN_POINT('Ctrl Pts',(52.1321815884692,-53.2838025291941,
-55.3469750522698));
#178450=CARTESIAN_POINT('Ctrl Pts',(52.1296756874241,-53.2978716577507,
-55.3374234998531));
#178451=CARTESIAN_POINT('Ctrl Pts',(52.1273146090356,-53.3111276941156,
-55.3284239569412));
#178452=CARTESIAN_POINT('Ctrl Pts',(52.1247628683279,-53.3254943241106,
-55.3195974076226));
#178453=CARTESIAN_POINT('Ctrl Pts',(52.1220241933538,-53.34101923469,-55.3111870425976));
#178454=CARTESIAN_POINT('Ctrl Pts',(52.1209256544364,-53.3472465959582,
-55.3078134720292));
#178455=CARTESIAN_POINT('Ctrl Pts',(52.1197971005136,-53.3536599563752,
-55.3045072865547));
#178456=CARTESIAN_POINT('Ctrl Pts',(52.1186390490883,-53.3602607645211,
-55.3012859404982));
#178457=CARTESIAN_POINT('Ctrl Pts',(52.115966476223,-53.3754942337384,-55.2938516574671));
#178458=CARTESIAN_POINT('Ctrl Pts',(52.1131421434498,-53.3917391401417,
-55.2868619640634));
#178459=CARTESIAN_POINT('Ctrl Pts',(52.1101547447912,-53.4089873541471,
-55.2805581080823));
#178460=CARTESIAN_POINT('Ctrl Pts',(52.1072491175401,-53.4257634481247,
-55.2744268019467));
#178461=CARTESIAN_POINT('Ctrl Pts',(52.1041891699554,-53.443488989223,-55.2689442788315));
#178462=CARTESIAN_POINT('Ctrl Pts',(52.1009710259383,-53.4621198498038,
-55.2643620190281));
#178463=CARTESIAN_POINT('Ctrl Pts',(52.0978518894124,-53.480177524488,-55.259920734285));
#178464=CARTESIAN_POINT('Ctrl Pts',(52.0945840982727,-53.4990858905757,
-55.2563251748323));
#178465=CARTESIAN_POINT('Ctrl Pts',(52.0911710656404,-53.5187660556456,
-55.2538325278704));
#178466=CARTESIAN_POINT('Ctrl Pts',(52.0877580330082,-53.5384462207154,
-55.2513398809084));
#178467=CARTESIAN_POINT('Ctrl Pts',(52.0841996828067,-53.5588985892674,
-55.24995));
#178468=CARTESIAN_POINT('Ctrl Pts',(52.0805074108605,-53.58000002,-55.24995));
#178469=CARTESIAN_POINT('',(60.,-53.58000002,-55.24995));
#178470=CARTESIAN_POINT('Origin',(60.,28.41999998,-55.24995));
#178471=CARTESIAN_POINT('',(52.0367630790975,-54.08000002,-55.24995));
#178472=CARTESIAN_POINT('',(59.2602401389193,28.4847205815761,-55.24995));
#178473=CARTESIAN_POINT('',(60.,-54.08000002,-55.24995));
#178474=CARTESIAN_POINT('Origin',(60.,-54.08000002,-55.74995));
#178475=CARTESIAN_POINT('',(51.9492744155716,-54.58000002,-55.74995));
#178476=CARTESIAN_POINT('Ctrl Pts',(52.0367630790975,-54.08000002,-55.24995));
#178477=CARTESIAN_POINT('Ctrl Pts',(52.0329861847726,-54.1015850698379,
-55.24995));
#178478=CARTESIAN_POINT('Ctrl Pts',(52.0293284334102,-54.1224892145297,
-55.2514041468282));
#178479=CARTESIAN_POINT('Ctrl Pts',(52.025812604289,-54.1425822699015,-55.2540052053876));
#178480=CARTESIAN_POINT('Ctrl Pts',(52.0223225188274,-54.1625281995854,
-55.256587218435));
#178481=CARTESIAN_POINT('Ctrl Pts',(52.0189721930573,-54.181675398978,-55.2602996172422));
#178482=CARTESIAN_POINT('Ctrl Pts',(52.0157756716516,-54.1999436024055,
-55.2648742467057));
#178483=CARTESIAN_POINT('Ctrl Pts',(52.012433722523,-54.2190429290726,-55.2696570017726));
#178484=CARTESIAN_POINT('Ctrl Pts',(52.0092598588055,-54.2371816432191,
-55.2753821626562));
#178485=CARTESIAN_POINT('Ctrl Pts',(52.0062619536595,-54.2543147495282,
-55.2817780783384));
#178486=CARTESIAN_POINT('Ctrl Pts',(52.0034615083816,-54.2703193675273,
-55.2877527209631));
#178487=CARTESIAN_POINT('Ctrl Pts',(52.0008144668557,-54.2854472790713,
-55.2943131225512));
#178488=CARTESIAN_POINT('Ctrl Pts',(51.9983217548574,-54.2996931933296,
-55.3012636513334));
#178489=CARTESIAN_POINT('Ctrl Pts',(51.9954258794196,-54.3162431971871,
-55.3093383368938));
#178490=CARTESIAN_POINT('Ctrl Pts',(51.9927365497521,-54.3316127865661,
-55.3179437622875));
#178491=CARTESIAN_POINT('Ctrl Pts',(51.9902476016194,-54.3458371902331,
-55.3268178701949));
#178492=CARTESIAN_POINT('Ctrl Pts',(51.9875709569559,-54.3611342844827,
-55.3363611922362));
#178493=CARTESIAN_POINT('Ctrl Pts',(51.9851258946601,-54.3751078794446,
-55.3462154234411));
#178494=CARTESIAN_POINT('Ctrl Pts',(51.982897837809,-54.3878412826151,-55.3561026477775));
#178495=CARTESIAN_POINT('Ctrl Pts',(51.9806310002184,-54.4007963187263,
-55.3661619655108));
#178496=CARTESIAN_POINT('Ctrl Pts',(51.9785887493121,-54.412467836063,-55.3762552368074));
#178497=CARTESIAN_POINT('Ctrl Pts',(51.9767506920852,-54.4229723811826,
-55.3861352301679));
#178498=CARTESIAN_POINT('Ctrl Pts',(51.9764819137112,-54.4245084566188,
-55.3875799776498));
#178499=CARTESIAN_POINT('Ctrl Pts',(51.9762174950408,-54.426019616235,-55.3890202398743));
#178500=CARTESIAN_POINT('Ctrl Pts',(51.9759573640587,-54.4275062716008,
-55.3904553319312));
#178501=CARTESIAN_POINT('Ctrl Pts',(51.9757360420398,-54.4287711327266,
-55.3916763224825));
#178502=CARTESIAN_POINT('Ctrl Pts',(51.9755897917165,-54.4296069571404,
-55.3924916493989));
#178503=CARTESIAN_POINT('Ctrl Pts',(51.9753858285837,-54.4307725552473,
-55.3936383709987));
#178504=CARTESIAN_POINT('Ctrl Pts',(51.9752572031324,-54.4315076174146,
-55.3943615290577));
#178505=CARTESIAN_POINT('Ctrl Pts',(51.9751056704388,-54.4323735725912,
-55.3952167714171));
#178506=CARTESIAN_POINT('Ctrl Pts',(51.9748992092877,-54.4335534087318,
-55.3963966075453));
#178507=CARTESIAN_POINT('Ctrl Pts',(51.9712989344309,-54.4541274216573,
-55.4169706202541));
#178508=CARTESIAN_POINT('Ctrl Pts',(51.9680709073607,-54.4725747479987,
-55.4391630475832));
#178509=CARTESIAN_POINT('Ctrl Pts',(51.9652226122223,-54.4888523769156,
-55.4624843705238));
#178510=CARTESIAN_POINT('Ctrl Pts',(51.9623708011184,-54.505150099109,-55.485834481551));
#178511=CARTESIAN_POINT('Ctrl Pts',(51.9598996566805,-54.5192727832056,
-55.510316262681));
#178512=CARTESIAN_POINT('Ctrl Pts',(51.9578126185396,-54.5312005418129,
-55.5354850646356));
#178513=CARTESIAN_POINT('Ctrl Pts',(51.9557220179087,-54.5431486606235,
-55.5606968287208));
#178514=CARTESIAN_POINT('Ctrl Pts',(51.9540168314626,-54.5528943804173,
-55.586597961014));
#178515=CARTESIAN_POINT('Ctrl Pts',(51.952696491472,-54.5604407216792,-55.6127884602357));
#178516=CARTESIAN_POINT('Ctrl Pts',(51.9513702043265,-54.5680210536256,
-55.63909692828));
#178517=CARTESIAN_POINT('Ctrl Pts',(51.9504322340363,-54.5733821741393,
-55.6656973722207));
#178518=CARTESIAN_POINT('Ctrl Pts',(51.9498780110353,-54.5765499745511,
-55.6922317349674));
#178519=CARTESIAN_POINT('Ctrl Pts',(51.9494745942481,-54.5788558042664,
-55.7115459953829));
#178520=CARTESIAN_POINT('Ctrl Pts',(51.9492744155716,-54.58000002,-55.7308262346054));
#178521=CARTESIAN_POINT('Ctrl Pts',(51.9492744155716,-54.58000002,-55.74995));
#178522=CARTESIAN_POINT('',(60.,-54.58000002,-55.74995));
#178523=CARTESIAN_POINT('Origin',(60.,-54.58000002,-55.24995));
#178524=CARTESIAN_POINT('',(51.9492744155716,-54.58000002,-59.64995));
#178525=CARTESIAN_POINT('',(51.9492744155716,-54.58000002,-55.24995));
#178526=CARTESIAN_POINT('Ctrl Pts',(51.9492744155716,-54.58000002,-59.64995));
#178527=CARTESIAN_POINT('Ctrl Pts',(51.9492744155546,-54.58000002,-59.8463349320562));
#178528=CARTESIAN_POINT('Ctrl Pts',(51.9100842947729,-54.58000002,-60.0425718399611));
#178529=CARTESIAN_POINT('Ctrl Pts',(51.7592308304456,-54.58000002,-60.4053784571342));
#178530=CARTESIAN_POINT('Ctrl Pts',(51.6476268087097,-54.58000002,-60.5717700902076));
#178531=CARTESIAN_POINT('Ctrl Pts',(51.3688859524529,-54.58000002,-60.8494502533521));
#178532=CARTESIAN_POINT('Ctrl Pts',(51.2018587304451,-54.58000002,-60.9606295880612));
#178533=CARTESIAN_POINT('Ctrl Pts',(50.8376662507899,-54.58000002,-61.1109090094727));
#178534=CARTESIAN_POINT('Ctrl Pts',(50.6406797499036,-54.58000002,-61.149949999985));
#178535=CARTESIAN_POINT('Ctrl Pts',(50.4435446592566,-54.58000002,-61.14995));
#178536=CARTESIAN_POINT('Ctrl Pts',(51.9492744155716,-54.58000002,-59.64995));
#178537=CARTESIAN_POINT('Ctrl Pts',(51.491108828563,-54.58000002,-59.64995));
#178538=CARTESIAN_POINT('Ctrl Pts',(51.4511770665258,-55.0364221486262,
-59.64995));
#178539=CARTESIAN_POINT('Ctrl Pts',(51.9492744155546,-54.58000002,-59.8463349320562));
#178540=CARTESIAN_POINT('Ctrl Pts',(51.4911088285445,-54.58000002,-59.7861314644994));
#178541=CARTESIAN_POINT('Ctrl Pts',(51.4511770665255,-55.0364221486294,
-59.7808732880376));
#178542=CARTESIAN_POINT('Ctrl Pts',(51.9100842947729,-54.58000002,-60.0425718399611));
#178543=CARTESIAN_POINT('Ctrl Pts',(51.4627154806765,-54.58000002,-59.9224177216068));
#178544=CARTESIAN_POINT('Ctrl Pts',(51.4249510883276,-55.0375563641359,
-59.9116978933072));
#178545=CARTESIAN_POINT('Ctrl Pts',(51.7592308304456,-54.58000002,-60.4053784571342));
#178546=CARTESIAN_POINT('Ctrl Pts',(51.3546036645756,-54.58000002,-60.1718710142638));
#178547=CARTESIAN_POINT('Ctrl Pts',(51.3240001449277,-55.0419222689988,
-60.153568971423));
#178548=CARTESIAN_POINT('Ctrl Pts',(51.6476268087097,-54.58000002,-60.5717700902076));
#178549=CARTESIAN_POINT('Ctrl Pts',(51.2745855330292,-54.58000002,-60.2852157712116));
#178550=CARTESIAN_POINT('Ctrl Pts',(51.2493148777934,-55.0451522414979,
-60.2644967268049));
#178551=CARTESIAN_POINT('Ctrl Pts',(51.3688859524529,-54.58000002,-60.8494502533521));
#178552=CARTESIAN_POINT('Ctrl Pts',(51.0776549189628,-54.58000002,-60.4706504746468));
#178553=CARTESIAN_POINT('Ctrl Pts',(51.0627818569665,-55.0532193817859,
-60.4496168355682));
#178554=CARTESIAN_POINT('Ctrl Pts',(51.2018587304451,-54.58000002,-60.9606295880612));
#178555=CARTESIAN_POINT('Ctrl Pts',(50.9603478356083,-54.5800000199993,
-60.5426326522464));
#178556=CARTESIAN_POINT('Ctrl Pts',(50.9510074558263,-55.0580533772402,
-60.5237363920407));
#178557=CARTESIAN_POINT('Ctrl Pts',(50.8376662507899,-54.58000002,-61.1109090094727));
#178558=CARTESIAN_POINT('Ctrl Pts',(50.7089726167645,-54.5800000200007,
-60.6353187454038));
#178559=CARTESIAN_POINT('Ctrl Pts',(50.707290319039,-55.0685936039748,-60.6239226729819));
#178560=CARTESIAN_POINT('Ctrl Pts',(50.6406797499036,-54.58000002,-61.149949999985));
#178561=CARTESIAN_POINT('Ctrl Pts',(50.5746911290892,-54.58000002,-60.6556217969812));
#178562=CARTESIAN_POINT('Ctrl Pts',(50.5754672071858,-55.0742946617933,
-60.64995));
#178563=CARTESIAN_POINT('Ctrl Pts',(50.4435446592566,-54.58000002,-61.14995));
#178564=CARTESIAN_POINT('Ctrl Pts',(50.4435446592566,-54.58000002,-60.64995));
#178565=CARTESIAN_POINT('Ctrl Pts',(50.4435446592566,-55.08000002,-60.64995));
#178566=CARTESIAN_POINT('',(51.4511770665258,-55.0364221486262,-59.64995));
#178567=CARTESIAN_POINT('Origin',(51.9492744155716,-55.08000002,-59.64995));
#178568=CARTESIAN_POINT('Ctrl Pts',(50.4435446592566,-55.08000002,-60.64995));
#178569=CARTESIAN_POINT('Ctrl Pts',(50.4717376569834,-55.0787807352492,
-60.64995));
#178570=CARTESIAN_POINT('Ctrl Pts',(50.4987528304453,-55.077612388791,-60.6487640563021));
#178571=CARTESIAN_POINT('Ctrl Pts',(50.5245169140085,-55.0764981492017,
-60.6466905424058));
#178572=CARTESIAN_POINT('Ctrl Pts',(50.5516203999557,-55.075325983424,-60.6445092323426));
#178573=CARTESIAN_POINT('Ctrl Pts',(50.5773396808283,-55.074213681452,-60.6413458430357));
#178574=CARTESIAN_POINT('Ctrl Pts',(50.6016351555871,-55.073162955943,-60.6375094925897));
#178575=CARTESIAN_POINT('Ctrl Pts',(50.6232165566326,-55.072229608115,-60.6341017049935));
#178576=CARTESIAN_POINT('Ctrl Pts',(50.6436754675382,-55.071344805501,-60.6301623056439));
#178577=CARTESIAN_POINT('Ctrl Pts',(50.6630080918224,-55.0705087122905,
-60.6258833725764));
#178578=CARTESIAN_POINT('Ctrl Pts',(50.6862762675633,-55.0695024151902,
-60.6207333750833));
#178579=CARTESIAN_POINT('Ctrl Pts',(50.707913749224,-55.0685666419995,-60.6150923632743));
#178580=CARTESIAN_POINT('Ctrl Pts',(50.7279455563559,-55.0677003106784,
-60.6092528148321));
#178581=CARTESIAN_POINT('Ctrl Pts',(50.748808680122,-55.0667980267528,-60.6031709261096));
#178582=CARTESIAN_POINT('Ctrl Pts',(50.7679309670258,-55.0659710301685,
-60.596873782305));
#178583=CARTESIAN_POINT('Ctrl Pts',(50.7853656316707,-55.0652170195116,
-60.5906417203197));
#178584=CARTESIAN_POINT('Ctrl Pts',(50.7928631219894,-55.0648927696499,
-60.5879617247275));
#178585=CARTESIAN_POINT('Ctrl Pts',(50.8000487033219,-55.0645820091614,
-60.5852931621332));
#178586=CARTESIAN_POINT('Ctrl Pts',(50.8069275976617,-55.0642845122066,
-60.5826554870772));
#178587=CARTESIAN_POINT('Ctrl Pts',(50.808671465437,-55.0642090937851,-60.5819868103532));
#178588=CARTESIAN_POINT('Ctrl Pts',(50.8094883279451,-55.0641737217418,
-60.5816714634925));
#178589=CARTESIAN_POINT('Ctrl Pts',(50.8112410587908,-55.0640978936747,
-60.5809901112017));
#178590=CARTESIAN_POINT('Ctrl Pts',(50.8120502073179,-55.0640628876332,
-60.5806755647874));
#178591=CARTESIAN_POINT('Ctrl Pts',(50.8130586841946,-55.0640192649628,
-60.5802826897809));
#178592=CARTESIAN_POINT('Ctrl Pts',(50.814448302058,-55.0639591688398,-60.579736993315));
#178593=CARTESIAN_POINT('Ctrl Pts',(50.8193803336296,-55.0637458756867,
-60.5778002074769));
#178594=CARTESIAN_POINT('Ctrl Pts',(50.8242806369343,-55.0635339542666,
-60.5758307565185));
#178595=CARTESIAN_POINT('Ctrl Pts',(50.8291488883492,-55.0633234186072,
-60.5738295347324));
#178596=CARTESIAN_POINT('Ctrl Pts',(50.8621978557542,-55.0618941608409,
-60.5602438942337));
#178597=CARTESIAN_POINT('Ctrl Pts',(50.8937577303036,-55.0605292840505,
-60.5452002171636));
#178598=CARTESIAN_POINT('Ctrl Pts',(50.9237804823248,-55.0592308752312,
-60.5290286719171));
#178599=CARTESIAN_POINT('Ctrl Pts',(50.9524579513628,-55.057990646531,-60.5135817539338));
#178600=CARTESIAN_POINT('Ctrl Pts',(50.9797334822037,-55.0568110401798,
-60.4971053444489));
#178601=CARTESIAN_POINT('Ctrl Pts',(51.00559583825,-55.0556925505231,-60.479855117644));
#178602=CARTESIAN_POINT('Ctrl Pts',(51.034637597282,-55.0544365587244,-60.4604842247053));
#178603=CARTESIAN_POINT('Ctrl Pts',(51.0618981348816,-55.0532576008103,
-60.4401373914491));
#178604=CARTESIAN_POINT('Ctrl Pts',(51.08740091482,-55.0521546620244,-60.4191325982561));
#178605=CARTESIAN_POINT('Ctrl Pts',(51.0993901420219,-55.0516361544843,
-60.4092579399431));
#178606=CARTESIAN_POINT('Ctrl Pts',(51.1109913826958,-55.0511344265027,
-60.3992372751482));
#178607=CARTESIAN_POINT('Ctrl Pts',(51.1222095012985,-55.0506492677027,
-60.3891007231335));
#178608=CARTESIAN_POINT('Ctrl Pts',(51.1276500479029,-55.0504139761039,
-60.3841847130967));
#178609=CARTESIAN_POINT('Ctrl Pts',(51.1326801607925,-55.0501964348529,
-60.3795368119712));
#178610=CARTESIAN_POINT('Ctrl Pts',(51.1377531641319,-55.049977032032,-60.3747537950781));
#178611=CARTESIAN_POINT('Ctrl Pts',(51.1426753735635,-55.0497641509116,
-60.3701129523094));
#178612=CARTESIAN_POINT('Ctrl Pts',(51.1476381129635,-55.0495495106959,
-60.3653448275671));
#178613=CARTESIAN_POINT('Ctrl Pts',(51.1530224316603,-55.0493166257935,
-60.3600469446924));
#178614=CARTESIAN_POINT('Ctrl Pts',(51.1540160724075,-55.0492736484102,
-60.35906925511));
#178615=CARTESIAN_POINT('Ctrl Pts',(51.155023969336,-55.0492300540593,-60.3580734250976));
#178616=CARTESIAN_POINT('Ctrl Pts',(51.1560483702627,-55.0491857454898,
-60.3570567840803));
#178617=CARTESIAN_POINT('Ctrl Pts',(51.1901033100392,-55.047712761985,-60.3232598128792));
#178618=CARTESIAN_POINT('Ctrl Pts',(51.2213719515089,-55.0463604151168,
-60.2873222686653));
#178619=CARTESIAN_POINT('Ctrl Pts',(51.2497281199733,-55.0451340889359,
-60.2497596531771));
#178620=CARTESIAN_POINT('Ctrl Pts',(51.2785117986632,-55.0438892741154,
-60.2116307269678));
#178621=CARTESIAN_POINT('Ctrl Pts',(51.3042945550902,-55.0427743071565,
-60.1718273266932));
#178622=CARTESIAN_POINT('Ctrl Pts',(51.3269711323931,-55.0417936659585,
-60.1308415655649));
#178623=CARTESIAN_POINT('Ctrl Pts',(51.3447218971007,-55.0410260399215,
-60.0987587431693));
#178624=CARTESIAN_POINT('Ctrl Pts',(51.360569916253,-55.0403406975752,-60.0659504756251));
#178625=CARTESIAN_POINT('Ctrl Pts',(51.3744756167235,-55.0397393152828,
-60.0326334324049));
#178626=CARTESIAN_POINT('Ctrl Pts',(51.375857460983,-55.0396795544193,-60.0293226344328));
#178627=CARTESIAN_POINT('Ctrl Pts',(51.3772201029237,-55.0396206236095,
-60.0260068878549));
#178628=CARTESIAN_POINT('Ctrl Pts',(51.3785635834251,-55.0395625210514,
-60.0226864252214));
#178629=CARTESIAN_POINT('Ctrl Pts',(51.3961159803762,-55.0388034187329,
-59.9793050154134));
#178630=CARTESIAN_POINT('Ctrl Pts',(51.4103970516706,-55.0381857940084,
-59.9351228143234));
#178631=CARTESIAN_POINT('Ctrl Pts',(51.4215008278151,-55.0377055802667,
-59.8906338472908));
#178632=CARTESIAN_POINT('Ctrl Pts',(51.4327391040554,-55.0372195496935,
-59.8456059851787));
#178633=CARTESIAN_POINT('Ctrl Pts',(51.440722662487,-55.0368742784617,-59.8002638479446));
#178634=CARTESIAN_POINT('Ctrl Pts',(51.4455573094817,-55.0366651906799,
-59.7550665530516));
#178635=CARTESIAN_POINT('Ctrl Pts',(51.4493215654944,-55.0365023949389,
-59.7198759405322));
#178636=CARTESIAN_POINT('Ctrl Pts',(51.4511770665258,-55.0364221486262,
-59.684772050632));
#178637=CARTESIAN_POINT('Ctrl Pts',(51.4511770665258,-55.0364221486262,
-59.64995));
#178638=CARTESIAN_POINT('Origin',(-83.2809572255632,-38.28000002,-55.2499500000007));
#178639=CARTESIAN_POINT('',(53.3753396310439,-38.28000002,-55.74995));
#178640=CARTESIAN_POINT('',(-83.2809572255632,-38.28000002,-55.74995));
#178641=CARTESIAN_POINT('',(53.3753396310439,-38.28000002,-60.0032396521563));
#178642=CARTESIAN_POINT('',(53.3753396310439,-38.28000002,-55.2499500000007));
#178643=CARTESIAN_POINT('Ctrl Pts',(53.3753396310439,-38.28000002,-60.0032396521563));
#178644=CARTESIAN_POINT('Ctrl Pts',(53.3753396310439,-38.28000002,-60.0589758767835));
#178645=CARTESIAN_POINT('Ctrl Pts',(53.3722852139107,-38.28000002,-60.1146939077158));
#178646=CARTESIAN_POINT('Ctrl Pts',(53.3663204826485,-38.28000002,-60.1700562792009));
#178647=CARTESIAN_POINT('Ctrl Pts',(53.3600346473474,-38.28000002,-60.2283990164902));
#178648=CARTESIAN_POINT('Ctrl Pts',(53.3505169273234,-38.28000002,-60.2863478004803));
#178649=CARTESIAN_POINT('Ctrl Pts',(53.3378827651207,-38.28000002,-60.3435292248106));
#178650=CARTESIAN_POINT('Ctrl Pts',(53.3251015247972,-38.28000002,-60.4013763154743));
#178651=CARTESIAN_POINT('Ctrl Pts',(53.3091307297629,-38.28000002,-60.4584393902281));
#178652=CARTESIAN_POINT('Ctrl Pts',(53.2900367865637,-38.2800000200001,
-60.5143350099522));
#178653=CARTESIAN_POINT('Ctrl Pts',(53.2713085336432,-38.2800000200001,
-60.5691601077554));
#178654=CARTESIAN_POINT('Ctrl Pts',(53.2495752764747,-38.2800000200002,
-60.622863235497));
#178655=CARTESIAN_POINT('Ctrl Pts',(53.2248527900283,-38.2800000200003,
-60.6750669890669));
#178656=CARTESIAN_POINT('Ctrl Pts',(53.2194501346315,-38.2800000200003,
-60.6864751818298));
#178657=CARTESIAN_POINT('Ctrl Pts',(53.2139045547126,-38.2800000200004,
-60.6978116715984));
#178658=CARTESIAN_POINT('Ctrl Pts',(53.2082159323664,-38.2800000200004,
-60.7090723322489));
#178659=CARTESIAN_POINT('Ctrl Pts',(53.2081854825349,-38.2800000200004,
-60.7091326078656));
#178660=CARTESIAN_POINT('Ctrl Pts',(53.2081550286956,-38.2800000200004,
-60.7091928811299));
#178661=CARTESIAN_POINT('Ctrl Pts',(53.2081245708486,-38.2800000200004,
-60.709253152041));
#178662=CARTESIAN_POINT('Ctrl Pts',(53.1761754390121,-38.2800000200006,
-60.7724750628697));
#178663=CARTESIAN_POINT('Ctrl Pts',(53.1397892479682,-38.2800000200007,
-60.8333871332408));
#178664=CARTESIAN_POINT('Ctrl Pts',(53.0993211720577,-38.2800000200006,
-60.8914909948819));
#178665=CARTESIAN_POINT('Ctrl Pts',(53.0593989894052,-38.2800000200005,
-60.9488110657047));
#178666=CARTESIAN_POINT('Ctrl Pts',(53.0155035526426,-38.2800000200003,
-61.0033990731716));
#178667=CARTESIAN_POINT('Ctrl Pts',(52.9679386190623,-38.2800000200002,
-61.0547432417683));
#178668=CARTESIAN_POINT('Ctrl Pts',(52.9223553337127,-38.2800000200001,
-61.1039483118066));
#178669=CARTESIAN_POINT('Ctrl Pts',(52.8734012103226,-38.28000002,-61.1501747492908));
#178670=CARTESIAN_POINT('Ctrl Pts',(52.8213200539949,-38.28000002,-61.192931263928));
#178671=CARTESIAN_POINT('Ctrl Pts',(52.7942271507165,-38.28000002,-61.215173437437));
#178672=CARTESIAN_POINT('Ctrl Pts',(52.7662877001539,-38.28000002,-61.2364758695291));
#178673=CARTESIAN_POINT('Ctrl Pts',(52.7375342894721,-38.28000002,-61.2567639997892));
#178674=CARTESIAN_POINT('Ctrl Pts',(53.3753396310439,-38.28000002,-60.0032396521563));
#178675=CARTESIAN_POINT('Ctrl Pts',(52.9171740440352,-38.28000002,-60.0032396521562));
#178676=CARTESIAN_POINT('Ctrl Pts',(52.877242281998,-38.7364221486262,-60.0032396521562));
#178677=CARTESIAN_POINT('Ctrl Pts',(53.3753396328414,-38.28000002,-60.244893556147));
#178678=CARTESIAN_POINT('Ctrl Pts',(52.9343465054118,-38.28000002,-60.1721379135101));
#178679=CARTESIAN_POINT('Ctrl Pts',(52.8788986395818,-38.7174898948119,
-60.1690974501184));
#178680=CARTESIAN_POINT('Ctrl Pts',(53.317850201657,-38.28000002,-60.4921247747839));
#178681=CARTESIAN_POINT('Ctrl Pts',(52.9111776732915,-38.28000002,-60.3567456822519));
#178682=CARTESIAN_POINT('Ctrl Pts',(52.8422535332614,-38.6982739394415,
-60.3389622441799));
#178683=CARTESIAN_POINT('Ctrl Pts',(53.0984000724383,-38.28000002,-60.9263821015509));
#178684=CARTESIAN_POINT('Ctrl Pts',(52.7751833670329,-38.28000002,-60.6874729542071));
#178685=CARTESIAN_POINT('Ctrl Pts',(52.6988044737759,-38.6656865171052,
-60.6372698562504));
#178686=CARTESIAN_POINT('Ctrl Pts',(52.9360725977236,-38.28000002,-61.1166772774171));
#178687=CARTESIAN_POINT('Ctrl Pts',(52.6635868839933,-38.28000002,-60.8378349680257));
#178688=CARTESIAN_POINT('Ctrl Pts',(52.5917711956707,-38.6521075044106,
-60.7679496692827));
#178689=CARTESIAN_POINT('Ctrl Pts',(52.7375342894721,-38.28000002,-61.2567639997892));
#178690=CARTESIAN_POINT('Ctrl Pts',(52.5193575501106,-38.28000002,-60.9475523661896));
#178691=CARTESIAN_POINT('Ctrl Pts',(52.4601060488526,-38.6442121687577,
-60.8635779995784));
#178692=CARTESIAN_POINT('',(52.8772422786263,-38.736422148331,-60.0032396521556));
#178693=CARTESIAN_POINT('Origin',(53.3753396310439,-38.78000002,-60.0032396521563));
#178694=CARTESIAN_POINT('Ctrl Pts',(52.4601061816814,-38.6442121767227,
-60.8635779031049));
#178695=CARTESIAN_POINT('Ctrl Pts',(52.4857623597633,-38.6457506363329,
-60.8449438340698));
#178696=CARTESIAN_POINT('Ctrl Pts',(52.5112243232531,-38.6475495400589,
-60.8244412198977));
#178697=CARTESIAN_POINT('Ctrl Pts',(52.536247504591,-38.6496228467422,-60.8019625565231));
#178698=CARTESIAN_POINT('Ctrl Pts',(52.5601660855939,-38.6516046312794,
-60.7804761706195));
#178699=CARTESIAN_POINT('Ctrl Pts',(52.5836838164615,-38.6538371698229,
-60.7571840989168));
#178700=CARTESIAN_POINT('Ctrl Pts',(52.6065464778335,-38.6563279032125,
-60.732017239825));
#178701=CARTESIAN_POINT('Ctrl Pts',(52.6142960302199,-38.6571721648918,
-60.7234866540913));
#178702=CARTESIAN_POINT('Ctrl Pts',(52.6219699584021,-38.6580460472365,
-60.714740899271));
#178703=CARTESIAN_POINT('Ctrl Pts',(52.6295572148155,-38.6589496944378,
-60.7057780511307));
#178704=CARTESIAN_POINT('Ctrl Pts',(52.6511165291618,-38.6615174228776,
-60.6803099701844));
#178705=CARTESIAN_POINT('Ctrl Pts',(52.6719774600956,-38.6643258339855,
-60.6530877674629));
#178706=CARTESIAN_POINT('Ctrl Pts',(52.6918501867659,-38.6673726516042,
-60.6241039054663));
#178707=CARTESIAN_POINT('Ctrl Pts',(52.7094328672616,-38.6700683672755,
-60.5984600170623));
#178708=CARTESIAN_POINT('Ctrl Pts',(52.7262421963706,-38.6729508212541,
-60.5714358630291));
#178709=CARTESIAN_POINT('Ctrl Pts',(52.7420475179718,-38.6760127168085,
-60.5430616037942));
#178710=CARTESIAN_POINT('Ctrl Pts',(52.7498509593379,-38.6775244432403,
-60.5290525963326));
#178711=CARTESIAN_POINT('Ctrl Pts',(52.7574093262473,-38.6790798381767,
-60.5147148820475));
#178712=CARTESIAN_POINT('Ctrl Pts',(52.7646922891108,-38.6806773954924,
-60.500056191524));
#178713=CARTESIAN_POINT('Ctrl Pts',(52.7663755524841,-38.6810466284222,
-60.4966682246594));
#178714=CARTESIAN_POINT('Ctrl Pts',(52.7683001317608,-38.6814754219272,
-60.4927379935618));
#178715=CARTESIAN_POINT('Ctrl Pts',(52.7699624760655,-38.6818517038284,
-60.4892922803886));
#178716=CARTESIAN_POINT('Ctrl Pts',(52.7701550375918,-38.6818952913193,
-60.4888931381737));
#178717=CARTESIAN_POINT('Ctrl Pts',(52.770344131837,-38.6819381701835,-60.4885005245996));
#178718=CARTESIAN_POINT('Ctrl Pts',(52.7705290151266,-38.6819801632172,
-60.4881160560812));
#178719=CARTESIAN_POINT('Ctrl Pts',(52.7711948210125,-38.6821313894804,
-60.4867314993527));
#178720=CARTESIAN_POINT('Ctrl Pts',(52.7718059718363,-38.6822711505817,
-60.4854523452323));
#178721=CARTESIAN_POINT('Ctrl Pts',(52.772328349338,-38.6823911134328,-60.4843545222568));
#178722=CARTESIAN_POINT('Ctrl Pts',(52.7827597911478,-38.6847866712374,
-60.462431915619));
#178723=CARTESIAN_POINT('Ctrl Pts',(52.7929574618894,-38.6873654107239,
-60.4389746467284));
#178724=CARTESIAN_POINT('Ctrl Pts',(52.802672590598,-38.6901321259938,-60.4139448759755));
#178725=CARTESIAN_POINT('Ctrl Pts',(52.8072602409309,-38.6914386163769,
-60.4021253891141));
#178726=CARTESIAN_POINT('Ctrl Pts',(52.8117398566731,-38.6927869530701,
-60.3899557998885));
#178727=CARTESIAN_POINT('Ctrl Pts',(52.816082856994,-38.6941772106881,-60.3774354714578));
#178728=CARTESIAN_POINT('Ctrl Pts',(52.8228528775337,-38.696344392805,-60.3579183463419));
#178729=CARTESIAN_POINT('Ctrl Pts',(52.8292924909856,-38.6986064410768,
-60.3375485860623));
#178730=CARTESIAN_POINT('Ctrl Pts',(52.8352842226712,-38.7009701754622,
-60.3163362365538));
#178731=CARTESIAN_POINT('Ctrl Pts',(52.838280088514,-38.7021520426549,-60.3057300617996));
#178732=CARTESIAN_POINT('Ctrl Pts',(52.8411638244454,-38.7033593973482,
-60.2949134970024));
#178733=CARTESIAN_POINT('Ctrl Pts',(52.8439198470878,-38.704593041393,-60.2838895088064));
#178734=CARTESIAN_POINT('Ctrl Pts',(52.845297858409,-38.7052098634154,-60.2783775147083));
#178735=CARTESIAN_POINT('Ctrl Pts',(52.8466439377268,-38.7058332566417,
-60.2728136617708));
#178736=CARTESIAN_POINT('Ctrl Pts',(52.8479560679907,-38.7064633552259,
-60.2671984626355));
#178737=CARTESIAN_POINT('Ctrl Pts',(52.8486121331227,-38.706778404518,-60.2643908630679));
#178738=CARTESIAN_POINT('Ctrl Pts',(52.8492597107986,-38.7070951300932,
-60.2615704268027));
#178739=CARTESIAN_POINT('Ctrl Pts',(52.8498985461022,-38.7074135496482,
-60.2587372223283));
#178740=CARTESIAN_POINT('Ctrl Pts',(52.8503738360279,-38.7076504520326,
-60.2566293338998));
#178741=CARTESIAN_POINT('Ctrl Pts',(52.8510433499346,-38.7079898874832,
-60.2536116819445));
#178742=CARTESIAN_POINT('Ctrl Pts',(52.8514616955767,-38.7082051395534,
-60.2516988745454));
#178743=CARTESIAN_POINT('Ctrl Pts',(52.8516056466525,-38.7082792069368,
-60.2510406851077));
#178744=CARTESIAN_POINT('Ctrl Pts',(52.8517203364549,-38.7083385534396,
-60.2505134212631));
#178745=CARTESIAN_POINT('Ctrl Pts',(52.8517885682409,-38.7083739084269,
-60.2501993750543));
#178746=CARTESIAN_POINT('Ctrl Pts',(52.8535288336456,-38.7092756444794,
-60.2421895634358));
#178747=CARTESIAN_POINT('Ctrl Pts',(52.8555656110489,-38.7103785356354,
-60.2324101905088));
#178748=CARTESIAN_POINT('Ctrl Pts',(52.8577577286042,-38.7116860742924,
-60.2208374968453));
#178749=CARTESIAN_POINT('Ctrl Pts',(52.8598955118563,-38.7129612040115,
-60.2095516464875));
#178750=CARTESIAN_POINT('Ctrl Pts',(52.8621809224268,-38.7144310546655,
-60.1965595734014));
#178751=CARTESIAN_POINT('Ctrl Pts',(52.8644347882344,-38.716098386014,-60.181845184474));
#178752=CARTESIAN_POINT('Ctrl Pts',(52.8666240780138,-38.7177179462679,
-60.1675523808925));
#178753=CARTESIAN_POINT('Ctrl Pts',(52.8687834948402,-38.7195239308079,
-60.151633801452));
#178754=CARTESIAN_POINT('Ctrl Pts',(52.8707043558886,-38.7215170266781,
-60.1340908447902));
#178755=CARTESIAN_POINT('Ctrl Pts',(52.8725619015244,-38.7234444261319,
-60.1171261389815));
#178756=CARTESIAN_POINT('Ctrl Pts',(52.8741962415673,-38.7255468982893,
-60.0986416700889));
#178757=CARTESIAN_POINT('Ctrl Pts',(52.8753781352092,-38.7278219393132,
-60.0786644558131));
#178758=CARTESIAN_POINT('Ctrl Pts',(52.8765007676189,-38.7299829076919,
-60.0596889173987));
#178759=CARTESIAN_POINT('Ctrl Pts',(52.8772149880542,-38.7322996416788,
-60.0393660615517));
#178760=CARTESIAN_POINT('Ctrl Pts',(52.877289594721,-38.7347659988467,-60.017751191729));
#178761=CARTESIAN_POINT('Ctrl Pts',(52.877306074807,-38.7353107997344,-60.0129766195702));
#178762=CARTESIAN_POINT('Ctrl Pts',(52.8772912114132,-38.7358628828515,
-60.0081391524345));
#178763=CARTESIAN_POINT('Ctrl Pts',(52.877242281998,-38.7364221486262,-60.0032396521562));
#178764=CARTESIAN_POINT('Origin',(0.,-12.9675000200281,-61.64995));
#178765=CARTESIAN_POINT('Ctrl Pts',(52.4601060654288,-38.6442120952127,
-60.8635774537264));
#178766=CARTESIAN_POINT('Ctrl Pts',(52.4334660241228,-38.7417025272771,
-60.8486996970615));
#178767=CARTESIAN_POINT('Ctrl Pts',(52.4037146585348,-38.8501763362785,
-60.8330778025515));
#178768=CARTESIAN_POINT('Ctrl Pts',(52.3707417991334,-38.9697354911175,
-60.8172970455499));
#178769=CARTESIAN_POINT('Ctrl Pts',(52.3399184262437,-39.0815006361153,
-60.8025450293045));
#178770=CARTESIAN_POINT('Ctrl Pts',(52.3062790584938,-39.2029553301362,
-60.7876567855608));
#178771=CARTESIAN_POINT('Ctrl Pts',(52.2697265354297,-39.3341621392828,
-60.7731334311792));
#178772=CARTESIAN_POINT('Ctrl Pts',(52.2381281819637,-39.447585749612,-60.7605785089251));
#178773=CARTESIAN_POINT('Ctrl Pts',(52.2043536425209,-39.5682934199092,
-60.7482981832768));
#178774=CARTESIAN_POINT('Ctrl Pts',(52.1683406202579,-39.696297737098,-60.7366073261809));
#178775=CARTESIAN_POINT('Ctrl Pts',(52.1503341091263,-39.7602998956925,
-60.7307618976329));
#178776=CARTESIAN_POINT('Ctrl Pts',(52.1317679882644,-39.8261258047343,
-60.725063559064));
#178777=CARTESIAN_POINT('Ctrl Pts',(52.1126344252469,-39.8937749956445,
-60.7195489815034));
#178778=CARTESIAN_POINT('Ctrl Pts',(52.1030676437381,-39.9275995910996,
-60.7167916927231));
#178779=CARTESIAN_POINT('Ctrl Pts',(52.0933589949976,-39.9618800079525,
-60.7140803064361));
#178780=CARTESIAN_POINT('Ctrl Pts',(52.0835075034003,-39.9966160398341,
-60.71141916003));
#178781=CARTESIAN_POINT('Ctrl Pts',(52.0785817576016,-40.0139840557749,
-60.7100885868269));
#178782=CARTESIAN_POINT('Ctrl Pts',(52.0736203003513,-40.0314659766725,
-60.7087705705402));
#178783=CARTESIAN_POINT('Ctrl Pts',(52.0686230077915,-40.0490617750148,
-60.7074656347461));
#178784=CARTESIAN_POINT('Ctrl Pts',(52.0661243615116,-40.057859674186,-60.7068131668491));
#178785=CARTESIAN_POINT('Ctrl Pts',(52.063616756388,-40.066686042688,-60.7061639688745));
#178786=CARTESIAN_POINT('Ctrl Pts',(52.0611001768525,-40.0755408768569,
-60.7055181050371));
#178787=CARTESIAN_POINT('Ctrl Pts',(52.0598418870847,-40.0799682939413,
-60.7051951731184));
#178788=CARTESIAN_POINT('Ctrl Pts',(52.0585813537179,-40.0844028274231,
-60.7048730747222));
#178789=CARTESIAN_POINT('Ctrl Pts',(52.0573185748043,-40.0888444768176,
-60.7045518177966));
#178790=CARTESIAN_POINT('Ctrl Pts',(52.0566871853474,-40.0910653015148,
-60.7043911893338));
#178791=CARTESIAN_POINT('Ctrl Pts',(52.056055234504,-40.0932879051895,-60.7042307712378));
#178792=CARTESIAN_POINT('Ctrl Pts',(52.055422722031,-40.0955122877773,-60.7040705644974));
#178793=CARTESIAN_POINT('Ctrl Pts',(52.0552260978451,-40.0962037641259,
-60.704020762286));
#178794=CARTESIAN_POINT('Ctrl Pts',(52.0550308665119,-40.096890323743,-60.7039713460818));
#178795=CARTESIAN_POINT('Ctrl Pts',(52.0548288548571,-40.0976007072079,
-60.7039202499623));
#178796=CARTESIAN_POINT('Ctrl Pts',(52.0543810233055,-40.0991755278765,
-60.7038069770203));
#178797=CARTESIAN_POINT('Ctrl Pts',(52.0539081791715,-40.1008382038806,
-60.7036875622797));
#178798=CARTESIAN_POINT('Ctrl Pts',(52.0534391812185,-40.1024872442081,
-60.7035693190069));
#178799=CARTESIAN_POINT('Ctrl Pts',(52.0526842447014,-40.1051416710633,
-60.7033789852027));
#178800=CARTESIAN_POINT('Ctrl Pts',(52.0519392685549,-40.1077607713129,
-60.7031917274615));
#178801=CARTESIAN_POINT('Ctrl Pts',(52.051324697943,-40.1099212352922,-60.7030375666888));
#178802=CARTESIAN_POINT('Ctrl Pts',(52.0511862974551,-40.1104077689191,
-60.703002849887));
#178803=CARTESIAN_POINT('Ctrl Pts',(52.0510545107586,-40.1108710430068,
-60.7029698095072));
#178804=CARTESIAN_POINT('Ctrl Pts',(52.0509307139482,-40.111306222927,-60.702938785362));
#178805=CARTESIAN_POINT('Ctrl Pts',(52.0508514050645,-40.111585015519,-60.7029189101301));
#178806=CARTESIAN_POINT('Ctrl Pts',(52.0507732062307,-40.1118599029495,
-60.702899318697));
#178807=CARTESIAN_POINT('Ctrl Pts',(52.0506944905704,-40.1121366041439,
-60.7028796033477));
#178808=CARTESIAN_POINT('Ctrl Pts',(52.0057005426572,-40.2702992757785,
-60.6916102905366));
#178809=CARTESIAN_POINT('Ctrl Pts',(51.9602026002465,-40.4292425721673,
-60.6820510418657));
#178810=CARTESIAN_POINT('Ctrl Pts',(51.9143651206563,-40.588388068656,-60.6743068341458));
#178811=CARTESIAN_POINT('Ctrl Pts',(51.8690090901036,-40.7458619975366,
-60.666643966879));
#178812=CARTESIAN_POINT('Ctrl Pts',(51.8233206500267,-40.9035338860859,
-60.6607583289389));
#178813=CARTESIAN_POINT('Ctrl Pts',(51.7774673696501,-41.0608420505297,
-60.6567013858634));
#178814=CARTESIAN_POINT('Ctrl Pts',(51.7320461923718,-41.2166678053247,
-60.6526826738078));
#178815=CARTESIAN_POINT('Ctrl Pts',(51.6864633051644,-41.3721366436965,
-60.6504584078783));
#178816=CARTESIAN_POINT('Ctrl Pts',(51.6408891881858,-41.5267015602231,
-60.6500277777421));
#178817=CARTESIAN_POINT('Ctrl Pts',(51.6353998048932,-41.5453188396495,
-60.6499759085227));
#178818=CARTESIAN_POINT('Ctrl Pts',(51.6299105575627,-41.5639230037829,
-60.64995));
#178819=CARTESIAN_POINT('Ctrl Pts',(51.6244217512083,-41.5825130958571,
-60.64995));
#178820=CARTESIAN_POINT('Origin',(-83.2809572255632,20.2699999800001,-55.24995));
#178821=CARTESIAN_POINT('',(52.6819919725962,20.26999998,-59.64995));
#178822=CARTESIAN_POINT('Ctrl Pts',(51.1762622162812,20.26999998,-61.14995));
#178823=CARTESIAN_POINT('Ctrl Pts',(51.3733973069281,20.26999998,-61.149949999985));
#178824=CARTESIAN_POINT('Ctrl Pts',(51.5703838078145,20.26999998,-61.1109090094727));
#178825=CARTESIAN_POINT('Ctrl Pts',(51.9345762874696,20.26999998,-60.9606295880612));
#178826=CARTESIAN_POINT('Ctrl Pts',(52.1016035094776,20.26999998,-60.849450253352));
#178827=CARTESIAN_POINT('Ctrl Pts',(52.3803443657342,20.26999998,-60.5717700902076));
#178828=CARTESIAN_POINT('Ctrl Pts',(52.4919483874702,20.26999998,-60.4053784571342));
#178829=CARTESIAN_POINT('Ctrl Pts',(52.6428018517975,20.26999998,-60.0425718399611));
#178830=CARTESIAN_POINT('Ctrl Pts',(52.6819919725819,20.26999998,-59.8463349320562));
#178831=CARTESIAN_POINT('Ctrl Pts',(52.6819919725962,20.26999998,-59.64995));
#178832=CARTESIAN_POINT('',(52.6819919725962,20.26999998,-55.74995));
#178833=CARTESIAN_POINT('',(52.6819919725962,20.26999998,-55.24995));
#178834=CARTESIAN_POINT('',(-83.2809572255632,20.2699999800001,-55.74995));
#178835=CARTESIAN_POINT('Origin',(-83.2809572255632,19.7699999800001,-55.74995));
#178836=CARTESIAN_POINT('',(52.7694806361221,19.76999998,-55.24995));
#178837=CARTESIAN_POINT('Ctrl Pts',(52.6819919725962,20.26999998,-55.74995));
#178838=CARTESIAN_POINT('Ctrl Pts',(52.6819919725961,20.26999998,-55.7240510278288));
#178839=CARTESIAN_POINT('Ctrl Pts',(52.6823594164764,20.2679000286179,-55.6978536074428));
#178840=CARTESIAN_POINT('Ctrl Pts',(52.6831016080547,20.2636583843413,-55.6716786004096));
#178841=CARTESIAN_POINT('Ctrl Pts',(52.68385006805,20.2593809158985,-55.645282523965));
#178842=CARTESIAN_POINT('Ctrl Pts',(52.6849796405233,20.2529253796767,-55.6189093033866));
#178843=CARTESIAN_POINT('Ctrl Pts',(52.68649281381,20.2442775547729,-55.5929324719567));
#178844=CARTESIAN_POINT('Ctrl Pts',(52.6870630090585,20.2410188740165,-55.5831438601805));
#178845=CARTESIAN_POINT('Ctrl Pts',(52.6876876222624,20.2374491932217,-55.5734119766137));
#178846=CARTESIAN_POINT('Ctrl Pts',(52.6883666017139,20.2335688078992,-55.5637583894405));
#178847=CARTESIAN_POINT('Ctrl Pts',(52.6901453360981,20.223403294376,-55.5384687177195));
#178848=CARTESIAN_POINT('Ctrl Pts',(52.692298393295,20.2110985161876,-55.513697484835));
#178849=CARTESIAN_POINT('Ctrl Pts',(52.6948256939525,20.1966549268352,-55.4898442374517));
#178850=CARTESIAN_POINT('Ctrl Pts',(52.6968758230015,20.1849383857046,-55.4704946459309));
#178851=CARTESIAN_POINT('Ctrl Pts',(52.6991724966386,20.1718128358059,-55.4517483678047));
#178852=CARTESIAN_POINT('Ctrl Pts',(52.7017125466146,20.1572963837663,-55.4338552809257));
#178853=CARTESIAN_POINT('Ctrl Pts',(52.7030843359257,20.1494565719781,-55.4241918705375));
#178854=CARTESIAN_POINT('Ctrl Pts',(52.704527066812,20.1412113272328,-55.4147778017497));
#178855=CARTESIAN_POINT('Ctrl Pts',(52.7060394414411,20.132568066677,-55.4056571306897));
#178856=CARTESIAN_POINT('Ctrl Pts',(52.7063406725299,20.1308465231268,-55.40384049768));
#178857=CARTESIAN_POINT('Ctrl Pts',(52.7067076790132,20.1287490714839,-55.4016626948181));
#178858=CARTESIAN_POINT('Ctrl Pts',(52.7070309911037,20.1269013041925,-55.3997779182201));
#178859=CARTESIAN_POINT('Ctrl Pts',(52.7072632840316,20.1255737223088,-55.398423745929));
#178860=CARTESIAN_POINT('Ctrl Pts',(52.7074727865942,20.1243763723405,-55.3972196111485));
#178861=CARTESIAN_POINT('Ctrl Pts',(52.7076167822125,20.1235533694274,-55.3963966082408));
#178862=CARTESIAN_POINT('Ctrl Pts',(52.7093254930192,20.1137872807912,-55.386630519669));
#178863=CARTESIAN_POINT('Ctrl Pts',(52.7112328483416,20.1028864179031,-55.3765717208586));
#178864=CARTESIAN_POINT('Ctrl Pts',(52.7133612017114,20.0907228045942,-55.3664552895126));
#178865=CARTESIAN_POINT('Ctrl Pts',(52.7153992958998,20.0790750256366,-55.3567678756524));
#178866=CARTESIAN_POINT('Ctrl Pts',(52.7176401664676,20.0662686121309,-55.3470275906972));
#178867=CARTESIAN_POINT('Ctrl Pts',(52.7200994879389,20.0522137836287,-55.3374815440121));
#178868=CARTESIAN_POINT('Ctrl Pts',(52.7224186275942,20.0389600831638,-55.3284796238985));
#178869=CARTESIAN_POINT('Ctrl Pts',(52.7249321027178,20.0245957839257,-55.3196505221431));
#178870=CARTESIAN_POINT('Ctrl Pts',(52.7276480673089,20.0090741146608,-55.3112377697569));
#178871=CARTESIAN_POINT('Ctrl Pts',(52.7287440891335,20.0028103775254,-55.3078428211445));
#178872=CARTESIAN_POINT('Ctrl Pts',(52.729873021253,19.9963585347733,-55.3045160977521));
#178873=CARTESIAN_POINT('Ctrl Pts',(52.7310351059163,19.9897171905324,-55.3012753797748));
#178874=CARTESIAN_POINT('Ctrl Pts',(52.7337031803283,19.9744690754941,-55.2938348920163));
#178875=CARTESIAN_POINT('Ctrl Pts',(52.7365482385913,19.9582094931193,-55.2868407235455));
#178876=CARTESIAN_POINT('Ctrl Pts',(52.7395689469865,19.9409460656444,-55.2805340045048));
#178877=CARTESIAN_POINT('Ctrl Pts',(52.7425051677173,19.9241654873818,-55.2744036811611));
#178878=CARTESIAN_POINT('Ctrl Pts',(52.7456074052925,19.9064361185113,-55.2689228588975));
#178879=CARTESIAN_POINT('Ctrl Pts',(52.7488680753396,19.8878013039202,-55.2643427579722));
#178880=CARTESIAN_POINT('Ctrl Pts',(52.7520256709167,19.8697555626212,-55.2599074406248));
#178881=CARTESIAN_POINT('Ctrl Pts',(52.7553318801676,19.8508604902903,-55.2563167977791));
#178882=CARTESIAN_POINT('Ctrl Pts',(52.7587730939723,19.8311938634032,-55.2538274761936));
#178883=CARTESIAN_POINT('Ctrl Pts',(52.7622143077771,19.8115272365161,-55.2513381546082));
#178884=CARTESIAN_POINT('Ctrl Pts',(52.7657906008408,19.7910886281323,-55.24995));
#178885=CARTESIAN_POINT('Ctrl Pts',(52.7694806361221,19.76999998,-55.24995));
#178886=CARTESIAN_POINT('',(60.,19.76999998,-55.24995));
#178887=CARTESIAN_POINT('Origin',(60.,28.41999998,-55.24995));
#178888=CARTESIAN_POINT('',(52.8132249678851,19.26999998,-55.24995));
#178889=CARTESIAN_POINT('',(52.0733761857257,27.7265102562164,-55.24995));
#178890=CARTESIAN_POINT('',(60.,19.26999998,-55.24995));
#178891=CARTESIAN_POINT('Origin',(60.,19.26999998,-55.74995));
#178892=CARTESIAN_POINT('',(52.900713631411,18.76999998,-55.74995));
#178893=CARTESIAN_POINT('Ctrl Pts',(52.8132249678851,19.26999998,-55.24995));
#178894=CARTESIAN_POINT('Ctrl Pts',(52.8170018622036,19.2484149301986,-55.24995));
#178895=CARTESIAN_POINT('Ctrl Pts',(52.820628852166,19.2274879325962,-55.2513479743294));
#178896=CARTESIAN_POINT('Ctrl Pts',(52.8241059377721,19.2073682602054,-55.2538882420751));
#178897=CARTESIAN_POINT('Ctrl Pts',(52.8275775058576,19.1872805141808,-55.2564244788646));
#178898=CARTESIAN_POINT('Ctrl Pts',(52.8308996449529,19.167996955483,-55.2600986723954));
#178899=CARTESIAN_POINT('Ctrl Pts',(52.834072355058,19.1496086400557,-55.2646604727419));
#178900=CARTESIAN_POINT('Ctrl Pts',(52.8373840007711,19.1304150850388,-55.2694220381106));
#178901=CARTESIAN_POINT('Ctrl Pts',(52.8405328437045,19.1121965820858,-55.2751499570336));
#178902=CARTESIAN_POINT('Ctrl Pts',(52.8435188838583,19.0950003125834,-55.2815750258563));
#178903=CARTESIAN_POINT('Ctrl Pts',(52.8462680137064,19.0791683828935,-55.2874903342807));
#178904=CARTESIAN_POINT('Ctrl Pts',(52.8488791492904,19.0642018444273,-55.2939965088991));
#178905=CARTESIAN_POINT('Ctrl Pts',(52.8513522906103,19.050102597673,-55.3009008476283));
#178906=CARTESIAN_POINT('Ctrl Pts',(52.854233915202,19.0336746095732,-55.3089455606869));
#178907=CARTESIAN_POINT('Ctrl Pts',(52.8569281965776,19.0184242891668,-55.3175297931872));
#178908=CARTESIAN_POINT('Ctrl Pts',(52.8594351347371,19.0043108258162,-55.3263826814435));
#178909=CARTESIAN_POINT('Ctrl Pts',(52.8614131894553,18.9931748499785,-55.3333678945884));
#178910=CARTESIAN_POINT('Ctrl Pts',(52.8632746095929,18.9827455690346,-55.3405210924567));
#178911=CARTESIAN_POINT('Ctrl Pts',(52.8650193951501,18.972987953445,-55.347726360613));
#178912=CARTESIAN_POINT('Ctrl Pts',(52.8669974371943,18.9619258640044,-55.3558948849884));
#178913=CARTESIAN_POINT('Ctrl Pts',(52.8688255748824,18.9517269109974,-55.36412990652));
#178914=CARTESIAN_POINT('Ctrl Pts',(52.8705038082142,18.9423264617821,-55.3722860416207));
#178915=CARTESIAN_POINT('Ctrl Pts',(52.8713429248801,18.9376262371744,-55.3763641091711));
#178916=CARTESIAN_POINT('Ctrl Pts',(52.872144565457,18.9331254533317,-55.3804228422457));
#178917=CARTESIAN_POINT('Ctrl Pts',(52.8729087299449,18.9288151725488,-55.3844463376867));
#178918=CARTESIAN_POINT('Ctrl Pts',(52.8732908121888,18.9266600321573,-55.3864580854071));
#178919=CARTESIAN_POINT('Ctrl Pts',(52.8736635254104,18.9245525258353,-55.3884610324748));
#178920=CARTESIAN_POINT('Ctrl Pts',(52.8740268696098,18.922491480226,-55.3904533482982));
#178921=CARTESIAN_POINT('Ctrl Pts',(52.8742524174911,18.921212074992,-55.3916900891451));
#178922=CARTESIAN_POINT('Ctrl Pts',(52.8744014321368,18.920371830749,-55.3925105847798));
#178923=CARTESIAN_POINT('Ctrl Pts',(52.8746097155931,18.9191841523716,-55.3936800811387));
#178924=CARTESIAN_POINT('Ctrl Pts',(52.874736964376,18.918458551641,-55.3943945737394));
#178925=CARTESIAN_POINT('Ctrl Pts',(52.8748863351359,18.9176035577891,-55.3952396410243));
#178926=CARTESIAN_POINT('Ctrl Pts',(52.8750887951412,18.9164465894067,-55.3963966094067));
#178927=CARTESIAN_POINT('Ctrl Pts',(52.8782312711263,18.8984887445873,-55.4143544542262));
#178928=CARTESIAN_POINT('Ctrl Pts',(52.8810847163286,18.8820748238315,-55.4335093827848));
#178929=CARTESIAN_POINT('Ctrl Pts',(52.883649130748,18.8673083263412,-55.4535728212673));
#178930=CARTESIAN_POINT('Ctrl Pts',(52.8862497990868,18.8523330703113,-55.4739199027816));
#178931=CARTESIAN_POINT('Ctrl Pts',(52.8885532066409,18.8390520083641,-55.4952007603898));
#178932=CARTESIAN_POINT('Ctrl Pts',(52.8905593534104,18.8275195753317,-55.5171172456793));
#178933=CARTESIAN_POINT('Ctrl Pts',(52.8926095204872,18.8157340894056,-55.539514638164));
#178934=CARTESIAN_POINT('Ctrl Pts',(52.8943492382359,18.8057746306867,-55.5625752640842));
#178935=CARTESIAN_POINT('Ctrl Pts',(52.8957785066566,18.7976461596386,-55.5859930898376));
#178936=CARTESIAN_POINT('Ctrl Pts',(52.8972258449116,18.7894149226424,-55.6097069805032));
#178937=CARTESIAN_POINT('Ctrl Pts',(52.8983548343716,18.783060901236,-55.6337866416403));
#178938=CARTESIAN_POINT('Ctrl Pts',(52.8991654750368,18.778539638464,-55.6579351495829));
#178939=CARTESIAN_POINT('Ctrl Pts',(52.8999913688049,18.7739333031199,-55.682538038477));
#178940=CARTESIAN_POINT('Ctrl Pts',(52.9004868208969,18.7712289400598,-55.7072119145565));
#178941=CARTESIAN_POINT('Ctrl Pts',(52.9006518313128,18.7703341785775,-55.7316719560988));
#178942=CARTESIAN_POINT('Ctrl Pts',(52.9006930313783,18.7701107730947,-55.7377791785246));
#178943=CARTESIAN_POINT('Ctrl Pts',(52.900713631411,18.76999998,-55.7438732289921));
#178944=CARTESIAN_POINT('Ctrl Pts',(52.900713631411,18.76999998,-55.74995));
#178945=CARTESIAN_POINT('',(-83.2809572255632,18.7699999800001,-55.74995));
#178946=CARTESIAN_POINT('Origin',(-83.2809572255632,18.7699999800001,-55.24995));
#178947=CARTESIAN_POINT('',(52.900713631411,18.76999998,-59.64995));
#178948=CARTESIAN_POINT('',(52.900713631411,18.76999998,-55.24995));
#178949=CARTESIAN_POINT('Ctrl Pts',(52.900713631411,18.76999998,-59.64995));
#178950=CARTESIAN_POINT('Ctrl Pts',(52.9007136313967,18.76999998,-59.8463349320561));
#178951=CARTESIAN_POINT('Ctrl Pts',(52.8615235106123,18.76999998,-60.0425718399612));
#178952=CARTESIAN_POINT('Ctrl Pts',(52.710670046285,18.76999998,-60.4053784571341));
#178953=CARTESIAN_POINT('Ctrl Pts',(52.5990660245491,18.76999998,-60.5717700902076));
#178954=CARTESIAN_POINT('Ctrl Pts',(52.3203251682923,18.76999998,-60.8494502533521));
#178955=CARTESIAN_POINT('Ctrl Pts',(52.1532979462845,18.76999998,-60.9606295880612));
#178956=CARTESIAN_POINT('Ctrl Pts',(51.7891054666292,18.76999998,-61.1109090094727));
#178957=CARTESIAN_POINT('Ctrl Pts',(51.592118965743,18.76999998,-61.149949999985));
#178958=CARTESIAN_POINT('Ctrl Pts',(51.394983875096,18.76999998,-61.14995));
#178959=CARTESIAN_POINT('Ctrl Pts',(52.900713631411,18.76999998,-59.64995));
#178960=CARTESIAN_POINT('Ctrl Pts',(52.3550593808763,18.76999998,-59.64995));
#178961=CARTESIAN_POINT('Ctrl Pts',(52.4026162823651,18.2264221086262,-59.64995));
#178962=CARTESIAN_POINT('Ctrl Pts',(52.9007136313967,18.76999998,-59.8463349320561));
#178963=CARTESIAN_POINT('Ctrl Pts',(52.3550593808723,18.76999998,-59.7746029379313));
#178964=CARTESIAN_POINT('Ctrl Pts',(52.402616282365,18.2264221086281,-59.7808732880371));
#178965=CARTESIAN_POINT('Ctrl Pts',(52.8615235106123,18.76999998,-60.0425718399612));
#178966=CARTESIAN_POINT('Ctrl Pts',(52.3316386425403,18.76999998,-59.8989712332646));
#178967=CARTESIAN_POINT('Ctrl Pts',(52.3763903041667,18.2275563241362,-59.9116978933078));
#178968=CARTESIAN_POINT('Ctrl Pts',(52.710670046285,18.76999998,-60.4053784571341));
#178969=CARTESIAN_POINT('Ctrl Pts',(52.239810099313,18.76999998,-60.1322291512602));
#178970=CARTESIAN_POINT('Ctrl Pts',(52.2754393607673,18.2319222289985,-60.1535689714224));
#178971=CARTESIAN_POINT('Ctrl Pts',(52.5990660245491,18.76999998,-60.5717700902076));
#178972=CARTESIAN_POINT('Ctrl Pts',(52.1717434473124,18.7699999799997,-60.2406767152624));
#178973=CARTESIAN_POINT('Ctrl Pts',(52.2007540936325,18.2351522014976,-60.2644967268053));
#178974=CARTESIAN_POINT('Ctrl Pts',(52.3203251682923,18.76999998,-60.8494502533521));
#178975=CARTESIAN_POINT('Ctrl Pts',(51.9977165994394,18.7699999800003,-60.4261994932772));
#178976=CARTESIAN_POINT('Ctrl Pts',(52.0142210728062,18.2432193417862,-60.4496168355678));
#178977=CARTESIAN_POINT('Ctrl Pts',(52.1532979462845,18.76999998,-60.9606295880612));
#178978=CARTESIAN_POINT('Ctrl Pts',(51.8922860151588,18.7699999800003,-60.5031527166051));
#178979=CARTESIAN_POINT('Ctrl Pts',(51.9024466716657,18.2480533372399,-60.5237363920407));
#178980=CARTESIAN_POINT('Ctrl Pts',(51.7891054666292,18.76999998,-61.1109090094727));
#178981=CARTESIAN_POINT('Ctrl Pts',(51.657019042446,18.7699999799997,-60.6120353079393));
#178982=CARTESIAN_POINT('Ctrl Pts',(51.6587295348784,18.2585935639752,-60.6239226729819));
#178983=CARTESIAN_POINT('Ctrl Pts',(51.592118965743,18.76999998,-61.149949999985));
#178984=CARTESIAN_POINT('Ctrl Pts',(51.5277022966008,18.7699999800007,-60.6442102195358));
#178985=CARTESIAN_POINT('Ctrl Pts',(51.5269064230252,18.264294621793,-60.64995));
#178986=CARTESIAN_POINT('Ctrl Pts',(51.394983875096,18.76999998,-61.14995));
#178987=CARTESIAN_POINT('Ctrl Pts',(51.394983875096,18.76999998,-60.64995));
#178988=CARTESIAN_POINT('Ctrl Pts',(51.394983875096,18.26999998,-60.64995));
#178989=CARTESIAN_POINT('',(52.4026162823651,18.2264221086262,-59.64995));
#178990=CARTESIAN_POINT('Origin',(52.900713631411,18.26999998,-59.64995));
#178991=CARTESIAN_POINT('Ctrl Pts',(51.394983875096,18.26999998,-60.64995));
#178992=CARTESIAN_POINT('Ctrl Pts',(51.4237727051561,18.2687549268196,-60.64995));
#178993=CARTESIAN_POINT('Ctrl Pts',(51.451335267364,18.2675736205104,-60.6487272519605));
#178994=CARTESIAN_POINT('Ctrl Pts',(51.4775920461836,18.2664491043645,-60.6465836174979));
#178995=CARTESIAN_POINT('Ctrl Pts',(51.5050161835672,18.265274592994,-60.6443446785022));
#178996=CARTESIAN_POINT('Ctrl Pts',(51.5310162920264,18.2641620725893,-60.6411017332696));
#178997=CARTESIAN_POINT('Ctrl Pts',(51.5555514746609,18.2631079651353,-60.6371711976494));
#178998=CARTESIAN_POINT('Ctrl Pts',(51.5807005119033,18.2620274845857,-60.633142322537));
#178999=CARTESIAN_POINT('Ctrl Pts',(51.6043110984276,18.2610084372763,-60.6283914211907));
#179000=CARTESIAN_POINT('Ctrl Pts',(51.6263811670969,18.2600506423559,-60.6232233711577));
#179001=CARTESIAN_POINT('Ctrl Pts',(51.6491770892134,18.2590613469108,-60.6178853512442));
#179002=CARTESIAN_POINT('Ctrl Pts',(51.6703302230382,18.2581374627052,-60.612102639129));
#179003=CARTESIAN_POINT('Ctrl Pts',(51.6898715157798,18.2572816972691,-60.6061674758653));
#179004=CARTESIAN_POINT('Ctrl Pts',(51.6928070816617,18.2571531409934,-60.6052758735025));
#179005=CARTESIAN_POINT('Ctrl Pts',(51.6957063201809,18.2570261261061,-60.6043807476975));
#179006=CARTESIAN_POINT('Ctrl Pts',(51.6985693825471,18.2569006658364,-60.6034830010222));
#179007=CARTESIAN_POINT('Ctrl Pts',(51.7111710647439,18.256348456263,-60.5995315962508));
#179008=CARTESIAN_POINT('Ctrl Pts',(51.7230716758463,18.2558263438253,-60.5955300976952));
#179009=CARTESIAN_POINT('Ctrl Pts',(51.7342861383916,18.2553356340763,-60.5915501614051));
#179010=CARTESIAN_POINT('Ctrl Pts',(51.7398933696642,18.2550902792017,-60.58956019326));
#179011=CARTESIAN_POINT('Ctrl Pts',(51.7453290261346,18.2548527717042,-60.5875755119223));
#179012=CARTESIAN_POINT('Ctrl Pts',(51.7505952924679,18.2546233027172,-60.5856042390434));
#179013=CARTESIAN_POINT('Ctrl Pts',(51.7532284256346,18.2545085682237,-60.584618602604));
#179014=CARTESIAN_POINT('Ctrl Pts',(51.7558192089008,18.2543958431508,-60.5836363114118));
#179015=CARTESIAN_POINT('Ctrl Pts',(51.7583679101829,18.2542851509382,-60.5826583363884));
#179016=CARTESIAN_POINT('Ctrl Pts',(51.7601161348254,18.2542092240906,-60.5819875162935));
#179017=CARTESIAN_POINT('Ctrl Pts',(51.7609326573293,18.2541734759912,-60.5816721106887));
#179018=CARTESIAN_POINT('Ctrl Pts',(51.7626946418676,18.2540972539743,-60.5809867219959));
#179019=CARTESIAN_POINT('Ctrl Pts',(51.7635014188846,18.2540623534573,-60.5806728964015));
#179020=CARTESIAN_POINT('Ctrl Pts',(51.7645062913134,18.2540189565485,-60.5802811765949));
#179021=CARTESIAN_POINT('Ctrl Pts',(51.7658880333948,18.2539591960934,-60.5797383010624));
#179022=CARTESIAN_POINT('Ctrl Pts',(51.7994271157594,18.2525086281088,-60.5665610609375));
#179023=CARTESIAN_POINT('Ctrl Pts',(51.8314973303886,18.2511292826187,-60.5518925917424));
#179024=CARTESIAN_POINT('Ctrl Pts',(51.8620286680791,18.2498150346114,-60.5360425708523));
#179025=CARTESIAN_POINT('Ctrl Pts',(51.8931419883397,18.2484757346577,-60.5198904198693));
#179026=CARTESIAN_POINT('Ctrl Pts',(51.9226575828774,18.2472040706567,-60.5025117129383));
#179027=CARTESIAN_POINT('Ctrl Pts',(51.9505524288216,18.2459980283681,-60.4842157548927));
#179028=CARTESIAN_POINT('Ctrl Pts',(51.9792094540704,18.2447590330217,-60.4654198908571));
#179029=CARTESIAN_POINT('Ctrl Pts',(52.0061563497031,18.243589329148,-60.4456563996028));
#179030=CARTESIAN_POINT('Ctrl Pts',(52.0314156457665,18.2424908878707,-60.4252343356306));
#179031=CARTESIAN_POINT('Ctrl Pts',(52.0333988373379,18.2424046455829,-60.4236309312824));
#179032=CARTESIAN_POINT('Ctrl Pts',(52.0353716476986,18.2423188444835,-60.4220234523116));
#179033=CARTESIAN_POINT('Ctrl Pts',(52.0373340985572,18.242233486472,-60.4204120405363));
#179034=CARTESIAN_POINT('Ctrl Pts',(52.0498612917415,18.2416886084713,-60.4101256853292));
#179035=CARTESIAN_POINT('Ctrl Pts',(52.0619661663755,18.2411617692931,-60.3996792357689));
#179036=CARTESIAN_POINT('Ctrl Pts',(52.0736557186227,18.2406535810223,-60.3891084430411));
#179037=CARTESIAN_POINT('Ctrl Pts',(52.0791075857478,18.240416568101,-60.3841783519528));
#179038=CARTESIAN_POINT('Ctrl Pts',(52.084147474518,18.2401960942946,-60.3795181564341));
#179039=CARTESIAN_POINT('Ctrl Pts',(52.0892317682909,18.2399752512423,-60.3747215662672));
#179040=CARTESIAN_POINT('Ctrl Pts',(52.0941767052513,18.2397604613383,-60.370056447165));
#179041=CARTESIAN_POINT('Ctrl Pts',(52.0991637980934,18.2395453354279,-60.3652622208462));
#179042=CARTESIAN_POINT('Ctrl Pts',(52.1045799184888,18.2393114302983,-60.359930701158));
#179043=CARTESIAN_POINT('Ctrl Pts',(52.1055352201106,18.2392701738392,-60.3589903215075));
#179044=CARTESIAN_POINT('Ctrl Pts',(52.1065037763543,18.2392283250547,-60.358033135595));
#179045=CARTESIAN_POINT('Ctrl Pts',(52.1074875832193,18.2391857716419,-60.3570567811866));
#179046=CARTESIAN_POINT('Ctrl Pts',(52.1379181186866,18.2378695345012,-60.3268567607196));
#179047=CARTESIAN_POINT('Ctrl Pts',(52.1661486617633,18.236668507618,-60.2949641541397));
#179048=CARTESIAN_POINT('Ctrl Pts',(52.1920517229949,18.2355715371104,-60.2617220237118));
#179049=CARTESIAN_POINT('Ctrl Pts',(52.2182622702554,18.2344615448559,-60.2280852877741));
#179050=CARTESIAN_POINT('Ctrl Pts',(52.2420898530018,18.2334581030591,-60.193067311089));
#179051=CARTESIAN_POINT('Ctrl Pts',(52.2634559174668,18.2325543391559,-60.1570220983486));
#179052=CARTESIAN_POINT('Ctrl Pts',(52.2850807034988,18.2316396315802,-60.1205404143085));
#179053=CARTESIAN_POINT('Ctrl Pts',(52.3041841730781,18.2308270458906,-60.0830069552407));
#179054=CARTESIAN_POINT('Ctrl Pts',(52.3207372784833,18.2301140407409,-60.0447796547096));
#179055=CARTESIAN_POINT('Ctrl Pts',(52.3375983740247,18.2293877692857,-60.0058410899653));
#179056=CARTESIAN_POINT('Ctrl Pts',(52.351813515365,18.2287648357927,-59.9661831062492));
#179057=CARTESIAN_POINT('Ctrl Pts',(52.3634032636446,18.2282470391287,-59.9261671553576));
#179058=CARTESIAN_POINT('Ctrl Pts',(52.3751177180226,18.2277236709544,-59.8857206314297));
#179059=CARTESIAN_POINT('Ctrl Pts',(52.3841503063993,18.2273077431756,-59.8449088095266));
#179060=CARTESIAN_POINT('Ctrl Pts',(52.3905700243695,18.2270052921247,-59.8040810753798));
#179061=CARTESIAN_POINT('Ctrl Pts',(52.3970915619048,18.2266980440664,-59.7626057953194));
#179062=CARTESIAN_POINT('Ctrl Pts',(52.4009170425841,18.2265079317809,-59.7211144793536));
#179063=CARTESIAN_POINT('Ctrl Pts',(52.4021626662287,18.2264451214354,-59.679942768914));
#179064=CARTESIAN_POINT('Ctrl Pts',(52.4024657503462,18.226429838474,-59.669924902299));
#179065=CARTESIAN_POINT('Ctrl Pts',(52.4026162823651,18.2264221086262,-59.6599258027971));
#179066=CARTESIAN_POINT('Ctrl Pts',(52.4026162823651,18.2264221086262,-59.64995));
#179067=CARTESIAN_POINT('Origin',(0.,-12.9675000200281,-60.64995));
#179068=CARTESIAN_POINT('',(51.6244217512084,15.6475130558006,-60.64995));
#179069=CARTESIAN_POINT('Origin',(0.,-12.9675000200281,-60.64995));
#179070=CARTESIAN_POINT('',(53.7167487055517,-8.26789346682159,-60.64995));
#179071=CARTESIAN_POINT('Origin',(0.,-12.9675000200281,-61.64995));
#179072=CARTESIAN_POINT('',(52.4885489491165,12.6049688303995,-60.8798615124595));
#179073=CARTESIAN_POINT('Ctrl Pts',(51.6244217512084,15.6475130558006,-60.64995));
#179074=CARTESIAN_POINT('Ctrl Pts',(51.6551646996741,15.5433894621099,-60.64995));
#179075=CARTESIAN_POINT('Ctrl Pts',(51.6891856571931,15.42785477597,-60.6507769894556));
#179076=CARTESIAN_POINT('Ctrl Pts',(51.7449269585569,15.2374765632288,-60.6540853355037));
#179077=CARTESIAN_POINT('Ctrl Pts',(51.7739758200045,15.1380192813913,-60.6562586768657));
#179078=CARTESIAN_POINT('Ctrl Pts',(51.809894806679,15.0145363819814,-60.6599052372727));
#179079=CARTESIAN_POINT('Ctrl Pts',(51.8283585992563,14.950936056674,-60.6620329872155));
#179080=CARTESIAN_POINT('Ctrl Pts',(51.8363794579957,14.9232808461768,-60.6630130104025));
#179081=CARTESIAN_POINT('Ctrl Pts',(51.8417506290901,14.9047556582866,-60.6636818234472));
#179082=CARTESIAN_POINT('Ctrl Pts',(51.8448598242051,14.8940282232909,-60.6640771410432));
#179083=CARTESIAN_POINT('Ctrl Pts',(51.883923482042,14.7592131237825,-60.6691236656757));
#179084=CARTESIAN_POINT('Ctrl Pts',(51.9387151074887,14.5688372951455,-60.6779958996905));
#179085=CARTESIAN_POINT('Ctrl Pts',(52.0022407624029,14.3467628952478,-60.6913501116407));
#179086=CARTESIAN_POINT('Ctrl Pts',(52.0339323134534,14.2357469132923,-60.6987687241444));
#179087=CARTESIAN_POINT('Ctrl Pts',(52.0497637801078,14.1802458880588,-60.7026621789418));
#179088=CARTESIAN_POINT('Ctrl Pts',(52.0565460034622,14.1564614021569,-60.7043701243749));
#179089=CARTESIAN_POINT('Ctrl Pts',(52.0610669293512,14.1406054681221,-60.7055174770928));
#179090=CARTESIAN_POINT('Ctrl Pts',(52.062782551509,14.134587959597,-60.7059551790868));
#179091=CARTESIAN_POINT('Ctrl Pts',(52.2450744027298,13.4951289417155,-60.752932396218));
#179092=CARTESIAN_POINT('Ctrl Pts',(52.3839308970543,12.9889668299485,-60.818448001159));
#179093=CARTESIAN_POINT('Ctrl Pts',(52.4885489491165,12.6049688303995,-60.8798615124595));
#179094=CARTESIAN_POINT('Ctrl Pts',(52.4885489491165,12.6049688303995,-60.8798615124595));
#179095=CARTESIAN_POINT('Ctrl Pts',(52.5003074888079,12.5618093982546,-60.8867640803813));
#179096=CARTESIAN_POINT('Ctrl Pts',(52.5123202735365,12.518720787882,-60.8936385283445));
#179097=CARTESIAN_POINT('Ctrl Pts',(52.5245819708709,12.4756972986243,-60.9004583201737));
#179098=CARTESIAN_POINT('Ctrl Pts',(52.813519414917,12.5211707144541,-60.5028360925953));
#179099=CARTESIAN_POINT('Ctrl Pts',(52.7011006011713,12.5792267001133,-60.7309116189004));
#179100=CARTESIAN_POINT('Ctrl Pts',(52.4885489491165,12.6049688303995,-60.8798615124595));
#179101=CARTESIAN_POINT('Ctrl Pts',(52.8184252363688,12.4804454574502,-60.5118893693287));
#179102=CARTESIAN_POINT('Ctrl Pts',(52.7083699494147,12.5371106789483,-60.7374192211269));
#179103=CARTESIAN_POINT('Ctrl Pts',(52.5003487858574,12.5616578171005,-60.8867883233088));
#179104=CARTESIAN_POINT('Ctrl Pts',(52.823766550455,12.4396518133592,-60.5210243207318));
#179105=CARTESIAN_POINT('Ctrl Pts',(52.7160214096145,12.4948853110753,-60.7440415583411));
#179106=CARTESIAN_POINT('Ctrl Pts',(52.5124335500125,12.5183120391401,-60.8937038544239));
#179107=CARTESIAN_POINT('Ctrl Pts',(52.8295491865184,12.3987982841401,-60.5301925771521));
#179108=CARTESIAN_POINT('Ctrl Pts',(52.7240626356492,12.4525613978151,-60.750736804912));
#179109=CARTESIAN_POINT('Ctrl Pts',(52.5248032674767,12.4749209213966,-60.9005813814078));
#179110=CARTESIAN_POINT('Origin',(51.9150548124647,12.3255619647296,-60.1097730249189));
#179111=CARTESIAN_POINT('Ctrl Pts',(53.2607580814926,12.11999998,-60.7033966151602));
#179112=CARTESIAN_POINT('Ctrl Pts',(52.8857929788877,12.11999998,-60.5379900686009));
#179113=CARTESIAN_POINT('Ctrl Pts',(52.81219032515,12.5218539749099,-60.5055220850798));
#179114=CARTESIAN_POINT('Ctrl Pts',(53.3498368505456,12.11999998,-60.5014612122216));
#179115=CARTESIAN_POINT('Ctrl Pts',(52.9388615253298,12.1199999799981,-60.3810288628603));
#179116=CARTESIAN_POINT('Ctrl Pts',(52.8700875991767,12.5389561241882,-60.3657903170377));
#179117=CARTESIAN_POINT('Ctrl Pts',(53.3950245780495,12.11999998,-60.2853240337268));
#179118=CARTESIAN_POINT('Ctrl Pts',(52.9540808994585,12.1199999800015,-60.2191862528169));
#179119=CARTESIAN_POINT('Ctrl Pts',(52.8985874779024,12.5574454029709,-60.2163866339305));
#179120=CARTESIAN_POINT('Ctrl Pts',(53.3950245803325,12.11999998,-60.0627241236311));
#179121=CARTESIAN_POINT('Ctrl Pts',(52.9368589933238,12.11999998,-60.0627241236309));
#179122=CARTESIAN_POINT('Ctrl Pts',(52.8969272312866,12.5764221086261,-60.0627241236309));
#179123=CARTESIAN_POINT('',(52.8969272306107,12.5764221085651,-60.0627241236309));
#179124=CARTESIAN_POINT('',(53.3950245803324,12.11999998,-60.0627241236309));
#179125=CARTESIAN_POINT('Origin',(53.3950245803325,12.61999998,-60.0627241236309));
#179126=CARTESIAN_POINT('Origin',(50.5588767643988,12.11999998,-59.7245163412853));
#179127=CARTESIAN_POINT('Ctrl Pts',(52.8969272312868,12.5764221086243,-60.0627241236309));
#179128=CARTESIAN_POINT('Ctrl Pts',(52.8972093867344,12.5731970571004,-60.0888387457683));
#179129=CARTESIAN_POINT('Ctrl Pts',(52.8966025741109,12.5702371653934,-60.1127979091318));
#179130=CARTESIAN_POINT('Ctrl Pts',(52.895492143609,12.5675483472939,-60.1345630157725));
#179131=CARTESIAN_POINT('Ctrl Pts',(52.8952383309491,12.5669337603633,-60.139537896776));
#179132=CARTESIAN_POINT('Ctrl Pts',(52.8949580002003,12.566333324942,-60.1443982053448));
#179133=CARTESIAN_POINT('Ctrl Pts',(52.8946553754963,12.5657470947143,-60.1491435666974));
#179134=CARTESIAN_POINT('Ctrl Pts',(52.8935370825506,12.5635807906436,-60.1666791612968));
#179135=CARTESIAN_POINT('Ctrl Pts',(52.8921164516363,12.5616084482314,-60.1826454242178));
#179136=CARTESIAN_POINT('Ctrl Pts',(52.8905899490122,12.559833631543,-60.1970148166353));
#179137=CARTESIAN_POINT('Ctrl Pts',(52.8896508802967,12.5587418058223,-60.2058545308072));
#179138=CARTESIAN_POINT('Ctrl Pts',(52.8886715980987,12.5577250679358,-60.2140871499417));
#179139=CARTESIAN_POINT('Ctrl Pts',(52.8876909467741,12.5567829255677,-60.2217165962902));
#179140=CARTESIAN_POINT('Ctrl Pts',(52.8859652650759,12.5551250092409,-60.2351423630245));
#179141=CARTESIAN_POINT('Ctrl Pts',(52.8842371940579,12.5536970103207,-60.2467090858731));
#179142=CARTESIAN_POINT('Ctrl Pts',(52.8826767053327,12.5524961277858,-60.2564379859943));
#179143=CARTESIAN_POINT('Ctrl Pts',(52.8811308498546,12.5513065063453,-60.2660756548253));
#179144=CARTESIAN_POINT('Ctrl Pts',(52.879749595859,12.5503398173612,-60.2739092846511));
#179145=CARTESIAN_POINT('Ctrl Pts',(52.878645753002,12.5495929425003,-60.2799623795994));
#179146=CARTESIAN_POINT('Ctrl Pts',(52.8784091261802,12.5494328376235,-60.2812599597849));
#179147=CARTESIAN_POINT('Ctrl Pts',(52.8781850597772,12.5492828377151,-60.2824756887368));
#179148=CARTESIAN_POINT('Ctrl Pts',(52.8779743558538,12.54914291719,-60.2836097586939));
#179149=CARTESIAN_POINT('Ctrl Pts',(52.8778077082517,12.5490322528056,-60.2845067046824));
#179150=CARTESIAN_POINT('Ctrl Pts',(52.8776494172265,12.5489278934755,-60.2853525696634));
#179151=CARTESIAN_POINT('Ctrl Pts',(52.8774998415707,12.5488297619182,-60.2861474384989));
#179152=CARTESIAN_POINT('Ctrl Pts',(52.8774624476567,12.5488052290289,-60.2863461557077));
#179153=CARTESIAN_POINT('Ctrl Pts',(52.8774483929893,12.54879592331,-60.2864207378837));
#179154=CARTESIAN_POINT('Ctrl Pts',(52.8774406506828,12.5487907192805,-60.286461911159));
#179155=CARTESIAN_POINT('Ctrl Pts',(52.8774329083763,12.5487855152511,-60.2865030844342));
#179156=CARTESIAN_POINT('Ctrl Pts',(52.8774314674585,12.5487844132509,-60.2865108462554));
#179157=CARTESIAN_POINT('Ctrl Pts',(52.8774192125423,12.548776290571,-60.2865759021724));
#179158=CARTESIAN_POINT('Ctrl Pts',(52.8773947027099,12.5487600452112,-60.2867060140063));
#179159=CARTESIAN_POINT('Ctrl Pts',(52.8773276045743,12.5487158014682,-60.2870654427123));
#179160=CARTESIAN_POINT('Ctrl Pts',(52.8770776120991,12.5485537277925,-60.2883791407993));
#179161=CARTESIAN_POINT('Ctrl Pts',(52.870030916608,12.5439852549261,-60.3254091769202));
#179162=CARTESIAN_POINT('Ctrl Pts',(52.8614724626347,12.5397015659191,-60.3601737018512));
#179163=CARTESIAN_POINT('Ctrl Pts',(52.8519633454955,12.5357049347099,-60.3926622296679));
#179164=CARTESIAN_POINT('Ctrl Pts',(52.8423230082821,12.5316531524035,-60.4255990795497));
#179165=CARTESIAN_POINT('Ctrl Pts',(52.8317061291368,12.5278962903145,-60.4561974030475));
#179166=CARTESIAN_POINT('Ctrl Pts',(52.8206579435906,12.5244306778137,-60.4844812536859));
#179167=CARTESIAN_POINT('Ctrl Pts',(52.8178604768424,12.5235531639729,-60.4916428940603));
#179168=CARTESIAN_POINT('Ctrl Pts',(52.8150351397417,12.5226942982607,-60.4986562874559));
#179169=CARTESIAN_POINT('Ctrl Pts',(52.81219032515,12.5218539749099,-60.5055220850798));
#179170=CARTESIAN_POINT('Origin',(-83.2809572255632,12.1199999800001,-55.24995));
#179171=CARTESIAN_POINT('',(53.3950245803324,12.11999998,-55.74995));
#179172=CARTESIAN_POINT('',(53.3950245803324,12.11999998,-55.24995));
#179173=CARTESIAN_POINT('',(-83.2809572255632,12.1199999800001,-55.74995));
#179174=CARTESIAN_POINT('Origin',(60.,28.41999998,-55.24995));
#179175=CARTESIAN_POINT('',(51.9689593648599,28.41999998,-59.64995));
#179176=CARTESIAN_POINT('Ctrl Pts',(50.4632296085449,28.41999998,-61.14995));
#179177=CARTESIAN_POINT('Ctrl Pts',(50.6603646991919,28.41999998,-61.149949999985));
#179178=CARTESIAN_POINT('Ctrl Pts',(50.8573512000782,28.41999998,-61.1109090094727));
#179179=CARTESIAN_POINT('Ctrl Pts',(51.2215436797334,28.41999998,-60.9606295880612));
#179180=CARTESIAN_POINT('Ctrl Pts',(51.3885709017413,28.41999998,-60.849450253352));
#179181=CARTESIAN_POINT('Ctrl Pts',(51.6673117579979,28.41999998,-60.5717700902076));
#179182=CARTESIAN_POINT('Ctrl Pts',(51.7789157797339,28.41999998,-60.4053784571342));
#179183=CARTESIAN_POINT('Ctrl Pts',(51.9297692440612,28.41999998,-60.0425718399611));
#179184=CARTESIAN_POINT('Ctrl Pts',(51.9689593648456,28.41999998,-59.8463349320562));
#179185=CARTESIAN_POINT('Ctrl Pts',(51.9689593648599,28.41999998,-59.64995));
#179186=CARTESIAN_POINT('',(51.9689593648599,28.41999998,-55.74995));
#179187=CARTESIAN_POINT('',(51.9689593648599,28.41999998,-55.24995));
#179188=CARTESIAN_POINT('',(60.,28.41999998,-55.74995));
#179189=CARTESIAN_POINT('Ctrl Pts',(50.4632296085449,28.41999998,-61.14995));
#179190=CARTESIAN_POINT('Ctrl Pts',(50.4632296085449,28.41999998,-60.64995));
#179191=CARTESIAN_POINT('Ctrl Pts',(50.4632296085449,28.91999998,-60.64995));
#179192=CARTESIAN_POINT('Ctrl Pts',(50.6603646991919,28.41999998,-61.149949999985));
#179193=CARTESIAN_POINT('Ctrl Pts',(50.5943760783778,28.4199999799973,-60.6556217969837));
#179194=CARTESIAN_POINT('Ctrl Pts',(50.5951521564739,28.9142946217921,-60.64995));
#179195=CARTESIAN_POINT('Ctrl Pts',(50.8573512000782,28.41999998,-61.1109090094727));
#179196=CARTESIAN_POINT('Ctrl Pts',(50.728657566052,28.4199999799997,-60.6353187454025));
#179197=CARTESIAN_POINT('Ctrl Pts',(50.7269752683276,28.9085935639752,-60.6239226729817));
#179198=CARTESIAN_POINT('Ctrl Pts',(51.2215436797334,28.41999998,-60.9606295880612));
#179199=CARTESIAN_POINT('Ctrl Pts',(50.9800327848971,28.4199999800004,-60.5426326522478));
#179200=CARTESIAN_POINT('Ctrl Pts',(50.9706924051143,28.8980533372399,-60.5237363920408));
#179201=CARTESIAN_POINT('Ctrl Pts',(51.3885709017413,28.41999998,-60.849450253352));
#179202=CARTESIAN_POINT('Ctrl Pts',(51.0973398682523,28.4199999799993,-60.4706504746461));
#179203=CARTESIAN_POINT('Ctrl Pts',(51.0824668062551,28.8932193417862,-60.4496168355678));
#179204=CARTESIAN_POINT('Ctrl Pts',(51.6673117579979,28.41999998,-60.5717700902076));
#179205=CARTESIAN_POINT('Ctrl Pts',(51.294270482316,28.4199999800007,-60.2852157712125));
#179206=CARTESIAN_POINT('Ctrl Pts',(51.2689998270813,28.8851522014976,-60.2644967268053));
#179207=CARTESIAN_POINT('Ctrl Pts',(51.7789157797339,28.41999998,-60.4053784571342));
#179208=CARTESIAN_POINT('Ctrl Pts',(51.3742886138646,28.4199999800003,-60.1718710142637));
#179209=CARTESIAN_POINT('Ctrl Pts',(51.343685094216,28.8819222289984,-60.153568971423));
#179210=CARTESIAN_POINT('Ctrl Pts',(51.9297692440612,28.41999998,-60.0425718399611));
#179211=CARTESIAN_POINT('Ctrl Pts',(51.4824004299641,28.4199999799996,-59.9224177216067));
#179212=CARTESIAN_POINT('Ctrl Pts',(51.4446360376159,28.8775563241362,-59.9116978933072));
#179213=CARTESIAN_POINT('Ctrl Pts',(51.9689593648456,28.41999998,-59.8463349320562));
#179214=CARTESIAN_POINT('Ctrl Pts',(51.5107937778383,28.4199999799973,-59.7861314644994));
#179215=CARTESIAN_POINT('Ctrl Pts',(51.4708620158139,28.8764221086278,-59.7808732880376));
#179216=CARTESIAN_POINT('Ctrl Pts',(51.9689593648599,28.41999998,-59.64995));
#179217=CARTESIAN_POINT('Ctrl Pts',(51.5107937778512,28.41999998,-59.6499499999999));
#179218=CARTESIAN_POINT('Ctrl Pts',(51.4708620158141,28.8764221086262,-59.64995));
#179219=CARTESIAN_POINT('',(51.4708620158141,28.8764221086262,-59.64995));
#179220=CARTESIAN_POINT('Ctrl Pts',(51.4708620158141,28.8764221086262,-59.64995));
#179221=CARTESIAN_POINT('Ctrl Pts',(51.4708620158141,28.8764221086262,-59.6947437542449));
#179222=CARTESIAN_POINT('Ctrl Pts',(51.4677914119307,28.8765549054479,-59.7400065139138));
#179223=CARTESIAN_POINT('Ctrl Pts',(51.4615373286702,28.8768253807065,-59.7853172193946));
#179224=CARTESIAN_POINT('Ctrl Pts',(51.4553593802397,28.8770925633022,-59.8300763295867));
#179225=CARTESIAN_POINT('Ctrl Pts',(51.4460749723573,28.8774940933935,-59.8748822598591));
#179226=CARTESIAN_POINT('Ctrl Pts',(51.433582992122,28.8780343438896,-59.9192791434306));
#179227=CARTESIAN_POINT('Ctrl Pts',(51.4237924546126,28.878457762967,-59.9540750161202));
#179228=CARTESIAN_POINT('Ctrl Pts',(51.4120317874587,28.8789663857909,-59.9886186686624));
#179229=CARTESIAN_POINT('Ctrl Pts',(51.3982557900138,28.8795621671893,-60.022668488024));
#179230=CARTESIAN_POINT('Ctrl Pts',(51.3969099642094,28.8796203711765,-60.0259949350354));
#179231=CARTESIAN_POINT('Ctrl Pts',(51.395544903161,28.8796794070455,-60.0293166615587));
#179232=CARTESIAN_POINT('Ctrl Pts',(51.394160565916,28.8797392765673,-60.0326334323651));
#179233=CARTESIAN_POINT('Ctrl Pts',(51.3763389976224,28.8805100199507,-60.0753326067533));
#179234=CARTESIAN_POINT('Ctrl Pts',(51.3553254607148,28.8814188089116,-60.1171993192663));
#179235=CARTESIAN_POINT('Ctrl Pts',(51.3312072018932,28.8824618702235,-60.1577697852322));
#179236=CARTESIAN_POINT('Ctrl Pts',(51.3081659897204,28.8834583516518,-60.1965284999963));
#179237=CARTESIAN_POINT('Ctrl Pts',(51.2822921557851,28.8845773377017,-60.2341031988361));
#179238=CARTESIAN_POINT('Ctrl Pts',(51.2536794880379,28.885814772252,-60.2700569697484));
#179239=CARTESIAN_POINT('Ctrl Pts',(51.2402309219474,28.8863963929691,-60.2869560114103));
#179240=CARTESIAN_POINT('Ctrl Pts',(51.2261775125214,28.8870041718217,-60.3034964088543));
#179241=CARTESIAN_POINT('Ctrl Pts',(51.2115313248591,28.887637587021,-60.31962880781));
#179242=CARTESIAN_POINT('Ctrl Pts',(51.2063396801368,28.8878621141644,-60.3253472709232));
#179243=CARTESIAN_POINT('Ctrl Pts',(51.2007966899397,28.8881018362233,-60.331313045859));
#179244=CARTESIAN_POINT('Ctrl Pts',(51.1952694028553,28.8883408744107,-60.3371156972533));
#179245=CARTESIAN_POINT('Ctrl Pts',(51.1895768899865,28.8885870581058,-60.3430918058271));
#179246=CARTESIAN_POINT('Ctrl Pts',(51.1839011962162,28.8888325093769,-60.3488947477628));
#179247=CARTESIAN_POINT('Ctrl Pts',(51.1786846053927,28.8890580952226,-60.3541155165136));
#179248=CARTESIAN_POINT('Ctrl Pts',(51.1776827065602,28.8891014212574,-60.3551182177591));
#179249=CARTESIAN_POINT('Ctrl Pts',(51.1766978520225,28.8891440097864,-60.3560995559722));
#179250=CARTESIAN_POINT('Ctrl Pts',(51.1757333189604,28.889185719042,-60.3570567834875));
#179251=CARTESIAN_POINT('Ctrl Pts',(51.1538095834162,28.8901337660555,-60.3788144647157));
#179252=CARTESIAN_POINT('Ctrl Pts',(51.1302168006257,28.8911541156617,-60.4001952306223));
#179253=CARTESIAN_POINT('Ctrl Pts',(51.1049004315856,28.8922490328123,-60.4209274438526));
#179254=CARTESIAN_POINT('Ctrl Pts',(51.0800414498951,28.8933241682456,-60.4412850910443));
#179255=CARTESIAN_POINT('Ctrl Pts',(51.0535203284385,28.8944712128831,-60.4610175331667));
#179256=CARTESIAN_POINT('Ctrl Pts',(51.0253174707832,28.895690924054,-60.4798306487176));
#179257=CARTESIAN_POINT('Ctrl Pts',(50.9984842726526,28.8968514004819,-60.4977301134883));
#179258=CARTESIAN_POINT('Ctrl Pts',(50.9701273672128,28.8980777738785,-60.5147982857245));
#179259=CARTESIAN_POINT('Ctrl Pts',(50.9402580440922,28.8993695559923,-60.5307488754987));
#179260=CARTESIAN_POINT('Ctrl Pts',(50.9111997131181,28.9006262644907,-60.5462663853875));
#179261=CARTESIAN_POINT('Ctrl Pts',(50.8807093109566,28.9019449068983,-60.5607262880739));
#179262=CARTESIAN_POINT('Ctrl Pts',(50.848833836721,28.9033234506075,-60.5738295325112));
#179263=CARTESIAN_POINT('Ctrl Pts',(50.8483100004268,28.9033461053678,-60.5740448690724));
#179264=CARTESIAN_POINT('Ctrl Pts',(50.8477857926334,28.9033687761946,-60.5742598379419));
#179265=CARTESIAN_POINT('Ctrl Pts',(50.8472612136072,28.9033914630764,-60.5744744380591));
#179266=CARTESIAN_POINT('Ctrl Pts',(50.8446281185304,28.9035053386106,-60.5755516113424));
#179267=CARTESIAN_POINT('Ctrl Pts',(50.8412782753391,28.9036501970354,-60.5769043222802));
#179268=CARTESIAN_POINT('Ctrl Pts',(50.838494961749,28.9037705514899,-60.5780123790327));
#179269=CARTESIAN_POINT('Ctrl Pts',(50.8366796282304,28.9038490491037,-60.5787350760979));
#179270=CARTESIAN_POINT('Ctrl Pts',(50.8351058488345,28.9039170988377,-60.5793550577221));
#179271=CARTESIAN_POINT('Ctrl Pts',(50.8341332510858,28.9039591509512,-60.5797369926547));
#179272=CARTESIAN_POINT('Ctrl Pts',(50.8185784237332,28.9046316934953,-60.5858453061323));
#179273=CARTESIAN_POINT('Ctrl Pts',(50.8013542666607,28.9053764998681,-60.5921640965717));
#179274=CARTESIAN_POINT('Ctrl Pts',(50.7823963801911,28.9061963347677,-60.5984375212453));
#179275=CARTESIAN_POINT('Ctrl Pts',(50.763113162345,28.9070302386416,-60.6048186025338));
#179276=CARTESIAN_POINT('Ctrl Pts',(50.742035176342,28.907941812522,-60.6111530887002));
#179277=CARTESIAN_POINT('Ctrl Pts',(50.7191146374363,28.9089331013732,-60.6171173698768));
#179278=CARTESIAN_POINT('Ctrl Pts',(50.6984237561229,28.9098279599125,-60.6225014594243));
#179279=CARTESIAN_POINT('Ctrl Pts',(50.6762310064599,28.9107877942718,-60.6275832962447));
#179280=CARTESIAN_POINT('Ctrl Pts',(50.6525261952328,28.9118130292334,-60.6320843347403));
#179281=CARTESIAN_POINT('Ctrl Pts',(50.6295865055205,28.9128051726289,-60.6364400929653));
#179282=CARTESIAN_POINT('Ctrl Pts',(50.6052302671986,28.9138585854426,-60.6402518751851));
#179283=CARTESIAN_POINT('Ctrl Pts',(50.5794793889038,28.9149723054461,-60.6432310344106));
#179284=CARTESIAN_POINT('Ctrl Pts',(50.5549130980113,28.9160347922967,-60.6460731468742));
#179285=CARTESIAN_POINT('Ctrl Pts',(50.5290771857652,28.9171521802695,-60.648157343778));
#179286=CARTESIAN_POINT('Ctrl Pts',(50.5020254916425,28.9183221279484,-60.649201067293));
#179287=CARTESIAN_POINT('Ctrl Pts',(50.489356743992,28.9188700334453,-60.6496898599641));
#179288=CARTESIAN_POINT('Ctrl Pts',(50.4764218916548,28.9194294429546,-60.64995));
#179289=CARTESIAN_POINT('Ctrl Pts',(50.4632296085449,28.91999998,-60.64995));
#179290=CARTESIAN_POINT('Origin',(51.9689593648599,28.91999998,-59.64995));
#179291=CARTESIAN_POINT('Origin',(60.,27.91999998,-55.74995));
#179292=CARTESIAN_POINT('',(52.0564480283858,27.91999998,-55.24995));
#179293=CARTESIAN_POINT('Ctrl Pts',(51.9689593648599,28.41999998,-55.74995));
#179294=CARTESIAN_POINT('Ctrl Pts',(51.9689593648599,28.41999998,-55.7240510277418));
#179295=CARTESIAN_POINT('Ctrl Pts',(51.9693268087427,28.4179000286038,-55.697853607272));
#179296=CARTESIAN_POINT('Ctrl Pts',(51.9700690003256,28.413658384301,-55.6716786001611));
#179297=CARTESIAN_POINT('Ctrl Pts',(51.9708174603259,28.4093809158292,-55.6452825236222));
#179298=CARTESIAN_POINT('Ctrl Pts',(51.9719470328068,28.4029253795636,-55.6189093029559));
#179299=CARTESIAN_POINT('Ctrl Pts',(51.9734602061033,28.3942775546035,-55.5929324714478));
#179300=CARTESIAN_POINT('Ctrl Pts',(51.9740304013453,28.3910188738844,-55.5831438598178));
#179301=CARTESIAN_POINT('Ctrl Pts',(51.974655014541,28.3874491931361,-55.5734119763965));
#179302=CARTESIAN_POINT('Ctrl Pts',(51.9753339939828,28.3835688078698,-55.5637583893672));
#179303=CARTESIAN_POINT('Ctrl Pts',(51.977112728374,28.3734032943058,-55.5384687175561));
#179304=CARTESIAN_POINT('Ctrl Pts',(51.9792657855805,28.361098516063,-55.5136974845899));
#179305=CARTESIAN_POINT('Ctrl Pts',(51.9817930862496,28.3466549266444,-55.4898442371366));
#179306=CARTESIAN_POINT('Ctrl Pts',(51.9838432153151,28.3349383854197,-55.4704946454921));
#179307=CARTESIAN_POINT('Ctrl Pts',(51.9861398889717,28.3218128354093,-55.451748367254));
#179308=CARTESIAN_POINT('Ctrl Pts',(51.98867993897,28.3072963832421,-55.4338552802796));
#179309=CARTESIAN_POINT('Ctrl Pts',(51.9900517282542,28.2994565716081,-55.4241918701149));
#179310=CARTESIAN_POINT('Ctrl Pts',(51.9914944591103,28.2912113270354,-55.4147778015411));
#179311=CARTESIAN_POINT('Ctrl Pts',(51.993006833706,28.2825680666705,-55.4056571306828));
#179312=CARTESIAN_POINT('Ctrl Pts',(51.993308064795,28.2808465231189,-55.4038404976718));
#179313=CARTESIAN_POINT('Ctrl Pts',(51.9936750712784,28.2787490714756,-55.4016626948096));
#179314=CARTESIAN_POINT('Ctrl Pts',(51.993998383369,28.2769013041842,-55.3997779182116));
#179315=CARTESIAN_POINT('Ctrl Pts',(51.9942306762961,28.2755737223049,-55.3984237459251));
#179316=CARTESIAN_POINT('Ctrl Pts',(51.9944401788581,28.2743763723404,-55.3972196111484));
#179317=CARTESIAN_POINT('Ctrl Pts',(51.9945841744765,28.2735533694274,-55.3963966082408));
#179318=CARTESIAN_POINT('Ctrl Pts',(51.996292885289,28.2637872807656,-55.3866305196434));
#179319=CARTESIAN_POINT('Ctrl Pts',(51.9982002406164,28.2528864178514,-55.3765717208114));
#179320=CARTESIAN_POINT('Ctrl Pts',(52.0003285939908,28.2407228045164,-55.3664552894479));
#179321=CARTESIAN_POINT('Ctrl Pts',(52.0023666881836,28.2290750255335,-55.3567678755708));
#179322=CARTESIAN_POINT('Ctrl Pts',(52.0046075587555,28.2162686120025,-55.3470275906024));
#179323=CARTESIAN_POINT('Ctrl Pts',(52.0070668802308,28.2022137834753,-55.337481543908));
#179324=CARTESIAN_POINT('Ctrl Pts',(52.0093860198903,28.1889600829847,-55.328479623784));
#179325=CARTESIAN_POINT('Ctrl Pts',(52.0118994950179,28.1745957837208,-55.3196505220217));
#179326=CARTESIAN_POINT('Ctrl Pts',(52.0146154596132,28.1590741144307,-55.3112377696321));
#179327=CARTESIAN_POINT('Ctrl Pts',(52.0157114814312,28.152810377332,-55.3078428210439));
#179328=CARTESIAN_POINT('Ctrl Pts',(52.0168404135437,28.1463585346195,-55.3045160976751));
#179329=CARTESIAN_POINT('Ctrl Pts',(52.0180024981996,28.1397171904213,-55.3012753797206));
#179330=CARTESIAN_POINT('Ctrl Pts',(52.0206705726152,28.1244690753626,-55.2938348919567));
#179331=CARTESIAN_POINT('Ctrl Pts',(52.0235156308817,28.1082094929675,-55.286840723483));
#179332=CARTESIAN_POINT('Ctrl Pts',(52.0265363392804,28.0909460654729,-55.2805340044421));
#179333=CARTESIAN_POINT('Ctrl Pts',(52.0294725600147,28.07416548719,-55.2744036810978));
#179334=CARTESIAN_POINT('Ctrl Pts',(52.0325747975933,28.0564361182996,-55.2689228588362));
#179335=CARTESIAN_POINT('Ctrl Pts',(52.0358354676438,28.0378013036895,-55.2643427579155));
#179336=CARTESIAN_POINT('Ctrl Pts',(52.0389930632159,28.0197555624189,-55.259907440584));
#179337=CARTESIAN_POINT('Ctrl Pts',(52.0422992724608,28.0008604901217,-55.2563167977524));
#179338=CARTESIAN_POINT('Ctrl Pts',(52.0457404862589,27.9811938632732,-55.2538274761772));
#179339=CARTESIAN_POINT('Ctrl Pts',(52.0491817000569,27.9615272364247,-55.2513381546019));
#179340=CARTESIAN_POINT('Ctrl Pts',(52.0527579931129,27.9410886280845,-55.24995));
#179341=CARTESIAN_POINT('Ctrl Pts',(52.0564480283858,27.91999998,-55.24995));
#179342=CARTESIAN_POINT('',(60.,27.91999998,-55.24995));
#179343=CARTESIAN_POINT('Origin',(60.,28.41999998,-55.24995));
#179344=CARTESIAN_POINT('',(52.1001923601488,27.41999998,-55.24995));
#179345=CARTESIAN_POINT('',(52.0733761857257,27.7265102562164,-55.24995));
#179346=CARTESIAN_POINT('',(60.,27.41999998,-55.24995));
#179347=CARTESIAN_POINT('Origin',(60.,27.41999998,-55.74995));
#179348=CARTESIAN_POINT('',(52.1876810236747,26.91999998,-55.74995));
#179349=CARTESIAN_POINT('Ctrl Pts',(52.1001923601488,27.41999998,-55.24995));
#179350=CARTESIAN_POINT('Ctrl Pts',(52.1039692544698,27.3984149301844,-55.24995));
#179351=CARTESIAN_POINT('Ctrl Pts',(52.1075962444343,27.3774879325696,-55.2513479743312));
#179352=CARTESIAN_POINT('Ctrl Pts',(52.1110733300424,27.3573682601684,-55.2538882420798));
#179353=CARTESIAN_POINT('Ctrl Pts',(52.1145448981266,27.3372805141512,-55.2564244788698));
#179354=CARTESIAN_POINT('Ctrl Pts',(52.1178670372207,27.3179969554615,-55.2600986724002));
#179355=CARTESIAN_POINT('Ctrl Pts',(52.1210397473245,27.2996086400427,-55.2646604727451));
#179356=CARTESIAN_POINT('Ctrl Pts',(52.1243513930363,27.2804150850335,-55.2694220381124));
#179357=CARTESIAN_POINT('Ctrl Pts',(52.1275002359685,27.2621965820888,-55.275149957033));
#179358=CARTESIAN_POINT('Ctrl Pts',(52.130486276121,27.2450003125949,-55.281575025852));
#179359=CARTESIAN_POINT('Ctrl Pts',(52.1332354059753,27.2291683828708,-55.2874903342887));
#179360=CARTESIAN_POINT('Ctrl Pts',(52.1358465415646,27.2142018443753,-55.2939965089216));
#179361=CARTESIAN_POINT('Ctrl Pts',(52.138319682889,27.2001025975964,-55.3009008476658));
#179362=CARTESIAN_POINT('Ctrl Pts',(52.1412013074786,27.1836746095095,-55.3089455607216));
#179363=CARTESIAN_POINT('Ctrl Pts',(52.1438955888521,27.1684242891165,-55.3175297932171));
#179364=CARTESIAN_POINT('Ctrl Pts',(52.1464025270093,27.1543108257794,-55.3263826814667));
#179365=CARTESIAN_POINT('Ctrl Pts',(52.1483805817288,27.1431748499345,-55.3333678946174));
#179366=CARTESIAN_POINT('Ctrl Pts',(52.1502420018674,27.1327455689858,-55.3405210924908));
#179367=CARTESIAN_POINT('Ctrl Pts',(52.151986787425,27.1229879533935,-55.3477263606511));
#179368=CARTESIAN_POINT('Ctrl Pts',(52.153964829468,27.1119258639597,-55.3558948850236));
#179369=CARTESIAN_POINT('Ctrl Pts',(52.1557929671545,27.1017269109606,-55.3641299065508));
#179370=CARTESIAN_POINT('Ctrl Pts',(52.1574712004845,27.0923264617539,-55.3722860416452));
#179371=CARTESIAN_POINT('Ctrl Pts',(52.1583103171494,27.0876262371506,-55.3763641091924));
#179372=CARTESIAN_POINT('Ctrl Pts',(52.1591119577253,27.0831254533124,-55.3804228422634));
#179373=CARTESIAN_POINT('Ctrl Pts',(52.1598761222121,27.0788151725342,-55.3844463377003));
#179374=CARTESIAN_POINT('Ctrl Pts',(52.1602582044554,27.0766600321451,-55.3864580854188));
#179375=CARTESIAN_POINT('Ctrl Pts',(52.1606309176765,27.0745525258254,-55.3884610324842));
#179376=CARTESIAN_POINT('Ctrl Pts',(52.1609942618754,27.0724914802186,-55.3904533483054));
#179377=CARTESIAN_POINT('Ctrl Pts',(52.1612198097561,27.0712120749871,-55.3916900891499));
#179378=CARTESIAN_POINT('Ctrl Pts',(52.1613688244011,27.0703718307476,-55.3925105847812));
#179379=CARTESIAN_POINT('Ctrl Pts',(52.1615771078567,27.0691841523735,-55.3936800811369));
#179380=CARTESIAN_POINT('Ctrl Pts',(52.1617043566395,27.0684585516433,-55.3943945737371));
#179381=CARTESIAN_POINT('Ctrl Pts',(52.1618537273994,27.0676035577912,-55.3952396410222));
#179382=CARTESIAN_POINT('Ctrl Pts',(52.1620561874049,27.0664465894067,-55.3963966094067));
#179383=CARTESIAN_POINT('Ctrl Pts',(52.1651986633863,27.0484887445991,-55.4143544542144));
#179384=CARTESIAN_POINT('Ctrl Pts',(52.1680521085855,27.0320748238547,-55.433509382758));
#179385=CARTESIAN_POINT('Ctrl Pts',(52.1706165230026,27.0173083263743,-55.4535728212224));
#179386=CARTESIAN_POINT('Ctrl Pts',(52.1732171913392,27.0023330703531,-55.4739199027201));
#179387=CARTESIAN_POINT('Ctrl Pts',(52.1755205988918,26.9890520084134,-55.4952007603085));
#179388=CARTESIAN_POINT('Ctrl Pts',(52.1775267456605,26.9775195753864,-55.5171172455752));
#179389=CARTESIAN_POINT('Ctrl Pts',(52.1795769127367,26.9657340894641,-55.53951463804));
#179390=CARTESIAN_POINT('Ctrl Pts',(52.1813166304854,26.9557746307472,-55.5625752639374));
#179391=CARTESIAN_POINT('Ctrl Pts',(52.1827458989067,26.9476461596984,-55.5859930896654));
#179392=CARTESIAN_POINT('Ctrl Pts',(52.1841932371623,26.9394149227008,-55.6097069803071));
#179393=CARTESIAN_POINT('Ctrl Pts',(52.1853222266237,26.9330609012905,-55.6337866414178));
#179394=CARTESIAN_POINT('Ctrl Pts',(52.1861328672907,26.928539638511,-55.6579351493319));
#179395=CARTESIAN_POINT('Ctrl Pts',(52.1869587610608,26.9239333031587,-55.6825380382005));
#179396=CARTESIAN_POINT('Ctrl Pts',(52.1874542131553,26.9212289400873,-55.7072119142524));
#179397=CARTESIAN_POINT('Ctrl Pts',(52.1876192235742,26.9203341785897,-55.7316719557658));
#179398=CARTESIAN_POINT('Ctrl Pts',(52.1876604236412,26.9201107730988,-55.7377791783033));
#179399=CARTESIAN_POINT('Ctrl Pts',(52.1876810236747,26.91999998,-55.7438732288818));
#179400=CARTESIAN_POINT('Ctrl Pts',(52.1876810236747,26.91999998,-55.74995));
#179401=CARTESIAN_POINT('',(-83.2809572255632,26.9199999800001,-55.74995));
#179402=CARTESIAN_POINT('Origin',(-83.2809572255632,26.9199999800001,-55.24995));
#179403=CARTESIAN_POINT('',(52.1876810236747,26.91999998,-59.64995));
#179404=CARTESIAN_POINT('',(52.1876810236747,26.91999998,-55.24995));
#179405=CARTESIAN_POINT('Ctrl Pts',(52.1876810236747,26.91999998,-59.64995));
#179406=CARTESIAN_POINT('Ctrl Pts',(52.1876810236604,26.91999998,-59.8463349320561));
#179407=CARTESIAN_POINT('Ctrl Pts',(52.148490902876,26.91999998,-60.0425718399612));
#179408=CARTESIAN_POINT('Ctrl Pts',(51.9976374385487,26.91999998,-60.4053784571341));
#179409=CARTESIAN_POINT('Ctrl Pts',(51.8860334168128,26.91999998,-60.5717700902076));
#179410=CARTESIAN_POINT('Ctrl Pts',(51.6072925605561,26.91999998,-60.8494502533521));
#179411=CARTESIAN_POINT('Ctrl Pts',(51.4402653385482,26.91999998,-60.9606295880611));
#179412=CARTESIAN_POINT('Ctrl Pts',(51.0760728588929,26.91999998,-61.1109090094727));
#179413=CARTESIAN_POINT('Ctrl Pts',(50.8790863580067,26.91999998,-61.149949999985));
#179414=CARTESIAN_POINT('Ctrl Pts',(50.6819512673597,26.91999998,-61.14995));
#179415=CARTESIAN_POINT('Ctrl Pts',(51.1762622162812,20.26999998,-61.14995));
#179416=CARTESIAN_POINT('Ctrl Pts',(51.1762622162812,20.26999998,-60.64995));
#179417=CARTESIAN_POINT('Ctrl Pts',(51.1762622162812,20.76999998,-60.64995));
#179418=CARTESIAN_POINT('Ctrl Pts',(51.3733973069281,20.26999998,-61.149949999985));
#179419=CARTESIAN_POINT('Ctrl Pts',(51.3074086861135,20.2699999799973,-60.6556217969837));
#179420=CARTESIAN_POINT('Ctrl Pts',(51.3081847642104,20.764294621792,-60.64995));
#179421=CARTESIAN_POINT('Ctrl Pts',(51.5703838078145,20.26999998,-61.1109090094727));
#179422=CARTESIAN_POINT('Ctrl Pts',(51.4416901737888,20.2699999799993,-60.6353187454032));
#179423=CARTESIAN_POINT('Ctrl Pts',(51.4400078760636,20.7585935639752,-60.6239226729818));
#179424=CARTESIAN_POINT('Ctrl Pts',(51.9345762874696,20.26999998,-60.9606295880612));
#179425=CARTESIAN_POINT('Ctrl Pts',(51.6930653926326,20.2699999800007,-60.5426326522471));
#179426=CARTESIAN_POINT('Ctrl Pts',(51.6837250128509,20.7480533372398,-60.5237363920407));
#179427=CARTESIAN_POINT('Ctrl Pts',(52.1016035094776,20.26999998,-60.849450253352));
#179428=CARTESIAN_POINT('Ctrl Pts',(51.810372475988,20.2699999799993,-60.4706504746462));
#179429=CARTESIAN_POINT('Ctrl Pts',(51.7954994139911,20.7432193417859,-60.4496168355681));
#179430=CARTESIAN_POINT('Ctrl Pts',(52.3803443657342,20.26999998,-60.5717700902076));
#179431=CARTESIAN_POINT('Ctrl Pts',(52.007303090053,20.2699999800007,-60.2852157712124));
#179432=CARTESIAN_POINT('Ctrl Pts',(51.9820324348179,20.7351522014979,-60.264496726805));
#179433=CARTESIAN_POINT('Ctrl Pts',(52.4919483874702,20.26999998,-60.4053784571342));
#179434=CARTESIAN_POINT('Ctrl Pts',(52.0873212216015,20.2699999800003,-60.1718710142637));
#179435=CARTESIAN_POINT('Ctrl Pts',(52.0567177019522,20.7319222289985,-60.153568971423));
#179436=CARTESIAN_POINT('Ctrl Pts',(52.6428018517975,20.26999998,-60.0425718399611));
#179437=CARTESIAN_POINT('Ctrl Pts',(52.1954330376997,20.2699999799997,-59.9224177216067));
#179438=CARTESIAN_POINT('Ctrl Pts',(52.1576686453522,20.7275563241362,-59.9116978933072));
#179439=CARTESIAN_POINT('Ctrl Pts',(52.6819919725819,20.26999998,-59.8463349320562));
#179440=CARTESIAN_POINT('Ctrl Pts',(52.2238263855712,20.2699999800007,-59.7861314644994));
#179441=CARTESIAN_POINT('Ctrl Pts',(52.1838946235501,20.7264221086281,-59.7808732880376));
#179442=CARTESIAN_POINT('Ctrl Pts',(52.6819919725962,20.26999998,-59.64995));
#179443=CARTESIAN_POINT('Ctrl Pts',(52.2238263855875,20.26999998,-59.6499499999999));
#179444=CARTESIAN_POINT('Ctrl Pts',(52.1838946235503,20.7264221086262,-59.64995));
#179445=CARTESIAN_POINT('',(52.1838946235503,20.7264221086262,-59.64995));
#179446=CARTESIAN_POINT('Ctrl Pts',(52.1838946235503,20.7264221086262,-59.64995));
#179447=CARTESIAN_POINT('Ctrl Pts',(52.1838946235503,20.7264221086262,-59.6947437539778));
#179448=CARTESIAN_POINT('Ctrl Pts',(52.1808240197036,20.7265549054463,-59.7400065133852));
#179449=CARTESIAN_POINT('Ctrl Pts',(52.1745699365138,20.7268253807018,-59.785317218617));
#179450=CARTESIAN_POINT('Ctrl Pts',(52.1683919881554,20.7270925632944,-59.8300763285467));
#179451=CARTESIAN_POINT('Ctrl Pts',(52.1591075803806,20.7274940933811,-59.874882258569));
#179452=CARTESIAN_POINT('Ctrl Pts',(52.1466156002861,20.7280343438711,-59.91927914191));
#179453=CARTESIAN_POINT('Ctrl Pts',(52.1368250627133,20.7284577629512,-59.9540750150364));
#179454=CARTESIAN_POINT('Ctrl Pts',(52.1250643954463,20.72896638578,-59.9886186680186));
#179455=CARTESIAN_POINT('Ctrl Pts',(52.1112883978351,20.7295621671856,-60.0226684878138));
#179456=CARTESIAN_POINT('Ctrl Pts',(52.1099425720032,20.729620371174,-60.0259949348954));
#179457=CARTESIAN_POINT('Ctrl Pts',(52.1085775109265,20.7296794070442,-60.0293166614888));
#179458=CARTESIAN_POINT('Ctrl Pts',(52.1071931736522,20.7297392765673,-60.0326334323651));
#179459=CARTESIAN_POINT('Ctrl Pts',(52.0893716054534,20.7305100199466,-60.0753326065261));
#179460=CARTESIAN_POINT('Ctrl Pts',(52.068358068671,20.7314188089021,-60.1171993188295));
#179461=CARTESIAN_POINT('Ctrl Pts',(52.0442398100001,20.7324618702076,-60.1577697846088));
#179462=CARTESIAN_POINT('Ctrl Pts',(52.021198598004,20.7334583516282,-60.1965284991394));
#179463=CARTESIAN_POINT('Ctrl Pts',(51.9953247642768,20.7345773376692,-60.23410319777));
#179464=CARTESIAN_POINT('Ctrl Pts',(51.9667120967645,20.7358147722093,-60.270056968504));
#179465=CARTESIAN_POINT('Ctrl Pts',(51.9532635303856,20.7363963929389,-60.2869560105833));
#179466=CARTESIAN_POINT('Ctrl Pts',(51.9392101206412,20.7370041718053,-60.3034964084302));
#179467=CARTESIAN_POINT('Ctrl Pts',(51.9245639326311,20.7376375870196,-60.3196288077707));
#179468=CARTESIAN_POINT('Ctrl Pts',(51.9193722879604,20.7378621141607,-60.3253472708277));
#179469=CARTESIAN_POINT('Ctrl Pts',(51.9138292978107,20.7381018362176,-60.3313130457146));
#179470=CARTESIAN_POINT('Ctrl Pts',(51.9083020107728,20.7383408744029,-60.3371156970632));
#179471=CARTESIAN_POINT('Ctrl Pts',(51.9026094979459,20.738587058096,-60.3430918055961));
#179472=CARTESIAN_POINT('Ctrl Pts',(51.8969338042165,20.7388325093651,-60.348894747494));
#179473=CARTESIAN_POINT('Ctrl Pts',(51.8917172134375,20.7390580952084,-60.3541155162049));
#179474=CARTESIAN_POINT('Ctrl Pts',(51.8907153144978,20.7391014212477,-60.3551182175586));
#179475=CARTESIAN_POINT('Ctrl Pts',(51.8897304598568,20.7391440097811,-60.3560995558751));
#179476=CARTESIAN_POINT('Ctrl Pts',(51.8887659266967,20.7391857190408,-60.3570567834876));
#179477=CARTESIAN_POINT('Ctrl Pts',(51.8668421914293,20.7401337660398,-60.3788144644414));
#179478=CARTESIAN_POINT('Ctrl Pts',(51.8432494089284,20.7411541156338,-60.4001952301119));
#179479=CARTESIAN_POINT('Ctrl Pts',(51.8179330401853,20.7422490327724,-60.4209274431457));
#179480=CARTESIAN_POINT('Ctrl Pts',(51.7930740583666,20.7433241682122,-60.4412850904884));
#179481=CARTESIAN_POINT('Ctrl Pts',(51.7665529367326,20.7444712128588,-60.4610175327789));
#179482=CARTESIAN_POINT('Ctrl Pts',(51.7383500788444,20.7456909240398,-60.479830648501));
#179483=CARTESIAN_POINT('Ctrl Pts',(51.7115168807664,20.7468514004655,-60.4977301132515));
#179484=CARTESIAN_POINT('Ctrl Pts',(51.68315997536,20.7480777738606,-60.514798285487));
#179485=CARTESIAN_POINT('Ctrl Pts',(51.6532906522493,20.749369555974,-60.5307488752741));
#179486=CARTESIAN_POINT('Ctrl Pts',(51.6242323211694,20.750626264477,-60.5462663852369));
#179487=CARTESIAN_POINT('Ctrl Pts',(51.5937419188686,20.7519449068907,-60.5607262880017));
#179488=CARTESIAN_POINT('Ctrl Pts',(51.5618664444573,20.7533234506075,-60.5738295325113));
#179489=CARTESIAN_POINT('Ctrl Pts',(51.5613426081777,20.7533461053672,-60.5740448690664));
#179490=CARTESIAN_POINT('Ctrl Pts',(51.5608184003988,20.7533687761933,-60.5742598379299));
#179491=CARTESIAN_POINT('Ctrl Pts',(51.5602938213872,20.7533914630745,-60.5744744380412));
#179492=CARTESIAN_POINT('Ctrl Pts',(51.5576607263164,20.7535053386084,-60.5755516113222));
#179493=CARTESIAN_POINT('Ctrl Pts',(51.5543108831315,20.753650197033,-60.5769043222577));
#179494=CARTESIAN_POINT('Ctrl Pts',(51.5515275695402,20.7537705514875,-60.5780123790108));
#179495=CARTESIAN_POINT('Ctrl Pts',(51.5497122359956,20.7538490491025,-60.5787350760865));
#179496=CARTESIAN_POINT('Ctrl Pts',(51.5481384565771,20.7539170988375,-60.5793550577197));
#179497=CARTESIAN_POINT('Ctrl Pts',(51.5471658588221,20.7539591509512,-60.5797369926547));
#179498=CARTESIAN_POINT('Ctrl Pts',(51.5316110315242,20.7546316934927,-60.5858453061108));
#179499=CARTESIAN_POINT('Ctrl Pts',(51.5143868745062,20.7553764998629,-60.592164096532));
#179500=CARTESIAN_POINT('Ctrl Pts',(51.4954289880907,20.7561963347601,-60.5984375211913));
#179501=CARTESIAN_POINT('Ctrl Pts',(51.4761457702625,20.7570302386331,-60.6048186024775));
#179502=CARTESIAN_POINT('Ctrl Pts',(51.45506778427,20.757941812513,-60.6111530886455));
#179503=CARTESIAN_POINT('Ctrl Pts',(51.4321472453672,20.7589331013641,-60.6171173698262));
#179504=CARTESIAN_POINT('Ctrl Pts',(51.411456364092,20.7598279599018,-60.6225014593681));
#179505=CARTESIAN_POINT('Ctrl Pts',(51.3892636144662,20.7607877942596,-60.627583296186));
#179506=CARTESIAN_POINT('Ctrl Pts',(51.3655588032748,20.7618130292197,-60.6320843346823));
#179507=CARTESIAN_POINT('Ctrl Pts',(51.342619113597,20.7628051726138,-60.636440092908));
#179508=CARTESIAN_POINT('Ctrl Pts',(51.3182628753082,20.7638585854262,-60.6402518751315));
#179509=CARTESIAN_POINT('Ctrl Pts',(51.2925119970447,20.7649723054284,-60.6432310343638));
#179510=CARTESIAN_POINT('Ctrl Pts',(51.2679457061843,20.7660347922777,-60.6460731468337));
#179511=CARTESIAN_POINT('Ctrl Pts',(51.2421097939689,20.7671521802492,-60.6481573437467));
#179512=CARTESIAN_POINT('Ctrl Pts',(51.2150580998752,20.7683221279269,-60.6492010672739));
#179513=CARTESIAN_POINT('Ctrl Pts',(51.2023893520667,20.7688700334307,-60.6496898599573));
#179514=CARTESIAN_POINT('Ctrl Pts',(51.1894544995639,20.7694294429471,-60.64995));
#179515=CARTESIAN_POINT('Ctrl Pts',(51.1762622162812,20.76999998,-60.64995));
#179516=CARTESIAN_POINT('Origin',(52.6819919725962,20.76999998,-59.64995));
#179517=CARTESIAN_POINT('Ctrl Pts',(52.1876810236747,26.91999998,-59.64995));
#179518=CARTESIAN_POINT('Ctrl Pts',(51.6420267731401,26.91999998,-59.64995));
#179519=CARTESIAN_POINT('Ctrl Pts',(51.6895836746289,26.3764221086262,-59.64995));
#179520=CARTESIAN_POINT('Ctrl Pts',(52.1876810236604,26.91999998,-59.8463349320561));
#179521=CARTESIAN_POINT('Ctrl Pts',(51.6420267731333,26.919999980002,-59.7746029379318));
#179522=CARTESIAN_POINT('Ctrl Pts',(51.6895836746287,26.3764221086278,-59.7808732880375));
#179523=CARTESIAN_POINT('Ctrl Pts',(52.148490902876,26.91999998,-60.0425718399612));
#179524=CARTESIAN_POINT('Ctrl Pts',(51.6186060348034,26.9199999800004,-59.8989712332639));
#179525=CARTESIAN_POINT('Ctrl Pts',(51.6633576964307,26.3775563241358,-59.9116978933072));
#179526=CARTESIAN_POINT('Ctrl Pts',(51.9976374385487,26.91999998,-60.4053784571341));
#179527=CARTESIAN_POINT('Ctrl Pts',(51.5267774915774,26.9199999799997,-60.1322291512607));
#179528=CARTESIAN_POINT('Ctrl Pts',(51.5624067530308,26.3819222289988,-60.1535689714229));
#179529=CARTESIAN_POINT('Ctrl Pts',(51.8860334168128,26.91999998,-60.5717700902076));
#179530=CARTESIAN_POINT('Ctrl Pts',(51.4587108395762,26.9199999799996,-60.2406767152617));
#179531=CARTESIAN_POINT('Ctrl Pts',(51.4877214858962,26.3851522014976,-60.2644967268053));
#179532=CARTESIAN_POINT('Ctrl Pts',(51.6072925605561,26.91999998,-60.8494502533521));
#179533=CARTESIAN_POINT('Ctrl Pts',(51.2846839917031,26.9199999800004,-60.4261994932779));
#179534=CARTESIAN_POINT('Ctrl Pts',(51.3011884650699,26.3932193417862,-60.4496168355678));
#179535=CARTESIAN_POINT('Ctrl Pts',(51.4402653385482,26.91999998,-60.9606295880611));
#179536=CARTESIAN_POINT('Ctrl Pts',(51.1792534074218,26.9199999799993,-60.5031527166058));
#179537=CARTESIAN_POINT('Ctrl Pts',(51.1894140639292,26.3980533372399,-60.5237363920408));
#179538=CARTESIAN_POINT('Ctrl Pts',(51.0760728588929,26.91999998,-61.1109090094727));
#179539=CARTESIAN_POINT('Ctrl Pts',(50.9439864347103,26.9199999800007,-60.6120353079387));
#179540=CARTESIAN_POINT('Ctrl Pts',(50.9456969271423,26.4085935639752,-60.6239226729817));
#179541=CARTESIAN_POINT('Ctrl Pts',(50.8790863580067,26.91999998,-61.149949999985));
#179542=CARTESIAN_POINT('Ctrl Pts',(50.8146696888639,26.9199999800028,-60.6442102195338));
#179543=CARTESIAN_POINT('Ctrl Pts',(50.8138738152888,26.4142946217921,-60.64995));
#179544=CARTESIAN_POINT('Ctrl Pts',(50.6819512673597,26.91999998,-61.14995));
#179545=CARTESIAN_POINT('Ctrl Pts',(50.6819512673597,26.91999998,-60.64995));
#179546=CARTESIAN_POINT('Ctrl Pts',(50.6819512673597,26.41999998,-60.64995));
#179547=CARTESIAN_POINT('',(51.6895836746288,26.3764221086262,-59.64995));
#179548=CARTESIAN_POINT('Origin',(52.1876810236747,26.41999998,-59.64995));
#179549=CARTESIAN_POINT('Ctrl Pts',(50.6819512673597,26.41999998,-60.64995));
#179550=CARTESIAN_POINT('Ctrl Pts',(50.7109216498289,26.4187470750797,-60.64995));
#179551=CARTESIAN_POINT('Ctrl Pts',(50.7386501990522,26.4175587192038,-60.6487118041208));
#179552=CARTESIAN_POINT('Ctrl Pts',(50.765056036357,26.4164278364053,-60.6465429519636));
#179553=CARTESIAN_POINT('Ctrl Pts',(50.7925707013286,26.415249465844,-60.6442830258803));
#179554=CARTESIAN_POINT('Ctrl Pts',(50.8186497119696,26.4141335381347,-60.6410132281087));
#179555=CARTESIAN_POINT('Ctrl Pts',(50.8432520459097,26.4130764642849,-60.6370534672329));
#179556=CARTESIAN_POINT('Ctrl Pts',(50.8636595387387,26.4121996276782,-60.6337688686304));
#179557=CARTESIAN_POINT('Ctrl Pts',(50.8830521268965,26.4113633856883,-60.6300090683738));
#179558=CARTESIAN_POINT('Ctrl Pts',(50.9014271157008,26.4105675025612,-60.6259392752378));
#179559=CARTESIAN_POINT('Ctrl Pts',(50.9247296256716,26.4095581917691,-60.6207781077323));
#179560=CARTESIAN_POINT('Ctrl Pts',(50.9463951635552,26.4086137504418,-60.6151198746454));
#179561=CARTESIAN_POINT('Ctrl Pts',(50.9664496076967,26.4077364426411,-60.6092623723524));
#179562=CARTESIAN_POINT('Ctrl Pts',(50.9729822346157,26.407450664361,-60.6073543226011));
#179563=CARTESIAN_POINT('Ctrl Pts',(50.9793441339268,26.4071720292579,-60.6054247759641));
#179564=CARTESIAN_POINT('Ctrl Pts',(50.9855367745778,26.4069006658479,-60.6034830010953));
#179565=CARTESIAN_POINT('Ctrl Pts',(50.9981384568014,26.4063484562733,-60.5995315963188));
#179566=CARTESIAN_POINT('Ctrl Pts',(51.0100390679368,26.4058263438341,-60.5955300977548));
#179567=CARTESIAN_POINT('Ctrl Pts',(51.021253530521,26.4053356340831,-60.5915501614527));
#179568=CARTESIAN_POINT('Ctrl Pts',(51.0268607618131,26.4050902792076,-60.5895601933016));
#179569=CARTESIAN_POINT('Ctrl Pts',(51.0322964183045,26.4048527717091,-60.5875755119569));
#179570=CARTESIAN_POINT('Ctrl Pts',(51.0375626846602,26.4046233027209,-60.5856042390701));
#179571=CARTESIAN_POINT('Ctrl Pts',(51.040195817838,26.4045085682269,-60.5846186026267));
#179572=CARTESIAN_POINT('Ctrl Pts',(51.0427866011158,26.4043958431534,-60.5836363114303));
#179573=CARTESIAN_POINT('Ctrl Pts',(51.0453353024098,26.4042851509401,-60.5826583364025));
#179574=CARTESIAN_POINT('Ctrl Pts',(51.0470835270635,26.404209224092,-60.5819875163034));
#179575=CARTESIAN_POINT('Ctrl Pts',(51.0479000495842,26.4041734759918,-60.5816721106921));
#179576=CARTESIAN_POINT('Ctrl Pts',(51.0496620341368,26.4040972539742,-60.5809867219938));
#179577=CARTESIAN_POINT('Ctrl Pts',(51.0504688111559,26.404062353457,-60.5806728963985));
#179578=CARTESIAN_POINT('Ctrl Pts',(51.0514736835841,26.4040189565482,-60.5802811765921));
#179579=CARTESIAN_POINT('Ctrl Pts',(51.0528554256585,26.4039591960934,-60.5797383010624));
#179580=CARTESIAN_POINT('Ctrl Pts',(51.0861692753423,26.4025183694385,-60.566649553076));
#179581=CARTESIAN_POINT('Ctrl Pts',(51.1180339754858,26.4011478167948,-60.5520895212465));
#179582=CARTESIAN_POINT('Ctrl Pts',(51.148380750499,26.3998415210777,-60.5363617345489));
#179583=CARTESIAN_POINT('Ctrl Pts',(51.1795224235809,26.3985010084812,-60.5202219769825));
#179584=CARTESIAN_POINT('Ctrl Pts',(51.2090659248564,26.3972281907555,-60.502852974953));
#179585=CARTESIAN_POINT('Ctrl Pts',(51.2369879076331,26.3960210253296,-60.4845643919205));
#179586=CARTESIAN_POINT('Ctrl Pts',(51.2393489032447,26.3959189511934,-60.4830179664884));
#179587=CARTESIAN_POINT('Ctrl Pts',(51.2416983328603,26.3958173488807,-60.481464953118));
#179588=CARTESIAN_POINT('Ctrl Pts',(51.244036197333,26.3957162184661,-60.4799055315775));
#179589=CARTESIAN_POINT('Ctrl Pts',(51.2725006891055,26.3944849127654,-60.4609189127518));
#179590=CARTESIAN_POINT('Ctrl Pts',(51.2992471043443,26.3933232424756,-60.4409847510347));
#179591=CARTESIAN_POINT('Ctrl Pts',(51.3243014907345,26.3922334864741,-60.4204120406075));
#179592=CARTESIAN_POINT('Ctrl Pts',(51.3368286839295,26.3916886084733,-60.4101256853938));
#179593=CARTESIAN_POINT('Ctrl Pts',(51.3489335585763,26.3911617692948,-60.3996792358246));
#179594=CARTESIAN_POINT('Ctrl Pts',(51.360623110838,26.3906535810237,-60.389108443085));
#179595=CARTESIAN_POINT('Ctrl Pts',(51.3660749779834,26.3904165681016,-60.384178351979));
#179596=CARTESIAN_POINT('Ctrl Pts',(51.3711148667758,26.3901960942943,-60.37951815644));
#179597=CARTESIAN_POINT('Ctrl Pts',(51.376199160571,26.3899752512413,-60.3747215662517));
#179598=CARTESIAN_POINT('Ctrl Pts',(51.3811440975544,26.3897604613364,-60.3700564471277));
#179599=CARTESIAN_POINT('Ctrl Pts',(51.3861311904196,26.3895453354251,-60.3652622207859));
#179600=CARTESIAN_POINT('Ctrl Pts',(51.3915473108369,26.3893114302946,-60.359930701075));
#179601=CARTESIAN_POINT('Ctrl Pts',(51.3925026124315,26.3892701738367,-60.3589903214509));
#179602=CARTESIAN_POINT('Ctrl Pts',(51.3934711686472,26.3892283250534,-60.3580331355661));
#179603=CARTESIAN_POINT('Ctrl Pts',(51.394454975483,26.3891857716419,-60.3570567811865));
#179604=CARTESIAN_POINT('Ctrl Pts',(51.4248855109459,26.3878695345018,-60.3268567607239));
#179605=CARTESIAN_POINT('Ctrl Pts',(51.4531160540184,26.3866685076191,-60.2949641541493));
#179606=CARTESIAN_POINT('Ctrl Pts',(51.4790191152461,26.3855715371119,-60.2617220237277));
#179607=CARTESIAN_POINT('Ctrl Pts',(51.5052296625032,26.3844615448578,-60.2280852877958));
#179608=CARTESIAN_POINT('Ctrl Pts',(51.5290572452464,26.3834581030612,-60.1930673111176));
#179609=CARTESIAN_POINT('Ctrl Pts',(51.5504233097089,26.3825543391582,-60.1570220983849));
#179610=CARTESIAN_POINT('Ctrl Pts',(51.5720480957387,26.3816396315826,-60.120540414352));
#179611=CARTESIAN_POINT('Ctrl Pts',(51.5911515653163,26.380827045893,-60.0830069552923));
#179612=CARTESIAN_POINT('Ctrl Pts',(51.6077046707207,26.3801140407432,-60.0447796547702));
#179613=CARTESIAN_POINT('Ctrl Pts',(51.624565766262,26.3793877692879,-60.0058410900331));
#179614=CARTESIAN_POINT('Ctrl Pts',(51.6387809076029,26.3787648357948,-59.9661831063249));
#179615=CARTESIAN_POINT('Ctrl Pts',(51.6503706558839,26.3782470391306,-59.9261671554418));
#179616=CARTESIAN_POINT('Ctrl Pts',(51.662085110263,26.3777236709561,-59.8857206315231));
#179617=CARTESIAN_POINT('Ctrl Pts',(51.6711176986419,26.377307743177,-59.8449088096299));
#179618=CARTESIAN_POINT('Ctrl Pts',(51.6775374166152,26.3770052921258,-59.8040810754937));
#179619=CARTESIAN_POINT('Ctrl Pts',(51.684058954154,26.3766980440672,-59.7626057954429));
#179620=CARTESIAN_POINT('Ctrl Pts',(51.6878844348378,26.3765079317815,-59.7211144794873));
#179621=CARTESIAN_POINT('Ctrl Pts',(51.6891300584881,26.3764451214357,-59.6799427690583));
#179622=CARTESIAN_POINT('Ctrl Pts',(51.6894331426085,26.3764298384741,-59.669924902395));
#179623=CARTESIAN_POINT('Ctrl Pts',(51.6895836746288,26.3764221086262,-59.6599258028449));
#179624=CARTESIAN_POINT('Ctrl Pts',(51.6895836746288,26.3764221086262,-59.64995));
#179625=CARTESIAN_POINT('Origin',(0.,-12.9675000200281,-60.64995));
#179626=CARTESIAN_POINT('',(53.7167487055517,-8.26789346682159,-60.64995));
#179627=CARTESIAN_POINT('Origin',(37.5,-9.33460238845303,-92.34995));
#179628=CARTESIAN_POINT('',(37.5,29.41999998,-91.84995));
#179629=CARTESIAN_POINT('',(37.5,39.429060187817,-59.64995));
#179630=CARTESIAN_POINT('Ctrl Pts',(37.5,37.923330431502,-61.14995));
#179631=CARTESIAN_POINT('Ctrl Pts',(37.5,38.1204655221491,-61.149949999985));
#179632=CARTESIAN_POINT('Ctrl Pts',(37.5,38.3174520230353,-61.1109090094727));
#179633=CARTESIAN_POINT('Ctrl Pts',(37.5,38.6816445026906,-60.9606295880611));
#179634=CARTESIAN_POINT('Ctrl Pts',(37.5,38.8486717246983,-60.8494502533514));
#179635=CARTESIAN_POINT('Ctrl Pts',(37.5,39.1274125809551,-60.5717700902082));
#179636=CARTESIAN_POINT('Ctrl Pts',(37.5,39.239016602691,-60.4053784571342));
#179637=CARTESIAN_POINT('Ctrl Pts',(37.5,39.3898700670183,-60.0425718399611));
#179638=CARTESIAN_POINT('Ctrl Pts',(37.5,39.4290601878028,-59.8463349320561));
#179639=CARTESIAN_POINT('Ctrl Pts',(37.5,39.4290601878171,-59.64995));
#179640=CARTESIAN_POINT('',(37.5,39.4290601878171,-55.74995));
#179641=CARTESIAN_POINT('',(37.5,39.4290601878171,-92.34995));
#179642=CARTESIAN_POINT('',(37.5,43.91999998,-55.74995));
#179643=CARTESIAN_POINT('Origin',(38.,-9.33460238845303,-55.74995));
#179644=CARTESIAN_POINT('',(38.,39.3415715242911,-55.24995));
#179645=CARTESIAN_POINT('Ctrl Pts',(37.5,39.4290601878171,-55.74995));
#179646=CARTESIAN_POINT('Ctrl Pts',(37.5,39.429060187816,-55.7240274876821));
#179647=CARTESIAN_POINT('Ctrl Pts',(37.5021037800324,39.4286870411454,-55.6978059978133));
#179648=CARTESIAN_POINT('Ctrl Pts',(37.5063531399508,39.4279374079327,-55.6716073785487));
#179649=CARTESIAN_POINT('Ctrl Pts',(37.5106395376341,39.4271812408562,-55.6451804099992));
#179650=CARTESIAN_POINT('Ctrl Pts',(37.5171091146894,39.4260419907227,-55.6187767699276));
#179651=CARTESIAN_POINT('Ctrl Pts',(37.5257761108222,39.4245212417519,-55.5927712420142));
#179652=CARTESIAN_POINT('Ctrl Pts',(37.5290201828345,39.423952022717,-55.5830373268288));
#179653=CARTESIAN_POINT('Ctrl Pts',(37.5325718289255,39.4233294053315,-55.573359626286));
#179654=CARTESIAN_POINT('Ctrl Pts',(37.5364307642167,39.4226536524692,-55.5637593428668));
#179655=CARTESIAN_POINT('Ctrl Pts',(37.5465845612258,39.4208755823864,-55.5384986629866));
#179656=CARTESIAN_POINT('Ctrl Pts',(37.5588727550735,39.4187275751124,-55.5137551371743));
#179657=CARTESIAN_POINT('Ctrl Pts',(37.5732950204316,39.4162093248656,-55.489926848832));
#179658=CARTESIAN_POINT('Ctrl Pts',(37.5761937619161,39.4157031799378,-55.4851375840245));
#179659=CARTESIAN_POINT('Ctrl Pts',(37.5791786699961,39.4151820858751,-55.480385454335));
#179660=CARTESIAN_POINT('Ctrl Pts',(37.5822496741218,39.4146460520141,-55.4756739402145));
#179661=CARTESIAN_POINT('Ctrl Pts',(37.5914248426836,39.413044555947,-55.4615974575831));
#179662=CARTESIAN_POINT('Ctrl Pts',(37.6013686732816,39.4113095928738,-55.447883452059));
#179663=CARTESIAN_POINT('Ctrl Pts',(37.6120727310924,39.4094411426509,-55.4346345056758));
#179664=CARTESIAN_POINT('Ctrl Pts',(37.6174247599977,39.4085069175394,-55.4280100324842));
#179665=CARTESIAN_POINT('Ctrl Pts',(37.6229667921261,39.4075393211592,-55.4215019155803));
#179666=CARTESIAN_POINT('Ctrl Pts',(37.6286966355404,39.4065383550014,-55.4151241749086));
#179667=CARTESIAN_POINT('Ctrl Pts',(37.6315615572476,39.4060378719225,-55.4119353045727));
#179668=CARTESIAN_POINT('Ctrl Pts',(37.6344734223788,39.4055290464556,-55.4087790343616));
#179669=CARTESIAN_POINT('Ctrl Pts',(37.6374318784904,39.4050118790486,-55.405657167355));
#179670=CARTESIAN_POINT('Ctrl Pts',(37.6391534315316,39.4047109345394,-55.4038405239988));
#179671=CARTESIAN_POINT('Ctrl Pts',(37.6412508897064,39.4043441565208,-55.4016627141526));
#179672=CARTESIAN_POINT('Ctrl Pts',(37.6430986611541,39.4040209803381,-55.39977793316));
#179673=CARTESIAN_POINT('Ctrl Pts',(37.6444262497453,39.4037887844064,-55.3984237539156));
#179674=CARTESIAN_POINT('Ctrl Pts',(37.6456236044489,39.4035793311953,-55.39721961437));
#179675=CARTESIAN_POINT('Ctrl Pts',(37.6464466082408,39.4034353248945,-55.3963966105727));
#179676=CARTESIAN_POINT('Ctrl Pts',(37.6562264477315,39.401724083074,-55.3866167710176));
#179677=CARTESIAN_POINT('Ctrl Pts',(37.6671430152984,39.3997858357212,-55.3765446165109));
#179678=CARTESIAN_POINT('Ctrl Pts',(37.6793251261276,39.3976147412181,-55.3664154209167));
#179679=CARTESIAN_POINT('Ctrl Pts',(37.6909838912123,39.3955369173381,-55.3567213774471));
#179680=CARTESIAN_POINT('Ctrl Pts',(37.7038025095349,39.3932457018356,-55.3469750520182));
#179681=CARTESIAN_POINT('Ctrl Pts',(37.7178716381578,39.3907398007779,-55.3374234995767));
#179682=CARTESIAN_POINT('Ctrl Pts',(37.7311276745897,39.3883787223767,-55.3284239566384));
#179683=CARTESIAN_POINT('Ctrl Pts',(37.7454943046515,39.3858269816568,-55.3195974073024));
#179684=CARTESIAN_POINT('Ctrl Pts',(37.7610192152964,39.3830883066716,-55.3111870422691));
#179685=CARTESIAN_POINT('Ctrl Pts',(37.7672465764655,39.3819897677719,-55.3078134717654));
#179686=CARTESIAN_POINT('Ctrl Pts',(37.7736599367756,39.3808612138681,-55.3045072863542));
#179687=CARTESIAN_POINT('Ctrl Pts',(37.7802607448068,39.3797031624633,-55.3012859403588));
#179688=CARTESIAN_POINT('Ctrl Pts',(37.7954942140763,39.3770305895897,-55.293851657314));
#179689=CARTESIAN_POINT('Ctrl Pts',(37.8117391205314,39.3742062568083,-55.286861963903));
#179690=CARTESIAN_POINT('Ctrl Pts',(37.8289873345872,39.3712188581417,-55.2805581079215));
#179691=CARTESIAN_POINT('Ctrl Pts',(37.8457634286169,39.3683132308824,-55.2744268017843));
#179692=CARTESIAN_POINT('Ctrl Pts',(37.8634889697662,39.3652532832896,-55.268944278674));
#179693=CARTESIAN_POINT('Ctrl Pts',(37.882119830396,39.3620351392646,-55.2643620188825));
#179694=CARTESIAN_POINT('Ctrl Pts',(37.9001775050072,39.3589160027518,-55.2599207341804));
#179695=CARTESIAN_POINT('Ctrl Pts',(37.9190858710086,39.3556482116274,-55.2563251747639));
#179696=CARTESIAN_POINT('Ctrl Pts',(37.9387660359793,39.3522351790126,-55.2538325278281));
#179697=CARTESIAN_POINT('Ctrl Pts',(37.9584462009501,39.3488221463977,-55.2513398808923));
#179698=CARTESIAN_POINT('Ctrl Pts',(37.9788985693902,39.3452637962159,-55.24995));
#179699=CARTESIAN_POINT('Ctrl Pts',(38.,39.3415715242911,-55.24995));
#179700=CARTESIAN_POINT('',(38.,38.8834059372824,-55.24995));
#179701=CARTESIAN_POINT('Origin',(0.,0.,-55.24995));
#179702=CARTESIAN_POINT('',(38.5,39.2978271925282,-55.24995));
#179703=CARTESIAN_POINT('',(38.5435778713738,39.2940146228024,-55.24995));
#179704=CARTESIAN_POINT('',(38.5,-1.68631645800828E-14,-55.24995));
#179705=CARTESIAN_POINT('Origin',(38.5,-1.68631645800828E-14,-55.74995));
#179706=CARTESIAN_POINT('',(39.,39.2103385290022,-55.74995));
#179707=CARTESIAN_POINT('Ctrl Pts',(38.5,39.2978271925282,-55.24995));
#179708=CARTESIAN_POINT('Ctrl Pts',(38.5215850497934,39.294050298211,-55.24995));
#179709=CARTESIAN_POINT('Ctrl Pts',(38.5424891944466,39.2903925468554,-55.2514041468222));
#179710=CARTESIAN_POINT('Ctrl Pts',(38.562582249786,39.2868767177398,-55.2540052053726));
#179711=CARTESIAN_POINT('Ctrl Pts',(38.5825281794975,39.2833866322734,-55.2565872184188));
#179712=CARTESIAN_POINT('Ctrl Pts',(38.6016753789192,39.2800363064982,-55.2602996172285));
#179713=CARTESIAN_POINT('Ctrl Pts',(38.6199435823765,39.2768397850872,-55.2648742466984));
#179714=CARTESIAN_POINT('Ctrl Pts',(38.6390429090693,39.2734978359541,-55.2696570017704));
#179715=CARTESIAN_POINT('Ctrl Pts',(38.657181623243,39.2703239722319,-55.2753821626628));
#179716=CARTESIAN_POINT('Ctrl Pts',(38.67431472958,39.267326067081,-55.2817780783575));
#179717=CARTESIAN_POINT('Ctrl Pts',(38.6903193474662,39.2645256218228,-55.2877527209421));
#179718=CARTESIAN_POINT('Ctrl Pts',(38.7054472589132,39.261878580314,-55.2943131224831));
#179719=CARTESIAN_POINT('Ctrl Pts',(38.7196931730899,39.2593858683299,-55.3012636512163));
#179720=CARTESIAN_POINT('Ctrl Pts',(38.7362431769865,39.2564899928853,-55.309338336785));
#179721=CARTESIAN_POINT('Ctrl Pts',(38.7516127664062,39.2538006632106,-55.317943762193));
#179722=CARTESIAN_POINT('Ctrl Pts',(38.7658371701146,39.2513117150707,-55.3268178701208));
#179723=CARTESIAN_POINT('Ctrl Pts',(38.7811342644143,39.2486350703984,-55.3363611921875));
#179724=CARTESIAN_POINT('Ctrl Pts',(38.795107859426,39.2461900080939,-55.346215423425));
#179725=CARTESIAN_POINT('Ctrl Pts',(38.8078412626453,39.2439619512343,-55.3561026478009));
#179726=CARTESIAN_POINT('Ctrl Pts',(38.820796298757,39.2416951136435,-55.3661619655362));
#179727=CARTESIAN_POINT('Ctrl Pts',(38.8324678161029,39.2396528627357,-55.3762552368417));
#179728=CARTESIAN_POINT('Ctrl Pts',(38.8429723612382,39.237814805506,-55.3861352302201));
#179729=CARTESIAN_POINT('Ctrl Pts',(38.844508436647,39.2375460271368,-55.3875799776767));
#179730=CARTESIAN_POINT('Ctrl Pts',(38.8460195962369,39.2372816084711,-55.3890202398763));
#179731=CARTESIAN_POINT('Ctrl Pts',(38.8475062515775,39.2370214774933,-55.3904553319087));
#179732=CARTESIAN_POINT('Ctrl Pts',(38.8487711127112,39.236800155473,-55.3916763224674));
#179733=CARTESIAN_POINT('Ctrl Pts',(38.8496069371356,39.2366539051479,-55.3924916493941));
#179734=CARTESIAN_POINT('Ctrl Pts',(38.8507725352525,39.2364499420131,-55.3936383710039));
#179735=CARTESIAN_POINT('Ctrl Pts',(38.8515075974215,39.2363213165615,-55.3943615290645));
#179736=CARTESIAN_POINT('Ctrl Pts',(38.8523735525978,39.2361697838677,-55.3952167714236));
#179737=CARTESIAN_POINT('Ctrl Pts',(38.8535533887318,39.2359633227174,-55.3963966075452));
#179738=CARTESIAN_POINT('Ctrl Pts',(38.8741274018139,39.2323630478275,-55.4169706204106));
#179739=CARTESIAN_POINT('Ctrl Pts',(38.8925747282859,39.2291350207311,-55.4391630479274));
#179740=CARTESIAN_POINT('Ctrl Pts',(38.9088523573029,39.2262867255737,-55.4624843710786));
#179741=CARTESIAN_POINT('Ctrl Pts',(38.9251500795738,39.2234349144546,-55.4858344822839));
#179742=CARTESIAN_POINT('Ctrl Pts',(38.9392727637231,39.2209637700076,-55.5103162636118));
#179743=CARTESIAN_POINT('Ctrl Pts',(38.9512005223542,39.2188767318635,-55.5354850657774));
#179744=CARTESIAN_POINT('Ctrl Pts',(38.9631486411807,39.2167861312309,-55.5606968300573));
#179745=CARTESIAN_POINT('Ctrl Pts',(38.9728943609641,39.2150809447883,-55.5865979625573));
#179746=CARTESIAN_POINT('Ctrl Pts',(38.9804407021853,39.2137606048068,-55.6127884619919));
#179747=CARTESIAN_POINT('Ctrl Pts',(38.9880210340836,39.2124343176718,-55.6390969302251));
#179748=CARTESIAN_POINT('Ctrl Pts',(38.9933821545229,39.2114963473967,-55.6656973743602));
#179749=CARTESIAN_POINT('Ctrl Pts',(38.9965499548298,39.2109421244155,-55.6922317373016));
#179750=CARTESIAN_POINT('Ctrl Pts',(38.9988557843579,39.2105387076621,-55.7115459969304));
#179751=CARTESIAN_POINT('Ctrl Pts',(39.,39.2103385290022,-55.7308262353698));
#179752=CARTESIAN_POINT('Ctrl Pts',(39.,39.2103385290022,-55.74995));
#179753=CARTESIAN_POINT('',(39.,46.91999998,-55.74995));
#179754=CARTESIAN_POINT('Origin',(39.,46.91999998,-129.34995));
#179755=CARTESIAN_POINT('',(39.,39.2103385290022,-59.64995));
#179756=CARTESIAN_POINT('',(39.,39.2103385290022,-59.64995));
#179757=CARTESIAN_POINT('Ctrl Pts',(39.,39.2103385290022,-59.64995));
#179758=CARTESIAN_POINT('Ctrl Pts',(39.,39.2103385289879,-59.8463349320561));
#179759=CARTESIAN_POINT('Ctrl Pts',(39.,39.1711484082035,-60.0425718399611));
#179760=CARTESIAN_POINT('Ctrl Pts',(39.,39.0957216760398,-60.2239751485477));
#179761=CARTESIAN_POINT('Ctrl Pts',(39.,39.0202949438762,-60.4053784571342));
#179762=CARTESIAN_POINT('Ctrl Pts',(39.,38.9086909221403,-60.5717700902082));
#179763=CARTESIAN_POINT('Ctrl Pts',(39.,38.7693204940119,-60.7106101717798));
#179764=CARTESIAN_POINT('Ctrl Pts',(39.,38.6299500658835,-60.8494502533514));
#179765=CARTESIAN_POINT('Ctrl Pts',(39.,38.4629228438757,-60.9606295880618));
#179766=CARTESIAN_POINT('Ctrl Pts',(39.,38.2808266040481,-61.0357692987669));
#179767=CARTESIAN_POINT('Ctrl Pts',(39.,38.0987303642205,-61.110909009472));
#179768=CARTESIAN_POINT('Ctrl Pts',(39.,37.9017438633342,-61.149949999985));
#179769=CARTESIAN_POINT('Ctrl Pts',(39.,37.7046087726872,-61.14995));
#179770=CARTESIAN_POINT('Ctrl Pts',(39.5,37.7046087726872,-60.64995));
#179771=CARTESIAN_POINT('Ctrl Pts',(39.,37.7046087726872,-60.64995));
#179772=CARTESIAN_POINT('Ctrl Pts',(39.,37.7046087726872,-61.14995));
#179773=CARTESIAN_POINT('Ctrl Pts',(39.4942946417934,37.8365313206165,-60.64995));
#179774=CARTESIAN_POINT('Ctrl Pts',(38.9999999999973,37.8357552425198,-60.655621796981));
#179775=CARTESIAN_POINT('Ctrl Pts',(39.,37.9017438633342,-61.149949999985));
#179776=CARTESIAN_POINT('Ctrl Pts',(39.4885935839755,37.9683544324696,-60.6239226729818));
#179777=CARTESIAN_POINT('Ctrl Pts',(39.,37.9700367301949,-60.6353187454024));
#179778=CARTESIAN_POINT('Ctrl Pts',(39.,38.0987303642205,-61.110909009472));
#179779=CARTESIAN_POINT('Ctrl Pts',(39.4780533572395,38.2120715692569,-60.5237363920407));
#179780=CARTESIAN_POINT('Ctrl Pts',(39.,38.2214119490388,-60.5426326522478));
#179781=CARTESIAN_POINT('Ctrl Pts',(39.,38.4629228438758,-60.9606295880618));
#179782=CARTESIAN_POINT('Ctrl Pts',(39.4732193617859,38.3238459703974,-60.4496168355678));
#179783=CARTESIAN_POINT('Ctrl Pts',(39.,38.3387190323947,-60.4706504746467));
#179784=CARTESIAN_POINT('Ctrl Pts',(39.,38.6299500658835,-60.8494502533514));
#179785=CARTESIAN_POINT('Ctrl Pts',(39.4651522214979,38.5103789912237,-60.2644967268053));
#179786=CARTESIAN_POINT('Ctrl Pts',(39.,38.5356496464585,-60.2852157712116));
#179787=CARTESIAN_POINT('Ctrl Pts',(39.,38.9086909221403,-60.5717700902082));
#179788=CARTESIAN_POINT('Ctrl Pts',(39.4619222489988,38.5850642583582,-60.153568971423));
#179789=CARTESIAN_POINT('Ctrl Pts',(39.,38.6156677780068,-60.1718710142637));
#179790=CARTESIAN_POINT('Ctrl Pts',(39.,39.0202949438762,-60.4053784571342));
#179791=CARTESIAN_POINT('Ctrl Pts',(39.4575563441359,38.6860152017583,-59.9116978933072));
#179792=CARTESIAN_POINT('Ctrl Pts',(39.,38.7237795941064,-59.9224177216067));
#179793=CARTESIAN_POINT('Ctrl Pts',(39.,39.1711484082035,-60.0425718399611));
#179794=CARTESIAN_POINT('Ctrl Pts',(39.4564221286291,38.7122411799561,-59.7808732880376));
#179795=CARTESIAN_POINT('Ctrl Pts',(39.,38.7521729419779,-59.7861314644994));
#179796=CARTESIAN_POINT('Ctrl Pts',(39.,39.2103385289879,-59.8463349320561));
#179797=CARTESIAN_POINT('Ctrl Pts',(39.4564221286262,38.7122411799564,-59.64995));
#179798=CARTESIAN_POINT('Ctrl Pts',(39.,38.7521729419935,-59.64995));
#179799=CARTESIAN_POINT('Ctrl Pts',(39.,39.2103385290023,-59.64995));
#179800=CARTESIAN_POINT('',(39.4564221286262,38.7122411799564,-59.64995));
#179801=CARTESIAN_POINT('Origin',(39.5,39.2103385290022,-59.64995));
#179802=CARTESIAN_POINT('Ctrl Pts',(39.5,37.7046087726872,-60.64995));
#179803=CARTESIAN_POINT('Ctrl Pts',(39.4987807152437,37.7328017705422,-60.64995));
#179804=CARTESIAN_POINT('Ctrl Pts',(39.4976123687796,37.7598169441407,-60.6487640562912));
#179805=CARTESIAN_POINT('Ctrl Pts',(39.4964981291842,37.7855810278475,-60.646690542373));
#179806=CARTESIAN_POINT('Ctrl Pts',(39.4953259634005,37.8126845139321,-60.6445092322876));
#179807=CARTESIAN_POINT('Ctrl Pts',(39.4942136614223,37.8384037949514,-60.6413458429473));
#179808=CARTESIAN_POINT('Ctrl Pts',(39.4931629359066,37.8626992698647,-60.6375094924559));
#179809=CARTESIAN_POINT('Ctrl Pts',(39.4922295881091,37.8842806702054,-60.6341017049524));
#179810=CARTESIAN_POINT('Ctrl Pts',(39.4913447855216,37.9047395805,-60.6301623057276));
#179811=CARTESIAN_POINT('Ctrl Pts',(39.4905086923334,37.9240722042669,-60.6258833727946));
#179812=CARTESIAN_POINT('Ctrl Pts',(39.4895023952214,37.9473403802787,-60.6207333752658));
#179813=CARTESIAN_POINT('Ctrl Pts',(39.4885666220187,37.9689778622202,-60.6150923633976));
#179814=CARTESIAN_POINT('Ctrl Pts',(39.487700290685,37.9890096696409,-60.6092528148745));
#179815=CARTESIAN_POINT('Ctrl Pts',(39.4867980067401,38.0098727938541,-60.603170926025));
#179816=CARTESIAN_POINT('Ctrl Pts',(39.485971010137,38.0289950811894,-60.5968737820667));
#179817=CARTESIAN_POINT('Ctrl Pts',(39.4852169994621,38.0464297462502,-60.590641719909));
#179818=CARTESIAN_POINT('Ctrl Pts',(39.4848927496207,38.053927236097,-60.5879617244752));
#179819=CARTESIAN_POINT('Ctrl Pts',(39.4845819891505,38.0611128170089,-60.5852931620339));
#179820=CARTESIAN_POINT('Ctrl Pts',(39.4842844922117,38.0679917109782,-60.5826554871209));
#179821=CARTESIAN_POINT('Ctrl Pts',(39.4842090737884,38.0697355787937,-60.5819868103817));
#179822=CARTESIAN_POINT('Ctrl Pts',(39.4841737017427,38.0705524413637,-60.5816714634972));
#179823=CARTESIAN_POINT('Ctrl Pts',(39.4840978736734,38.0723051722649,-60.5809901111847));
#179824=CARTESIAN_POINT('Ctrl Pts',(39.4840628676318,38.0731143207956,-60.580675564769));
#179825=CARTESIAN_POINT('Ctrl Pts',(39.4840192449618,38.0741227976636,-60.5802826897657));
#179826=CARTESIAN_POINT('Ctrl Pts',(39.4839591488405,38.0755124154886,-60.5797369933149));
#179827=CARTESIAN_POINT('Ctrl Pts',(39.4837458556873,38.0804444470589,-60.5778002074773));
#179828=CARTESIAN_POINT('Ctrl Pts',(39.4835339342671,38.0853447503636,-60.575830756519));
#179829=CARTESIAN_POINT('Ctrl Pts',(39.4833233986077,38.0902130017798,-60.5738295347324));
#179830=CARTESIAN_POINT('Ctrl Pts',(39.4818941408137,38.1232619698137,-60.5602438939751));
#179831=CARTESIAN_POINT('Ctrl Pts',(39.4805292639958,38.154821844994,-60.5452002165668));
#179832=CARTESIAN_POINT('Ctrl Pts',(39.4792308551495,38.1848445976366,-60.5290286709037));
#179833=CARTESIAN_POINT('Ctrl Pts',(39.4779906264952,38.2135220656132,-60.5135817534141));
#179834=CARTESIAN_POINT('Ctrl Pts',(39.4768110201833,38.2407975955461,-60.49710534447));
#179835=CARTESIAN_POINT('Ctrl Pts',(39.4756925305597,38.2666599508293,-60.4798551182117));
#179836=CARTESIAN_POINT('Ctrl Pts',(39.4744365387292,38.2957017105978,-60.4604842248241));
#179837=CARTESIAN_POINT('Ctrl Pts',(39.4732575807838,38.322962248921,-60.4401373910195));
#179838=CARTESIAN_POINT('Ctrl Pts',(39.4721546419679,38.3484650295551,-60.4191325971816));
#179839=CARTESIAN_POINT('Ctrl Pts',(39.4716361344536,38.3604542561586,-60.4092579393278));
#179840=CARTESIAN_POINT('Ctrl Pts',(39.4711344064957,38.3720554962878,-60.3992372749932));
#179841=CARTESIAN_POINT('Ctrl Pts',(39.470649247717,38.383273614397,-60.3891007234335));
#179842=CARTESIAN_POINT('Ctrl Pts',(39.4704139561111,38.3887141611663,-60.3841847132522));
#179843=CARTESIAN_POINT('Ctrl Pts',(39.4701964148523,38.393744274237,-60.3795368119607));
#179844=CARTESIAN_POINT('Ctrl Pts',(39.4699770120232,38.3988172777583,-60.3747537948934));
#179845=CARTESIAN_POINT('Ctrl Pts',(39.4697641308945,38.403739487377,-60.3701129519459));
#179846=CARTESIAN_POINT('Ctrl Pts',(39.4695494906704,38.4087022269652,-60.3653448270166));
#179847=CARTESIAN_POINT('Ctrl Pts',(39.4693166057594,38.4140865458396,-60.3600469439559));
#179848=CARTESIAN_POINT('Ctrl Pts',(39.4692736283864,38.4150801863462,-60.3590692546082));
#179849=CARTESIAN_POINT('Ctrl Pts',(39.4692300340461,38.4160880830258,-60.3580734248406));
#179850=CARTESIAN_POINT('Ctrl Pts',(39.4691857254875,38.4171124836934,-60.3570567840804));
#179851=CARTESIAN_POINT('Ctrl Pts',(39.4677127419675,38.4511674236831,-60.3232598126683));
#179852=CARTESIAN_POINT('Ctrl Pts',(39.4663603950896,38.4824360653392,-60.2873222682081));
#179853=CARTESIAN_POINT('Ctrl Pts',(39.4651340689026,38.5107922339571,-60.2497596524454));
#179854=CARTESIAN_POINT('Ctrl Pts',(39.4638892540765,38.5395759127878,-60.2116307259771));
#179855=CARTESIAN_POINT('Ctrl Pts',(39.4627742871156,38.5653586693248,-60.1718273254161));
#179856=CARTESIAN_POINT('Ctrl Pts',(39.4617936459168,38.5880352467008,-60.1308415639801));
#179857=CARTESIAN_POINT('Ctrl Pts',(39.4610260198971,38.6057860110494,-60.0987587420958));
#179858=CARTESIAN_POINT('Ctrl Pts',(39.4603406775651,38.6216340299095,-60.0659504750838));
#179859=CARTESIAN_POINT('Ctrl Pts',(39.4597392952827,38.6355397301541,-60.0326334324049));
#179860=CARTESIAN_POINT('Ctrl Pts',(39.459679534421,38.636921574372,-60.0293226345325));
#179861=CARTESIAN_POINT('Ctrl Pts',(39.4596206036131,38.6382842162723,-60.0260068880544));
#179862=CARTESIAN_POINT('Ctrl Pts',(39.4595625010567,38.6396276967345,-60.0226864255211));
#179863=CARTESIAN_POINT('Ctrl Pts',(39.4588033987318,38.6571800938303,-59.9793050153962));
#179864=CARTESIAN_POINT('Ctrl Pts',(39.4581857740029,38.6714611652261,-59.9351228139635));
#179865=CARTESIAN_POINT('Ctrl Pts',(39.4577055602589,38.6825649414251,-59.8906338465719));
#179866=CARTESIAN_POINT('Ctrl Pts',(39.4572195296836,38.6938032177146,-59.8456059841206));
#179867=CARTESIAN_POINT('Ctrl Pts',(39.4568742584516,38.701786776151,-59.8002638465307));
#179868=CARTESIAN_POINT('Ctrl Pts',(39.4566651706717,38.7066214231023,-59.7550665512749));
#179869=CARTESIAN_POINT('Ctrl Pts',(39.4565023749363,38.7103856789864,-59.7198759393599));
#179870=CARTESIAN_POINT('Ctrl Pts',(39.4564221286262,38.7122411799564,-59.6847720500554));
#179871=CARTESIAN_POINT('Ctrl Pts',(39.4564221286262,38.7122411799564,-59.64995));
#179872=CARTESIAN_POINT('Ctrl Pts',(29.,38.7048160259599,-61.150138786574));
#179873=CARTESIAN_POINT('Ctrl Pts',(29.,38.6926240909195,-60.6436056187277));
#179874=CARTESIAN_POINT('Ctrl Pts',(28.4933647440612,38.6927858841383,-60.650327573148));
#179875=CARTESIAN_POINT('Ctrl Pts',(29.,38.8968977730653,-61.1455154974199));
#179876=CARTESIAN_POINT('Ctrl Pts',(29.0000000000007,38.8211017330502,-60.6340675708554));
#179877=CARTESIAN_POINT('Ctrl Pts',(28.4870505338491,38.8213938162437,-60.647315885492));
#179878=CARTESIAN_POINT('Ctrl Pts',(29.,39.0908916037092,-61.103090199825));
#179879=CARTESIAN_POINT('Ctrl Pts',(28.9999999999993,38.9470356871939,-60.5993042062512));
#179880=CARTESIAN_POINT('Ctrl Pts',(28.4808526630789,38.9512642676271,-60.6191174333591));
#179881=CARTESIAN_POINT('Ctrl Pts',(29.,39.4441857876827,-60.9504725910835));
#179882=CARTESIAN_POINT('Ctrl Pts',(29.0000000000007,39.1728401027082,-60.4895768580073));
#179883=CARTESIAN_POINT('Ctrl Pts',(28.4702284641343,39.1877232210837,-60.5175376561534));
#179884=CARTESIAN_POINT('Ctrl Pts',(29.,39.6084483440092,-60.8383643971029));
#179885=CARTESIAN_POINT('Ctrl Pts',(29.0000000000007,39.2753871003781,-60.4130391624567));
#179886=CARTESIAN_POINT('Ctrl Pts',(28.465656656414,39.2976315760154,-60.4428805969007));
#179887=CARTESIAN_POINT('Ctrl Pts',(29.,39.8127532432739,-60.6300880930806));
#179888=CARTESIAN_POINT('Ctrl Pts',(28.9999999999996,39.4020840949312,-60.2760820218603));
#179889=CARTESIAN_POINT('Ctrl Pts',(28.4606134496588,39.434276061177,-60.3041245704241));
#179890=CARTESIAN_POINT('Ctrl Pts',(29.,39.8731969861748,-60.5550848424531));
#179891=CARTESIAN_POINT('Ctrl Pts',(29.,39.439411822071,-60.2273142826608));
#179892=CARTESIAN_POINT('Ctrl Pts',(28.4592438293891,39.4746917169037,-60.2541491598715));
#179893=CARTESIAN_POINT('Ctrl Pts',(29.,39.9791737873547,-60.3942177709194));
#179894=CARTESIAN_POINT('Ctrl Pts',(29.,39.5049075987374,-60.1236050817051));
#179895=CARTESIAN_POINT('Ctrl Pts',(28.4570887248156,39.5455314661108,-60.1469471546371));
#179896=CARTESIAN_POINT('Ctrl Pts',(29.,40.025042572592,-60.3073218018945));
#179897=CARTESIAN_POINT('Ctrl Pts',(29.0000000000002,39.5332188379146,-60.0680634823705));
#179898=CARTESIAN_POINT('Ctrl Pts',(28.4563005932054,39.5761796095201,-60.0890325252997));
#179899=CARTESIAN_POINT('Ctrl Pts',(29.,40.1347632142717,-60.0389178342029));
#179900=CARTESIAN_POINT('Ctrl Pts',(28.9999999999997,39.6014080499751,-59.8970923098554));
#179901=CARTESIAN_POINT('Ctrl Pts',(28.4548707416055,39.6494517959669,-59.9101257001469));
#179902=CARTESIAN_POINT('Ctrl Pts',(29.,40.1727138319509,-59.8469756744913));
#179903=CARTESIAN_POINT('Ctrl Pts',(29.,39.6256255569264,-59.7761492712348));
#179904=CARTESIAN_POINT('Ctrl Pts',(28.4551199545093,39.6747304042147,-59.7821590925224));
#179905=CARTESIAN_POINT('Ctrl Pts',(29.,40.1727138277874,-59.6524466674074));
#179906=CARTESIAN_POINT('Ctrl Pts',(29.,39.6270595772528,-59.6524466674074));
#179907=CARTESIAN_POINT('Ctrl Pts',(28.4564221286262,39.6746164787415,-59.6524466674074));
#179908=CARTESIAN_POINT('',(28.4564221286262,39.6746164787415,-59.6524466674074));
#179909=CARTESIAN_POINT('',(29.,40.1727138277873,-59.6524466674074));
#179910=CARTESIAN_POINT('Origin',(28.5,40.1727138277873,-59.6524466674074));
#179911=CARTESIAN_POINT('Ctrl Pts',(29.,38.7048160259599,-61.150138786574));
#179912=CARTESIAN_POINT('Ctrl Pts',(29.,38.7587438294331,-61.1488407776135));
#179913=CARTESIAN_POINT('Ctrl Pts',(29.0000000000001,38.8125135208639,-61.1445744929232));
#179914=CARTESIAN_POINT('Ctrl Pts',(28.9999999999995,38.8658121354595,-61.1374999313474));
#179915=CARTESIAN_POINT('Ctrl Pts',(28.999999999999,38.9206199981761,-61.1302250405726));
#179916=CARTESIAN_POINT('Ctrl Pts',(28.9999999999976,38.9749308760973,-61.1199805166189));
#179917=CARTESIAN_POINT('Ctrl Pts',(28.9999999999961,39.0284204191816,-61.1068862346652));
#179918=CARTESIAN_POINT('Ctrl Pts',(28.9999999999946,39.0824266406294,-61.0936654694443));
#179919=CARTESIAN_POINT('Ctrl Pts',(28.9999999999932,39.1355968678683,-61.0775394193002));
#179920=CARTESIAN_POINT('Ctrl Pts',(28.9999999999937,39.1875946577396,-61.0585793760252));
#179921=CARTESIAN_POINT('Ctrl Pts',(28.999999999994,39.2145745592176,-61.0487416482901));
#179922=CARTESIAN_POINT('Ctrl Pts',(28.9999999999949,39.2412386526435,-61.038140115953));
#179923=CARTESIAN_POINT('Ctrl Pts',(28.999999999996,39.2675379042626,-61.0267795633668));
#179924=CARTESIAN_POINT('Ctrl Pts',(28.999999999996,39.2679181300168,-61.02661531631));
#179925=CARTESIAN_POINT('Ctrl Pts',(28.9999999999961,39.268298302465,-61.0264509016639));
#179926=CARTESIAN_POINT('Ctrl Pts',(28.9999999999961,39.268678421493,-61.0262863194886));
#179927=CARTESIAN_POINT('Ctrl Pts',(29.0000000000039,39.4448840602191,-60.9499936185261));
#179928=CARTESIAN_POINT('Ctrl Pts',(29.,39.6087415856579,-60.8380654560188));
#179929=CARTESIAN_POINT('Ctrl Pts',(29.,39.7446514854509,-60.6995134053984));
#179930=CARTESIAN_POINT('Ctrl Pts',(29.,39.744751813756,-60.6994111266649));
#179931=CARTESIAN_POINT('Ctrl Pts',(29.,39.7448521254371,-60.6993088358292));
#179932=CARTESIAN_POINT('Ctrl Pts',(29.,39.7449524204946,-60.6992065328918));
#179933=CARTESIAN_POINT('Ctrl Pts',(28.9999999999999,39.812931097784,-60.6298669408688));
#179934=CARTESIAN_POINT('Ctrl Pts',(29.,39.8732750955302,-60.554966232983));
#179935=CARTESIAN_POINT('Ctrl Pts',(29.,39.9261853767363,-60.4746513000797));
#179936=CARTESIAN_POINT('Ctrl Pts',(29.,39.9261884127568,-60.4746466915656));
#179937=CARTESIAN_POINT('Ctrl Pts',(29.,39.9261914487538,-60.4746420830304));
#179938=CARTESIAN_POINT('Ctrl Pts',(29.,39.9261944847274,-60.4746374744739));
#179939=CARTESIAN_POINT('Ctrl Pts',(29.,39.9791069872139,-60.3943171935884));
#179940=CARTESIAN_POINT('Ctrl Pts',(29.0000000000001,40.0249202649622,-60.3075521828599));
#179941=CARTESIAN_POINT('Ctrl Pts',(28.9999999999999,40.0614666645048,-60.2182183202257));
#179942=CARTESIAN_POINT('Ctrl Pts',(28.9999999999999,40.0615163877946,-60.218096776829));
#179943=CARTESIAN_POINT('Ctrl Pts',(28.9999999999999,40.0615660940304,-60.2179752284374));
#179944=CARTESIAN_POINT('Ctrl Pts',(28.9999999999999,40.0616157832065,-60.2178536750606));
#179945=CARTESIAN_POINT('Ctrl Pts',(28.9999999999996,40.0995205469998,-60.1251282086845));
#179946=CARTESIAN_POINT('Ctrl Pts',(28.9999999999997,40.128027334411,-60.0287688634757));
#179947=CARTESIAN_POINT('Ctrl Pts',(28.9999999999998,40.1466650082863,-59.9302710126543));
#179948=CARTESIAN_POINT('Ctrl Pts',(29.,40.1639177847725,-59.8390921769278));
#179949=CARTESIAN_POINT('Ctrl Pts',(29.,40.1727138277874,-59.7460820250092));
#179950=CARTESIAN_POINT('Ctrl Pts',(29.,40.1727138277873,-59.6524466674074));
#179951=CARTESIAN_POINT('Ctrl Pts',(28.4564221286157,39.6746164786217,-59.6524466674074));
#179952=CARTESIAN_POINT('Ctrl Pts',(28.4560930610391,39.6746447582207,-59.6852214163602));
#179953=CARTESIAN_POINT('Ctrl Pts',(28.4558631142718,39.6730442805713,-59.7182876085465));
#179954=CARTESIAN_POINT('Ctrl Pts',(28.4557164536146,39.6697525629344,-59.7513995669006));
#179955=CARTESIAN_POINT('Ctrl Pts',(28.4555706011372,39.6664789844466,-59.7843290604097));
#179956=CARTESIAN_POINT('Ctrl Pts',(28.4555070608883,39.6615324787802,-59.8173029960901));
#179957=CARTESIAN_POINT('Ctrl Pts',(28.455514149446,39.6549009331809,-59.8500663155775));
#179958=CARTESIAN_POINT('Ctrl Pts',(28.4555212161303,39.6482898508114,-59.8827285359583));
#179959=CARTESIAN_POINT('Ctrl Pts',(28.4555984368539,39.6400040729076,-59.9151805618179));
#179960=CARTESIAN_POINT('Ctrl Pts',(28.4557388532419,39.6300831646837,-59.9471690591856));
#179961=CARTESIAN_POINT('Ctrl Pts',(28.4558640822193,39.6212353000596,-59.9756976865905));
#179962=CARTESIAN_POINT('Ctrl Pts',(28.4560396318297,39.6110877023737,-60.0038572147082));
#179963=CARTESIAN_POINT('Ctrl Pts',(28.4562639562526,39.5997023822614,-60.0314760384073));
#179964=CARTESIAN_POINT('Ctrl Pts',(28.4565164554916,39.5868870827672,-60.0625637455503));
#179965=CARTESIAN_POINT('Ctrl Pts',(28.4568306655563,39.5725031725775,-60.0929653078116));
#179966=CARTESIAN_POINT('Ctrl Pts',(28.4572093049085,39.5566832670391,-60.1224589103904));
#179967=CARTESIAN_POINT('Ctrl Pts',(28.4575668544929,39.5417445116846,-60.1503097538976));
#179968=CARTESIAN_POINT('Ctrl Pts',(28.4579819214458,39.525526105916,-60.1773507351382));
#179969=CARTESIAN_POINT('Ctrl Pts',(28.4584608345725,39.5081717079878,-60.2034231684565));
#179970=CARTESIAN_POINT('Ctrl Pts',(28.4589538718475,39.4903054926235,-60.2302645322804));
#179971=CARTESIAN_POINT('Ctrl Pts',(28.4595146018092,39.4712358021277,-60.2560788724074));
#179972=CARTESIAN_POINT('Ctrl Pts',(28.4601537361126,39.4511448059234,-60.280729779171));
#179973=CARTESIAN_POINT('Ctrl Pts',(28.4604733032643,39.4410993078213,-60.2930552325527));
#179974=CARTESIAN_POINT('Ctrl Pts',(28.4608125277711,39.4307988255083,-60.3050904439814));
#179975=CARTESIAN_POINT('Ctrl Pts',(28.4611730509995,39.4202677347106,-60.3168221741449));
#179976=CARTESIAN_POINT('Ctrl Pts',(28.4613533126137,39.4150021893117,-60.3226880392267));
#179977=CARTESIAN_POINT('Ctrl Pts',(28.4615389017733,39.4096790191687,-60.3284780588577));
#179978=CARTESIAN_POINT('Ctrl Pts',(28.4617300396149,39.4043013196553,-60.3341908410452));
#179979=CARTESIAN_POINT('Ctrl Pts',(28.4618256085357,39.4016124698986,-60.337047232139));
#179980=CARTESIAN_POINT('Ctrl Pts',(28.461922564793,39.3989099893976,-60.3398843152446));
#179981=CARTESIAN_POINT('Ctrl Pts',(28.4620209369187,39.3961942701274,-60.3427019292839));
#179982=CARTESIAN_POINT('Ctrl Pts',(28.4620916599414,39.3942418484026,-60.3447276065778));
#179983=CARTESIAN_POINT('Ctrl Pts',(28.4621842200406,39.3917236897839,-60.347315551478));
#179984=CARTESIAN_POINT('Ctrl Pts',(28.4622529756521,39.3898442388991,-60.3492302412195));
#179985=CARTESIAN_POINT('Ctrl Pts',(28.4622798555975,39.3891094692389,-60.3499787874795));
#179986=CARTESIAN_POINT('Ctrl Pts',(28.4623031592114,39.3884728476581,-60.3506249265858));
#179987=CARTESIAN_POINT('Ctrl Pts',(28.4623203300338,39.3880077918452,-60.3510962110302));
#179988=CARTESIAN_POINT('Ctrl Pts',(28.4627572830568,39.376173324127,-60.3630891813141));
#179989=CARTESIAN_POINT('Ctrl Pts',(28.4633159972543,39.3629930253315,-60.3758362809693));
#179990=CARTESIAN_POINT('Ctrl Pts',(28.4639775759014,39.348327220407,-60.389138830442));
#179991=CARTESIAN_POINT('Ctrl Pts',(28.4646091527633,39.3343264918589,-60.4018381255111));
#179992=CARTESIAN_POINT('Ctrl Pts',(28.4653343723215,39.3189710193108,-60.4150435155025));
#179993=CARTESIAN_POINT('Ctrl Pts',(28.4661368014099,39.3021490027413,-60.4285362299288));
#179994=CARTESIAN_POINT('Ctrl Pts',(28.466917321566,39.2857862821131,-60.4416605492256));
#179995=CARTESIAN_POINT('Ctrl Pts',(28.4677707873882,39.2680350960101,-60.455056495446));
#179996=CARTESIAN_POINT('Ctrl Pts',(28.4686835930123,39.2488152070403,-60.4684805223839));
#179997=CARTESIAN_POINT('Ctrl Pts',(28.4695604420901,39.2303524133495,-60.4813757602411));
#179998=CARTESIAN_POINT('Ctrl Pts',(28.4704919580951,39.2105336346547,-60.4942963815287));
#179999=CARTESIAN_POINT('Ctrl Pts',(28.4714689033925,39.1893205542289,-60.5069926037893));
#180000=CARTESIAN_POINT('Ctrl Pts',(28.4722342090465,39.1727029499133,-60.516938391652));
#180001=CARTESIAN_POINT('Ctrl Pts',(28.4730274301954,39.1552302186206,-60.5267456851722));
#180002=CARTESIAN_POINT('Ctrl Pts',(28.4738459588635,39.1369030987336,-60.5362827351625));
#180003=CARTESIAN_POINT('Ctrl Pts',(28.4748434548321,39.1145688434842,-60.5479050146109));
#180004=CARTESIAN_POINT('Ctrl Pts',(28.4758783442967,39.0909640246873,-60.5591258135412));
#180005=CARTESIAN_POINT('Ctrl Pts',(28.4769502258775,39.0661321619779,-60.5696935979207));
#180006=CARTESIAN_POINT('Ctrl Pts',(28.4779986229512,39.0418443556902,-60.5800298462685));
#180007=CARTESIAN_POINT('Ctrl Pts',(28.4790823682872,39.0163824910683,-60.5897405006454));
#180008=CARTESIAN_POINT('Ctrl Pts',(28.4802064426117,38.9898368116951,-60.598587708987));
#180009=CARTESIAN_POINT('Ctrl Pts',(28.4813019955003,38.9639646828817,-60.6072104347661));
#180010=CARTESIAN_POINT('Ctrl Pts',(28.4824358508781,38.9370631630029,-60.6150121023343));
#180011=CARTESIAN_POINT('Ctrl Pts',(28.483618096623,38.9092638074563,-60.6217829758405));
#180012=CARTESIAN_POINT('Ctrl Pts',(28.4847852969212,38.8818182309136,-60.6284676821375));
#180013=CARTESIAN_POINT('Ctrl Pts',(28.4859996780555,38.8534978249802,-60.6341468182533));
#180014=CARTESIAN_POINT('Ctrl Pts',(28.487276309583,38.8244736151779,-60.6386416291119));
#180015=CARTESIAN_POINT('Ctrl Pts',(28.488536054244,38.7958333281812,-60.6430769840745));
#180016=CARTESIAN_POINT('Ctrl Pts',(28.4898564588711,38.7665082903692,-60.6463584329082));
#180017=CARTESIAN_POINT('Ctrl Pts',(28.4912568106162,38.7366999833481,-60.6483483554661));
#180018=CARTESIAN_POINT('Ctrl Pts',(28.4919395182101,38.7221676648519,-60.6493184940377));
#180019=CARTESIAN_POINT('Ctrl Pts',(28.4926412967995,38.7075209967316,-60.6499822472411));
#180020=CARTESIAN_POINT('Ctrl Pts',(28.493364741833,38.6927858841118,-60.6503273734803));
#180021=CARTESIAN_POINT('Origin',(29.,-9.33460238845303,-92.34995));
#180022=CARTESIAN_POINT('',(29.,40.1727138277873,-55.74995));
#180023=CARTESIAN_POINT('',(29.,40.1727138277874,-92.34995));
#180024=CARTESIAN_POINT('',(29.,43.91999998,-55.74995));
#180025=CARTESIAN_POINT('',(29.,29.41999998,-91.84995));
#180026=CARTESIAN_POINT('Origin',(29.5,-9.33460238845303,-55.74995));
#180027=CARTESIAN_POINT('',(29.5,40.0852251642615,-55.24995));
#180028=CARTESIAN_POINT('Ctrl Pts',(29.,40.1727138277873,-55.74995));
#180029=CARTESIAN_POINT('Ctrl Pts',(29.,40.1727138277863,-55.724027487683));
#180030=CARTESIAN_POINT('Ctrl Pts',(29.0021037800322,40.1723406811158,-55.6978059978151));
#180031=CARTESIAN_POINT('Ctrl Pts',(29.0063531399503,40.171591047903,-55.6716073785514));
#180032=CARTESIAN_POINT('Ctrl Pts',(29.0106395376334,40.1708348808266,-55.6451804100022));
#180033=CARTESIAN_POINT('Ctrl Pts',(29.0171091146883,40.1696956306932,-55.6187767699309));
#180034=CARTESIAN_POINT('Ctrl Pts',(29.0257761108208,40.1681748817224,-55.5927712420178));
#180035=CARTESIAN_POINT('Ctrl Pts',(29.0290201828335,40.1676056626875,-55.5830373268311));
#180036=CARTESIAN_POINT('Ctrl Pts',(29.0325718289249,40.1669830453019,-55.5733596262871));
#180037=CARTESIAN_POINT('Ctrl Pts',(29.0364307642165,40.1663072924394,-55.5637593428667));
#180038=CARTESIAN_POINT('Ctrl Pts',(29.0465845612265,40.1645292223565,-55.5384986629846));
#180039=CARTESIAN_POINT('Ctrl Pts',(29.0588727550753,40.1623812150824,-55.5137551371703));
#180040=CARTESIAN_POINT('Ctrl Pts',(29.0732950204348,40.1598629648353,-55.4899268488264));
#180041=CARTESIAN_POINT('Ctrl Pts',(29.0761937619183,40.1593568199077,-55.4851375840208));
#180042=CARTESIAN_POINT('Ctrl Pts',(29.0791786699972,40.1588357258452,-55.4803854543331));
#180043=CARTESIAN_POINT('Ctrl Pts',(29.0822496741217,40.1582996919844,-55.4756739402144));
#180044=CARTESIAN_POINT('Ctrl Pts',(29.0914248426835,40.1566981959173,-55.461597457583));
#180045=CARTESIAN_POINT('Ctrl Pts',(29.1013686732816,40.1549632328441,-55.4478834520589));
#180046=CARTESIAN_POINT('Ctrl Pts',(29.1120727310923,40.1530947826212,-55.4346345056757));
#180047=CARTESIAN_POINT('Ctrl Pts',(29.1174247599977,40.1521605575097,-55.4280100324841));
#180048=CARTESIAN_POINT('Ctrl Pts',(29.1229667921261,40.1511929611295,-55.4215019155803));
#180049=CARTESIAN_POINT('Ctrl Pts',(29.1286966355404,40.1501919949717,-55.4151241749086));
#180050=CARTESIAN_POINT('Ctrl Pts',(29.1315615572475,40.1496915118928,-55.4119353045727));
#180051=CARTESIAN_POINT('Ctrl Pts',(29.1344734223787,40.1491826864259,-55.4087790343615));
#180052=CARTESIAN_POINT('Ctrl Pts',(29.1374318784903,40.1486655190189,-55.4056571673549));
#180053=CARTESIAN_POINT('Ctrl Pts',(29.1391534315316,40.1483645745097,-55.4038405239987));
#180054=CARTESIAN_POINT('Ctrl Pts',(29.1412508897063,40.1479977964911,-55.4016627141525));
#180055=CARTESIAN_POINT('Ctrl Pts',(29.143098661154,40.1476746203084,-55.3997779331599));
#180056=CARTESIAN_POINT('Ctrl Pts',(29.1444262497453,40.1474424243767,-55.3984237539156));
#180057=CARTESIAN_POINT('Ctrl Pts',(29.1456236044489,40.1472329711656,-55.39721961437));
#180058=CARTESIAN_POINT('Ctrl Pts',(29.1464466082408,40.1470889648648,-55.3963966105726));
#180059=CARTESIAN_POINT('Ctrl Pts',(29.1562264477315,40.1453777230443,-55.3866167710174));
#180060=CARTESIAN_POINT('Ctrl Pts',(29.1671430152986,40.1434394756915,-55.3765446165107));
#180061=CARTESIAN_POINT('Ctrl Pts',(29.1793251261279,40.1412683811884,-55.3664154209164));
#180062=CARTESIAN_POINT('Ctrl Pts',(29.1909838912127,40.1391905573084,-55.3567213774467));
#180063=CARTESIAN_POINT('Ctrl Pts',(29.2038025095355,40.1368993418058,-55.3469750520176));
#180064=CARTESIAN_POINT('Ctrl Pts',(29.2178716381586,40.1343934407481,-55.337423499576));
#180065=CARTESIAN_POINT('Ctrl Pts',(29.2311276745907,40.1320323623469,-55.3284239566376));
#180066=CARTESIAN_POINT('Ctrl Pts',(29.2454943046528,40.1294806216269,-55.3195974073015));
#180067=CARTESIAN_POINT('Ctrl Pts',(29.2610192152979,40.1267419466417,-55.3111870422682));
#180068=CARTESIAN_POINT('Ctrl Pts',(29.2672465764664,40.1256434077421,-55.3078134717647));
#180069=CARTESIAN_POINT('Ctrl Pts',(29.2736599367761,40.1245148538384,-55.3045072863538));
#180070=CARTESIAN_POINT('Ctrl Pts',(29.2802607448067,40.1233568024336,-55.3012859403587));
#180071=CARTESIAN_POINT('Ctrl Pts',(29.2954942140765,40.12068422956,-55.2938516573137));
#180072=CARTESIAN_POINT('Ctrl Pts',(29.3117391205319,40.1178598967785,-55.2868619639026));
#180073=CARTESIAN_POINT('Ctrl Pts',(29.3289873345881,40.1148724981119,-55.280558107921));
#180074=CARTESIAN_POINT('Ctrl Pts',(29.3457634286183,40.1119668708526,-55.2744268017837));
#180075=CARTESIAN_POINT('Ctrl Pts',(29.3634889697681,40.1089069232597,-55.2689442786734));
#180076=CARTESIAN_POINT('Ctrl Pts',(29.3821198303984,40.1056887792346,-55.2643620188818));
#180077=CARTESIAN_POINT('Ctrl Pts',(29.4001775050092,40.1025696427219,-55.2599207341799));
#180078=CARTESIAN_POINT('Ctrl Pts',(29.4190858710103,40.0993018515975,-55.2563251747636));
#180079=CARTESIAN_POINT('Ctrl Pts',(29.4387660359806,40.0958888189828,-55.2538325278279));
#180080=CARTESIAN_POINT('Ctrl Pts',(29.458446200951,40.092475786368,-55.2513398808922));
#180081=CARTESIAN_POINT('Ctrl Pts',(29.4788985693907,40.0889174361862,-55.24995));
#180082=CARTESIAN_POINT('Ctrl Pts',(29.5,40.0852251642615,-55.24995));
#180083=CARTESIAN_POINT('',(29.5,39.6270595772528,-55.24995));
#180084=CARTESIAN_POINT('Origin',(0.,0.,-55.24995));
#180085=CARTESIAN_POINT('',(30.,40.0414808324985,-55.24995));
#180086=CARTESIAN_POINT('',(30.0435778713739,40.0376682627727,-55.24995));
#180087=CARTESIAN_POINT('',(30.,43.91999998,-55.24995));
#180088=CARTESIAN_POINT('Origin',(30.,0.,-55.74995));
#180089=CARTESIAN_POINT('',(30.5,39.9539921689726,-55.74995));
#180090=CARTESIAN_POINT('Ctrl Pts',(30.,40.0414808324985,-55.24995));
#180091=CARTESIAN_POINT('Ctrl Pts',(30.0215850498355,40.037703938174,-55.24995));
#180092=CARTESIAN_POINT('Ctrl Pts',(30.0424891945252,40.0340461868119,-55.2514041468278));
#180093=CARTESIAN_POINT('Ctrl Pts',(30.0625822498953,40.030530357691,-55.2540052053868));
#180094=CARTESIAN_POINT('Ctrl Pts',(30.0825281795813,40.0270402722291,-55.2565872184341));
#180095=CARTESIAN_POINT('Ctrl Pts',(30.101675378976,40.0236899464585,-55.2602996172416));
#180096=CARTESIAN_POINT('Ctrl Pts',(30.1199435824056,40.0204934250524,-55.2648742467056));
#180097=CARTESIAN_POINT('Ctrl Pts',(30.1390429090745,40.0171514759235,-55.2696570017729));
#180098=CARTESIAN_POINT('Ctrl Pts',(30.1571816232228,40.0139776122057,-55.2753821626572));
#180099=CARTESIAN_POINT('Ctrl Pts',(30.1743147295337,40.0109797070594,-55.2817780783403));
#180100=CARTESIAN_POINT('Ctrl Pts',(30.1903193475258,40.0081792617827,-55.2877527209626));
#180101=CARTESIAN_POINT('Ctrl Pts',(30.2054472590637,40.0055322202579,-55.2943131225478));
#180102=CARTESIAN_POINT('Ctrl Pts',(30.2196931733167,40.0030395082604,-55.3012636513269));
#180103=CARTESIAN_POINT('Ctrl Pts',(30.2362431771765,40.0001436328223,-55.3093383368879));
#180104=CARTESIAN_POINT('Ctrl Pts',(30.2516127665579,39.9974543031544,-55.3179437622824));
#180105=CARTESIAN_POINT('Ctrl Pts',(30.2658371702272,39.9949653550214,-55.326817870191));
#180106=CARTESIAN_POINT('Ctrl Pts',(30.2811342644793,39.9922887103574,-55.3363611922337));
#180107=CARTESIAN_POINT('Ctrl Pts',(30.2951078594437,39.9898436480612,-55.3462154234402));
#180108=CARTESIAN_POINT('Ctrl Pts',(30.3078412626167,39.9876155912096,-55.3561026477787));
#180109=CARTESIAN_POINT('Ctrl Pts',(30.3207962986518,39.9853487536323,-55.3661619654529));
#180110=CARTESIAN_POINT('Ctrl Pts',(30.3324678159279,39.9833065027367,-55.3762552366905));
#180111=CARTESIAN_POINT('Ctrl Pts',(30.3429723610003,39.981468445518,-55.3861352299963));
#180112=CARTESIAN_POINT('Ctrl Pts',(30.3445084364987,39.9811996671331,-55.3875799775354));
#180113=CARTESIAN_POINT('Ctrl Pts',(30.3460195961753,39.9809352484522,-55.3890202398166));
#180114=CARTESIAN_POINT('Ctrl Pts',(30.3475062515996,39.9806751174598,-55.39045533193));
#180115=CARTESIAN_POINT('Ctrl Pts',(30.3487711127258,39.9804537954408,-55.3916763224817));
#180116=CARTESIAN_POINT('Ctrl Pts',(30.3496069371401,39.9803075451175,-55.3924916493986));
#180117=CARTESIAN_POINT('Ctrl Pts',(30.3507725352476,39.9801035819845,-55.393638370999));
#180118=CARTESIAN_POINT('Ctrl Pts',(30.351507597415,39.9799749565333,-55.3943615290581));
#180119=CARTESIAN_POINT('Ctrl Pts',(30.3523735525915,39.9798234238397,-55.3952167714174));
#180120=CARTESIAN_POINT('Ctrl Pts',(30.3535533887318,39.9796169626886,-55.3963966075452));
#180121=CARTESIAN_POINT('Ctrl Pts',(30.3741274016675,39.9760166878297,-55.4169706202642));
#180122=CARTESIAN_POINT('Ctrl Pts',(30.3925747280172,39.9727886607578,-55.4391630476053));
#180123=CARTESIAN_POINT('Ctrl Pts',(30.4088523569405,39.9699403656182,-55.4624843705594));
#180124=CARTESIAN_POINT('Ctrl Pts',(30.4251500791383,39.9670885545135,-55.485834481597));
#180125=CARTESIAN_POINT('Ctrl Pts',(30.4392727632377,39.9646174100751,-55.5103162627385));
#180126=CARTESIAN_POINT('Ctrl Pts',(30.4512005218462,39.9625303719341,-55.5354850647054));
#180127=CARTESIAN_POINT('Ctrl Pts',(30.4631486406572,39.9604397713032,-55.5606968288014));
#180128=CARTESIAN_POINT('Ctrl Pts',(30.47289436045,39.9587345848572,-55.5865979611061));
#180129=CARTESIAN_POINT('Ctrl Pts',(30.4804407017092,39.9574142448672,-55.6127884603395));
#180130=CARTESIAN_POINT('Ctrl Pts',(30.4880210336523,39.9560879577225,-55.6390969283934));
#180131=CARTESIAN_POINT('Ctrl Pts',(30.4933821541613,39.9551499874332,-55.6656973723438));
#180132=CARTESIAN_POINT('Ctrl Pts',(30.496549954567,39.9545957644334,-55.6922317351003));
#180133=CARTESIAN_POINT('Ctrl Pts',(30.4988557842716,39.9541923476481,-55.711545995471));
#180134=CARTESIAN_POINT('Ctrl Pts',(30.5,39.9539921689726,-55.730826234649));
#180135=CARTESIAN_POINT('Ctrl Pts',(30.5,39.9539921689726,-55.74995));
#180136=CARTESIAN_POINT('',(30.5,39.4958265819638,-55.74995));
#180137=CARTESIAN_POINT('Origin',(30.5,-9.33460238845303,-92.34995));
#180138=CARTESIAN_POINT('',(30.5,39.9539921689726,-59.64995));
#180139=CARTESIAN_POINT('',(30.5,39.9539921689726,-92.34995));
#180140=CARTESIAN_POINT('Ctrl Pts',(30.5,39.9539921689726,-59.64995));
#180141=CARTESIAN_POINT('Ctrl Pts',(30.5,39.9539921689583,-59.8463349320561));
#180142=CARTESIAN_POINT('Ctrl Pts',(30.5,39.9148020481738,-60.0425718399611));
#180143=CARTESIAN_POINT('Ctrl Pts',(30.5,39.7639485838465,-60.4053784571342));
#180144=CARTESIAN_POINT('Ctrl Pts',(30.5,39.65234456211,-60.5717700902076));
#180145=CARTESIAN_POINT('Ctrl Pts',(30.5,39.3736037058546,-60.8494502533521));
#180146=CARTESIAN_POINT('Ctrl Pts',(30.5,39.206576483846,-60.9606295880612));
#180147=CARTESIAN_POINT('Ctrl Pts',(30.5,38.8423840041908,-61.1109090094727));
#180148=CARTESIAN_POINT('Ctrl Pts',(30.5,38.6453975033045,-61.149949999985));
#180149=CARTESIAN_POINT('Ctrl Pts',(30.5,38.4482624126576,-61.14995));
#180150=CARTESIAN_POINT('',(30.5,46.41999998,-91.84995));
#180151=CARTESIAN_POINT('Ctrl Pts',(37.5,37.9232037521398,-61.1499499946262));
#180152=CARTESIAN_POINT('Ctrl Pts',(37.5,37.9232456375444,-60.6498941830815));
#180153=CARTESIAN_POINT('Ctrl Pts',(36.9999441887055,37.9232456578392,-60.6499499995188));
#180154=CARTESIAN_POINT('Ctrl Pts',(37.5,38.1203811322273,-61.149966723533));
#180155=CARTESIAN_POINT('Ctrl Pts',(37.5000000000028,38.0559860700137,-60.6441634129654));
#180156=CARTESIAN_POINT('Ctrl Pts',(36.9942372710435,38.0551964119617,-60.6499618311932));
#180157=CARTESIAN_POINT('Ctrl Pts',(37.5,38.3174130179182,-61.110925104441));
#180158=CARTESIAN_POINT('Ctrl Pts',(37.5,38.1853247811951,-60.6119868070542));
#180159=CARTESIAN_POINT('Ctrl Pts',(36.9885345754041,38.1870501910475,-60.6239348042609));
#180160=CARTESIAN_POINT('Ctrl Pts',(37.5,38.6816445026906,-60.9606295880611));
#180161=CARTESIAN_POINT('Ctrl Pts',(37.5,38.4206008165402,-60.5030970594214));
#180162=CARTESIAN_POINT('Ctrl Pts',(36.977992646032,38.4307944117744,-60.5237387895065));
#180163=CARTESIAN_POINT('Ctrl Pts',(37.5,38.8486717246983,-60.8494502533514));
#180164=CARTESIAN_POINT('Ctrl Pts',(37.4999999999993,38.5260237066865,-60.4261477374108));
#180165=CARTESIAN_POINT('Ctrl Pts',(36.9731583992956,38.5425695414996,-60.4496195485703));
#180166=CARTESIAN_POINT('Ctrl Pts',(37.5,39.1274125809551,-60.5717700902082));
#180167=CARTESIAN_POINT('Ctrl Pts',(37.5000000000008,38.7000372987261,-60.2406358789592));
#180168=CARTESIAN_POINT('Ctrl Pts',(36.9650908553591,38.7291039816193,-60.2644994621534));
#180169=CARTESIAN_POINT('Ctrl Pts',(37.5,39.239016602691,-60.4053784571342));
#180170=CARTESIAN_POINT('Ctrl Pts',(37.4999999999994,38.7680983778313,-60.1321953438305));
#180171=CARTESIAN_POINT('Ctrl Pts',(36.9618607274251,38.8037899942061,-60.1535714132619));
#180172=CARTESIAN_POINT('Ctrl Pts',(37.5,39.3898862234668,-60.0425329832704));
#180173=CARTESIAN_POINT('Ctrl Pts',(37.5000000000007,38.8599291842782,-59.8989282761481));
#180174=CARTESIAN_POINT('Ctrl Pts',(36.9574941496163,38.9047527687766,-59.9116734379898));
#180175=CARTESIAN_POINT('Ctrl Pts',(37.5,39.429076975232,-59.8462508632634));
#180176=CARTESIAN_POINT('Ctrl Pts',(37.5,38.8833480398924,-59.7745406636058));
#180177=CARTESIAN_POINT('Ctrl Pts',(36.9563598640845,38.9309794818232,-59.7808179550133));
#180178=CARTESIAN_POINT('Ctrl Pts',(37.5,39.4290601824227,-59.649823802691));
#180179=CARTESIAN_POINT('Ctrl Pts',(37.5,38.8833379930089,-59.6498699040797));
#180180=CARTESIAN_POINT('Ctrl Pts',(36.9563603497081,38.9309682439904,-59.6498658680024));
#180181=CARTESIAN_POINT('',(36.9564221286262,38.9309628387712,-59.64995));
#180182=CARTESIAN_POINT('Origin',(37.,39.4290601878171,-59.64995));
#180183=CARTESIAN_POINT('Ctrl Pts',(36.9564221286262,38.9309628387712,-59.64995));
#180184=CARTESIAN_POINT('Ctrl Pts',(36.9564221286262,38.9309628387712,-59.6909727320563));
#180185=CARTESIAN_POINT('Ctrl Pts',(36.9565526533189,38.928414270096,-59.7323929145967));
#180186=CARTESIAN_POINT('Ctrl Pts',(36.9568026461917,38.9231907562272,-59.7738824505257));
#180187=CARTESIAN_POINT('Ctrl Pts',(36.9570478117228,38.9180681079776,-59.8145708269595));
#180188=CARTESIAN_POINT('Ctrl Pts',(36.9574078479651,38.9103725010286,-59.8553255347459));
#180189=CARTESIAN_POINT('Ctrl Pts',(36.9578758048445,38.9000244956702,-59.8958071083368));
#180190=CARTESIAN_POINT('Ctrl Pts',(36.9583385886206,38.889790883973,-59.9358411719725));
#180191=CARTESIAN_POINT('Ctrl Pts',(36.9589068918223,38.8769628684199,-59.9756077254562));
#180192=CARTESIAN_POINT('Ctrl Pts',(36.9595778517683,38.8615077284126,-60.0147542801158));
#180193=CARTESIAN_POINT('Ctrl Pts',(36.9602378669453,38.8463046942708,-60.0532622720685));
#180194=CARTESIAN_POINT('Ctrl Pts',(36.9609971979412,38.8285593256615,-60.0911698882792));
#180195=CARTESIAN_POINT('Ctrl Pts',(36.9618572198749,38.8082873402642,-60.1281241918774));
#180196=CARTESIAN_POINT('Ctrl Pts',(36.9624155228255,38.7951273162926,-60.1521139250818));
#180197=CARTESIAN_POINT('Ctrl Pts',(36.9630163436043,38.7809034729076,-60.1757015644984));
#180198=CARTESIAN_POINT('Ctrl Pts',(36.9636610617812,38.7656315786673,-60.1987879162352));
#180199=CARTESIAN_POINT('Ctrl Pts',(36.9644459532149,38.747039301619,-60.2268936535308));
#180200=CARTESIAN_POINT('Ctrl Pts',(36.9652958498083,38.7268930680149,-60.2542563740827));
#180201=CARTESIAN_POINT('Ctrl Pts',(36.9662149260452,38.7052405924212,-60.2806949719394));
#180202=CARTESIAN_POINT('Ctrl Pts',(36.9666744641636,38.6944143546243,-60.2939142708678));
#180203=CARTESIAN_POINT('Ctrl Pts',(36.9671513266945,38.6832118935344,-60.3069025151661));
#180204=CARTESIAN_POINT('Ctrl Pts',(36.9676462162085,38.6716412395726,-60.3196370305188));
#180205=CARTESIAN_POINT('Ctrl Pts',(36.9678688531808,38.6664359254737,-60.3253659333559));
#180206=CARTESIAN_POINT('Ctrl Pts',(36.9681087471589,38.6608777513272,-60.331343277216));
#180207=CARTESIAN_POINT('Ctrl Pts',(36.9683470528149,38.6553368998154,-60.3371563979268));
#180208=CARTESIAN_POINT('Ctrl Pts',(36.9685931263345,38.6496154374899,-60.343159004398));
#180209=CARTESIAN_POINT('Ctrl Pts',(36.9688375221239,38.6439126264018,-60.3489863692137));
#180210=CARTESIAN_POINT('Ctrl Pts',(36.9690630932701,38.6386772127086,-60.3542239166839));
#180211=CARTESIAN_POINT('Ctrl Pts',(36.9691046552039,38.6377125772892,-60.3551889452559));
#180212=CARTESIAN_POINT('Ctrl Pts',(36.9691455867854,38.6367639091397,-60.35613405381));
#180213=CARTESIAN_POINT('Ctrl Pts',(36.9691857916419,38.6358341396253,-60.3570567811866));
#180214=CARTESIAN_POINT('Ctrl Pts',(36.9701363384957,38.6138519821401,-60.3788724443089));
#180215=CARTESIAN_POINT('Ctrl Pts',(36.9711666068585,38.5902025659925,-60.4003228463237));
#180216=CARTESIAN_POINT('Ctrl Pts',(36.9722706959613,38.5648184450851,-60.4211192429472));
#180217=CARTESIAN_POINT('Ctrl Pts',(36.9733490218504,38.5400266464176,-60.4414303689452));
#180218=CARTESIAN_POINT('Ctrl Pts',(36.9744977238215,38.5135797007575,-60.4611173555234));
#180219=CARTESIAN_POINT('Ctrl Pts',(36.9757145657962,38.485452049613,-60.479881063412));
#180220=CARTESIAN_POINT('Ctrl Pts',(36.9769459440814,38.4569883874845,-60.4988689212632));
#180221=CARTESIAN_POINT('Ctrl Pts',(36.9782470364914,38.4268028979539,-60.516911045168));
#180222=CARTESIAN_POINT('Ctrl Pts',(36.9796197088919,38.3949169079658,-60.5336701568701));
#180223=CARTESIAN_POINT('Ctrl Pts',(36.9803060450922,38.3789739129717,-60.5420497127212));
#180224=CARTESIAN_POINT('Ctrl Pts',(36.9810103472633,38.3626066040907,-60.5501081143651));
#180225=CARTESIAN_POINT('Ctrl Pts',(36.9817333133923,38.34582295935,-60.5578010744457));
#180226=CARTESIAN_POINT('Ctrl Pts',(36.9820947964567,38.3374311369797,-60.5616475544861));
#180227=CARTESIAN_POINT('Ctrl Pts',(36.98246094573,38.3289352331521,-60.5654026797547));
#180228=CARTESIAN_POINT('Ctrl Pts',(36.9828318859725,38.3203366738844,-60.569060776422));
#180229=CARTESIAN_POINT('Ctrl Pts',(36.9830173560938,38.3160373942505,-60.5708898247557));
#180230=CARTESIAN_POINT('Ctrl Pts',(36.9832040239853,38.3117124510762,-60.5726946166406));
#180231=CARTESIAN_POINT('Ctrl Pts',(36.9833919065741,38.3073620378383,-60.5744744411355));
#180232=CARTESIAN_POINT('Ctrl Pts',(36.9835059768349,38.3047207458701,-60.5755550364458));
#180233=CARTESIAN_POINT('Ctrl Pts',(36.9836515904334,38.3013582757846,-60.5769130552655));
#180234=CARTESIAN_POINT('Ctrl Pts',(36.9837720133312,38.2985699856306,-60.5780234113379));
#180235=CARTESIAN_POINT('Ctrl Pts',(36.9838499363092,38.2967657451051,-60.5787418980494));
#180236=CARTESIAN_POINT('Ctrl Pts',(36.9839173597185,38.2952024681103,-60.5793580291786));
#180237=CARTESIAN_POINT('Ctrl Pts',(36.9839592160933,38.2942345898009,-60.5797383010624));
#180238=CARTESIAN_POINT('Ctrl Pts',(36.9846243076896,38.2788551468116,-60.5857807649761));
#180239=CARTESIAN_POINT('Ctrl Pts',(36.9853695593922,38.2618442765263,-60.5920329995529));
#180240=CARTESIAN_POINT('Ctrl Pts',(36.9861894744502,38.2431391507943,-60.5982457366593));
#180241=CARTESIAN_POINT('Ctrl Pts',(36.9869913344616,38.2248459237255,-60.6043216653772));
#180242=CARTESIAN_POINT('Ctrl Pts',(36.9878645390643,38.204931474406,-60.6103597069373));
#180243=CARTESIAN_POINT('Ctrl Pts',(36.9888053528999,38.1833531074951,-60.6160795510658));
#180244=CARTESIAN_POINT('Ctrl Pts',(36.9897095219953,38.1626152189253,-60.6215766070136));
#180245=CARTESIAN_POINT('Ctrl Pts',(36.9906760796327,38.140339861999,-60.6267794470962));
#180246=CARTESIAN_POINT('Ctrl Pts',(36.9917039045611,38.1165142207585,-60.6313985665783));
#180247=CARTESIAN_POINT('Ctrl Pts',(36.9927058043032,38.0932895419716,-60.6359011763997));
#180248=CARTESIAN_POINT('Ctrl Pts',(36.9937658627523,38.0685911496967,-60.6398488185077));
#180249=CARTESIAN_POINT('Ctrl Pts',(36.9948859960183,38.0424409451686,-60.6429384340034));
#180250=CARTESIAN_POINT('Ctrl Pts',(36.9959640318133,38.0172735321624,-60.6459119338523));
#180251=CARTESIAN_POINT('Ctrl Pts',(36.9970976705001,37.9907609104651,-60.6480902255593));
#180252=CARTESIAN_POINT('Ctrl Pts',(36.998292087359,37.9629622338,-60.6491761921129));
#180253=CARTESIAN_POINT('Ctrl Pts',(36.9988478997837,37.9500263397988,-60.649681538047));
#180254=CARTESIAN_POINT('Ctrl Pts',(36.9994169271496,37.9368125746484,-60.64995));
#180255=CARTESIAN_POINT('Ctrl Pts',(37.,37.923330431502,-60.64995));
#180256=CARTESIAN_POINT('Ctrl Pts',(30.5,39.9539921689726,-59.64995));
#180257=CARTESIAN_POINT('Ctrl Pts',(30.5,39.4958265819639,-59.64995));
#180258=CARTESIAN_POINT('Ctrl Pts',(30.9564221286262,39.4558948199267,-59.64995));
#180259=CARTESIAN_POINT('Ctrl Pts',(30.5,39.9539921689583,-59.8463349320561));
#180260=CARTESIAN_POINT('Ctrl Pts',(30.5,39.4958265819509,-59.7861314644993));
#180261=CARTESIAN_POINT('Ctrl Pts',(30.9564221286278,39.4558948199266,-59.7808732880376));
#180262=CARTESIAN_POINT('Ctrl Pts',(30.5,39.9148020481738,-60.0425718399611));
#180263=CARTESIAN_POINT('Ctrl Pts',(30.4999999999997,39.4674332340768,-59.9224177216067));
#180264=CARTESIAN_POINT('Ctrl Pts',(30.9575563441362,39.4296688417285,-59.9116978933072));
#180265=CARTESIAN_POINT('Ctrl Pts',(30.5,39.7639485838465,-60.4053784571342));
#180266=CARTESIAN_POINT('Ctrl Pts',(30.5000000000003,39.3593214179772,-60.1718710142636));
#180267=CARTESIAN_POINT('Ctrl Pts',(30.9619222489984,39.3287178983286,-60.153568971423));
#180268=CARTESIAN_POINT('Ctrl Pts',(30.5,39.65234456211,-60.5717700902076));
#180269=CARTESIAN_POINT('Ctrl Pts',(30.5000000000001,39.2793032864295,-60.2852157712117));
#180270=CARTESIAN_POINT('Ctrl Pts',(30.9651522214976,39.2540326311941,-60.2644967268053));
#180271=CARTESIAN_POINT('Ctrl Pts',(30.5,39.3736037058546,-60.8494502533521));
#180272=CARTESIAN_POINT('Ctrl Pts',(30.5,39.0823726723643,-60.4706504746469));
#180273=CARTESIAN_POINT('Ctrl Pts',(30.9732193617862,39.0674996103677,-60.4496168355678));
#180274=CARTESIAN_POINT('Ctrl Pts',(30.5,39.206576483846,-60.9606295880612));
#180275=CARTESIAN_POINT('Ctrl Pts',(30.5,38.9650655890091,-60.5426326522477));
#180276=CARTESIAN_POINT('Ctrl Pts',(30.9780533572398,38.9557252092273,-60.5237363920407));
#180277=CARTESIAN_POINT('Ctrl Pts',(30.5,38.8423840041908,-61.1109090094727));
#180278=CARTESIAN_POINT('Ctrl Pts',(30.5,38.7136903701654,-60.6353187454024));
#180279=CARTESIAN_POINT('Ctrl Pts',(30.9885935839752,38.71200807244,-60.6239226729818));
#180280=CARTESIAN_POINT('Ctrl Pts',(30.5,38.6453975033045,-61.149949999985));
#180281=CARTESIAN_POINT('Ctrl Pts',(30.4999999999973,38.5794088824901,-60.655621796981));
#180282=CARTESIAN_POINT('Ctrl Pts',(30.994294641792,38.5801849605867,-60.64995));
#180283=CARTESIAN_POINT('Ctrl Pts',(30.5,38.4482624126576,-61.14995));
#180284=CARTESIAN_POINT('Ctrl Pts',(30.5,38.4482624126575,-60.64995));
#180285=CARTESIAN_POINT('Ctrl Pts',(31.,38.4482624126576,-60.64995));
#180286=CARTESIAN_POINT('',(30.9564221286262,39.4558948199267,-59.64995));
#180287=CARTESIAN_POINT('Origin',(31.,39.9539921689726,-59.64995));
#180288=CARTESIAN_POINT('Ctrl Pts',(31.,38.4482624126576,-60.64995));
#180289=CARTESIAN_POINT('Ctrl Pts',(30.9987818467218,38.476429247827,-60.64995));
#180290=CARTESIAN_POINT('Ctrl Pts',(30.9976145369588,38.5034204502283,-60.6487662512907));
#180291=CARTESIAN_POINT('Ctrl Pts',(30.9965012313162,38.5291629385428,-60.6466963126423));
#180292=CARTESIAN_POINT('Ctrl Pts',(30.9953475221318,38.5558396606057,-60.6445512527966));
#180293=CARTESIAN_POINT('Ctrl Pts',(30.9942517893313,38.5811758196397,-60.6414545916582));
#180294=CARTESIAN_POINT('Ctrl Pts',(30.9932156801214,38.6051333279912,-60.6377013130332));
#180295=CARTESIAN_POINT('Ctrl Pts',(30.9921218554365,38.6304253664877,-60.6337389616033));
#180296=CARTESIAN_POINT('Ctrl Pts',(30.9910944719623,38.654181113399,-60.6290450673587));
#180297=CARTESIAN_POINT('Ctrl Pts',(30.990133679575,38.6763971032037,-60.6239244744924));
#180298=CARTESIAN_POINT('Ctrl Pts',(30.989141234533,38.6993449837517,-60.618635187161));
#180299=CARTESIAN_POINT('Ctrl Pts',(30.9882197863802,38.720651233716,-60.6128905529596));
#180300=CARTESIAN_POINT('Ctrl Pts',(30.9873680866258,38.7403447214142,-60.6069806688732));
#180301=CARTESIAN_POINT('Ctrl Pts',(30.9864834145568,38.7608006137855,-60.600841992238));
#180302=CARTESIAN_POINT('Ctrl Pts',(30.9856739565944,38.7795173626662,-60.594525091633));
#180303=CARTESIAN_POINT('Ctrl Pts',(30.9849373158678,38.7965503898717,-60.588305157651));
#180304=CARTESIAN_POINT('Ctrl Pts',(30.9847129878412,38.8017374305014,-60.586411011068));
#180305=CARTESIAN_POINT('Ctrl Pts',(30.9844954066137,38.8067684677967,-60.5845255017482));
#180306=CARTESIAN_POINT('Ctrl Pts',(30.9842844922129,38.8116453509173,-60.5826554871329));
#180307=CARTESIAN_POINT('Ctrl Pts',(30.9842090737892,38.8133892187453,-60.5819868103889));
#180308=CARTESIAN_POINT('Ctrl Pts',(30.9841737017427,38.8142060813347,-60.581671463497));
#180309=CARTESIAN_POINT('Ctrl Pts',(30.9840978736727,38.8159588122539,-60.5809901111774));
#180310=CARTESIAN_POINT('Ctrl Pts',(30.9840628676311,38.8167679607848,-60.5806755647617));
#180311=CARTESIAN_POINT('Ctrl Pts',(30.9840192449614,38.8177764376487,-60.5802826897599));
#180312=CARTESIAN_POINT('Ctrl Pts',(30.9839591488407,38.819166055459,-60.5797369933149));
#180313=CARTESIAN_POINT('Ctrl Pts',(30.9837458556875,38.8240980870287,-60.5778002074775));
#180314=CARTESIAN_POINT('Ctrl Pts',(30.9835339342674,38.8289983903335,-60.5758307565192));
#180315=CARTESIAN_POINT('Ctrl Pts',(30.9833233986079,38.8338666417501,-60.5738295347323));
#180316=CARTESIAN_POINT('Ctrl Pts',(30.9818941408027,38.8669156100438,-60.5602438938683));
#180317=CARTESIAN_POINT('Ctrl Pts',(30.9805292639735,38.8984754854848,-60.5452002163202));
#180318=CARTESIAN_POINT('Ctrl Pts',(30.9792308551162,38.928498238384,-60.5290286704852));
#180319=CARTESIAN_POINT('Ctrl Pts',(30.9779906264808,38.9571757059225,-60.5135817531992));
#180320=CARTESIAN_POINT('Ctrl Pts',(30.9768110201851,38.9844512354806,-60.4971053444783));
#180321=CARTESIAN_POINT('Ctrl Pts',(30.9756925305751,39.0103135904489,-60.4798551184457));
#180322=CARTESIAN_POINT('Ctrl Pts',(30.9744365387299,39.0393553505584,-60.460484224848));
#180323=CARTESIAN_POINT('Ctrl Pts',(30.9732575807701,39.0666158892126,-60.4401373907899));
#180324=CARTESIAN_POINT('Ctrl Pts',(30.9721546419406,39.0921186701619,-60.4191325966574));
#180325=CARTESIAN_POINT('Ctrl Pts',(30.9716361344385,39.1041078964837,-60.4092579390191));
#180326=CARTESIAN_POINT('Ctrl Pts',(30.9711344064916,39.1157091363555,-60.3992372749015));
#180327=CARTESIAN_POINT('Ctrl Pts',(30.9706492477231,39.1269272542305,-60.3891007235571));
#180328=CARTESIAN_POINT('Ctrl Pts',(30.970413956114,39.1323678010709,-60.3841847133134));
#180329=CARTESIAN_POINT('Ctrl Pts',(30.9701964148518,39.1373979142195,-60.3795368119505));
#180330=CARTESIAN_POINT('Ctrl Pts',(30.9699770120193,39.1424709178192,-60.3747537948081));
#180331=CARTESIAN_POINT('Ctrl Pts',(30.9697641308869,39.1473931275184,-60.3701129517834));
#180332=CARTESIAN_POINT('Ctrl Pts',(30.969549490659,39.1523558671877,-60.3653448267733));
#180333=CARTESIAN_POINT('Ctrl Pts',(30.9693166057443,39.1577401861387,-60.3600469436324));
#180334=CARTESIAN_POINT('Ctrl Pts',(30.9692736283757,39.1587338265396,-60.3590692543879));
#180335=CARTESIAN_POINT('Ctrl Pts',(30.96923003404,39.1597417231099,-60.3580734247277));
#180336=CARTESIAN_POINT('Ctrl Pts',(30.9691857254863,39.1607661236638,-60.3570567840805));
#180337=CARTESIAN_POINT('Ctrl Pts',(30.9677127419572,39.1948210637802,-60.3232598125428));
#180338=CARTESIAN_POINT('Ctrl Pts',(30.9663603950735,39.2260897055471,-60.2873222679365));
#180339=CARTESIAN_POINT('Ctrl Pts',(30.9651340688828,39.254445874256,-60.2497596520108));
#180340=CARTESIAN_POINT('Ctrl Pts',(30.9638892540534,39.2832295531698,-60.2116307253895));
#180341=CARTESIAN_POINT('Ctrl Pts',(30.9627742870912,39.3090123097717,-60.1718273246592));
#180342=CARTESIAN_POINT('Ctrl Pts',(30.9617936458919,39.3316888871906,-60.1308415630416));
#180343=CARTESIAN_POINT('Ctrl Pts',(30.9610260198825,39.3494396513267,-60.0987587414601));
#180344=CARTESIAN_POINT('Ctrl Pts',(30.960340677559,39.3652876700136,-60.0659504747633));
#180345=CARTESIAN_POINT('Ctrl Pts',(30.9597392952827,39.3791933701244,-60.032633432405));
#180346=CARTESIAN_POINT('Ctrl Pts',(30.9596795344221,39.380575214318,-60.0293226345908));
#180347=CARTESIAN_POINT('Ctrl Pts',(30.9596206036152,39.3819378561946,-60.0260068881712));
#180348=CARTESIAN_POINT('Ctrl Pts',(30.9595625010598,39.3832813366339,-60.0226864256965));
#180349=CARTESIAN_POINT('Ctrl Pts',(30.9588033987314,39.4008337338138,-59.9793050153876));
#180350=CARTESIAN_POINT('Ctrl Pts',(30.9581857739999,39.4151148052685,-59.9351228137558));
#180351=CARTESIAN_POINT('Ctrl Pts',(30.9577055602545,39.4262185814993,-59.8906338461556));
#180352=CARTESIAN_POINT('Ctrl Pts',(30.9572195296779,39.4374568578174,-59.8456059835076));
#180353=CARTESIAN_POINT('Ctrl Pts',(30.9568742584458,39.4454404162565,-59.8002638457115));
#180354=CARTESIAN_POINT('Ctrl Pts',(30.956665170667,39.4502750631828,-59.7550665502451));
#180355=CARTESIAN_POINT('Ctrl Pts',(30.9565023749348,39.4540393189924,-59.7198759386805));
#180356=CARTESIAN_POINT('Ctrl Pts',(30.9564221286262,39.4558948199267,-59.6847720497212));
#180357=CARTESIAN_POINT('Ctrl Pts',(30.9564221286262,39.4558948199267,-59.64995));
#180358=CARTESIAN_POINT('Origin',(0.,-12.9675000200281,-60.64995));
#180359=CARTESIAN_POINT('',(4.69960655320655,40.7492486855235,-60.64995));
#180360=CARTESIAN_POINT('Origin',(33.35,67.7009572055632,-55.24995));
#180361=CARTESIAN_POINT('',(33.35,-65.63964951798,-59.64995));
#180362=CARTESIAN_POINT('Ctrl Pts',(33.35,-64.133919761665,-61.14995));
#180363=CARTESIAN_POINT('Ctrl Pts',(33.35,-64.3310548523114,-61.149949999985));
#180364=CARTESIAN_POINT('Ctrl Pts',(33.35,-64.5280413531989,-61.1109090094727));
#180365=CARTESIAN_POINT('Ctrl Pts',(33.35,-64.8922338328527,-60.9606295880612));
#180366=CARTESIAN_POINT('Ctrl Pts',(33.35,-65.0592610548614,-60.849450253352));
#180367=CARTESIAN_POINT('Ctrl Pts',(33.35,-65.338001911118,-60.5717700902076));
#180368=CARTESIAN_POINT('Ctrl Pts',(33.35,-65.4496059328539,-60.4053784571335));
#180369=CARTESIAN_POINT('Ctrl Pts',(33.35,-65.6004593971813,-60.0425718399618));
#180370=CARTESIAN_POINT('Ctrl Pts',(33.35,-65.6396495179636,-59.8463349320557));
#180371=CARTESIAN_POINT('Ctrl Pts',(33.35,-65.63964951798,-59.64995));
#180372=CARTESIAN_POINT('',(33.35,-65.63964951798,-55.74995));
#180373=CARTESIAN_POINT('',(33.35,-65.63964951798,-55.24995));
#180374=CARTESIAN_POINT('',(33.35,67.7009572055632,-55.74995));
#180375=CARTESIAN_POINT('Origin',(32.85,67.7009572055632,-55.74995));
#180376=CARTESIAN_POINT('',(32.85,-65.7271381815059,-55.24995));
#180377=CARTESIAN_POINT('Ctrl Pts',(33.35,-65.63964951798,-55.74995));
#180378=CARTESIAN_POINT('Ctrl Pts',(33.35,-65.63964951798,-55.7240510278047));
#180379=CARTESIAN_POINT('Ctrl Pts',(33.347900048614,-65.640016961861,-55.6978536073956));
#180380=CARTESIAN_POINT('Ctrl Pts',(33.3436584043302,-65.6407591534406,
-55.6716786003409));
#180381=CARTESIAN_POINT('Ctrl Pts',(33.3393809358794,-65.6415076134371,
-55.6452825238705));
#180382=CARTESIAN_POINT('Ctrl Pts',(33.3329253996456,-65.6426371859126,
-55.6189093032682));
#180383=CARTESIAN_POINT('Ctrl Pts',(33.3242775747263,-65.6441503592019,
-55.5929324718169));
#180384=CARTESIAN_POINT('Ctrl Pts',(33.3210188939802,-65.6447205544486,
-55.583143860081));
#180385=CARTESIAN_POINT('Ctrl Pts',(33.3174492131982,-65.6453451676502,
-55.5734119765541));
#180386=CARTESIAN_POINT('Ctrl Pts',(33.3135688278912,-65.6460241470991,
-55.5637583894205));
#180387=CARTESIAN_POINT('Ctrl Pts',(33.3034033143569,-65.6478028814851,
-55.5384687176752));
#180388=CARTESIAN_POINT('Ctrl Pts',(33.2910985361539,-65.6499559386847,
-55.5136974847687));
#180389=CARTESIAN_POINT('Ctrl Pts',(33.2766549467837,-65.6524832393453,
-55.4898442373666));
#180390=CARTESIAN_POINT('Ctrl Pts',(33.2649384053914,-65.6545333684401,
-55.4704946454223));
#180391=CARTESIAN_POINT('Ctrl Pts',(33.2518128551695,-65.6568300421337,
-55.4517483669));
#180392=CARTESIAN_POINT('Ctrl Pts',(33.2372964027467,-65.6593700921767,
-55.4338552796691));
#180393=CARTESIAN_POINT('Ctrl Pts',(33.2294565912626,-65.6607418814347,
-55.4241918697206));
#180394=CARTESIAN_POINT('Ctrl Pts',(33.2212113468568,-65.6621846122616,
-55.414777801353));
#180395=CARTESIAN_POINT('Ctrl Pts',(33.2125680866752,-65.6636969868252,
-55.4056571306878));
#180396=CARTESIAN_POINT('Ctrl Pts',(33.2108465431246,-65.6639982179141,
-55.4038404976778));
#180397=CARTESIAN_POINT('Ctrl Pts',(33.2087490914815,-65.6643652243974,
-55.4016626948158));
#180398=CARTESIAN_POINT('Ctrl Pts',(33.2069013241902,-65.6646885364879,
-55.3997779182178));
#180399=CARTESIAN_POINT('Ctrl Pts',(33.2055737423077,-65.6649208294156,
-55.3984237459279));
#180400=CARTESIAN_POINT('Ctrl Pts',(33.2043763923404,-65.6651303319781,
-55.3972196111485));
#180401=CARTESIAN_POINT('Ctrl Pts',(33.2035533894273,-65.6652743275964,
-55.3963966082408));
#180402=CARTESIAN_POINT('Ctrl Pts',(33.1937873007841,-65.6669830384047,
-55.3866305196621));
#180403=CARTESIAN_POINT('Ctrl Pts',(33.182886437889,-65.6688903937285,-55.3765717208458));
#180404=CARTESIAN_POINT('Ctrl Pts',(33.170722824573,-65.6710187470995,-55.3664552894951));
#180405=CARTESIAN_POINT('Ctrl Pts',(33.1590750456085,-65.6730568412891,
-55.3567678756303));
#180406=CARTESIAN_POINT('Ctrl Pts',(33.1462686320959,-65.675297711858,-55.3470275906715));
#180407=CARTESIAN_POINT('Ctrl Pts',(33.132213803587,-65.6777570333304,-55.3374815439839));
#180408=CARTESIAN_POINT('Ctrl Pts',(33.1189601031151,-65.6800761729868,
-55.3284796238675));
#180409=CARTESIAN_POINT('Ctrl Pts',(33.10459580387,-65.6825896481115,-55.3196505221102));
#180410=CARTESIAN_POINT('Ctrl Pts',(33.0890741345983,-65.6853056127038,
-55.311237769723));
#180411=CARTESIAN_POINT('Ctrl Pts',(33.0828103974728,-65.6864016345265,
-55.3078428211172));
#180412=CARTESIAN_POINT('Ctrl Pts',(33.0763585547313,-65.6875305666442,
-55.3045160977312));
#180413=CARTESIAN_POINT('Ctrl Pts',(33.069717210502,-65.6886926513055,-55.3012753797601));
#180414=CARTESIAN_POINT('Ctrl Pts',(33.0544690954581,-65.6913607257185,
-55.293834892));
#180415=CARTESIAN_POINT('Ctrl Pts',(33.0382095130778,-65.6942057839824,
-55.2868407235284));
#180416=CARTESIAN_POINT('Ctrl Pts',(33.0209460855975,-65.6972264923786,
-55.2805340044877));
#180417=CARTESIAN_POINT('Ctrl Pts',(33.0041655073293,-65.7001627131103,
-55.2744036811438));
#180418=CARTESIAN_POINT('Ctrl Pts',(32.9864361384534,-65.7032649506864,
-55.2689228588808));
#180419=CARTESIAN_POINT('Ctrl Pts',(32.9678013238571,-65.7065256207345,
-55.2643427579567));
#180420=CARTESIAN_POINT('Ctrl Pts',(32.9497555825658,-65.7096832163102,
-55.2599074406136));
#180421=CARTESIAN_POINT('Ctrl Pts',(32.9308605102442,-65.7129894255594,
-55.2563167977718));
#180422=CARTESIAN_POINT('Ctrl Pts',(32.9111938833676,-65.7164306393623,
-55.2538274761891));
#180423=CARTESIAN_POINT('Ctrl Pts',(32.8915272564911,-65.7198718531653,
-55.2513381546065));
#180424=CARTESIAN_POINT('Ctrl Pts',(32.8710886481192,-65.7234481462268,
-55.24995));
#180425=CARTESIAN_POINT('Ctrl Pts',(32.85,-65.7271381815059,-55.24995));
#180426=CARTESIAN_POINT('',(32.85,-73.08000002,-55.24995));
#180427=CARTESIAN_POINT('Origin',(41.5,-73.08000002,-55.24995));
#180428=CARTESIAN_POINT('',(32.35,-65.7708825132688,-55.24995));
#180429=CARTESIAN_POINT('',(40.7958880023324,-65.0319630596553,-55.24995));
#180430=CARTESIAN_POINT('',(32.35,-73.08000002,-55.24995));
#180431=CARTESIAN_POINT('Origin',(32.35,-73.08000002,-55.74995));
#180432=CARTESIAN_POINT('',(31.85,-65.8583711767947,-55.74995));
#180433=CARTESIAN_POINT('Ctrl Pts',(32.35,-65.7708825132688,-55.24995));
#180434=CARTESIAN_POINT('Ctrl Pts',(32.3291548218245,-65.7745299468279,
-55.24995));
#180435=CARTESIAN_POINT('Ctrl Pts',(32.3089230360357,-65.7780375764609,
-55.2512537778699));
#180436=CARTESIAN_POINT('Ctrl Pts',(32.2894400315174,-65.7814054021679,
-55.2536310599852));
#180437=CARTESIAN_POINT('Ctrl Pts',(32.2694040627665,-65.784868813089,-55.2560758138285));
#180438=CARTESIAN_POINT('Ctrl Pts',(32.2501597157281,-65.7881843716721,
-55.2596551840712));
#180439=CARTESIAN_POINT('Ctrl Pts',(32.2317985474285,-65.7913520779171,
-55.2641224414877));
#180440=CARTESIAN_POINT('Ctrl Pts',(32.2125512297628,-65.7946726644602,
-55.2688052983293));
#180441=CARTESIAN_POINT('Ctrl Pts',(32.1942741291894,-65.7978307829405,
-55.2744631104736));
#180442=CARTESIAN_POINT('Ctrl Pts',(32.1770162849582,-65.8008264333581,
-55.2808267386599));
#180443=CARTESIAN_POINT('Ctrl Pts',(32.1592871390005,-65.8039038932528,
-55.2873641538449));
#180444=CARTESIAN_POINT('Ctrl Pts',(32.1426330780179,-65.8068098900981,
-55.294645913793));
#180445=CARTESIAN_POINT('Ctrl Pts',(32.127056183543,-65.809544423894,-55.3024055276807));
#180446=CARTESIAN_POINT('Ctrl Pts',(32.1107544016718,-65.8124062121363,
-55.3105262434758));
#180447=CARTESIAN_POINT('Ctrl Pts',(32.0956317582546,-65.8150802075761,
-55.3191697908562));
#180448=CARTESIAN_POINT('Ctrl Pts',(32.0816447916951,-65.8175664102134,
-55.3280667434282));
#180449=CARTESIAN_POINT('Ctrl Pts',(32.0715059985561,-65.8193685947067,
-55.3345159160427));
#180450=CARTESIAN_POINT('Ctrl Pts',(32.0619629273805,-65.8210721048226,
-55.3410990294536));
#180451=CARTESIAN_POINT('Ctrl Pts',(32.052987973319,-65.8226769405612,-55.3477263607061));
#180452=CARTESIAN_POINT('Ctrl Pts',(32.0419258838949,-65.8246549826024,
-55.3558948850746));
#180453=CARTESIAN_POINT('Ctrl Pts',(32.0317269309072,-65.8264831202867,
-55.3641299065953));
#180454=CARTESIAN_POINT('Ctrl Pts',(32.0223264817131,-65.8281613536139,
-55.3722860416806));
#180455=CARTESIAN_POINT('Ctrl Pts',(32.017626257116,-65.8290004702776,-55.3763641092233));
#180456=CARTESIAN_POINT('Ctrl Pts',(32.0131254732844,-65.829802110852,-55.380422842289));
#180457=CARTESIAN_POINT('Ctrl Pts',(32.008815192513,-65.8305662753372,-55.38444633772));
#180458=CARTESIAN_POINT('Ctrl Pts',(32.0066600521273,-65.8309483575797,
-55.3864580854356));
#180459=CARTESIAN_POINT('Ctrl Pts',(32.0045525458112,-65.8313210708,-55.3884610324979));
#180460=CARTESIAN_POINT('Ctrl Pts',(32.0024915002078,-65.831684414998,-55.3904533483158));
#180461=CARTESIAN_POINT('Ctrl Pts',(32.00121209498,-65.831909962878,-55.3916900891568));
#180462=CARTESIAN_POINT('Ctrl Pts',(32.0003718507455,-65.832058977522,-55.3925105847833));
#180463=CARTESIAN_POINT('Ctrl Pts',(31.9991841723761,-65.8322672609766,
-55.3936800811344));
#180464=CARTESIAN_POINT('Ctrl Pts',(31.9984585716465,-65.8323945097593,
-55.3943945737339));
#180465=CARTESIAN_POINT('Ctrl Pts',(31.9976035777943,-65.832543880519,-55.3952396410192));
#180466=CARTESIAN_POINT('Ctrl Pts',(31.9964466094067,-65.832746340525,-55.3963966094067));
#180467=CARTESIAN_POINT('Ctrl Pts',(31.9784887646162,-65.835888816501,-55.4143544541973));
#180468=CARTESIAN_POINT('Ctrl Pts',(31.9620748438882,-65.8387422616958,
-55.4335093827193));
#180469=CARTESIAN_POINT('Ctrl Pts',(31.9473083464221,-65.8413066761094,
-55.4535728211574));
#180470=CARTESIAN_POINT('Ctrl Pts',(31.9323330904136,-65.8439073444429,
-55.473919902631));
#180471=CARTESIAN_POINT('Ctrl Pts',(31.9190520284849,-65.8462107519933,
-55.4952007601908));
#180472=CARTESIAN_POINT('Ctrl Pts',(31.9075195954657,-65.8482168987607,
-55.5171172454247));
#180473=CARTESIAN_POINT('Ctrl Pts',(31.8957341095488,-65.8502670658361,
-55.5395146378605));
#180474=CARTESIAN_POINT('Ctrl Pts',(31.8857746508348,-65.8520067835848,
-55.5625752637249));
#180475=CARTESIAN_POINT('Ctrl Pts',(31.8776461797849,-65.853436052007,-55.5859930894161));
#180476=CARTESIAN_POINT('Ctrl Pts',(31.8694149427853,-65.8548833902637,
-55.6097069800233));
#180477=CARTESIAN_POINT('Ctrl Pts',(31.8630609213692,-65.8560123797269,
-55.6337866410958));
#180478=CARTESIAN_POINT('Ctrl Pts',(31.8585396585789,-65.8568230203966,
-55.6579351489687));
#180479=CARTESIAN_POINT('Ctrl Pts',(31.8539333232147,-65.8576489141696,
-55.6825380378005));
#180480=CARTESIAN_POINT('Ctrl Pts',(31.851228960127,-65.8581443662676,-55.7072119138125));
#180481=CARTESIAN_POINT('Ctrl Pts',(31.8503341986073,-65.8583093766908,
-55.7316719552839));
#180482=CARTESIAN_POINT('Ctrl Pts',(31.8501107931046,-65.8583505767601,
-55.737779177983));
#180483=CARTESIAN_POINT('Ctrl Pts',(31.85,-65.8583711767947,-55.7438732287223));
#180484=CARTESIAN_POINT('Ctrl Pts',(31.85,-65.8583711767947,-55.74995));
#180485=CARTESIAN_POINT('',(31.85,67.7009572055632,-55.74995));
#180486=CARTESIAN_POINT('Origin',(31.85,67.7009572055632,-55.24995));
#180487=CARTESIAN_POINT('',(31.85,-65.8583711767947,-59.64995));
#180488=CARTESIAN_POINT('',(31.85,-65.8583711767947,-55.24995));
#180489=CARTESIAN_POINT('Ctrl Pts',(31.85,-65.8583711767947,-59.64995));
#180490=CARTESIAN_POINT('Ctrl Pts',(31.85,-65.8583711767784,-59.8463349320561));
#180491=CARTESIAN_POINT('Ctrl Pts',(31.85,-65.819181055996,-60.0425718399612));
#180492=CARTESIAN_POINT('Ctrl Pts',(31.85,-65.6683275916687,-60.4053784571341));
#180493=CARTESIAN_POINT('Ctrl Pts',(31.85,-65.5567235699328,-60.5717700902076));
#180494=CARTESIAN_POINT('Ctrl Pts',(31.85,-65.2779827136761,-60.8494502533521));
#180495=CARTESIAN_POINT('Ctrl Pts',(31.85,-65.1109554916676,-60.9606295880612));
#180496=CARTESIAN_POINT('Ctrl Pts',(31.85,-64.7467630120136,-61.1109090094727));
#180497=CARTESIAN_POINT('Ctrl Pts',(31.85,-64.5497765111262,-61.149949999985));
#180498=CARTESIAN_POINT('Ctrl Pts',(31.85,-64.3526414204797,-61.14995));
#180499=CARTESIAN_POINT('Ctrl Pts',(31.85,-65.8583711767947,-59.64995));
#180500=CARTESIAN_POINT('Ctrl Pts',(31.8499999999999,-65.3127169262601,
-59.64995));
#180501=CARTESIAN_POINT('Ctrl Pts',(31.3064221286262,-65.3602738277489,
-59.64995));
#180502=CARTESIAN_POINT('Ctrl Pts',(31.85,-65.8583711767784,-59.8463349320561));
#180503=CARTESIAN_POINT('Ctrl Pts',(31.8499999999999,-65.3127169262533,
-59.7746029379323));
#180504=CARTESIAN_POINT('Ctrl Pts',(31.3064221286269,-65.3602738277488,
-59.7808732880376));
#180505=CARTESIAN_POINT('Ctrl Pts',(31.85,-65.819181055996,-60.0425718399612));
#180506=CARTESIAN_POINT('Ctrl Pts',(31.8499999999999,-65.2892961879233,
-59.8989712332632));
#180507=CARTESIAN_POINT('Ctrl Pts',(31.3075563441358,-65.3340478495507,
-59.9116978933073));
#180508=CARTESIAN_POINT('Ctrl Pts',(31.85,-65.6683275916687,-60.4053784571341));
#180509=CARTESIAN_POINT('Ctrl Pts',(31.8499999999999,-65.1974676446973,
-60.1322291512615));
#180510=CARTESIAN_POINT('Ctrl Pts',(31.3119222489988,-65.2330969061508,
-60.1535689714229));
#180511=CARTESIAN_POINT('Ctrl Pts',(31.85,-65.5567235699328,-60.5717700902076));
#180512=CARTESIAN_POINT('Ctrl Pts',(31.8499999999999,-65.1294009926956,
-60.2406767152616));
#180513=CARTESIAN_POINT('Ctrl Pts',(31.3151522214972,-65.1584116390162,
-60.2644967268053));
#180514=CARTESIAN_POINT('Ctrl Pts',(31.85,-65.2779827136761,-60.8494502533521));
#180515=CARTESIAN_POINT('Ctrl Pts',(31.8499999999999,-64.9553741448238,
-60.4261994932778));
#180516=CARTESIAN_POINT('Ctrl Pts',(31.3232193617865,-64.9718786181899,
-60.4496168355678));
#180517=CARTESIAN_POINT('Ctrl Pts',(31.85,-65.1109554916676,-60.9606295880612));
#180518=CARTESIAN_POINT('Ctrl Pts',(31.8499999999993,-64.8499435605403,
-60.5031527166052));
#180519=CARTESIAN_POINT('Ctrl Pts',(31.3280533572402,-64.8601042170482,
-60.5237363920412));
#180520=CARTESIAN_POINT('Ctrl Pts',(31.85,-64.7467630120136,-61.1109090094727));
#180521=CARTESIAN_POINT('Ctrl Pts',(31.8500000000006,-64.6146765878316,
-60.6120353079394));
#180522=CARTESIAN_POINT('Ctrl Pts',(31.3385935839747,-64.6163870802633,
-60.6239226729814));
#180523=CARTESIAN_POINT('Ctrl Pts',(31.85,-64.5497765111262,-61.149949999985));
#180524=CARTESIAN_POINT('Ctrl Pts',(31.85,-64.4853598419829,-60.6442102195366));
#180525=CARTESIAN_POINT('Ctrl Pts',(31.3442946417934,-64.4845639684081,
-60.64995));
#180526=CARTESIAN_POINT('Ctrl Pts',(31.85,-64.3526414204797,-61.14995));
#180527=CARTESIAN_POINT('Ctrl Pts',(31.8499999999999,-64.3526414204797,
-60.64995));
#180528=CARTESIAN_POINT('Ctrl Pts',(31.35,-64.3526414204797,-60.64995));
#180529=CARTESIAN_POINT('',(31.3064221286262,-65.3602738277489,-59.64995));
#180530=CARTESIAN_POINT('Origin',(31.35,-65.8583711767947,-59.64995));
#180531=CARTESIAN_POINT('Ctrl Pts',(31.35,-64.3526414204797,-60.64995));
#180532=CARTESIAN_POINT('Ctrl Pts',(31.3487470950754,-64.3816118030486,
-60.64995));
#180533=CARTESIAN_POINT('Ctrl Pts',(31.3475587391951,-64.4093403523785,
-60.6487118041122));
#180534=CARTESIAN_POINT('Ctrl Pts',(31.346427856392,-64.4357461897957,-60.6465429519375));
#180535=CARTESIAN_POINT('Ctrl Pts',(31.3452494858262,-64.4632608548783,
-60.6442830258363));
#180536=CARTESIAN_POINT('Ctrl Pts',(31.3441335581122,-64.4893398656373,
-60.6410132280374));
#180537=CARTESIAN_POINT('Ctrl Pts',(31.3430764842574,-64.5139421997014,
-60.6370534671247));
#180538=CARTESIAN_POINT('Ctrl Pts',(31.3421996476743,-64.5343496919854,
-60.6337688685959));
#180539=CARTESIAN_POINT('Ctrl Pts',(31.3413634057054,-64.5537422796669,
-60.6300090684365));
#180540=CARTESIAN_POINT('Ctrl Pts',(31.3405675225963,-64.5721172680631,
-60.6259392754056));
#180541=CARTESIAN_POINT('Ctrl Pts',(31.3395582117953,-64.5954197782508,
-60.6207781078708));
#180542=CARTESIAN_POINT('Ctrl Pts',(31.3386137704587,-64.6170853163577,
-60.6151198747361));
#180543=CARTESIAN_POINT('Ctrl Pts',(31.3377364626481,-64.6371397607276,
-60.6092623723784));
#180544=CARTESIAN_POINT('Ctrl Pts',(31.3374506843755,-64.643672387478,-60.6073543226769));
#180545=CARTESIAN_POINT('Ctrl Pts',(31.3371720492791,-64.6500342866337,
-60.6054247760897));
#180546=CARTESIAN_POINT('Ctrl Pts',(31.3369006858754,-64.6562269271424,
-60.6034830012694));
#180547=CARTESIAN_POINT('Ctrl Pts',(31.3363484762979,-64.66882860943,-60.5995315964807));
#180548=CARTESIAN_POINT('Ctrl Pts',(31.335826363855,-64.6807292206441,-60.595530097897));
#180549=CARTESIAN_POINT('Ctrl Pts',(31.3353356540994,-64.6919436833211,
-60.5915501615662));
#180550=CARTESIAN_POINT('Ctrl Pts',(31.3350902992217,-64.6975509146595,
-60.5895601934008));
#180551=CARTESIAN_POINT('Ctrl Pts',(31.3348527917206,-64.7029865712008,
-60.5875755120395));
#180552=CARTESIAN_POINT('Ctrl Pts',(31.3346233227297,-64.7082528376098,
-60.5856042391339));
#180553=CARTESIAN_POINT('Ctrl Pts',(31.3345085882343,-64.7108859708144,
-60.584618602681));
#180554=CARTESIAN_POINT('Ctrl Pts',(31.3343958631594,-64.7134767541197,
-60.5836363114746));
#180555=CARTESIAN_POINT('Ctrl Pts',(31.3342851709446,-64.7160254554421,
-60.5826583364361));
#180556=CARTESIAN_POINT('Ctrl Pts',(31.3342092440951,-64.7177736801244,
-60.5819875163263));
#180557=CARTESIAN_POINT('Ctrl Pts',(31.3341734959929,-64.7185902026884,
-60.5816721106983));
#180558=CARTESIAN_POINT('Ctrl Pts',(31.3340972739735,-64.7203521872788,
-60.5809867219852));
#180559=CARTESIAN_POINT('Ctrl Pts',(31.3340623734561,-64.7211589643018,
-60.5806728963884));
#180560=CARTESIAN_POINT('Ctrl Pts',(31.3340189765473,-64.7221638367264,
-60.5802811765834));
#180561=CARTESIAN_POINT('Ctrl Pts',(31.3339592160933,-64.7235455787786,
-60.5797383010624));
#180562=CARTESIAN_POINT('Ctrl Pts',(31.3325183894219,-64.7568594287527,
-60.5666495529621));
#180563=CARTESIAN_POINT('Ctrl Pts',(31.3311478367635,-64.7887241291916,
-60.5520895209809));
#180564=CARTESIAN_POINT('Ctrl Pts',(31.3298415410329,-64.8190709044992,
-60.5363617340931));
#180565=CARTESIAN_POINT('Ctrl Pts',(31.3285010284235,-64.8502125778615,
-60.5202219763426));
#180566=CARTESIAN_POINT('Ctrl Pts',(31.3272282106861,-64.8797560794186,
-60.5028529740901));
#180567=CARTESIAN_POINT('Ctrl Pts',(31.3260210452493,-64.9076780624719,
-60.4845643907951));
#180568=CARTESIAN_POINT('Ctrl Pts',(31.3259189711447,-64.9100390573538,
-60.4830179658341));
#180569=CARTESIAN_POINT('Ctrl Pts',(31.3258173688633,-64.912388486247,-60.4814649529386));
#180570=CARTESIAN_POINT('Ctrl Pts',(31.3257162384798,-64.9147263500048,
-60.4799055318768));
#180571=CARTESIAN_POINT('Ctrl Pts',(31.3244849327799,-64.9431908417874,
-60.4609189130664));
#180572=CARTESIAN_POINT('Ctrl Pts',(31.32332326249,-64.9699372570743,-60.4409847513383));
#180573=CARTESIAN_POINT('Ctrl Pts',(31.3222335064864,-64.9949916435422,
-60.420412040864));
#180574=CARTESIAN_POINT('Ctrl Pts',(31.3216886284846,-65.0075188367761,
-60.4101256856269));
#180575=CARTESIAN_POINT('Ctrl Pts',(31.3211617893047,-65.019623711469,-60.3996792360251));
#180576=CARTESIAN_POINT('Ctrl Pts',(31.3206536010315,-65.0313132637831,
-60.3891084432431));
#180577=CARTESIAN_POINT('Ctrl Pts',(31.320416588106,-65.0367651310102,-60.3841783520656));
#180578=CARTESIAN_POINT('Ctrl Pts',(31.3201961142949,-65.0418050198924,
-60.3795181564444));
#180579=CARTESIAN_POINT('Ctrl Pts',(31.319975271238,-65.0468893137778,-60.3747215661699));
#180580=CARTESIAN_POINT('Ctrl Pts',(31.3197604813291,-65.0518342508541,
-60.370056446957));
#180581=CARTESIAN_POINT('Ctrl Pts',(31.3195453554136,-65.0568213438128,
-60.3652622205224));
#180582=CARTESIAN_POINT('Ctrl Pts',(31.3193114502791,-65.0622374643184,
-60.3599307007192));
#180583=CARTESIAN_POINT('Ctrl Pts',(31.3192701938261,-65.0631927657966,
-60.3589903212088));
#180584=CARTESIAN_POINT('Ctrl Pts',(31.319228345048,-65.0641613218921,-60.3580331354422));
#180585=CARTESIAN_POINT('Ctrl Pts',(31.3191857916419,-65.065145128603,-60.3570567811865));
#180586=CARTESIAN_POINT('Ctrl Pts',(31.3178695544998,-65.0955756640795,
-60.3268567607105));
#180587=CARTESIAN_POINT('Ctrl Pts',(31.3166685276156,-65.1238062071651,
-60.2949641541196));
#180588=CARTESIAN_POINT('Ctrl Pts',(31.3155715571072,-65.1497092684046,
-60.2617220236787));
#180589=CARTESIAN_POINT('Ctrl Pts',(31.3144615648519,-65.1759198156724,
-60.2280852877289));
#180590=CARTESIAN_POINT('Ctrl Pts',(31.3134581230547,-65.1997473984253,
-60.1930673110297));
#180591=CARTESIAN_POINT('Ctrl Pts',(31.3125543591512,-65.2211134628954,
-60.1570220982733));
#180592=CARTESIAN_POINT('Ctrl Pts',(31.3116396515752,-65.2427382489321,
-60.1205404142181));
#180593=CARTESIAN_POINT('Ctrl Pts',(31.3108270658856,-65.2618417185149,
-60.0830069551332));
#180594=CARTESIAN_POINT('Ctrl Pts',(31.3101140607359,-65.278394823922,-60.0447796545834));
#180595=CARTESIAN_POINT('Ctrl Pts',(31.3093877892809,-65.2952559194645,
-60.0058410898217));
#180596=CARTESIAN_POINT('Ctrl Pts',(31.3087648557882,-65.3094710608044,
-59.9661831060864));
#180597=CARTESIAN_POINT('Ctrl Pts',(31.3082470591246,-65.3210608090817,
-59.9261671551741));
#180598=CARTESIAN_POINT('Ctrl Pts',(31.3077236909507,-65.3327752634566,
-59.8857206312273));
#180599=CARTESIAN_POINT('Ctrl Pts',(31.3073077631725,-65.3418078518286,
-59.8449088093039));
#180600=CARTESIAN_POINT('Ctrl Pts',(31.3070053121221,-65.3482275697917,
-59.8040810751356));
#180601=CARTESIAN_POINT('Ctrl Pts',(31.3066980640645,-65.3547491073195,
-59.7626057950556));
#180602=CARTESIAN_POINT('Ctrl Pts',(31.3065079517797,-65.3585745879892,
-59.721114479069));
#180603=CARTESIAN_POINT('Ctrl Pts',(31.3064451414349,-65.3598202116218,
-59.6799427686078));
#180604=CARTESIAN_POINT('Ctrl Pts',(31.3064298584737,-65.3601232957331,
-59.6699249020953));
#180605=CARTESIAN_POINT('Ctrl Pts',(31.3064221286262,-65.3602738277488,
-59.6599258026955));
#180606=CARTESIAN_POINT('Ctrl Pts',(31.3064221286262,-65.3602738277488,
-59.64995));
#180607=CARTESIAN_POINT('Origin',(0.,-12.9675000200281,-60.64995));
#180608=CARTESIAN_POINT('',(28.6150130758292,-64.5919217712362,-60.64995));
#180609=CARTESIAN_POINT('Origin',(0.,-12.9675000200281,-60.64995));
#180610=CARTESIAN_POINT('',(4.6996065532056,-66.6842487255793,-60.64995));
#180611=CARTESIAN_POINT('Origin',(0.,-12.9675000200281,-61.64995));
#180612=CARTESIAN_POINT('Ctrl Pts',(28.6150130758292,-64.5919217712362,
-60.64995));
#180613=CARTESIAN_POINT('Ctrl Pts',(28.5105903987178,-64.6227530253959,
-60.64995));
#180614=CARTESIAN_POINT('Ctrl Pts',(28.3946324532739,-64.6568987835949,
-60.6507816129708));
#180615=CARTESIAN_POINT('Ctrl Pts',(28.2034335369725,-64.7128787401875,
-60.6541161203403));
#180616=CARTESIAN_POINT('Ctrl Pts',(28.1035194656054,-64.7420598028733,
-60.6563073997376));
#180617=CARTESIAN_POINT('Ctrl Pts',(27.9794226958293,-64.7781550526993,
-60.6599865693629));
#180618=CARTESIAN_POINT('Ctrl Pts',(27.9154952583806,-64.7967124481223,
-60.6621339738737));
#180619=CARTESIAN_POINT('Ctrl Pts',(27.8876955404672,-64.8047745920356,
-60.6631231848173));
#180620=CARTESIAN_POINT('Ctrl Pts',(27.8690730559331,-64.8101735462903,
-60.6637982981373));
#180621=CARTESIAN_POINT('Ctrl Pts',(27.8582817452337,-64.8133010022486,
-60.6641976300943));
#180622=CARTESIAN_POINT('Ctrl Pts',(27.7228740588381,-64.8525331605392,
-60.6692875251728));
#180623=CARTESIAN_POINT('Ctrl Pts',(27.5316692268163,-64.9075566246321,
-60.6782360197703));
#180624=CARTESIAN_POINT('Ctrl Pts',(27.3086424509084,-64.9713454327537,
-60.6917045527587));
#180625=CARTESIAN_POINT('Ctrl Pts',(27.1971541509212,-65.0031671303415,
-60.6991865024269));
#180626=CARTESIAN_POINT('Ctrl Pts',(27.1414179550069,-65.019063362529,-60.7031131487649));
#180627=CARTESIAN_POINT('Ctrl Pts',(27.1175328956354,-65.0258732819076,
-60.7048356431027));
#180628=CARTESIAN_POINT('Ctrl Pts',(27.1016099604076,-65.0304126589274,
-60.7059927668089));
#180629=CARTESIAN_POINT('Ctrl Pts',(27.0955676348509,-65.0321351095429,
-60.7064341515018));
#180630=CARTESIAN_POINT('Ctrl Pts',(26.4533713134215,-65.2151811972912,
-60.7538140910806));
#180631=CARTESIAN_POINT('Ctrl Pts',(25.9451849881814,-65.3545420411632,
-60.8199026865955));
#180632=CARTESIAN_POINT('Ctrl Pts',(25.5598256882386,-65.4594929016689,
-60.8818893816956));
#180633=CARTESIAN_POINT('Origin',(25.2,67.7009572055632,-55.24995));
#180634=CARTESIAN_POINT('',(25.2,-66.3526821257161,-60.0322609860583));
#180635=CARTESIAN_POINT('Ctrl Pts',(25.2,-65.7473676730038,-61.2659196908451));
#180636=CARTESIAN_POINT('Ctrl Pts',(25.2,-65.7793674058564,-61.2419322158013));
#180637=CARTESIAN_POINT('Ctrl Pts',(25.2,-65.8101247224077,-61.2167624788248));
#180638=CARTESIAN_POINT('Ctrl Pts',(25.2,-65.8397093268158,-61.190493472528));
#180639=CARTESIAN_POINT('Ctrl Pts',(25.2,-65.8701731473596,-61.1634437853781));
#180640=CARTESIAN_POINT('Ctrl Pts',(25.2,-65.8993940496694,-61.1352280130909));
#180641=CARTESIAN_POINT('Ctrl Pts',(25.2,-65.9274189899594,-61.1058889488372));
#180642=CARTESIAN_POINT('Ctrl Pts',(25.2,-65.9536751279189,-61.0784016282335));
#180643=CARTESIAN_POINT('Ctrl Pts',(25.2,-65.9788815373658,-61.0499274395305));
#180644=CARTESIAN_POINT('Ctrl Pts',(25.2,-66.003048363658,-61.0204714365432));
#180645=CARTESIAN_POINT('Ctrl Pts',(25.2,-66.0310884832234,-60.9862944272951));
#180646=CARTESIAN_POINT('Ctrl Pts',(25.2,-66.0577887607455,-60.9507091443266));
#180647=CARTESIAN_POINT('Ctrl Pts',(25.2,-66.0829136816561,-60.9139799086626));
#180648=CARTESIAN_POINT('Ctrl Pts',(25.2,-66.1080535088058,-60.8772288820934));
#180649=CARTESIAN_POINT('Ctrl Pts',(25.2,-66.1316155749522,-60.8393332860652));
#180650=CARTESIAN_POINT('Ctrl Pts',(25.2,-66.1534043153338,-60.8005903813967));
#180651=CARTESIAN_POINT('Ctrl Pts',(25.2,-66.1680937996896,-60.7744707764053));
#180652=CARTESIAN_POINT('Ctrl Pts',(25.2,-66.181978126642,-60.7479667212963));
#180653=CARTESIAN_POINT('Ctrl Pts',(25.2,-66.195009507084,-60.7211749919405));
#180654=CARTESIAN_POINT('Ctrl Pts',(25.2,-66.2246788862433,-60.6601765443753));
#180655=CARTESIAN_POINT('Ctrl Pts',(25.2,-66.2502610540202,-60.5971407842143));
#180656=CARTESIAN_POINT('Ctrl Pts',(25.2,-66.271692317881,-60.5326135007579));
#180657=CARTESIAN_POINT('Ctrl Pts',(25.2,-66.2932651285273,-60.4676600348046));
#180658=CARTESIAN_POINT('Ctrl Pts',(25.2,-66.310632319108,-60.4011940592067));
#180659=CARTESIAN_POINT('Ctrl Pts',(25.2,-66.3236799285615,-60.3337525436261));
#180660=CARTESIAN_POINT('Ctrl Pts',(25.2,-66.3364083911875,-60.2679606594062));
#180661=CARTESIAN_POINT('Ctrl Pts',(25.2,-66.3450260486911,-60.2012392211527));
#180662=CARTESIAN_POINT('Ctrl Pts',(25.2,-66.3493785138873,-60.1340856777927));
#180663=CARTESIAN_POINT('Ctrl Pts',(25.2,-66.3515726828268,-60.1002321689489));
#180664=CARTESIAN_POINT('Ctrl Pts',(25.2,-66.3526821241379,-60.0662689342669));
#180665=CARTESIAN_POINT('Ctrl Pts',(25.2,-66.3526821257161,-60.0322609860583));
#180666=CARTESIAN_POINT('',(25.2,-66.3526821257161,-55.74995));
#180667=CARTESIAN_POINT('',(25.2,-66.3526821257161,-55.24995));
#180668=CARTESIAN_POINT('',(25.2,67.7009572055632,-55.74995));
#180669=CARTESIAN_POINT('Ctrl Pts',(25.2,-65.6297999215446,-61.3450435291692));
#180670=CARTESIAN_POINT('Ctrl Pts',(25.2,-65.4367639336817,-61.0276731545924));
#180671=CARTESIAN_POINT('Ctrl Pts',(25.5556761922697,-65.381444422022,-60.9359047563459));
#180672=CARTESIAN_POINT('Ctrl Pts',(25.2,-65.8726226849417,-61.1992598451423));
#180673=CARTESIAN_POINT('Ctrl Pts',(25.2,-65.616119634334,-60.9126182039811));
#180674=CARTESIAN_POINT('Ctrl Pts',(25.5637941426607,-65.5425594624733,
-60.8363160388081));
#180675=CARTESIAN_POINT('Ctrl Pts',(25.2,-66.0709810864818,-60.9761699132095));
#180676=CARTESIAN_POINT('Ctrl Pts',(25.2,-65.7526726487211,-60.7337823944688));
#180677=CARTESIAN_POINT('Ctrl Pts',(25.5808970595347,-65.6733118931737,
-60.6825252684264));
#180678=CARTESIAN_POINT('Ctrl Pts',(25.2,-66.3190379296928,-60.466180071647));
#180679=CARTESIAN_POINT('Ctrl Pts',(25.2,-65.9037505527713,-60.3438811720847));
#180680=CARTESIAN_POINT('Ctrl Pts',(25.6216004744624,-65.8351484356237,
-60.3310508170863));
#180681=CARTESIAN_POINT('Ctrl Pts',(25.2,-66.3724466929311,-60.1737447607176));
#180682=CARTESIAN_POINT('Ctrl Pts',(25.1999999999999,-65.9181936015569,
-60.1252597984462));
#180683=CARTESIAN_POINT('Ctrl Pts',(25.645585200326,-65.8686915591478,-60.1295475465719));
#180684=CARTESIAN_POINT('Ctrl Pts',(25.2,-66.3461220698509,-59.8897891189412));
#180685=CARTESIAN_POINT('Ctrl Pts',(25.2,-65.8782260298731,-59.9318867276305));
#180686=CARTESIAN_POINT('Ctrl Pts',(25.6688194082641,-65.8491452831382,
-59.9342430075604));
#180687=CARTESIAN_POINT('',(25.6564221281367,-65.8545847710806,-60.0322609860566));
#180688=CARTESIAN_POINT('Ctrl Pts',(25.6564221286262,-65.8545847766702,
-60.0322609860583));
#180689=CARTESIAN_POINT('Ctrl Pts',(25.6426414728709,-65.855767307974,-60.1482566280702));
#180690=CARTESIAN_POINT('Ctrl Pts',(25.631577400267,-65.8390726440188,-60.2474362362412));
#180691=CARTESIAN_POINT('Ctrl Pts',(25.6175941734372,-65.8084997917476,
-60.365156334888));
#180692=CARTESIAN_POINT('Ctrl Pts',(25.6134196234492,-65.7973422361654,
-60.3994162323209));
#180693=CARTESIAN_POINT('Ctrl Pts',(25.6079980779481,-65.781066673351,-60.44373294877));
#180694=CARTESIAN_POINT('Ctrl Pts',(25.6063320607753,-65.775711534389,-60.4573306677679));
#180695=CARTESIAN_POINT('Ctrl Pts',(25.6040646535256,-65.7679639572994,
-60.4760386697017));
#180696=CARTESIAN_POINT('Ctrl Pts',(25.6029888858038,-65.7641608584646,
-60.4849706489919));
#180697=CARTESIAN_POINT('Ctrl Pts',(25.6018397215795,-65.7598809973385,
-60.4946694093824));
#180698=CARTESIAN_POINT('Ctrl Pts',(25.6013703968771,-65.7580836463387,
-60.4986731111241));
#180699=CARTESIAN_POINT('Ctrl Pts',(25.6010627166154,-65.7568939550516,
-60.5013084614098));
#180700=CARTESIAN_POINT('Ctrl Pts',(25.6010641599103,-65.7569055709527,
-60.501290081512));
#180701=CARTESIAN_POINT('Ctrl Pts',(25.5814801284086,-65.6796646649316,
-60.6704949285918));
#180702=CARTESIAN_POINT('Ctrl Pts',(25.5679173424065,-65.5708000415401,
-60.7954955609311));
#180703=CARTESIAN_POINT('Ctrl Pts',(25.5598256882386,-65.4594929016689,
-60.8818893816956));
#180704=CARTESIAN_POINT('Origin',(25.7,-66.3526821257161,-60.0322609860583));
#180705=CARTESIAN_POINT('Ctrl Pts',(41.5,-63.4208871539288,-61.14995));
#180706=CARTESIAN_POINT('Ctrl Pts',(41.4999999999999,-63.4208871539288,
-60.64995));
#180707=CARTESIAN_POINT('Ctrl Pts',(42.,-63.4208871539288,-60.64995));
#180708=CARTESIAN_POINT('Ctrl Pts',(41.5,-63.6180222445752,-61.149949999985));
#180709=CARTESIAN_POINT('Ctrl Pts',(41.5,-63.5520336237608,-60.6556217969809));
#180710=CARTESIAN_POINT('Ctrl Pts',(41.9942946417934,-63.5528097018572,
-60.64995));
#180711=CARTESIAN_POINT('Ctrl Pts',(41.5,-63.8150087454628,-61.1109090094727));
#180712=CARTESIAN_POINT('Ctrl Pts',(41.4999999999993,-63.6863151114373,
-60.6353187454032));
#180713=CARTESIAN_POINT('Ctrl Pts',(41.9885935839755,-63.6846328137124,
-60.6239226729814));
#180714=CARTESIAN_POINT('Ctrl Pts',(41.5,-64.1792012251166,-60.9606295880612));
#180715=CARTESIAN_POINT('Ctrl Pts',(41.5000000000007,-63.9376903302796,
-60.5426326522472));
#180716=CARTESIAN_POINT('Ctrl Pts',(41.9780533572395,-63.9283499504973,
-60.5237363920413));
#180717=CARTESIAN_POINT('Ctrl Pts',(41.5,-64.3462284471252,-60.849450253352));
#180718=CARTESIAN_POINT('Ctrl Pts',(41.5,-64.0549974136357,-60.4706504746468));
#180719=CARTESIAN_POINT('Ctrl Pts',(41.9732193617859,-64.0401243516391,
-60.4496168355678));
#180720=CARTESIAN_POINT('Ctrl Pts',(41.5,-64.6249693033818,-60.5717700902076));
#180721=CARTESIAN_POINT('Ctrl Pts',(41.4999999999999,-64.2519280277007,
-60.2852157712117));
#180722=CARTESIAN_POINT('Ctrl Pts',(41.9651522214979,-64.2266573724653,
-60.2644967268053));
#180723=CARTESIAN_POINT('Ctrl Pts',(41.5,-64.7365733251178,-60.4053784571342));
#180724=CARTESIAN_POINT('Ctrl Pts',(41.5,-64.3319461592471,-60.1718710142637));
#180725=CARTESIAN_POINT('Ctrl Pts',(41.9619222489988,-64.3013426395998,
-60.153568971423));
#180726=CARTESIAN_POINT('Ctrl Pts',(41.5,-64.8874267894451,-60.0425718399611));
#180727=CARTESIAN_POINT('Ctrl Pts',(41.5,-64.4400579753494,-59.9224177216068));
#180728=CARTESIAN_POINT('Ctrl Pts',(41.9575563441358,-64.4022935829999,
-59.9116978933072));
#180729=CARTESIAN_POINT('Ctrl Pts',(41.5,-64.9266169102275,-59.8463349320562));
#180730=CARTESIAN_POINT('Ctrl Pts',(41.5,-64.4684513232201,-59.7861314644994));
#180731=CARTESIAN_POINT('Ctrl Pts',(41.9564221286289,-64.4285195611977,
-59.7808732880376));
#180732=CARTESIAN_POINT('Ctrl Pts',(41.5,-64.9266169102438,-59.64995));
#180733=CARTESIAN_POINT('Ctrl Pts',(41.5,-64.4684513232351,-59.64995));
#180734=CARTESIAN_POINT('Ctrl Pts',(41.9564221286262,-64.428519561198,-59.64995));
#180735=CARTESIAN_POINT('',(41.9564221286262,-64.428519561198,-59.64995));
#180736=CARTESIAN_POINT('',(41.5,-64.9266169102438,-59.64995));
#180737=CARTESIAN_POINT('Origin',(42.,-64.9266169102438,-59.64995));
#180738=CARTESIAN_POINT('Ctrl Pts',(41.5,-63.4208871539288,-61.14995));
#180739=CARTESIAN_POINT('Ctrl Pts',(41.5,-63.6180222445752,-61.149949999985));
#180740=CARTESIAN_POINT('Ctrl Pts',(41.5,-63.8150087454628,-61.1109090094727));
#180741=CARTESIAN_POINT('Ctrl Pts',(41.5,-64.1792012251166,-60.9606295880612));
#180742=CARTESIAN_POINT('Ctrl Pts',(41.5,-64.3462284471252,-60.849450253352));
#180743=CARTESIAN_POINT('Ctrl Pts',(41.5,-64.6249693033818,-60.5717700902076));
#180744=CARTESIAN_POINT('Ctrl Pts',(41.5,-64.7365733251178,-60.4053784571342));
#180745=CARTESIAN_POINT('Ctrl Pts',(41.5,-64.8874267894451,-60.0425718399611));
#180746=CARTESIAN_POINT('Ctrl Pts',(41.5,-64.9266169102275,-59.8463349320562));
#180747=CARTESIAN_POINT('Ctrl Pts',(41.5,-64.9266169102438,-59.64995));
#180748=CARTESIAN_POINT('Ctrl Pts',(41.9564221286262,-64.428519561198,-59.64995));
#180749=CARTESIAN_POINT('Ctrl Pts',(41.9564221286262,-64.428519561198,-59.6947437536983));
#180750=CARTESIAN_POINT('Ctrl Pts',(41.9565549254446,-64.4254489573896,
-59.740006512832));
#180751=CARTESIAN_POINT('Ctrl Pts',(41.9568254006969,-64.4191948742738,
-59.7853172178034));
#180752=CARTESIAN_POINT('Ctrl Pts',(41.9570925832862,-64.413016925991,-59.8300763274576));
#180753=CARTESIAN_POINT('Ctrl Pts',(41.9574941133679,-64.4037325183291,
-59.8748822572172));
#180754=CARTESIAN_POINT('Ctrl Pts',(41.9580343638515,-64.3912405383823,
-59.9192791403161));
#180755=CARTESIAN_POINT('Ctrl Pts',(41.9584577829345,-64.381450000743,-59.9540750139001));
#180756=CARTESIAN_POINT('Ctrl Pts',(41.9589664057685,-64.3696893333576,
-59.9886186673433));
#180757=CARTESIAN_POINT('Ctrl Pts',(41.9595621871816,-64.3559133355721,
-60.0226684875927));
#180758=CARTESIAN_POINT('Ctrl Pts',(41.9596203911713,-64.3545675097113,
-60.0259949347482));
#180759=CARTESIAN_POINT('Ctrl Pts',(41.9596794270429,-64.3532024486048,
-60.0293166614153));
#180760=CARTESIAN_POINT('Ctrl Pts',(41.9597392965673,-64.3518181112998,
-60.0326334323651));
#180761=CARTESIAN_POINT('Ctrl Pts',(41.9605100399423,-64.3339965432011,
-60.0753326062864));
#180762=CARTESIAN_POINT('Ctrl Pts',(41.9614188288922,-64.3129830065508,
-60.1171993183685));
#180763=CARTESIAN_POINT('Ctrl Pts',(41.9624618901908,-64.2888647480389,
-60.1577697839508));
#180764=CARTESIAN_POINT('Ctrl Pts',(41.9634583716055,-64.2658235361815,
-60.1965284983154));
#180765=CARTESIAN_POINT('Ctrl Pts',(41.9645773576394,-64.2399497026142,
-60.2341031968009));
#180766=CARTESIAN_POINT('Ctrl Pts',(41.9658147921719,-64.211337035279,-60.2700569674147));
#180767=CARTESIAN_POINT('Ctrl Pts',(41.9663964129123,-64.1978884686497,
-60.2869560098567));
#180768=CARTESIAN_POINT('Ctrl Pts',(41.9670041917906,-64.1838350586287,
-60.303496408054));
#180769=CARTESIAN_POINT('Ctrl Pts',(41.967637607018,-64.1691888703163,-60.3196288077294));
#180770=CARTESIAN_POINT('Ctrl Pts',(41.9678621341568,-64.1639972256964,
-60.3253472707311));
#180771=CARTESIAN_POINT('Ctrl Pts',(41.9681018562117,-64.1584542355935,
-60.3313130455697));
#180772=CARTESIAN_POINT('Ctrl Pts',(41.9683408943949,-64.1529269486012,
-60.3371156968734));
#180773=CARTESIAN_POINT('Ctrl Pts',(41.9685870780861,-64.1472344358157,
-60.3430918053661));
#180774=CARTESIAN_POINT('Ctrl Pts',(41.9688325293532,-64.1415587421265,
-60.348894747227));
#180775=CARTESIAN_POINT('Ctrl Pts',(41.9690581151941,-64.1363421513913,
-60.3541155158986));
#180776=CARTESIAN_POINT('Ctrl Pts',(41.969101441238,-64.1353402523451,-60.3551182173598));
#180777=CARTESIAN_POINT('Ctrl Pts',(41.9691440297757,-64.1343553976018,
-60.3560995557786));
#180778=CARTESIAN_POINT('Ctrl Pts',(41.9691857390395,-64.1333908643444,
-60.3570567834876));
#180779=CARTESIAN_POINT('Ctrl Pts',(41.9701337860241,-64.1114671293489,
-60.3788144641718));
#180780=CARTESIAN_POINT('Ctrl Pts',(41.9711541356061,-64.087874347133,-60.40019522961));
#180781=CARTESIAN_POINT('Ctrl Pts',(41.972249052733,-64.0625579786825,-60.4209274424502));
#180782=CARTESIAN_POINT('Ctrl Pts',(41.9733241881793,-64.0376989967361,
-60.4412850899425));
#180783=CARTESIAN_POINT('Ctrl Pts',(41.9744712328351,-64.0111778749262,
-60.4610175323995));
#180784=CARTESIAN_POINT('Ctrl Pts',(41.975690944026,-63.9829750168074,-60.4798306482905));
#180785=CARTESIAN_POINT('Ctrl Pts',(41.9768514204353,-63.9561418191073,
-60.4977301128035));
#180786=CARTESIAN_POINT('Ctrl Pts',(41.9780777938133,-63.9277849140972,
-60.5147982848406));
#180787=CARTESIAN_POINT('Ctrl Pts',(41.979369575909,-63.8979155913966,-60.5307488744733));
#180788=CARTESIAN_POINT('Ctrl Pts',(41.9806262844306,-63.8688572598861,
-60.5462663847288));
#180789=CARTESIAN_POINT('Ctrl Pts',(41.981944926866,-63.8383668570856,-60.5607262877677));
#180790=CARTESIAN_POINT('Ctrl Pts',(41.9833234706075,-63.8064913821049,
-60.5738295325114));
#180791=CARTESIAN_POINT('Ctrl Pts',(41.9833461253665,-63.8059675458395,
-60.5740448690607));
#180792=CARTESIAN_POINT('Ctrl Pts',(41.9833687961921,-63.8054433380748,
-60.5742598379184));
#180793=CARTESIAN_POINT('Ctrl Pts',(41.9833914830727,-63.8049187590774,
-60.5744744380238));
#180794=CARTESIAN_POINT('Ctrl Pts',(41.9835053586064,-63.8022856640096,
-60.5755516113038));
#180795=CARTESIAN_POINT('Ctrl Pts',(41.9836502170309,-63.7989358208272,
-60.5769043222385));
#180796=CARTESIAN_POINT('Ctrl Pts',(41.9837705714856,-63.796152507233,-60.5780123789929));
#180797=CARTESIAN_POINT('Ctrl Pts',(41.9838490691014,-63.794337173667,-60.5787350760773));
#180798=CARTESIAN_POINT('Ctrl Pts',(41.9839171188373,-63.79276339423,-60.5793550577177));
#180799=CARTESIAN_POINT('Ctrl Pts',(41.9839591709512,-63.7917907964698,
-60.5797369926548));
#180800=CARTESIAN_POINT('Ctrl Pts',(41.984631713491,-63.7762359692054,-60.5858453060977));
#180801=CARTESIAN_POINT('Ctrl Pts',(41.9853765198597,-63.7590118122209,
-60.5921640965077));
#180802=CARTESIAN_POINT('Ctrl Pts',(41.9861963547554,-63.7400539258389,
-60.598437521158));
#180803=CARTESIAN_POINT('Ctrl Pts',(41.9870302586278,-63.7207707080213,
-60.604818602443));
#180804=CARTESIAN_POINT('Ctrl Pts',(41.9879418325075,-63.6996927220351,
-60.6111530886119));
#180805=CARTESIAN_POINT('Ctrl Pts',(41.9889331213585,-63.6767721831338,
-60.6171173697952));
#180806=CARTESIAN_POINT('Ctrl Pts',(41.9898279798952,-63.6560813018846,
-60.622501459333));
#180807=CARTESIAN_POINT('Ctrl Pts',(41.9907878142519,-63.6338885522843,
-60.6275832961487));
#180808=CARTESIAN_POINT('Ctrl Pts',(41.991813049211,-63.6101837411181,-60.6320843346451));
#180809=CARTESIAN_POINT('Ctrl Pts',(41.9928051926042,-63.5872440514646,
-60.6364400928708));
#180810=CARTESIAN_POINT('Ctrl Pts',(41.9938586054156,-63.5628878131996,
-60.6402518750963));
#180811=CARTESIAN_POINT('Ctrl Pts',(41.9949723254169,-63.5371369349592,
-60.6432310343329));
#180812=CARTESIAN_POINT('Ctrl Pts',(41.9960348122651,-63.5125706441231,
-60.6460731468065));
#180813=CARTESIAN_POINT('Ctrl Pts',(41.9971522002356,-63.4867347319315,
-60.6481573437254));
#180814=CARTESIAN_POINT('Ctrl Pts',(41.9983221479124,-63.4596830378611,
-60.6492010672608));
#180815=CARTESIAN_POINT('Ctrl Pts',(41.9988700534207,-63.4470142899449,
-60.6496898599526));
#180816=CARTESIAN_POINT('Ctrl Pts',(41.999429462942,-63.4340794373293,-60.64995));
#180817=CARTESIAN_POINT('Ctrl Pts',(42.,-63.4208871539288,-60.64995));
#180818=CARTESIAN_POINT('Origin',(41.5,-73.08000002,-177.34995));
#180819=CARTESIAN_POINT('',(41.5,-64.9266169102438,-55.74995));
#180820=CARTESIAN_POINT('',(41.5,-64.9266169102438,-177.34995));
#180821=CARTESIAN_POINT('',(41.5,-73.08000002,-55.74995));
#180822=CARTESIAN_POINT('Origin',(41.,-73.08000002,-55.74995));
#180823=CARTESIAN_POINT('',(41.,-65.0141055737697,-55.24995));
#180824=CARTESIAN_POINT('Ctrl Pts',(41.5,-64.9266169102438,-55.74995));
#180825=CARTESIAN_POINT('Ctrl Pts',(41.5,-64.9266169102438,-55.7240510278259));
#180826=CARTESIAN_POINT('Ctrl Pts',(41.4979000486174,-64.9269843541242,
-55.697853607437));
#180827=CARTESIAN_POINT('Ctrl Pts',(41.49365840434,-64.9277265457027,-55.6716786004013));
#180828=CARTESIAN_POINT('Ctrl Pts',(41.4893809358961,-64.9284750056981,
-55.6452825239533));
#180829=CARTESIAN_POINT('Ctrl Pts',(41.4829253996728,-64.9296045781717,
-55.6189093033718));
#180830=CARTESIAN_POINT('Ctrl Pts',(41.474277574767,-64.9311177514586,-55.5929324719393));
#180831=CARTESIAN_POINT('Ctrl Pts',(41.4710188940119,-64.9316879467069,
-55.583143860168));
#180832=CARTESIAN_POINT('Ctrl Pts',(41.4674492132186,-64.9323125599105,
-55.573411976606));
#180833=CARTESIAN_POINT('Ctrl Pts',(41.463568827898,-64.9329915393618,-55.5637583894376));
#180834=CARTESIAN_POINT('Ctrl Pts',(41.453403314373,-64.9347702737462,-55.5384687177127));
#180835=CARTESIAN_POINT('Ctrl Pts',(41.4410985361824,-64.9369233309436,
-55.5136974848248));
#180836=CARTESIAN_POINT('Ctrl Pts',(41.4266549468271,-64.9394506316016,
-55.4898442374385));
#180837=CARTESIAN_POINT('Ctrl Pts',(41.414938405636,-64.9415007606612,-55.470494645819));
#180838=CARTESIAN_POINT('Ctrl Pts',(41.4018128556624,-64.9437974343114,
-55.4517483676005));
#180839=CARTESIAN_POINT('Ctrl Pts',(41.3872964035339,-64.9463374843029,
-55.4338552806394));
#180840=CARTESIAN_POINT('Ctrl Pts',(41.3794565918151,-64.9477092736019,
-55.4241918703515));
#180841=CARTESIAN_POINT('Ctrl Pts',(41.3712113471472,-64.9491520044747,
-55.4147778016595));
#180842=CARTESIAN_POINT('Ctrl Pts',(41.3625680866767,-64.9506643790888,
-55.4056571306895));
#180843=CARTESIAN_POINT('Ctrl Pts',(41.3608465431265,-64.9509656101776,
-55.4038404976798));
#180844=CARTESIAN_POINT('Ctrl Pts',(41.3587490914835,-64.9513326166609,
-55.4016626948178));
#180845=CARTESIAN_POINT('Ctrl Pts',(41.3569013241922,-64.9516559287514,
-55.3997779182198));
#180846=CARTESIAN_POINT('Ctrl Pts',(41.3555737423086,-64.9518882216793,
-55.3984237459289));
#180847=CARTESIAN_POINT('Ctrl Pts',(41.3543763923405,-64.9520977242419,
-55.3972196111486));
#180848=CARTESIAN_POINT('Ctrl Pts',(41.3535533894273,-64.9522417198603,
-55.3963966082408));
#180849=CARTESIAN_POINT('Ctrl Pts',(41.3437873007902,-64.9539504306672,
-55.3866305196681));
#180850=CARTESIAN_POINT('Ctrl Pts',(41.3328864379011,-64.9558577859898,
-55.3765717208569));
#180851=CARTESIAN_POINT('Ctrl Pts',(41.3207228245913,-64.9579861393597,
-55.3664552895103));
#180852=CARTESIAN_POINT('Ctrl Pts',(41.3090750456328,-64.9600242335483,
-55.3567678756495));
#180853=CARTESIAN_POINT('Ctrl Pts',(41.2962686321262,-64.9622651041163,
-55.3470275906937));
#180854=CARTESIAN_POINT('Ctrl Pts',(41.2822138036231,-64.9647244255877,
-55.3374815440083));
#180855=CARTESIAN_POINT('Ctrl Pts',(41.2689601031572,-64.9670435652432,
-55.3284796238943));
#180856=CARTESIAN_POINT('Ctrl Pts',(41.2545958039182,-64.969557040367,-55.3196505221386));
#180857=CARTESIAN_POINT('Ctrl Pts',(41.2390741346523,-64.9722730049582,
-55.3112377697523));
#180858=CARTESIAN_POINT('Ctrl Pts',(41.2328103975183,-64.9733690267825,
-55.3078428211408));
#180859=CARTESIAN_POINT('Ctrl Pts',(41.2263585547675,-64.9744979589017,
-55.3045160977493));
#180860=CARTESIAN_POINT('Ctrl Pts',(41.2197172105282,-64.9756600435648,
-55.3012753797728));
#180861=CARTESIAN_POINT('Ctrl Pts',(41.204469095489,-64.978328117977,-55.293834892014));
#180862=CARTESIAN_POINT('Ctrl Pts',(41.1882095131135,-64.9811731762401,
-55.2868407235431));
#180863=CARTESIAN_POINT('Ctrl Pts',(41.1709460856378,-64.9841938846355,
-55.2805340045024));
#180864=CARTESIAN_POINT('Ctrl Pts',(41.1541655073744,-64.9871301053663,
-55.2744036811586));
#180865=CARTESIAN_POINT('Ctrl Pts',(41.1364361385031,-64.9902323429417,
-55.2689228588952));
#180866=CARTESIAN_POINT('Ctrl Pts',(41.1178013239113,-64.9934930129889,
-55.26434275797));
#180867=CARTESIAN_POINT('Ctrl Pts',(41.0997555826134,-64.9966506085658,
-55.2599074406232));
#180868=CARTESIAN_POINT('Ctrl Pts',(41.0808605102839,-64.9999568178164,
-55.2563167977781));
#180869=CARTESIAN_POINT('Ctrl Pts',(41.0611938833982,-65.0033980316209,
-55.253827476193));
#180870=CARTESIAN_POINT('Ctrl Pts',(41.0415272565126,-65.0068392454254,
-55.2513381546079));
#180871=CARTESIAN_POINT('Ctrl Pts',(41.0210886481305,-65.0104155384887,
-55.24995));
#180872=CARTESIAN_POINT('Ctrl Pts',(41.,-65.0141055737697,-55.24995));
#180873=CARTESIAN_POINT('',(41.,-73.08000002,-55.24995));
#180874=CARTESIAN_POINT('Origin',(41.5,-73.08000002,-55.24995));
#180875=CARTESIAN_POINT('',(40.5,-65.0578499055327,-55.24995));
#180876=CARTESIAN_POINT('',(40.7958880023324,-65.0319630596553,-55.24995));
#180877=CARTESIAN_POINT('',(40.5,-73.08000002,-55.24995));
#180878=CARTESIAN_POINT('Origin',(40.5,-73.08000002,-55.74995));
#180879=CARTESIAN_POINT('',(40.,-65.1453385690586,-55.74995));
#180880=CARTESIAN_POINT('Ctrl Pts',(40.5,-65.0578499055327,-55.24995));
#180881=CARTESIAN_POINT('Ctrl Pts',(40.478414950197,-65.0616267998515,-55.24995));
#180882=CARTESIAN_POINT('Ctrl Pts',(40.4574879525933,-65.0652537898141,
-55.2513479743296));
#180883=CARTESIAN_POINT('Ctrl Pts',(40.4373682802013,-65.0687308754204,
-55.2538882420756));
#180884=CARTESIAN_POINT('Ctrl Pts',(40.4172805341775,-65.0722024435058,
-55.2564244788652));
#180885=CARTESIAN_POINT('Ctrl Pts',(40.3979969754806,-65.0755245826009,
-55.2600986723959));
#180886=CARTESIAN_POINT('Ctrl Pts',(40.3796086600543,-65.0786972927059,
-55.2646604727422));
#180887=CARTESIAN_POINT('Ctrl Pts',(40.3604151050382,-65.0820089384189,
-55.2694220381108));
#180888=CARTESIAN_POINT('Ctrl Pts',(40.3421966020862,-65.0851577813522,
-55.2751499570335));
#180889=CARTESIAN_POINT('Ctrl Pts',(40.3250003325847,-65.0881438215058,
-55.2815750258559));
#180890=CARTESIAN_POINT('Ctrl Pts',(40.309168402891,-65.0908929513546,-55.2874903342815));
#180891=CARTESIAN_POINT('Ctrl Pts',(40.2942018644216,-65.0935040869392,
-55.2939965089016));
#180892=CARTESIAN_POINT('Ctrl Pts',(40.2801026176646,-65.0959772282596,
-55.3009008476324));
#180893=CARTESIAN_POINT('Ctrl Pts',(40.2636746295662,-65.0988588528511,
-55.3089455606908));
#180894=CARTESIAN_POINT('Ctrl Pts',(40.2484243091612,-65.1015531342264,
-55.3175297931905));
#180895=CARTESIAN_POINT('Ctrl Pts',(40.2343108458121,-65.1040600723857,
-55.3263826814461));
#180896=CARTESIAN_POINT('Ctrl Pts',(40.2231748699736,-65.106038127104,-55.3333678945917));
#180897=CARTESIAN_POINT('Ctrl Pts',(40.2127455890291,-65.1078995472417,
-55.3405210924605));
#180898=CARTESIAN_POINT('Ctrl Pts',(40.2029879734393,-65.1096443327989,
-55.3477263606172));
#180899=CARTESIAN_POINT('Ctrl Pts',(40.1919258839995,-65.111622374843,-55.3558948849923));
#180900=CARTESIAN_POINT('Ctrl Pts',(40.1817269309934,-65.1134505125309,
-55.3641299065234));
#180901=CARTESIAN_POINT('Ctrl Pts',(40.172326481779,-65.1151287458626,-55.3722860416234));
#180902=CARTESIAN_POINT('Ctrl Pts',(40.1676262571718,-65.1159678625284,
-55.3763641091735));
#180903=CARTESIAN_POINT('Ctrl Pts',(40.1631254733296,-65.1167695031052,
-55.3804228422476));
#180904=CARTESIAN_POINT('Ctrl Pts',(40.1588151925472,-65.1175336675929,
-55.3844463376882));
#180905=CARTESIAN_POINT('Ctrl Pts',(40.156660052156,-65.1179157498367,-55.3864580854084));
#180906=CARTESIAN_POINT('Ctrl Pts',(40.1545525458342,-65.1182884630583,
-55.3884610324758));
#180907=CARTESIAN_POINT('Ctrl Pts',(40.1524915002252,-65.1186518072577,
-55.390453348299));
#180908=CARTESIAN_POINT('Ctrl Pts',(40.1512120949914,-65.1188773551389,
-55.3916900891456));
#180909=CARTESIAN_POINT('Ctrl Pts',(40.1503718507489,-65.1190263697845,
-55.3925105847799));
#180910=CARTESIAN_POINT('Ctrl Pts',(40.1491841723718,-65.1192346532407,
-55.3936800811385));
#180911=CARTESIAN_POINT('Ctrl Pts',(40.1484585716412,-65.1193619020236,
-55.3943945737391));
#180912=CARTESIAN_POINT('Ctrl Pts',(40.1476035777893,-65.1195112727835,
-55.3952396410241));
#180913=CARTESIAN_POINT('Ctrl Pts',(40.1464466094067,-65.1197137327888,
-55.3963966094067));
#180914=CARTESIAN_POINT('Ctrl Pts',(40.1284887645886,-65.1228562087736,
-55.4143544542249));
#180915=CARTESIAN_POINT('Ctrl Pts',(40.1120748438341,-65.1257096539755,
-55.4335093827818));
#180916=CARTESIAN_POINT('Ctrl Pts',(40.0973083463449,-65.1282740683946,
-55.4535728212623));
#180917=CARTESIAN_POINT('Ctrl Pts',(40.0823330903159,-65.1308747367331,
-55.4739199027748));
#180918=CARTESIAN_POINT('Ctrl Pts',(40.0690520283695,-65.1331781442871,
-55.4952007603808));
#180919=CARTESIAN_POINT('Ctrl Pts',(40.0575195953378,-65.1351842910565,
-55.5171172456677));
#180920=CARTESIAN_POINT('Ctrl Pts',(40.045734109412,-65.1372344581332,-55.5395146381502));
#180921=CARTESIAN_POINT('Ctrl Pts',(40.0357746506934,-65.138974175882,-55.562575264068));
#180922=CARTESIAN_POINT('Ctrl Pts',(40.0276461796452,-65.1404034443027,
-55.5859930898185));
#180923=CARTESIAN_POINT('Ctrl Pts',(40.0194149426489,-65.1418507825577,
-55.6097069804814));
#180924=CARTESIAN_POINT('Ctrl Pts',(40.0130609212421,-65.1429797720179,
-55.6337866416156));
#180925=CARTESIAN_POINT('Ctrl Pts',(40.0085396584692,-65.1437904126833,
-55.657935149555));
#180926=CARTESIAN_POINT('Ctrl Pts',(40.0039333231242,-65.1446163064516,
-55.6825380384463));
#180927=CARTESIAN_POINT('Ctrl Pts',(40.0012289600629,-65.1451117585439,
-55.7072119145227));
#180928=CARTESIAN_POINT('Ctrl Pts',(40.0003341985789,-65.1452767689602,
-55.7316719560618));
#180929=CARTESIAN_POINT('Ctrl Pts',(40.0001107930952,-65.1453179690258,
-55.7377791785));
#180930=CARTESIAN_POINT('Ctrl Pts',(40.,-65.1453385690586,-55.7438732289798));
#180931=CARTESIAN_POINT('Ctrl Pts',(40.,-65.1453385690586,-55.74995));
#180932=CARTESIAN_POINT('',(40.,67.7009572055632,-55.74995));
#180933=CARTESIAN_POINT('Origin',(40.,67.7009572055632,-55.24995));
#180934=CARTESIAN_POINT('',(40.,-65.1453385690586,-59.64995));
#180935=CARTESIAN_POINT('',(40.,-65.1453385690586,-55.24995));
#180936=CARTESIAN_POINT('Ctrl Pts',(40.,-65.1453385690586,-59.64995));
#180937=CARTESIAN_POINT('Ctrl Pts',(40.,-65.1453385690423,-59.8463349320561));
#180938=CARTESIAN_POINT('Ctrl Pts',(40.,-65.1061484482599,-60.0425718399612));
#180939=CARTESIAN_POINT('Ctrl Pts',(40.,-64.9552949839326,-60.4053784571341));
#180940=CARTESIAN_POINT('Ctrl Pts',(40.,-64.8436909621967,-60.5717700902076));
#180941=CARTESIAN_POINT('Ctrl Pts',(40.,-64.5649501059399,-60.8494502533521));
#180942=CARTESIAN_POINT('Ctrl Pts',(40.,-64.3979228839314,-60.9606295880612));
#180943=CARTESIAN_POINT('Ctrl Pts',(40.,-64.0337304042775,-61.1109090094727));
#180944=CARTESIAN_POINT('Ctrl Pts',(40.,-63.8367439033901,-61.149949999985));
#180945=CARTESIAN_POINT('Ctrl Pts',(40.,-63.6396088127436,-61.14995));
#180946=CARTESIAN_POINT('Ctrl Pts',(33.35,-64.133919761665,-61.14995));
#180947=CARTESIAN_POINT('Ctrl Pts',(33.35,-64.1339197616649,-60.64995));
#180948=CARTESIAN_POINT('Ctrl Pts',(33.85,-64.133919761665,-60.64995));
#180949=CARTESIAN_POINT('Ctrl Pts',(33.35,-64.3310548523114,-61.149949999985));
#180950=CARTESIAN_POINT('Ctrl Pts',(33.35,-64.265066231498,-60.6556217969808));
#180951=CARTESIAN_POINT('Ctrl Pts',(33.8442946417933,-64.2658423095942,
-60.64995));
#180952=CARTESIAN_POINT('Ctrl Pts',(33.35,-64.5280413531989,-61.1109090094727));
#180953=CARTESIAN_POINT('Ctrl Pts',(33.3499999999993,-64.399347719172,-60.6353187454038));
#180954=CARTESIAN_POINT('Ctrl Pts',(33.8385935839748,-64.3976654214474,
-60.6239226729819));
#180955=CARTESIAN_POINT('Ctrl Pts',(33.35,-64.8922338328527,-60.9606295880612));
#180956=CARTESIAN_POINT('Ctrl Pts',(33.3500000000007,-64.6507229380173,
-60.5426326522465));
#180957=CARTESIAN_POINT('Ctrl Pts',(33.8280533572402,-64.6413825582346,
-60.5237363920407));
#180958=CARTESIAN_POINT('Ctrl Pts',(33.35,-65.0592610548614,-60.849450253352));
#180959=CARTESIAN_POINT('Ctrl Pts',(33.35,-64.7680300213717,-60.4706504746468));
#180960=CARTESIAN_POINT('Ctrl Pts',(33.8232193617858,-64.7531569593752,
-60.4496168355678));
#180961=CARTESIAN_POINT('Ctrl Pts',(33.35,-65.338001911118,-60.5717700902076));
#180962=CARTESIAN_POINT('Ctrl Pts',(33.35,-64.9649606354368,-60.2852157712117));
#180963=CARTESIAN_POINT('Ctrl Pts',(33.8151522214979,-64.9396899802014,
-60.2644967268053));
#180964=CARTESIAN_POINT('Ctrl Pts',(33.35,-65.4496059328539,-60.4053784571335));
#180965=CARTESIAN_POINT('Ctrl Pts',(33.35,-65.0449787669832,-60.1718710142623));
#180966=CARTESIAN_POINT('Ctrl Pts',(33.8119222489988,-65.0143752473362,
-60.1535689714224));
#180967=CARTESIAN_POINT('Ctrl Pts',(33.35,-65.6004593971813,-60.0425718399618));
#180968=CARTESIAN_POINT('Ctrl Pts',(33.35,-65.1530905830856,-59.9224177216081));
#180969=CARTESIAN_POINT('Ctrl Pts',(33.8075563441358,-65.1153261907357,
-59.9116978933078));
#180970=CARTESIAN_POINT('Ctrl Pts',(33.35,-65.6396495179636,-59.8463349320557));
#180971=CARTESIAN_POINT('Ctrl Pts',(33.35,-65.1814839309564,-59.7861314644984));
#180972=CARTESIAN_POINT('Ctrl Pts',(33.8064221286289,-65.1415521689339,
-59.7808732880372));
#180973=CARTESIAN_POINT('Ctrl Pts',(33.35,-65.63964951798,-59.64995));
#180974=CARTESIAN_POINT('Ctrl Pts',(33.3499999999999,-65.1814839309712,
-59.64995));
#180975=CARTESIAN_POINT('Ctrl Pts',(33.8064221286261,-65.1415521689341,
-59.64995));
#180976=CARTESIAN_POINT('',(33.8064221286261,-65.1415521689341,-59.64995));
#180977=CARTESIAN_POINT('Ctrl Pts',(33.8064221286261,-65.1415521689341,
-59.64995));
#180978=CARTESIAN_POINT('Ctrl Pts',(33.8064221286261,-65.1415521689341,
-59.6947437540757));
#180979=CARTESIAN_POINT('Ctrl Pts',(33.8065549254468,-65.1384815650739,
-59.740006513579));
#180980=CARTESIAN_POINT('Ctrl Pts',(33.8068254007034,-65.1322274818581,
-59.7853172189021));
#180981=CARTESIAN_POINT('Ctrl Pts',(33.8070925832971,-65.1260495334742,
-59.8300763289218));
#180982=CARTESIAN_POINT('Ctrl Pts',(33.8074941133853,-65.1167651256616,
-59.8748822590296));
#180983=CARTESIAN_POINT('Ctrl Pts',(33.8080343638775,-65.1042731455181,
-59.9192791424491));
#180984=CARTESIAN_POINT('Ctrl Pts',(33.8084577829567,-65.0944826079675,
-59.9540750154215));
#180985=CARTESIAN_POINT('Ctrl Pts',(33.8089664057838,-65.0827219407404,
-59.9886186682484));
#180986=CARTESIAN_POINT('Ctrl Pts',(33.8095621871869,-65.0689459431877,
-60.0226684878905));
#180987=CARTESIAN_POINT('Ctrl Pts',(33.8096203911749,-65.0676001173659,
-60.0259949349465));
#180988=CARTESIAN_POINT('Ctrl Pts',(33.8096794270447,-65.0662350562995,
-60.0293166615144));
#180989=CARTESIAN_POINT('Ctrl Pts',(33.8097392965673,-65.0648507190359,
-60.0326334323651));
#180990=CARTESIAN_POINT('Ctrl Pts',(33.8105100399482,-65.0470291508023,
-60.0753326066097));
#180991=CARTESIAN_POINT('Ctrl Pts',(33.8114188289058,-65.0260156139738,
-60.1171993189902));
#180992=CARTESIAN_POINT('Ctrl Pts',(33.8124618902136,-65.0018973552474,
-60.1577697848382));
#180993=CARTESIAN_POINT('Ctrl Pts',(33.8134583716327,-64.9788561432871,
-60.1965284992851));
#180994=CARTESIAN_POINT('Ctrl Pts',(33.8145773576715,-64.9529823096089,
-60.2341031978335));
#180995=CARTESIAN_POINT('Ctrl Pts',(33.8158147922089,-64.9243696421593,
-60.2700569684901));
#180996=CARTESIAN_POINT('Ctrl Pts',(33.8163964129388,-64.9109210757727,
-60.2869560105797));
#180997=CARTESIAN_POINT('Ctrl Pts',(33.8170041918055,-64.8968676660202,
-60.3034964084361));
#180998=CARTESIAN_POINT('Ctrl Pts',(33.8176376070201,-64.8822214780019,
-60.319628807785));
#180999=CARTESIAN_POINT('Ctrl Pts',(33.8178621341635,-64.8770298332783,
-60.3253472709001));
#181000=CARTESIAN_POINT('Ctrl Pts',(33.8181018562225,-64.8714868430797,
-60.3313130458379));
#181001=CARTESIAN_POINT('Ctrl Pts',(33.8183408944099,-64.8659595559936,
-60.3371156972342));
#181002=CARTESIAN_POINT('Ctrl Pts',(33.8185870781049,-64.8602670431233,
-60.34309180581));
#181003=CARTESIAN_POINT('Ctrl Pts',(33.8188325293759,-64.8545913493511,
-60.3488947477477));
#181004=CARTESIAN_POINT('Ctrl Pts',(33.8190581152215,-64.8493747585253,
-60.3541155165011));
#181005=CARTESIAN_POINT('Ctrl Pts',(33.8191014412564,-64.8483728596886,
-60.3551182177509));
#181006=CARTESIAN_POINT('Ctrl Pts',(33.8191440297855,-64.8473880051467,
-60.3560995559683));
#181007=CARTESIAN_POINT('Ctrl Pts',(33.8191857390412,-64.8464234720805,
-60.3570567834875));
#181008=CARTESIAN_POINT('Ctrl Pts',(33.8201337860552,-64.8244997364875,
-60.3788144647644));
#181009=CARTESIAN_POINT('Ctrl Pts',(33.8211541356638,-64.8009069536454,
-60.400195230713));
#181010=CARTESIAN_POINT('Ctrl Pts',(33.8222490528173,-64.775590584552,-60.4209274439786));
#181011=CARTESIAN_POINT('Ctrl Pts',(33.8233241882501,-64.7507316028861,
-60.4412850911419));
#181012=CARTESIAN_POINT('Ctrl Pts',(33.8244712328871,-64.7242104814626,
-60.4610175332332));
#181013=CARTESIAN_POINT('Ctrl Pts',(33.8256909440562,-64.6960076238503,
-60.479830648753));
#181014=CARTESIAN_POINT('Ctrl Pts',(33.8268514204858,-64.6691744256828,
-60.4977301135459));
#181015=CARTESIAN_POINT('Ctrl Pts',(33.828077793884,-64.640817520206,-60.5147982857993));
#181016=CARTESIAN_POINT('Ctrl Pts',(33.8293695759994,-64.6109481970491,
-60.5307488755859));
#181017=CARTESIAN_POINT('Ctrl Pts',(33.8306262844959,-64.5818898661206,
-60.5462663854435));
#181018=CARTESIAN_POINT('Ctrl Pts',(33.8319449269011,-64.5513994640134,
-60.5607262880999));
#181019=CARTESIAN_POINT('Ctrl Pts',(33.8333234706075,-64.519523989841,-60.5738295325113));
#181020=CARTESIAN_POINT('Ctrl Pts',(33.8333461253679,-64.5190001535445,
-60.5740448690734));
#181021=CARTESIAN_POINT('Ctrl Pts',(33.8333687961948,-64.5184759457487,
-60.5742598379439));
#181022=CARTESIAN_POINT('Ctrl Pts',(33.8333914830767,-64.5179513667201,
-60.574474438062));
#181023=CARTESIAN_POINT('Ctrl Pts',(33.8335053586103,-64.5153182716555,
-60.5755516113404));
#181024=CARTESIAN_POINT('Ctrl Pts',(33.833650217034,-64.5119684284898,-60.5769043222679));
#181025=CARTESIAN_POINT('Ctrl Pts',(33.833770571488,-64.5091851149092,-60.5780123790167));
#181026=CARTESIAN_POINT('Ctrl Pts',(33.8338490691023,-64.5073697813782,
-60.578735076087));
#181027=CARTESIAN_POINT('Ctrl Pts',(33.833917118837,-64.505796001968,-60.5793550577169));
#181028=CARTESIAN_POINT('Ctrl Pts',(33.8339591709511,-64.504823404206,-60.5797369926547));
#181029=CARTESIAN_POINT('Ctrl Pts',(33.8346317135054,-64.4892685766439,
-60.5858453062145));
#181030=CARTESIAN_POINT('Ctrl Pts',(33.8353765198879,-64.4720444193626,
-60.5921640967238));
#181031=CARTESIAN_POINT('Ctrl Pts',(33.8361963547969,-64.4530865326853,
-60.5984375214524));
#181032=CARTESIAN_POINT('Ctrl Pts',(33.837030258674,-64.4338033147713,-60.6048186027495));
#181033=CARTESIAN_POINT('Ctrl Pts',(33.8379418325563,-64.4127253287281,
-60.6111530889097));
#181034=CARTESIAN_POINT('Ctrl Pts',(33.8389331214077,-64.389804789812,-60.6171173700705));
#181035=CARTESIAN_POINT('Ctrl Pts',(33.8398279799534,-64.3691139083493,
-60.6225014596402));
#181036=CARTESIAN_POINT('Ctrl Pts',(33.8407878143187,-64.3469211585411,
-60.6275832964709));
#181037=CARTESIAN_POINT('Ctrl Pts',(33.8418130492861,-64.3232163471738,
-60.6320843349643));
#181038=CARTESIAN_POINT('Ctrl Pts',(33.8428051926872,-64.3002766573262,
-60.636440093187));
#181039=CARTESIAN_POINT('Ctrl Pts',(33.8438586055063,-64.2759204188738,
-60.6402518753928));
#181040=CARTESIAN_POINT('Ctrl Pts',(33.8449723255149,-64.2501695404544,
-60.6432310345922));
#181041=CARTESIAN_POINT('Ctrl Pts',(33.8460348123706,-64.2256032494346,
-60.6460731470319));
#181042=CARTESIAN_POINT('Ctrl Pts',(33.8471522003485,-64.1997673370657,
-60.6481573439003));
#181043=CARTESIAN_POINT('Ctrl Pts',(33.8483221480323,-64.1727156428264,
-60.6492010673677));
#181044=CARTESIAN_POINT('Ctrl Pts',(33.8488700535025,-64.1600468957922,
-60.6496898599907));
#181045=CARTESIAN_POINT('Ctrl Pts',(33.8494294629838,-64.1471120441008,
-60.64995));
#181046=CARTESIAN_POINT('Ctrl Pts',(33.85,-64.133919761665,-60.64995));
#181047=CARTESIAN_POINT('Origin',(33.85,-65.63964951798,-59.64995));
#181048=CARTESIAN_POINT('Ctrl Pts',(40.,-65.1453385690586,-59.64995));
#181049=CARTESIAN_POINT('Ctrl Pts',(39.9999999999999,-64.599684318524,-59.64995));
#181050=CARTESIAN_POINT('Ctrl Pts',(39.4564221286262,-64.6472412200127,
-59.64995));
#181051=CARTESIAN_POINT('Ctrl Pts',(40.,-65.1453385690423,-59.8463349320561));
#181052=CARTESIAN_POINT('Ctrl Pts',(39.9999999999999,-64.5996843185171,
-59.7746029379318));
#181053=CARTESIAN_POINT('Ctrl Pts',(39.4564221286269,-64.6472412200127,
-59.7808732880376));
#181054=CARTESIAN_POINT('Ctrl Pts',(40.,-65.1061484482599,-60.0425718399612));
#181055=CARTESIAN_POINT('Ctrl Pts',(40.,-64.5762635801886,-59.898971233264));
#181056=CARTESIAN_POINT('Ctrl Pts',(39.4575563441365,-64.6210152418146,
-59.9116978933072));
#181057=CARTESIAN_POINT('Ctrl Pts',(40.,-64.9552949839326,-60.4053784571341));
#181058=CARTESIAN_POINT('Ctrl Pts',(39.9999999999999,-64.4844350369598,
-60.1322291512609));
#181059=CARTESIAN_POINT('Ctrl Pts',(39.4619222489981,-64.5200642984147,
-60.153568971423));
#181060=CARTESIAN_POINT('Ctrl Pts',(40.,-64.8436909621967,-60.5717700902076));
#181061=CARTESIAN_POINT('Ctrl Pts',(39.9999999999999,-64.4163683849594,
-60.2406767152616));
#181062=CARTESIAN_POINT('Ctrl Pts',(39.4651522214972,-64.4453790312801,
-60.2644967268053));
#181063=CARTESIAN_POINT('Ctrl Pts',(40.,-64.5649501059399,-60.8494502533521));
#181064=CARTESIAN_POINT('Ctrl Pts',(39.9999999999999,-64.2423415370877,
-60.4261994932778));
#181065=CARTESIAN_POINT('Ctrl Pts',(39.4732193617865,-64.2588460104538,
-60.4496168355678));
#181066=CARTESIAN_POINT('Ctrl Pts',(40.,-64.3979228839314,-60.9606295880612));
#181067=CARTESIAN_POINT('Ctrl Pts',(39.9999999999993,-64.1369109528056,
-60.5031527166045));
#181068=CARTESIAN_POINT('Ctrl Pts',(39.4780533572402,-64.1470716093135,
-60.5237363920406));
#181069=CARTESIAN_POINT('Ctrl Pts',(40.,-64.0337304042775,-61.1109090094727));
#181070=CARTESIAN_POINT('Ctrl Pts',(40.0000000000006,-63.9016439800941,
-60.6120353079401));
#181071=CARTESIAN_POINT('Ctrl Pts',(39.4885935839748,-63.9033544725257,
-60.623922672982));
#181072=CARTESIAN_POINT('Ctrl Pts',(40.,-63.8367439033901,-61.149949999985));
#181073=CARTESIAN_POINT('Ctrl Pts',(39.9999999999999,-63.7723272342478,
-60.6442102195365));
#181074=CARTESIAN_POINT('Ctrl Pts',(39.4942946417933,-63.771531360673,-60.64995));
#181075=CARTESIAN_POINT('Ctrl Pts',(40.,-63.6396088127436,-61.14995));
#181076=CARTESIAN_POINT('Ctrl Pts',(39.9999999999999,-63.6396088127435,
-60.64995));
#181077=CARTESIAN_POINT('Ctrl Pts',(39.5,-63.6396088127436,-60.64995));
#181078=CARTESIAN_POINT('',(39.4564221286262,-64.6472412200127,-59.64995));
#181079=CARTESIAN_POINT('Origin',(39.5,-65.1453385690586,-59.64995));
#181080=CARTESIAN_POINT('Ctrl Pts',(39.5,-63.6396088127436,-60.64995));
#181081=CARTESIAN_POINT('Ctrl Pts',(39.4987470950733,-63.668579195362,-60.64995));
#181082=CARTESIAN_POINT('Ctrl Pts',(39.4975587391908,-63.6963077447446,
-60.648711804108));
#181083=CARTESIAN_POINT('Ctrl Pts',(39.4964278563854,-63.7227135822176,
-60.6465429519245));
#181084=CARTESIAN_POINT('Ctrl Pts',(39.4952494858174,-63.7502282473553,
-60.6442830258145));
#181085=CARTESIAN_POINT('Ctrl Pts',(39.494133558101,-63.7763072581729,-60.6410132280021));
#181086=CARTESIAN_POINT('Ctrl Pts',(39.4930764842437,-63.8009095922985,
-60.6370534670711));
#181087=CARTESIAN_POINT('Ctrl Pts',(39.4921996476724,-63.8213170843124,
-60.6337688685788));
#181088=CARTESIAN_POINT('Ctrl Pts',(39.4913634057138,-63.8407096717578,
-60.6300090684675));
#181089=CARTESIAN_POINT('Ctrl Pts',(39.4905675226138,-63.8590846599517,
-60.6259392754887));
#181090=CARTESIAN_POINT('Ctrl Pts',(39.4895582118083,-63.8823871702473,
-60.6207781079392));
#181091=CARTESIAN_POINT('Ctrl Pts',(39.4886137704671,-63.9040527084652,
-60.6151198747808));
#181092=CARTESIAN_POINT('Ctrl Pts',(39.4877364626516,-63.9241071529484,
-60.6092623723909));
#181093=CARTESIAN_POINT('Ctrl Pts',(39.4874506843826,-63.930639779615,-60.6073543227143));
#181094=CARTESIAN_POINT('Ctrl Pts',(39.4871720492897,-63.9370016786934,
-60.6054247761517));
#181095=CARTESIAN_POINT('Ctrl Pts',(39.486900685889,-63.9431943191312,-60.6034830013555));
#181096=CARTESIAN_POINT('Ctrl Pts',(39.4863484763101,-63.9557960014505,
-60.5995315965609));
#181097=CARTESIAN_POINT('Ctrl Pts',(39.4858263638654,-63.9676966127036,
-60.5955300979674));
#181098=CARTESIAN_POINT('Ctrl Pts',(39.4853356541076,-63.9789110754265,
-60.5915501616224));
#181099=CARTESIAN_POINT('Ctrl Pts',(39.4850902992287,-63.984518306788,-60.5895601934499));
#181100=CARTESIAN_POINT('Ctrl Pts',(39.4848527917264,-63.9899539633539,
-60.5875755120804));
#181101=CARTESIAN_POINT('Ctrl Pts',(39.4846233227342,-63.9952202297894,
-60.5856042391654));
#181102=CARTESIAN_POINT('Ctrl Pts',(39.4845085882381,-63.9978533630071,
-60.5846186027079));
#181103=CARTESIAN_POINT('Ctrl Pts',(39.4843958631624,-64.0004441463261,
-60.5836363114965));
#181104=CARTESIAN_POINT('Ctrl Pts',(39.484285170947,-64.0029928476625,-60.5826583364528));
#181105=CARTESIAN_POINT('Ctrl Pts',(39.4842092440968,-64.0047410723553,
-60.581987516339));
#181106=CARTESIAN_POINT('Ctrl Pts',(39.484173495994,-64.0055575949344,-60.5816721107052));
#181107=CARTESIAN_POINT('Ctrl Pts',(39.484097273974,-64.0073195795363,-60.5809867219877));
#181108=CARTESIAN_POINT('Ctrl Pts',(39.4840623734564,-64.0081263565634,
-60.5806728963894));
#181109=CARTESIAN_POINT('Ctrl Pts',(39.4840189765475,-64.0091312289906,
-60.5802811765833));
#181110=CARTESIAN_POINT('Ctrl Pts',(39.4839592160933,-64.0105129710424,
-60.5797383010624));
#181111=CARTESIAN_POINT('Ctrl Pts',(39.4825183894221,-64.0438268209682,
-60.5666495529811));
#181112=CARTESIAN_POINT('Ctrl Pts',(39.4811478367641,-64.0756915213578,
-60.5520895210254));
#181113=CARTESIAN_POINT('Ctrl Pts',(39.4798415410344,-64.1060382966163,
-60.5363617341694));
#181114=CARTESIAN_POINT('Ctrl Pts',(39.4785010284258,-64.1371799699317,
-60.5202219764498));
#181115=CARTESIAN_POINT('Ctrl Pts',(39.4772282106895,-64.1667234714416,
-60.5028529742347));
#181116=CARTESIAN_POINT('Ctrl Pts',(39.4760210452544,-64.1946454544485,
-60.4845643909836));
#181117=CARTESIAN_POINT('Ctrl Pts',(39.4759189711445,-64.1970064494526,
-60.4830179659437));
#181118=CARTESIAN_POINT('Ctrl Pts',(39.4758173688579,-64.1993558784669,
-60.4814649529687));
#181119=CARTESIAN_POINT('Ctrl Pts',(39.4757162384692,-64.2016937423444,
-60.4799055318267));
#181120=CARTESIAN_POINT('Ctrl Pts',(39.4744780032632,-64.2303184257544,
-60.4608120606792));
#181121=CARTESIAN_POINT('Ctrl Pts',(39.4733101859453,-64.2572056002202,
-60.440760379908));
#181122=CARTESIAN_POINT('Ctrl Pts',(39.4722151146508,-64.2823818764487,
-60.4200646444817));
#181123=CARTESIAN_POINT('Ctrl Pts',(39.4716767714853,-64.2947586744769,
-60.4098905053401));
#181124=CARTESIAN_POINT('Ctrl Pts',(39.4711560693644,-64.3067226760081,
-60.3995602559987));
#181125=CARTESIAN_POINT('Ctrl Pts',(39.4706536010265,-64.3182806560766,
-60.3891084432166));
#181126=CARTESIAN_POINT('Ctrl Pts',(39.4704165881026,-64.3237325232786,
-60.3841783520614));
#181127=CARTESIAN_POINT('Ctrl Pts',(39.4701961142932,-64.3287724121334,
-60.3795181564655));
#181128=CARTESIAN_POINT('Ctrl Pts',(39.4699752712379,-64.3338567059913,
-60.3747215662175));
#181129=CARTESIAN_POINT('Ctrl Pts',(39.4697604813308,-64.3388016430389,
-60.3700564470324));
#181130=CARTESIAN_POINT('Ctrl Pts',(39.4695453554172,-64.3437887359688,
-60.3652622206266));
#181131=CARTESIAN_POINT('Ctrl Pts',(39.4693114502845,-64.3492048564472,
-60.3599307008521));
#181132=CARTESIAN_POINT('Ctrl Pts',(39.4692701938298,-64.350160157969,-60.3589903212992));
#181133=CARTESIAN_POINT('Ctrl Pts',(39.4692283450499,-64.3511287141094,
-60.3580331354884));
#181134=CARTESIAN_POINT('Ctrl Pts',(39.4691857916419,-64.3521125208669,
-60.3570567811865));
#181135=CARTESIAN_POINT('Ctrl Pts',(39.4678695545057,-64.3825430563033,
-60.3268567607499));
#181136=CARTESIAN_POINT('Ctrl Pts',(39.466668527626,-64.4107735993503,-60.2949641542072));
#181137=CARTESIAN_POINT('Ctrl Pts',(39.465571557121,-64.436676660555,-60.2617220238234));
#181138=CARTESIAN_POINT('Ctrl Pts',(39.464461564869,-64.4628872077912,-60.2280852879266));
#181139=CARTESIAN_POINT('Ctrl Pts',(39.4634581230739,-64.4867147905155,
-60.1930673112892));
#181140=CARTESIAN_POINT('Ctrl Pts',(39.4625543591717,-64.5080808549628,
-60.157022098603));
#181141=CARTESIAN_POINT('Ctrl Pts',(39.4616396515968,-64.5297056409793,
-60.1205404146136));
#181142=CARTESIAN_POINT('Ctrl Pts',(39.4608270659075,-64.5488091105469,
-60.0830069556029));
#181143=CARTESIAN_POINT('Ctrl Pts',(39.4601140607574,-64.5653622159461,
-60.0447796551349));
#181144=CARTESIAN_POINT('Ctrl Pts',(39.4593877893017,-64.582223311484,-60.0058410904482));
#181145=CARTESIAN_POINT('Ctrl Pts',(39.4587648558077,-64.5964384528258,
-59.9661831067956));
#181146=CARTESIAN_POINT('Ctrl Pts',(39.4582470591423,-64.6080282011136,
-59.9261671559726));
#181147=CARTESIAN_POINT('Ctrl Pts',(39.4577236909665,-64.6197426555013,
-59.8857206321091));
#181148=CARTESIAN_POINT('Ctrl Pts',(39.4573077631859,-64.6287752438938,
-59.8449088102755));
#181149=CARTESIAN_POINT('Ctrl Pts',(39.457005312133,-64.6351949618876,-59.8040810762024));
#181150=CARTESIAN_POINT('Ctrl Pts',(39.4566980640726,-64.6417164994481,
-59.762605796209));
#181151=CARTESIAN_POINT('Ctrl Pts',(39.4565079517849,-64.6455419801596,
-59.7211144803144));
#181152=CARTESIAN_POINT('Ctrl Pts',(39.4564451414371,-64.646787603845,-59.679942769949));
#181153=CARTESIAN_POINT('Ctrl Pts',(39.4564298584745,-64.6470906879835,
-59.6699249029873));
#181154=CARTESIAN_POINT('Ctrl Pts',(39.4564221286262,-64.6472412200127,
-59.6599258031402));
#181155=CARTESIAN_POINT('Ctrl Pts',(39.4564221286262,-64.6472412200127,
-59.64995));
#181156=CARTESIAN_POINT('Origin',(0.,-12.9675000200281,-60.64995));
#181157=CARTESIAN_POINT('',(4.6996065532056,-66.6842487255793,-60.64995));
#181158=CARTESIAN_POINT('Origin',(-83.2809572255632,10.6199999800001,-55.24995));
#181159=CARTESIAN_POINT('',(54.1729175880533,10.61999998,-55.74995));
#181160=CARTESIAN_POINT('',(-83.2809572255632,10.6199999800001,-55.74995));
#181161=CARTESIAN_POINT('',(54.1729175880533,10.61999998,-60.42825533736));
#181162=CARTESIAN_POINT('',(54.1729175880533,10.61999998,-55.24995));
#181163=CARTESIAN_POINT('Origin',(52.5839997448578,10.6200000169308,-60.4356500018632));
#181164=CARTESIAN_POINT('Ctrl Pts',(54.1724511599876,10.6199999790607,-60.3911473089588));
#181165=CARTESIAN_POINT('Ctrl Pts',(53.416196631659,10.6200463510678,-60.4116134442483));
#181166=CARTESIAN_POINT('Ctrl Pts',(53.7125918503827,9.92402752715887,-60.4035185821655));
#181167=CARTESIAN_POINT('Ctrl Pts',(54.1790134480683,10.6199999790597,-60.6361119980572));
#181168=CARTESIAN_POINT('Ctrl Pts',(53.4174513698511,10.620046463598,-60.5214955398529));
#181169=CARTESIAN_POINT('Ctrl Pts',(53.7172936685715,9.92326040045893,-60.566814107113));
#181170=CARTESIAN_POINT('Ctrl Pts',(54.1205022571197,10.6199999790689,-60.8773492053644));
#181171=CARTESIAN_POINT('Ctrl Pts',(53.4068684094037,10.6200454844905,-60.6288932216045));
#181172=CARTESIAN_POINT('Ctrl Pts',(53.6753724344268,9.93009784663694,-60.727656118488));
#181173=CARTESIAN_POINT('Ctrl Pts',(54.002743499603,10.6199999790876,-61.0954353510634));
#181174=CARTESIAN_POINT('Ctrl Pts',(53.3671997002943,10.6200436156875,-60.7521773893818));
#181175=CARTESIAN_POINT('Ctrl Pts',(53.5909494181196,9.94395845212251,-60.8730306626286));
#181176=CARTESIAN_POINT('',(53.7129480054761,9.92396941324122,-60.42825533736));
#181177=CARTESIAN_POINT('Origin',(54.1729175880533,10.11999998,-60.42825533736));
#181178=CARTESIAN_POINT('Origin',(52.476085995332,10.1269498711132,-60.4132651018033));
#181179=CARTESIAN_POINT('Origin',(0.,-12.9675000200281,-60.64995));
#181180=CARTESIAN_POINT('Origin',(0.,-12.9675000200281,-60.8508735991007));
#181181=CARTESIAN_POINT('Origin',(-83.2809572255632,3.96999998000007,-55.24995));
#181182=CARTESIAN_POINT('',(56.2465221147258,3.96999998000001,-60.42825533736));
#181183=CARTESIAN_POINT('Origin',(54.7700863540663,3.96999970901095,-60.4480774066699));
#181184=CARTESIAN_POINT('',(56.2465221147258,3.96999998000001,-55.74995));
#181185=CARTESIAN_POINT('',(56.2465221147258,3.96999998000001,-55.24995));
#181186=CARTESIAN_POINT('',(-83.2809572255632,3.96999998000007,-55.74995));
#181187=CARTESIAN_POINT('Ctrl Pts',(56.0692321081993,3.96999998739438,-61.1207654305588));
#181188=CARTESIAN_POINT('Ctrl Pts',(55.7339281824781,3.96993431898627,-60.9380383069125));
#181189=CARTESIAN_POINT('Ctrl Pts',(55.6456300835169,4.33828227850038,-60.8898982295148));
#181190=CARTESIAN_POINT('Ctrl Pts',(56.1954681966718,3.96999998716033,-60.8888693966731));
#181191=CARTESIAN_POINT('Ctrl Pts',(55.8351750163154,3.96993697857448,-60.7722679906112));
#181192=CARTESIAN_POINT('Ctrl Pts',(55.7334016533014,4.32662458144452,-60.7353258635364));
#181193=CARTESIAN_POINT('Ctrl Pts',(56.2573698974904,3.96999998704652,-60.6289874486284));
#181194=CARTESIAN_POINT('Ctrl Pts',(55.8870156345094,3.96993824711687,-60.5772788420628));
#181195=CARTESIAN_POINT('Ctrl Pts',(55.7764277962604,4.32095586851412,-60.5620589091497));
#181196=CARTESIAN_POINT('Ctrl Pts',(56.2450717652166,3.96999998706915,-60.3615697395426));
#181197=CARTESIAN_POINT('Ctrl Pts',(55.8768003135833,3.96993799744088,-60.3787010736661));
#181198=CARTESIAN_POINT('Ctrl Pts',(55.7678794768585,4.32208288640323,-60.3838032961762));
#181199=CARTESIAN_POINT('',(55.7689460407313,4.32194224278905,-60.42825533736));
#181200=CARTESIAN_POINT('Origin',(54.4436711570071,4.49782642787904,-60.3799664581841));
#181201=CARTESIAN_POINT('Origin',(56.2465221147258,4.46999998000001,-60.42825533736));
#181202=CARTESIAN_POINT('Origin',(-83.2809572255632,3.46999998000007,-55.74995));
#181203=CARTESIAN_POINT('',(56.5468500449175,3.46999998000001,-55.24995));
#181204=CARTESIAN_POINT('Ctrl Pts',(56.2465221147258,3.96999998000001,-55.74995));
#181205=CARTESIAN_POINT('Ctrl Pts',(56.2465221147258,3.96999998000007,-55.686368912174));
#181206=CARTESIAN_POINT('Ctrl Pts',(56.2546769398593,3.95769679945019,-55.6201894474605));
#181207=CARTESIAN_POINT('Ctrl Pts',(56.2791414152599,3.91807934032033,-55.5254586103449));
#181208=CARTESIAN_POINT('Ctrl Pts',(56.2893349466768,3.90137943739412,-55.4946694819177));
#181209=CARTESIAN_POINT('Ctrl Pts',(56.3076833032272,3.87113398900435,-55.4509423050929));
#181210=CARTESIAN_POINT('Ctrl Pts',(56.3143090986482,3.86018937895708,-55.4367771782512));
#181211=CARTESIAN_POINT('Ctrl Pts',(56.3250123066359,3.84251454883922,-55.4163122595723));
#181212=CARTESIAN_POINT('Ctrl Pts',(56.3305550393438,3.83336299245163,-55.4062755461285));
#181213=CARTESIAN_POINT('Ctrl Pts',(56.3373560360861,3.82214803813549,-55.3949454630808));
#181214=CARTESIAN_POINT('Ctrl Pts',(56.3403424222434,3.81722780003639,-55.3901749729312));
#181215=CARTESIAN_POINT('Ctrl Pts',(56.3423492737411,3.8139225179561,-55.3870140318245));
#181216=CARTESIAN_POINT('Ctrl Pts',(56.3438588567501,3.81143737568338,-55.3846804045353));
#181217=CARTESIAN_POINT('Ctrl Pts',(56.361057122823,3.78313205655798,-55.3583458815392));
#181218=CARTESIAN_POINT('Ctrl Pts',(56.3862681784529,3.74351664372742,-55.3267620226715));
#181219=CARTESIAN_POINT('Ctrl Pts',(56.4537581879826,3.63103405333309,-55.272490622966));
#181220=CARTESIAN_POINT('Ctrl Pts',(56.4960371418825,3.55740103272273,-55.24995));
#181221=CARTESIAN_POINT('Ctrl Pts',(56.5468500449175,3.46999998000001,-55.24995));
#181222=CARTESIAN_POINT('',(60.,3.46999998000001,-55.24995));
#181223=CARTESIAN_POINT('Origin',(60.,28.41999998,-55.24995));
#181224=CARTESIAN_POINT('',(56.6898028749653,2.96999998000001,-55.24995));
#181225=CARTESIAN_POINT('Origin',(0.,-12.9675000200281,-55.24995));
#181226=CARTESIAN_POINT('',(60.,2.96999998000001,-55.24995));
#181227=CARTESIAN_POINT('Origin',(60.,2.96999998000001,-55.74995));
#181228=CARTESIAN_POINT('',(56.9614672388491,2.46999998000001,-55.74995));
#181229=CARTESIAN_POINT('Ctrl Pts',(56.6898028749653,2.96999998000001,-55.24995));
#181230=CARTESIAN_POINT('Ctrl Pts',(56.7016858677395,2.94886603433927,-55.24995));
#181231=CARTESIAN_POINT('Ctrl Pts',(56.7130997678492,2.92831734088818,-55.251290341342));
#181232=CARTESIAN_POINT('Ctrl Pts',(56.7240445752942,2.90849659442475,-55.2537470842863));
#181233=CARTESIAN_POINT('Ctrl Pts',(56.7352878404614,2.8881353492022,-55.2562708209998));
#181234=CARTESIAN_POINT('Ctrl Pts',(56.7460360804399,2.86854206979626,-55.2599719929299));
#181235=CARTESIAN_POINT('Ctrl Pts',(56.7562892952297,2.84981633432805,-55.264608994816));
#181236=CARTESIAN_POINT('Ctrl Pts',(56.7669895691989,2.83027412206672,-55.2694481785837));
#181237=CARTESIAN_POINT('Ctrl Pts',(56.7771507088437,2.81167651123943,-55.2753058962585));
#181238=CARTESIAN_POINT('Ctrl Pts',(56.7867727141642,2.79408090808442,-55.281919573493));
#181239=CARTESIAN_POINT('Ctrl Pts',(56.7966458647433,2.77602603971819,-55.288705875209));
#181240=CARTESIAN_POINT('Ctrl Pts',(56.805951369667,2.75902562801291,-55.2962875599196));
#181241=CARTESIAN_POINT('Ctrl Pts',(56.8146892289353,2.74309056699916,-55.3044030122517));
#181242=CARTESIAN_POINT('Ctrl Pts',(56.8237709347523,2.72652843983979,-55.3128378185799));
#181243=CARTESIAN_POINT('Ctrl Pts',(56.8322394406538,2.71111658244293,-55.3218487259178));
#181244=CARTESIAN_POINT('Ctrl Pts',(56.8400947466399,2.69682129663479,-55.3311739178811));
#181245=CARTESIAN_POINT('Ctrl Pts',(56.8417981058405,2.69372148019865,-55.3331960098984));
#181246=CARTESIAN_POINT('Ctrl Pts',(56.8434726321392,2.69067401918578,-55.3352330097888));
#181247=CARTESIAN_POINT('Ctrl Pts',(56.845118325536,2.68767834227143,-55.3372824669056));
#181248=CARTESIAN_POINT('Ctrl Pts',(56.8513033738781,2.67641961900722,-55.3449849899678));
#181249=CARTESIAN_POINT('Ctrl Pts',(56.8570811575868,2.66589325897712,-55.3528622338493));
#181250=CARTESIAN_POINT('Ctrl Pts',(56.8624516766619,2.6560608759135,-55.3607941971069));
#181251=CARTESIAN_POINT('Ctrl Pts',(56.8651369361995,2.65114468438169,-55.3647601787357));
#181252=CARTESIAN_POINT('Ctrl Pts',(56.8677203795787,2.64640180079946,-55.3687400904442));
#181253=CARTESIAN_POINT('Ctrl Pts',(56.8702020067996,2.64182647258519,-55.3727204292728));
#181254=CARTESIAN_POINT('Ctrl Pts',(56.87144282041,2.63953880847806,-55.3747105986871));
#181255=CARTESIAN_POINT('Ctrl Pts',(56.8726581799808,2.63729303714207,-55.3767008793231));
#181256=CARTESIAN_POINT('Ctrl Pts',(56.8738480855121,2.63508837452534,-55.3786896917009));
#181257=CARTESIAN_POINT('Ctrl Pts',(56.8745753673205,2.63374086333822,-55.3799052731271));
#181258=CARTESIAN_POINT('Ctrl Pts',(56.8750639043184,2.6328406229317,-55.3807258982356));
#181259=CARTESIAN_POINT('Ctrl Pts',(56.8757340298677,2.63159363101243,-55.3818723682905));
#181260=CARTESIAN_POINT('Ctrl Pts',(56.8761602965125,2.63080041985652,-55.382601637521));
#181261=CARTESIAN_POINT('Ctrl Pts',(56.876660038025,2.62986715642403,-55.3834630493362));
#181262=CARTESIAN_POINT('Ctrl Pts',(56.877341439987,2.6285969462065,-55.384650166279));
#181263=CARTESIAN_POINT('Ctrl Pts',(56.8874008790818,2.60984501557851,-55.4021754028516));
#181264=CARTESIAN_POINT('Ctrl Pts',(56.8965581664324,2.59260115861937,-55.4210010720015));
#181265=CARTESIAN_POINT('Ctrl Pts',(56.9048133020388,2.57699487761218,-55.4408432393215));
#181266=CARTESIAN_POINT('Ctrl Pts',(56.9131728876986,2.56119113444783,-55.4609364643509));
#181267=CARTESIAN_POINT('Ctrl Pts',(56.920607347811,2.54706661269637,-55.4820714680664));
#181268=CARTESIAN_POINT('Ctrl Pts',(56.927116682376,2.53470241338362,-55.5039499420776));
#181269=CARTESIAN_POINT('Ctrl Pts',(56.9337559148161,2.5220914786786,-55.5262650148309));
#181270=CARTESIAN_POINT('Ctrl Pts',(56.9394327303715,2.51131172280586,-55.549352923377));
#181271=CARTESIAN_POINT('Ctrl Pts',(56.9441471290424,2.50239512141821,-55.5729028417887));
#181272=CARTESIAN_POINT('Ctrl Pts',(56.9489146230984,2.49337809780968,-55.5967179885095));
#181273=CARTESIAN_POINT('Ctrl Pts',(56.9526978999716,2.48626615248355,-55.6210050571164));
#181274=CARTESIAN_POINT('Ctrl Pts',(56.9554969596619,2.48104061804632,-55.6454572138478));
#181275=CARTESIAN_POINT('Ctrl Pts',(56.9583447950378,2.4757240248062,-55.6703354674975));
#181276=CARTESIAN_POINT('Ctrl Pts',(56.9601738129421,2.47235983313047,-55.6953840925332));
#181277=CARTESIAN_POINT('Ctrl Pts',(56.9609840133748,2.47087968510979,-55.7203032256611));
#181278=CARTESIAN_POINT('Ctrl Pts',(56.961306163691,2.47029115154007,-55.7302115227836));
#181279=CARTESIAN_POINT('Ctrl Pts',(56.9614672388491,2.46999998000001,-55.7400996449202));
#181280=CARTESIAN_POINT('Ctrl Pts',(56.9614672388491,2.46999998000001,-55.74995));
#181281=CARTESIAN_POINT('',(-83.2809572255632,2.46999998000007,-55.74995));
#181282=CARTESIAN_POINT('Origin',(-83.2809572255632,2.46999998000007,-55.24995));
#181283=CARTESIAN_POINT('',(56.9614672388491,2.46999998000001,-60.42825533736));
#181284=CARTESIAN_POINT('',(56.9614672388491,2.46999998000001,-55.24995));
#181285=CARTESIAN_POINT('Origin',(55.5227769329619,2.47000037335106,-60.4517448637211));
#181286=CARTESIAN_POINT('Ctrl Pts',(56.9600934028813,2.46999996959074,-60.3623927486908));
#181287=CARTESIAN_POINT('Ctrl Pts',(56.3127916612335,2.47013219497061,-60.3918959659146));
#181288=CARTESIAN_POINT('Ctrl Pts',(56.4768060379592,1.84328648456651,-60.3843526253219));
#181289=CARTESIAN_POINT('Ctrl Pts',(56.9719086646405,2.46999996957515,-60.6262162467223));
#181290=CARTESIAN_POINT('Ctrl Pts',(56.3176950849992,2.47013256123684,-60.5376645429823));
#181291=CARTESIAN_POINT('Ctrl Pts',(56.4849292473983,1.84234741764349,-60.5602093497011));
#181292=CARTESIAN_POINT('Ctrl Pts',(56.9126832861355,2.46999996965326,-60.8861329835762));
#181293=CARTESIAN_POINT('Ctrl Pts',(56.2937114156122,2.47013073129461,-60.6793039133547));
#181294=CARTESIAN_POINT('Ctrl Pts',(56.4442115172646,1.84705094373349,-60.7334982606779));
#181295=CARTESIAN_POINT('Ctrl Pts',(56.7859903733788,2.46999996982182,-61.1215882796171));
#181296=CARTESIAN_POINT('Ctrl Pts',(56.232192761867,2.47012691510116,-60.8230951160809));
#181297=CARTESIAN_POINT('Ctrl Pts',(56.3570930423877,1.85720121361396,-60.8904421107847));
#181298=CARTESIAN_POINT('',(56.4778207328943,1.84316915851819,-60.42825533736));
#181299=CARTESIAN_POINT('Origin',(56.9614672388491,1.96999998000001,-60.42825533736));
#181300=CARTESIAN_POINT('Origin',(55.1149251185314,2.00184215512154,-60.3653056244591));
#181301=CARTESIAN_POINT('Origin',(0.,-12.9675000200281,-60.64995));
#181302=CARTESIAN_POINT('Origin',(0.,-12.9675000200281,-60.8508735991007));
#181303=CARTESIAN_POINT('Origin',(-83.2809572255632,-4.18000001999993,-55.24995));
#181304=CARTESIAN_POINT('',(58.1504944089282,-4.18000001999999,-60.42825533736));
#181305=CARTESIAN_POINT('Origin',(56.7672600194274,-4.18000063577663,-60.4581517878592));
#181306=CARTESIAN_POINT('',(58.1504944089236,-4.18000003396406,-55.9233081330193));
#181307=CARTESIAN_POINT('',(58.1504944089282,-4.18000001999999,-55.24995));
#181308=CARTESIAN_POINT('Ctrl Pts',(58.150494408916,-4.18000007585629,-55.9233081330339));
#181309=CARTESIAN_POINT('Ctrl Pts',(58.2011234110627,-4.1800000934009,-55.949571966873));
#181310=CARTESIAN_POINT('Ctrl Pts',(58.2508802238442,-4.18000007907268,
-55.9776159745793));
#181311=CARTESIAN_POINT('Ctrl Pts',(58.2996228616342,-4.18000005788133,
-56.007327702339));
#181312=CARTESIAN_POINT('Ctrl Pts',(58.3611066386641,-4.18000003115063,
-56.0448059621868));
#181313=CARTESIAN_POINT('Ctrl Pts',(58.4211714230486,-4.18000002563093,
-56.0849815311994));
#181314=CARTESIAN_POINT('Ctrl Pts',(58.4791990630188,-4.18000002261545,
-56.1275622952347));
#181315=CARTESIAN_POINT('Ctrl Pts',(58.5015978396009,-4.18000002145147,
-56.1439985490754));
#181316=CARTESIAN_POINT('Ctrl Pts',(58.5236932870566,-4.18000002089499,
-56.1607926562338));
#181317=CARTESIAN_POINT('Ctrl Pts',(58.5454508633043,-4.18000002055973,
-56.177925994858));
#181318=CARTESIAN_POINT('Ctrl Pts',(58.601384203271,-4.18000001969785,-56.2219715651514));
#181319=CARTESIAN_POINT('Ctrl Pts',(58.6553029072665,-4.18000001999999,
-56.2682684120419));
#181320=CARTESIAN_POINT('Ctrl Pts',(58.7070968429494,-4.18000001999999,
-56.3167184080419));
#181321=CARTESIAN_POINT('Ctrl Pts',(58.7466278917693,-4.18000001999999,
-56.3536972383227));
#181322=CARTESIAN_POINT('Ctrl Pts',(58.7849870908598,-4.18000001999997,
-56.3919927767765));
#181323=CARTESIAN_POINT('Ctrl Pts',(58.8221712586797,-4.18000002000008,
-56.4316087082659));
#181324=CARTESIAN_POINT('Ctrl Pts',(58.9081478861484,-4.18000002000031,
-56.5232080201017));
#181325=CARTESIAN_POINT('Ctrl Pts',(58.9882663096845,-4.18000002000183,
-56.6226714971191));
#181326=CARTESIAN_POINT('Ctrl Pts',(59.059488987448,-4.18000002000189,-56.7262515801497));
#181327=CARTESIAN_POINT('Ctrl Pts',(59.0864350865984,-4.18000002000191,
-56.7654396488238));
#181328=CARTESIAN_POINT('Ctrl Pts',(59.1121963184049,-4.18000002000164,
-56.8052844356691));
#181329=CARTESIAN_POINT('Ctrl Pts',(59.1367770480425,-4.18000002000115,
-56.845783548759));
#181330=CARTESIAN_POINT('Ctrl Pts',(59.1771662439534,-4.18000002000036,
-56.9123286284587));
#181331=CARTESIAN_POINT('Ctrl Pts',(59.2143783070055,-4.1800000199807,-56.9806361125577));
#181332=CARTESIAN_POINT('Ctrl Pts',(59.2484246951019,-4.18000002050115,
-57.0506994175354));
#181333=CARTESIAN_POINT('Ctrl Pts',(59.3031923634924,-4.18000002133835,
-57.1634045844535));
#181334=CARTESIAN_POINT('Ctrl Pts',(59.3500454603234,-4.18000002397293,
-57.2816264448194));
#181335=CARTESIAN_POINT('Ctrl Pts',(59.3874625053509,-4.18000002286791,
-57.4021771888577));
#181336=CARTESIAN_POINT('Ctrl Pts',(59.3945407287637,-4.18000002265887,
-57.4249819052179));
#181337=CARTESIAN_POINT('Ctrl Pts',(59.4012856253719,-4.18000002232778,
-57.4478436795316));
#181338=CARTESIAN_POINT('Ctrl Pts',(59.4076964194498,-4.18000002192605,
-57.4707623700245));
#181339=CARTESIAN_POINT('Ctrl Pts',(59.4578200392972,-4.18000001878511,
-57.6499551058582));
#181340=CARTESIAN_POINT('Ctrl Pts',(59.4876405140726,-4.18000002000073,
-57.8326096057543));
#181341=CARTESIAN_POINT('Ctrl Pts',(59.4968871656957,-4.18000002000007,
-58.0187658449578));
#181342=CARTESIAN_POINT('Ctrl Pts',(59.4989612576688,-4.18000001999992,
-58.0605220586904));
#181343=CARTESIAN_POINT('Ctrl Pts',(59.5,-4.18000001999999,-58.1024544069542));
#181344=CARTESIAN_POINT('Ctrl Pts',(59.5,-4.18000001999999,-58.1445632485962));
#181345=CARTESIAN_POINT('Ctrl Pts',(57.9789048525842,-4.18000000314622,
-61.1211158812059));
#181346=CARTESIAN_POINT('Ctrl Pts',(57.5947641336392,-4.18011275636211,
-60.9185429056887));
#181347=CARTESIAN_POINT('Ctrl Pts',(57.5408897718184,-3.75014666797429,
-60.8901206419018));
#181348=CARTESIAN_POINT('Ctrl Pts',(58.1017608867775,-4.18000000339119,
-60.8877040749259));
#181349=CARTESIAN_POINT('Ctrl Pts',(57.6864075516799,-4.18011051227318,
-60.7564968901202));
#181350=CARTESIAN_POINT('Ctrl Pts',(57.6237851397972,-3.75639532415342,
-60.7345335560658));
#181351=CARTESIAN_POINT('Ctrl Pts',(58.1609260730227,-4.18000000350811,
-60.6285977191473));
#181352=CARTESIAN_POINT('Ctrl Pts',(57.7319155584137,-4.18010945496987,
-60.5708624589658));
#181353=CARTESIAN_POINT('Ctrl Pts',(57.6637036934156,-3.75937776709444,
-60.5618009361651));
#181354=CARTESIAN_POINT('Ctrl Pts',(58.14915342597,-4.18000000348483,-60.3617046583731));
#181355=CARTESIAN_POINT('Ctrl Pts',(57.7229085994607,-4.18010966305884,
-60.3808564105654));
#181356=CARTESIAN_POINT('Ctrl Pts',(57.6557606890352,-3.75878386386294,
-60.3838931293299));
#181357=CARTESIAN_POINT('',(57.6567521511579,-3.75885801193397,-60.42825533736));
#181358=CARTESIAN_POINT('Origin',(56.2207276362741,-3.65069918556939,-60.3392403554045));
#181359=CARTESIAN_POINT('Origin',(58.1504944089282,-3.68000001999999,-60.42825533736));
#181360=CARTESIAN_POINT('Ctrl Pts',(59.5,-4.18000001999999,-58.1445632485962));
#181361=CARTESIAN_POINT('Ctrl Pts',(59.9999999999999,-4.18000001999999,
-58.144563248596));
#181362=CARTESIAN_POINT('Ctrl Pts',(60.,-4.68000001999999,-58.1445632485961));
#181363=CARTESIAN_POINT('Ctrl Pts',(59.4999999931196,-4.18000001999999,
-57.8907708245007));
#181364=CARTESIAN_POINT('Ctrl Pts',(59.9980183704624,-4.18000001999736,
-57.8406912127677));
#181365=CARTESIAN_POINT('Ctrl Pts',(60.,-4.67801447919764,-57.8400901274889));
#181366=CARTESIAN_POINT('Ctrl Pts',(59.4622668978632,-4.18000001999999,
-57.6432940448109));
#181367=CARTESIAN_POINT('Ctrl Pts',(59.9509926566885,-4.18000002000109,
-57.5443378186833));
#181368=CARTESIAN_POINT('Ctrl Pts',(59.9547202743521,-4.67607375656258,
-57.5431941162335));
#181369=CARTESIAN_POINT('Ctrl Pts',(59.3499835921793,-4.18000001999999,
-57.2816425794726));
#181370=CARTESIAN_POINT('Ctrl Pts',(59.8137304682065,-4.18000001999945,
-57.1117161950833));
#181371=CARTESIAN_POINT('Ctrl Pts',(59.819980312157,-4.67323178879642,-57.1093239470213));
#181372=CARTESIAN_POINT('Ctrl Pts',(59.3031535768727,-4.18000001999999,
-57.163418767372));
#181373=CARTESIAN_POINT('Ctrl Pts',(59.756837410337,-4.18000002,-56.9705421764153));
#181374=CARTESIAN_POINT('Ctrl Pts',(59.7637842928231,-4.67230172637259,
-56.9674919122442));
#181375=CARTESIAN_POINT('Ctrl Pts',(59.1936555403131,-4.18000001999999,
-56.9379996304409));
#181376=CARTESIAN_POINT('Ctrl Pts',(59.6242664035215,-4.18000001999999,
-56.7016181941089));
#181377=CARTESIAN_POINT('Ctrl Pts',(59.6323866477998,-4.67052667748359,
-56.6970587190125));
#181378=CARTESIAN_POINT('Ctrl Pts',(59.130710421318,-4.18000001999999,-56.8298323231333));
#181379=CARTESIAN_POINT('Ctrl Pts',(59.5482752170826,-4.18000001999972,
-56.5726707527956));
#181380=CARTESIAN_POINT('Ctrl Pts',(59.5568525046157,-4.66967405412828,
-56.567291481448));
#181381=CARTESIAN_POINT('Ctrl Pts',(58.9882652846901,-4.18000001999999,
-56.622672397275));
#181382=CARTESIAN_POINT('Ctrl Pts',(59.3766737402574,-4.18000002000027,
-56.3259306460082));
#181383=CARTESIAN_POINT('Ctrl Pts',(59.385918342594,-4.66803974391678,-56.318763868979));
#181384=CARTESIAN_POINT('Ctrl Pts',(58.9081472639374,-4.18000001999999,
-56.5232083679403));
#181385=CARTESIAN_POINT('Ctrl Pts',(59.280338735327,-4.18000002000033,-56.2075385111788));
#181386=CARTESIAN_POINT('Ctrl Pts',(59.289776717509,-4.6672543224009,-56.1994379500303));
#181387=CARTESIAN_POINT('Ctrl Pts',(58.7361948243045,-4.18000001999999,
-56.3400094513659));
#181388=CARTESIAN_POINT('Ctrl Pts',(59.0738973083079,-4.18000001999967,
-55.9896554831564));
#181389=CARTESIAN_POINT('Ctrl Pts',(59.0834337883813,-4.66580663221926,
-55.9796562580523));
#181390=CARTESIAN_POINT('Ctrl Pts',(58.6439367094154,-4.18000001999999,
-56.2554694851693));
#181391=CARTESIAN_POINT('Ctrl Pts',(58.9632803249174,-4.18000001999956,
-55.889161374227));
#181392=CARTESIAN_POINT('Ctrl Pts',(58.9727240508436,-4.66513801841297,
-55.8782346380825));
#181393=CARTESIAN_POINT('Ctrl Pts',(58.3484352743845,-4.18000001999999,
-56.0228947878735));
#181394=CARTESIAN_POINT('Ctrl Pts',(58.6095926714098,-4.18000002000086,
-55.6130627249839));
#181395=CARTESIAN_POINT('Ctrl Pts',(58.6181223301711,-4.66329754200289,
-55.5992175260631));
#181396=CARTESIAN_POINT('Ctrl Pts',(58.1237304207495,-4.18000001999999,
-55.8958235878219));
#181397=CARTESIAN_POINT('Ctrl Pts',(58.3409094947055,-4.18000001999966,
-55.4621795466313));
#181398=CARTESIAN_POINT('Ctrl Pts',(58.3484766058291,-4.66229039631671,
-55.4467718445047));
#181399=CARTESIAN_POINT('Ctrl Pts',(57.8914800739755,-4.18000001999999,
-55.8071084335971));
#181400=CARTESIAN_POINT('Ctrl Pts',(58.0634433345606,-4.18000001999999,
-55.3569201007255));
#181401=CARTESIAN_POINT('Ctrl Pts',(58.0697760887706,-4.66158691772347,
-55.3403413730918));
#181402=CARTESIAN_POINT('',(58.1110275344003,-4.66169335124394,-55.3564444851427));
#181403=CARTESIAN_POINT('Ctrl Pts',(58.1504944089282,-4.18000001999999,
-55.9233081330105));
#181404=CARTESIAN_POINT('Ctrl Pts',(58.1255832655986,-4.18002563226572,
-55.8494414008824));
#181405=CARTESIAN_POINT('Ctrl Pts',(58.106061751409,-4.18906412849159,-55.7771234176855));
#181406=CARTESIAN_POINT('Ctrl Pts',(58.0848889116252,-4.21822496899639,
-55.6769666313789));
#181407=CARTESIAN_POINT('Ctrl Pts',(58.0791815576356,-4.23049738117328,
-55.6450063090449));
#181408=CARTESIAN_POINT('Ctrl Pts',(58.0726729084789,-4.2524838218079,-55.60011339569));
#181409=CARTESIAN_POINT('Ctrl Pts',(58.070845779328,-4.26040501329147,-55.5856570568498));
#181410=CARTESIAN_POINT('Ctrl Pts',(58.0678857794548,-4.27734550201828,
-55.5579032741482));
#181411=CARTESIAN_POINT('Ctrl Pts',(58.0668113719992,-4.2856510384432,-55.5455553613248));
#181412=CARTESIAN_POINT('Ctrl Pts',(58.0626229210173,-4.33677697787841,
-55.4775428495961));
#181413=CARTESIAN_POINT('Ctrl Pts',(58.0657423370089,-4.39105200316426,
-55.4304066092172));
#181414=CARTESIAN_POINT('Ctrl Pts',(58.0816469319102,-4.51822213561182,
-55.3676734969558));
#181415=CARTESIAN_POINT('Ctrl Pts',(58.0943306756589,-4.59067482665232,
-55.3525872058048));
#181416=CARTESIAN_POINT('Ctrl Pts',(58.1110275345658,-4.6616933513699,-55.3564444847807));
#181417=CARTESIAN_POINT('Ctrl Pts',(60.,-4.68000002001403,-58.1445632485962));
#181418=CARTESIAN_POINT('Ctrl Pts',(60.,-4.67968193473502,-58.0957864029195));
#181419=CARTESIAN_POINT('Ctrl Pts',(60.0001069700172,-4.67911123269946,
-57.9996463919644));
#181420=CARTESIAN_POINT('Ctrl Pts',(59.9786990588644,-4.67769206152654,
-57.7800155067677));
#181421=CARTESIAN_POINT('Ctrl Pts',(59.9677216248097,-4.67712392184851,
-57.6942072801069));
#181422=CARTESIAN_POINT('Ctrl Pts',(59.9403282083143,-4.67613383465996,
-57.5467897991993));
#181423=CARTESIAN_POINT('Ctrl Pts',(59.9293574169479,-4.67578123721416,
-57.4945438081253));
#181424=CARTESIAN_POINT('Ctrl Pts',(59.909338151382,-4.67522481561811,-57.4116862694014));
#181425=CARTESIAN_POINT('Ctrl Pts',(59.8984361717243,-4.67493979997739,
-57.3691373259717));
#181426=CARTESIAN_POINT('Ctrl Pts',(59.8839645568739,-4.6745976975898,-57.3175982234888));
#181427=CARTESIAN_POINT('Ctrl Pts',(59.8762657221293,-4.67442462296945,
-57.2913638064885));
#181428=CARTESIAN_POINT('Ctrl Pts',(59.8728643213804,-4.67435005691444,
-57.2800219834145));
#181429=CARTESIAN_POINT('Ctrl Pts',(59.8705737762876,-4.67430026422302,
-57.2724390085803));
#181430=CARTESIAN_POINT('Ctrl Pts',(59.8690658802887,-4.67426782042607,
-57.2674905949537));
#181431=CARTESIAN_POINT('Ctrl Pts',(59.8159468167407,-4.67313231177498,
-57.0941268506631));
#181432=CARTESIAN_POINT('Ctrl Pts',(59.7524064365091,-4.67210570835516,
-56.9412163113079));
#181433=CARTESIAN_POINT('Ctrl Pts',(59.6526118787519,-4.67078986804054,
-56.7405532202682));
#181434=CARTESIAN_POINT('Ctrl Pts',(59.6185865942576,-4.67038626128515,
-56.6783902434988));
#181435=CARTESIAN_POINT('Ctrl Pts',(59.5677476238807,-4.66982743481146,
-56.5920631572585));
#181436=CARTESIAN_POINT('Ctrl Pts',(59.5423750359475,-4.66955952799355,
-56.5506254635554));
#181437=CARTESIAN_POINT('Ctrl Pts',(59.5131167474978,-4.66926458425048,
-56.5052339948439));
#181438=CARTESIAN_POINT('Ctrl Pts',(59.4986034670532,-4.66912113088379,
-56.4832661884672));
#181439=CARTESIAN_POINT('Ctrl Pts',(59.4924114798316,-4.66906046991237,
-56.4740062865164));
#181440=CARTESIAN_POINT('Ctrl Pts',(59.4882900528469,-4.66902020644244,
-56.4678673070977));
#181441=CARTESIAN_POINT('Ctrl Pts',(59.4870552619242,-4.66900815629358,
-56.4660306178073));
#181442=CARTESIAN_POINT('Ctrl Pts',(59.3000750839401,-4.66719140687508,
-56.1897207163246));
#181443=CARTESIAN_POINT('Ctrl Pts',(59.0770215284036,-4.66554103026006,
-55.958077091566));
#181444=CARTESIAN_POINT('Ctrl Pts',(58.6035557387933,-4.66312250108001,
-55.5901274066993));
#181445=CARTESIAN_POINT('Ctrl Pts',(58.3537971827932,-4.66233339403273,
-55.4532846740592));
#181446=CARTESIAN_POINT('Ctrl Pts',(58.1110275345658,-4.6616933513699,-55.3564444847807));
#181447=CARTESIAN_POINT('Ctrl Pts',(60.,-5.2768578914742,-58.1207219873789));
#181448=CARTESIAN_POINT('Ctrl Pts',(60.,-5.19571559048276,-56.120630739736));
#181449=CARTESIAN_POINT('Ctrl Pts',(58.1516269266116,-5.16456703757977,
-55.3528444275806));
#181450=CARTESIAN_POINT('Ctrl Pts',(60.,-5.07672217607537,-58.12884135333));
#181451=CARTESIAN_POINT('Ctrl Pts',(60.0000000000006,-4.99483472640268,
-56.1098379052426));
#181452=CARTESIAN_POINT('Ctrl Pts',(58.1275061007745,-4.96483231244511,
-55.3509116092302));
#181453=CARTESIAN_POINT('Ctrl Pts',(60.,-4.87658373874773,-58.1368637570314));
#181454=CARTESIAN_POINT('Ctrl Pts',(60.,-4.79479350162989,-56.0981738677457));
#181455=CARTESIAN_POINT('Ctrl Pts',(58.1024667524305,-4.76557632116263,
-55.3488500157625));
#181456=CARTESIAN_POINT('Ctrl Pts',(60.,-4.67644015442612,-58.1447026957153));
#181457=CARTESIAN_POINT('Ctrl Pts',(60.,-4.59579029342123,-56.0855524411385));
#181458=CARTESIAN_POINT('Ctrl Pts',(58.076516464363,-4.56684999234778,-55.3466493905885));
#181459=CARTESIAN_POINT('',(58.1702687711893,-5.16134041355483,-55.3608060965004));
#181460=CARTESIAN_POINT('Origin',(-8.53841912444452,-12.9124206793298,-44.4755403801697));
#181461=CARTESIAN_POINT('Ctrl Pts',(58.1702680635503,-5.1613404812212,-55.3608077644985));
#181462=CARTESIAN_POINT('Ctrl Pts',(58.2293679865849,-5.16151080175455,
-55.3858749805777));
#181463=CARTESIAN_POINT('Ctrl Pts',(58.2887638153911,-5.16169733448923,
-55.4133706067893));
#181464=CARTESIAN_POINT('Ctrl Pts',(58.3482572799606,-5.16190080218818,
-55.4433902018123));
#181465=CARTESIAN_POINT('Ctrl Pts',(58.403616216128,-5.1620901297965,-55.4713235699003));
#181466=CARTESIAN_POINT('Ctrl Pts',(58.4590597681318,-5.16229412242843,
-55.5014425932498));
#181467=CARTESIAN_POINT('Ctrl Pts',(58.5143821205383,-5.16251339670694,
-55.533829596536));
#181468=CARTESIAN_POINT('Ctrl Pts',(58.5678568240666,-5.16272534769104,
-55.5651349428123));
#181469=CARTESIAN_POINT('Ctrl Pts',(58.6212186041567,-5.16295157818672,
-55.5985595365485));
#181470=CARTESIAN_POINT('Ctrl Pts',(58.674233727342,-5.16319265297962,-55.6341791820485));
#181471=CARTESIAN_POINT('Ctrl Pts',(58.724850775648,-5.16342282304629,-55.6681876160309));
#181472=CARTESIAN_POINT('Ctrl Pts',(58.7751519844302,-5.16366652617554,
-55.7041972055608));
#181473=CARTESIAN_POINT('Ctrl Pts',(58.8248862984456,-5.16392424073454,
-55.7422722725144));
#181474=CARTESIAN_POINT('Ctrl Pts',(58.8429167479943,-5.16401767138591,
-55.756075832237));
#181475=CARTESIAN_POINT('Ctrl Pts',(58.8608722079922,-5.16411294336124,
-55.7701508313742));
#181476=CARTESIAN_POINT('Ctrl Pts',(58.8787389942346,-5.16421007847508,
-55.7845002009921));
#181477=CARTESIAN_POINT('Ctrl Pts',(58.8877315595404,-5.1642589677293,-55.7917224088159));
#181478=CARTESIAN_POINT('Ctrl Pts',(58.8967002296909,-5.16430831845212,
-55.7990129909257));
#181479=CARTESIAN_POINT('Ctrl Pts',(58.9056418555102,-5.1643581249773,-55.8063711221161));
#181480=CARTESIAN_POINT('Ctrl Pts',(58.9547410211116,-5.16463161649632,
-55.8467751950593));
#181481=CARTESIAN_POINT('Ctrl Pts',(59.0032025284632,-5.16491917470784,
-55.8892637408267));
#181482=CARTESIAN_POINT('Ctrl Pts',(59.0507464151713,-5.16522063109444,
-55.9338141127236));
#181483=CARTESIAN_POINT('Ctrl Pts',(59.0851940552815,-5.16543904952494,
-55.9660928194963));
#181484=CARTESIAN_POINT('Ctrl Pts',(59.1191606577678,-5.1656647588043,-55.9994531466577));
#181485=CARTESIAN_POINT('Ctrl Pts',(59.1525514248973,-5.16589760591263,
-56.0338733480834));
#181486=CARTESIAN_POINT('Ctrl Pts',(59.1688316709293,-5.16601113454756,
-56.0506555126113));
#181487=CARTESIAN_POINT('Ctrl Pts',(59.1849751809062,-5.16612635884093,
-56.0676894609806));
#181488=CARTESIAN_POINT('Ctrl Pts',(59.2009718553721,-5.16624325431463,
-56.084971674898));
#181489=CARTESIAN_POINT('Ctrl Pts',(59.2086173598447,-5.16629912373104,
-56.0932315944259));
#181490=CARTESIAN_POINT('Ctrl Pts',(59.2162292961149,-5.16635537467518,
-56.1015481927566));
#181491=CARTESIAN_POINT('Ctrl Pts',(59.223804757728,-5.16641198994052,-56.1099189366056));
#181492=CARTESIAN_POINT('Ctrl Pts',(59.2616457504517,-5.16669479486428,
-56.1517325280744));
#181493=CARTESIAN_POINT('Ctrl Pts',(59.2986201578731,-5.16698737347321,
-56.1949983504194));
#181494=CARTESIAN_POINT('Ctrl Pts',(59.334592750423,-5.16728901377668,-56.2396124277012));
#181495=CARTESIAN_POINT('Ctrl Pts',(59.3627978021414,-5.16752552106615,
-56.2745930134168));
#181496=CARTESIAN_POINT('Ctrl Pts',(59.3903847865505,-5.16776758215009,
-56.3103999425124));
#181497=CARTESIAN_POINT('Ctrl Pts',(59.4172896232573,-5.16801502688971,
-56.347008807102));
#181498=CARTESIAN_POINT('Ctrl Pts',(59.4307420416106,-5.16813874925952,
-56.3653132393969));
#181499=CARTESIAN_POINT('Ctrl Pts',(59.4440233093318,-5.16826381502988,
-56.3838177857316));
#181500=CARTESIAN_POINT('Ctrl Pts',(59.4571231780776,-5.16839020075939,
-56.4025190864527));
#181501=CARTESIAN_POINT('Ctrl Pts',(59.4636731124505,-5.16845339362415,
-56.4118697368133));
#181502=CARTESIAN_POINT('Ctrl Pts',(59.4701776705325,-5.16851691642642,
-56.4212695681817));
#181503=CARTESIAN_POINT('Ctrl Pts',(59.4766354471753,-5.1685807662935,-56.4307181700234));
#181504=CARTESIAN_POINT('Ctrl Pts',(59.4798643354967,-5.16861269122705,
-56.4354424709443));
#181505=CARTESIAN_POINT('Ctrl Pts',(59.4830815277213,-5.16864469793323,
-56.4401789654471));
#181506=CARTESIAN_POINT('Ctrl Pts',(59.4862868401399,-5.1686767860573,-56.444927602916));
#181507=CARTESIAN_POINT('Ctrl Pts',(59.4881839064004,-5.1686957774346,-56.4477380871213));
#181508=CARTESIAN_POINT('Ctrl Pts',(59.4900768113164,-5.16871479733262,
-56.4505528250125));
#181509=CARTESIAN_POINT('Ctrl Pts',(59.4919655159692,-5.16873384567906,
-56.453371806289));
#181510=CARTESIAN_POINT('Ctrl Pts',(59.4923738111192,-5.16873796349995,
-56.453981206166));
#181511=CARTESIAN_POINT('Ctrl Pts',(59.4927819099767,-5.1687420826503,-56.4545908043469));
#181512=CARTESIAN_POINT('Ctrl Pts',(59.4931898121432,-5.16874620312938,
-56.4552006007266));
#181513=CARTESIAN_POINT('Ctrl Pts',(59.4935348212275,-5.16874968828546,
-56.4557163746249));
#181514=CARTESIAN_POINT('Ctrl Pts',(59.4938768919222,-5.16875314605702,
-56.4562280969254));
#181515=CARTESIAN_POINT('Ctrl Pts',(59.4942319876593,-5.16875673802937,
-56.4567596810523));
#181516=CARTESIAN_POINT('Ctrl Pts',(59.4947963331228,-5.16876244666815,
-56.4576045154423));
#181517=CARTESIAN_POINT('Ctrl Pts',(59.4953854025968,-5.16876841190205,
-56.4584873269797));
#181518=CARTESIAN_POINT('Ctrl Pts',(59.4959812520547,-5.16877445315147,
-56.459381391727));
#181519=CARTESIAN_POINT('Ctrl Pts',(59.4976582299457,-5.16879145583827,
-56.4618976763262));
#181520=CARTESIAN_POINT('Ctrl Pts',(59.4993887673974,-5.16880906498809,
-56.4645037433353));
#181521=CARTESIAN_POINT('Ctrl Pts',(59.5007780026249,-5.16882323807628,
-56.4666013076562));
#181522=CARTESIAN_POINT('Ctrl Pts',(59.5012057242936,-5.16882760172673,
-56.4672471116884));
#181523=CARTESIAN_POINT('Ctrl Pts',(59.5016011421813,-5.16883163948576,
-56.4678446867341));
#181524=CARTESIAN_POINT('Ctrl Pts',(59.5019528364327,-5.1688352329881,-56.4683765142999));
#181525=CARTESIAN_POINT('Ctrl Pts',(59.5020914168666,-5.16883664895982,
-56.4685860738663));
#181526=CARTESIAN_POINT('Ctrl Pts',(59.5022224204933,-5.16883798787953,
-56.4687842301391));
#181527=CARTESIAN_POINT('Ctrl Pts',(59.5023556731693,-5.16883935012867,
-56.4689858392624));
#181528=CARTESIAN_POINT('Ctrl Pts',(59.5367190266159,-5.1691906485059,-56.5209770320496));
#181529=CARTESIAN_POINT('Ctrl Pts',(59.5720464018835,-5.16957535427328,
-56.5779234018272));
#181530=CARTESIAN_POINT('Ctrl Pts',(59.6073637659921,-5.16999470741441,
-56.6400158796074));
#181531=CARTESIAN_POINT('Ctrl Pts',(59.6250224480463,-5.17020438398497,
-56.6710621184975));
#181532=CARTESIAN_POINT('Ctrl Pts',(59.6426779759392,-5.17042272465395,
-56.7033952452903));
#181533=CARTESIAN_POINT('Ctrl Pts',(59.6602057424287,-5.17064989395518,
-56.737040707197));
#181534=CARTESIAN_POINT('Ctrl Pts',(59.6692056644245,-5.17076653779524,
-56.7543165268432));
#181535=CARTESIAN_POINT('Ctrl Pts',(59.678171880244,-5.17088550935595,-56.7719383531722));
#181536=CARTESIAN_POINT('Ctrl Pts',(59.6870874171233,-5.17100683121914,
-56.7899096887854));
#181537=CARTESIAN_POINT('Ctrl Pts',(59.6949339875807,-5.17111360667871,
-56.8057262742597));
#181538=CARTESIAN_POINT('Ctrl Pts',(59.7027422687428,-5.17122221778135,
-56.8218158271959));
#181539=CARTESIAN_POINT('Ctrl Pts',(59.7104915013929,-5.1713325453633,-56.8381608041646));
#181540=CARTESIAN_POINT('Ctrl Pts',(59.7110853572087,-5.17134100022317,
-56.8394133874938));
#181541=CARTESIAN_POINT('Ctrl Pts',(59.7116788790019,-5.17134946533307,
-56.8406674959841));
#181542=CARTESIAN_POINT('Ctrl Pts',(59.7122720621043,-5.17135794070217,
-56.8419231310425));
#181543=CARTESIAN_POINT('Ctrl Pts',(59.7310456793957,-5.17162617716265,
-56.8816626515144));
#181544=CARTESIAN_POINT('Ctrl Pts',(59.7495101056959,-5.17190543441427,
-56.9230417182683));
#181545=CARTESIAN_POINT('Ctrl Pts',(59.7674630265172,-5.17219523865143,
-56.9659917048944));
#181546=CARTESIAN_POINT('Ctrl Pts',(59.7767445993801,-5.17234506603439,
-56.9881966393615));
#181547=CARTESIAN_POINT('Ctrl Pts',(59.7858882493597,-5.1724976925733,-57.0108185107494));
#181548=CARTESIAN_POINT('Ctrl Pts',(59.7948671257502,-5.17265307882307,
-57.0338517122053));
#181549=CARTESIAN_POINT('Ctrl Pts',(59.81336526154,-5.17297320305947,-57.0813043409843));
#181550=CARTESIAN_POINT('Ctrl Pts',(59.831174391683,-5.17330518579884,-57.1305243118636));
#181551=CARTESIAN_POINT('Ctrl Pts',(59.8480354461201,-5.1736486439555,-57.1814572501127));
#181552=CARTESIAN_POINT('Ctrl Pts',(59.8557610573697,-5.17380601395919,
-57.204794348168));
#181553=CARTESIAN_POINT('Ctrl Pts',(59.8632871078165,-5.1739657909383,-57.2284907502416));
#181554=CARTESIAN_POINT('Ctrl Pts',(59.8705856169753,-5.17412792478141,
-57.2525392933092));
#181555=CARTESIAN_POINT('Ctrl Pts',(59.8708716782384,-5.1741342795329,-57.2534818634225));
#181556=CARTESIAN_POINT('Ctrl Pts',(59.8711094072179,-5.17413957064867,
-57.2542666695859));
#181557=CARTESIAN_POINT('Ctrl Pts',(59.8713509930359,-5.17414495466206,
-57.255065256389));
#181558=CARTESIAN_POINT('Ctrl Pts',(59.8717781024019,-5.17415447327771,
-57.2564771103876));
#181559=CARTESIAN_POINT('Ctrl Pts',(59.8722177914959,-5.17416428149958,
-57.2579319209848));
#181560=CARTESIAN_POINT('Ctrl Pts',(59.8729531199112,-5.17418077643834,
-57.260378593094));
#181561=CARTESIAN_POINT('Ctrl Pts',(59.8901771646284,-5.1745671474214,-57.3176884820356));
#181562=CARTESIAN_POINT('Ctrl Pts',(59.9047902755263,-5.17494006942135,
-57.3723845060344));
#181563=CARTESIAN_POINT('Ctrl Pts',(59.9172918928915,-5.17529687618782,
-57.4243847420007));
#181564=CARTESIAN_POINT('Ctrl Pts',(59.9297460126649,-5.17565232733272,
-57.4761874126511));
#181565=CARTESIAN_POINT('Ctrl Pts',(59.940104664728,-5.17599178574173,-57.5253147523025));
#181566=CARTESIAN_POINT('Ctrl Pts',(59.9488107393967,-5.17631268775669,
-57.5716951741607));
#181567=CARTESIAN_POINT('Ctrl Pts',(59.957500830105,-5.17663300061002,-57.6179904436559));
#181568=CARTESIAN_POINT('Ctrl Pts',(59.9645444268708,-5.17693482538332,
-57.6615488807856));
#181569=CARTESIAN_POINT('Ctrl Pts',(59.9703309265957,-5.17721568088245,
-57.7023085376325));
#181570=CARTESIAN_POINT('Ctrl Pts',(59.9761053124188,-5.17749594841716,
-57.7429828650907));
#181571=CARTESIAN_POINT('Ctrl Pts',(59.9806278704376,-5.17775533461081,
-57.780870126715));
#181572=CARTESIAN_POINT('Ctrl Pts',(59.9842344277409,-5.17799143846795,
-57.8159178531054));
#181573=CARTESIAN_POINT('Ctrl Pts',(59.9853062159365,-5.17806160325551,
-57.8263332537956));
#181574=CARTESIAN_POINT('Ctrl Pts',(59.9862967636936,-5.17812971229608,
-57.8364979428509));
#181575=CARTESIAN_POINT('Ctrl Pts',(59.9872140100181,-5.17819570363422,
-57.8464106967552));
#181576=CARTESIAN_POINT('Ctrl Pts',(59.9902384336499,-5.1784132959616,-57.8790958832314));
#181577=CARTESIAN_POINT('Ctrl Pts',(59.9924757817619,-5.17861044222754,
-57.9091051245478));
#181578=CARTESIAN_POINT('Ctrl Pts',(59.9941764596193,-5.17878851414488,
-57.9364589604608));
#181579=CARTESIAN_POINT('Ctrl Pts',(59.9959106434735,-5.17897009435573,
-57.9643517094501));
#181580=CARTESIAN_POINT('Ctrl Pts',(59.9970867643637,-5.17913184124641,
-57.989483403455));
#181581=CARTESIAN_POINT('Ctrl Pts',(59.9979167550151,-5.17927526458926,
-58.0118850205988));
#181582=CARTESIAN_POINT('Ctrl Pts',(59.9987570399822,-5.17942046680174,
-58.0345644834223));
#181583=CARTESIAN_POINT('Ctrl Pts',(59.9992424352802,-5.17954688819776,
-58.0544457527));
#181584=CARTESIAN_POINT('Ctrl Pts',(59.9995397872028,-5.17965615075566,
-58.0715700091907));
#181585=CARTESIAN_POINT('Ctrl Pts',(59.999842885112,-5.17976752468784,-58.0890251724035));
#181586=CARTESIAN_POINT('Ctrl Pts',(59.9999505202322,-5.17986107023935,
-58.1036157585654));
#181587=CARTESIAN_POINT('Ctrl Pts',(59.9999860523665,-5.17993856173551,
-58.1153944010507));
#181588=CARTESIAN_POINT('Ctrl Pts',(59.9999960187236,-5.17996029721361,
-58.11869817551));
#181589=CARTESIAN_POINT('Ctrl Pts',(60.,-5.17998076999238,-58.121780776237));
#181590=CARTESIAN_POINT('Ctrl Pts',(60.,-5.18000001999999,-58.1246434856214));
#181591=CARTESIAN_POINT('Ctrl Pts',(60.,-5.18000001999999,-58.1246434856214));
#181592=CARTESIAN_POINT('Ctrl Pts',(60.,-5.68000001999998,-58.1246434856214));
#181593=CARTESIAN_POINT('Ctrl Pts',(59.5,-5.68000001999999,-58.1246434856214));
#181594=CARTESIAN_POINT('Ctrl Pts',(60.,-5.17800220042073,-57.8275435066813));
#181595=CARTESIAN_POINT('Ctrl Pts',(60.0020017947382,-5.68000001999912,
-57.8269512006129));
#181596=CARTESIAN_POINT('Ctrl Pts',(59.4999999932887,-5.68000001999999,
-57.8769929082306));
#181597=CARTESIAN_POINT('Ctrl Pts',(59.9568439660775,-5.17605025203681,
-57.5376710843709));
#181598=CARTESIAN_POINT('Ctrl Pts',(59.9606548869199,-5.68000002000021,
-57.5365322236183));
#181599=CARTESIAN_POINT('Ctrl Pts',(59.4640366407682,-5.68000001999999,
-57.6353667913546));
#181600=CARTESIAN_POINT('Ctrl Pts',(59.8286045065143,-5.17319230589712,
-57.1137623423983));
#181601=CARTESIAN_POINT('Ctrl Pts',(59.8350835786331,-5.68000001999988,
-57.1113495469635));
#181602=CARTESIAN_POINT('Ctrl Pts',(59.3571704209101,-5.68000001999999,
-57.2820131603569));
#181603=CARTESIAN_POINT('Ctrl Pts',(59.7749715022372,-5.17225378701852,
-56.9746437275083));
#181604=CARTESIAN_POINT('Ctrl Pts',(59.7822107642191,-5.68000001999999,
-56.971551755675));
#181605=CARTESIAN_POINT('Ctrl Pts',(59.3124762512969,-5.68000001999999,
-57.1660493315578));
#181606=CARTESIAN_POINT('Ctrl Pts',(59.6495726219715,-5.17046209438582,
-56.7092025345767));
#181607=CARTESIAN_POINT('Ctrl Pts',(59.6581215271118,-5.68000001999999,
-56.7045411154571));
#181608=CARTESIAN_POINT('Ctrl Pts',(59.2079771855437,-5.68000001999999,
-56.9447878986704));
#181609=CARTESIAN_POINT('Ctrl Pts',(59.5774882635866,-5.16960084340769,
-56.5816816551612));
#181610=CARTESIAN_POINT('Ctrl Pts',(59.5865663613646,-5.68000001999988,
-56.5761588403972));
#181611=CARTESIAN_POINT('Ctrl Pts',(59.1479068869942,-5.68000001999999,
-56.8384914380986));
#181612=CARTESIAN_POINT('Ctrl Pts',(59.4144742405229,-5.16794806289525,
-56.3370811282929));
#181613=CARTESIAN_POINT('Ctrl Pts',(59.4243672282747,-5.6800000200001,-56.3296643856923));
#181614=CARTESIAN_POINT('Ctrl Pts',(59.0120618664304,-5.68000001999999,
-56.6346018834074));
#181615=CARTESIAN_POINT('Ctrl Pts',(59.3226768695123,-5.16715091135939,
-56.219170776799));
#181616=CARTESIAN_POINT('Ctrl Pts',(59.332837232209,-5.68000001999999,-56.210751177698));
#181617=CARTESIAN_POINT('Ctrl Pts',(58.9355640571429,-5.68000001999999,
-56.5363163451986));
#181618=CARTESIAN_POINT('Ctrl Pts',(59.1249326459437,-5.16567306852165,
-56.0006670964121));
#181619=CARTESIAN_POINT('Ctrl Pts',(59.1353297626326,-5.68000001999999,
-55.9901841613723));
#181620=CARTESIAN_POINT('Ctrl Pts',(58.770777205737,-5.68000001999999,-56.3541800398345));
#181621=CARTESIAN_POINT('Ctrl Pts',(59.0188424909195,-5.16498867365063,
-55.8995247770565));
#181622=CARTESIAN_POINT('Ctrl Pts',(59.0292080232237,-5.68000001999941,
-55.8880220414995));
#181623=CARTESIAN_POINT('Ctrl Pts',(58.6823687426766,-5.68000001999999,
-56.2698716578318));
#181624=CARTESIAN_POINT('Ctrl Pts',(58.6792405846915,-5.16309702763064,
-55.6200638122352));
#181625=CARTESIAN_POINT('Ctrl Pts',(58.6888368836822,-5.68000002000116,
-55.6053191370788));
#181626=CARTESIAN_POINT('Ctrl Pts',(58.3993671534221,-5.68000001999999,
-56.0369236173554));
#181627=CARTESIAN_POINT('Ctrl Pts',(58.4205568275121,-5.16204487752377,
-55.4647607356853));
#181628=CARTESIAN_POINT('Ctrl Pts',(58.4292417891598,-5.68000002000209,
-55.4482158581579));
#181629=CARTESIAN_POINT('Ctrl Pts',(58.1837972805939,-5.68000001999999,
-55.907468794294));
#181630=CARTESIAN_POINT('Ctrl Pts',(58.1509320687249,-5.16128538415681,
-55.3526885469843));
#181631=CARTESIAN_POINT('Ctrl Pts',(58.1583910096328,-5.68000001999999,
-55.3347486595489));
#181632=CARTESIAN_POINT('Ctrl Pts',(57.9591100572707,-5.68000001999999,
-55.8140496618682));
#181633=CARTESIAN_POINT('',(58.4950211556755,-5.6800000188644,-56.1192785199307));
#181634=CARTESIAN_POINT('Ctrl Pts',(58.1702690071152,-5.1613403910001,-55.3608055405081));
#181635=CARTESIAN_POINT('Ctrl Pts',(58.1743010560335,-5.17971624712748,
-55.3617697445889));
#181636=CARTESIAN_POINT('Ctrl Pts',(58.1786605683368,-5.19843216096695,
-55.3640065173544));
#181637=CARTESIAN_POINT('Ctrl Pts',(58.1833338005993,-5.21729373711926,
-55.3675776810761));
#181638=CARTESIAN_POINT('Ctrl Pts',(58.1886003610624,-5.238550038038,-55.3716022509258));
#181639=CARTESIAN_POINT('Ctrl Pts',(58.1942644441856,-5.25998821833413,
-55.3773204200167));
#181640=CARTESIAN_POINT('Ctrl Pts',(58.2003004346904,-5.28132166139531,
-55.3847821412548));
#181641=CARTESIAN_POINT('Ctrl Pts',(58.2049489607054,-5.29775128715139,
-55.3905286720463));
#181642=CARTESIAN_POINT('Ctrl Pts',(58.2098170367296,-5.31411560706899,
-55.397307215209));
#181643=CARTESIAN_POINT('Ctrl Pts',(58.2148923285532,-5.33028191493914,
-55.4051322059263));
#181644=CARTESIAN_POINT('Ctrl Pts',(58.2179849955258,-5.3401329753622,-55.4099004224533));
#181645=CARTESIAN_POINT('Ctrl Pts',(58.2211548043489,-5.34991112945887,
-55.4150574115756));
#181646=CARTESIAN_POINT('Ctrl Pts',(58.2243993450601,-5.35958637151734,
-55.4206069630805));
#181647=CARTESIAN_POINT('Ctrl Pts',(58.225967677309,-5.36426314875238,-55.4232894816145));
#181648=CARTESIAN_POINT('Ctrl Pts',(58.2275531794575,-5.36891497012945,
-55.4260632460597));
#181649=CARTESIAN_POINT('Ctrl Pts',(58.2291548526485,-5.3735363894443,-55.4289272873457));
#181650=CARTESIAN_POINT('Ctrl Pts',(58.2322364375269,-5.38242790111934,
-55.4344376413728));
#181651=CARTESIAN_POINT('Ctrl Pts',(58.2353848093176,-5.39122539639531,
-55.4402896686793));
#181652=CARTESIAN_POINT('Ctrl Pts',(58.238590591582,-5.39989093914508,-55.446460107076));
#181653=CARTESIAN_POINT('Ctrl Pts',(58.246168886576,-5.42037581111278,-55.4610466879965));
#181654=CARTESIAN_POINT('Ctrl Pts',(58.2540760482587,-5.44014466797659,
-55.4774287888053));
#181655=CARTESIAN_POINT('Ctrl Pts',(58.2622671943584,-5.45895665222149,
-55.4954084723211));
#181656=CARTESIAN_POINT('Ctrl Pts',(58.2685149026784,-5.47330529025757,
-55.5091222819551));
#181657=CARTESIAN_POINT('Ctrl Pts',(58.2749265025766,-5.48709521200839,
-55.5237615867766));
#181658=CARTESIAN_POINT('Ctrl Pts',(58.2814834890395,-5.50023570165083,
-55.5392311468777));
#181659=CARTESIAN_POINT('Ctrl Pts',(58.2874403289831,-5.51217347123809,
-55.5532848122378));
#181660=CARTESIAN_POINT('Ctrl Pts',(58.2935173976588,-5.52357605097868,
-55.5680240251301));
#181661=CARTESIAN_POINT('Ctrl Pts',(58.2997030672209,-5.53438410012245,
-55.5833799347695));
#181662=CARTESIAN_POINT('Ctrl Pts',(58.3013528163782,-5.53726666114311,
-55.5874754330388));
#181663=CARTESIAN_POINT('Ctrl Pts',(58.3030102474301,-5.54010686303733,
-55.5916146862691));
#181664=CARTESIAN_POINT('Ctrl Pts',(58.3046747425696,-5.54290298011746,
-55.595795358714));
#181665=CARTESIAN_POINT('Ctrl Pts',(58.3078403074174,-5.54822068260218,
-55.6037462318752));
#181666=CARTESIAN_POINT('Ctrl Pts',(58.3110339379717,-5.55338494923171,
-55.6118495944318));
#181667=CARTESIAN_POINT('Ctrl Pts',(58.3142526856721,-5.5583911824196,-55.6200917359245));
#181668=CARTESIAN_POINT('Ctrl Pts',(58.3154017686965,-5.56017839226279,
-55.6230341550751));
#181669=CARTESIAN_POINT('Ctrl Pts',(58.3167208420302,-5.56220365178525,
-55.6264272301895));
#181670=CARTESIAN_POINT('Ctrl Pts',(58.3179172203805,-5.56401232361543,
-55.629515338728));
#181671=CARTESIAN_POINT('Ctrl Pts',(58.3187709907203,-5.5653030443667,-55.6317191026759));
#181672=CARTESIAN_POINT('Ctrl Pts',(58.3195620560738,-5.56648459869974,
-55.6337664233606));
#181673=CARTESIAN_POINT('Ctrl Pts',(58.3201818027189,-5.56740338582579,
-55.6353714169426));
#181674=CARTESIAN_POINT('Ctrl Pts',(58.3283265601308,-5.57947815591762,
-55.6564643643198));
#181675=CARTESIAN_POINT('Ctrl Pts',(58.3368294939587,-5.59085195679983,
-55.6789219744901));
#181676=CARTESIAN_POINT('Ctrl Pts',(58.3456769886582,-5.60135110653471,
-55.7026578450694));
#181677=CARTESIAN_POINT('Ctrl Pts',(58.354632662861,-5.6119786307803,-55.726683937319));
#181678=CARTESIAN_POINT('Ctrl Pts',(58.3639414182481,-5.62170967284456,
-55.7520195442927));
#181679=CARTESIAN_POINT('Ctrl Pts',(58.3735831197023,-5.63039022337626,
-55.7785283749466));
#181680=CARTESIAN_POINT('Ctrl Pts',(58.3801401585359,-5.63629361161166,
-55.7965562544508));
#181681=CARTESIAN_POINT('Ctrl Pts',(58.3868510568775,-5.64171170086708,
-55.8151257580514));
#181682=CARTESIAN_POINT('Ctrl Pts',(58.3937077869254,-5.64660389354624,
-55.8341828715336));
#181683=CARTESIAN_POINT('Ctrl Pts',(58.4041124185868,-5.65402747045364,
-55.8631007733512));
#181684=CARTESIAN_POINT('Ctrl Pts',(58.4148250996874,-5.66023123059033,
-55.8930476615929));
#181685=CARTESIAN_POINT('Ctrl Pts',(58.4258082587751,-5.66518292561411,
-55.9238779014503));
#181686=CARTESIAN_POINT('Ctrl Pts',(58.4371557904385,-5.6702988959484,-55.9557309521233));
#181687=CARTESIAN_POINT('Ctrl Pts',(58.4487920759403,-5.67407831455118,
-55.9885267929902));
#181688=CARTESIAN_POINT('Ctrl Pts',(58.4606680081683,-5.67653409743918,
-56.0220755701741));
#181689=CARTESIAN_POINT('Ctrl Pts',(58.4719200139395,-5.67886086073644,
-56.0538617935414));
#181690=CARTESIAN_POINT('Ctrl Pts',(58.4833870699745,-5.68000001999999,
-56.0863234260588));
#181691=CARTESIAN_POINT('Ctrl Pts',(58.4950211556756,-5.68000001999999,
-56.1192785199305));
#181692=CARTESIAN_POINT('Ctrl Pts',(59.5,-5.68000001999999,-58.1246434856214));
#181693=CARTESIAN_POINT('Ctrl Pts',(59.5,-5.68000001999999,-58.0267693974302));
#181694=CARTESIAN_POINT('Ctrl Pts',(59.4943836373774,-5.68000001999999,
-57.9298568609375));
#181695=CARTESIAN_POINT('Ctrl Pts',(59.4831953566826,-5.68000001999999,
-57.8338865707097));
#181696=CARTESIAN_POINT('Ctrl Pts',(59.4720070759879,-5.68000001999999,
-57.7379162804819));
#181697=CARTESIAN_POINT('Ctrl Pts',(59.455245939737,-5.68000002032169,-57.6428888905768));
#181698=CARTESIAN_POINT('Ctrl Pts',(59.4329732446822,-5.68000001967878,
-57.548806713199));
#181699=CARTESIAN_POINT('Ctrl Pts',(59.4211509304572,-5.68000001933753,
-57.4988680299284));
#181700=CARTESIAN_POINT('Ctrl Pts',(59.4077647649327,-5.68000001901105,
-57.4491949286452));
#181701=CARTESIAN_POINT('Ctrl Pts',(59.3928232159439,-5.68000001896984,
-57.3997884127162));
#181702=CARTESIAN_POINT('Ctrl Pts',(59.3572029910943,-5.68000001887159,
-57.2820046937892));
#181703=CARTESIAN_POINT('Ctrl Pts',(59.3124912608683,-5.68000001980192,
-57.1660436798562));
#181704=CARTESIAN_POINT('Ctrl Pts',(59.2602343180242,-5.68000001992935,
-57.0554150259142));
#181705=CARTESIAN_POINT('Ctrl Pts',(59.2518183841936,-5.68000001994988,
-57.0375983803036));
#181706=CARTESIAN_POINT('Ctrl Pts',(59.2431998624486,-5.68000001996158,
-57.0198940947568));
#181707=CARTESIAN_POINT('Ctrl Pts',(59.2343787360437,-5.68000001996808,
-57.002302188435));
#181708=CARTESIAN_POINT('Ctrl Pts',(59.1884199680699,-5.68000002000192,
-56.9106469616823));
#181709=CARTESIAN_POINT('Ctrl Pts',(59.136987353068,-5.68000001969244,-56.8220653476532));
#181710=CARTESIAN_POINT('Ctrl Pts',(59.0800102832678,-5.68000001903091,
-56.7365294000527));
#181711=CARTESIAN_POINT('Ctrl Pts',(59.0296633903433,-5.68000001844636,
-56.6609469032671));
#181712=CARTESIAN_POINT('Ctrl Pts',(58.974589118716,-5.68000001849974,-56.587361786818));
#181713=CARTESIAN_POINT('Ctrl Pts',(58.9158341632416,-5.68000001947823,
-56.5172160817437));
#181714=CARTESIAN_POINT('Ctrl Pts',(58.8953629897436,-5.68000001981915,
-56.4927761874893));
#181715=CARTESIAN_POINT('Ctrl Pts',(58.8744667885101,-5.68000001977524,
-56.468763578303));
#181716=CARTESIAN_POINT('Ctrl Pts',(58.8531845723455,-5.68000001964656,
-56.4452355795564));
#181717=CARTESIAN_POINT('Ctrl Pts',(58.8093620434502,-5.68000001938158,
-56.396788726233));
#181718=CARTESIAN_POINT('Ctrl Pts',(58.7638692855098,-5.6800000177515,-56.3502656276834));
#181719=CARTESIAN_POINT('Ctrl Pts',(58.7166522079594,-5.68000001767937,
-56.3056325667689));
#181720=CARTESIAN_POINT('Ctrl Pts',(58.6815782873768,-5.68000001762579,
-56.2724781125951));
#181721=CARTESIAN_POINT('Ctrl Pts',(58.6455688559318,-5.680000018255,-56.2403749966795));
#181722=CARTESIAN_POINT('Ctrl Pts',(58.6086287388195,-5.68000001901365,
-56.2093177964104));
#181723=CARTESIAN_POINT('Ctrl Pts',(58.6017994579946,-5.68000001915391,
-56.203576116122));
#181724=CARTESIAN_POINT('Ctrl Pts',(58.5949404401232,-5.68000001924633,
-56.1978709269311));
#181725=CARTESIAN_POINT('Ctrl Pts',(58.5880516973688,-5.68000001929971,
-56.1922018795935));
#181726=CARTESIAN_POINT('Ctrl Pts',(58.5576786887571,-5.68000001953509,
-56.1672066040053));
#181727=CARTESIAN_POINT('Ctrl Pts',(58.5266453103076,-5.68000002035884,
-56.1428933547174));
#181728=CARTESIAN_POINT('Ctrl Pts',(58.4950211556752,-5.68000001545765,
-56.119278519931));
#181729=CARTESIAN_POINT('Origin',(-83.2809572255632,-5.68000001999993,-55.24995));
#181730=CARTESIAN_POINT('',(58.4950211556756,-5.68000001999999,-60.42825533736));
#181731=CARTESIAN_POINT('',(58.4950211556756,-5.68000001999999,-55.24995));
#181732=CARTESIAN_POINT('Origin',(56.3184043809282,-5.68000001999999,-60.2809146158445));
#181733=CARTESIAN_POINT('Ctrl Pts',(58.4950211556756,-5.68000001999999,
-60.42825533736));
#181734=CARTESIAN_POINT('Ctrl Pts',(57.9336485918015,-5.68000002,-60.4282553373601));
#181735=CARTESIAN_POINT('Ctrl Pts',(57.9983536018174,-6.23763109620483,
-60.42825533736));
#181736=CARTESIAN_POINT('Ctrl Pts',(58.4950211389271,-5.68000001999999,
-60.6471359124214));
#181737=CARTESIAN_POINT('Ctrl Pts',(57.9336485820782,-5.68000001999705,
-60.5646181976572));
#181738=CARTESIAN_POINT('Ctrl Pts',(57.9983536015968,-6.23763109430342,
-60.5741740417057));
#181739=CARTESIAN_POINT('Ctrl Pts',(58.4475018470026,-5.68000001999999,
-60.8620252214211));
#181740=CARTESIAN_POINT('Ctrl Pts',(57.9064697980399,-5.68000002000461,
-60.6982006050192));
#181741=CARTESIAN_POINT('Ctrl Pts',(57.9664686566087,-6.23586779901857,
-60.7174374956191));
#181742=CARTESIAN_POINT('Ctrl Pts',(58.3535376001277,-5.68000001999999,
-61.0621827299711));
#181743=CARTESIAN_POINT('Ctrl Pts',(57.8507724536939,-5.68000001999999,
-60.826158857425));
#181744=CARTESIAN_POINT('Ctrl Pts',(57.9034184448965,-6.23235646472971,
-60.8508735991007));
#181745=CARTESIAN_POINT('',(57.9983536018174,-6.23763109620483,-60.42825533736));
#181746=CARTESIAN_POINT('Origin',(58.4950211556756,-6.18000001999999,-60.42825533736));
#181747=CARTESIAN_POINT('Origin',(56.5401910842268,-6.15643070639488,-60.3303564555173));
#181748=CARTESIAN_POINT('Origin',(0.,-12.9675000200281,-60.64995));
#181749=CARTESIAN_POINT('Origin',(0.,-12.9675000200281,-60.8508735991007));
#181750=CARTESIAN_POINT('Origin',(-83.2809572255632,-12.3300000199999,-55.24995));
#181751=CARTESIAN_POINT('',(58.8765127194474,-12.33000002,-60.42825533736));
#181752=CARTESIAN_POINT('Origin',(56.649087690066,-12.33000002,-60.2675479548571));
#181753=CARTESIAN_POINT('',(58.8765127194368,-12.33000002,-56.2580153373943));
#181754=CARTESIAN_POINT('',(58.8765127194474,-12.33000002,-55.24995));
#181755=CARTESIAN_POINT('Ctrl Pts',(58.8765127194368,-12.330000020523,-56.2580153373943));
#181756=CARTESIAN_POINT('Ctrl Pts',(58.9314422324003,-12.3300000222489,
-56.3204146345377));
#181757=CARTESIAN_POINT('Ctrl Pts',(58.983370298854,-12.3300000263278,-56.3857545682243));
#181758=CARTESIAN_POINT('Ctrl Pts',(59.0318187534811,-12.3300000260899,
-56.4533283814552));
#181759=CARTESIAN_POINT('Ctrl Pts',(59.0712668703448,-12.3300000258962,
-56.5083489120742));
#181760=CARTESIAN_POINT('Ctrl Pts',(59.1084086074745,-12.3300000229817,
-56.5648494607724));
#181761=CARTESIAN_POINT('Ctrl Pts',(59.1430095719442,-12.3300000210667,
-56.6224388634736));
#181762=CARTESIAN_POINT('Ctrl Pts',(59.159023041084,-12.3300000201805,-56.6490914766904));
#181763=CARTESIAN_POINT('Ctrl Pts',(59.1745444070377,-12.3300000202428,
-56.6760375771056));
#181764=CARTESIAN_POINT('Ctrl Pts',(59.1895265613474,-12.3300000204054,
-56.7032144429067));
#181765=CARTESIAN_POINT('Ctrl Pts',(59.2106099692481,-12.3300000206344,
-56.7414586723615));
#181766=CARTESIAN_POINT('Ctrl Pts',(59.2307479204425,-12.3300000215029,
-56.7803865151708));
#181767=CARTESIAN_POINT('Ctrl Pts',(59.2498439227782,-12.3300000247794,
-56.8197986433709));
#181768=CARTESIAN_POINT('Ctrl Pts',(59.2732105276415,-12.3300000287887,
-56.8680248432995));
#181769=CARTESIAN_POINT('Ctrl Pts',(59.2950576358123,-12.3300000325183,
-56.9170923843789));
#181770=CARTESIAN_POINT('Ctrl Pts',(59.3153788043352,-12.330000032611,-56.9670066834531));
#181771=CARTESIAN_POINT('Ctrl Pts',(59.3234660778811,-12.3300000326479,
-56.9868712197865));
#181772=CARTESIAN_POINT('Ctrl Pts',(59.3313111418658,-12.3300000321978,
-57.0068701006064));
#181773=CARTESIAN_POINT('Ctrl Pts',(59.3389114029545,-12.3300000313575,
-57.0270043936979));
#181774=CARTESIAN_POINT('Ctrl Pts',(59.3711805702217,-12.3300000277898,
-57.1124905189758));
#181775=CARTESIAN_POINT('Ctrl Pts',(59.398787967634,-12.3300000251841,-57.1996595335916));
#181776=CARTESIAN_POINT('Ctrl Pts',(59.4213798740153,-12.3300000234584,
-57.2876290029532));
#181777=CARTESIAN_POINT('Ctrl Pts',(59.4552355589985,-12.3300000208724,
-57.4194579240095));
#181778=CARTESIAN_POINT('Ctrl Pts',(59.4782525129323,-12.3300000202447,
-57.553036259047));
#181779=CARTESIAN_POINT('Ctrl Pts',(59.4902475546029,-12.3300000200727,
-57.6884558476612));
#181780=CARTESIAN_POINT('Ctrl Pts',(59.4967374324385,-12.3300000199797,
-57.7617241705877));
#181781=CARTESIAN_POINT('Ctrl Pts',(59.5,-12.33000002,-57.8355316833217));
#181782=CARTESIAN_POINT('Ctrl Pts',(59.5,-12.33000002,-57.909894348981));
#181783=CARTESIAN_POINT('Ctrl Pts',(58.7359481105893,-12.33000002,-61.0621827299711));
#181784=CARTESIAN_POINT('Ctrl Pts',(58.2906927660831,-12.33000002,-60.8545178210735));
#181785=CARTESIAN_POINT('Ctrl Pts',(58.2828791719688,-11.838774304476,-60.8508735991007));
#181786=CARTESIAN_POINT('Ctrl Pts',(58.8284361535292,-12.33000002,-60.863878626764));
#181787=CARTESIAN_POINT('Ctrl Pts',(58.3533698277338,-12.3300000200013,
-60.7214865958624));
#181788=CARTESIAN_POINT('Ctrl Pts',(58.3445491382077,-11.8393573204241,
-60.7186709323925));
#181789=CARTESIAN_POINT('Ctrl Pts',(58.8765127155019,-12.33000002,-60.64928853347));
#181790=CARTESIAN_POINT('Ctrl Pts',(58.3860794582448,-12.330000020003,-60.5770127531963));
#181791=CARTESIAN_POINT('Ctrl Pts',(58.3766060098775,-11.8396582665817,
-60.575610749785));
#181792=CARTESIAN_POINT('Ctrl Pts',(58.8765127194474,-12.33000002,-60.42825533736));
#181793=CARTESIAN_POINT('Ctrl Pts',(58.3860794606436,-12.33000002,-60.42825533736));
#181794=CARTESIAN_POINT('Ctrl Pts',(58.376606009879,-11.839658266657,-60.42825533736));
#181795=CARTESIAN_POINT('',(58.376606009879,-11.839658266657,-60.42825533736));
#181796=CARTESIAN_POINT('Origin',(56.8912646065068,-11.8256176540576,-60.3210832102212));
#181797=CARTESIAN_POINT('Origin',(58.8765127194474,-11.83000002,-60.42825533736));
#181798=CARTESIAN_POINT('Ctrl Pts',(59.5,-12.33000002,-57.909894348981));
#181799=CARTESIAN_POINT('Ctrl Pts',(60.,-12.33000002,-57.909894348981));
#181800=CARTESIAN_POINT('Ctrl Pts',(60.,-12.83000002,-57.909894348981));
#181801=CARTESIAN_POINT('Ctrl Pts',(59.4999999942389,-12.33000002,-57.6980379098391));
#181802=CARTESIAN_POINT('Ctrl Pts',(59.9999466862306,-12.33000002,-57.6556802065741));
#181803=CARTESIAN_POINT('Ctrl Pts',(60.,-12.8299467103192,-57.6556666887753));
#181804=CARTESIAN_POINT('Ctrl Pts',(59.4734910794084,-12.33000002,-57.4906424667705));
#181805=CARTESIAN_POINT('Ctrl Pts',(59.9680873501793,-12.33000002,-57.4068180594886));
#181806=CARTESIAN_POINT('Ctrl Pts',(59.9681892936719,-12.8298948327809,
-57.4067922228916));
#181807=CARTESIAN_POINT('Ctrl Pts',(59.3691547532245,-12.33000002,-57.0846448139696));
#181808=CARTESIAN_POINT('Ctrl Pts',(59.8427924853442,-12.33000002,-56.9196714028451));
#181809=CARTESIAN_POINT('Ctrl Pts',(59.8429857054876,-12.8297938242694,
-56.9195951650643));
#181810=CARTESIAN_POINT('Ctrl Pts',(59.290326767749,-12.33000002,-56.8861589103251));
#181811=CARTESIAN_POINT('Ctrl Pts',(59.748161991806,-12.3300000200003,-56.6815232165248));
#181812=CARTESIAN_POINT('Ctrl Pts',(59.74839212134,-12.8297447315641,-56.6814121423199));
#181813=CARTESIAN_POINT('Ctrl Pts',(59.0886910851255,-12.33000002,-56.5202894131685));
#181814=CARTESIAN_POINT('Ctrl Pts',(59.5061445952809,-12.3300000199996,
-56.2425672751971));
#181815=CARTESIAN_POINT('Ctrl Pts',(59.5064293021094,-12.8296546666343,
-56.2423688578572));
#181816=CARTESIAN_POINT('Ctrl Pts',(58.9630665125599,-12.33000002,-56.3477358485963));
#181817=CARTESIAN_POINT('Ctrl Pts',(59.3553799746847,-12.3300000199993,
-56.035551183714));
#181818=CARTESIAN_POINT('Ctrl Pts',(59.3556798163584,-12.8296124190124,
-56.0353046315662));
#181819=CARTESIAN_POINT('Ctrl Pts',(58.6754296377554,-12.33000002,-56.0425683262376));
#181820=CARTESIAN_POINT('Ctrl Pts',(59.010210485167,-12.3300000200007,-55.6694530297022));
#181821=CARTESIAN_POINT('Ctrl Pts',(59.0105155640199,-12.8295379828168,
-55.6691036993668));
#181822=CARTESIAN_POINT('Ctrl Pts',(58.5142608782156,-12.33000002,-55.909436466106));
#181823=CARTESIAN_POINT('Ctrl Pts',(58.8168178148591,-12.330000020004,-55.5097431582292));
#181824=CARTESIAN_POINT('Ctrl Pts',(58.8171130576816,-12.8295056604635,
-55.509345500426));
#181825=CARTESIAN_POINT('Ctrl Pts',(58.3352984336861,-12.33000002,-55.7963700340195));
#181826=CARTESIAN_POINT('Ctrl Pts',(58.6020797386365,-12.33000002,-55.3741064461589));
#181827=CARTESIAN_POINT('Ctrl Pts',(58.6023581204233,-12.8294782784431,
-55.3736658212353));
#181828=CARTESIAN_POINT('',(58.6177174583857,-12.8294802501407,-55.3834349955086));
#181829=CARTESIAN_POINT('Ctrl Pts',(58.8765127194368,-12.33000002,-56.2580153373943));
#181830=CARTESIAN_POINT('Ctrl Pts',(58.8585209852578,-12.33000002,-56.2013005886069));
#181831=CARTESIAN_POINT('Ctrl Pts',(58.8410467971147,-12.3317761042405,
-56.1466276693133));
#181832=CARTESIAN_POINT('Ctrl Pts',(58.8243297325639,-12.3355548376282,
-56.0941100560183));
#181833=CARTESIAN_POINT('Ctrl Pts',(58.8101222933883,-12.3387662940775,
-56.0494765742092));
#181834=CARTESIAN_POINT('Ctrl Pts',(58.7964612333196,-12.3434255254537,
-56.0063987737953));
#181835=CARTESIAN_POINT('Ctrl Pts',(58.7834723352659,-12.3496919826154,
-55.964950401463));
#181836=CARTESIAN_POINT('Ctrl Pts',(58.7721737244199,-12.3551429654902,
-55.9288958395407));
#181837=CARTESIAN_POINT('Ctrl Pts',(58.7613678456248,-12.3618082266203,
-55.8940914777598));
#181838=CARTESIAN_POINT('Ctrl Pts',(58.7511110095659,-12.3697427827767,
-55.8606865226652));
#181839=CARTESIAN_POINT('Ctrl Pts',(58.7485351583987,-12.3717354280347,
-55.8522973671719));
#181840=CARTESIAN_POINT('Ctrl Pts',(58.7459938818405,-12.3738079285447,
-55.8439963184254));
#181841=CARTESIAN_POINT('Ctrl Pts',(58.7434879609094,-12.3759607512694,
-55.8357854220371));
#181842=CARTESIAN_POINT('Ctrl Pts',(58.7372458107547,-12.3813233477253,
-55.8153324031393));
#181843=CARTESIAN_POINT('Ctrl Pts',(58.7312234476295,-12.3871841683652,
-55.7954422699836));
#181844=CARTESIAN_POINT('Ctrl Pts',(58.7254354390637,-12.3935385577579,
-55.776158418215));
#181845=CARTESIAN_POINT('Ctrl Pts',(58.7225414347808,-12.3967157524543,
-55.7665164923307));
#181846=CARTESIAN_POINT('Ctrl Pts',(58.7197060675874,-12.400016186663,-55.7570260800124));
#181847=CARTESIAN_POINT('Ctrl Pts',(58.716931377285,-12.4034379210099,-55.7476928448876));
#181848=CARTESIAN_POINT('Ctrl Pts',(58.7155440321339,-12.4051487881833,
-55.7430262273252));
#181849=CARTESIAN_POINT('Ctrl Pts',(58.7141718606559,-12.4068899689845,
-55.7383988984847));
#181850=CARTESIAN_POINT('Ctrl Pts',(58.7128151416172,-12.4086611457118,
-55.7338115415017));
#181851=CARTESIAN_POINT('Ctrl Pts',(58.7119862494055,-12.4097432522886,
-55.7310088798105));
#181852=CARTESIAN_POINT('Ctrl Pts',(58.711318655935,-12.4106293729785,-55.728748087835));
#181853=CARTESIAN_POINT('Ctrl Pts',(58.7105263555936,-12.411696929288,-55.7260616020732));
#181854=CARTESIAN_POINT('Ctrl Pts',(58.7100218299517,-12.412376734034,-55.7243508859686));
#181855=CARTESIAN_POINT('Ctrl Pts',(58.7094668993149,-12.4131305686249,
-55.7224679456879));
#181856=CARTESIAN_POINT('Ctrl Pts',(58.708790617811,-12.4140639728075,-55.720169869264));
#181857=CARTESIAN_POINT('Ctrl Pts',(58.7018689859341,-12.4236172137396,
-55.6966494285302));
#181858=CARTESIAN_POINT('Ctrl Pts',(58.6953220673045,-12.4340096898909,
-55.6741234338963));
#181859=CARTESIAN_POINT('Ctrl Pts',(58.689142117507,-12.445322354964,-55.6524879771236));
#181860=CARTESIAN_POINT('Ctrl Pts',(58.688816090098,-12.4459191622203,-55.6513465840468));
#181861=CARTESIAN_POINT('Ctrl Pts',(58.6884910866061,-12.446518539468,-55.6502076772876));
#181862=CARTESIAN_POINT('Ctrl Pts',(58.6881671067845,-12.4471205016216,
-55.6490712442391));
#181863=CARTESIAN_POINT('Ctrl Pts',(58.6822938973485,-12.4580330633458,
-55.6284696238332));
#181864=CARTESIAN_POINT('Ctrl Pts',(58.6768067549597,-12.4696378308611,
-55.6089711514779));
#181865=CARTESIAN_POINT('Ctrl Pts',(58.6716658155591,-12.4820239191974,
-55.5904692077895));
#181866=CARTESIAN_POINT('Ctrl Pts',(58.6673122851234,-12.492512899586,-55.5748011034429));
#181867=CARTESIAN_POINT('Ctrl Pts',(58.6632208372979,-12.5035377526021,
-55.559896507031));
#181868=CARTESIAN_POINT('Ctrl Pts',(58.6594008505869,-12.5150268717868,
-55.5458324782439));
#181869=CARTESIAN_POINT('Ctrl Pts',(58.6588054148674,-12.5168177240764,
-55.5436402650942));
#181870=CARTESIAN_POINT('Ctrl Pts',(58.6582165495055,-12.5186197948547,
-55.541468396291));
#181871=CARTESIAN_POINT('Ctrl Pts',(58.6576342627611,-12.5204327441162,
-55.5393170772352));
#181872=CARTESIAN_POINT('Ctrl Pts',(58.6573186116315,-12.5214155236278,
-55.5381508712437));
#181873=CARTESIAN_POINT('Ctrl Pts',(58.6570048287531,-12.5224020674201,
-55.5369904365143));
#181874=CARTESIAN_POINT('Ctrl Pts',(58.6566929376964,-12.5233922269756,
-55.5358358934946));
#181875=CARTESIAN_POINT('Ctrl Pts',(58.6544037514851,-12.5306596992319,
-55.5273618962297));
#181876=CARTESIAN_POINT('Ctrl Pts',(58.6522201109272,-12.5381094452888,
-55.5192190766978));
#181877=CARTESIAN_POINT('Ctrl Pts',(58.6501344233983,-12.5457163433171,
-55.5114100449473));
#181878=CARTESIAN_POINT('Ctrl Pts',(58.6492541007718,-12.5489270469142,
-55.5081140251719));
#181879=CARTESIAN_POINT('Ctrl Pts',(58.6484620869347,-12.5519030887435,
-55.505141591748));
#181880=CARTESIAN_POINT('Ctrl Pts',(58.6476675535267,-12.5549708718073,
-55.502151001651));
#181881=CARTESIAN_POINT('Ctrl Pts',(58.6469162785288,-12.5578716292723,
-55.4993232343778));
#181882=CARTESIAN_POINT('Ctrl Pts',(58.6461627427164,-12.5608547253247,
-55.4964791002201));
#181883=CARTESIAN_POINT('Ctrl Pts',(58.6453413104498,-12.5642180477029,
-55.4933660627625));
#181884=CARTESIAN_POINT('Ctrl Pts',(58.6449732503413,-12.5657250554621,
-55.4919712004579));
#181885=CARTESIAN_POINT('Ctrl Pts',(58.6445917142175,-12.5673086803814,
-55.4905228663659));
#181886=CARTESIAN_POINT('Ctrl Pts',(58.6441917094418,-12.5689972084979,
-55.4890014166344));
#181887=CARTESIAN_POINT('Ctrl Pts',(58.6409514218902,-12.5826753367812,
-55.4766767272197));
#181888=CARTESIAN_POINT('Ctrl Pts',(58.6379842407909,-12.5969255263037,
-55.4652509528636));
#181889=CARTESIAN_POINT('Ctrl Pts',(58.6353347443317,-12.6115648322177,
-55.4549431359274));
#181890=CARTESIAN_POINT('Ctrl Pts',(58.632214720523,-12.6288039505554,-55.4428047410464));
#181891=CARTESIAN_POINT('Ctrl Pts',(58.6294915613887,-12.6467684309172,
-55.4320739374645));
#181892=CARTESIAN_POINT('Ctrl Pts',(58.6271856679341,-12.6652382398481,
-55.4228838761748));
#181893=CARTESIAN_POINT('Ctrl Pts',(58.6249108991176,-12.6834587457953,
-55.4138178610899));
#181894=CARTESIAN_POINT('Ctrl Pts',(58.6230422205788,-12.7021702479696,
-55.4062515812779));
#181895=CARTESIAN_POINT('Ctrl Pts',(58.6215869171453,-12.7211486377003,
-55.4002663143306));
#181896=CARTESIAN_POINT('Ctrl Pts',(58.6201684206881,-12.7396470332751,
-55.39443242446));
#181897=CARTESIAN_POINT('Ctrl Pts',(58.6191426248752,-12.7583983182253,
-55.3901006812464));
#181898=CARTESIAN_POINT('Ctrl Pts',(58.6185046694614,-12.777193300316,-55.3872990548521));
#181899=CARTESIAN_POINT('Ctrl Pts',(58.6179125173504,-12.7946388585472,
-55.3846985769072));
#181900=CARTESIAN_POINT('Ctrl Pts',(58.6176544005564,-12.8121216806621,
-55.383416046038));
#181901=CARTESIAN_POINT('Ctrl Pts',(58.6177174583935,-12.8294802501407,
-55.3834349955049));
#181902=CARTESIAN_POINT('Ctrl Pts',(60.,-12.83000002,-57.909894348981));
#181903=CARTESIAN_POINT('Ctrl Pts',(59.9999999999989,-12.8299744710484,
-57.8359337179673));
#181904=CARTESIAN_POINT('Ctrl Pts',(59.9972617701648,-12.8299480939923,
-57.7612058529128));
#181905=CARTESIAN_POINT('Ctrl Pts',(59.9916341638385,-12.8299212660683,
-57.6860080728811));
#181906=CARTESIAN_POINT('Ctrl Pts',(59.9860637906075,-12.829894710986,-57.6115750588015));
#181907=CARTESIAN_POINT('Ctrl Pts',(59.9776620832511,-12.8298677147732,
-57.5366821156517));
#181908=CARTESIAN_POINT('Ctrl Pts',(59.9663234619368,-12.8298406785937,
-57.4616474786362));
#181909=CARTESIAN_POINT('Ctrl Pts',(59.955082109238,-12.8298138743447,-57.3872565279253));
#181910=CARTESIAN_POINT('Ctrl Pts',(59.9409536887295,-12.829787031524,-57.3127268637753));
#181911=CARTESIAN_POINT('Ctrl Pts',(59.9238814614563,-12.8297605661022,
-57.2383904352127));
#181912=CARTESIAN_POINT('Ctrl Pts',(59.906928323879,-12.8297342852936,-57.1645725507473));
#181913=CARTESIAN_POINT('Ctrl Pts',(59.8870720994784,-12.8297083774193,
-57.0909458358442));
#181914=CARTESIAN_POINT('Ctrl Pts',(59.8643069244052,-12.8296832634698,
-57.0178481696535));
#181915=CARTESIAN_POINT('Ctrl Pts',(59.8416638492725,-12.8296582842178,
-56.94514255934));
#181916=CARTESIAN_POINT('Ctrl Pts',(59.816142868814,-12.8296340912156,-56.8729609924185));
#181917=CARTESIAN_POINT('Ctrl Pts',(59.7877896743797,-12.8296111003244,
-56.8016391523904));
#181918=CARTESIAN_POINT('Ctrl Pts',(59.7588375756144,-12.8295876237967,
-56.7288107816261));
#181919=CARTESIAN_POINT('Ctrl Pts',(59.7269321908296,-12.8295654016406,
-56.6568795902393));
#181920=CARTESIAN_POINT('Ctrl Pts',(59.6921781196006,-12.8295448649116,
-56.5861956626463));
#181921=CARTESIAN_POINT('Ctrl Pts',(59.6583339412711,-12.8295248658526,
-56.5173623039665));
#181922=CARTESIAN_POINT('Ctrl Pts',(59.6217887002356,-12.8295064658391,
-56.4497123447422));
#181923=CARTESIAN_POINT('Ctrl Pts',(59.58268887405,-12.8294900397982,-56.383552355395));
#181924=CARTESIAN_POINT('Ctrl Pts',(59.5435861500292,-12.82947361254,-56.3173874626821));
#181925=CARTESIAN_POINT('Ctrl Pts',(59.5019287886767,-12.829459160258,-56.252713343921));
#181926=CARTESIAN_POINT('Ctrl Pts',(59.4579086639815,-12.8294470237429,
-56.1898108483834));
#181927=CARTESIAN_POINT('Ctrl Pts',(59.4138217494082,-12.8294348688135,
-56.126812913543));
#181928=CARTESIAN_POINT('Ctrl Pts',(59.3673653387337,-12.8294250372887,
-56.0655924845596));
#181929=CARTESIAN_POINT('Ctrl Pts',(59.3187719001662,-12.8294178272532,
-56.006397628351));
#181930=CARTESIAN_POINT('Ctrl Pts',(59.2679932684043,-12.8294102929903,
-55.9445408449204));
#181931=CARTESIAN_POINT('Ctrl Pts',(59.2148814599025,-12.8294056222363,
-55.8848966808624));
#181932=CARTESIAN_POINT('Ctrl Pts',(59.1597391818534,-12.8294040942622,
-55.8277007148089));
#181933=CARTESIAN_POINT('Ctrl Pts',(59.106411665564,-12.8294026165744,-55.772387098482));
#181934=CARTESIAN_POINT('Ctrl Pts',(59.0511859407705,-12.8294040781501,
-55.7193631715755));
#181935=CARTESIAN_POINT('Ctrl Pts',(58.9943604122752,-12.8294086705796,
-55.6687939358799));
#181936=CARTESIAN_POINT('Ctrl Pts',(58.9346341825115,-12.829413497433,-55.6156433560243));
#181937=CARTESIAN_POINT('Ctrl Pts',(58.8731413017213,-12.8294217836238,
-55.5652050465767));
#181938=CARTESIAN_POINT('Ctrl Pts',(58.8102451196153,-12.8294336770107,
-55.5176113120292));
#181939=CARTESIAN_POINT('Ctrl Pts',(58.7473489375092,-12.8294455703977,
-55.4700175774817));
#181940=CARTESIAN_POINT('Ctrl Pts',(58.6830502669702,-12.8294610708343,
-55.4252683304837));
#181941=CARTESIAN_POINT('Ctrl Pts',(58.6177174583777,-12.8294802501408,
-55.3834349955295));
#181942=CARTESIAN_POINT('Ctrl Pts',(60.,-13.3330000856764,-57.9104187956072));
#181943=CARTESIAN_POINT('Ctrl Pts',(59.9999999999999,-13.3385258667613,
-56.2566220904403));
#181944=CARTESIAN_POINT('Ctrl Pts',(58.6015900410175,-13.3414758787461,
-55.3737206461528));
#181945=CARTESIAN_POINT('Ctrl Pts',(60.,-13.1643269532066,-57.9098552131434));
#181946=CARTESIAN_POINT('Ctrl Pts',(59.999999999998,-13.1673253991122,-56.2568074836808));
#181947=CARTESIAN_POINT('Ctrl Pts',(58.6025724987196,-13.1689005967759,
-55.3737643179335));
#181948=CARTESIAN_POINT('Ctrl Pts',(60.,-12.9956563413871,-57.9096813403539));
#181949=CARTESIAN_POINT('Ctrl Pts',(60.0000000000016,-12.9960742306928,
-56.2568641234304));
#181950=CARTESIAN_POINT('Ctrl Pts',(58.6028748593257,-12.996307708263,-55.3737777024909));
#181951=CARTESIAN_POINT('Ctrl Pts',(60.,-12.827000187199,-57.9098981644024));
#181952=CARTESIAN_POINT('Ctrl Pts',(60.,-12.8248749582876,-56.2567930570856));
#181953=CARTESIAN_POINT('Ctrl Pts',(58.6024972248876,-12.82373973381,-55.3737609414448));
#181954=CARTESIAN_POINT('',(58.6168863951182,-13.3313694067286,-55.3834094543327));
#181955=CARTESIAN_POINT('Origin',(-9.50671311766895,-12.9674995491444,-53.303688922601));
#181956=CARTESIAN_POINT('Ctrl Pts',(58.6168867413708,-13.3313694084883,
-55.383408913088));
#181957=CARTESIAN_POINT('Ctrl Pts',(58.6518309768615,-13.3313575313466,
-55.4057635202508));
#181958=CARTESIAN_POINT('Ctrl Pts',(58.6887187014103,-13.33134768207,-55.4303640415874));
#181959=CARTESIAN_POINT('Ctrl Pts',(58.727302437496,-13.3313387189539,-55.457512498856));
#181960=CARTESIAN_POINT('Ctrl Pts',(58.7659617189431,-13.3313297382884,
-55.4847141116824));
#181961=CARTESIAN_POINT('Ctrl Pts',(58.8063236557285,-13.3313216472882,
-55.5144736674302));
#181962=CARTESIAN_POINT('Ctrl Pts',(58.8481041920362,-13.3313132749985,
-55.5471338395576));
#181963=CARTESIAN_POINT('Ctrl Pts',(58.8900448541703,-13.3313048706217,
-55.5799191832962));
#181964=CARTESIAN_POINT('Ctrl Pts',(58.9334150085969,-13.3312961828305,
-55.6156274393693));
#181965=CARTESIAN_POINT('Ctrl Pts',(58.9778919914789,-13.3312860039637,
-55.6546440918516));
#181966=CARTESIAN_POINT('Ctrl Pts',(58.9877571607387,-13.3312837462511,
-55.6632981384112));
#181967=CARTESIAN_POINT('Ctrl Pts',(58.9976766455109,-13.3312814150908,
-55.6721150982506));
#181968=CARTESIAN_POINT('Ctrl Pts',(59.0076466909832,-13.3312789971485,
-55.6810994335804));
#181969=CARTESIAN_POINT('Ctrl Pts',(59.0556433273577,-13.3312673569707,
-55.7243507785303));
#181970=CARTESIAN_POINT('Ctrl Pts',(59.1046913605823,-13.331253607827,-55.7713670635205));
#181971=CARTESIAN_POINT('Ctrl Pts',(59.1543509096943,-13.3312365517527,
-55.8226288107561));
#181972=CARTESIAN_POINT('Ctrl Pts',(59.1636794475872,-13.3312333477721,
-55.8322583212952));
#181973=CARTESIAN_POINT('Ctrl Pts',(59.1730294636469,-13.3312300270276,
-55.8420377522441));
#181974=CARTESIAN_POINT('Ctrl Pts',(59.1823979034467,-13.331226581481,-55.8519704376614));
#181975=CARTESIAN_POINT('Ctrl Pts',(59.2181174888655,-13.3312134444486,
-55.889841354568));
#181976=CARTESIAN_POINT('Ctrl Pts',(59.254065600552,-13.3311984763158,-55.9299702151753));
#181977=CARTESIAN_POINT('Ctrl Pts',(59.2899681543462,-13.3311812861886,
-55.9724384503647));
#181978=CARTESIAN_POINT('Ctrl Pts',(59.324473058904,-13.3311647652552,-56.0132534411409));
#181979=CARTESIAN_POINT('Ctrl Pts',(59.3589358950507,-13.3311461918562,
-56.0562294085373));
#181980=CARTESIAN_POINT('Ctrl Pts',(59.3930756919653,-13.3311252335256,
-56.1014093033857));
#181981=CARTESIAN_POINT('Ctrl Pts',(59.413702619857,-13.3311125707094,-56.1287065493398));
#181982=CARTESIAN_POINT('Ctrl Pts',(59.4342108937052,-13.331099037572,-56.1568077491432));
#181983=CARTESIAN_POINT('Ctrl Pts',(59.4545314055103,-13.3310845637658,
-56.1857163908717));
#181984=CARTESIAN_POINT('Ctrl Pts',(59.4867505663134,-13.3310616148414,
-56.231552449795));
#181985=CARTESIAN_POINT('Ctrl Pts',(59.5185638745705,-13.3310360998369,
-56.2795149251563));
#181986=CARTESIAN_POINT('Ctrl Pts',(59.5495967522417,-13.3310081949687,
-56.329505884133));
#181987=CARTESIAN_POINT('Ctrl Pts',(59.5760753065559,-13.3309843853634,
-56.3721602694758));
#181988=CARTESIAN_POINT('Ctrl Pts',(59.6019852850859,-13.3309588362789,
-56.4162906742891));
#181989=CARTESIAN_POINT('Ctrl Pts',(59.6270838367082,-13.3309316719345,
-56.4618080042972));
#181990=CARTESIAN_POINT('Ctrl Pts',(59.655560094013,-13.3309008518747,-56.5134509524899));
#181991=CARTESIAN_POINT('Ctrl Pts',(59.6831787738492,-13.3308677658063,
-56.5672241087531));
#181992=CARTESIAN_POINT('Ctrl Pts',(59.7096306137844,-13.3308326091658,
-56.622973427477));
#181993=CARTESIAN_POINT('Ctrl Pts',(59.7363440874793,-13.3307971047927,
-56.6792741597847));
#181994=CARTESIAN_POINT('Ctrl Pts',(59.7618673284164,-13.3307594886723,
-56.7375903532155));
#181995=CARTESIAN_POINT('Ctrl Pts',(59.7858777491114,-13.3307199907229,
-56.7977099174592));
#181996=CARTESIAN_POINT('Ctrl Pts',(59.8046199401192,-13.3306891591885,
-56.8446383895037));
#181997=CARTESIAN_POINT('Ctrl Pts',(59.8224402294923,-13.3306571816186,
-56.8926645786094));
#181998=CARTESIAN_POINT('Ctrl Pts',(59.8391847459088,-13.3306241792105,
-56.9416655717737));
#181999=CARTESIAN_POINT('Ctrl Pts',(59.8585155095614,-13.3305860794687,
-56.9982349341872));
#182000=CARTESIAN_POINT('Ctrl Pts',(59.8765034568221,-13.3305464398981,
-57.0563771337676));
#182001=CARTESIAN_POINT('Ctrl Pts',(59.8928364815615,-13.3305059511937,
-57.1157678786086));
#182002=CARTESIAN_POINT('Ctrl Pts',(59.8971772508625,-13.3304951906562,
-57.1315519434763));
#182003=CARTESIAN_POINT('Ctrl Pts',(59.9014012664531,-13.3304843702828,
-57.1474239430367));
#182004=CARTESIAN_POINT('Ctrl Pts',(59.9055029853774,-13.3304735033315,
-57.1633772637068));
#182005=CARTESIAN_POINT('Ctrl Pts',(59.9215992705231,-13.3304308583944,
-57.2259825282955));
#182006=CARTESIAN_POINT('Ctrl Pts',(59.9358873636991,-13.3303875029055,
-57.2898305753006));
#182007=CARTESIAN_POINT('Ctrl Pts',(59.9481455905804,-13.330344124173,-57.3547362848755));
#182008=CARTESIAN_POINT('Ctrl Pts',(59.960235295645,-13.330301341796,-57.418749693452));
#182009=CARTESIAN_POINT('Ctrl Pts',(59.9703504144349,-13.3302585367883,
-57.4837919018522));
#182010=CARTESIAN_POINT('Ctrl Pts',(59.9783274566335,-13.3302163744338,
-57.549676722112));
#182011=CARTESIAN_POINT('Ctrl Pts',(59.9861782130125,-13.3301748795582,
-57.614518509338));
#182012=CARTESIAN_POINT('Ctrl Pts',(59.9919579901404,-13.3301340071369,
-57.6801764442022));
#182013=CARTESIAN_POINT('Ctrl Pts',(59.9955604092132,-13.3300943973881,
-57.7464645030732));
#182014=CARTESIAN_POINT('Ctrl Pts',(59.9985092463069,-13.330061973982,-57.8007260098339));
#182015=CARTESIAN_POINT('Ctrl Pts',(60.,-13.3300303967464,-57.8554095840285));
#182016=CARTESIAN_POINT('Ctrl Pts',(60.,-13.33000002,-57.9104088126279));
#182017=CARTESIAN_POINT('Ctrl Pts',(60.,-13.33000002,-57.9104088126279));
#182018=CARTESIAN_POINT('Ctrl Pts',(60.,-13.83000002,-57.9104088126279));
#182019=CARTESIAN_POINT('Ctrl Pts',(59.5,-13.83000002,-57.9104088126279));
#182020=CARTESIAN_POINT('Ctrl Pts',(60.,-13.3301404965737,-57.6560661294349));
#182021=CARTESIAN_POINT('Ctrl Pts',(59.9998595361682,-13.830000019997,-57.6561017631169));
#182022=CARTESIAN_POINT('Ctrl Pts',(59.4999999942362,-13.83000002,-57.6984561889535));
#182023=CARTESIAN_POINT('Ctrl Pts',(59.9681611381428,-13.3302771999651,
-57.4070813040103));
#182024=CARTESIAN_POINT('Ctrl Pts',(59.9678925924923,-13.8300000200007,
-57.4071493963694));
#182025=CARTESIAN_POINT('Ctrl Pts',(59.4734676164696,-13.83000002,-57.4909684574329));
#182026=CARTESIAN_POINT('Ctrl Pts',(59.8428449408308,-13.3305433698035,
-56.9196731955795));
#182027=CARTESIAN_POINT('Ctrl Pts',(59.8423361500656,-13.8300000199993,
-56.9198740502323));
#182028=CARTESIAN_POINT('Ctrl Pts',(59.3690374493417,-13.83000002,-57.084794303535));
#182029=CARTESIAN_POINT('Ctrl Pts',(59.7481694456677,-13.3306727288355,
-56.6814017112205));
#182030=CARTESIAN_POINT('Ctrl Pts',(59.7475635896442,-13.8300000199991,
-56.6816942845782));
#182031=CARTESIAN_POINT('Ctrl Pts',(59.2901412046916,-13.83000002,-56.8862343787282));
#182032=CARTESIAN_POINT('Ctrl Pts',(59.5059986510887,-13.3309100420639,
-56.2422140639419));
#182033=CARTESIAN_POINT('Ctrl Pts',(59.5052494150047,-13.8300000200009,
-56.2427365274425));
#182034=CARTESIAN_POINT('Ctrl Pts',(59.0883322092721,-13.83000002,-56.5202440244056));
#182035=CARTESIAN_POINT('Ctrl Pts',(59.3551153361278,-13.3310213578394,
-56.0350898960933));
#182036=CARTESIAN_POINT('Ctrl Pts',(59.3543264440767,-13.8300000199994,
-56.0357389914811));
#182037=CARTESIAN_POINT('Ctrl Pts',(58.9625961123716,-13.83000002,-56.3476402489859));
#182038=CARTESIAN_POINT('Ctrl Pts',(59.0096808365833,-13.3312174510841,
-55.6688506341933));
#182039=CARTESIAN_POINT('Ctrl Pts',(59.0088785326184,-13.8300000200005,
-55.6697700183809));
#182040=CARTESIAN_POINT('Ctrl Pts',(58.6747340315543,-13.83000002,-56.0424403288692));
#182041=CARTESIAN_POINT('Ctrl Pts',(58.8161264695431,-13.3313025928017,
-55.509091871258));
#182042=CARTESIAN_POINT('Ctrl Pts',(58.8153502371001,-13.83000002,-55.510138275251));
#182043=CARTESIAN_POINT('Ctrl Pts',(58.5134387215907,-13.83000002,-55.9093078011895));
#182044=CARTESIAN_POINT('Ctrl Pts',(58.6011960412544,-13.3313747072047,
-55.3734386342923));
#182045=CARTESIAN_POINT('Ctrl Pts',(58.6004643384094,-13.83000002,-55.3745979500414));
#182046=CARTESIAN_POINT('Ctrl Pts',(58.3343300343787,-13.83000002,-55.796263236946));
#182047=CARTESIAN_POINT('',(58.871735578318,-13.83000002,-56.2531111209796));
#182048=CARTESIAN_POINT('Ctrl Pts',(58.6168862797061,-13.3313694061423,
-55.3834096347511));
#182049=CARTESIAN_POINT('Ctrl Pts',(58.6166586051978,-13.3551390166932,
-55.3833412426932));
#182050=CARTESIAN_POINT('Ctrl Pts',(58.6170436760351,-13.3791016137262,
-55.3857576231866));
#182051=CARTESIAN_POINT('Ctrl Pts',(58.6180546690853,-13.4028729528674,
-55.3906118450551));
#182052=CARTESIAN_POINT('Ctrl Pts',(58.6189770783085,-13.4245614327907,
-55.395040737046));
#182053=CARTESIAN_POINT('Ctrl Pts',(58.6204203983464,-13.446089860864,-55.4014982059527));
#182054=CARTESIAN_POINT('Ctrl Pts',(58.6223869358216,-13.4671538689141,
-55.4099138186837));
#182055=CARTESIAN_POINT('Ctrl Pts',(58.6239470623716,-13.4838647216817,
-55.4165902339681));
#182056=CARTESIAN_POINT('Ctrl Pts',(58.6258366760205,-13.5002878550557,
-55.4244998730337));
#182057=CARTESIAN_POINT('Ctrl Pts',(58.6280557462051,-13.5162767774032,
-55.4336019959238));
#182058=CARTESIAN_POINT('Ctrl Pts',(58.6294397837303,-13.5262490931366,
-55.4392790041255));
#182059=CARTESIAN_POINT('Ctrl Pts',(58.6309521702184,-13.536053772359,-55.4454206393065));
#182060=CARTESIAN_POINT('Ctrl Pts',(58.6325920811364,-13.5456516620568,
-55.4520136060124));
#182061=CARTESIAN_POINT('Ctrl Pts',(58.632764313496,-13.5466596846097,-55.4527060352171));
#182062=CARTESIAN_POINT('Ctrl Pts',(58.6329379451287,-13.5476653862635,
-55.4534034132351));
#182063=CARTESIAN_POINT('Ctrl Pts',(58.6331129708765,-13.5486687027769,
-55.4541057080602));
#182064=CARTESIAN_POINT('Ctrl Pts',(58.6338940693833,-13.553146267024,-55.4572398837245));
#182065=CARTESIAN_POINT('Ctrl Pts',(58.6347033046008,-13.5575800115132,
-55.460471484084));
#182066=CARTESIAN_POINT('Ctrl Pts',(58.6355400649534,-13.5619665751822,
-55.4637967328783));
#182067=CARTESIAN_POINT('Ctrl Pts',(58.6362806787559,-13.5658491080835,
-55.4667398995169));
#182068=CARTESIAN_POINT('Ctrl Pts',(58.6370885831823,-13.5699392454374,
-55.4699453141178));
#182069=CARTESIAN_POINT('Ctrl Pts',(58.6379115394895,-13.5739434469271,
-55.4731988144793));
#182070=CARTESIAN_POINT('Ctrl Pts',(58.6387771554018,-13.5781552143021,
-55.4766209666143));
#182071=CARTESIAN_POINT('Ctrl Pts',(58.639659469486,-13.5822717024859,-55.4800963524606));
#182072=CARTESIAN_POINT('Ctrl Pts',(58.6404820528253,-13.5859780462294,
-55.4833231160771));
#182073=CARTESIAN_POINT('Ctrl Pts',(58.6408738203898,-13.5877432476288,
-55.4848599102995));
#182074=CARTESIAN_POINT('Ctrl Pts',(58.6412518113189,-13.5894158200307,
-55.4863395554386));
#182075=CARTESIAN_POINT('Ctrl Pts',(58.6416067387722,-13.5909636222847,
-55.4877260831397));
#182076=CARTESIAN_POINT('Ctrl Pts',(58.6452240649327,-13.6067384109956,
-55.501857204523));
#182077=CARTESIAN_POINT('Ctrl Pts',(58.6492790136846,-13.6219316887321,
-55.5173867126378));
#182078=CARTESIAN_POINT('Ctrl Pts',(58.6537511347767,-13.6364297661259,
-55.5342058470857));
#182079=CARTESIAN_POINT('Ctrl Pts',(58.6582232558689,-13.6509278435197,
-55.5510249815336));
#182080=CARTESIAN_POINT('Ctrl Pts',(58.6631086854053,-13.664731889532,-55.5691315342369));
#182081=CARTESIAN_POINT('Ctrl Pts',(58.6683895962004,-13.677740540402,-55.5884071874342));
#182082=CARTESIAN_POINT('Ctrl Pts',(58.6734857856715,-13.6902941608225,
-55.6070085962979));
#182083=CARTESIAN_POINT('Ctrl Pts',(58.6789585654752,-13.7021035078633,
-55.6266987231872));
#182084=CARTESIAN_POINT('Ctrl Pts',(58.6848066915835,-13.7130962049731,
-55.6473929364424));
#182085=CARTESIAN_POINT('Ctrl Pts',(58.6850186683171,-13.7134946567136,
-55.6481430385517));
#182086=CARTESIAN_POINT('Ctrl Pts',(58.6852311114247,-13.7138920091911,
-55.6488943444074));
#182087=CARTESIAN_POINT('Ctrl Pts',(58.6854440202128,-13.714288263411,-55.6496468513027));
#182088=CARTESIAN_POINT('Ctrl Pts',(58.6884873946672,-13.7199524258969,
-55.660403383631));
#182089=CARTESIAN_POINT('Ctrl Pts',(58.6916307191757,-13.7254008529457,
-55.6714221893279));
#182090=CARTESIAN_POINT('Ctrl Pts',(58.6948685872551,-13.7306305586263,
-55.6826868898889));
#182091=CARTESIAN_POINT('Ctrl Pts',(58.6964875212948,-13.7332454114665,
-55.6883192401695));
#182092=CARTESIAN_POINT('Ctrl Pts',(58.6981269348003,-13.7358066437677,
-55.6940124136505));
#182093=CARTESIAN_POINT('Ctrl Pts',(58.6997902120213,-13.7383127952728,
-55.6997653245961));
#182094=CARTESIAN_POINT('Ctrl Pts',(58.700772181751,-13.7397923832122,-55.7031617424241));
#182095=CARTESIAN_POINT('Ctrl Pts',(58.7019008874974,-13.741455747517,-55.707056057204));
#182096=CARTESIAN_POINT('Ctrl Pts',(58.7029322179606,-13.7429404982508,
-55.7106055006442));
#182097=CARTESIAN_POINT('Ctrl Pts',(58.703647772778,-13.743970643852,-55.7130681655639));
#182098=CARTESIAN_POINT('Ctrl Pts',(58.7043160412341,-13.7449159120308,
-55.715363796439));
#182099=CARTESIAN_POINT('Ctrl Pts',(58.7048515824868,-13.745665830996,-55.7172013174975));
#182100=CARTESIAN_POINT('Ctrl Pts',(58.712506737924,-13.7563853530031,-55.7434672853407));
#182101=CARTESIAN_POINT('Ctrl Pts',(58.7207003301415,-13.766106376615,-55.7711504373378));
#182102=CARTESIAN_POINT('Ctrl Pts',(58.7294033729206,-13.7747791161279,
-55.8001204503051));
#182103=CARTESIAN_POINT('Ctrl Pts',(58.7383662274934,-13.7837107627916,
-55.8299553045956));
#182104=CARTESIAN_POINT('Ctrl Pts',(58.7478693856264,-13.7915305679036,
-55.8611548223526));
#182105=CARTESIAN_POINT('Ctrl Pts',(58.757866232067,-13.7982186853384,-55.8935359318098));
#182106=CARTESIAN_POINT('Ctrl Pts',(58.7609230306435,-13.8002637530481,
-55.9034373071967));
#182107=CARTESIAN_POINT('Ctrl Pts',(58.7640258871556,-13.8022032479972,
-55.9134488916051));
#182108=CARTESIAN_POINT('Ctrl Pts',(58.7671732088176,-13.8040372220194,
-55.9235647720032));
#182109=CARTESIAN_POINT('Ctrl Pts',(58.7785673284148,-13.8106766829931,
-55.9601868791367));
#182110=CARTESIAN_POINT('Ctrl Pts',(58.7905137904197,-13.8159523307797,
-55.9980782289915));
#182111=CARTESIAN_POINT('Ctrl Pts',(58.8029474500823,-13.8199543646308,
-56.0372588901943));
#182112=CARTESIAN_POINT('Ctrl Pts',(58.8158027247144,-13.8240921040927,
-56.0777681347526));
#182113=CARTESIAN_POINT('Ctrl Pts',(58.8291786964963,-13.8268688821086,
-56.1196563252059));
#182114=CARTESIAN_POINT('Ctrl Pts',(58.842987608089,-13.8284327204152,-56.1629215142385));
#182115=CARTESIAN_POINT('Ctrl Pts',(58.8523806495261,-13.8294964681201,
-56.1923511843931));
#182116=CARTESIAN_POINT('Ctrl Pts',(58.8619736743151,-13.83000002,-56.2224174707967));
#182117=CARTESIAN_POINT('Ctrl Pts',(58.871735578318,-13.83000002,-56.2531111209796));
#182118=CARTESIAN_POINT('Ctrl Pts',(59.5,-13.83000002,-57.9104088126279));
#182119=CARTESIAN_POINT('Ctrl Pts',(59.5,-13.83000002,-57.7635265772541));
#182120=CARTESIAN_POINT('Ctrl Pts',(59.4872752713113,-13.8300000201995,
-57.6187932998347));
#182121=CARTESIAN_POINT('Ctrl Pts',(59.4620787130121,-13.8300000189704,
-57.4761129700929));
#182122=CARTESIAN_POINT('Ctrl Pts',(59.4509269987812,-13.8300000184264,
-57.4129642557027));
#182123=CARTESIAN_POINT('Ctrl Pts',(59.4373315644232,-13.8300000175808,
-57.3502178600952));
#182124=CARTESIAN_POINT('Ctrl Pts',(59.4213112185568,-13.8300000163283,
-57.287866292));
#182125=CARTESIAN_POINT('Ctrl Pts',(59.3984317821363,-13.8300000145396,
-57.1988189799231));
#182126=CARTESIAN_POINT('Ctrl Pts',(59.370414675224,-13.8300000118888,-57.1106006512125));
#182127=CARTESIAN_POINT('Ctrl Pts',(59.3376309673359,-13.8300000085315,
-57.0241300655719));
#182128=CARTESIAN_POINT('Ctrl Pts',(59.3184526052594,-13.8300000065676,
-56.9735450552968));
#182129=CARTESIAN_POINT('Ctrl Pts',(59.2977312649333,-13.8300000075911,
-56.9238144825167));
#182130=CARTESIAN_POINT('Ctrl Pts',(59.2754924251816,-13.8300000109221,
-56.874925908888));
#182131=CARTESIAN_POINT('Ctrl Pts',(59.2665370422075,-13.8300000122635,
-56.8552389151062));
#182132=CARTESIAN_POINT('Ctrl Pts',(59.2573350139601,-13.8300000139055,
-56.8356886347883));
#182133=CARTESIAN_POINT('Ctrl Pts',(59.2478858052507,-13.8300000154741,
-56.8162751713274));
#182134=CARTESIAN_POINT('Ctrl Pts',(59.2292919233252,-13.8300000185606,
-56.778073914645));
#182135=CARTESIAN_POINT('Ctrl Pts',(59.209718687562,-13.8300000193634,-56.7403307398674));
#182136=CARTESIAN_POINT('Ctrl Pts',(59.1892544368186,-13.8300000195901,
-56.7032294252422));
#182137=CARTESIAN_POINT('Ctrl Pts',(59.1734934512784,-13.8300000197646,
-56.6746550449402));
#182138=CARTESIAN_POINT('Ctrl Pts',(59.1571354382929,-13.8300000198488,
-56.6463349492494));
#182139=CARTESIAN_POINT('Ctrl Pts',(59.140235511425,-13.8300000188361,-56.6183428976771));
#182140=CARTESIAN_POINT('Ctrl Pts',(59.0995076542862,-13.8300000163955,
-56.5508836544291));
#182141=CARTESIAN_POINT('Ctrl Pts',(59.0552769615229,-13.8300000132201,
-56.4849168102432));
#182142=CARTESIAN_POINT('Ctrl Pts',(59.0079404245019,-13.8300000140848,
-56.4210933496137));
#182143=CARTESIAN_POINT('Ctrl Pts',(58.9649853093638,-13.8300000148695,
-56.3631773238039));
#182144=CARTESIAN_POINT('Ctrl Pts',(58.9194738360314,-13.8300000183267,
-56.3070268147755));
#182145=CARTESIAN_POINT('Ctrl Pts',(58.871735578318,-13.8300000195957,-56.2531111209796));
#182146=CARTESIAN_POINT('Origin',(-83.2809572255632,-13.8300000199999,-55.24995));
#182147=CARTESIAN_POINT('',(58.871735578318,-13.83000002,-60.42825533736));
#182148=CARTESIAN_POINT('',(58.871735578318,-13.83000002,-55.24995));
#182149=CARTESIAN_POINT('Origin',(56.6451562406488,-13.83000002,-60.2668362080947));
#182150=CARTESIAN_POINT('Ctrl Pts',(58.871735578318,-13.83000002,-60.42825533736));
#182151=CARTESIAN_POINT('Ctrl Pts',(58.383173457336,-13.83000002,-60.42825533736));
#182152=CARTESIAN_POINT('Ctrl Pts',(58.3718694303385,-14.3184313509278,
-60.42825533736));
#182153=CARTESIAN_POINT('Ctrl Pts',(58.871735561804,-13.83000002,-60.6470682084222));
#182154=CARTESIAN_POINT('Ctrl Pts',(58.3831734460811,-13.83000002,-60.57578605024));
#182155=CARTESIAN_POINT('Ctrl Pts',(58.3718694303297,-14.3184313513064,
-60.574130507918));
#182156=CARTESIAN_POINT('Ctrl Pts',(58.8245931841484,-13.83000002,-60.8618675123431));
#182157=CARTESIAN_POINT('Ctrl Pts',(58.3509717578384,-13.8300000200006,
-60.7206801175402));
#182158=CARTESIAN_POINT('Ctrl Pts',(58.3404329537672,-14.3187847426543,
-60.7173302229433));
#182159=CARTESIAN_POINT('Ctrl Pts',(58.7311595360587,-13.83000002,-61.0621827299711));
#182160=CARTESIAN_POINT('Ctrl Pts',(58.2874540965012,-13.83000002,-60.8552238163692));
#182161=CARTESIAN_POINT('Ctrl Pts',(58.2781275348581,-14.3194901627709,
-60.8508735991007));
#182162=CARTESIAN_POINT('',(58.3718694303385,-14.3184313509278,-60.42825533736));
#182163=CARTESIAN_POINT('Origin',(58.871735578318,-14.33000002,-60.42825533736));
#182164=CARTESIAN_POINT('Origin',(56.8873836197281,-14.3352374210018,-60.3207000331269));
#182165=CARTESIAN_POINT('Origin',(0.,-12.9675000200281,-60.64995));
#182166=CARTESIAN_POINT('Origin',(0.,-12.9675000200281,-60.8508735991007));
#182167=CARTESIAN_POINT('Origin',(-83.2809572255632,-20.4800000199999,-55.24995));
#182168=CARTESIAN_POINT('',(58.4684744114614,-20.48000002,-60.42825533736));
#182169=CARTESIAN_POINT('Origin',(56.2951177527026,-20.48000002,-60.2827926082911));
#182170=CARTESIAN_POINT('',(58.468474411447,-20.4800000218326,-56.1088024963487));
#182171=CARTESIAN_POINT('',(58.4684744114614,-20.48000002,-55.24995));
#182172=CARTESIAN_POINT('Ctrl Pts',(58.4684744114466,-20.4800000273303,
-56.1088024963493));
#182173=CARTESIAN_POINT('Ctrl Pts',(58.5045026577905,-20.4800000196856,
-56.1349726812018));
#182174=CARTESIAN_POINT('Ctrl Pts',(58.5397642385222,-20.48000002049,-56.1620276028471));
#182175=CARTESIAN_POINT('Ctrl Pts',(58.5742078503022,-20.4800000209351,
-56.1899586284693));
#182176=CARTESIAN_POINT('Ctrl Pts',(58.5777936723552,-20.4800000209814,
-56.1928664445334));
#182177=CARTESIAN_POINT('Ctrl Pts',(58.5813717160946,-20.4800000210458,
-56.1957839761558));
#182178=CARTESIAN_POINT('Ctrl Pts',(58.5849420358152,-20.4800000211331,
-56.1987112930781));
#182179=CARTESIAN_POINT('Ctrl Pts',(58.671257587695,-20.4800000232427,-56.2694816989377));
#182180=CARTESIAN_POINT('Ctrl Pts',(58.7525761504989,-20.4800000208245,
-56.3458655479472));
#182181=CARTESIAN_POINT('Ctrl Pts',(58.828900482798,-20.4800000205608,-56.4278416205054));
#182182=CARTESIAN_POINT('Ctrl Pts',(58.8336560351529,-20.4800000205444,
-56.4329493167426));
#182183=CARTESIAN_POINT('Ctrl Pts',(58.8383922119725,-20.4800000205339,
-56.4380787336291));
#182184=CARTESIAN_POINT('Ctrl Pts',(58.8431090189103,-20.4800000205297,
-56.4432298704634));
#182185=CARTESIAN_POINT('Ctrl Pts',(58.8623175352579,-20.480000020513,-56.4642071327073));
#182186=CARTESIAN_POINT('Ctrl Pts',(58.8812170617046,-20.4800000205714,
-56.4855758533909));
#182187=CARTESIAN_POINT('Ctrl Pts',(58.8997746305286,-20.4800000209296,
-56.5072905946435));
#182188=CARTESIAN_POINT('Ctrl Pts',(58.9619336923861,-20.4800000221292,
-56.580024688077));
#182189=CARTESIAN_POINT('Ctrl Pts',(59.0202267572588,-20.4800000217717,
-56.6567158251598));
#182190=CARTESIAN_POINT('Ctrl Pts',(59.0733581645971,-20.4800000210417,
-56.73565959907));
#182191=CARTESIAN_POINT('Ctrl Pts',(59.1299234282924,-20.4800000202645,
-56.8197054697148));
#182192=CARTESIAN_POINT('Ctrl Pts',(59.1811132500065,-20.480000019999,-56.9067351897848));
#182193=CARTESIAN_POINT('Ctrl Pts',(59.2269658512281,-20.4800000200342,
-56.9966989899188));
#182194=CARTESIAN_POINT('Ctrl Pts',(59.2370332340863,-20.4800000200419,
-57.016451413886));
#182195=CARTESIAN_POINT('Ctrl Pts',(59.2468434784441,-20.4800000200569,
-57.0363464697384));
#182196=CARTESIAN_POINT('Ctrl Pts',(59.2563966865596,-20.480000020085,-57.0563840875552));
#182197=CARTESIAN_POINT('Ctrl Pts',(59.3094659573342,-20.4800000202415,
-57.1676955708539));
#182198=CARTESIAN_POINT('Ctrl Pts',(59.354874917347,-20.4800000213417,-57.2844044844238));
#182199=CARTESIAN_POINT('Ctrl Pts',(59.3910801060422,-20.4800000212014,
-57.4030935519939));
#182200=CARTESIAN_POINT('Ctrl Pts',(59.4059237316432,-20.4800000211439,
-57.4517544247976));
#182201=CARTESIAN_POINT('Ctrl Pts',(59.4192561241221,-20.4800000207682,
-57.5006743231195));
#182202=CARTESIAN_POINT('Ctrl Pts',(59.4310694056707,-20.480000020378,-57.5498521826326));
#182203=CARTESIAN_POINT('Ctrl Pts',(59.453976422087,-20.4800000196214,-57.6452124794769));
#182204=CARTESIAN_POINT('Ctrl Pts',(59.4712138943901,-20.48000002,-57.7415452546604));
#182205=CARTESIAN_POINT('Ctrl Pts',(59.4827195432934,-20.48000002,-57.8388478504797));
#182206=CARTESIAN_POINT('Ctrl Pts',(59.4942251921967,-20.48000002,-57.936150446299));
#182207=CARTESIAN_POINT('Ctrl Pts',(59.5,-20.48000002,-58.0344221425213));
#182208=CARTESIAN_POINT('Ctrl Pts',(59.5,-20.48000002,-58.1336824582564));
#182209=CARTESIAN_POINT('Ctrl Pts',(58.3269264615434,-20.48000002,-61.0621827299711));
#182210=CARTESIAN_POINT('Ctrl Pts',(57.8224346115608,-20.48000002,-60.8252402001721));
#182211=CARTESIAN_POINT('Ctrl Pts',(57.8770125754992,-19.9259080025173,
-60.8508735991007));
#182212=CARTESIAN_POINT('Ctrl Pts',(58.4199720320461,-20.48000002,-60.8640724920291));
#182213=CARTESIAN_POINT('Ctrl Pts',(57.8773360553627,-20.480000020003,-60.6987815996246));
#182214=CARTESIAN_POINT('Ctrl Pts',(57.9394736727847,-19.9223173742648,
-60.7188022088811));
#182215=CARTESIAN_POINT('Ctrl Pts',(58.4684744074159,-20.48000002,-60.6493857962184));
#182216=CARTESIAN_POINT('Ctrl Pts',(57.9049228489562,-20.4800000199977,
-60.5656525957412));
#182217=CARTESIAN_POINT('Ctrl Pts',(57.9720322597472,-19.9204585218543,
-60.5756740647443));
#182218=CARTESIAN_POINT('Ctrl Pts',(58.4684744114614,-20.48000002,-60.42825533736));
#182219=CARTESIAN_POINT('Ctrl Pts',(57.9049228508695,-20.48000002,-60.42825533736));
#182220=CARTESIAN_POINT('Ctrl Pts',(57.9720322598041,-19.92045852138,-60.42825533736));
#182221=CARTESIAN_POINT('',(57.9720322598041,-19.92045852138,-60.42825533736));
#182222=CARTESIAN_POINT('Origin',(56.5149409813996,-20.0042112779349,-60.3314878981508));
#182223=CARTESIAN_POINT('Origin',(58.4684744114614,-19.98000002,-60.42825533736));
#182224=CARTESIAN_POINT('Ctrl Pts',(59.5,-20.48000002,-58.1336824582564));
#182225=CARTESIAN_POINT('Ctrl Pts',(60.,-20.48000002,-58.1336824582564));
#182226=CARTESIAN_POINT('Ctrl Pts',(60.,-20.98000002,-58.1336824582564));
#182227=CARTESIAN_POINT('Ctrl Pts',(59.4999999932334,-20.48000002,-57.8840234061944));
#182228=CARTESIAN_POINT('Ctrl Pts',(60.0019943000202,-20.4800000199965,
-57.8335762296713));
#182229=CARTESIAN_POINT('Ctrl Pts',(60.,-20.9819903749844,-57.8341710601268));
#182230=CARTESIAN_POINT('Ctrl Pts',(59.4634620545497,-20.48000002,-57.6404834185301));
#182231=CARTESIAN_POINT('Ctrl Pts',(59.9599487537765,-20.4800000200004,
-57.5408569976555));
#182232=CARTESIAN_POINT('Ctrl Pts',(59.9561544625383,-20.9839354847036,
-57.5420008057396));
#182233=CARTESIAN_POINT('Ctrl Pts',(59.3548394021004,-20.48000002,-57.2844137892711));
#182234=CARTESIAN_POINT('Ctrl Pts',(59.8322564407851,-20.4800000199998,
-57.1124079291466));
#182235=CARTESIAN_POINT('Ctrl Pts',(59.8258072839812,-20.986783840298,-57.1148311652303));
#182236=CARTESIAN_POINT('Ctrl Pts',(59.3094493357903,-20.48000002,-57.1677018516063));
#182237=CARTESIAN_POINT('Ctrl Pts',(59.7785418471728,-20.4800000199998,
-56.971709946724));
#182238=CARTESIAN_POINT('Ctrl Pts',(59.7713392035954,-20.9877182523804,
-56.9748142265907));
#182239=CARTESIAN_POINT('Ctrl Pts',(59.2033273904236,-20.48000002,-56.945074258738));
#182240=CARTESIAN_POINT('Ctrl Pts',(59.6524902953505,-20.4800000200002,
-56.7030545690594));
#182241=CARTESIAN_POINT('Ctrl Pts',(59.6439928678614,-20.9895019296767,
-56.7077325083257));
#182242=CARTESIAN_POINT('Ctrl Pts',(59.1423240613999,-20.48000002,-56.8381621017045));
#182243=CARTESIAN_POINT('Ctrl Pts',(59.5798070038494,-20.4800000200006,
-56.5739310816022));
#182244=CARTESIAN_POINT('Ctrl Pts',(59.5707888728218,-20.9903591646404,
-56.5794722449985));
#182245=CARTESIAN_POINT('Ctrl Pts',(59.0043387205048,-20.48000002,-56.6331931445326));
#182246=CARTESIAN_POINT('Ctrl Pts',(59.4150201769345,-20.4800000199993,
-56.3261371955428));
#182247=CARTESIAN_POINT('Ctrl Pts',(59.4052064654638,-20.9920036864946,
-56.333575365965));
#182248=CARTESIAN_POINT('Ctrl Pts',(58.9266500387652,-20.48000002,-56.5344951934464));
#182249=CARTESIAN_POINT('Ctrl Pts',(59.322050076116,-20.4800000199998,-56.2067284595684));
#182250=CARTESIAN_POINT('Ctrl Pts',(59.3119800474081,-20.9927961294943,
-56.2151695770875));
#182251=CARTESIAN_POINT('Ctrl Pts',(58.7595340502496,-20.48000002,-56.3519956346149));
#182252=CARTESIAN_POINT('Ctrl Pts',(59.1217230649246,-20.4800000200002,
-55.9857285998647));
#182253=CARTESIAN_POINT('Ctrl Pts',(59.1114408594098,-20.9942622260151,
-55.9962288706011));
#182254=CARTESIAN_POINT('Ctrl Pts',(58.6698748748721,-20.48000002,-56.2676023678844));
#182255=CARTESIAN_POINT('Ctrl Pts',(59.0140876322601,-20.4800000199996,
-55.8834675579712));
#182256=CARTESIAN_POINT('Ctrl Pts',(59.0038498495005,-20.9949406197357,
-55.8949841496734));
#182257=CARTESIAN_POINT('Ctrl Pts',(58.3828160087866,-20.48000002,-56.0347423933717));
#182258=CARTESIAN_POINT('Ctrl Pts',(58.6688057859238,-20.4800000200008,
-55.6008859078189));
#182259=CARTESIAN_POINT('Ctrl Pts',(58.6593792112359,-20.9968132967355,
-55.6156272797255));
#182260=CARTESIAN_POINT('Ctrl Pts',(58.1642057412792,-20.48000002,-55.9059968521648));
#182261=CARTESIAN_POINT('Ctrl Pts',(58.4055356761976,-20.48000002,-55.4446537909846));
#182262=CARTESIAN_POINT('Ctrl Pts',(58.3970469849622,-20.9978498953169,
-55.4611742661273));
#182263=CARTESIAN_POINT('Ctrl Pts',(57.9370780887383,-20.48000002,-55.8140933660895));
#182264=CARTESIAN_POINT('Ctrl Pts',(58.1317309492636,-20.48000002,-55.333033840343));
#182265=CARTESIAN_POINT('Ctrl Pts',(58.124493706486,-20.9985901469525,-55.3509197556537));
#182266=CARTESIAN_POINT('',(58.1440639001758,-20.9985364556102,-55.3589167601746));
#182267=CARTESIAN_POINT('Ctrl Pts',(58.4684744114473,-20.48000002,-56.1088024963483));
#182268=CARTESIAN_POINT('Ctrl Pts',(58.4586150911592,-20.48000002,-56.0809060452476));
#182269=CARTESIAN_POINT('Ctrl Pts',(58.4488675441718,-20.4808273659407,
-56.0533341538256));
#182270=CARTESIAN_POINT('Ctrl Pts',(58.439271777189,-20.4825381006774,-56.0262356118932));
#182271=CARTESIAN_POINT('Ctrl Pts',(58.4296891837088,-20.48424648684,-55.9991742720642));
#182272=CARTESIAN_POINT('Ctrl Pts',(58.4202577260069,-20.4868361379938,
-55.9725846325975));
#182273=CARTESIAN_POINT('Ctrl Pts',(58.4110077262225,-20.4903202028564,
-55.9465867869018));
#182274=CARTESIAN_POINT('Ctrl Pts',(58.4017480313994,-20.4938079194103,
-55.9205616925438));
#182275=CARTESIAN_POINT('Ctrl Pts',(58.3926699352244,-20.498192148329,-55.8951292415358));
#182276=CARTESIAN_POINT('Ctrl Pts',(58.3837978306082,-20.5034393255163,
-55.8703873223567));
#182277=CARTESIAN_POINT('Ctrl Pts',(58.3807115576895,-20.5052646219429,
-55.8617805353066));
#182278=CARTESIAN_POINT('Ctrl Pts',(58.3776501749549,-20.5071939136685,
-55.8532571361302));
#182279=CARTESIAN_POINT('Ctrl Pts',(58.3746146206988,-20.5092244012644,
-55.8448207432431));
#182280=CARTESIAN_POINT('Ctrl Pts',(58.372584139124,-20.5105825939711,-55.8391776418951));
#182281=CARTESIAN_POINT('Ctrl Pts',(58.3705639943634,-20.5119868533931,
-55.8335700753922));
#182282=CARTESIAN_POINT('Ctrl Pts',(58.3685538250691,-20.513436845991,-55.8279973372639));
#182283=CARTESIAN_POINT('Ctrl Pts',(58.356908165411,-20.5218371933395,-55.7957123890315));
#182284=CARTESIAN_POINT('Ctrl Pts',(58.345722168638,-20.5317310834707,-55.7649671511734));
#182285=CARTESIAN_POINT('Ctrl Pts',(58.3349661329889,-20.5429610115905,
-55.7358347356634));
#182286=CARTESIAN_POINT('Ctrl Pts',(58.331203594624,-20.5468893209383,-55.7256440079089));
#182287=CARTESIAN_POINT('Ctrl Pts',(58.3274943627873,-20.5509806039353,
-55.7156522861301));
#182288=CARTESIAN_POINT('Ctrl Pts',(58.3238427942605,-20.5552206711044,
-55.7058765663973));
#182289=CARTESIAN_POINT('Ctrl Pts',(58.3170555585969,-20.5631017597089,
-55.6877062614668));
#182290=CARTESIAN_POINT('Ctrl Pts',(58.3104649056126,-20.5715004822433,
-55.6702758635727));
#182291=CARTESIAN_POINT('Ctrl Pts',(58.3040799989639,-20.5803327986885,
-55.6536339393015));
#182292=CARTESIAN_POINT('Ctrl Pts',(58.3025560644027,-20.5824408752864,
-55.6496618838029));
#182293=CARTESIAN_POINT('Ctrl Pts',(58.3010438398826,-20.5845735942753,
-55.6457346626762));
#182294=CARTESIAN_POINT('Ctrl Pts',(58.2995426903113,-20.5867294931232,
-55.6418526824923));
#182295=CARTESIAN_POINT('Ctrl Pts',(58.2985759382629,-20.5881179088196,
-55.6393526569341));
#182296=CARTESIAN_POINT('Ctrl Pts',(58.2977808636943,-20.5892719552472,
-55.6373028066408));
#182297=CARTESIAN_POINT('Ctrl Pts',(58.2968349661429,-20.590661088457,-55.6348682143808));
#182298=CARTESIAN_POINT('Ctrl Pts',(58.2963120964897,-20.5914289682328,
-55.6335224297249));
#182299=CARTESIAN_POINT('Ctrl Pts',(58.2957432270931,-20.5922691774031,
-55.6320595294283));
#182300=CARTESIAN_POINT('Ctrl Pts',(58.2950747550774,-20.5932660660372,
-55.6303431344072));
#182301=CARTESIAN_POINT('Ctrl Pts',(58.2900178290309,-20.6008074319887,
-55.6173587723347));
#182302=CARTESIAN_POINT('Ctrl Pts',(58.2850433892305,-20.6086930001856,
-55.6047650614861));
#182303=CARTESIAN_POINT('Ctrl Pts',(58.2801491749767,-20.6169112684622,
-55.592573393822));
#182304=CARTESIAN_POINT('Ctrl Pts',(58.2713709378619,-20.6316515115047,
-55.5707064823976));
#182305=CARTESIAN_POINT('Ctrl Pts',(58.2627681449031,-20.6476358689355,
-55.5499597889634));
#182306=CARTESIAN_POINT('Ctrl Pts',(58.254476934651,-20.6644577685415,-55.5307492203234));
#182307=CARTESIAN_POINT('Ctrl Pts',(58.2536586343129,-20.6661180045886,
-55.5288532347755));
#182308=CARTESIAN_POINT('Ctrl Pts',(58.2528433587981,-20.6677864207776,
-55.5269721777696));
#182309=CARTESIAN_POINT('Ctrl Pts',(58.2520312322312,-20.6694626407703,
-55.5251064264037));
#182310=CARTESIAN_POINT('Ctrl Pts',(58.2480809834245,-20.6776159093564,
-55.5160312620064));
#182311=CARTESIAN_POINT('Ctrl Pts',(58.2441869744578,-20.6859920750144,
-55.5072765956881));
#182312=CARTESIAN_POINT('Ctrl Pts',(58.2403741015214,-20.6945317630243,
-55.4989136304009));
#182313=CARTESIAN_POINT('Ctrl Pts',(58.23462630594,-20.7074050955028,-55.4863067023113));
#182314=CARTESIAN_POINT('Ctrl Pts',(58.2290253841356,-20.7207049709202,
-55.4744915876949));
#182315=CARTESIAN_POINT('Ctrl Pts',(58.2235931329491,-20.7343275732196,
-55.4635422532062));
#182316=CARTESIAN_POINT('Ctrl Pts',(58.2233045901595,-20.7350511597281,
-55.4629606616323));
#182317=CARTESIAN_POINT('Ctrl Pts',(58.2230165181509,-20.7357756590578,
-55.4623814942482));
#182318=CARTESIAN_POINT('Ctrl Pts',(58.2227289185889,-20.7365010563778,
-55.4618047562331));
#182319=CARTESIAN_POINT('Ctrl Pts',(58.2211799409448,-20.7404079616034,
-55.4586985126577));
#182320=CARTESIAN_POINT('Ctrl Pts',(58.2197601559258,-20.7440451813824,
-55.455891187346));
#182321=CARTESIAN_POINT('Ctrl Pts',(58.2182954339984,-20.7478497743153,
-55.4530339549268));
#182322=CARTESIAN_POINT('Ctrl Pts',(58.2169581009907,-20.7513234764663,
-55.4504252200174));
#182323=CARTESIAN_POINT('Ctrl Pts',(58.215583381558,-20.7549368044839,-55.4477750853123));
#182324=CARTESIAN_POINT('Ctrl Pts',(58.214044479382,-20.7590469742192,-55.4448585269748));
#182325=CARTESIAN_POINT('Ctrl Pts',(58.2138978898006,-20.7594384923225,
-55.4445807074535));
#182326=CARTESIAN_POINT('Ctrl Pts',(58.2137498149301,-20.7598345391474,
-55.4443005040552));
#182327=CARTESIAN_POINT('Ctrl Pts',(58.213600148105,-20.7602354371672,-55.4440177446864));
#182328=CARTESIAN_POINT('Ctrl Pts',(58.2104546875774,-20.7686608774503,
-55.4380751556515));
#182329=CARTESIAN_POINT('Ctrl Pts',(58.2073520730329,-20.7772343205362,
-55.4324114748485));
#182330=CARTESIAN_POINT('Ctrl Pts',(58.2042901618585,-20.7859515214014,
-55.4270285632346));
#182331=CARTESIAN_POINT('Ctrl Pts',(58.1971740881793,-20.806210843145,-55.4145183389103));
#182332=CARTESIAN_POINT('Ctrl Pts',(58.19034522719,-20.8270685485376,-55.4036834413138));
#182333=CARTESIAN_POINT('Ctrl Pts',(58.1838456279207,-20.8482481887169,
-55.3945762010636));
#182334=CARTESIAN_POINT('Ctrl Pts',(58.1774578070436,-20.8690635870367,
-55.3856255847266));
#182335=CARTESIAN_POINT('Ctrl Pts',(58.1713880933815,-20.8901892328584,
-55.3783437776686));
#182336=CARTESIAN_POINT('Ctrl Pts',(58.1656668372239,-20.9113682799489,
-55.3727319242401));
#182337=CARTESIAN_POINT('Ctrl Pts',(58.1600697310871,-20.9320877462992,
-55.3672418468169));
#182338=CARTESIAN_POINT('Ctrl Pts',(58.1548061566892,-20.9528577928021,
-55.3633499650214));
#182339=CARTESIAN_POINT('Ctrl Pts',(58.1498945349745,-20.973452350577,-55.3610106076793));
#182340=CARTESIAN_POINT('Ctrl Pts',(58.1478923796479,-20.9818474400081,
-55.3600570006967));
#182341=CARTESIAN_POINT('Ctrl Pts',(58.1459485875571,-20.9902135813046,
-55.3593608307665));
#182342=CARTESIAN_POINT('Ctrl Pts',(58.1440639002148,-20.9985364556096,
-55.3589167601806));
#182343=CARTESIAN_POINT('Ctrl Pts',(60.,-20.98000002,-58.1336824582564));
#182344=CARTESIAN_POINT('Ctrl Pts',(59.9999999997674,-20.9803021616334,
-58.0882157632118));
#182345=CARTESIAN_POINT('Ctrl Pts',(60.0003031804244,-20.9808684474578,
-57.9944661926472));
#182346=CARTESIAN_POINT('Ctrl Pts',(59.9796366043166,-20.9822991402003,
-57.777034661397));
#182347=CARTESIAN_POINT('Ctrl Pts',(59.9689735227541,-20.9828743238743,
-57.6917239003171));
#182348=CARTESIAN_POINT('Ctrl Pts',(59.942094721024,-20.9838800398805,-57.544675306863));
#182349=CARTESIAN_POINT('Ctrl Pts',(59.9313020397326,-20.9842386835097,
-57.4924893380618));
#182350=CARTESIAN_POINT('Ctrl Pts',(59.9115468165673,-20.9848053002678,
-57.4096254596961));
#182351=CARTESIAN_POINT('Ctrl Pts',(59.9007760151545,-20.9850956924844,
-57.3670492763596));
#182352=CARTESIAN_POINT('Ctrl Pts',(59.8864524794301,-20.9854444946362,
-57.3154362005822));
#182353=CARTESIAN_POINT('Ctrl Pts',(59.878825961181,-20.9856210151906,-57.2891542770501));
#182354=CARTESIAN_POINT('Ctrl Pts',(59.8754551313071,-20.9856970774085,
-57.2777898441744));
#182355=CARTESIAN_POINT('Ctrl Pts',(59.8731848670668,-20.9857478716902,
-57.2701912967782));
#182356=CARTESIAN_POINT('Ctrl Pts',(59.8716798328276,-20.9857811954749,
-57.2651985555473));
#182357=CARTESIAN_POINT('Ctrl Pts',(59.8196830912949,-20.9869250078408,
-57.0936552223813));
#182358=CARTESIAN_POINT('Ctrl Pts',(59.757474576671,-20.9879592746227,-56.9421719733048));
#182359=CARTESIAN_POINT('Ctrl Pts',(59.6596400021207,-20.9892878172319,
-56.743058949969));
#182360=CARTESIAN_POINT('Ctrl Pts',(59.6262622512368,-20.9896958019818,
-56.6813165976652));
#182361=CARTESIAN_POINT('Ctrl Pts',(59.5763474792179,-20.9902612715535,
-56.595487236136));
#182362=CARTESIAN_POINT('Ctrl Pts',(59.5514253393024,-20.9905325160149,
-56.5542652258299));
#182363=CARTESIAN_POINT('Ctrl Pts',(59.5226651625736,-20.9908313281143,
-56.5090707039936));
#182364=CARTESIAN_POINT('Ctrl Pts',(59.5083933141467,-20.9909767015006,
-56.4871881701081));
#182365=CARTESIAN_POINT('Ctrl Pts',(59.5023030840063,-20.9910381814721,
-56.4779620351937));
#182366=CARTESIAN_POINT('Ctrl Pts',(59.4982491056196,-20.9910789899889,
-56.4718449554271));
#182367=CARTESIAN_POINT('Ctrl Pts',(59.4970283633816,-20.9910912648199,
-56.470005589356));
#182368=CARTESIAN_POINT('Ctrl Pts',(59.313480930561,-20.9929287419126,-56.1952337005415));
#182369=CARTESIAN_POINT('Ctrl Pts',(59.0944609290821,-20.9945975243808,
-55.9642839660056));
#182370=CARTESIAN_POINT('Ctrl Pts',(58.629062442157,-20.9970596244464,-55.5957578652104));
#182371=CARTESIAN_POINT('Ctrl Pts',(58.3833111942037,-20.997873466999,-55.4576663025591));
#182372=CARTESIAN_POINT('Ctrl Pts',(58.1440639002148,-20.9985364556097,
-55.3589167601806));
#182373=CARTESIAN_POINT('Ctrl Pts',(60.,-21.4835561881163,-58.1534328789326));
#182374=CARTESIAN_POINT('Ctrl Pts',(60.,-21.563522065113,-56.0718305306274));
#182375=CARTESIAN_POINT('Ctrl Pts',(58.0481390063499,-21.5914605167321,
-55.3445609916381));
#182376=CARTESIAN_POINT('Ctrl Pts',(60.,-21.2836204844253,-58.1457522408661));
#182377=CARTESIAN_POINT('Ctrl Pts',(60.,-21.3649831049967,-56.0851953591943));
#182378=CARTESIAN_POINT('Ctrl Pts',(58.0747408021896,-21.3932704964989,
-55.3468739572293));
#182379=CARTESIAN_POINT('Ctrl Pts',(60.,-21.0836896865644,-58.1378552621726));
#182380=CARTESIAN_POINT('Ctrl Pts',(59.9999999999994,-21.1653697703472,
-56.0975649789357));
#182381=CARTESIAN_POINT('Ctrl Pts',(58.1004355836544,-21.1945366814225,
-55.3490436413214));
#182382=CARTESIAN_POINT('Ctrl Pts',(60.,-20.883761812232,-58.1298294552074));
#182383=CARTESIAN_POINT('Ctrl Pts',(60.,-20.9648839320844,-56.1090266406885));
#182384=CARTESIAN_POINT('Ctrl Pts',(58.125215629935,-20.9953105578148,-55.3510803367175));
#182385=CARTESIAN_POINT('',(58.0831736435082,-21.4980516422208,-55.3542805423663));
#182386=CARTESIAN_POINT('Origin',(-8.40711756300142,-13.0336338896511,-43.9501499496686));
#182387=CARTESIAN_POINT('Ctrl Pts',(58.0831736437664,-21.4980516416407,
-55.3542805420642));
#182388=CARTESIAN_POINT('Ctrl Pts',(58.328880105512,-21.4974329387565,-55.4494594480312));
#182389=CARTESIAN_POINT('Ctrl Pts',(58.5819986525787,-21.496667325676,-55.5851943042097));
#182390=CARTESIAN_POINT('Ctrl Pts',(58.9421891742166,-21.4948870882606,
-55.8607175379279));
#182391=CARTESIAN_POINT('Ctrl Pts',(59.0588349730988,-21.4941941804047,
-55.9643994055085));
#182392=CARTESIAN_POINT('Ctrl Pts',(59.2238479950859,-21.4930296920426,
-56.1371500164854));
#182393=CARTESIAN_POINT('Ctrl Pts',(59.277189135564,-21.4926213279021,-56.1975881869849));
#182394=CARTESIAN_POINT('Ctrl Pts',(59.3540961478811,-21.4919877224573,
-56.2923012574398));
#182395=CARTESIAN_POINT('Ctrl Pts',(59.3917736538965,-21.4916657225195,
-56.3406700118079));
#182396=CARTESIAN_POINT('Ctrl Pts',(59.4342429947178,-21.4912836974144,
-56.3988037705104));
#182397=CARTESIAN_POINT('Ctrl Pts',(59.4550899460893,-21.4910914903132,
-56.4282866914381));
#182398=CARTESIAN_POINT('Ctrl Pts',(59.4639395974477,-21.4910089034144,
-56.4410102944696));
#182399=CARTESIAN_POINT('Ctrl Pts',(59.4698203457393,-21.4909538032558,
-56.4495121422603));
#182400=CARTESIAN_POINT('Ctrl Pts',(59.4735908274035,-21.4909183023144,
-56.4550001430341));
#182401=CARTESIAN_POINT('Ctrl Pts',(59.542285134935,-21.4902695208188,-56.555417590677));
#182402=CARTESIAN_POINT('Ctrl Pts',(59.6128041666099,-21.4895473392752,
-56.6706953615194));
#182403=CARTESIAN_POINT('Ctrl Pts',(59.7142648109625,-21.4882466783812,
-56.8726506836425));
#182404=CARTESIAN_POINT('Ctrl Pts',(59.7473290208614,-21.4877779516545,
-56.9447822044543));
#182405=CARTESIAN_POINT('Ctrl Pts',(59.7942525909409,-21.4870264865754,
-57.060112388415));
#182406=CARTESIAN_POINT('Ctrl Pts',(59.809446818066,-21.4867680588891,-57.0997414460801));
#182407=CARTESIAN_POINT('Ctrl Pts',(59.8313655304725,-21.486370290246,-57.1609210038875));
#182408=CARTESIAN_POINT('Ctrl Pts',(59.8421066577016,-21.4861688880082,
-57.1919444189843));
#182409=CARTESIAN_POINT('Ctrl Pts',(59.8542113411722,-21.4859300541667,
-57.2288840491873));
#182410=CARTESIAN_POINT('Ctrl Pts',(59.8601514196854,-21.4858097506293,
-57.2475383191946));
#182411=CARTESIAN_POINT('Ctrl Pts',(59.8626725113407,-21.4857580107985,
-57.2555723150833));
#182412=CARTESIAN_POINT('Ctrl Pts',(59.8643476932872,-21.4857234783297,
-57.2609370226343));
#182413=CARTESIAN_POINT('Ctrl Pts',(59.8648369543695,-21.4857133796908,
-57.2625060652884));
#182414=CARTESIAN_POINT('Ctrl Pts',(59.9413789268569,-21.4841213872645,
-57.5100727167539));
#182415=CARTESIAN_POINT('Ctrl Pts',(59.9705840598595,-21.4827732241292,
-57.7085238060111));
#182416=CARTESIAN_POINT('Ctrl Pts',(59.9999460396104,-21.4809004491039,
-58.003826414933));
#182417=CARTESIAN_POINT('Ctrl Pts',(60.,-21.4803288263114,-58.1018950252691));
#182418=CARTESIAN_POINT('Ctrl Pts',(60.,-21.48000002,-58.1532962439713));
#182419=CARTESIAN_POINT('Ctrl Pts',(60.,-21.48000002,-58.1532962439713));
#182420=CARTESIAN_POINT('Ctrl Pts',(60.,-21.98000002,-58.1532962439712));
#182421=CARTESIAN_POINT('Ctrl Pts',(59.5,-21.98000002,-58.1532962439713));
#182422=CARTESIAN_POINT('Ctrl Pts',(60.,-21.4819649551771,-57.8461243349599));
#182423=CARTESIAN_POINT('Ctrl Pts',(59.9980388947882,-21.98000002,-57.846724408982));
#182424=CARTESIAN_POINT('Ctrl Pts',(59.4999999930587,-21.98000002,-57.8972567292831));
#182425=CARTESIAN_POINT('Ctrl Pts',(59.9539303867693,-21.4838860106857,
-57.5466594347187));
#182426=CARTESIAN_POINT('Ctrl Pts',(59.9502437945621,-21.9800000199991,
-57.5478013960511));
#182427=CARTESIAN_POINT('Ctrl Pts',(59.4616086582853,-21.98000002,-57.6476410381502));
#182428=CARTESIAN_POINT('Ctrl Pts',(59.8167663234865,-21.4866995950233,
-57.1091506902012));
#182429=CARTESIAN_POINT('Ctrl Pts',(59.8105866338858,-21.9800000200004,
-57.1115394631459));
#182430=CARTESIAN_POINT('Ctrl Pts',(59.34730526825,-21.98000002,-57.282960076491));
#182431=CARTESIAN_POINT('Ctrl Pts',(59.7596240701279,-21.4876191423699,
-56.9663510387935));
#182432=CARTESIAN_POINT('Ctrl Pts',(59.7527585815745,-21.9800000200004,
-56.9693956543515));
#182433=CARTESIAN_POINT('Ctrl Pts',(59.29968672466,-21.98000002,-57.1639308209523));
#182434=CARTESIAN_POINT('Ctrl Pts',(59.6259954411174,-21.4893742131836,
-56.694110313108));
#182435=CARTESIAN_POINT('Ctrl Pts',(59.6179788443353,-21.9800000199995,
-56.6986593938776));
#182436=CARTESIAN_POINT('Ctrl Pts',(59.1883295347111,-21.98000002,-56.9370071244832));
#182437=CARTESIAN_POINT('Ctrl Pts',(59.5491776307125,-21.4902170457339,
-56.5635325439996));
#182438=CARTESIAN_POINT('Ctrl Pts',(59.5407153644089,-21.9800000200004,
-56.5688983662156));
#182439=CARTESIAN_POINT('Ctrl Pts',(59.1243146931145,-21.98000002,-56.8281652030541));
#182440=CARTESIAN_POINT('Ctrl Pts',(59.3752915646391,-21.4918319317587,
-56.3135970508604));
#182441=CARTESIAN_POINT('Ctrl Pts',(59.3661855631985,-21.9800000199995,
-56.3207427939796));
#182442=CARTESIAN_POINT('Ctrl Pts',(58.9794096363452,-21.98000002,-56.6198336495764));
#182443=CARTESIAN_POINT('Ctrl Pts',(59.2775781171727,-21.4926066631124,
-56.1938276864606));
#182444=CARTESIAN_POINT('Ctrl Pts',(59.268291108539,-21.98000002,-56.2019010018047));
#182445=CARTESIAN_POINT('Ctrl Pts',(58.897981763705,-21.98000002,-56.5200008958119));
#182446=CARTESIAN_POINT('Ctrl Pts',(59.0680465560033,-21.4940322909708,
-55.9736253396869));
#182447=CARTESIAN_POINT('Ctrl Pts',(59.058685939558,-21.98000002,-55.9835815924875));
#182448=CARTESIAN_POINT('Ctrl Pts',(58.7233721306083,-21.98000002,-56.3364530063454));
#182449=CARTESIAN_POINT('Ctrl Pts',(58.9556221515304,-21.4946900550471,
-55.8721285607086));
#182450=CARTESIAN_POINT('Ctrl Pts',(58.9463663728276,-21.98000002,-55.8830032045419));
#182451=CARTESIAN_POINT('Ctrl Pts',(58.6296851267041,-21.98000002,-56.251851153689));
#182452=CARTESIAN_POINT('Ctrl Pts',(58.5954423658223,-21.4964978360334,
-55.5933734977247));
#182453=CARTESIAN_POINT('Ctrl Pts',(58.587136508474,-21.98000002,-55.607131606824));
#182454=CARTESIAN_POINT('Ctrl Pts',(58.3295353039945,-21.98000002,-56.0194969731979));
#182455=CARTESIAN_POINT('Ctrl Pts',(58.3219561351612,-21.4974802329133,
-55.4421752934307));
#182456=CARTESIAN_POINT('Ctrl Pts',(58.3146314565664,-21.9800000200043,
-55.4574637281066));
#182457=CARTESIAN_POINT('Ctrl Pts',(58.1016300300823,-21.98000002,-55.8934667289665));
#182458=CARTESIAN_POINT('Ctrl Pts',(58.0398165251616,-21.4981583243581,
-55.3378696135325));
#182459=CARTESIAN_POINT('Ctrl Pts',(58.0337433152366,-21.98000002,-55.3542930871701));
#182460=CARTESIAN_POINT('Ctrl Pts',(57.866513770968,-21.98000002,-55.8065234638013));
#182461=CARTESIAN_POINT('',(58.1141118834537,-21.9800000069849,-55.913606468422));
#182462=CARTESIAN_POINT('Ctrl Pts',(58.0831736436236,-21.4980516422303,
-55.3542805420318));
#182463=CARTESIAN_POINT('Ctrl Pts',(58.077688301736,-21.5206990055623,-55.3530326053872));
#182464=CARTESIAN_POINT('Ctrl Pts',(58.0725563121906,-21.543329300244,-55.3536411745602));
#182465=CARTESIAN_POINT('Ctrl Pts',(58.0678467194416,-21.5655936151685,
-55.3560017266602));
#182466=CARTESIAN_POINT('Ctrl Pts',(58.0651885351446,-21.5781600206881,
-55.3573340674503));
#182467=CARTESIAN_POINT('Ctrl Pts',(58.0626646730493,-21.5906101815618,
-55.3592237425858));
#182468=CARTESIAN_POINT('Ctrl Pts',(58.0602853929275,-21.6028853626772,
-55.3616460932885));
#182469=CARTESIAN_POINT('Ctrl Pts',(58.0581274670246,-21.6140185331889,
-55.363843082739));
#182470=CARTESIAN_POINT('Ctrl Pts',(58.0561201685456,-21.6248395435586,
-55.3664403549057));
#182471=CARTESIAN_POINT('Ctrl Pts',(58.0542338762529,-21.6354769720973,
-55.3694355679586));
#182472=CARTESIAN_POINT('Ctrl Pts',(58.0523609362085,-21.646039102874,-55.3724095791921));
#182473=CARTESIAN_POINT('Ctrl Pts',(58.0506071882539,-21.6564208249666,
-55.3757761530634));
#182474=CARTESIAN_POINT('Ctrl Pts',(58.0489554951375,-21.6667374214667,
-55.3795809979916));
#182475=CARTESIAN_POINT('Ctrl Pts',(58.0477878397693,-21.6740306826454,
-55.3822708121959));
#182476=CARTESIAN_POINT('Ctrl Pts',(58.0466714218907,-21.6812912032906,
-55.3851806278496));
#182477=CARTESIAN_POINT('Ctrl Pts',(58.0456043472203,-21.6885540001523,
-55.3883406910768));
#182478=CARTESIAN_POINT('Ctrl Pts',(58.0450552768195,-21.6922911208005,
-55.3899667227229));
#182479=CARTESIAN_POINT('Ctrl Pts',(58.0445190796661,-21.6960309511488,
-55.3916600870712));
#182480=CARTESIAN_POINT('Ctrl Pts',(58.0439958538933,-21.6997781149038,
-55.3934253930027));
#182481=CARTESIAN_POINT('Ctrl Pts',(58.041921572838,-21.7146334052805,-55.400423788037));
#182482=CARTESIAN_POINT('Ctrl Pts',(58.0401111928462,-21.7292088227908,
-55.4083741119359));
#182483=CARTESIAN_POINT('Ctrl Pts',(58.0386022975759,-21.7433237632393,
-55.4171742771625));
#182484=CARTESIAN_POINT('Ctrl Pts',(58.0370898725513,-21.757471722728,-55.4259950285905));
#182485=CARTESIAN_POINT('Ctrl Pts',(58.0358805473388,-21.7711563450861,
-55.4356690560707));
#182486=CARTESIAN_POINT('Ctrl Pts',(58.0349963567716,-21.7842200732956,
-55.4460497826742));
#182487=CARTESIAN_POINT('Ctrl Pts',(58.0341155424912,-21.7972339175853,
-55.4563908704147));
#182488=CARTESIAN_POINT('Ctrl Pts',(58.0335575229446,-21.8096310261443,
-55.4674326276423));
#182489=CARTESIAN_POINT('Ctrl Pts',(58.0333258610528,-21.8212893245516,
-55.4789957790404));
#182490=CARTESIAN_POINT('Ctrl Pts',(58.0331490294813,-21.830188307514,-55.4878221346276));
#182491=CARTESIAN_POINT('Ctrl Pts',(58.0331619852258,-21.838657468733,-55.4969515115536));
#182492=CARTESIAN_POINT('Ctrl Pts',(58.0333585110965,-21.8466585948979,
-55.5062941612126));
#182493=CARTESIAN_POINT('Ctrl Pts',(58.0334888523122,-21.8519651558504,
-55.5124904564405));
#182494=CARTESIAN_POINT('Ctrl Pts',(58.0337006581951,-21.8570756893028,
-55.5187903954443));
#182495=CARTESIAN_POINT('Ctrl Pts',(58.0339893274825,-21.861986887608,-55.5251637203642));
#182496=CARTESIAN_POINT('Ctrl Pts',(58.0350033551333,-21.8792387779142,
-55.5475517192948));
#182497=CARTESIAN_POINT('Ctrl Pts',(58.0370308035539,-21.8947384255673,
-55.5717746381603));
#182498=CARTESIAN_POINT('Ctrl Pts',(58.0400916132891,-21.9083235411587,
-55.5973841240798));
#182499=CARTESIAN_POINT('Ctrl Pts',(58.0407096798096,-21.9110667711702,
-55.6025554242342));
#182500=CARTESIAN_POINT('Ctrl Pts',(58.041369802248,-21.9137320745735,-55.6077832055866));
#182501=CARTESIAN_POINT('Ctrl Pts',(58.0420720205664,-21.9163183295388,
-55.6130637074408));
#182502=CARTESIAN_POINT('Ctrl Pts',(58.0441619042696,-21.9240153262748,
-55.6287790974864));
#182503=CARTESIAN_POINT('Ctrl Pts',(58.0466233370326,-21.9310133400415,
-55.6449634250592));
#182504=CARTESIAN_POINT('Ctrl Pts',(58.0494650175479,-21.9372880694643,
-55.6615286492183));
#182505=CARTESIAN_POINT('Ctrl Pts',(58.0505762686844,-21.9397418288384,
-55.6680065499095));
#182506=CARTESIAN_POINT('Ctrl Pts',(58.0517907300022,-21.9421772063289,
-55.6747968723622));
#182507=CARTESIAN_POINT('Ctrl Pts',(58.0530602395296,-21.9444746087411,
-55.6815997527206));
#182508=CARTESIAN_POINT('Ctrl Pts',(58.0535478411702,-21.9453570102994,
-55.6842126481357));
#182509=CARTESIAN_POINT('Ctrl Pts',(58.0540433298046,-21.9462194821836,
-55.6868271396655));
#182510=CARTESIAN_POINT('Ctrl Pts',(58.05454309135,-21.9470568630598,-55.6894253280722));
#182511=CARTESIAN_POINT('Ctrl Pts',(58.0559071998638,-21.9493425098708,
-55.6965171320703));
#182512=CARTESIAN_POINT('Ctrl Pts',(58.0573071807538,-21.9514417852041,
-55.7034977235522));
#182513=CARTESIAN_POINT('Ctrl Pts',(58.0586499612016,-21.9532837016386,
-55.709985247384));
#182514=CARTESIAN_POINT('Ctrl Pts',(58.0588097209061,-21.9535028469396,
-55.7107571121312));
#182515=CARTESIAN_POINT('Ctrl Pts',(58.0589686435043,-21.95371839633,-55.7115219721044));
#182516=CARTESIAN_POINT('Ctrl Pts',(58.0591265512438,-21.9539302663629,
-55.7122791654125));
#182517=CARTESIAN_POINT('Ctrl Pts',(58.0650058136374,-21.9618186670249,
-55.7404711853563));
#182518=CARTESIAN_POINT('Ctrl Pts',(58.0720079755593,-21.9679281060019,
-55.7699383340652));
#182519=CARTESIAN_POINT('Ctrl Pts',(58.0801172540501,-21.9722379734285,
-55.8003568758901));
#182520=CARTESIAN_POINT('Ctrl Pts',(58.0886478415444,-21.9767717554675,
-55.8323557809448));
#182521=CARTESIAN_POINT('Ctrl Pts',(58.098403737083,-21.9793141024895,-55.8654069450485));
#182522=CARTESIAN_POINT('Ctrl Pts',(58.1093418112629,-21.9798788055287,
-55.8990986009792));
#182523=CARTESIAN_POINT('Ctrl Pts',(58.1109077045422,-21.9799596483424,
-55.9039218940676));
#182524=CARTESIAN_POINT('Ctrl Pts',(58.112497784602,-21.98000002,-55.9087582670901));
#182525=CARTESIAN_POINT('Ctrl Pts',(58.1141118834575,-21.98000002,-55.9136064684135));
#182526=CARTESIAN_POINT('Ctrl Pts',(59.5,-21.98000002,-58.1532962439713));
#182527=CARTESIAN_POINT('Ctrl Pts',(59.5,-21.98000002,-57.9611810443397));
#182528=CARTESIAN_POINT('Ctrl Pts',(59.4783898617073,-21.9800000201789,
-57.7727385086976));
#182529=CARTESIAN_POINT('Ctrl Pts',(59.4354406742177,-21.9800000198205,
-57.5879375289838));
#182530=CARTESIAN_POINT('Ctrl Pts',(59.4262406555719,-21.9800000197437,
-57.5483518567391));
#182531=CARTESIAN_POINT('Ctrl Pts',(59.4160613127747,-21.9800000196281,
-57.5089332628385));
#182532=CARTESIAN_POINT('Ctrl Pts',(59.4049049949538,-21.9800000194259,
-57.469681421663));
#182533=CARTESIAN_POINT('Ctrl Pts',(59.3987196130206,-21.9800000193138,
-57.4479190773891));
#182534=CARTESIAN_POINT('Ctrl Pts',(59.3922287663824,-21.9800000192153,
-57.4261931844644));
#182535=CARTESIAN_POINT('Ctrl Pts',(59.3854342581924,-21.9800000191476,
-57.4045116647966));
#182536=CARTESIAN_POINT('Ctrl Pts',(59.3665370601269,-21.9800000189591,
-57.3442100270521));
#182537=CARTESIAN_POINT('Ctrl Pts',(59.3452714576316,-21.9800000190536,
-57.284476265955));
#182538=CARTESIAN_POINT('Ctrl Pts',(59.3218795388586,-21.9800000193212,
-57.2258422130816));
#182539=CARTESIAN_POINT('Ctrl Pts',(59.3106878533866,-21.9800000194493,
-57.1977891968211));
#182540=CARTESIAN_POINT('Ctrl Pts',(59.2990101624397,-21.9800000196077,
-57.1699876439614));
#182541=CARTESIAN_POINT('Ctrl Pts',(59.2868766202345,-21.9800000197421,
-57.1424936459686));
#182542=CARTESIAN_POINT('Ctrl Pts',(59.2731919149499,-21.9800000198936,
-57.1114847902475));
#182543=CARTESIAN_POINT('Ctrl Pts',(59.2588942022727,-21.9800000199412,
-57.0807856309711));
#182544=CARTESIAN_POINT('Ctrl Pts',(59.2440132425671,-21.9800000199676,
-57.0504664636976));
#182545=CARTESIAN_POINT('Ctrl Pts',(59.2100364625766,-21.9800000200278,
-56.9812405739477));
#182546=CARTESIAN_POINT('Ctrl Pts',(59.1729132668609,-21.9800000200007,
-56.9136446874669));
#182547=CARTESIAN_POINT('Ctrl Pts',(59.1326772603373,-21.9800000199982,
-56.8478208127119));
#182548=CARTESIAN_POINT('Ctrl Pts',(59.1305108981501,-21.9800000199981,
-56.8442767643431));
#182549=CARTESIAN_POINT('Ctrl Pts',(59.1283355234418,-21.9800000199979,
-56.840737847095));
#182550=CARTESIAN_POINT('Ctrl Pts',(59.1261511452891,-21.9800000199978,
-56.8372040811614));
#182551=CARTESIAN_POINT('Ctrl Pts',(59.1024586951324,-21.980000019996,-56.7988757481558));
#182552=CARTESIAN_POINT('Ctrl Pts',(59.0776978833329,-21.9800000199944,
-56.7611395583364));
#182553=CARTESIAN_POINT('Ctrl Pts',(59.051864196737,-21.9800000199939,-56.7239980129522));
#182554=CARTESIAN_POINT('Ctrl Pts',(58.9794118018617,-21.9800000199925,
-56.6198319311016));
#182555=CARTESIAN_POINT('Ctrl Pts',(58.897983005211,-21.9800000199984,-56.5200000236488));
#182556=CARTESIAN_POINT('Ctrl Pts',(58.8106774361301,-21.9800000199995,
-56.4282264859168));
#182557=CARTESIAN_POINT('Ctrl Pts',(58.7700668687888,-21.9800000200001,
-56.385537623414));
#182558=CARTESIAN_POINT('Ctrl Pts',(58.7280754192644,-21.98000002,-56.3444004714051));
#182559=CARTESIAN_POINT('Ctrl Pts',(58.6847050658881,-21.98000002,-56.3048126520436));
#182560=CARTESIAN_POINT('Ctrl Pts',(58.6494885520049,-21.98000002,-56.2726675371986));
#182561=CARTESIAN_POINT('Ctrl Pts',(58.6132573779996,-21.98000002,-56.2414509676764));
#182562=CARTESIAN_POINT('Ctrl Pts',(58.5760924793011,-21.98000002,-56.2112492084261));
#182563=CARTESIAN_POINT('Ctrl Pts',(58.5607621926364,-21.98000002,-56.1987911729328));
#182564=CARTESIAN_POINT('Ctrl Pts',(58.5452724940628,-21.98000002,-56.1865050278662));
#182565=CARTESIAN_POINT('Ctrl Pts',(58.5296351858009,-21.98000002,-56.174399760192));
#182566=CARTESIAN_POINT('Ctrl Pts',(58.50318856599,-21.98000002,-56.1539267090422));
#182567=CARTESIAN_POINT('Ctrl Pts',(58.4762743935287,-21.98000002,-56.1339724230775));
#182568=CARTESIAN_POINT('Ctrl Pts',(58.4489601509993,-21.98000002,-56.1145700874369));
#182569=CARTESIAN_POINT('Ctrl Pts',(58.3958489442448,-21.98000002,-56.0768431961047));
#182570=CARTESIAN_POINT('Ctrl Pts',(58.3412467373532,-21.9800000154289,
-56.0410944834472));
#182571=CARTESIAN_POINT('Ctrl Pts',(58.2853645640813,-21.9799999916842,
-56.0075334770553));
#182572=CARTESIAN_POINT('Ctrl Pts',(58.2574234774454,-21.9799999798118,
-55.9907529738594));
#182573=CARTESIAN_POINT('Ctrl Pts',(58.2291619777336,-21.9799999666902,
-55.9745206253323));
#182574=CARTESIAN_POINT('Ctrl Pts',(58.2006099144576,-21.9799999607144,
-55.95885870079));
#182575=CARTESIAN_POINT('Ctrl Pts',(58.1720578511817,-21.9799999547386,
-55.9431967762476));
#182576=CARTESIAN_POINT('Ctrl Pts',(58.1432152243425,-21.9799999567774,
-55.9281052756887));
#182577=CARTESIAN_POINT('Ctrl Pts',(58.1141118834472,-21.9799999679397,
-55.9136064684357));
#182578=CARTESIAN_POINT('Origin',(-83.2809572255632,-21.9800000199999,-55.24995));
#182579=CARTESIAN_POINT('',(58.1141118834647,-21.98000002,-60.42825533736));
#182580=CARTESIAN_POINT('',(58.1141118834647,-21.98000002,-55.24995));
#182581=CARTESIAN_POINT('Origin',(55.9860799622262,-21.98000002,-60.2945890942193));
#182582=CARTESIAN_POINT('Ctrl Pts',(58.1141118834647,-21.98000002,-60.42825533736));
#182583=CARTESIAN_POINT('Ctrl Pts',(57.6893011240826,-21.98000002,-60.42825533736));
#182584=CARTESIAN_POINT('Ctrl Pts',(57.6206785412152,-22.3992316056509,
-60.42825533736));
#182585=CARTESIAN_POINT('Ctrl Pts',(58.1141118664761,-21.98000002,-60.6472062522327));
#182586=CARTESIAN_POINT('Ctrl Pts',(57.6893011111963,-21.9800000199989,
-60.5843987403017));
#182587=CARTESIAN_POINT('Ctrl Pts',(57.6206785407758,-22.3992316083349,
-60.574219492927));
#182588=CARTESIAN_POINT('Ctrl Pts',(58.0662048046675,-21.98000002,-60.8621882839625));
#182589=CARTESIAN_POINT('Ctrl Pts',(57.6525421683829,-21.98000002,-60.7382102053579));
#182590=CARTESIAN_POINT('Ctrl Pts',(57.5883338458808,-22.4017068994087,
-60.7175481239357));
#182591=CARTESIAN_POINT('Ctrl Pts',(57.9716987024741,-21.98000002,-61.0621827299711));
#182592=CARTESIAN_POINT('Ctrl Pts',(57.5817506954797,-21.98000002,-60.8779152752782));
#182593=CARTESIAN_POINT('Ctrl Pts',(57.5245249214072,-22.4066238608121,
-60.8508735991007));
#182594=CARTESIAN_POINT('',(57.6206785412152,-22.3992316056509,-60.42825533736));
#182595=CARTESIAN_POINT('Origin',(58.1141118834647,-22.48000002,-60.42825533736));
#182596=CARTESIAN_POINT('Origin',(56.1878807306156,-22.5096307883003,-60.3396608599486));
#182597=CARTESIAN_POINT('Origin',(0.,-12.9675000200281,-60.64995));
#182598=CARTESIAN_POINT('Origin',(0.,-12.9675000200281,-60.8508735991007));
#182599=CARTESIAN_POINT('Origin',(-83.2809572255632,-28.6300000199999,-55.24995));
#182600=CARTESIAN_POINT('',(56.9019881023868,-28.63000002,-60.42825533736));
#182601=CARTESIAN_POINT('Origin',(55.4600042524515,-28.6300004012302,-60.4518437845562));
#182602=CARTESIAN_POINT('',(56.9019881023868,-28.63000002,-55.74995));
#182603=CARTESIAN_POINT('',(56.9019881023868,-28.63000002,-55.24995));
#182604=CARTESIAN_POINT('',(-83.2809572255632,-28.6300000199999,-55.74995));
#182605=CARTESIAN_POINT('Ctrl Pts',(56.7267007677588,-28.6300000101017,
-61.1208879979441));
#182606=CARTESIAN_POINT('Ctrl Pts',(56.1708458184293,-28.6301256542592,
-60.8213741500007));
#182607=CARTESIAN_POINT('Ctrl Pts',(56.2981381510249,-28.0154717851087,
-60.8899762078857));
#182608=CARTESIAN_POINT('Ctrl Pts',(56.8517546922174,-28.6300000099381,
-60.8884604222472));
#182609=CARTESIAN_POINT('Ctrl Pts',(56.231166166104,-28.630129440528,-60.6796100628425));
#182610=CARTESIAN_POINT('Ctrl Pts',(56.3842107337159,-28.0053123694987,
-60.7350480688662));
#182611=CARTESIAN_POINT('Ctrl Pts',(56.9126898510831,-28.630000009859,-60.6288526395369));
#182612=CARTESIAN_POINT('Ctrl Pts',(56.2556311178187,-28.6301313253205,
-60.5386217481864));
#182613=CARTESIAN_POINT('Ctrl Pts',(56.4261416440025,-28.000404297649,-60.56196856935));
#182614=CARTESIAN_POINT('Ctrl Pts',(56.900577244494,-28.6300000098748,-60.3616165536491));
#182615=CARTESIAN_POINT('Ctrl Pts',(56.25064863923,-28.6301309522558,-60.3916281028846));
#182616=CARTESIAN_POINT('Ctrl Pts',(56.4178064988839,-28.0013806349218,
-60.3838347631882));
#182617=CARTESIAN_POINT('',(56.418846619879,-28.001258776103,-60.42825533736));
#182618=CARTESIAN_POINT('Origin',(55.0583726900799,-28.1617123603415,-60.3669939749617));
#182619=CARTESIAN_POINT('Origin',(56.9019881023868,-28.13000002,-60.42825533736));
#182620=CARTESIAN_POINT('Origin',(-83.2809572255632,-29.13000002,-55.74995));
#182621=CARTESIAN_POINT('',(56.6260651114328,-29.13000002,-55.24995));
#182622=CARTESIAN_POINT('Ctrl Pts',(56.9019881023868,-28.63000002,-55.74995));
#182623=CARTESIAN_POINT('Ctrl Pts',(56.9019881023868,-28.63000002,-55.7252977300075));
#182624=CARTESIAN_POINT('Ctrl Pts',(56.9009624215127,-28.6318266319377,
-55.7004051558798));
#182625=CARTESIAN_POINT('Ctrl Pts',(56.8989110597644,-28.6355653333565,
-55.6755568508274));
#182626=CARTESIAN_POINT('Ctrl Pts',(56.8968844354924,-28.6392589495835,
-55.6510081927576));
#182627=CARTESIAN_POINT('Ctrl Pts',(56.8938567186674,-28.6448191959989,
-55.6265031833395));
#182628=CARTESIAN_POINT('Ctrl Pts',(56.8898279092893,-28.6522850499302,
-55.6023410322127));
#182629=CARTESIAN_POINT('Ctrl Pts',(56.8858213427979,-28.6597096851966,
-55.5783122793039));
#182630=CARTESIAN_POINT('Ctrl Pts',(56.8808247072189,-28.6690193040358,
-55.5546231087945));
#182631=CARTESIAN_POINT('Ctrl Pts',(56.8748380025521,-28.6802034444929,
-55.5315855325101));
#182632=CARTESIAN_POINT('Ctrl Pts',(56.8688512978853,-28.6913875849501,
-55.5085479562256));
#182633=CARTESIAN_POINT('Ctrl Pts',(56.8618745241307,-28.7044465800051,
-55.4861625569417));
#182634=CARTESIAN_POINT('Ctrl Pts',(56.8539076812883,-28.71931576493,-55.4647510472712));
#182635=CARTESIAN_POINT('Ctrl Pts',(56.8485654122774,-28.7292864882659,
-55.4503932838693));
#182636=CARTESIAN_POINT('Ctrl Pts',(56.8427779541822,-28.7400700413755,
-55.436473634921));
#182637=CARTESIAN_POINT('Ctrl Pts',(56.8365453070028,-28.7516322157917,
-55.4230894720395));
#182638=CARTESIAN_POINT('Ctrl Pts',(56.8334289834131,-28.7574133029998,
-55.4163973905988));
#182639=CARTESIAN_POINT('Ctrl Pts',(56.8302013625523,-28.7633889371214,
-55.4098390835444));
#182640=CARTESIAN_POINT('Ctrl Pts',(56.8268624444205,-28.7695536079699,
-55.4034267193179));
#182641=CARTESIAN_POINT('Ctrl Pts',(56.8251929853546,-28.7726359433942,
-55.4002205372046));
#182642=CARTESIAN_POINT('Ctrl Pts',(56.8234957019709,-28.77576552988,-55.3970508341267));
#182643=CARTESIAN_POINT('Ctrl Pts',(56.8217705942694,-28.7789416179907,
-55.3939191047413));
#182644=CARTESIAN_POINT('Ctrl Pts',(56.8207703368452,-28.7807831874823,
-55.3921032554666));
#182645=CARTESIAN_POINT('Ctrl Pts',(56.8195504803749,-28.783019971304,-55.3899329326252));
#182646=CARTESIAN_POINT('Ctrl Pts',(56.8184767390232,-28.7849946292223,
-55.3880504554654));
#182647=CARTESIAN_POINT('Ctrl Pts',(56.8176986376089,-28.7864255921973,
-55.3866862925428));
#182648=CARTESIAN_POINT('Ctrl Pts',(56.8169972667262,-28.787717598042,-55.3854719748343));
#182649=CARTESIAN_POINT('Ctrl Pts',(56.8165117982118,-28.7886085997452,
-55.3846393128084));
#182650=CARTESIAN_POINT('Ctrl Pts',(56.8105283129488,-28.7995903532519,
-55.3743766061371));
#182651=CARTESIAN_POINT('Ctrl Pts',(56.8038505141232,-28.8116563698921,
-55.3640262829591));
#182652=CARTESIAN_POINT('Ctrl Pts',(56.7964784017351,-28.8249085696917,
-55.3538197096297));
#182653=CARTESIAN_POINT('Ctrl Pts',(56.789362571463,-28.8377000736109,-55.343967954848));
#182654=CARTESIAN_POINT('Ctrl Pts',(56.7815998623955,-28.8515974361167,
-55.3342503317759));
#182655=CARTESIAN_POINT('Ctrl Pts',(56.7731902745328,-28.8666658348978,
-55.3249145815269));
#182656=CARTESIAN_POINT('Ctrl Pts',(56.765061435188,-28.8812311851711,-55.3158904991135));
#182657=CARTESIAN_POINT('Ctrl Pts',(56.7563281873323,-28.8968913261992,
-55.3072235542836));
#182658=CARTESIAN_POINT('Ctrl Pts',(56.7469905309656,-28.9136701987031,
-55.2991713310086));
#182659=CARTESIAN_POINT('Ctrl Pts',(56.7380901202547,-28.929663382719,-55.2914961616225));
#182660=CARTESIAN_POINT('Ctrl Pts',(56.7286405798967,-28.9466733880094,
-55.2843799874074));
#182661=CARTESIAN_POINT('Ctrl Pts',(56.7186419098915,-28.96468138259,-55.2780710450498));
#182662=CARTESIAN_POINT('Ctrl Pts',(56.7088984654859,-28.9822297059132,
-55.2719231444702));
#182663=CARTESIAN_POINT('Ctrl Pts',(56.6986335677516,-29.0007261634318,
-55.266542291755));
#182664=CARTESIAN_POINT('Ctrl Pts',(56.6878472166885,-29.0201084881562,
-55.2621756144189));
#182665=CARTESIAN_POINT('Ctrl Pts',(56.67746927325,-29.0387569327062,-55.2579742742118));
#182666=CARTESIAN_POINT('Ctrl Pts',(56.6666086168719,-29.0582256425946,
-55.2547123448343));
#182667=CARTESIAN_POINT('Ctrl Pts',(56.6552652475542,-29.0784125612096,
-55.2526183861893));
#182668=CARTESIAN_POINT('Ctrl Pts',(56.6458634762107,-29.0951441678102,
-55.2508828418522));
#182669=CARTESIAN_POINT('Ctrl Pts',(56.6361300975035,-29.1123684482571,
-55.24995));
#182670=CARTESIAN_POINT('Ctrl Pts',(56.6260651114328,-29.13000002,-55.24995));
#182671=CARTESIAN_POINT('',(60.,-29.13000002,-55.24995));
#182672=CARTESIAN_POINT('Origin',(60.,28.41999998,-55.24995));
#182673=CARTESIAN_POINT('',(56.4809591809864,-29.63000002,-55.24995));
#182674=CARTESIAN_POINT('Origin',(0.,-12.9675000200281,-55.24995));
#182675=CARTESIAN_POINT('',(60.,-29.63000002,-55.24995));
#182676=CARTESIAN_POINT('Origin',(60.,-29.63000002,-55.74995));
#182677=CARTESIAN_POINT('',(56.1762739063771,-30.13000002,-55.74995));
#182678=CARTESIAN_POINT('Ctrl Pts',(56.4809591809864,-29.63000002,-55.24995));
#182679=CARTESIAN_POINT('Ctrl Pts',(56.4715391886809,-29.6459655172457,
-55.24995));
#182680=CARTESIAN_POINT('Ctrl Pts',(56.462662754235,-29.660958555519,-55.2507099202142));
#182681=CARTESIAN_POINT('Ctrl Pts',(56.454349949937,-29.6749641824274,-55.2519734860076));
#182682=CARTESIAN_POINT('Ctrl Pts',(56.4445637737142,-29.6914521843244,
-55.253461007797));
#182683=CARTESIAN_POINT('Ctrl Pts',(56.435554593509,-29.7065787354348,-55.2556468104043));
#182684=CARTESIAN_POINT('Ctrl Pts',(56.4273466888451,-29.7203275029284,
-55.2581719078906));
#182685=CARTESIAN_POINT('Ctrl Pts',(56.422431254882,-29.7285611705276,-55.2596841025922));
#182686=CARTESIAN_POINT('Ctrl Pts',(56.4178030918222,-29.7363007600898,
-55.2613190749055));
#182687=CARTESIAN_POINT('Ctrl Pts',(56.4134686415036,-29.7435398696061,
-55.2630072596282));
#182688=CARTESIAN_POINT('Ctrl Pts',(56.4084051403986,-29.7519965910681,
-55.2649793955578));
#182689=CARTESIAN_POINT('Ctrl Pts',(56.4037382707669,-29.7597773623134,
-55.267025073771));
#182690=CARTESIAN_POINT('Ctrl Pts',(56.3994596075599,-29.7669020737305,
-55.2690538840585));
#182691=CARTESIAN_POINT('Ctrl Pts',(56.395622622375,-29.7732913151433,-55.2708732642339));
#182692=CARTESIAN_POINT('Ctrl Pts',(56.3920987368373,-29.7791514240126,
-55.2726789076247));
#182693=CARTESIAN_POINT('Ctrl Pts',(56.3888834537717,-29.7844933511438,
-55.2744148706152));
#182694=CARTESIAN_POINT('Ctrl Pts',(56.3856587578915,-29.7898509168888,
-55.2761559156769));
#182695=CARTESIAN_POINT('Ctrl Pts',(56.3827332174854,-29.7946845005768,
-55.2778259230685));
#182696=CARTESIAN_POINT('Ctrl Pts',(56.3801058680076,-29.7990071903381,
-55.2793787374307));
#182697=CARTESIAN_POINT('Ctrl Pts',(56.3787921932687,-29.8011685352187,
-55.2801551446118));
#182698=CARTESIAN_POINT('Ctrl Pts',(56.3775562038427,-29.8032029432388,
-55.2809026966681));
#182699=CARTESIAN_POINT('Ctrl Pts',(56.3763978997437,-29.8051120362293,
-55.2816166210347));
#182700=CARTESIAN_POINT('Ctrl Pts',(56.3758187476942,-29.8060665827245,
-55.2819735832181));
#182701=CARTESIAN_POINT('Ctrl Pts',(56.3752590169764,-29.8069897973416,
-55.2823221473967));
#182702=CARTESIAN_POINT('Ctrl Pts',(56.3747187075913,-29.807881865021,-55.282661770634));
#182703=CARTESIAN_POINT('Ctrl Pts',(56.3744485528987,-29.8083278988607,
-55.2828315822527));
#182704=CARTESIAN_POINT('Ctrl Pts',(56.3743666403179,-29.8084621276635,
-55.2828830019629));
#182705=CARTESIAN_POINT('Ctrl Pts',(56.3741978897377,-29.8087407981391,
-55.2829896821112));
#182706=CARTESIAN_POINT('Ctrl Pts',(56.3740291391576,-29.8090194686147,
-55.2830963622595));
#182707=CARTESIAN_POINT('Ctrl Pts',(56.37377355065,-29.8094427998715,-55.2832577411222));
#182708=CARTESIAN_POINT('Ctrl Pts',(56.3731560434326,-29.8104648021674,
-55.2836533109053));
#182709=CARTESIAN_POINT('Ctrl Pts',(56.3716295461241,-29.8129912240618,
-55.2846311718795));
#182710=CARTESIAN_POINT('Ctrl Pts',(56.3701127933845,-29.8155010721099,
-55.285626187063));
#182711=CARTESIAN_POINT('Ctrl Pts',(56.3686057879999,-29.817994256596,-55.2866378253316));
#182712=CARTESIAN_POINT('Ctrl Pts',(56.3569538600269,-29.8372711658571,
-55.2944596528853));
#182713=CARTESIAN_POINT('Ctrl Pts',(56.3459518915256,-29.8554415567586,
-55.3032348643387));
#182714=CARTESIAN_POINT('Ctrl Pts',(56.3355845836553,-29.8725024376886,
-55.3126982643438));
#182715=CARTESIAN_POINT('Ctrl Pts',(56.3299355776219,-29.8817986812761,
-55.3178547431901));
#182716=CARTESIAN_POINT('Ctrl Pts',(56.3244746239002,-29.890766138149,-55.3232161626166));
#182717=CARTESIAN_POINT('Ctrl Pts',(56.3191967850647,-29.8994084321092,
-55.3287439230168));
#182718=CARTESIAN_POINT('Ctrl Pts',(56.311088424142,-29.9126856163533,-55.3372362392501));
#182719=CARTESIAN_POINT('Ctrl Pts',(56.3034308285875,-29.9251885096071,
-55.3461168072432));
#182720=CARTESIAN_POINT('Ctrl Pts',(56.2962223827156,-29.9369337314948,
-55.3552490742658));
#182721=CARTESIAN_POINT('Ctrl Pts',(56.2908160483117,-29.9457426479105,
-55.3620982745327));
#182722=CARTESIAN_POINT('Ctrl Pts',(56.2856621173763,-29.9541257111972,
-55.3690893077384));
#182723=CARTESIAN_POINT('Ctrl Pts',(56.2807554399466,-29.9620950592301,
-55.3761691040139));
#182724=CARTESIAN_POINT('Ctrl Pts',(56.2797154356931,-29.963784217723,-55.3776697158528));
#182725=CARTESIAN_POINT('Ctrl Pts',(56.2788888440829,-29.9651263359666,
-55.3788776896832));
#182726=CARTESIAN_POINT('Ctrl Pts',(56.2778887710329,-29.96674961639,-55.3803565877314));
#182727=CARTESIAN_POINT('Ctrl Pts',(56.2773160826108,-29.9676791823895,
-55.3812034736561));
#182728=CARTESIAN_POINT('Ctrl Pts',(56.276686724301,-29.9687005704798,-55.3821396856299));
#182729=CARTESIAN_POINT('Ctrl Pts',(56.2759307274251,-29.9699271388893,
-55.3832767047358));
#182730=CARTESIAN_POINT('Ctrl Pts',(56.273906754129,-29.9732109377857,-55.3863207600499));
#182731=CARTESIAN_POINT('Ctrl Pts',(56.2719114898357,-29.9764461032282,
-55.3894018338609));
#182732=CARTESIAN_POINT('Ctrl Pts',(56.2699450791873,-29.9796325533428,
-55.3925187595796));
#182733=CARTESIAN_POINT('Ctrl Pts',(56.2599035103954,-29.995904311256,-55.4084354878831));
#182734=CARTESIAN_POINT('Ctrl Pts',(56.2506758252138,-30.010814772085,-55.4252755403774));
#182735=CARTESIAN_POINT('Ctrl Pts',(56.2422529089667,-30.0243957048183,
-55.4428177801253));
#182736=CARTESIAN_POINT('Ctrl Pts',(56.2333441945075,-30.0387599283557,
-55.4613717821245));
#182737=CARTESIAN_POINT('Ctrl Pts',(56.2253354486514,-30.0516372998195,
-55.4807116725759));
#182738=CARTESIAN_POINT('Ctrl Pts',(56.2182201680098,-30.0630550384973,
-55.5006334806367));
#182739=CARTESIAN_POINT('Ctrl Pts',(56.2149590325741,-30.068288112788,-55.5097642117323));
#182740=CARTESIAN_POINT('Ctrl Pts',(56.2118856697234,-30.0732143865641,
-55.5190179172689));
#182741=CARTESIAN_POINT('Ctrl Pts',(56.2090000040314,-30.0778354020999,
-55.5283783295249));
#182742=CARTESIAN_POINT('Ctrl Pts',(56.2022281272477,-30.0886796755407,
-55.5503446850238));
#182743=CARTESIAN_POINT('Ctrl Pts',(56.1964989578389,-30.097829016622,-55.5728762690722));
#182744=CARTESIAN_POINT('Ctrl Pts',(56.1918296761308,-30.1052731127711,
-55.5956766399725));
#182745=CARTESIAN_POINT('Ctrl Pts',(56.1889265498164,-30.1099014802093,
-55.6098527725933));
#182746=CARTESIAN_POINT('Ctrl Pts',(56.1864326699304,-30.1138713642342,
-55.624133303115));
#182747=CARTESIAN_POINT('Ctrl Pts',(56.1843473599668,-30.117187484339,-55.6384523996636));
#182748=CARTESIAN_POINT('Ctrl Pts',(56.1813648251625,-30.1219303972874,
-55.6589324264064));
#182749=CARTESIAN_POINT('Ctrl Pts',(56.1792205673271,-30.1253320589938,
-55.6794841526094));
#182750=CARTESIAN_POINT('Ctrl Pts',(56.1778972989043,-30.1274293092601,
-55.6998970462423));
#182751=CARTESIAN_POINT('Ctrl Pts',(56.1768073239574,-30.1291568123186,
-55.7167111273986));
#182752=CARTESIAN_POINT('Ctrl Pts',(56.1762739063772,-30.1300000200003,
-55.7334312082419));
#182753=CARTESIAN_POINT('Ctrl Pts',(56.1762739063772,-30.1300000200003,
-55.74995));
#182754=CARTESIAN_POINT('',(-83.2809572255632,-30.13000002,-55.74995));
#182755=CARTESIAN_POINT('Origin',(-83.2809572255632,-30.13000002,-55.24995));
#182756=CARTESIAN_POINT('',(56.1762739063772,-30.13000002,-60.42825533736));
#182757=CARTESIAN_POINT('',(56.1762739063772,-30.13000002,-55.24995));
#182758=CARTESIAN_POINT('Origin',(54.6965997032562,-30.1299997573523,-60.4472632078221));
#182759=CARTESIAN_POINT('Ctrl Pts',(56.174853661752,-30.1300000267474,-60.3623460050376));
#182760=CARTESIAN_POINT('Ctrl Pts',(55.8081167820838,-30.1299397177969,
-60.3792327034747));
#182761=CARTESIAN_POINT('Ctrl Pts',(55.6982488612463,-30.4801711525811,
-60.3843213671005));
#182762=CARTESIAN_POINT('Ctrl Pts',(56.1868831687146,-30.1300000267259,
-60.6263466339185));
#182763=CARTESIAN_POINT('Ctrl Pts',(55.8181378939596,-30.1299399603517,
-60.5754394884542));
#182764=CARTESIAN_POINT('Ctrl Pts',(55.7066195808876,-30.47905606799,-60.5602959714918));
#182765=CARTESIAN_POINT('Ctrl Pts',(56.1265462537083,-30.1300000268336,
-60.886588202509));
#182766=CARTESIAN_POINT('Ctrl Pts',(55.7674480546492,-30.1299387371113,
-60.7710090719053));
#182767=CARTESIAN_POINT('Ctrl Pts',(55.6646352974887,-30.4846448609915,
-60.733808800051));
#182768=CARTESIAN_POINT('Ctrl Pts',(55.9983862620518,-30.1300000270643,
-61.1214514057001));
#182769=CARTESIAN_POINT('Ctrl Pts',(55.6644710959106,-30.1299360711904,
-60.9390296786082));
#182770=CARTESIAN_POINT('Ctrl Pts',(55.5754321736229,-30.4966175475299,
-60.8903552940655));
#182771=CARTESIAN_POINT('',(55.6992942935022,-30.4800318603739,-60.42825533736));
#182772=CARTESIAN_POINT('Origin',(56.1762739063772,-30.63000002,-60.42825533736));
#182773=CARTESIAN_POINT('Origin',(54.3783008183434,-30.6572029381318,-60.3807755792598));
#182774=CARTESIAN_POINT('Origin',(0.,-12.9675000200281,-60.64995));
#182775=CARTESIAN_POINT('Origin',(0.,-12.9675000200281,-60.8508735991007));
#182776=CARTESIAN_POINT('Ctrl Pts',(53.903079465118,-36.78000002,-61.1007217352389));
#182777=CARTESIAN_POINT('Ctrl Pts',(53.2672382848488,-36.7800000200009,
-60.7532634257798));
#182778=CARTESIAN_POINT('Ctrl Pts',(53.4928740664966,-36.1025529613072,
-60.8765730017782));
#182779=CARTESIAN_POINT('Ctrl Pts',(54.0233453777872,-36.78000002,-60.8807385305411));
#182780=CARTESIAN_POINT('Ctrl Pts',(53.3073297453563,-36.7800000199946,
-60.6286940607591));
#182781=CARTESIAN_POINT('Ctrl Pts',(53.5792270344601,-36.0882821494794,
-60.7299113961242));
#182782=CARTESIAN_POINT('Ctrl Pts',(54.0836727915734,-36.78000002,-60.6340939082454));
#182783=CARTESIAN_POINT('Ctrl Pts',(53.3177002646766,-36.7800000200061,
-60.5197710189114));
#182784=CARTESIAN_POINT('Ctrl Pts',(53.6225015011258,-36.0811780755465,
-60.565486568279));
#182785=CARTESIAN_POINT('Ctrl Pts',(54.0757885469763,-36.78000002,-60.3849343801088));
#182786=CARTESIAN_POINT('Ctrl Pts',(53.3162520055491,-36.7800000199989,
-60.4089987140158));
#182787=CARTESIAN_POINT('Ctrl Pts',(53.6168456207784,-36.0821069256242,
-60.3993736717233));
#182788=CARTESIAN_POINT('',(53.6173229282256,-36.0820590308261,-60.42825533736));
#182789=CARTESIAN_POINT('',(54.076473627675,-36.78000002,-60.42825533736));
#182790=CARTESIAN_POINT('Origin',(54.076473627675,-36.28000002,-60.42825533736));
#182791=CARTESIAN_POINT('Origin',(52.6143300188006,-36.78000002,-60.4624709867154));
#182792=CARTESIAN_POINT('Ctrl Pts',(53.6173229282257,-36.0820590308261,
-60.42825533736));
#182793=CARTESIAN_POINT('Ctrl Pts',(53.6173229282257,-36.0820590308261,
-60.4718732914667));
#182794=CARTESIAN_POINT('Ctrl Pts',(53.6139639100269,-36.0826317730148,
-60.5156743630418));
#182795=CARTESIAN_POINT('Ctrl Pts',(53.6072032158688,-36.0837570727629,
-60.5592767125907));
#182796=CARTESIAN_POINT('Ctrl Pts',(53.6004830965447,-36.0848756189367,
-60.6026173792329));
#182797=CARTESIAN_POINT('Ctrl Pts',(53.5904018582716,-36.0865400407211,
-60.6457612486292));
#182798=CARTESIAN_POINT('Ctrl Pts',(53.5769646226219,-36.0887472436547,
-60.6883213233074));
#182799=CARTESIAN_POINT('Ctrl Pts',(53.5636388975191,-36.0909361298442,
-60.7305282079898));
#182800=CARTESIAN_POINT('Ctrl Pts',(53.5470125747611,-36.0936587800579,
-60.7721604735197));
#182801=CARTESIAN_POINT('Ctrl Pts',(53.5271386403121,-36.0969295254175,
-60.8128357523528));
#182802=CARTESIAN_POINT('Ctrl Pts',(53.5208954705939,-36.0979569927486,
-60.8256134270373));
#182803=CARTESIAN_POINT('Ctrl Pts',(53.5143321784749,-36.0990386798933,
-60.8382966552944));
#182804=CARTESIAN_POINT('Ctrl Pts',(53.5074514076768,-36.1001753985996,
-60.8508735991007));
#182805=CARTESIAN_POINT('Origin',(-83.2809572255632,-36.78000002,-55.24995));
#182806=CARTESIAN_POINT('',(54.076473627675,-36.78000002,-55.74995));
#182807=CARTESIAN_POINT('',(54.076473627675,-36.78000002,-55.24995));
#182808=CARTESIAN_POINT('',(-83.2809572255632,-36.78000002,-55.74995));
#182809=CARTESIAN_POINT('Origin',(-83.2809572255632,-37.28000002,-55.74995));
#182810=CARTESIAN_POINT('',(53.7823432375799,-37.1153847305994,-55.2778252214768));
#182811=CARTESIAN_POINT('Ctrl Pts',(54.076473627675,-36.78000002,-55.74995));
#182812=CARTESIAN_POINT('Ctrl Pts',(54.0764736237006,-36.78000002,-55.7254348582675));
#182813=CARTESIAN_POINT('Ctrl Pts',(54.0748711940854,-36.7818350468828,
-55.7007325233529));
#182814=CARTESIAN_POINT('Ctrl Pts',(54.0716496717766,-36.7855406125626,
-55.6761136367726));
#182815=CARTESIAN_POINT('Ctrl Pts',(54.068323113487,-36.7893669961938,-55.6506920647993));
#182816=CARTESIAN_POINT('Ctrl Pts',(54.0632701595081,-36.7951876895575,
-55.6253595447221));
#182817=CARTESIAN_POINT('Ctrl Pts',(54.0565037344636,-36.8030047692021,
-55.6004402933233));
#182818=CARTESIAN_POINT('Ctrl Pts',(54.0554730514243,-36.8041954912383,
-55.5966445149615));
#182819=CARTESIAN_POINT('Ctrl Pts',(54.0544026690462,-36.8054324694357,
-55.592858372319));
#182820=CARTESIAN_POINT('Ctrl Pts',(54.0532926938187,-36.806715643047,-55.5890830610468));
#182821=CARTESIAN_POINT('Ctrl Pts',(54.045565771698,-36.815648259124,-55.5628018112867));
#182822=CARTESIAN_POINT('Ctrl Pts',(54.0359072128158,-36.8268241578973,
-55.5370354066851));
#182823=CARTESIAN_POINT('Ctrl Pts',(54.0243169062867,-36.8402147976036,
-55.5121923007281));
#182824=CARTESIAN_POINT('Ctrl Pts',(54.0185217530221,-36.8469101174568,
-55.4997707477495));
#182825=CARTESIAN_POINT('Ctrl Pts',(54.0122436577221,-36.8541587109129,
-55.4875806630813));
#182826=CARTESIAN_POINT('Ctrl Pts',(54.0054826167242,-36.861953334192,-55.4756781686146));
#182827=CARTESIAN_POINT('Ctrl Pts',(54.0021020962253,-36.8658506458316,
-55.4697269213813));
#182828=CARTESIAN_POINT('Ctrl Pts',(53.9986008398608,-36.8698844412374,
-55.4638475980883));
#182829=CARTESIAN_POINT('Ctrl Pts',(53.9949788498558,-36.8740534181339,
-55.4580476645523));
#182830=CARTESIAN_POINT('Ctrl Pts',(53.9942871097817,-36.8748496236407,
-55.4569399733525));
#182831=CARTESIAN_POINT('Ctrl Pts',(53.9935547350079,-36.8756923521775,
-55.4557774965243));
#182832=CARTESIAN_POINT('Ctrl Pts',(53.9928014458625,-36.8765589029471,
-55.4545938334076));
#182833=CARTESIAN_POINT('Ctrl Pts',(53.9909351836162,-36.8787057691218,
-55.4516613262808));
#182834=CARTESIAN_POINT('Ctrl Pts',(53.9889418285035,-36.880997110987,-55.4486056977901));
#182835=CARTESIAN_POINT('Ctrl Pts',(53.9871466296489,-36.8830591828349,
-55.4459130461622));
#182836=CARTESIAN_POINT('Ctrl Pts',(53.9858723589523,-36.8845228857128,
-55.4440017442156));
#182837=CARTESIAN_POINT('Ctrl Pts',(53.9846988573795,-36.8858700336466,
-55.4422722514467));
#182838=CARTESIAN_POINT('Ctrl Pts',(53.9837506400808,-36.8869578372551,
-55.4408885206699));
#182839=CARTESIAN_POINT('Ctrl Pts',(53.9735107226483,-36.8987051647392,
-55.4259454386124));
#182840=CARTESIAN_POINT('Ctrl Pts',(53.9621990035396,-36.9116599662525,
-55.4112184958409));
#182841=CARTESIAN_POINT('Ctrl Pts',(53.9497544034244,-36.9258791059603,
-55.3969517565364));
#182842=CARTESIAN_POINT('Ctrl Pts',(53.9378712005585,-36.9394567958953,
-55.3833286143042));
#182843=CARTESIAN_POINT('Ctrl Pts',(53.9249549238256,-36.9541874350935,
-55.3701252127202));
#182844=CARTESIAN_POINT('Ctrl Pts',(53.9109800116058,-36.9700858487164,
-55.3575709377622));
#182845=CARTESIAN_POINT('Ctrl Pts',(53.8972917642908,-36.98565814099,-55.3452741864279));
#182846=CARTESIAN_POINT('Ctrl Pts',(53.8825877148145,-37.0023509706149,
-55.3336002534511));
#182847=CARTESIAN_POINT('Ctrl Pts',(53.8668729413441,-37.0201419084753,
-55.322780146583));
#182848=CARTESIAN_POINT('Ctrl Pts',(53.8515575866294,-37.0374806581908,
-55.3122350518637));
#182849=CARTESIAN_POINT('Ctrl Pts',(53.8352821576126,-37.0558624917925,
-55.3025009940998));
#182850=CARTESIAN_POINT('Ctrl Pts',(53.818080891982,-37.0752298715344,-55.2938058043885));
#182851=CARTESIAN_POINT('Ctrl Pts',(53.8065758593464,-37.0881837053268,
-55.2879900438771));
#182852=CARTESIAN_POINT('Ctrl Pts',(53.7946572537875,-37.1015776749406,
-55.2826393142049));
#182853=CARTESIAN_POINT('Ctrl Pts',(53.7823432375799,-37.1153847305994,
-55.2778252214768));
#182854=CARTESIAN_POINT('',(53.65082011387,-37.28000002,-55.24995));
#182855=CARTESIAN_POINT('Ctrl Pts',(53.7823432375799,-37.1153847305994,
-55.2778252214768));
#182856=CARTESIAN_POINT('Ctrl Pts',(53.7292323645857,-37.1749351436578,
-55.2570618366145));
#182857=CARTESIAN_POINT('Ctrl Pts',(53.6853913233491,-37.2312368757479,
-55.24995));
#182858=CARTESIAN_POINT('Ctrl Pts',(53.65082011387,-37.28000002,-55.24995));
#182859=CARTESIAN_POINT('',(60.,-37.28000002,-55.24995));
#182860=CARTESIAN_POINT('Origin',(60.,28.41999998,-55.24995));
#182861=CARTESIAN_POINT('',(53.5055391860638,-37.78000002,-55.24995));
#182862=CARTESIAN_POINT('Origin',(57.8922230010149,-38.7834964612722,-55.24995));
#182863=CARTESIAN_POINT('',(60.,-37.78000002,-55.24995));
#182864=CARTESIAN_POINT('Origin',(60.,-37.78000002,-55.74995));
#182865=CARTESIAN_POINT('',(53.4093468596018,-38.0856478194539,-55.3542488214713));
#182866=CARTESIAN_POINT('Ctrl Pts',(53.5055391860638,-37.78000002,-55.24995));
#182867=CARTESIAN_POINT('Ctrl Pts',(53.4934324707211,-37.806461664537,-55.24995));
#182868=CARTESIAN_POINT('Ctrl Pts',(53.4823161171381,-37.8331687413443,
-55.2520788136903));
#182869=CARTESIAN_POINT('Ctrl Pts',(53.4722294340858,-37.8597633672056,
-55.2563959926891));
#182870=CARTESIAN_POINT('Ctrl Pts',(53.4622707511287,-37.8860205070348,
-55.2606583866491));
#182871=CARTESIAN_POINT('Ctrl Pts',(53.4533156112428,-37.9121671500672,
-55.2670537868195));
#182872=CARTESIAN_POINT('Ctrl Pts',(53.44537582615,-37.9378357595513,-55.2755941342185));
#182873=CARTESIAN_POINT('Ctrl Pts',(53.4372230919462,-37.9641928143152,
-55.2843635381178));
#182874=CARTESIAN_POINT('Ctrl Pts',(53.4301408735503,-37.9900449202448,
-55.2953945620593));
#182875=CARTESIAN_POINT('Ctrl Pts',(53.4241155832649,-38.0149832204437,
-55.3086523082856));
#182876=CARTESIAN_POINT('Ctrl Pts',(53.4181787909317,-38.0395552331459,
-55.3217153280615));
#182877=CARTESIAN_POINT('Ctrl Pts',(53.41326787339,-38.063239083628,-55.336939849031));
#182878=CARTESIAN_POINT('Ctrl Pts',(53.4093468596018,-38.0856478194539,
-55.3542488214713));
#182879=CARTESIAN_POINT('Origin',(53.4522739634651,-37.8403182980825,-55.7203377623201));
#182880=CARTESIAN_POINT('Origin',(-83.2809572255632,11.6199999800001,-55.74995));
#182881=CARTESIAN_POINT('',(53.4093468596018,12.0381477794281,-55.475810586866));
#182882=CARTESIAN_POINT('Origin',(53.4672824165089,11.7070445566108,-55.7239619428824));
#182883=CARTESIAN_POINT('',(53.5631588418786,11.61999998,-55.24995));
#182884=CARTESIAN_POINT('Ctrl Pts',(53.4093468596018,12.0381477794281,-55.475810586866));
#182885=CARTESIAN_POINT('Ctrl Pts',(53.411271555201,12.0271480752568,-55.4590326196229));
#182886=CARTESIAN_POINT('Ctrl Pts',(53.4135176755445,12.0153190624728,-55.4432762206355));
#182887=CARTESIAN_POINT('Ctrl Pts',(53.416096779611,12.0028976523553,-55.4285379015408));
#182888=CARTESIAN_POINT('Ctrl Pts',(53.4188144250206,11.9898090032297,-55.413007886389));
#182889=CARTESIAN_POINT('Ctrl Pts',(53.4219016576878,11.976062431537,-55.3986080182298));
#182890=CARTESIAN_POINT('Ctrl Pts',(53.4253639809393,11.9618801590715,-55.3853184129368));
#182891=CARTESIAN_POINT('Ctrl Pts',(53.4263179288633,11.9579726240456,-55.3816568277932));
#182892=CARTESIAN_POINT('Ctrl Pts',(53.4273003127235,11.954031716205,-55.3780794498407));
#182893=CARTESIAN_POINT('Ctrl Pts',(53.428311168957,11.950061432097,-55.3745857064195));
#182894=CARTESIAN_POINT('Ctrl Pts',(53.431076440011,11.9392004299527,-55.3650283161277));
#182895=CARTESIAN_POINT('Ctrl Pts',(53.434029674615,11.928216282372,-55.3561764344811));
#182896=CARTESIAN_POINT('Ctrl Pts',(53.4371890974518,11.9170932442165,-55.3479256972112));
#182897=CARTESIAN_POINT('Ctrl Pts',(53.4403923945095,11.905815742838,-55.3395603837388));
#182898=CARTESIAN_POINT('Ctrl Pts',(53.4438074174171,11.8943947184568,-55.3318125871665));
#182899=CARTESIAN_POINT('Ctrl Pts',(53.4474716139716,11.8827770512412,-55.3246073283533));
#182900=CARTESIAN_POINT('Ctrl Pts',(53.450288870995,11.8738446825559,-55.3190674874371));
#182901=CARTESIAN_POINT('Ctrl Pts',(53.4532537656305,11.8647952569811,-55.3138489850583));
#182902=CARTESIAN_POINT('Ctrl Pts',(53.4563919355982,11.8555940534045,-55.3089336366617));
#182903=CARTESIAN_POINT('Ctrl Pts',(53.4570281012091,11.8537287977445,-55.307937203821));
#182904=CARTESIAN_POINT('Ctrl Pts',(53.4576720413956,11.8518563454007,-55.3069526932524));
#182905=CARTESIAN_POINT('Ctrl Pts',(53.4583239030131,11.8499764038232,-55.3059799159839));
#182906=CARTESIAN_POINT('Ctrl Pts',(53.4661611528671,11.8273741037968,-55.2942843378106));
#182907=CARTESIAN_POINT('Ctrl Pts',(53.4751104310767,11.8038199874285,-55.2843487566791));
#182908=CARTESIAN_POINT('Ctrl Pts',(53.4851501145903,11.7795869692876,-55.2762231679919));
#182909=CARTESIAN_POINT('Ctrl Pts',(53.4949709984344,11.75588207301,-55.2682746641818));
#182910=CARTESIAN_POINT('Ctrl Pts',(53.5058355767072,11.7315262142338,-55.2620580158118));
#182911=CARTESIAN_POINT('Ctrl Pts',(53.5177437847908,11.7067803310973,-55.2576643682367));
#182912=CARTESIAN_POINT('Ctrl Pts',(53.5289856773389,11.6834190867124,-55.2535165641685));
#182913=CARTESIAN_POINT('Ctrl Pts',(53.5411579876986,11.6597092930614,-55.2509935902076));
#182914=CARTESIAN_POINT('Ctrl Pts',(53.5542743627635,11.6358913899761,-55.2502114786518));
#182915=CARTESIAN_POINT('Ctrl Pts',(53.5571891134863,11.6305985213373,-55.2500376760416));
#182916=CARTESIAN_POINT('Ctrl Pts',(53.5601505311349,11.6253004309346,-55.24995));
#182917=CARTESIAN_POINT('Ctrl Pts',(53.5631588418786,11.61999998,-55.24995));
#182918=CARTESIAN_POINT('',(60.,11.61999998,-55.24995));
#182919=CARTESIAN_POINT('Origin',(60.,28.41999998,-55.24995));
#182920=CARTESIAN_POINT('',(53.7374305810854,11.11999998,-55.24995));
#182921=CARTESIAN_POINT('Origin',(57.8922230010151,12.8484964212155,-55.24995));
#182922=CARTESIAN_POINT('',(60.,11.11999998,-55.24995));
#182923=CARTESIAN_POINT('Origin',(60.,11.11999998,-55.74995));
#182924=CARTESIAN_POINT('',(53.7823432375846,11.067884690566,-55.2526734204115));
#182925=CARTESIAN_POINT('Ctrl Pts',(53.7374305810854,11.11999998,-55.24995));
#182926=CARTESIAN_POINT('Ctrl Pts',(53.7521098206901,11.1023577124241,-55.24995));
#182927=CARTESIAN_POINT('Ctrl Pts',(53.7671137595184,11.084960698582,-55.2508838306004));
#182928=CARTESIAN_POINT('Ctrl Pts',(53.7823432375846,11.067884690566,-55.2526734204115));
#182929=CARTESIAN_POINT('Ctrl Pts',(53.7823432375846,11.067884690566,-55.2526734204115));
#182930=CARTESIAN_POINT('Ctrl Pts',(53.8011235246843,11.0468273478585,-55.2548802597339));
#182931=CARTESIAN_POINT('Ctrl Pts',(53.8191049193374,11.02648059754,-55.2583653100953));
#182932=CARTESIAN_POINT('Ctrl Pts',(53.8362874215441,11.0069647460792,-55.2628945248306));
#182933=CARTESIAN_POINT('Ctrl Pts',(53.8541929651849,10.9866276656112,-55.267614329381));
#182934=CARTESIAN_POINT('Ctrl Pts',(53.8712309668023,10.9671927270046,-55.27346732726));
#182935=CARTESIAN_POINT('Ctrl Pts',(53.8874014263962,10.9487392110445,-55.280195011717));
#182936=CARTESIAN_POINT('Ctrl Pts',(53.9039667551484,10.9298350755907,-55.2870869806263));
#182937=CARTESIAN_POINT('Ctrl Pts',(53.9196216552579,10.9119604190137,-55.2948962748775));
#182938=CARTESIAN_POINT('Ctrl Pts',(53.9343661267246,10.8951470539327,-55.3033616418457));
#182939=CARTESIAN_POINT('Ctrl Pts',(53.9496905615744,10.877672346998,-55.3121599880513));
#182940=CARTESIAN_POINT('Ctrl Pts',(53.9640315370416,10.8613435812081,-55.3216664686702));
#182941=CARTESIAN_POINT('Ctrl Pts',(53.9773890531262,10.8461466461998,-55.3316147856485));
#182942=CARTESIAN_POINT('Ctrl Pts',(53.9837559739738,10.8389029579489,-55.3363566962228));
#182943=CARTESIAN_POINT('Ctrl Pts',(53.9898994532802,10.8319157554432,-55.3411994334459));
#182944=CARTESIAN_POINT('Ctrl Pts',(53.9958194910456,10.825180276009,-55.3461166901571));
#182945=CARTESIAN_POINT('Ctrl Pts',(54.00467766823,10.8151019500565,-55.3534744018704));
#182946=CARTESIAN_POINT('Ctrl Pts',(54.0130355763021,10.8055875154472,-55.3609985450547));
#182947=CARTESIAN_POINT('Ctrl Pts',(54.0208932152617,10.7966139956126,-55.3686082830298));
#182948=CARTESIAN_POINT('Ctrl Pts',(54.0248220347416,10.7921272356953,-55.3724131520174));
#182949=CARTESIAN_POINT('Ctrl Pts',(54.0286257869433,10.787775720653,-55.3762394382259));
#182950=CARTESIAN_POINT('Ctrl Pts',(54.0323044718669,10.7835557757841,-55.3800779985596));
#182951=CARTESIAN_POINT('Ctrl Pts',(54.0341438143287,10.7814458033496,-55.3819972787265));
#182952=CARTESIAN_POINT('Ctrl Pts',(54.035951889971,10.7793687254093,-55.3839196297065));
#182953=CARTESIAN_POINT('Ctrl Pts',(54.0377286987937,10.7773240721282,-55.3858439410498));
#182954=CARTESIAN_POINT('Ctrl Pts',(54.0388203296637,10.7760678837239,-55.3870261941086));
#182955=CARTESIAN_POINT('Ctrl Pts',(54.039525317404,10.7752615357712,-55.3877925642775));
#182956=CARTESIAN_POINT('Ctrl Pts',(54.040534543656,10.7740965012651,-55.3889087511113));
#182957=CARTESIAN_POINT('Ctrl Pts',(54.0411679991548,10.7733652504551,-55.3896093419712));
#182958=CARTESIAN_POINT('Ctrl Pts',(54.0419213132897,10.7724929242244,-55.3904480137501));
#182959=CARTESIAN_POINT('Ctrl Pts',(54.0429653248035,10.7712869097631,-55.3916216664204));
#182960=CARTESIAN_POINT('Ctrl Pts',(54.0588511417924,10.752936034543,-55.4094801203573));
#182961=CARTESIAN_POINT('Ctrl Pts',(54.0732805056091,10.7361175475333,-55.4285968746425));
#182962=CARTESIAN_POINT('Ctrl Pts',(54.0862534162535,10.7209515952271,-55.44868535453));
#182963=CARTESIAN_POINT('Ctrl Pts',(54.0993947773437,10.7055887163023,-55.4690346789947));
#182964=CARTESIAN_POINT('Ctrl Pts',(54.1110416162365,10.6919214842835,-55.4903805240241));
#182965=CARTESIAN_POINT('Ctrl Pts',(54.1211939329318,10.6800213281955,-55.5124236099793));
#182966=CARTESIAN_POINT('Ctrl Pts',(54.131551448063,10.6678806463743,-55.5349122303772));
#182967=CARTESIAN_POINT('Ctrl Pts',(54.1403534159387,10.6575790662613,-55.5581259619573));
#182968=CARTESIAN_POINT('Ctrl Pts',(54.1475998365589,10.6491386635634,-55.5817548137324));
#182969=CARTESIAN_POINT('Ctrl Pts',(54.1549301223136,10.640600577396,-55.6056571297372));
#182970=CARTESIAN_POINT('Ctrl Pts',(54.1606686467721,10.6339666934735,-55.6299836882972));
#182971=CARTESIAN_POINT('Ctrl Pts',(54.1648154099345,10.6292088063485,-55.654430243584));
#182972=CARTESIAN_POINT('Ctrl Pts',(54.1690341997196,10.6243682777686,-55.6793014198929));
#182973=CARTESIAN_POINT('Ctrl Pts',(54.1716054522323,10.621469129154,-55.7042962935649));
#182974=CARTESIAN_POINT('Ctrl Pts',(54.1725291674727,10.6204340720944,-55.7291196457432));
#182975=CARTESIAN_POINT('Ctrl Pts',(54.1727881145264,10.6201439123522,-55.7360784287428));
#182976=CARTESIAN_POINT('Ctrl Pts',(54.1729175880533,10.61999998,-55.7430239067242));
#182977=CARTESIAN_POINT('Ctrl Pts',(54.1729175880533,10.61999998,-55.74995));
#182978=CARTESIAN_POINT('Origin',(3.5,-9.33460238845303,-92.34995));
#182979=CARTESIAN_POINT('',(3.5,45.7028119503364,-61.0621827299711));
#182980=CARTESIAN_POINT('',(3.5,45.8435334367418,-60.42825533736));
#182981=CARTESIAN_POINT('Origin',(3.5,43.6249324139852,-60.2700376788023));
#182982=CARTESIAN_POINT('',(3.50000000126666,45.8435334367292,-56.3263223051815));
#182983=CARTESIAN_POINT('',(3.5,45.8435334367418,-92.34995));
#182984=CARTESIAN_POINT('Ctrl Pts',(3.50000000506663,45.8435334367288,-56.3263223051817));
#182985=CARTESIAN_POINT('Ctrl Pts',(3.50000001032463,45.8894626566105,-56.3816811876747));
#182986=CARTESIAN_POINT('Ctrl Pts',(3.50000001775255,45.9328922004513,-56.438876382961));
#182987=CARTESIAN_POINT('Ctrl Pts',(3.50000002291889,45.9736813029624,-56.4976009415836));
#182988=CARTESIAN_POINT('Ctrl Pts',(3.50000002818049,46.0152224330363,-56.5574082032809));
#182989=CARTESIAN_POINT('Ctrl Pts',(3.50000003120722,46.0540257195003,-56.6188027368888));
#182990=CARTESIAN_POINT('Ctrl Pts',(3.50000003122783,46.0899059446862,-56.6814984159273));
#182991=CARTESIAN_POINT('Ctrl Pts',(3.50000003123068,46.0948520295369,-56.6901410079592));
#182992=CARTESIAN_POINT('Ctrl Pts',(3.50000003118087,46.0997425008543,-56.6988083694207));
#182993=CARTESIAN_POINT('Ctrl Pts',(3.5000000310803,46.1045768057904,-56.7074997895477));
#182994=CARTESIAN_POINT('Ctrl Pts',(3.50000003035461,46.1394632249473,-56.7702208072802));
#182995=CARTESIAN_POINT('Ctrl Pts',(3.50000002687238,46.1717681199834,-56.8347988963916));
#182996=CARTESIAN_POINT('Ctrl Pts',(3.50000002225516,46.2013495572016,-56.9009409523228));
#182997=CARTESIAN_POINT('Ctrl Pts',(3.5000000182853,46.2267835376253,-56.9578095805551));
#182998=CARTESIAN_POINT('Ctrl Pts',(3.50000001353393,46.2502037235481,-57.0158352648145));
#182999=CARTESIAN_POINT('Ctrl Pts',(3.50000000945277,46.2714898142467,-57.0748386052854));
#183000=CARTESIAN_POINT('Ctrl Pts',(3.50000000440193,46.2978334233143,-57.1478609820601));
#183001=CARTESIAN_POINT('Ctrl Pts',(3.5000000025334,46.3207458812431,-57.221900953307));
#183002=CARTESIAN_POINT('Ctrl Pts',(3.50000000146594,46.3400500971326,-57.2964727656199));
#183003=CARTESIAN_POINT('Ctrl Pts',(3.50000000013692,46.3640841940101,-57.3893160166336));
#183004=CARTESIAN_POINT('Ctrl Pts',(3.5000000001043,46.3827251371296,-57.4829234266614));
#183005=CARTESIAN_POINT('Ctrl Pts',(3.50000000003929,46.3959468792823,-57.577409970123));
#183006=CARTESIAN_POINT('Ctrl Pts',(3.49999999997471,46.4090811642661,-57.6712715183694));
#183007=CARTESIAN_POINT('Ctrl Pts',(3.50000000000001,46.4168677320184,-57.7660006115251));
#183008=CARTESIAN_POINT('Ctrl Pts',(3.5,46.4192300563852,-57.8617170363515));
#183009=CARTESIAN_POINT('Ctrl Pts',(3.5,46.4197429699982,-57.8824992193464));
#183010=CARTESIAN_POINT('Ctrl Pts',(3.5,46.41999998,-57.90332797385));
#183011=CARTESIAN_POINT('Ctrl Pts',(3.5,46.41999998,-57.9242045702762));
#183012=CARTESIAN_POINT('',(3.5,32.1080106234021,-91.84995));
#183013=CARTESIAN_POINT('',(3.5,32.0719455778696,-91.84995));
#183014=CARTESIAN_POINT('',(3.5,31.6538440087773,-91.1386408691296));
#183015=CARTESIAN_POINT('Ctrl Pts',(3.5,32.1080106234021,-91.84995));
#183016=CARTESIAN_POINT('Ctrl Pts',(3.5,31.9390236361236,-91.84995));
#183017=CARTESIAN_POINT('Ctrl Pts',(3.5,31.7764555346939,-91.7610777969008));
#183018=CARTESIAN_POINT('Ctrl Pts',(3.5,31.5945841314222,-91.476580999558));
#183019=CARTESIAN_POINT('Ctrl Pts',(3.5,31.5822909477801,-91.2917412718895));
#183020=CARTESIAN_POINT('Ctrl Pts',(3.5,31.6538440087773,-91.1386408691296));
#183021=CARTESIAN_POINT('Ctrl Pts',(3.5,31.6538440087773,-91.1386408691296));
#183022=CARTESIAN_POINT('Ctrl Pts',(3.5,36.3389063125119,-81.1141231801469));
#183023=CARTESIAN_POINT('Ctrl Pts',(3.5,41.0213995348935,-71.0884053145847));
#183024=CARTESIAN_POINT('Ctrl Pts',(3.5,45.7028119503364,-61.0621827299711));
#183025=CARTESIAN_POINT('Ctrl Pts',(3.5,46.41999998,-57.9242045702762));
#183026=CARTESIAN_POINT('Ctrl Pts',(3.5,46.91999998,-57.9242045702762));
#183027=CARTESIAN_POINT('Ctrl Pts',(4.,46.91999998,-57.9242045702762));
#183028=CARTESIAN_POINT('Ctrl Pts',(3.5,46.4199999742014,-57.7104514486517));
#183029=CARTESIAN_POINT('Ctrl Pts',(3.49999999999703,46.9215247752432,-57.6673651906402));
#183030=CARTESIAN_POINT('Ctrl Pts',(4.00152248707584,46.91999998,-57.6677551135179));
#183031=CARTESIAN_POINT('Ctrl Pts',(3.5,46.3930553625334,-57.5012311233074));
#183032=CARTESIAN_POINT('Ctrl Pts',(3.50000000000037,46.8905945241102,-57.4159945765447));
#183033=CARTESIAN_POINT('Ctrl Pts',(4.00300631304518,46.8876664373662,-57.4167435210981));
#183034=CARTESIAN_POINT('Ctrl Pts',(3.5,46.2869707037134,-57.0917336115785));
#183035=CARTESIAN_POINT('Ctrl Pts',(3.49999999999963,46.7659528393486,-56.9232257271801));
#183036=CARTESIAN_POINT('Ctrl Pts',(4.00589913432669,46.76036485013,-56.9254492364038));
#183037=CARTESIAN_POINT('Ctrl Pts',(3.5,46.2068681522152,-56.8917559154199));
#183038=CARTESIAN_POINT('Ctrl Pts',(3.50000000000004,46.6709152176612,-56.6822760272594));
#183039=CARTESIAN_POINT('Ctrl Pts',(4.00730581971222,46.6642417866207,-56.6855258491379));
#183040=CARTESIAN_POINT('Ctrl Pts',(3.5,46.0019773297039,-56.5234150618225));
#183041=CARTESIAN_POINT('Ctrl Pts',(3.49999999999995,46.4266646204127,-56.237771148346));
#183042=CARTESIAN_POINT('Ctrl Pts',(4.00988782131373,46.4183727996822,-56.2436081635303));
#183043=CARTESIAN_POINT('Ctrl Pts',(3.5,45.8742601250717,-56.3498268696058));
#183044=CARTESIAN_POINT('Ctrl Pts',(3.50000000000055,46.2738584100651,-56.0280733151404));
#183045=CARTESIAN_POINT('Ctrl Pts',(4.01109981373647,46.2651121552776,-56.0353451211632));
#183046=CARTESIAN_POINT('Ctrl Pts',(3.5,45.5823366328578,-56.0438443443254));
#183047=CARTESIAN_POINT('Ctrl Pts',(3.49999999999944,45.923712698628,-55.6579003398743));
#183048=CARTESIAN_POINT('Ctrl Pts',(4.01323028458345,45.9148039622378,-55.6682412064214));
#183049=CARTESIAN_POINT('Ctrl Pts',(3.5,45.4187493558633,-55.9106117044594));
#183050=CARTESIAN_POINT('Ctrl Pts',(3.50000000000323,45.7271164793515,-55.4966052387911));
#183051=CARTESIAN_POINT('Ctrl Pts',(4.01415476126711,45.7184991995766,-55.5083945642206));
#183052=CARTESIAN_POINT('Ctrl Pts',(3.5,45.2369942737712,-55.7978959562326));
#183053=CARTESIAN_POINT('Ctrl Pts',(3.49999999999999,45.5085033459109,-55.3600853439128));
#183054=CARTESIAN_POINT('Ctrl Pts',(4.01493543718735,45.5003931325255,-55.3731631297134));
#183055=CARTESIAN_POINT('',(4.01487932081911,45.5159632631672,-55.3828828377617));
#183056=CARTESIAN_POINT('Ctrl Pts',(3.5,45.8435334367294,-56.3263223051813));
#183057=CARTESIAN_POINT('Ctrl Pts',(3.5,45.829358462004,-56.2803914253743));
#183058=CARTESIAN_POINT('Ctrl Pts',(3.50100911575913,45.81531891597,-56.2356741862333));
#183059=CARTESIAN_POINT('Ctrl Pts',(3.50319349738481,45.801532809318,-56.1922448897079));
#183060=CARTESIAN_POINT('Ctrl Pts',(3.50366373776018,45.7985650202235,-56.1828956951989));
#183061=CARTESIAN_POINT('Ctrl Pts',(3.50418834634078,45.7956089381192,-56.173606026137));
#183062=CARTESIAN_POINT('Ctrl Pts',(3.50476880342442,45.792665672551,-56.1643763716752));
#183063=CARTESIAN_POINT('Ctrl Pts',(3.50726608643662,45.7800029498262,-56.1246679075265));
#183064=CARTESIAN_POINT('Ctrl Pts',(3.51079967824771,45.7675756095608,-56.0860750894433));
#183065=CARTESIAN_POINT('Ctrl Pts',(3.5154626655906,45.7554812444811,-56.0486556359451));
#183066=CARTESIAN_POINT('Ctrl Pts',(3.5169182402212,45.7517059284254,-56.0369749679103));
#183067=CARTESIAN_POINT('Ctrl Pts',(3.51848356681841,45.7479629575273,-56.0254084224728));
#183068=CARTESIAN_POINT('Ctrl Pts',(3.5201606028619,45.7442550148173,-56.0139572347226));
#183069=CARTESIAN_POINT('Ctrl Pts',(3.5221138261158,45.7399364195471,-56.0006201771886));
#183070=CARTESIAN_POINT('Ctrl Pts',(3.52421598894358,45.7356632838244,-55.9874497786217));
#183071=CARTESIAN_POINT('Ctrl Pts',(3.52646915533919,45.7314373927165,-55.9744418027717));
#183072=CARTESIAN_POINT('Ctrl Pts',(3.532348013131,45.7204113926327,-55.9405019924094));
#183073=CARTESIAN_POINT('Ctrl Pts',(3.53931414435956,45.7096879193575,-55.9076222761818));
#183074=CARTESIAN_POINT('Ctrl Pts',(3.54733023764625,45.699331249749,-55.8759996527637));
#183075=CARTESIAN_POINT('Ctrl Pts',(3.55287443235247,45.6921682352026,-55.8541284026321));
#183076=CARTESIAN_POINT('Ctrl Pts',(3.55892529436838,45.6851783107518,-55.8328413711166));
#183077=CARTESIAN_POINT('Ctrl Pts',(3.56547679288292,45.6783782894728,-55.8121802779607));
#183078=CARTESIAN_POINT('Ctrl Pts',(3.56875254214019,45.6749782788333,-55.8018497313828));
#183079=CARTESIAN_POINT('Ctrl Pts',(3.5721534672821,45.6716257509134,-55.791675655454));
#183080=CARTESIAN_POINT('Ctrl Pts',(3.57567833916439,45.6683227328112,-55.7816639721859));
#183081=CARTESIAN_POINT('Ctrl Pts',(3.57744077510554,45.6666712237602,-55.7766581305518));
#183082=CARTESIAN_POINT('Ctrl Pts',(3.5792341947625,45.6650320925117,-55.7716928867672));
#183083=CARTESIAN_POINT('Ctrl Pts',(3.58105841475146,45.6634055913715,-55.7667689928578));
#183084=CARTESIAN_POINT('Ctrl Pts',(3.58217199249725,45.6624127092169,-55.763763248642));
#183085=CARTESIAN_POINT('Ctrl Pts',(3.58309000391777,45.6616058713521,-55.7613218019833));
#183086=CARTESIAN_POINT('Ctrl Pts',(3.58418948277663,45.6606524681087,-55.7584376140889));
#183087=CARTESIAN_POINT('Ctrl Pts',(3.58489112765552,45.6600440430373,-55.7565970369377));
#183088=CARTESIAN_POINT('Ctrl Pts',(3.58566712536705,45.6593760501822,-55.7545765750859));
#183089=CARTESIAN_POINT('Ctrl Pts',(3.58662326907452,45.6585642310943,-55.7521221209547));
#183090=CARTESIAN_POINT('Ctrl Pts',(3.59663011570348,45.6500678627766,-55.7264341978348));
#183091=CARTESIAN_POINT('Ctrl Pts',(3.60756604207596,45.6418597808983,-55.7017516640631));
#183092=CARTESIAN_POINT('Ctrl Pts',(3.61939706851692,45.6340025528844,-55.6782726631486));
#183093=CARTESIAN_POINT('Ctrl Pts',(3.63078081980458,45.6264423694999,-55.6556812922116));
#183094=CARTESIAN_POINT('Ctrl Pts',(3.64309699882947,45.6191369624624,-55.6340209971509));
#183095=CARTESIAN_POINT('Ctrl Pts',(3.65611874522813,45.6121805085348,-55.613620522482));
#183096=CARTESIAN_POINT('Ctrl Pts',(3.66837924235669,45.6056307278222,-55.5944126563908));
#183097=CARTESIAN_POINT('Ctrl Pts',(3.6813233321023,45.5993584819171,-55.576222352987));
#183098=CARTESIAN_POINT('Ctrl Pts',(3.6948712464061,45.5934033229125,-55.5592148304515));
#183099=CARTESIAN_POINT('Ctrl Pts',(3.69890468364327,45.5916303739889,-55.5541514108602));
#183100=CARTESIAN_POINT('Ctrl Pts',(3.70299535045606,45.5898820494173,-55.54918217229));
#183101=CARTESIAN_POINT('Ctrl Pts',(3.70713510324855,45.5881616196546,-55.5443179945211));
#183102=CARTESIAN_POINT('Ctrl Pts',(3.71544271509736,45.5847090795157,-55.5345566143387));
#183103=CARTESIAN_POINT('Ctrl Pts',(3.72395514919793,45.5813659716028,-55.5252102230316));
#183104=CARTESIAN_POINT('Ctrl Pts',(3.73265162864498,45.5781355148738,-55.5162981662384));
#183105=CARTESIAN_POINT('Ctrl Pts',(3.73484642489412,45.5773202200922,-55.514048963105));
#183106=CARTESIAN_POINT('Ctrl Pts',(3.73677184059151,45.5766149280199,-55.5121100079521));
#183107=CARTESIAN_POINT('Ctrl Pts',(3.73889480346159,45.5758469968331,-55.5100058353679));
#183108=CARTESIAN_POINT('Ctrl Pts',(3.74058370382036,45.5752360774076,-55.5083318834197));
#183109=CARTESIAN_POINT('Ctrl Pts',(3.74239786108271,45.5745856139785,-55.506553746141));
#183110=CARTESIAN_POINT('Ctrl Pts',(3.74458472597647,45.5738132672584,-55.5044511731915));
#183111=CARTESIAN_POINT('Ctrl Pts',(3.75851748247104,45.568892561452,-55.4910554499346));
#183112=CARTESIAN_POINT('Ctrl Pts',(3.77302864720422,45.5641994060292,-55.478603396186));
#183113=CARTESIAN_POINT('Ctrl Pts',(3.78811621274905,45.5597292245555,-55.4671280662862));
#183114=CARTESIAN_POINT('Ctrl Pts',(3.80697700690182,45.554141101518,-55.4527828868446));
#183115=CARTESIAN_POINT('Ctrl Pts',(3.82647622225123,45.5489811037732,-55.4401969432647));
#183116=CARTESIAN_POINT('Ctrl Pts',(3.84639858082278,45.5442730215576,-55.4294510255291));
#183117=CARTESIAN_POINT('Ctrl Pts',(3.86604041389509,45.5396312335565,-55.4188564203967));
#183118=CARTESIAN_POINT('Ctrl Pts',(3.88609303497988,45.5354287546197,-55.4100505420465));
#183119=CARTESIAN_POINT('Ctrl Pts',(3.90634809031781,45.5316770625223,-55.4030622934231));
#183120=CARTESIAN_POINT('Ctrl Pts',(3.92624802272963,45.527991147183,-55.3961965666717));
#183121=CARTESIAN_POINT('Ctrl Pts',(3.94634292913325,45.5247403526288,-55.3910853208616));
#183122=CARTESIAN_POINT('Ctrl Pts',(3.96644019345904,45.5219243282022,-55.387707510953));
#183123=CARTESIAN_POINT('Ctrl Pts',(3.98261682616291,45.5196576618492,-55.3849886538314));
#183124=CARTESIAN_POINT('Ctrl Pts',(3.99879500906382,45.5176724685726,-55.3833919689501));
#183125=CARTESIAN_POINT('Ctrl Pts',(4.01487931457847,45.5159631508241,-55.382883017845));
#183126=CARTESIAN_POINT('Ctrl Pts',(4.,46.91999998,-57.9242045702762));
#183127=CARTESIAN_POINT('Ctrl Pts',(4.00007924273952,46.91999998,-57.9108568329946));
#183128=CARTESIAN_POINT('Ctrl Pts',(4.00017352383104,46.9199165136016,-57.8947589318435));
#183129=CARTESIAN_POINT('Ctrl Pts',(4.00028378860392,46.9196162946768,-57.8758666509881));
#183130=CARTESIAN_POINT('Ctrl Pts',(4.00039284318993,46.9193193707392,-57.8571817182253));
#183131=CARTESIAN_POINT('Ctrl Pts',(4.00051753261627,46.9188105351354,-57.8357633855592));
#183132=CARTESIAN_POINT('Ctrl Pts',(4.00065871293216,46.9179113977889,-57.8115772708384));
#183133=CARTESIAN_POINT('Ctrl Pts',(4.00080188348403,46.9169995851945,-57.7870502015335));
#183134=CARTESIAN_POINT('Ctrl Pts',(4.00096201348742,46.9156867135283,-57.7596767045056));
#183135=CARTESIAN_POINT('Ctrl Pts',(4.00113993168569,46.9137320375537,-57.7294302718212));
#183136=CARTESIAN_POINT('Ctrl Pts',(4.00131784988395,46.9117773615791,-57.6991838391367));
#183137=CARTESIAN_POINT('Ctrl Pts',(4.00151355645692,46.9091810715407,-57.6660644317711));
#183138=CARTESIAN_POINT('Ctrl Pts',(4.00172781289727,46.9056444043791,-57.6300555409693));
#183139=CARTESIAN_POINT('Ctrl Pts',(4.00194116627368,46.9021226438248,-57.5941984231133));
#183140=CARTESIAN_POINT('Ctrl Pts',(4.00217295382255,46.8976670534823,-57.5554657535219));
#183141=CARTESIAN_POINT('Ctrl Pts',(4.00242156630219,46.8919278848425,-57.5138872726071));
#183142=CARTESIAN_POINT('Ctrl Pts',(4.00267017878182,46.8861887162028,-57.4723087916922));
#183143=CARTESIAN_POINT('Ctrl Pts',(4.00293561629726,46.8791659866484,-57.4278844868078));
#183144=CARTESIAN_POINT('Ctrl Pts',(4.00321619974068,46.8704546297142,-57.3806538858939));
#183145=CARTESIAN_POINT('Ctrl Pts',(4.00328167929394,46.8684216667091,-57.3696317150546));
#183146=CARTESIAN_POINT('Ctrl Pts',(4.00335108852505,46.8661920116224,-57.3579141065444));
#183147=CARTESIAN_POINT('Ctrl Pts',(4.00341791351284,46.8639726084551,-57.3466154543736));
#183148=CARTESIAN_POINT('Ctrl Pts',(4.00348900771395,46.8616114154297,-57.3345949710762));
#183149=CARTESIAN_POINT('Ctrl Pts',(4.00355717719454,46.8592620513759,-57.3230486483617));
#183150=CARTESIAN_POINT('Ctrl Pts',(4.00361465014622,46.8572339429933,-57.3133081235097));
#183151=CARTESIAN_POINT('Ctrl Pts',(4.0036188984494,46.8570840286589,-57.3125881204212));
#183152=CARTESIAN_POINT('Ctrl Pts',(4.00362308833456,46.8569358921357,-57.3118779802164));
#183153=CARTESIAN_POINT('Ctrl Pts',(4.00362721667444,46.8567896681397,-57.3111782390562));
#183154=CARTESIAN_POINT('Ctrl Pts',(4.00373969128349,46.852805866605,-57.2921141320444));
#183155=CARTESIAN_POINT('Ctrl Pts',(4.00385082294783,46.8486732798078,-57.2732633244349));
#183156=CARTESIAN_POINT('Ctrl Pts',(4.003960635391,46.8444045670847,-57.2546306622253));
#183157=CARTESIAN_POINT('Ctrl Pts',(4.00412774291756,46.8379086363488,-57.2262763336519));
#183158=CARTESIAN_POINT('Ctrl Pts',(4.0042917882471,46.8310977738947,-57.1984284029624));
#183159=CARTESIAN_POINT('Ctrl Pts',(4.00445272368593,46.8240156437481,-57.171096378751));
#183160=CARTESIAN_POINT('Ctrl Pts',(4.0047257259229,46.8120018984446,-57.1247318004805));
#183161=CARTESIAN_POINT('Ctrl Pts',(4.00498965630254,46.799169649036,-57.0798715656276));
#183162=CARTESIAN_POINT('Ctrl Pts',(4.00524431666679,46.7857397829609,-57.0365571992696));
#183163=CARTESIAN_POINT('Ctrl Pts',(4.00553764088511,46.7702709251338,-56.9866666217082));
#183164=CARTESIAN_POINT('Ctrl Pts',(4.00581865521741,46.7540101778699,-56.9388289010681));
#183165=CARTESIAN_POINT('Ctrl Pts',(4.0060872420386,46.737261956176,-56.8930744281488));
#183166=CARTESIAN_POINT('Ctrl Pts',(4.00638137976372,46.71892046121,-56.8429672914));
#183167=CARTESIAN_POINT('Ctrl Pts',(4.00666061547987,46.6999945698815,-56.7953582140595));
#183168=CARTESIAN_POINT('Ctrl Pts',(4.00692505591205,46.6808375688148,-56.7502406324356));
#183169=CARTESIAN_POINT('Ctrl Pts',(4.00719094249502,46.6615758034652,-56.7048763153719));
#183170=CARTESIAN_POINT('Ctrl Pts',(4.00744186332538,46.6420808938963,-56.662032202587));
#183171=CARTESIAN_POINT('Ctrl Pts',(4.00767810377334,46.6226709619017,-56.6216696645318));
#183172=CARTESIAN_POINT('Ctrl Pts',(4.0079264310232,46.6022679569391,-56.5792420524993));
#183173=CARTESIAN_POINT('Ctrl Pts',(4.00815854179178,46.5819587512262,-56.5395556683638));
#183174=CARTESIAN_POINT('Ctrl Pts',(4.00837493639319,46.5620675828846,-56.50253498429));
#183175=CARTESIAN_POINT('Ctrl Pts',(4.00841906033974,46.5580116737128,-56.4949862807898));
#183176=CARTESIAN_POINT('Ctrl Pts',(4.00846253140605,46.5539729912662,-56.4875483092653));
#183177=CARTESIAN_POINT('Ctrl Pts',(4.00850535448981,46.5499540635142,-56.4802203087462));
#183178=CARTESIAN_POINT('Ctrl Pts',(4.00852061045761,46.5485222975845,-56.4776096667733));
#183179=CARTESIAN_POINT('Ctrl Pts',(4.00852856980572,46.5477743781799,-56.4762464665642));
#183180=CARTESIAN_POINT('Ctrl Pts',(4.00855086918121,46.5456663975,-56.4724302181349));
#183181=CARTESIAN_POINT('Ctrl Pts',(4.00856620879158,46.5442163298814,-56.4698050430919));
#183182=CARTESIAN_POINT('Ctrl Pts',(4.00858152375101,46.5427632883518,-56.467183969051));
#183183=CARTESIAN_POINT('Ctrl Pts',(4.00859681400415,46.5413072932493,-56.4645670062797));
#183184=CARTESIAN_POINT('Ctrl Pts',(4.00896054749668,46.5066712294084,-56.4023131639001));
#183185=CARTESIAN_POINT('Ctrl Pts',(4.00931319598185,46.470088502395,-56.3418910107853));
#183186=CARTESIAN_POINT('Ctrl Pts',(4.00965406429937,46.431893439433,-56.2834331861898));
#183187=CARTESIAN_POINT('Ctrl Pts',(4.01000373713251,46.3927118106592,-56.2234654153681));
#183188=CARTESIAN_POINT('Ctrl Pts',(4.01034101480063,46.351833327529,-56.1655645089445));
#183189=CARTESIAN_POINT('Ctrl Pts',(4.01066532568298,46.3095728022947,-56.1098411585262));
#183190=CARTESIAN_POINT('Ctrl Pts',(4.01100339145799,46.2655198950584,-56.0517544316515));
#183191=CARTESIAN_POINT('Ctrl Pts',(4.01132736838532,46.2199651772572,-55.9960336844979));
#183192=CARTESIAN_POINT('Ctrl Pts',(4.01163678119951,46.1732171831732,-55.9427728835428));
#183193=CARTESIAN_POINT('Ctrl Pts',(4.01181788083476,46.1458555346277,-55.911599282503));
#183194=CARTESIAN_POINT('Ctrl Pts',(4.0119939942426,46.1180842067542,-55.8812678356419));
#183195=CARTESIAN_POINT('Ctrl Pts',(4.0121650491596,46.0899580587577,-55.8517931637923));
#183196=CARTESIAN_POINT('Ctrl Pts',(4.01220547809655,46.0833104260319,-55.8448268066077));
#183197=CARTESIAN_POINT('Ctrl Pts',(4.01224563317101,46.0766440200839,-55.8379068481933));
#183198=CARTESIAN_POINT('Ctrl Pts',(4.0122855169593,46.0699590233885,-55.8310328738311));
#183199=CARTESIAN_POINT('Ctrl Pts',(4.01259435546335,46.0181940214239,-55.7778045309336));
#183200=CARTESIAN_POINT('Ctrl Pts',(4.01288644492606,45.9653889456504,-55.7274166744311));
#183201=CARTESIAN_POINT('Ctrl Pts',(4.01316209893909,45.9118461763452,-55.67982860949));
#183202=CARTESIAN_POINT('Ctrl Pts',(4.01344237678578,45.857405278057,-55.6314423000628));
#183203=CARTESIAN_POINT('Ctrl Pts',(4.01370566398607,45.8022018384633,-55.5859503887996));
#183204=CARTESIAN_POINT('Ctrl Pts',(4.01395252112905,45.7465895304821,-55.5432689102761));
#183205=CARTESIAN_POINT('Ctrl Pts',(4.01420785359687,45.6890678899609,-55.4991220522573));
#183206=CARTESIAN_POINT('Ctrl Pts',(4.01444560917555,45.6311089169403,-55.4579818299398));
#183207=CARTESIAN_POINT('Ctrl Pts',(4.01466664258002,45.5731406032728,-55.4197129653607));
#183208=CARTESIAN_POINT('Ctrl Pts',(4.01473933218221,45.5540769976138,-55.4071277701532));
#183209=CARTESIAN_POINT('Ctrl Pts',(4.01481021504988,45.5350126608396,-55.3948527899582));
#183210=CARTESIAN_POINT('Ctrl Pts',(4.0148793265843,45.515963602184,-55.3828822983059));
#183211=CARTESIAN_POINT('Ctrl Pts',(4.0117049092053,45.5008851266717,-55.3733547413106));
#183212=CARTESIAN_POINT('Ctrl Pts',(3.98080144737803,46.91999998,-56.2527140593899));
#183213=CARTESIAN_POINT('Ctrl Pts',(3.92215684205867,46.91999998,-57.921448793088));
#183214=CARTESIAN_POINT('Ctrl Pts',(4.20907605864183,45.4888071699417,-55.3727975967646));
#183215=CARTESIAN_POINT('Ctrl Pts',(4.17733814927366,46.9199999800018,-56.2502970131543));
#183216=CARTESIAN_POINT('Ctrl Pts',(4.11592937444032,46.91999998,-57.928258571556));
#183217=CARTESIAN_POINT('Ctrl Pts',(4.4062116365889,45.4758414047913,-55.3721833857794));
#183218=CARTESIAN_POINT('Ctrl Pts',(4.37353389556208,46.91999998,-56.2475777730215));
#183219=CARTESIAN_POINT('Ctrl Pts',(4.30969200192382,46.91999998,-57.9354449440051));
#183220=CARTESIAN_POINT('Ctrl Pts',(4.60306732532638,45.461992503193,-55.3715051982969));
#183221=CARTESIAN_POINT('Ctrl Pts',(4.5692462665161,46.9199999800001,-56.2445032348437));
#183222=CARTESIAN_POINT('Ctrl Pts',(4.50344622215482,46.91999998,-57.9429512300502));
#183223=CARTESIAN_POINT('',(4.51630724700544,45.4845441378501,-55.3818234152652));
#183224=CARTESIAN_POINT('Origin',(-0.00205740951117972,-22.4761263385902,
-51.448280968311));
#183225=CARTESIAN_POINT('Ctrl Pts',(4.51630724691536,45.4845441364184,-55.3818234176142));
#183226=CARTESIAN_POINT('Ctrl Pts',(4.51609516365136,45.539686183746,-55.4155436161894));
#183227=CARTESIAN_POINT('Ctrl Pts',(4.51587384346763,45.5949145728422,-55.4517660043098));
#183228=CARTESIAN_POINT('Ctrl Pts',(4.51563780342165,45.6499431393258,-55.4906255200563));
#183229=CARTESIAN_POINT('Ctrl Pts',(4.51540569412177,45.7040553218034,-55.5288379130265));
#183230=CARTESIAN_POINT('Ctrl Pts',(4.51515932999363,45.7579739851358,-55.5696008805653));
#183231=CARTESIAN_POINT('Ctrl Pts',(4.51489474095432,45.8113906483242,-55.6130088438551));
#183232=CARTESIAN_POINT('Ctrl Pts',(4.51463612804323,45.8636008184923,-55.6554363751671));
#183233=CARTESIAN_POINT('Ctrl Pts',(4.51436008730205,45.9153309682504,-55.7003912001386));
#183234=CARTESIAN_POINT('Ctrl Pts',(4.51406438647219,45.9662634802363,-55.7479217231849));
#183235=CARTESIAN_POINT('Ctrl Pts',(4.513901763993,45.9942741265869,-55.7740614249196));
#183236=CARTESIAN_POINT('Ctrl Pts',(4.51373322290916,46.0220430358204,-55.800979408275));
#183237=CARTESIAN_POINT('Ctrl Pts',(4.51355861607773,46.0495142484638,-55.8286777245581));
#183238=CARTESIAN_POINT('Ctrl Pts',(4.51324936416135,46.0981694189724,-55.8777351258112));
#183239=CARTESIAN_POINT('Ctrl Pts',(4.51292097533616,46.1458914126912,-55.9292432583753));
#183240=CARTESIAN_POINT('Ctrl Pts',(4.51257402801332,46.1923566835266,-55.9831763724683));
#183241=CARTESIAN_POINT('Ctrl Pts',(4.51223332955441,46.2379850689438,-56.0361380979107));
#183242=CARTESIAN_POINT('Ctrl Pts',(4.51187472815627,46.2824009821158,-56.0914384019429));
#183243=CARTESIAN_POINT('Ctrl Pts',(4.51150062802555,46.325289847004,-56.1490037731485));
#183244=CARTESIAN_POINT('Ctrl Pts',(4.5111957254623,46.3602455280244,-56.1959212366655));
#183245=CARTESIAN_POINT('Ctrl Pts',(4.51088056044139,46.394186514714,-56.2443424456773));
#183246=CARTESIAN_POINT('Ctrl Pts',(4.51055741037206,46.4269428333146,-56.2942019278305));
#183247=CARTESIAN_POINT('Ctrl Pts',(4.5103701770366,46.4459218630936,-56.3230905403786));
#183248=CARTESIAN_POINT('Ctrl Pts',(4.5101802797067,46.464503221912,-56.3524615517062));
#183249=CARTESIAN_POINT('Ctrl Pts',(4.50998830130491,46.4826544281561,-56.3822985621361));
#183250=CARTESIAN_POINT('Ctrl Pts',(4.50989231210402,46.4917300312782,-56.397217067351));
#183251=CARTESIAN_POINT('Ctrl Pts',(4.50979580322036,46.5006981216228,-56.4122520571168));
#183252=CARTESIAN_POINT('Ctrl Pts',(4.50969885839879,46.5095546859655,-56.4274011973728));
#183253=CARTESIAN_POINT('Ctrl Pts',(4.509650385988,46.5139829681369,-56.4349757675007));
#183254=CARTESIAN_POINT('Ctrl Pts',(4.50960180463459,46.5183833705597,-56.4425788741622));
#183255=CARTESIAN_POINT('Ctrl Pts',(4.50955312522921,46.5227553995485,-56.450210214626));
#183256=CARTESIAN_POINT('Ctrl Pts',(4.50952878552652,46.5249414140428,-56.4540258848579));
#183257=CARTESIAN_POINT('Ctrl Pts',(4.50950442131329,46.5271203352908,-56.4578486134765));
#183258=CARTESIAN_POINT('Ctrl Pts',(4.509480033991,46.5292921018848,-56.4616783615944));
#183259=CARTESIAN_POINT('Ctrl Pts',(4.50945700999974,46.531342459627,-56.4652940142739));
#183260=CARTESIAN_POINT('Ctrl Pts',(4.50942733452829,46.5339732395003,-56.4699603792029));
#183261=CARTESIAN_POINT('Ctrl Pts',(4.50940978857118,46.5355223682823,-56.472719241285));
#183262=CARTESIAN_POINT('Ctrl Pts',(4.50940874961371,46.5356140976146,-56.4728826031562));
#183263=CARTESIAN_POINT('Ctrl Pts',(4.50940775346655,46.5357020474182,-56.4730392698743));
#183264=CARTESIAN_POINT('Ctrl Pts',(4.50940680411579,46.5357858766478,-56.4731886251067));
#183265=CARTESIAN_POINT('Ctrl Pts',(4.50917570372938,46.5561924199199,-56.5095461584502));
#183266=CARTESIAN_POINT('Ctrl Pts',(4.50893178738087,46.577039509979,-56.5484586717076));
#183267=CARTESIAN_POINT('Ctrl Pts',(4.5086714158295,46.5980094018699,-56.5900119371826));
#183268=CARTESIAN_POINT('Ctrl Pts',(4.5084201314999,46.6182474240276,-56.6301149530582));
#183269=CARTESIAN_POINT('Ctrl Pts',(4.50815349630828,46.6385994455066,-56.6726782274364));
#183270=CARTESIAN_POINT('Ctrl Pts',(4.50786926894805,46.658740870374,-56.7177508957582));
#183271=CARTESIAN_POINT('Ctrl Pts',(4.50759076325134,46.6784768365417,-56.7619162248224));
#183272=CARTESIAN_POINT('Ctrl Pts',(4.50729534264338,46.6980101846824,-56.8084915435727));
#183273=CARTESIAN_POINT('Ctrl Pts',(4.50698225975394,46.7170030890835,-56.8574866815265));
#183274=CARTESIAN_POINT('Ctrl Pts',(4.50667871612507,46.7354173024404,-56.9049889963217));
#183275=CARTESIAN_POINT('Ctrl Pts',(4.50635855369438,46.7533229382722,-56.9547663298399));
#183276=CARTESIAN_POINT('Ctrl Pts',(4.50602267297348,46.7703885525615,-57.0067857649177));
#183277=CARTESIAN_POINT('Ctrl Pts',(4.50570201438208,46.7866807524379,-57.0564476768403));
#183278=CARTESIAN_POINT('Ctrl Pts',(4.50536702439257,46.8022067287499,-57.108153197194));
#183279=CARTESIAN_POINT('Ctrl Pts',(4.50502009884594,46.816664840301,-57.1618313115726));
#183280=CARTESIAN_POINT('Ctrl Pts',(4.50478709911119,46.8263750971247,-57.1978822352764));
#183281=CARTESIAN_POINT('Ctrl Pts',(4.50454874890674,46.8356034052046,-57.2348220520186));
#183282=CARTESIAN_POINT('Ctrl Pts',(4.50430622795092,46.8442569719706,-57.2726173865685));
#183283=CARTESIAN_POINT('Ctrl Pts',(4.50427591283144,46.8453386678164,-57.2773418033873));
#183284=CARTESIAN_POINT('Ctrl Pts',(4.50424553256607,46.8464113858651,-57.282079587099));
#183285=CARTESIAN_POINT('Ctrl Pts',(4.50421509076819,46.8474749396687,-57.2868306384043));
#183286=CARTESIAN_POINT('Ctrl Pts',(4.50418933320097,46.8483748391652,-57.2908506218439));
#183287=CARTESIAN_POINT('Ctrl Pts',(4.50415006884132,46.8497337805172,-57.2969770600281));
#183288=CARTESIAN_POINT('Ctrl Pts',(4.50411307286254,46.850990933455,-57.3027394373521));
#183289=CARTESIAN_POINT('Ctrl Pts',(4.50410634483202,46.8512195573111,-57.3037873742293));
#183290=CARTESIAN_POINT('Ctrl Pts',(4.50409969227911,46.8514449591298,-57.3048232627625));
#183291=CARTESIAN_POINT('Ctrl Pts',(4.50409321069445,46.8516639680635,-57.3058322336321));
#183292=CARTESIAN_POINT('Ctrl Pts',(4.50400896587206,46.8545105510662,-57.3189463987905));
#183293=CARTESIAN_POINT('Ctrl Pts',(4.50392566897696,46.8572242490104,-57.3318723306552));
#183294=CARTESIAN_POINT('Ctrl Pts',(4.50384341100556,46.8598131773404,-57.3446078874438));
#183295=CARTESIAN_POINT('Ctrl Pts',(4.50367889506276,46.8649910340005,-57.3700790010209));
#183296=CARTESIAN_POINT('Ctrl Pts',(4.50351853721598,46.8696701094606,-57.3947885521014));
#183297=CARTESIAN_POINT('Ctrl Pts',(4.50336288846785,46.8739125904307,-57.4187239095837));
#183298=CARTESIAN_POINT('Ctrl Pts',(4.50308835635982,46.8813954469139,-57.4609409156648));
#183299=CARTESIAN_POINT('Ctrl Pts',(4.50282854915127,46.8875224206904,-57.5007475455008));
#183300=CARTESIAN_POINT('Ctrl Pts',(4.50258522254136,46.8926036856479,-57.5381066004158));
#183301=CARTESIAN_POINT('Ctrl Pts',(4.50233588603805,46.8978104521307,-57.5763883819389));
#183302=CARTESIAN_POINT('Ctrl Pts',(4.50210382724618,46.9019194749012,-57.6121009010535));
#183303=CARTESIAN_POINT('Ctrl Pts',(4.50188963153007,46.9052193199389,-57.6452367975947));
#183304=CARTESIAN_POINT('Ctrl Pts',(4.50167067848076,46.9085924552491,-57.6791086495693));
#183305=CARTESIAN_POINT('Ctrl Pts',(4.50147036401527,46.9111201960475,-57.7102888532685));
#183306=CARTESIAN_POINT('Ctrl Pts',(4.50128838525139,46.9130612164935,-57.7387923258709));
#183307=CARTESIAN_POINT('Ctrl Pts',(4.50110143803939,46.9150552313614,-57.7680740102931));
#183308=CARTESIAN_POINT('Ctrl Pts',(4.50093381660528,46.9164301379209,-57.794531453623));
#183309=CARTESIAN_POINT('Ctrl Pts',(4.50078462327284,46.9174129714368,-57.818194171919));
#183310=CARTESIAN_POINT('Ctrl Pts',(4.50063367521126,46.9184073644949,-57.8421351979676));
#183311=CARTESIAN_POINT('Ctrl Pts',(4.50050156910709,46.9190003132005,-57.8632159463878));
#183312=CARTESIAN_POINT('Ctrl Pts',(4.50038716315524,46.9193733106124,-57.8814710357105));
#183313=CARTESIAN_POINT('Ctrl Pts',(4.50027133005522,46.9197509609516,-57.8999538467285));
#183314=CARTESIAN_POINT('Ctrl Pts',(4.50017362402679,46.919903046673,-57.9155405128008));
#183315=CARTESIAN_POINT('Ctrl Pts',(4.50009294576135,46.9199647097641,-57.9282632801726));
#183316=CARTESIAN_POINT('Ctrl Pts',(4.50005896270807,46.9199906833036,-57.9336223255003));
#183317=CARTESIAN_POINT('Ctrl Pts',(4.50002800331669,46.9199999799999,-57.9384731640903));
#183318=CARTESIAN_POINT('Ctrl Pts',(4.5,46.91999998,-57.9428177527387));
#183319=CARTESIAN_POINT('Ctrl Pts',(4.5,46.91999998,-57.9428177527387));
#183320=CARTESIAN_POINT('Ctrl Pts',(4.99999999999999,46.91999998,-57.9428177527387));
#183321=CARTESIAN_POINT('Ctrl Pts',(5.,46.41999998,-57.9428177527387));
#183322=CARTESIAN_POINT('Ctrl Pts',(4.50167566539267,46.91999998,-57.6828458026853));
#183323=CARTESIAN_POINT('Ctrl Pts',(4.99999999999699,46.9183271035242,-57.6832796231231));
#183324=CARTESIAN_POINT('Ctrl Pts',(5.,46.4199999741246,-57.7261203908743));
#183325=CARTESIAN_POINT('Ctrl Pts',(4.50330917749558,46.8867913077729,-57.4284566847483));
#183326=CARTESIAN_POINT('Ctrl Pts',(4.99999999999981,46.8836068729329,-57.4292829235226));
#183327=CARTESIAN_POINT('Ctrl Pts',(5.,46.3923260879484,-57.5140768479069));
#183328=CARTESIAN_POINT('Ctrl Pts',(4.50569802055499,46.7886864007714,-57.055145939945));
#183329=CARTESIAN_POINT('Ctrl Pts',(5.00000000000009,46.7833158134961,-57.0568766116336));
#183330=CARTESIAN_POINT('Ctrl Pts',(5.,46.310571996574,-57.2029077562381));
#183331=CARTESIAN_POINT('Ctrl Pts',(4.50648947498932,46.7474324008918,-56.931237732302));
#183332=CARTESIAN_POINT('Ctrl Pts',(4.99999999999935,46.7414185265942,-56.9334556299756));
#183333=CARTESIAN_POINT('Ctrl Pts',(5.,46.2761936631225,-57.0996254934279));
#183334=CARTESIAN_POINT('Ctrl Pts',(4.50801451396916,46.6501749278894,-56.6920779475246));
#183335=CARTESIAN_POINT('Ctrl Pts',(5.00000000000065,46.6430202500091,-56.6954228782697));
#183336=CARTESIAN_POINT('Ctrl Pts',(5.,46.1951457708619,-56.9002767254212));
#183337=CARTESIAN_POINT('Ctrl Pts',(4.50874992208284,46.5942418273256,-56.5765450470161));
#183338=CARTESIAN_POINT('Ctrl Pts',(4.99999999999985,46.5866051720245,-56.5805088850576));
#183339=CARTESIAN_POINT('Ctrl Pts',(5.,46.1485348528389,-56.8039757263989));
#183340=CARTESIAN_POINT('Ctrl Pts',(4.51087720078722,46.404990940203,-56.2418316606537));
#183341=CARTESIAN_POINT('Ctrl Pts',(5.00000000000027,46.3962887395937,-56.2480691534848));
#183342=CARTESIAN_POINT('Ctrl Pts',(5.,45.9908257800341,-56.5249797415912));
#183343=CARTESIAN_POINT('Ctrl Pts',(4.51220710564129,46.2476195396021,-56.0318427103247));
#183344=CARTESIAN_POINT('Ctrl Pts',(4.99999999999943,46.2385095854938,-56.0395648256266));
#183345=CARTESIAN_POINT('Ctrl Pts',(5.,45.859682945468,-56.349946411749));
#183346=CARTESIAN_POINT('Ctrl Pts',(4.51453310829638,45.888934282536,-55.6636820506581));
#183347=CARTESIAN_POINT('Ctrl Pts',(5.00000000000056,45.8798007876186,-55.6745387763548));
#183348=CARTESIAN_POINT('Ctrl Pts',(5.,45.5607785663138,-56.0430715492057));
#183349=CARTESIAN_POINT('Ctrl Pts',(4.51553991135993,45.6878102784858,-55.5038410313454));
#183350=CARTESIAN_POINT('Ctrl Pts',(5.,45.6790509243108,-55.5161529972778));
#183351=CARTESIAN_POINT('Ctrl Pts',(5.,45.3931752587345,-55.909838595577));
#183352=CARTESIAN_POINT('Ctrl Pts',(4.51638378732469,45.4644662248635,-55.3696531657294));
#183353=CARTESIAN_POINT('Ctrl Pts',(5.00000000000001,45.4562991060438,-55.383243356978));
#183354=CARTESIAN_POINT('Ctrl Pts',(5.,45.207055184053,-55.7979884638099));
#183355=CARTESIAN_POINT('',(4.9999999999955,45.6625902180235,-56.1488949301451));
#183356=CARTESIAN_POINT('Ctrl Pts',(4.51630724703539,45.4845441383311,-55.3818234144752));
#183357=CARTESIAN_POINT('Ctrl Pts',(4.54554286097715,45.4810304530569,-55.3807925506137));
#183358=CARTESIAN_POINT('Ctrl Pts',(4.57492336620464,45.4783968837311,-55.3834494769118));
#183359=CARTESIAN_POINT('Ctrl Pts',(4.60372984498934,45.4767192880502,-55.3896124857592));
#183360=CARTESIAN_POINT('Ctrl Pts',(4.61692192850124,45.4759510239911,-55.3924348691545));
#183361=CARTESIAN_POINT('Ctrl Pts',(4.62999357791384,45.4753830811306,-55.3959918367187));
#183362=CARTESIAN_POINT('Ctrl Pts',(4.64287614689165,45.4750218250454,-55.4002624573002));
#183363=CARTESIAN_POINT('Ctrl Pts',(4.65907655647388,45.4745675292792,-55.4056329546529));
#183364=CARTESIAN_POINT('Ctrl Pts',(4.67498108665864,45.4744400229746,-55.4121331306033));
#183365=CARTESIAN_POINT('Ctrl Pts',(4.69045701352468,45.4746510551925,-55.4197196712408));
#183366=CARTESIAN_POINT('Ctrl Pts',(4.69992582232718,45.4747801733861,-55.4243614289457));
#183367=CARTESIAN_POINT('Ctrl Pts',(4.70923612563516,45.4750360700629,-55.4294108958238));
#183368=CARTESIAN_POINT('Ctrl Pts',(4.71835329427959,45.4754210331403,-55.4348548259434));
#183369=CARTESIAN_POINT('Ctrl Pts',(4.71971079370954,45.4754783521588,-55.4356653990854));
#183370=CARTESIAN_POINT('Ctrl Pts',(4.72106393555446,45.475538528032,-55.4364846672862));
#183371=CARTESIAN_POINT('Ctrl Pts',(4.7224125609678,45.4756015634809,-55.4373125493747));
#183372=CARTESIAN_POINT('Ctrl Pts',(4.72531069163288,45.4757370236061,-55.4390916278676));
#183373=CARTESIAN_POINT('Ctrl Pts',(4.72818974066629,45.4758856810229,-55.4409104977034));
#183374=CARTESIAN_POINT('Ctrl Pts',(4.73104870708458,45.476047465006,-55.4427680187092));
#183375=CARTESIAN_POINT('Ctrl Pts',(4.73524115531564,45.4762847084271,-55.4454919264141));
#183376=CARTESIAN_POINT('Ctrl Pts',(4.7395886482537,45.476560471502,-55.4484311931122));
#183377=CARTESIAN_POINT('Ctrl Pts',(4.7438160849823,45.4768612403157,-55.451409022755));
#183378=CARTESIAN_POINT('Ctrl Pts',(4.74821455107906,45.4771741773306,-55.4545073264238));
#183379=CARTESIAN_POINT('Ctrl Pts',(4.75248292729602,45.4775141874115,-55.4576472006047));
#183380=CARTESIAN_POINT('Ctrl Pts',(4.75633522119668,45.4778490772923,-55.4605795883408));
#183381=CARTESIAN_POINT('Ctrl Pts',(4.75694303796767,45.4779019163776,-55.461042261878));
#183382=CARTESIAN_POINT('Ctrl Pts',(4.75754054294109,45.4779545964434,-55.4614996805176));
#183383=CARTESIAN_POINT('Ctrl Pts',(4.75812666234957,45.4780069577562,-55.4619507724367));
#183384=CARTESIAN_POINT('Ctrl Pts',(4.77386912235803,45.4794133194305,-55.4740665570259));
#183385=CARTESIAN_POINT('Ctrl Pts',(4.78904026416503,45.4812848835081,-55.4875078892351));
#183386=CARTESIAN_POINT('Ctrl Pts',(4.80352937623848,45.483614772575,-55.502161797825));
#183387=CARTESIAN_POINT('Ctrl Pts',(4.81801848831193,45.485944661642,-55.516815706415));
#183388=CARTESIAN_POINT('Ctrl Pts',(4.83182669596583,45.4887279060849,-55.5326796339206));
#183389=CARTESIAN_POINT('Ctrl Pts',(4.84485334429627,45.4919602456486,-55.5496336015971));
#183390=CARTESIAN_POINT('Ctrl Pts',(4.85787999262672,45.4951925852123,-55.5665875692735));
#183391=CARTESIAN_POINT('Ctrl Pts',(4.87012510664492,45.498883128266,-55.584636804503));
#183392=CARTESIAN_POINT('Ctrl Pts',(4.88150057758231,45.5030354799701,-55.6036686664228));
#183393=CARTESIAN_POINT('Ctrl Pts',(4.88174544212233,45.5031248620885,-55.6040783398456));
#183394=CARTESIAN_POINT('Ctrl Pts',(4.88198991600439,45.5032144625561,-55.6044884887332));
#183395=CARTESIAN_POINT('Ctrl Pts',(4.88223399810205,45.5033042813681,-55.6048991117999));
#183396=CARTESIAN_POINT('Ctrl Pts',(4.88765947683183,45.5053007819683,-55.6140264781068));
#183397=CARTESIAN_POINT('Ctrl Pts',(4.8928884876451,45.5074026169808,-55.6233733771008));
#183398=CARTESIAN_POINT('Ctrl Pts',(4.89792023215919,45.5096069594328,-55.6329271738964));
#183399=CARTESIAN_POINT('Ctrl Pts',(4.90054928878365,45.5107587152721,-55.6379189759809));
#183400=CARTESIAN_POINT('Ctrl Pts',(4.90312551250806,45.5119342888916,-55.6429660247168));
#183401=CARTESIAN_POINT('Ctrl Pts',(4.90564745040342,45.5131379411177,-55.6480674173699));
#183402=CARTESIAN_POINT('Ctrl Pts',(4.90715323516841,45.5138566111484,-55.6511133287506));
#183403=CARTESIAN_POINT('Ctrl Pts',(4.90884019027815,45.5146843292354,-55.6545940823321));
#183404=CARTESIAN_POINT('Ctrl Pts',(4.91034649665343,45.5154450020354,-55.6577675133901));
#183405=CARTESIAN_POINT('Ctrl Pts',(4.91136300178359,45.5159583290824,-55.6599090491384));
#183406=CARTESIAN_POINT('Ctrl Pts',(4.91229825558978,45.5164406191502,-55.6619096504392));
#183407=CARTESIAN_POINT('Ctrl Pts',(4.91305024972244,45.5168332118384,-55.6635325496486));
#183408=CARTESIAN_POINT('Ctrl Pts',(4.92411677602688,45.5226107001487,-55.6874155242751));
#183409=CARTESIAN_POINT('Ctrl Pts',(4.93418172838201,45.5290383944735,-55.7127029485112));
#183410=CARTESIAN_POINT('Ctrl Pts',(4.9431758910437,45.5361068199836,-55.7392571266968));
#183411=CARTESIAN_POINT('Ctrl Pts',(4.95243919302711,45.5433867594854,-55.7666059062005));
#183412=CARTESIAN_POINT('Ctrl Pts',(4.96056657366829,45.5513463741598,-55.7952981524042));
#183413=CARTESIAN_POINT('Ctrl Pts',(4.96751435343842,45.5599579987963,-55.8251415997744));
#183414=CARTESIAN_POINT('Ctrl Pts',(4.96956337324642,45.5624977150859,-55.8339429459345));
#183415=CARTESIAN_POINT('Ctrl Pts',(4.97151000621998,45.5650940280755,-55.8428441635502));
#183416=CARTESIAN_POINT('Ctrl Pts',(4.97335365356651,45.5677459505796,-55.8518397101609));
#183417=CARTESIAN_POINT('Ctrl Pts',(4.98019532371398,45.5775870837354,-55.8852216705573));
#183418=CARTESIAN_POINT('Ctrl Pts',(4.98563127466986,45.5881340252677,-55.919722555685));
#183419=CARTESIAN_POINT('Ctrl Pts',(4.98975026681294,45.5993409247369,-55.9553543305821));
#183420=CARTESIAN_POINT('Ctrl Pts',(4.99400798721088,45.6109252742114,-55.9921861888437));
#183421=CARTESIAN_POINT('Ctrl Pts',(4.99685902938038,45.6232147674421,-56.0302270542062));
#183422=CARTESIAN_POINT('Ctrl Pts',(4.99844839489109,45.6361384783249,-56.0694667702205));
#183423=CARTESIAN_POINT('Ctrl Pts',(4.99949969638536,45.6446869943655,-56.0954222674317));
#183424=CARTESIAN_POINT('Ctrl Pts',(4.99999994524809,45.6535125756061,-56.121901794988));
#183425=CARTESIAN_POINT('Ctrl Pts',(4.9999999999955,45.6625902180235,-56.1488949301451));
#183426=CARTESIAN_POINT('Ctrl Pts',(5.,46.41999998,-57.9428177527387));
#183427=CARTESIAN_POINT('Ctrl Pts',(5.,46.41999998,-57.7745740624592));
#183428=CARTESIAN_POINT('Ctrl Pts',(5.00000000017611,46.4033211412152,-57.6091706164621));
#183429=CARTESIAN_POINT('Ctrl Pts',(4.99999999982344,46.3703757696924,-57.4465347800693));
#183430=CARTESIAN_POINT('Ctrl Pts',(4.99999999972182,46.3608819639002,-57.3996683167638));
#183431=CARTESIAN_POINT('Ctrl Pts',(4.99999999967221,46.3500332431698,-57.3530322594102));
#183432=CARTESIAN_POINT('Ctrl Pts',(4.99999999969245,46.3378403217705,-57.3066263304899));
#183433=CARTESIAN_POINT('Ctrl Pts',(4.99999999973771,46.3105877995303,-57.202903968263));
#183434=CARTESIAN_POINT('Ctrl Pts',(4.99999999996081,46.2762003337233,-57.0996231221188));
#183435=CARTESIAN_POINT('Ctrl Pts',(4.9999999999857,46.2356732197596,-56.9999496853278));
#183436=CARTESIAN_POINT('Ctrl Pts',(4.99999999998832,46.2314106238701,-56.9894661462744));
#183437=CARTESIAN_POINT('Ctrl Pts',(4.99999999999009,46.2270807552915,-56.9790199139327));
#183438=CARTESIAN_POINT('Ctrl Pts',(4.99999999999128,46.2226837784916,-56.9686108996226));
#183439=CARTESIAN_POINT('Ctrl Pts',(5.00000000000135,46.1852595852368,-56.8800161717308));
#183440=CARTESIAN_POINT('Ctrl Pts',(5.00000000035917,46.1429808775709,-56.7941365878385));
#183441=CARTESIAN_POINT('Ctrl Pts',(4.99999999927331,46.0959886291946,-56.7109637993559));
#183442=CARTESIAN_POINT('Ctrl Pts',(4.99999999847595,46.061481441272,-56.6498886403374));
#183443=CARTESIAN_POINT('Ctrl Pts',(4.9999999969677,46.0241995329013,-56.5900309298165));
#183444=CARTESIAN_POINT('Ctrl Pts',(4.9999999904409,45.9844424230139,-56.5317775549116));
#183445=CARTESIAN_POINT('Ctrl Pts',(4.99999998658713,45.9609677338277,-56.4973816978229));
#183446=CARTESIAN_POINT('Ctrl Pts',(4.99999998917526,45.9365437147868,-56.4634809785609));
#183447=CARTESIAN_POINT('Ctrl Pts',(4.99999999269503,45.9112549501108,-56.4301707952614));
#183448=CARTESIAN_POINT('Ctrl Pts',(4.99999999800588,45.8730976568612,-56.379910276464));
#183449=CARTESIAN_POINT('Ctrl Pts',(4.99999999856442,45.8329742633927,-56.3309419284987));
#183450=CARTESIAN_POINT('Ctrl Pts',(4.99999999917036,45.7911678591845,-56.2836825816833));
#183451=CARTESIAN_POINT('Ctrl Pts',(4.99999999955207,45.7648322159121,-56.2539118964834));
#183452=CARTESIAN_POINT('Ctrl Pts',(4.99999999973279,45.7378296447702,-56.224818928837));
#183453=CARTESIAN_POINT('Ctrl Pts',(4.99999999986749,45.7102390019053,-56.1965009486372));
#183454=CARTESIAN_POINT('Ctrl Pts',(4.99999999994411,45.6945455669802,-56.1803938074714));
#183455=CARTESIAN_POINT('Ctrl Pts',(5.,45.6786637148754,-56.1645219339327));
#183456=CARTESIAN_POINT('Ctrl Pts',(5.,45.6625994185597,-56.1488914421297));
#183457=CARTESIAN_POINT('Origin',(5.,-9.33460238845303,-92.34995));
#183458=CARTESIAN_POINT('',(5.,45.6625917098448,-60.42825533736));
#183459=CARTESIAN_POINT('',(5.,45.6625917098448,-92.34995));
#183460=CARTESIAN_POINT('Origin',(5.,43.4682849810557,-60.2759318175826));
#183461=CARTESIAN_POINT('',(5.,46.41999998,-91.84995));
#183462=CARTESIAN_POINT('Ctrl Pts',(5.,45.6625917098448,-60.42825533736));
#183463=CARTESIAN_POINT('Ctrl Pts',(5.,45.2073007626125,-60.42825533736));
#183464=CARTESIAN_POINT('Ctrl Pts',(5.4533007853959,45.1647773033082,-60.42825533736));
#183465=CARTESIAN_POINT('Ctrl Pts',(5.,45.6625916931772,-60.6471114271654));
#183466=CARTESIAN_POINT('Ctrl Pts',(5.00000000000228,45.2073007505585,-60.5804098497461));
#183467=CARTESIAN_POINT('Ctrl Pts',(5.45330078693253,45.1647773031641,-60.574158272758));
#183468=CARTESIAN_POINT('Ctrl Pts',(5.,45.6152082879987,-60.8619682722934));
#183469=CARTESIAN_POINT('Ctrl Pts',(4.99999999999914,45.1727790578482,-60.730071400192));
#183470=CARTESIAN_POINT('Ctrl Pts',(5.45472878287372,45.1330538591303,-60.717398791161));
#183471=CARTESIAN_POINT('Ctrl Pts',(5.,45.5214348882082,-61.0621827299711));
#183472=CARTESIAN_POINT('Ctrl Pts',(4.99999999999999,45.1055585268382,-60.8674008824012));
#183473=CARTESIAN_POINT('Ctrl Pts',(5.45757488824865,45.0702713246265,-60.8508735991007));
#183474=CARTESIAN_POINT('',(5.4533007853959,45.1647773033082,-60.42825533736));
#183475=CARTESIAN_POINT('Origin',(5.5,45.6625917098448,-60.42825533736));
#183476=CARTESIAN_POINT('Origin',(5.51981953730066,43.6973226909656,-60.3269478376544));
#183477=CARTESIAN_POINT('Origin',(0.,-12.9675000200281,-60.64995));
#183478=CARTESIAN_POINT('Origin',(1.1373643128445E-15,-12.9675000200281,
-90.9273317382593));
#183479=CARTESIAN_POINT('Origin',(0.,-12.9675000200281,-60.8508735991007));
#183480=CARTESIAN_POINT('Origin',(12.,-9.33460238845303,-92.34995));
#183481=CARTESIAN_POINT('',(12.,44.7861808691872,-60.42825533736));
#183482=CARTESIAN_POINT('Origin',(12.0000005388087,43.3853963400085,-60.456295971705));
#183483=CARTESIAN_POINT('',(12.,44.7862606093016,-55.9010529569358));
#183484=CARTESIAN_POINT('',(12.,44.7861808691872,-92.34995));
#183485=CARTESIAN_POINT('Ctrl Pts',(12.,44.7862606093016,-55.9010529569358));
#183486=CARTESIAN_POINT('Ctrl Pts',(12.,44.8788753121608,-55.9352619713498));
#183487=CARTESIAN_POINT('Ctrl Pts',(11.9999999998966,44.9692347958784,-55.9749445041685));
#183488=CARTESIAN_POINT('Ctrl Pts',(12.0000000001034,45.0573639465224,-56.0200426809281));
#183489=CARTESIAN_POINT('Ctrl Pts',(12.0000000001611,45.0819593060274,-56.0326288214085));
#183490=CARTESIAN_POINT('Ctrl Pts',(12.0000000002553,45.1063808622814,-56.0456370713455));
#183491=CARTESIAN_POINT('Ctrl Pts',(12.0000000004528,45.1306289434624,-56.0590668658914));
#183492=CARTESIAN_POINT('Ctrl Pts',(12.0000000005851,45.1468544406639,-56.0680533540261));
#183493=CARTESIAN_POINT('Ctrl Pts',(12.0000000007159,45.1630095639554,-56.0772339702067));
#183494=CARTESIAN_POINT('Ctrl Pts',(12.0000000008214,45.179090134652,-56.0866066905108));
#183495=CARTESIAN_POINT('Ctrl Pts',(12.0000000011901,45.2352779195468,-56.1193562988592));
#183496=CARTESIAN_POINT('Ctrl Pts',(12.0000000011541,45.2902554021732,-56.1543787808435));
#183497=CARTESIAN_POINT('Ctrl Pts',(12.0000000008796,45.3436294771401,-56.1913642361008));
#183498=CARTESIAN_POINT('Ctrl Pts',(12.0000000006945,45.3796048513583,-56.2162932975287));
#183499=CARTESIAN_POINT('Ctrl Pts',(12.0000000004393,45.4148522843584,-56.242113151159));
#183500=CARTESIAN_POINT('Ctrl Pts',(12.0000000002603,45.4492603972454,-56.268719019813));
#183501=CARTESIAN_POINT('Ctrl Pts',(12.0000000001101,45.478118138608,-56.2910330966957));
#183502=CARTESIAN_POINT('Ctrl Pts',(12.0000000000612,45.5064639161954,-56.3139578240496));
#183503=CARTESIAN_POINT('Ctrl Pts',(12.0000000000338,45.5342394837982,-56.3374491395215));
#183504=CARTESIAN_POINT('Ctrl Pts',(11.9999999999739,45.5949303219844,-56.3887786981636));
#183505=CARTESIAN_POINT('Ctrl Pts',(12.,45.653197014409,-56.4429844895137));
#183506=CARTESIAN_POINT('Ctrl Pts',(12.,45.7088856859501,-56.5000343749657));
#183507=CARTESIAN_POINT('Ctrl Pts',(12.,45.7160867166447,-56.5074114224853));
#183508=CARTESIAN_POINT('Ctrl Pts',(12.,45.7232446868781,-56.5148359705657));
#183509=CARTESIAN_POINT('Ctrl Pts',(12.,45.7303593052335,-56.522307900516));
#183510=CARTESIAN_POINT('Ctrl Pts',(12.,45.7679171901077,-56.5617520239876));
#183511=CARTESIAN_POINT('Ctrl Pts',(12.,45.8043465692001,-56.6026021164951));
#183512=CARTESIAN_POINT('Ctrl Pts',(12.,45.8395823893984,-56.6448353261774));
#183513=CARTESIAN_POINT('Ctrl Pts',(12.,45.8717319797964,-56.6833694197455));
#183514=CARTESIAN_POINT('Ctrl Pts',(12.,45.9026476453863,-56.7227444562638));
#183515=CARTESIAN_POINT('Ctrl Pts',(12.,45.9322838293524,-56.7628973708158));
#183516=CARTESIAN_POINT('Ctrl Pts',(12.,45.9443118404631,-56.7791936558878));
#183517=CARTESIAN_POINT('Ctrl Pts',(12.,45.956129209429,-56.7956179995257));
#183518=CARTESIAN_POINT('Ctrl Pts',(12.,45.9677333562169,-56.8121658960379));
#183519=CARTESIAN_POINT('Ctrl Pts',(12.,45.9798251442283,-56.8294091850376));
#183520=CARTESIAN_POINT('Ctrl Pts',(12.,45.9916897000825,-56.8467926205779));
#183521=CARTESIAN_POINT('Ctrl Pts',(12.,46.0033285107085,-56.8643184852531));
#183522=CARTESIAN_POINT('Ctrl Pts',(12.,46.0482762655458,-56.9320013691878));
#183523=CARTESIAN_POINT('Ctrl Pts',(12.,46.0898342762704,-57.0017828740038));
#183524=CARTESIAN_POINT('Ctrl Pts',(12.,46.1278764894322,-57.0734367367491));
#183525=CARTESIAN_POINT('Ctrl Pts',(12.,46.1404078986321,-57.0970400920794));
#183526=CARTESIAN_POINT('Ctrl Pts',(12.,46.1525581757048,-57.1208464092098));
#183527=CARTESIAN_POINT('Ctrl Pts',(12.,46.164323905515,-57.144847012895));
#183528=CARTESIAN_POINT('Ctrl Pts',(12.,46.1884069401605,-57.1939733636938));
#183529=CARTESIAN_POINT('Ctrl Pts',(12.0000000000007,46.2108248057517,-57.2437789527949));
#183530=CARTESIAN_POINT('Ctrl Pts',(12.0000000001545,46.231652580328,-57.2944049984518));
#183531=CARTESIAN_POINT('Ctrl Pts',(12.000000000255,46.245256447615,-57.3274719016804));
#183532=CARTESIAN_POINT('Ctrl Pts',(12.0000000004148,46.2581810194019,-57.360889338337));
#183533=CARTESIAN_POINT('Ctrl Pts',(12.0000000005167,46.2704364630794,-57.3947019825787));
#183534=CARTESIAN_POINT('Ctrl Pts',(12.0000000006197,46.2828321131732,-57.4289014548942));
#183535=CARTESIAN_POINT('Ctrl Pts',(12.0000000006374,46.2944781423922,-57.4633231278189));
#183536=CARTESIAN_POINT('Ctrl Pts',(12.0000000004958,46.3053795309571,-57.4980138584003));
#183537=CARTESIAN_POINT('Ctrl Pts',(12.0000000001659,46.3307739116041,-57.5788246296216));
#183538=CARTESIAN_POINT('Ctrl Pts',(12.0000000000875,46.351920054225,-57.6603617613545));
#183539=CARTESIAN_POINT('Ctrl Pts',(12.0000000000438,46.3688636122321,-57.7426155626079));
#183540=CARTESIAN_POINT('Ctrl Pts',(12.,46.3858667849633,-57.82515876811));
#183541=CARTESIAN_POINT('Ctrl Pts',(12.0000000000021,46.3986378015382,-57.9084239530163));
#183542=CARTESIAN_POINT('Ctrl Pts',(12.0000000000007,46.4071710877912,-57.9924112496634));
#183543=CARTESIAN_POINT('Ctrl Pts',(11.9999999999993,46.4157043740442,-58.0763985463105));
#183544=CARTESIAN_POINT('Ctrl Pts',(12.,46.41999998,-58.1611082160512));
#183545=CARTESIAN_POINT('Ctrl Pts',(12.,46.41999998,-58.2465463958495));
#183546=CARTESIAN_POINT('',(12.,30.5847864844252,-91.84995));
#183547=CARTESIAN_POINT('Ctrl Pts',(11.9999999857978,44.6134318801692,-61.1210441133876));
#183548=CARTESIAN_POINT('Ctrl Pts',(12.0001420550745,44.0869928457662,-60.8415158913112));
#183549=CARTESIAN_POINT('Ctrl Pts',(11.4131406659365,44.1784219329663,-60.890075338912));
#183550=CARTESIAN_POINT('Ctrl Pts',(11.9999999856108,44.7369792722067,-60.8879413106956));
#183551=CARTESIAN_POINT('Ctrl Pts',(12.000145286376,44.1531002254807,-60.6958383983959));
#183552=CARTESIAN_POINT('Ctrl Pts',(11.4054134166098,44.2623189763507,-60.7346949078221));
#183553=CARTESIAN_POINT('Ctrl Pts',(11.9999999855212,44.7966973993881,-60.6286788556915));
#183554=CARTESIAN_POINT('Ctrl Pts',(12.0001468655555,44.1818517612737,-60.5455762622013));
#183555=CARTESIAN_POINT('Ctrl Pts',(11.4017112009619,44.3028668820625,-60.5618538448931));
#183556=CARTESIAN_POINT('Ctrl Pts',(11.9999999855391,44.7848185198866,-60.36167670255));
#183557=CARTESIAN_POINT('Ctrl Pts',(12.0001465537004,44.1760490867645,-60.3893137401235));
#183558=CARTESIAN_POINT('Ctrl Pts',(11.4024481915019,44.294801171802,-60.3838747332568));
#183559=CARTESIAN_POINT('',(11.402356187646,44.2958078622741,-60.42825533736));
#183560=CARTESIAN_POINT('Origin',(11.5321932041777,42.8849831558857,-60.3485062043524));
#183561=CARTESIAN_POINT('Origin',(11.5,44.7861808691872,-60.42825533736));
#183562=CARTESIAN_POINT('Ctrl Pts',(12.,46.41999998,-58.2465463958495));
#183563=CARTESIAN_POINT('Ctrl Pts',(12.,46.91999998,-58.2465463958495));
#183564=CARTESIAN_POINT('Ctrl Pts',(12.5,46.91999998,-58.2465463958495));
#183565=CARTESIAN_POINT('Ctrl Pts',(12.,46.4199999720693,-57.9548688319462));
#183566=CARTESIAN_POINT('Ctrl Pts',(12.0000000000051,46.9205971329195,-57.8963321594437));
#183567=CARTESIAN_POINT('Ctrl Pts',(12.5005968089278,46.91999998,-57.8965394261518));
#183568=CARTESIAN_POINT('Ctrl Pts',(12.,46.3698845360764,-57.6691983000707));
#183569=CARTESIAN_POINT('Ctrl Pts',(12.,46.8609831927853,-57.553339017633));
#183570=CARTESIAN_POINT('Ctrl Pts',(12.5011890520215,46.8598614514991,-57.5537408849781));
#183571=CARTESIAN_POINT('Ctrl Pts',(12.,46.170945649571,-57.1202211534365));
#183572=CARTESIAN_POINT('Ctrl Pts',(12.,46.6232060214067,-56.8937940810153));
#183573=CARTESIAN_POINT('Ctrl Pts',(12.5023407943396,46.6211347792778,-56.8949802448316));
#183574=CARTESIAN_POINT('Ctrl Pts',(12.,46.0263211387953,-56.8686580359845));
#183575=CARTESIAN_POINT('Ctrl Pts',(11.9999999999992,46.4499499105921,-56.5914299423666));
#183576=CARTESIAN_POINT('Ctrl Pts',(12.5028756040753,46.4475853737583,-56.5931100772464));
#183577=CARTESIAN_POINT('Ctrl Pts',(12.,45.7462130147,-56.5329239712738));
#183578=CARTESIAN_POINT('Ctrl Pts',(12.0000000000004,46.1140832559457,-56.187732860667));
#183579=CARTESIAN_POINT('Ctrl Pts',(12.503595797933,46.111455620038,-56.190236748787));
#183580=CARTESIAN_POINT('Ctrl Pts',(12.,45.64434144227,-56.430563765138));
#183581=CARTESIAN_POINT('Ctrl Pts',(12.0000000000004,45.9918445187629,-56.0645984007596));
#183582=CARTESIAN_POINT('Ctrl Pts',(12.5038165641686,45.9892097344963,-56.0674068194903));
#183583=CARTESIAN_POINT('Ctrl Pts',(12.,45.4241300187908,-56.2443433906185));
#183584=CARTESIAN_POINT('Ctrl Pts',(11.9999999999996,45.7274985396918,-55.840523660562));
#183585=CARTESIAN_POINT('Ctrl Pts',(12.5042197091625,45.7249560267766,-55.8439466125607));
#183586=CARTESIAN_POINT('Ctrl Pts',(12.,45.3048009887765,-56.159928342783));
#183587=CARTESIAN_POINT('Ctrl Pts',(12.,45.584205738319,-55.7389336239012));
#183588=CARTESIAN_POINT('Ctrl Pts',(12.5044033037043,45.5817611915078,-55.7426504905235));
#183589=CARTESIAN_POINT('Ctrl Pts',(12.,44.9276251211566,-55.9400376669437));
#183590=CARTESIAN_POINT('Ctrl Pts',(12.,45.1310727951979,-55.4742001436884));
#183591=CARTESIAN_POINT('Ctrl Pts',(12.5048829251119,45.1291501474361,-55.4787867514921));
#183592=CARTESIAN_POINT('Ctrl Pts',(12.,44.6565552133068,-55.8394367317102));
#183593=CARTESIAN_POINT('Ctrl Pts',(12.0000000000043,44.8053592277238,-55.3530984350278));
#183594=CARTESIAN_POINT('Ctrl Pts',(12.5051042651495,44.8038662560613,-55.3580679820572));
#183595=CARTESIAN_POINT('Ctrl Pts',(12.,44.367939553595,-55.7868701958087));
#183596=CARTESIAN_POINT('Ctrl Pts',(12.,44.4584726259965,-55.289799987766));
#183597=CARTESIAN_POINT('Ctrl Pts',(12.5052199580625,44.4575274683141,-55.2949893590463));
#183598=CARTESIAN_POINT('',(12.5052115665125,44.4820819006474,-55.29956472357));
#183599=CARTESIAN_POINT('Ctrl Pts',(12.,44.7862606093016,-55.9010529569358));
#183600=CARTESIAN_POINT('Ctrl Pts',(12.,44.7810881048319,-55.8832279833769));
#183601=CARTESIAN_POINT('Ctrl Pts',(12.0006703786237,44.7761284457092,-55.8662789181114));
#183602=CARTESIAN_POINT('Ctrl Pts',(12.0018185320163,44.7713976894101,-55.8503503808216));
#183603=CARTESIAN_POINT('Ctrl Pts',(12.0029958851643,44.7665466208536,-55.8340167501054));
#183604=CARTESIAN_POINT('Ctrl Pts',(12.0046741004194,44.7619366243899,-55.8187562997276));
#183605=CARTESIAN_POINT('Ctrl Pts',(12.0066350018515,44.7576008702921,-55.8046721293254));
#183606=CARTESIAN_POINT('Ctrl Pts',(12.0086618529174,44.7531192947929,-55.7901142758176));
#183607=CARTESIAN_POINT('Ctrl Pts',(12.0109892097238,44.7489312326591,-55.776812707229));
#183608=CARTESIAN_POINT('Ctrl Pts',(12.01338895859,44.7450830701278,-55.7648282080662));
#183609=CARTESIAN_POINT('Ctrl Pts',(12.0145579946409,44.7432084403313,-55.7589899673359));
#183610=CARTESIAN_POINT('Ctrl Pts',(12.0157445499893,44.7414145675279,-55.753463543691));
#183611=CARTESIAN_POINT('Ctrl Pts',(12.0169247969219,44.7397070404721,-55.7482523157339));
#183612=CARTESIAN_POINT('Ctrl Pts',(12.0193743177247,44.7361631862757,-55.7374367728701));
#183613=CARTESIAN_POINT('Ctrl Pts',(12.0217934301679,44.7329917135447,-55.727981421325));
#183614=CARTESIAN_POINT('Ctrl Pts',(12.0239997929904,44.7302399365573,-55.719894641493));
#183615=CARTESIAN_POINT('Ctrl Pts',(12.0255011769565,44.728367409607,-55.7143917561773));
#183616=CARTESIAN_POINT('Ctrl Pts',(12.0269049293583,44.7266891531487,-55.7095219207423));
#183617=CARTESIAN_POINT('Ctrl Pts',(12.028166402091,44.7252178005542,-55.7052830189335));
#183618=CARTESIAN_POINT('Ctrl Pts',(12.0297240387712,44.7234010091868,-55.7000489232846));
#183619=CARTESIAN_POINT('Ctrl Pts',(12.0310639389098,44.7218999447325,-55.6957766099129));
#183620=CARTESIAN_POINT('Ctrl Pts',(12.032125593107,44.7207326580353,-55.6924594693962));
#183621=CARTESIAN_POINT('Ctrl Pts',(12.0326564202055,44.7201490146867,-55.6908008991379));
#183622=CARTESIAN_POINT('Ctrl Pts',(12.0331180993725,44.7196487070603,-55.689381107546));
#183623=CARTESIAN_POINT('Ctrl Pts',(12.0335055719087,44.7192332875689,-55.688199347834));
#183624=CARTESIAN_POINT('Ctrl Pts',(12.0336993081768,44.7190255778231,-55.687608467978));
#183625=CARTESIAN_POINT('Ctrl Pts',(12.0338745398092,44.7188390802319,-55.6870771089147));
#183626=CARTESIAN_POINT('Ctrl Pts',(12.0340209511352,44.7186847214685,-55.6866348437614));
#183627=CARTESIAN_POINT('Ctrl Pts',(12.0341565853872,44.7185417247758,-55.6862251329499));
#183628=CARTESIAN_POINT('Ctrl Pts',(12.0342815026087,44.7184086826423,-55.6858404822045));
#183629=CARTESIAN_POINT('Ctrl Pts',(12.0348997710397,44.7177699474642,-55.6840011548822));
#183630=CARTESIAN_POINT('Ctrl Pts',(12.0349488967186,44.7177191955615,-55.6838550076768));
#183631=CARTESIAN_POINT('Ctrl Pts',(12.0350011653746,44.7176652423143,-55.683699681487));
#183632=CARTESIAN_POINT('Ctrl Pts',(12.0350568496592,44.7176078229384,-55.6835344375599));
#183633=CARTESIAN_POINT('Ctrl Pts',(12.0400192739913,44.7124907722303,-55.6688083709579));
#183634=CARTESIAN_POINT('Ctrl Pts',(12.0455323832357,44.7073153008005,-55.6542232562084));
#183635=CARTESIAN_POINT('Ctrl Pts',(12.0515296105903,44.7021205803995,-55.6399679408847));
#183636=CARTESIAN_POINT('Ctrl Pts',(12.0575194673347,44.6969322443252,-55.6257301453858));
#183637=CARTESIAN_POINT('Ctrl Pts',(12.0639919255376,44.6917245922883,-55.6118222192763));
#183638=CARTESIAN_POINT('Ctrl Pts',(12.0708341936134,44.6865526882755,-55.5984147538958));
#183639=CARTESIAN_POINT('Ctrl Pts',(12.0738508627112,44.6842724614794,-55.5925035726843));
#183640=CARTESIAN_POINT('Ctrl Pts',(12.0769388402072,44.6819994029677,-55.5866893624224));
#183641=CARTESIAN_POINT('Ctrl Pts',(12.0800859445827,44.6797392728956,-55.5809850306869));
#183642=CARTESIAN_POINT('Ctrl Pts',(12.0888020038362,44.67347973229,-55.5651866053801));
#183643=CARTESIAN_POINT('Ctrl Pts',(12.0979705023152,44.6673192139475,-55.550233182973));
#183644=CARTESIAN_POINT('Ctrl Pts',(12.107436545151,44.6612968646264,-55.536152291111));
#183645=CARTESIAN_POINT('Ctrl Pts',(12.1121695665689,44.6582856899659,-55.5291118451801));
#183646=CARTESIAN_POINT('Ctrl Pts',(12.1169770158129,44.6553091603234,-55.5222889725919));
#183647=CARTESIAN_POINT('Ctrl Pts',(12.1218401517797,44.6523726449418,-55.5156839551032));
#183648=CARTESIAN_POINT('Ctrl Pts',(12.124271719763,44.650904387251,-55.5123814463588));
#183649=CARTESIAN_POINT('Ctrl Pts',(12.1264248812969,44.6496156231053,-55.5095206617904));
#183650=CARTESIAN_POINT('Ctrl Pts',(12.1287304945814,44.6482552261011,-55.5065159503596));
#183651=CARTESIAN_POINT('Ctrl Pts',(12.1308308081185,44.6470159635314,-55.5037787887829));
#183652=CARTESIAN_POINT('Ctrl Pts',(12.1330577988297,44.6457172533762,-55.5009220320754));
#183653=CARTESIAN_POINT('Ctrl Pts',(12.1357691629899,44.6441547189305,-55.4975308599801));
#183654=CARTESIAN_POINT('Ctrl Pts',(12.136034191219,44.6440019855783,-55.4971993824353));
#183655=CARTESIAN_POINT('Ctrl Pts',(12.1363038761111,44.6438467179213,-55.4968628261204));
#183656=CARTESIAN_POINT('Ctrl Pts',(12.1365785717202,44.6436887155227,-55.496520823035));
#183657=CARTESIAN_POINT('Ctrl Pts',(12.1503224351533,44.635783371146,-55.4794093602218));
#183658=CARTESIAN_POINT('Ctrl Pts',(12.1649684649224,44.6278663758516,-55.4632013862314));
#183659=CARTESIAN_POINT('Ctrl Pts',(12.180359028425,44.6199535701122,-55.4480419954723));
#183660=CARTESIAN_POINT('Ctrl Pts',(12.1957795617725,44.6120253558688,-55.4328530850279));
#183661=CARTESIAN_POINT('Ctrl Pts',(12.2119466676888,44.6041014451226,-55.4187174594865));
#183662=CARTESIAN_POINT('Ctrl Pts',(12.2286720669685,44.5962094010195,-55.4057393699402));
#183663=CARTESIAN_POINT('Ctrl Pts',(12.2455602690405,44.588240536818,-55.3926349534117));
#183664=CARTESIAN_POINT('Ctrl Pts',(12.2630166775616,44.5803043277691,-55.3807110574856));
#183665=CARTESIAN_POINT('Ctrl Pts',(12.2808314202136,44.5724390158208,-55.3700251504023));
#183666=CARTESIAN_POINT('Ctrl Pts',(12.2910044870969,44.5679475479355,-55.3639229883004));
#183667=CARTESIAN_POINT('Ctrl Pts',(12.3012941967153,44.5634793675054,-55.3582235755147));
#183668=CARTESIAN_POINT('Ctrl Pts',(12.3116611113438,44.5590426551015,-55.35293008267));
#183669=CARTESIAN_POINT('Ctrl Pts',(12.330242046542,44.551090601031,-55.3434423950556));
#183670=CARTESIAN_POINT('Ctrl Pts',(12.3490698679653,44.5432394914724,-55.3352615934425));
#183671=CARTESIAN_POINT('Ctrl Pts',(12.367925946783,44.5355401121287,-55.3283642382583));
#183672=CARTESIAN_POINT('Ctrl Pts',(12.3870281440011,44.5277402368681,-55.3213768555534));
#183673=CARTESIAN_POINT('Ctrl Pts',(12.4061584607799,44.5200963409835,-55.315706063824));
#183674=CARTESIAN_POINT('Ctrl Pts',(12.4251133117475,44.5126625795231,-55.3112789150626));
#183675=CARTESIAN_POINT('Ctrl Pts',(12.4445420037074,44.5050429859021,-55.3067410946549));
#183676=CARTESIAN_POINT('Ctrl Pts',(12.4637856538272,44.4976444151584,-55.3035090922607));
#183677=CARTESIAN_POINT('Ctrl Pts',(12.4826620933969,44.4905226144073,-55.3014640358961));
#183678=CARTESIAN_POINT('Ctrl Pts',(12.4902405930691,44.4876633588544,-55.3006429881063));
#183679=CARTESIAN_POINT('Ctrl Pts',(12.4977603698057,44.4848486652911,-55.3000128805774));
#183680=CARTESIAN_POINT('Ctrl Pts',(12.5052115665125,44.4820819006474,-55.29956472357));
#183681=CARTESIAN_POINT('Ctrl Pts',(12.5,46.91999998,-58.2465463958495));
#183682=CARTESIAN_POINT('Ctrl Pts',(12.5001183587732,46.91999998,-58.1771332324744));
#183683=CARTESIAN_POINT('Ctrl Pts',(12.5002387653141,46.9176304364579,-58.1066977317926));
#183684=CARTESIAN_POINT('Ctrl Pts',(12.5003607390257,46.9126568864611,-58.0355338419799));
#183685=CARTESIAN_POINT('Ctrl Pts',(12.5004799036527,46.9077978785483,-57.9660088741151));
#183686=CARTESIAN_POINT('Ctrl Pts',(12.5006005637387,46.9004533625675,-57.8957888763114));
#183687=CARTESIAN_POINT('Ctrl Pts',(12.5007222595679,46.8904542319157,-57.8251501703648));
#183688=CARTESIAN_POINT('Ctrl Pts',(12.5008427738672,46.8805521815852,-57.7551972868673));
#183689=CARTESIAN_POINT('Ctrl Pts',(12.5009643035452,46.8680467092278,-57.6848339807686));
#183690=CARTESIAN_POINT('Ctrl Pts',(12.5010863958673,46.8528241024531,-57.6143279303507));
#183691=CARTESIAN_POINT('Ctrl Pts',(12.5011989872684,46.8387860811076,-57.5493084855601));
#183692=CARTESIAN_POINT('Ctrl Pts',(12.5013120568632,46.8224378094746,-57.4841677663372));
#183693=CARTESIAN_POINT('Ctrl Pts',(12.5014252487982,46.803729758825,-57.4191129723427));
#183694=CARTESIAN_POINT('Ctrl Pts',(12.5014818447657,46.7943757335003,-57.3865855753455));
#183695=CARTESIAN_POINT('Ctrl Pts',(12.5015384713309,46.7844323670111,-57.3540796050202));
#183696=CARTESIAN_POINT('Ctrl Pts',(12.5015950842516,46.7738971294599,-57.3216205428715));
#183697=CARTESIAN_POINT('Ctrl Pts',(12.5016240374496,46.7685091576696,-57.305020204213));
#183698=CARTESIAN_POINT('Ctrl Pts',(12.5016529870829,46.7629664190283,-57.2884321293601));
#183699=CARTESIAN_POINT('Ctrl Pts',(12.5016819272638,46.7572688248593,-57.2718596907753));
#183700=CARTESIAN_POINT('Ctrl Pts',(12.5017002181372,46.7536678116307,-57.2613855206603));
#183701=CARTESIAN_POINT('Ctrl Pts',(12.5017185112997,46.7500037826327,-57.2509141211986));
#183702=CARTESIAN_POINT('Ctrl Pts',(12.5017368193113,46.7462736677078,-57.2404383183051));
#183703=CARTESIAN_POINT('Ctrl Pts',(12.5017461844914,46.7443655851079,-57.2350795833535));
#183704=CARTESIAN_POINT('Ctrl Pts',(12.5017555524955,46.7424404182948,-57.2297203041163));
#183705=CARTESIAN_POINT('Ctrl Pts',(12.5017649231805,46.7404981153884,-57.2243605649049));
#183706=CARTESIAN_POINT('Ctrl Pts',(12.5018983791374,46.7128361149721,-57.1480279250182));
#183707=CARTESIAN_POINT('Ctrl Pts',(12.5020310524357,46.6819657867095,-57.0723595244106));
#183708=CARTESIAN_POINT('Ctrl Pts',(12.5021624247027,46.6478092902251,-56.9976379018118));
#183709=CARTESIAN_POINT('Ctrl Pts',(12.5022609539029,46.6221919178619,-56.9415966848627));
#183710=CARTESIAN_POINT('Ctrl Pts',(12.5023587512966,46.5947268663747,-56.8860878972876));
#183711=CARTESIAN_POINT('Ctrl Pts',(12.5024556013402,46.5653957155416,-56.8312270386029));
#183712=CARTESIAN_POINT('Ctrl Pts',(12.5024879138153,46.5556098440363,-56.8129235865218));
#183713=CARTESIAN_POINT('Ctrl Pts',(12.5025201230294,46.5456156675934,-56.7946910048095));
#183714=CARTESIAN_POINT('Ctrl Pts',(12.502552214228,46.5354149923617,-56.7765373631373));
#183715=CARTESIAN_POINT('Ctrl Pts',(12.5026571797921,46.5020500923837,-56.7171594861959));
#183716=CARTESIAN_POINT('Ctrl Pts',(12.5027607887523,46.46650156848,-56.6586795783787));
#183717=CARTESIAN_POINT('Ctrl Pts',(12.5028626133423,46.4288572096057,-56.6013268548767));
#183718=CARTESIAN_POINT('Ctrl Pts',(12.5029644347431,46.3912140298327,-56.5439759277839));
#183719=CARTESIAN_POINT('Ctrl Pts',(12.5030644713976,46.3514752242191,-56.487752338115));
#183720=CARTESIAN_POINT('Ctrl Pts',(12.5031623352766,46.3097745333203,-56.4328599106678));
#183721=CARTESIAN_POINT('Ctrl Pts',(12.5032057291689,46.2912840002589,-56.4085200203049));
#183722=CARTESIAN_POINT('Ctrl Pts',(12.503248696564,46.2724082816963,-56.3844414254211));
#183723=CARTESIAN_POINT('Ctrl Pts',(12.5032912070703,46.253161566843,-56.3606398144933));
#183724=CARTESIAN_POINT('Ctrl Pts',(12.5033026087216,46.2479994469195,-56.3542560357072));
#183725=CARTESIAN_POINT('Ctrl Pts',(12.5033150347087,46.242326326167,-56.3473004870475));
#183726=CARTESIAN_POINT('Ctrl Pts',(12.5033226268458,46.2371892796758,-56.34105451554));
#183727=CARTESIAN_POINT('Ctrl Pts',(12.5033255608336,46.2352040636999,-56.3386407545504));
#183728=CARTESIAN_POINT('Ctrl Pts',(12.5033277734457,46.2332994091198,-56.3363326367253));
#183729=CARTESIAN_POINT('Ctrl Pts',(12.5033289283955,46.2315374506266,-56.3342029953547));
#183730=CARTESIAN_POINT('Ctrl Pts',(12.5033306780701,46.2288681968597,-56.3309767256823));
#183731=CARTESIAN_POINT('Ctrl Pts',(12.5033324843988,46.2261887108314,-56.3277516232274));
#183732=CARTESIAN_POINT('Ctrl Pts',(12.5033343465982,46.2234989811437,-56.3245277666109));
#183733=CARTESIAN_POINT('Ctrl Pts',(12.5033641174473,46.1804984645187,-56.2729882008824));
#183734=CARTESIAN_POINT('Ctrl Pts',(12.5034073345385,46.1352351800247,-56.2222326288015));
#183735=CARTESIAN_POINT('Ctrl Pts',(12.5034608380734,46.087711103095,-56.1725503029996));
#183736=CARTESIAN_POINT('Ctrl Pts',(12.5035136995659,46.0407573150335,-56.1234641650498));
#183737=CARTESIAN_POINT('Ctrl Pts',(12.503576601829,45.9915966301208,-56.0754257125406));
#183738=CARTESIAN_POINT('Ctrl Pts',(12.5036465507219,45.9402647963719,-56.0286758909813));
#183739=CARTESIAN_POINT('Ctrl Pts',(12.50368351247,45.9131405028007,-56.0039727819793));
#183740=CARTESIAN_POINT('Ctrl Pts',(12.5037224426879,45.8854105601039,-55.9796288363907));
#183741=CARTESIAN_POINT('Ctrl Pts',(12.5037629060975,45.8570841630398,-55.9556751995434));
#183742=CARTESIAN_POINT('Ctrl Pts',(12.5038367165705,45.8054131647529,-55.911980679351));
#183743=CARTESIAN_POINT('Ctrl Pts',(12.5039158143411,45.7515724745622,-55.8694834215562));
#183744=CARTESIAN_POINT('Ctrl Pts',(12.5039972401431,45.6958258044151,-55.8285461839375));
#183745=CARTESIAN_POINT('Ctrl Pts',(12.5040803823153,45.6389040530895,-55.7867460324031));
#183746=CARTESIAN_POINT('Ctrl Pts',(12.5041659501983,45.5799955860921,-55.7465731230012));
#183747=CARTESIAN_POINT('Ctrl Pts',(12.504250825276,45.5194303742208,-55.7083917193762));
#183748=CARTESIAN_POINT('Ctrl Pts',(12.5042720272466,45.5043010585236,-55.6988539254619));
#183749=CARTESIAN_POINT('Ctrl Pts',(12.5042931862015,45.4890685752725,-55.6894402665091));
#183750=CARTESIAN_POINT('Ctrl Pts',(12.5043142540053,45.4737384761356,-55.6801561248251));
#183751=CARTESIAN_POINT('Ctrl Pts',(12.5043337369422,45.4595616137896,-55.6715704009183));
#183752=CARTESIAN_POINT('Ctrl Pts',(12.5043531362203,45.445277774059,-55.6630812139221));
#183753=CARTESIAN_POINT('Ctrl Pts',(12.5043724239116,45.4308917019908,-55.6546944382596));
#183754=CARTESIAN_POINT('Ctrl Pts',(12.5044489649122,45.3738022176376,-55.6214124766727));
#183755=CARTESIAN_POINT('Ctrl Pts',(12.504523615977,45.3153574552296,-55.5898123426925));
#183756=CARTESIAN_POINT('Ctrl Pts',(12.5045949328901,45.2557176044418,-55.5600969950934));
#183757=CARTESIAN_POINT('Ctrl Pts',(12.504667418844,45.1951001255114,-55.5298945476827));
#183758=CARTESIAN_POINT('Ctrl Pts',(12.5047364597886,45.133248026582,-55.5016394962639));
#183759=CARTESIAN_POINT('Ctrl Pts',(12.5048006288673,45.0703524782732,-55.4754938425311));
#183760=CARTESIAN_POINT('Ctrl Pts',(12.504862813151,45.0094023337473,-55.450156892356));
#183761=CARTESIAN_POINT('Ctrl Pts',(12.5049204224477,44.9474724509303,-55.4268007245137));
#183762=CARTESIAN_POINT('Ctrl Pts',(12.5049722441512,44.8847569474852,-55.4055245870557));
#183763=CARTESIAN_POINT('Ctrl Pts',(12.5050265469188,44.8190388184043,-55.383229813499));
#183764=CARTESIAN_POINT('Ctrl Pts',(12.5050744936202,44.7524579555756,-55.3632195169086));
#183765=CARTESIAN_POINT('Ctrl Pts',(12.5051147929775,44.6852599725649,-55.3455504977554));
#183766=CARTESIAN_POINT('Ctrl Pts',(12.5051550923347,44.6180619895543,-55.3278814786021));
#183767=CARTESIAN_POINT('Ctrl Pts',(12.5051877442253,44.550246997649,-55.3125537481411));
#183768=CARTESIAN_POINT('Ctrl Pts',(12.5052115665125,44.4820819006474,-55.29956472357));
#183769=CARTESIAN_POINT('Ctrl Pts',(12.5022360800201,44.4589702388883,-55.2952207669972));
#183770=CARTESIAN_POINT('Ctrl Pts',(12.4974463012635,46.91999998,-55.7446487532608));
#183771=CARTESIAN_POINT('Ctrl Pts',(12.4707855792057,46.91999998,-58.2462412559184));
#183772=CARTESIAN_POINT('Ctrl Pts',(12.6722965314195,44.4249835190402,-55.2908259090661));
#183773=CARTESIAN_POINT('Ctrl Pts',(12.6696732210372,46.9199999799984,-55.7170654011496));
#183774=CARTESIAN_POINT('Ctrl Pts',(12.6482571751841,46.91999998,-58.2481326596478));
#183775=CARTESIAN_POINT('Ctrl Pts',(12.8416972953071,44.3903034748093,-55.2862462023727));
#183776=CARTESIAN_POINT('Ctrl Pts',(12.8404286525071,46.9199999800016,-55.6879841619147));
#183777=CARTESIAN_POINT('Ctrl Pts',(12.8257146119078,46.91999998,-58.2493381002745));
#183778=CARTESIAN_POINT('Ctrl Pts',(13.0103905133279,44.3549359954419,-55.2814750420179));
#183779=CARTESIAN_POINT('Ctrl Pts',(13.0094744794619,46.91999998,-55.6573244385171));
#183780=CARTESIAN_POINT('Ctrl Pts',(13.0031560751435,46.91999998,-58.2497705672942));
#183781=CARTESIAN_POINT('',(13.0012809027682,44.3884783289294,-55.2865616735083));
#183782=CARTESIAN_POINT('Origin',(1.07162825033821,-13.9448070428209,-29.8942234462249));
#183783=CARTESIAN_POINT('Ctrl Pts',(13.0012808995197,44.3884779737753,-55.2865639194009));
#183784=CARTESIAN_POINT('Ctrl Pts',(13.0012784804915,44.4224225696128,-55.291931744549));
#183785=CARTESIAN_POINT('Ctrl Pts',(13.0012795549047,44.4587969009803,-55.2982778660883));
#183786=CARTESIAN_POINT('Ctrl Pts',(13.0012832293302,44.4975897490736,-55.3058907712396));
#183787=CARTESIAN_POINT('Ctrl Pts',(13.001286788091,44.5351614641449,-55.3132640350567));
#183788=CARTESIAN_POINT('Ctrl Pts',(13.0012927856775,44.5750021428636,-55.3218257397261));
#183789=CARTESIAN_POINT('Ctrl Pts',(13.0013003931539,44.6170743841883,-55.3318782262809));
#183790=CARTESIAN_POINT('Ctrl Pts',(13.001307851158,44.6583199869194,-55.3417332008163));
#183791=CARTESIAN_POINT('Ctrl Pts',(13.0013168563583,44.7017107050852,-55.3530210451754));
#183792=CARTESIAN_POINT('Ctrl Pts',(13.0013266117605,44.7471795754749,-55.3660642415441));
#183793=CARTESIAN_POINT('Ctrl Pts',(13.0013360521284,44.7911801048528,-55.3786862297325));
#183794=CARTESIAN_POINT('Ctrl Pts',(13.0013461949353,44.8371270376683,-55.392952211358));
#183795=CARTESIAN_POINT('Ctrl Pts',(13.0013563039396,44.8849248079065,-55.4091878548454));
#183796=CARTESIAN_POINT('Ctrl Pts',(13.0013625568311,44.9144899625084,-55.4192303590746));
#183797=CARTESIAN_POINT('Ctrl Pts',(13.0013687965186,44.9447625482416,-55.4300271052118));
#183798=CARTESIAN_POINT('Ctrl Pts',(13.0013748461807,44.9757120742321,-55.4416614421933));
#183799=CARTESIAN_POINT('Ctrl Pts',(13.0013842994568,45.0240741828949,-55.4598413997633));
#183800=CARTESIAN_POINT('Ctrl Pts',(13.0013931365079,45.0739799904631,-55.480023475315));
#183801=CARTESIAN_POINT('Ctrl Pts',(13.0014006105319,45.1252883103609,-55.5025313874079));
#183802=CARTESIAN_POINT('Ctrl Pts',(13.0014080845559,45.1765966302588,-55.5250392995008));
#183803=CARTESIAN_POINT('Ctrl Pts',(13.0014141955141,45.2293080017412,-55.5498730913657));
#183804=CARTESIAN_POINT('Ctrl Pts',(13.0014181864254,45.2832346253654,-55.5773823016361));
#183805=CARTESIAN_POINT('Ctrl Pts',(13.0014212224514,45.324258496423,-55.5983095212391));
#183806=CARTESIAN_POINT('Ctrl Pts',(13.0014229932898,45.3661059324401,-55.620873256131));
#183807=CARTESIAN_POINT('Ctrl Pts',(13.001423187548,45.4086013945452,-55.6451824135397));
#183808=CARTESIAN_POINT('Ctrl Pts',(13.0014233761988,45.4498701797213,-55.6687898611403));
#183809=CARTESIAN_POINT('Ctrl Pts',(13.0014220778889,45.491750347972,-55.6940436013212));
#183810=CARTESIAN_POINT('Ctrl Pts',(13.0014190141657,45.5340352237576,-55.7210302653281));
#183811=CARTESIAN_POINT('Ctrl Pts',(13.0014160783273,45.5745550598512,-55.7468904619577));
#183812=CARTESIAN_POINT('Ctrl Pts',(13.0014115213251,45.6154466101278,-55.7743420547962));
#183813=CARTESIAN_POINT('Ctrl Pts',(13.0014051054231,45.6564831493748,-55.803446918885));
#183814=CARTESIAN_POINT('Ctrl Pts',(13.0014003177448,45.6871054606683,-55.8251655682798));
#183815=CARTESIAN_POINT('Ctrl Pts',(13.0013944950829,45.7178076447179,-55.8478045670992));
#183816=CARTESIAN_POINT('Ctrl Pts',(13.0013875417864,45.7484775027769,-55.8713833924002));
#183817=CARTESIAN_POINT('Ctrl Pts',(13.0013845863314,45.7615135336423,-55.8814054242532));
#183818=CARTESIAN_POINT('Ctrl Pts',(13.0013814246616,45.7745560975569,-55.8916015678972));
#183819=CARTESIAN_POINT('Ctrl Pts',(13.001378047929,45.7876015846557,-55.9019767609528));
#183820=CARTESIAN_POINT('Ctrl Pts',(13.001364045054,45.8416995386273,-55.9450013496182));
#183821=CARTESIAN_POINT('Ctrl Pts',(13.0013463714257,45.8958236427124,-55.9910913928745));
#183822=CARTESIAN_POINT('Ctrl Pts',(13.0013248738051,45.9494882400812,-56.0403852266349));
#183823=CARTESIAN_POINT('Ctrl Pts',(13.0013043548959,46.0007096762087,-56.0874348847192));
#183824=CARTESIAN_POINT('Ctrl Pts',(13.0012803522366,46.05151236301,-56.1374034046404));
#183825=CARTESIAN_POINT('Ctrl Pts',(13.0012527501323,46.1015059085735,-56.1903752317056));
#183826=CARTESIAN_POINT('Ctrl Pts',(13.0012438014241,46.117714008136,-56.2075489015745));
#183827=CARTESIAN_POINT('Ctrl Pts',(13.0012344745285,46.1338373274142,-56.2250379434666));
#183828=CARTESIAN_POINT('Ctrl Pts',(13.0012247659273,46.1498633603297,-56.2428443395582));
#183829=CARTESIAN_POINT('Ctrl Pts',(13.0012122281624,46.1705595068598,-56.2658396612717));
#183830=CARTESIAN_POINT('Ctrl Pts',(13.0011990522377,46.1910800397285,-56.2893686136245));
#183831=CARTESIAN_POINT('Ctrl Pts',(13.0011852444629,46.2113780675757,-56.3134034792177));
#183832=CARTESIAN_POINT('Ctrl Pts',(13.0011589283363,46.2500639152882,-56.3592113358786));
#183833=CARTESIAN_POINT('Ctrl Pts',(13.0011302667257,46.2880812313484,-56.407022697181));
#183834=CARTESIAN_POINT('Ctrl Pts',(13.0010995292298,46.3251101019611,-56.4566907268017));
#183835=CARTESIAN_POINT('Ctrl Pts',(13.001068713536,46.3622331759606,-56.5064851144921));
#183836=CARTESIAN_POINT('Ctrl Pts',(13.0010358113699,46.3983627102444,-56.5581456580717));
#183837=CARTESIAN_POINT('Ctrl Pts',(13.0010011156225,46.4331522164086,-56.6114777846261));
#183838=CARTESIAN_POINT('Ctrl Pts',(13.00098565621,46.448653405088,-56.6352410238193));
#183839=CARTESIAN_POINT('Ctrl Pts',(13.0009698409937,46.4638882394776,-56.6593355083877));
#183840=CARTESIAN_POINT('Ctrl Pts',(13.0009536972384,46.4788245868152,-56.6837410472069));
#183841=CARTESIAN_POINT('Ctrl Pts',(13.0009158262526,46.5138631629177,-56.7409930185162));
#183842=CARTESIAN_POINT('Ctrl Pts',(13.0008760648962,46.5474441336558,-56.8001434760018));
#183843=CARTESIAN_POINT('Ctrl Pts',(13.0008346277944,46.579354801289,-56.8612467488641));
#183844=CARTESIAN_POINT('Ctrl Pts',(13.0007667564146,46.6316224779404,-56.9613300860422));
#183845=CARTESIAN_POINT('Ctrl Pts',(13.0006948249235,46.6789483102667,-57.0657671806725));
#183846=CARTESIAN_POINT('Ctrl Pts',(13.0006212178572,46.7207925144095,-57.1747907392822));
#183847=CARTESIAN_POINT('Ctrl Pts',(13.0005547235128,46.7585932726127,-57.2732792459199));
#183848=CARTESIAN_POINT('Ctrl Pts',(13.0004873134537,46.7914885412403,-57.3744677788747));
#183849=CARTESIAN_POINT('Ctrl Pts',(13.0004209511923,46.8190634696687,-57.4780082586315));
#183850=CARTESIAN_POINT('Ctrl Pts',(13.0004110986384,46.8231574149527,-57.493380521878));
#183851=CARTESIAN_POINT('Ctrl Pts',(13.0004012692221,46.8271340931422,-57.5088045337419));
#183852=CARTESIAN_POINT('Ctrl Pts',(13.0003914694124,46.8309921521592,-57.5242790574659));
#183853=CARTESIAN_POINT('Ctrl Pts',(13.0003482734639,46.8479978415686,-57.592488212134));
#183854=CARTESIAN_POINT('Ctrl Pts',(13.0003057279034,46.862674870022,-57.6616003148738));
#183855=CARTESIAN_POINT('Ctrl Pts',(13.0002646122398,46.8749074169579,-57.7313289963579));
#183856=CARTESIAN_POINT('Ctrl Pts',(13.0002235302982,46.8871299310971,-57.801000488306));
#183857=CARTESIAN_POINT('Ctrl Pts',(13.0001838760848,46.8969118661664,-57.8712871464115));
#183858=CARTESIAN_POINT('Ctrl Pts',(13.0001464311036,46.9041881318259,-57.9418906507672));
#183859=CARTESIAN_POINT('Ctrl Pts',(13.0001090362543,46.911454655917,-58.0123996301437));
#183860=CARTESIAN_POINT('Ctrl Pts',(13.0000738449037,46.9162221582274,-58.0832241957229));
#183861=CARTESIAN_POINT('Ctrl Pts',(13.0000416366651,46.9184773550183,-58.1540607093264));
#183862=CARTESIAN_POINT('Ctrl Pts',(13.0000271287854,46.919493185916,-58.1859683102483));
#183863=CARTESIAN_POINT('Ctrl Pts',(13.0000132261682,46.91999998,-58.2178782852586));
#183864=CARTESIAN_POINT('Ctrl Pts',(13.,46.91999998,-58.2497627936531));
#183865=CARTESIAN_POINT('Ctrl Pts',(13.,46.91999998,-58.2497627936531));
#183866=CARTESIAN_POINT('Ctrl Pts',(13.5,46.9199999800001,-58.2497627936531));
#183867=CARTESIAN_POINT('Ctrl Pts',(13.5,46.41999998,-58.2497627936531));
#183868=CARTESIAN_POINT('Ctrl Pts',(13.0001524477397,46.91999998,-57.8822548982638));
#183869=CARTESIAN_POINT('Ctrl Pts',(13.5,46.9198475451862,-57.8823102041449));
#183870=CARTESIAN_POINT('Ctrl Pts',(13.5,46.4199999716718,-57.9435058971265));
#183871=CARTESIAN_POINT('Ctrl Pts',(13.0003057176052,46.8526943145044,-57.5184560311191));
#183872=CARTESIAN_POINT('Ctrl Pts',(13.5000000000013,46.8524085179432,-57.5185641386525));
#183873=CARTESIAN_POINT('Ctrl Pts',(13.5,46.363911922201,-57.6403398562409));
#183874=CARTESIAN_POINT('Ctrl Pts',(13.0005259614006,46.6548418679923,-57.0029579960184));
#183875=CARTESIAN_POINT('Ctrl Pts',(13.4999999999993,46.6543661205181,-57.0031847607698));
#183876=CARTESIAN_POINT('Ctrl Pts',(13.5,46.1990348882699,-57.2107576948721));
#183877=CARTESIAN_POINT('Ctrl Pts',(13.0005963858014,46.5740565196337,-56.8393464452647));
#183878=CARTESIAN_POINT('Ctrl Pts',(13.5000000000001,46.5735338055633,-56.8396334804064));
#183879=CARTESIAN_POINT('Ctrl Pts',(13.5,46.1317137634759,-57.0744145874655));
#183880=CARTESIAN_POINT('Ctrl Pts',(13.0007311732941,46.3835934539471,-56.5281351595755));
#183881=CARTESIAN_POINT('Ctrl Pts',(13.4999999999999,46.3829981626758,-56.5285611340859));
#183882=CARTESIAN_POINT('Ctrl Pts',(13.5,45.9729945411748,-56.8150715642796));
#183883=CARTESIAN_POINT('Ctrl Pts',(13.0007961467471,46.2725429511699,-56.3791516167841));
#183884=CARTESIAN_POINT('Ctrl Pts',(13.4999999999992,46.2719244986749,-56.3796526797414));
#183885=CARTESIAN_POINT('Ctrl Pts',(13.5,45.8804524549659,-56.6909184744131));
#183886=CARTESIAN_POINT('Ctrl Pts',(13.0009156805798,46.0271849103864,-56.1065360355095));
#183887=CARTESIAN_POINT('Ctrl Pts',(13.5000000000008,46.0265477969208,-56.1071944318285));
#183888=CARTESIAN_POINT('Ctrl Pts',(13.5,45.6759874229978,-56.4637385666375));
#183889=CARTESIAN_POINT('Ctrl Pts',(13.0009702923331,45.8933503604458,-55.9827597531144));
#183890=CARTESIAN_POINT('Ctrl Pts',(13.5,45.892718112414,-55.9834952073023));
#183891=CARTESIAN_POINT('Ctrl Pts',(13.5,45.5644586309065,-56.3605915480362));
#183892=CARTESIAN_POINT('Ctrl Pts',(13.0010689871371,45.6036057246554,-55.7600056274797));
#183893=CARTESIAN_POINT('Ctrl Pts',(13.5,45.6030118434335,-55.7608945639374));
#183894=CARTESIAN_POINT('Ctrl Pts',(13.5,45.3230047666778,-56.1749628998404));
#183895=CARTESIAN_POINT('Ctrl Pts',(13.0011133171869,45.4461379323356,-55.6604821166903));
#183896=CARTESIAN_POINT('Ctrl Pts',(13.5,45.4455768559353,-55.6614429290966));
#183897=CARTESIAN_POINT('Ctrl Pts',(13.5,45.1917816064929,-56.0920265457655));
#183898=CARTESIAN_POINT('Ctrl Pts',(13.0012246935303,44.9574289489744,-55.4111808336381));
#183899=CARTESIAN_POINT('Ctrl Pts',(13.5,44.9570225707288,-55.4123450088757));
#183900=CARTESIAN_POINT('Ctrl Pts',(13.5,44.7845241217188,-55.8842752341532));
#183901=CARTESIAN_POINT('Ctrl Pts',(13.0012724779463,44.6023831565444,-55.3052501647884));
#183902=CARTESIAN_POINT('Ctrl Pts',(13.4999999999989,44.6020983302816,-55.3064963379004));
#183903=CARTESIAN_POINT('Ctrl Pts',(13.5,44.4886526268701,-55.795999572546));
#183904=CARTESIAN_POINT('Ctrl Pts',(13.0012899687735,44.235970178777,-55.2664423715086));
#183905=CARTESIAN_POINT('Ctrl Pts',(13.5,44.2358346644988,-55.2677218601875));
#183906=CARTESIAN_POINT('Ctrl Pts',(13.5,44.1833084789809,-55.7636597096568));
#183907=CARTESIAN_POINT('',(13.5,44.2316053598049,-55.7692503840784));
#183908=CARTESIAN_POINT('Ctrl Pts',(13.0012809046046,44.3884784470435,-55.2865609246976));
#183909=CARTESIAN_POINT('Ctrl Pts',(13.0227142078398,44.3801663262956,-55.2853023719116));
#183910=CARTESIAN_POINT('Ctrl Pts',(13.0440107500575,44.3720139890709,-55.2855217204714));
#183911=CARTESIAN_POINT('Ctrl Pts',(13.0649088497358,44.3641004291774,-55.2871102328437));
#183912=CARTESIAN_POINT('Ctrl Pts',(13.07963394808,44.3585244222926,-55.2882295212604));
#183913=CARTESIAN_POINT('Ctrl Pts',(13.0941615775764,44.3530667901527,-55.2900276155907));
#183914=CARTESIAN_POINT('Ctrl Pts',(13.1084088949827,44.3477516451068,-55.2924539725048));
#183915=CARTESIAN_POINT('Ctrl Pts',(13.1263525788297,44.3410575230077,-55.2955098306798));
#183916=CARTESIAN_POINT('Ctrl Pts',(13.1438410905178,44.3345933820395,-55.2995626257775));
#183917=CARTESIAN_POINT('Ctrl Pts',(13.1606968582402,44.3284113220637,-55.3044726413883));
#183918=CARTESIAN_POINT('Ctrl Pts',(13.1707483356885,44.3247248191731,-55.3074005953086));
#183919=CARTESIAN_POINT('Ctrl Pts',(13.1805753892938,44.3211383949467,-55.3106326202861));
#183920=CARTESIAN_POINT('Ctrl Pts',(13.1901463329097,44.3176608512962,-55.3141329365288));
#183921=CARTESIAN_POINT('Ctrl Pts',(13.2062128737933,44.3118231722252,-55.3200088434692));
#183922=CARTESIAN_POINT('Ctrl Pts',(13.2215361856163,44.3062995177508,-55.3266347825946));
#183923=CARTESIAN_POINT('Ctrl Pts',(13.2360675230861,44.3011033236774,-55.3338157321858));
#183924=CARTESIAN_POINT('Ctrl Pts',(13.2508326372236,44.2958235344816,-55.3411122071695));
#183925=CARTESIAN_POINT('Ctrl Pts',(13.2647743335246,44.2908839262016,-55.3489796349329));
#183926=CARTESIAN_POINT('Ctrl Pts',(13.2778504785041,44.2862936857036,-55.3572086642283));
#183927=CARTESIAN_POINT('Ctrl Pts',(13.2917257824545,44.2814229090171,-55.3659406171754));
#183928=CARTESIAN_POINT('Ctrl Pts',(13.3046252124269,44.276945916979,-55.3750777732145));
#183929=CARTESIAN_POINT('Ctrl Pts',(13.3165555674972,44.2728515348509,-55.3843944010043));
#183930=CARTESIAN_POINT('Ctrl Pts',(13.3257156128518,44.2697078961434,-55.3915476443573));
#183931=CARTESIAN_POINT('Ctrl Pts',(13.334304802766,44.2667896094788,-55.3988066151504));
#183932=CARTESIAN_POINT('Ctrl Pts',(13.3423419835487,44.2640855375983,-55.4060797210799));
#183933=CARTESIAN_POINT('Ctrl Pts',(13.3437380359519,44.2636158422972,-55.4073430542419));
#183934=CARTESIAN_POINT('Ctrl Pts',(13.3447368700783,44.2632803863473,-55.4082577144236));
#183935=CARTESIAN_POINT('Ctrl Pts',(13.3460250420018,44.2628483898243,-55.4094489617215));
#183936=CARTESIAN_POINT('Ctrl Pts',(13.3468856642166,44.2625597747741,-55.4102448290038));
#183937=CARTESIAN_POINT('Ctrl Pts',(13.3478751830343,44.2622281818022,-55.4111644618157));
#183938=CARTESIAN_POINT('Ctrl Pts',(13.3491900716332,44.2617885001658,-55.4124034829403));
#183939=CARTESIAN_POINT('Ctrl Pts',(13.3502012869711,44.2614503629161,-55.413356352382));
#183940=CARTESIAN_POINT('Ctrl Pts',(13.3512075120241,44.2611143783486,-55.4143131401545));
#183941=CARTESIAN_POINT('Ctrl Pts',(13.3522087210251,44.2607805556637,-55.4152737974554));
#183942=CARTESIAN_POINT('Ctrl Pts',(13.3693116047043,44.2550781193665,-55.4316839676167));
#183943=CARTESIAN_POINT('Ctrl Pts',(13.385004867505,44.2499909927695,-55.4493057513444));
#183944=CARTESIAN_POINT('Ctrl Pts',(13.399206340252,44.2455733147497,-55.4677825303627));
#183945=CARTESIAN_POINT('Ctrl Pts',(13.4057661780247,44.2435327340538,-55.4763171855412));
#183946=CARTESIAN_POINT('Ctrl Pts',(13.4120080885646,44.2416347832483,-55.4850348789939));
#183947=CARTESIAN_POINT('Ctrl Pts',(13.4179258006775,44.2398837690247,-55.4939035459242));
#183948=CARTESIAN_POINT('Ctrl Pts',(13.4267579302379,44.2372703967975,-55.5071399477399));
#183949=CARTESIAN_POINT('Ctrl Pts',(13.434866597522,44.2349850099162,-55.5207117442571));
#183950=CARTESIAN_POINT('Ctrl Pts',(13.4422285502336,44.2330409773694,-55.5345026349037));
#183951=CARTESIAN_POINT('Ctrl Pts',(13.4466064922102,44.2318849170109,-55.5427036817486));
#183952=CARTESIAN_POINT('Ctrl Pts',(13.4507229889113,44.2308488595923,-55.5509872047721));
#183953=CARTESIAN_POINT('Ctrl Pts',(13.4545706886585,44.22993571514,-55.5593210232526));
#183954=CARTESIAN_POINT('Ctrl Pts',(13.45698655648,44.2293623761468,-55.564553605112));
#183955=CARTESIAN_POINT('Ctrl Pts',(13.4592960808803,44.2288375697856,-55.5698051015885));
#183956=CARTESIAN_POINT('Ctrl Pts',(13.4614975299841,44.2283617435815,-55.5750655327987));
#183957=CARTESIAN_POINT('Ctrl Pts',(13.4646117992954,44.2276886183467,-55.5825071763295));
#183958=CARTESIAN_POINT('Ctrl Pts',(13.4675178248527,44.2271123449583,-55.5899868231329));
#183959=CARTESIAN_POINT('Ctrl Pts',(13.4702175294607,44.2266320008153,-55.5974728767516));
#183960=CARTESIAN_POINT('Ctrl Pts',(13.4767530004062,44.2254691790824,-55.6155951875323));
#183961=CARTESIAN_POINT('Ctrl Pts',(13.482090699869,44.2248660187073,-55.6337741617638));
#183962=CARTESIAN_POINT('Ctrl Pts',(13.4863540935445,44.2247860760356,-55.6518477306354));
#183963=CARTESIAN_POINT('Ctrl Pts',(13.4884747832457,44.224746311094,-55.6608378531263));
#183964=CARTESIAN_POINT('Ctrl Pts',(13.4903294038769,44.2248360355357,-55.6698027247168));
#183965=CARTESIAN_POINT('Ctrl Pts',(13.4919316006163,44.2250510335979,-55.6787268228452));
#183966=CARTESIAN_POINT('Ctrl Pts',(13.495482214722,44.2255274889129,-55.6985034382359));
#183967=CARTESIAN_POINT('Ctrl Pts',(13.4977914721084,44.2266204765841,-55.7180759667749));
#183968=CARTESIAN_POINT('Ctrl Pts',(13.4989942129331,44.2282757402414,-55.7372300434814));
#183969=CARTESIAN_POINT('Ctrl Pts',(13.4996734185077,44.2292104921684,-55.7480466345614));
#183970=CARTESIAN_POINT('Ctrl Pts',(13.5,44.2303242845141,-55.7587306797949));
#183971=CARTESIAN_POINT('Ctrl Pts',(13.5,44.231605359804,-55.7692503840715));
#183972=CARTESIAN_POINT('Ctrl Pts',(13.5,46.41999998,-58.2497627936531));
#183973=CARTESIAN_POINT('Ctrl Pts',(13.5,46.41999998,-58.1672776827351));
#183974=CARTESIAN_POINT('Ctrl Pts',(13.5,46.4159357655689,-58.0853150765277));
#183975=CARTESIAN_POINT('Ctrl Pts',(13.5,46.4079129436513,-58.0040039069953));
#183976=CARTESIAN_POINT('Ctrl Pts',(13.5,46.3998480609524,-57.9222664521286));
#183977=CARTESIAN_POINT('Ctrl Pts',(13.5,46.3877828714201,-57.8411867135009));
#183978=CARTESIAN_POINT('Ctrl Pts',(13.4999999999999,46.3717717336869,-57.7608954152443));
#183979=CARTESIAN_POINT('Ctrl Pts',(13.4999999999999,46.3557907741678,-57.6807554521413));
#183980=CARTESIAN_POINT('Ctrl Pts',(13.4999999999998,46.3358786103981,-57.6014003971058));
#183981=CARTESIAN_POINT('Ctrl Pts',(13.4999999999993,46.3120383093697,-57.5229684754947));
#183982=CARTESIAN_POINT('Ctrl Pts',(13.499999999999,46.2959527721241,-57.4700488586318));
#183983=CARTESIAN_POINT('Ctrl Pts',(13.4999999999985,46.2780779115088,-57.4175496722019));
#183984=CARTESIAN_POINT('Ctrl Pts',(13.4999999999976,46.2584018781846,-57.3655174652213));
#183985=CARTESIAN_POINT('Ctrl Pts',(13.4999999999975,46.2569427240896,-57.361658811059));
#183986=CARTESIAN_POINT('Ctrl Pts',(13.4999999999974,46.2554739003334,-57.3578033707196));
#183987=CARTESIAN_POINT('Ctrl Pts',(13.4999999999974,46.2539954124749,-57.3539511680007));
#183988=CARTESIAN_POINT('Ctrl Pts',(13.4999999999961,46.219672138924,-57.2645218183184));
#183989=CARTESIAN_POINT('Ctrl Pts',(13.4999999999986,46.1805716042438,-57.1778714284205));
#183990=CARTESIAN_POINT('Ctrl Pts',(13.4999999999971,46.1367457679112,-57.0938423224731));
#183991=CARTESIAN_POINT('Ctrl Pts',(13.4999999999963,46.1131655316061,-57.0486309508129));
#183992=CARTESIAN_POINT('Ctrl Pts',(13.4999999999953,46.0882165583815,-57.0041788421777));
#183993=CARTESIAN_POINT('Ctrl Pts',(13.4999999999852,46.0619014378574,-56.9604643403198));
#183994=CARTESIAN_POINT('Ctrl Pts',(13.499999999984,46.0587398032398,-56.9552122540816));
#183995=CARTESIAN_POINT('Ctrl Pts',(13.4999999999826,46.0555586143243,-56.9499710767904));
#183996=CARTESIAN_POINT('Ctrl Pts',(13.4999999999808,46.0523578866491,-56.9447407904478));
#183997=CARTESIAN_POINT('Ctrl Pts',(13.4999999999437,45.9841670777467,-56.8333106743359));
#183998=CARTESIAN_POINT('Ctrl Pts',(13.4999999995698,45.9062654719836,-56.7259689765119));
#183999=CARTESIAN_POINT('Ctrl Pts',(13.4999999997703,45.8207975744062,-56.6258771140376));
#184000=CARTESIAN_POINT('Ctrl Pts',(13.4999999997905,45.8121551558405,-56.6157559364371));
#184001=CARTESIAN_POINT('Ctrl Pts',(13.4999999998158,45.803435351967,-56.6057089285334));
#184002=CARTESIAN_POINT('Ctrl Pts',(13.4999999998434,45.7946403691178,-56.5957393884661));
#184003=CARTESIAN_POINT('Ctrl Pts',(13.4999999998604,45.7891977407958,-56.5895699050165));
#184004=CARTESIAN_POINT('Ctrl Pts',(13.4999999998752,45.7837267069275,-56.5834303340926));
#184005=CARTESIAN_POINT('Ctrl Pts',(13.4999999998881,45.778227802301,-56.5773214434301));
#184006=CARTESIAN_POINT('Ctrl Pts',(13.5000000001116,45.6828400874147,-56.4713524986363));
#184007=CARTESIAN_POINT('Ctrl Pts',(13.5000000000272,45.5794120988332,-56.3745067808491));
#184008=CARTESIAN_POINT('Ctrl Pts',(13.4999999999695,45.4679575974401,-56.2866310284186));
#184009=CARTESIAN_POINT('Ctrl Pts',(13.4999999999653,45.4599257124734,-56.2802983282937));
#184010=CARTESIAN_POINT('Ctrl Pts',(13.4999999999594,45.4518518043016,-56.2740118496439));
#184011=CARTESIAN_POINT('Ctrl Pts',(13.4999999999509,45.443735968515,-56.2677716701563));
#184012=CARTESIAN_POINT('Ctrl Pts',(13.4999999998703,45.3663292591542,-56.2082544777622));
#184013=CARTESIAN_POINT('Ctrl Pts',(13.4999999992365,45.2845712727012,-56.1527648487191));
#184014=CARTESIAN_POINT('Ctrl Pts',(13.4999999991445,45.2001155591256,-56.102385462588));
#184015=CARTESIAN_POINT('Ctrl Pts',(13.4999999991047,45.1634675983677,-56.0805242801082));
#184016=CARTESIAN_POINT('Ctrl Pts',(13.4999999992486,45.1263121785355,-56.0596248906738));
#184017=CARTESIAN_POINT('Ctrl Pts',(13.4999999995196,45.0887860427418,-56.0397731680737));
#184018=CARTESIAN_POINT('Ctrl Pts',(13.4999999995982,45.0778983802498,-56.0340134794998));
#184019=CARTESIAN_POINT('Ctrl Pts',(13.4999999996575,45.0669811451102,-56.0283421588346));
#184020=CARTESIAN_POINT('Ctrl Pts',(13.4999999997046,45.0560369222135,-56.022760797256));
#184021=CARTESIAN_POINT('Ctrl Pts',(13.4999999999911,44.9893496905531,-55.988751479638));
#184022=CARTESIAN_POINT('Ctrl Pts',(13.4999999999377,44.9212851553068,-55.9578058140961));
#184023=CARTESIAN_POINT('Ctrl Pts',(13.4999999999181,44.8519312666017,-55.9299466722255));
#184024=CARTESIAN_POINT('Ctrl Pts',(13.4999999999016,44.7935541183739,-55.906496837114));
#184025=CARTESIAN_POINT('Ctrl Pts',(13.4999999998496,44.7342628547591,-55.8852345670544));
#184026=CARTESIAN_POINT('Ctrl Pts',(13.4999999998385,44.6741009867898,-55.8662006918549));
#184027=CARTESIAN_POINT('Ctrl Pts',(13.4999999998289,44.6219934836799,-55.8497150383233));
#184028=CARTESIAN_POINT('Ctrl Pts',(13.4999999998617,44.5690884019705,-55.8348617736589));
#184029=CARTESIAN_POINT('Ctrl Pts',(13.4999999998979,44.5156559887646,-55.8217533863186));
#184030=CARTESIAN_POINT('Ctrl Pts',(13.4999999999339,44.4624243034296,-55.8086942428459));
#184031=CARTESIAN_POINT('Ctrl Pts',(13.4999999999687,44.4086696615075,-55.7973670287964));
#184032=CARTESIAN_POINT('Ctrl Pts',(13.4999999999845,44.3546736478472,-55.7878333559404));
#184033=CARTESIAN_POINT('Ctrl Pts',(13.4999999999965,44.3137472492196,-55.7806072873986));
#184034=CARTESIAN_POINT('Ctrl Pts',(13.4999999999993,44.2726825223299,-55.7744105877406));
#184035=CARTESIAN_POINT('Ctrl Pts',(13.4999999999998,44.2316053598049,-55.7692503840784));
#184036=CARTESIAN_POINT('Origin',(13.5,-9.33460238845303,-92.34995));
#184037=CARTESIAN_POINT('',(13.5,44.2316053598056,-60.42825533736));
#184038=CARTESIAN_POINT('',(13.5,44.2316053598056,-92.34995));
#184039=CARTESIAN_POINT('Origin',(13.4999995641033,42.8035277781091,-60.4528540700958));
#184040=CARTESIAN_POINT('',(13.5,46.41999998,-91.84995));
#184041=CARTESIAN_POINT('Ctrl Pts',(13.5000000114112,44.2302441743789,-60.3624063574045));
#184042=CARTESIAN_POINT('Ctrl Pts',(13.4999161431561,43.8380646295733,-60.3801294486319));
#184043=CARTESIAN_POINT('Ctrl Pts',(13.8812391026075,43.7449355503387,-60.3843616038035));
#184044=CARTESIAN_POINT('Ctrl Pts',(13.5000000113849,44.2419957581615,-60.6261785981702));
#184045=CARTESIAN_POINT('Ctrl Pts',(13.4999163945295,43.8475317166231,-60.5727811392321));
#184046=CARTESIAN_POINT('Ctrl Pts',(13.8803600752771,43.7529853273083,-60.5601847150614));
#184047=CARTESIAN_POINT('Ctrl Pts',(13.5000000115167,44.1831007301227,-60.8859969728056));
#184048=CARTESIAN_POINT('Ctrl Pts',(13.4999151269544,43.7997377261502,-60.7643333157514));
#184049=CARTESIAN_POINT('Ctrl Pts',(13.884762026428,43.7126430688856,-60.7334063315744));
#184050=CARTESIAN_POINT('Ctrl Pts',(13.5000000118016,44.056847986027,-61.1216298968641));
#184051=CARTESIAN_POINT('Ctrl Pts',(13.4999123453879,43.7012956163657,-60.9308210213385));
#184052=CARTESIAN_POINT('Ctrl Pts',(13.8942821039575,43.6261495705425,-60.8904677863889));
#184053=CARTESIAN_POINT('',(13.8811292719168,43.7459411239336,-60.42825533736));
#184054=CARTESIAN_POINT('Origin',(14.,44.2316053598056,-60.42825533736));
#184055=CARTESIAN_POINT('Origin',(14.0325246236231,42.3694154213074,-60.3603044162484));
#184056=CARTESIAN_POINT('Origin',(0.,-12.9675000200281,-60.64995));
#184057=CARTESIAN_POINT('Origin',(0.,-12.9675000200281,-60.8508735991007));
#184058=CARTESIAN_POINT('Ctrl Pts',(20.4999999961793,42.2396703210244,-61.1205979678028));
#184059=CARTESIAN_POINT('Ctrl Pts',(20.5000844423969,41.6420275017582,-60.7898798297297));
#184060=CARTESIAN_POINT('Ctrl Pts',(19.8489174898872,41.8225779837155,-60.8897941554007));
#184061=CARTESIAN_POINT('Ctrl Pts',(20.4999999961011,42.3674932175841,-60.8894198661636));
#184062=CARTESIAN_POINT('Ctrl Pts',(20.5000878549352,41.6934063086951,-60.6536629857367));
#184063=CARTESIAN_POINT('Ctrl Pts',(19.8355865710622,41.9126116301234,-60.7356962259096));
#184064=CARTESIAN_POINT('Ctrl Pts',(20.4999999960627,42.4307087138456,-60.6291716490909));
#184065=CARTESIAN_POINT('Ctrl Pts',(20.5000896090864,41.7106252645569,-60.5273413240714));
#184066=CARTESIAN_POINT('Ctrl Pts',(19.8290476963325,41.9571155016239,-60.5621838877489));
#184067=CARTESIAN_POINT('Ctrl Pts',(20.4999999960703,42.4181586164624,-60.3615059809689));
#184068=CARTESIAN_POINT('Ctrl Pts',(20.5000892602553,41.7070302221805,-60.3953720501034));
#184069=CARTESIAN_POINT('Ctrl Pts',(19.8303467534611,41.9482798096484,-60.3837601067579));
#184070=CARTESIAN_POINT('',(19.8301846741669,41.9493820112901,-60.42825533736));
#184071=CARTESIAN_POINT('',(20.5,42.4196614549321,-60.42825533736));
#184072=CARTESIAN_POINT('Origin',(20.,42.4196614549321,-60.42825533736));
#184073=CARTESIAN_POINT('Origin',(20.5000001497348,40.8982420780939,-60.4432551283903));
#184074=CARTESIAN_POINT('Origin',(20.0202631746512,40.6646653164194,-60.3952359560179));
#184075=CARTESIAN_POINT('Origin',(20.5,-9.33460238845303,-92.34995));
#184076=CARTESIAN_POINT('',(20.5,42.4196614549321,-55.74995));
#184077=CARTESIAN_POINT('',(20.5,42.4196614549321,-92.34995));
#184078=CARTESIAN_POINT('',(20.5,43.91999998,-55.74995));
#184079=CARTESIAN_POINT('',(20.5,29.41999998,-91.84995));
#184080=CARTESIAN_POINT('Origin',(21.,-9.33460238845303,-55.74995));
#184081=CARTESIAN_POINT('',(21.,42.0482945870964,-55.24995));
#184082=CARTESIAN_POINT('Ctrl Pts',(20.5,42.4196614549321,-55.74995));
#184083=CARTESIAN_POINT('Ctrl Pts',(20.5,42.4196614516742,-55.7252336462626));
#184084=CARTESIAN_POINT('Ctrl Pts',(20.5018810104879,42.4183057454763,-55.7004056886026));
#184085=CARTESIAN_POINT('Ctrl Pts',(20.5056026268981,42.4156171851572,-55.6757346618476));
#184086=CARTESIAN_POINT('Ctrl Pts',(20.5072707200331,42.4144121257108,-55.6646766790177));
#184087=CARTESIAN_POINT('Ctrl Pts',(20.5093091111243,42.4129389164194,-55.6536504525491));
#184088=CARTESIAN_POINT('Ctrl Pts',(20.5117166035502,42.4111978238051,-55.6426817760817));
#184089=CARTESIAN_POINT('Ctrl Pts',(20.5156059801789,42.408385036172,-55.6249615484114));
#184090=CARTESIAN_POINT('Ctrl Pts',(20.5204586741507,42.4048731188197,-55.6073877775764));
#184091=CARTESIAN_POINT('Ctrl Pts',(20.5262807670998,42.4006531055946,-55.5900728502967));
#184092=CARTESIAN_POINT('Ctrl Pts',(20.5291918135744,42.3985430989821,-55.5814153866568));
#184093=CARTESIAN_POINT('Ctrl Pts',(20.5323453818808,42.396255277344,-55.572822881862));
#184094=CARTESIAN_POINT('Ctrl Pts',(20.5357431944094,42.3937914700978,-55.5643110251239));
#184095=CARTESIAN_POINT('Ctrl Pts',(20.5371996176046,42.3927353947577,-55.5606625408467));
#184096=CARTESIAN_POINT('Ctrl Pts',(20.538779463254,42.3915902962302,-55.5568379466272));
#184097=CARTESIAN_POINT('Ctrl Pts',(20.5403859724756,42.3904256854597,-55.5530872414329));
#184098=CARTESIAN_POINT('Ctrl Pts',(20.5422793680974,42.3890531014094,-55.5486667446824));
#184099=CARTESIAN_POINT('Ctrl Pts',(20.5442112770272,42.3876522392155,-55.5443462699024));
#184100=CARTESIAN_POINT('Ctrl Pts',(20.5459814138442,42.3863675094681,-55.5405139093958));
#184101=CARTESIAN_POINT('Ctrl Pts',(20.5462133215967,42.3861991954794,-55.5400118272385));
#184102=CARTESIAN_POINT('Ctrl Pts',(20.5464423987541,42.3860329144334,-55.5395180940952));
#184103=CARTESIAN_POINT('Ctrl Pts',(20.5466681499119,42.3858690241902,-55.5390335577791));
#184104=CARTESIAN_POINT('Ctrl Pts',(20.5557618200603,42.3792672249949,-55.5195155474249));
#184105=CARTESIAN_POINT('Ctrl Pts',(20.566266949781,42.3716306571955,-55.5003023874531));
#184106=CARTESIAN_POINT('Ctrl Pts',(20.5781780765197,42.3629513503403,-55.481597463984));
#184107=CARTESIAN_POINT('Ctrl Pts',(20.5841379506068,42.3586085558124,-55.4722382328104));
#184108=CARTESIAN_POINT('Ctrl Pts',(20.5904496883736,42.3540047687641,-55.4630069755533));
#184109=CARTESIAN_POINT('Ctrl Pts',(20.5971114211574,42.3491396151076,-55.4539339992414));
#184110=CARTESIAN_POINT('Ctrl Pts',(20.6070992019679,42.3418454035403,-55.4403310971674));
#184111=CARTESIAN_POINT('Ctrl Pts',(20.6178748962852,42.333960942261,-55.4270812214323));
#184112=CARTESIAN_POINT('Ctrl Pts',(20.6294360364031,42.3254888876759,-55.4142951564802));
#184113=CARTESIAN_POINT('Ctrl Pts',(20.6352166064621,42.3212528603834,-55.4079021240042));
#184114=CARTESIAN_POINT('Ctrl Pts',(20.6411936694523,42.3168699308927,-55.4016252063396));
#184115=CARTESIAN_POINT('Ctrl Pts',(20.6473664072578,42.3123400985445,-55.3954807245231));
#184116=CARTESIAN_POINT('Ctrl Pts',(20.6489354846463,42.3111886390568,-55.393918829658));
#184117=CARTESIAN_POINT('Ctrl Pts',(20.6505955882827,42.3099701456555,-55.3922880019796));
#184118=CARTESIAN_POINT('Ctrl Pts',(20.652288151315,42.3087274579678,-55.3906500274103));
#184119=CARTESIAN_POINT('Ctrl Pts',(20.6553966463593,42.3064451863802,-55.3876417874015));
#184120=CARTESIAN_POINT('Ctrl Pts',(20.6586197595993,42.3040773966064,-55.3846084828431));
#184121=CARTESIAN_POINT('Ctrl Pts',(20.6615675916911,42.3019102893165,-55.3819000447302));
#184122=CARTESIAN_POINT('Ctrl Pts',(20.6633290593156,42.3006153412967,-55.3802816262111));
#184123=CARTESIAN_POINT('Ctrl Pts',(20.6649914729747,42.2993926349966,-55.3787783400392));
#184124=CARTESIAN_POINT('Ctrl Pts',(20.6664667151896,42.2983070444802,-55.3774588325365));
#184125=CARTESIAN_POINT('Ctrl Pts',(20.6795781583414,42.2886586910115,-55.3657315057044));
#184126=CARTESIAN_POINT('Ctrl Pts',(20.693699816926,42.2782395230549,-55.3543567742932));
#184127=CARTESIAN_POINT('Ctrl Pts',(20.7088448932229,42.2670360188918,-55.3435177790002));
#184128=CARTESIAN_POINT('Ctrl Pts',(20.7181341509916,42.2601643309555,-55.3368696631865));
#184129=CARTESIAN_POINT('Ctrl Pts',(20.7278079142016,42.2529979095219,-55.3304237404641));
#184130=CARTESIAN_POINT('Ctrl Pts',(20.73786336317,42.2455375240791,-55.3242291726904));
#184131=CARTESIAN_POINT('Ctrl Pts',(20.7510882195251,42.2357256771745,-55.3160821203563));
#184132=CARTESIAN_POINT('Ctrl Pts',(20.7649759751849,42.2254056105031,-55.3083675584016));
#184133=CARTESIAN_POINT('Ctrl Pts',(20.7795148740232,42.2145773218488,-55.3012102632954));
#184134=CARTESIAN_POINT('Ctrl Pts',(20.7867843234423,42.2091631775217,-55.2976316157423));
#184135=CARTESIAN_POINT('Ctrl Pts',(20.7942163726021,42.2036219771159,-55.2941925896406));
#184136=CARTESIAN_POINT('Ctrl Pts',(20.8018081090145,42.1979537193815,-55.2909108896379));
#184137=CARTESIAN_POINT('Ctrl Pts',(20.8056039772207,42.1951195905143,-55.2892700396365));
#184138=CARTESIAN_POINT('Ctrl Pts',(20.8094397672318,42.1922536973269,-55.2876685379919));
#184139=CARTESIAN_POINT('Ctrl Pts',(20.81331496872,42.1893560400312,-55.2861087627962));
#184140=CARTESIAN_POINT('Ctrl Pts',(20.8134763372388,42.1892353777464,-55.2860438116927));
#184141=CARTESIAN_POINT('Ctrl Pts',(20.8136400186047,42.1891129814804,-55.2859780296338));
#184142=CARTESIAN_POINT('Ctrl Pts',(20.8138057335169,42.1889890598484,-55.2859115369424));
#184143=CARTESIAN_POINT('Ctrl Pts',(20.8161824273861,42.1872117678775,-55.28495789451));
#184144=CARTESIAN_POINT('Ctrl Pts',(20.818981029976,42.1851178159589,-55.2838618636164));
#184145=CARTESIAN_POINT('Ctrl Pts',(20.8213680973811,42.183330845312,-55.2829496179739));
#184146=CARTESIAN_POINT('Ctrl Pts',(20.8228115398189,42.1822502770544,-55.2823979896155));
#184147=CARTESIAN_POINT('Ctrl Pts',(20.8241039729083,42.1812824064973,-55.2819122535834));
#184148=CARTESIAN_POINT('Ctrl Pts',(20.8250580089822,42.1805677763321,-55.2815563854263));
#184149=CARTESIAN_POINT('Ctrl Pts',(20.8356250604287,42.1726524218427,-55.2776147345526));
#184150=CARTESIAN_POINT('Ctrl Pts',(20.8471636556639,42.1639963345819,-55.2737212004608));
#184151=CARTESIAN_POINT('Ctrl Pts',(20.8597159721465,42.1545594711244,-55.2700623357848));
#184152=CARTESIAN_POINT('Ctrl Pts',(20.8715417960198,42.1456687866585,-55.2666152358575));
#184153=CARTESIAN_POINT('Ctrl Pts',(20.8842679311292,42.1360846843665,-55.2633765413884));
#184154=CARTESIAN_POINT('Ctrl Pts',(20.8979055823712,42.1257902400343,-55.2605340913107));
#184155=CARTESIAN_POINT('Ctrl Pts',(20.910887194157,42.1159910101303,-55.2578283773446));
#184156=CARTESIAN_POINT('Ctrl Pts',(20.9246952124769,42.1055477777859,-55.2554817619339));
#184157=CARTESIAN_POINT('Ctrl Pts',(20.9393096591675,42.0944667980502,-55.2536848471438));
#184158=CARTESIAN_POINT('Ctrl Pts',(20.9530056083917,42.0840822423413,-55.2520008659267));
#184159=CARTESIAN_POINT('Ctrl Pts',(20.9674100846602,42.0731373698124,-55.2507997850775));
#184160=CARTESIAN_POINT('Ctrl Pts',(20.9824748540747,42.0616599653893,-55.2502628085272));
#184161=CARTESIAN_POINT('Ctrl Pts',(20.9882222136164,42.0572812213137,-55.2500579466262));
#184162=CARTESIAN_POINT('Ctrl Pts',(20.9940653121634,42.0528252294229,-55.24995));
#184163=CARTESIAN_POINT('Ctrl Pts',(21.,42.0482945870964,-55.24995));
#184164=CARTESIAN_POINT('',(21.,41.7028772994424,-55.24995));
#184165=CARTESIAN_POINT('Origin',(0.,0.,-55.24995));
#184166=CARTESIAN_POINT('',(21.5,41.8548280612684,-55.24995));
#184167=CARTESIAN_POINT('Origin',(0.,-12.9675000200281,-55.24995));
#184168=CARTESIAN_POINT('',(21.5,43.91999998,-55.24995));
#184169=CARTESIAN_POINT('Origin',(21.5,0.,-55.74995));
#184170=CARTESIAN_POINT('',(22.,41.4520521304013,-55.74995));
#184171=CARTESIAN_POINT('Ctrl Pts',(21.5,41.8548280612684,-55.24995));
#184172=CARTESIAN_POINT('Ctrl Pts',(21.583715168139,41.7891659057934,-55.24995));
#184173=CARTESIAN_POINT('Ctrl Pts',(21.6546620826866,41.7342782074004,-55.2706498665447));
#184174=CARTESIAN_POINT('Ctrl Pts',(21.7369340153389,41.6681083454341,-55.3086173399654));
#184175=CARTESIAN_POINT('Ctrl Pts',(21.7605396074291,41.6487453390492,-55.3225002178965));
#184176=CARTESIAN_POINT('Ctrl Pts',(21.7907977214966,41.6237412508776,-55.3430283417078));
#184177=CARTESIAN_POINT('Ctrl Pts',(21.8000301990784,41.616079958388,-55.3498287160269));
#184178=CARTESIAN_POINT('Ctrl Pts',(21.812698596049,41.6055981250051,-55.3597598174085));
#184179=CARTESIAN_POINT('Ctrl Pts',(21.8187378809943,41.6006097346515,-55.3646586201736));
#184180=CARTESIAN_POINT('Ctrl Pts',(21.8252905599244,41.5952318669969,-55.3702183104546));
#184181=CARTESIAN_POINT('Ctrl Pts',(21.8279956516036,41.5930217639502,-55.3725639246649));
#184182=CARTESIAN_POINT('Ctrl Pts',(21.8297763865557,41.5915694057806,-55.374119011126));
#184183=CARTESIAN_POINT('Ctrl Pts',(21.8297528299007,41.5915871184344,-55.3740927601813));
#184184=CARTESIAN_POINT('Ctrl Pts',(21.9448313704802,41.498084291402,-55.4760225654778));
#184185=CARTESIAN_POINT('Ctrl Pts',(22.,41.4520521304013,-55.6193427204272));
#184186=CARTESIAN_POINT('Ctrl Pts',(22.,41.4520521304013,-55.74995));
#184187=CARTESIAN_POINT('',(22.,41.1166950488946,-55.74995));
#184188=CARTESIAN_POINT('Origin',(22.,-9.33460238845303,-92.34995));
#184189=CARTESIAN_POINT('',(22.,41.4520521304013,-60.5010370523947));
#184190=CARTESIAN_POINT('',(22.,41.4520521304013,-92.34995));
#184191=CARTESIAN_POINT('Origin',(22.,40.1816528160858,-60.6046736522147));
#184192=CARTESIAN_POINT('',(22.,46.41999998,-91.84995));
#184193=CARTESIAN_POINT('Ctrl Pts',(22.,41.4520521304013,-60.5010370523947));
#184194=CARTESIAN_POINT('Ctrl Pts',(22.,41.1177283573993,-60.5010370523946));
#184195=CARTESIAN_POINT('Ctrl Pts',(22.3089577584378,40.9899884313956,-60.5010370523947));
#184196=CARTESIAN_POINT('Ctrl Pts',(22.,41.4520521024983,-60.811367390836));
#184197=CARTESIAN_POINT('Ctrl Pts',(22.,41.1177283336776,-60.7368788147381));
#184198=CARTESIAN_POINT('Ctrl Pts',(22.3089577682091,40.9899884273556,-60.7079658702078));
#184199=CARTESIAN_POINT('Ctrl Pts',(22.,41.345292929857,-61.115492429943));
#184200=CARTESIAN_POINT('Ctrl Pts',(21.9999999999979,41.0241336396768,-60.969503986646));
#184201=CARTESIAN_POINT('Ctrl Pts',(22.3211558478618,40.913825471773,-60.9106181484486));
#184202=CARTESIAN_POINT('Ctrl Pts',(22.,41.1573899115079,-61.3627217630986));
#184203=CARTESIAN_POINT('Ctrl Pts',(22.,40.8698280768405,-61.1441646043173));
#184204=CARTESIAN_POINT('Ctrl Pts',(22.3428990418276,40.7794755973204,-61.0754935261973));
#184205=CARTESIAN_POINT('',(22.3089577584378,40.9899884313956,-60.5010370523947));
#184206=CARTESIAN_POINT('Origin',(22.5,41.4520521304013,-60.5010370523947));
#184207=CARTESIAN_POINT('Ctrl Pts',(22.3428990418276,40.7794755973204,-61.0754935261973));
#184208=CARTESIAN_POINT('Ctrl Pts',(22.3377419172472,40.8113411518324,-61.0363878307135));
#184209=CARTESIAN_POINT('Ctrl Pts',(22.3331666192763,40.8396559950365,-60.9954985853989));
#184210=CARTESIAN_POINT('Ctrl Pts',(22.3291795158032,40.8643584296857,-60.9533649602018));
#184211=CARTESIAN_POINT('Ctrl Pts',(22.3251648482087,40.8892316401655,-60.9109400517796));
#184212=CARTESIAN_POINT('Ctrl Pts',(22.3217465334641,40.9104423379139,-60.867253492917));
#184213=CARTESIAN_POINT('Ctrl Pts',(22.318927347672,40.9279527481794,-60.8228093460738));
#184214=CARTESIAN_POINT('Ctrl Pts',(22.3160956734992,40.9455407257593,-60.7781683213132));
#184215=CARTESIAN_POINT('Ctrl Pts',(22.3138684433435,40.9593955910944,-60.7327629502039));
#184216=CARTESIAN_POINT('Ctrl Pts',(22.3122447822525,40.9695040445439,-60.6870577134218));
#184217=CARTESIAN_POINT('Ctrl Pts',(22.3106095906062,40.9796842839609,-60.6410278973498));
#184218=CARTESIAN_POINT('Ctrl Pts',(22.309586567221,40.9860647363956,-60.5946939227373));
#184219=CARTESIAN_POINT('Ctrl Pts',(22.309171148035,40.9886566936033,-60.548483719008));
#184220=CARTESIAN_POINT('Ctrl Pts',(22.3090287948283,40.9895448890273,-60.5326487000593));
#184221=CARTESIAN_POINT('Ctrl Pts',(22.3089577584378,40.9899884313956,-60.5168278168827));
#184222=CARTESIAN_POINT('Ctrl Pts',(22.3089577584378,40.9899884313956,-60.5010370523947));
#184223=CARTESIAN_POINT('Origin',(0.,-12.9675000200281,-61.64995));
#184224=CARTESIAN_POINT('',(23.7057274034393,40.1924568448808,-61.0754935261973));
#184225=CARTESIAN_POINT('Origin',(0.,-12.9675000200281,-61.0754935261978));
#184226=CARTESIAN_POINT('',(25.572468850428,39.5210489290882,-60.8798615124594));
#184227=CARTESIAN_POINT('Ctrl Pts',(23.7057274034393,40.1924568448808,-61.0754935261973));
#184228=CARTESIAN_POINT('Ctrl Pts',(23.7856215193862,40.1568294998727,-61.0754935259541));
#184229=CARTESIAN_POINT('Ctrl Pts',(23.866734154227,40.1215775850188,-61.0739308915428));
#184230=CARTESIAN_POINT('Ctrl Pts',(23.9491177092649,40.08673029059,-61.0708731209178));
#184231=CARTESIAN_POINT('Ctrl Pts',(24.0222987307133,40.0557755618236,-61.0681569140535));
#184232=CARTESIAN_POINT('Ctrl Pts',(24.0964813835287,40.025140878248,-61.064260490718));
#184233=CARTESIAN_POINT('Ctrl Pts',(24.1716800708621,39.9948688249072,-61.0592331555073));
#184234=CARTESIAN_POINT('Ctrl Pts',(24.2654661289297,39.9571142223586,-61.0529631796778));
#184235=CARTESIAN_POINT('Ctrl Pts',(24.3608469638927,39.9199159378361,-61.0449325668214));
#184236=CARTESIAN_POINT('Ctrl Pts',(24.4578931367489,39.8833739107453,-61.0352435975212));
#184237=CARTESIAN_POINT('Ctrl Pts',(24.4948792676916,39.8694470534658,-61.03155094817));
#184238=CARTESIAN_POINT('Ctrl Pts',(24.5321075118773,39.8556158911211,-61.0276175607063));
#184239=CARTESIAN_POINT('Ctrl Pts',(24.5695823113615,39.8418876611333,-61.0234498250998));
#184240=CARTESIAN_POINT('Ctrl Pts',(24.5835560000295,39.8367686474373,-61.0218957503451));
#184241=CARTESIAN_POINT('Ctrl Pts',(24.5985392591505,39.8313093182609,-61.020197828724));
#184242=CARTESIAN_POINT('Ctrl Pts',(24.6125102748754,39.826246917928,-61.0185854547281));
#184243=CARTESIAN_POINT('Ctrl Pts',(24.618761985811,39.8239816092242,-61.0178639541342));
#184244=CARTESIAN_POINT('Ctrl Pts',(24.6248112932983,39.8217952378057,-61.0171600142893));
#184245=CARTESIAN_POINT('Ctrl Pts',(24.6304783782186,39.8197514190012,-61.0164960432401));
#184246=CARTESIAN_POINT('Ctrl Pts',(24.6384559079717,39.8168743445348,-61.0155613742039));
#184247=CARTESIAN_POINT('Ctrl Pts',(24.6464463947879,39.8140013804444,-61.0146162258341));
#184248=CARTESIAN_POINT('Ctrl Pts',(24.6544495579384,39.8111327371535,-61.0136606912691));
#184249=CARTESIAN_POINT('Ctrl Pts',(24.7320816974161,39.7833063750169,-61.0043918320403));
#184250=CARTESIAN_POINT('Ctrl Pts',(24.8111148007942,39.7557842793819,-60.9942079554682));
#184251=CARTESIAN_POINT('Ctrl Pts',(24.8915816511647,39.7286727517594,-60.9832055061413));
#184252=CARTESIAN_POINT('Ctrl Pts',(24.9702730942374,39.7021594084049,-60.9724458130394));
#184253=CARTESIAN_POINT('Ctrl Pts',(25.0503356257557,39.6760387443915,-60.9609030790891));
#184254=CARTESIAN_POINT('Ctrl Pts',(25.1318184288227,39.6504095486071,-60.94871246542));
#184255=CARTESIAN_POINT('Ctrl Pts',(25.2106570898813,39.6256120281047,-60.9369174409121));
#184256=CARTESIAN_POINT('Ctrl Pts',(25.2908253028013,39.6012746209597,-60.9245158192693));
#184257=CARTESIAN_POINT('Ctrl Pts',(25.3723860166305,39.5774858297392,-60.9116744369215));
#184258=CARTESIAN_POINT('Ctrl Pts',(25.4381601942134,39.558301493252,-60.9013185765654));
#184259=CARTESIAN_POINT('Ctrl Pts',(25.5048403019683,39.5394739391454,-60.8906774714747));
#184260=CARTESIAN_POINT('Ctrl Pts',(25.572468850428,39.5210489290882,-60.8798615124595));
#184261=CARTESIAN_POINT('Ctrl Pts',(25.572468850428,39.5210489290882,-60.8798615124595));
#184262=CARTESIAN_POINT('Ctrl Pts',(25.6431029505261,39.5018050733993,-60.8685648702497));
#184263=CARTESIAN_POINT('Ctrl Pts',(25.7138823092578,39.4824629375756,-60.857758843244));
#184264=CARTESIAN_POINT('Ctrl Pts',(25.7847107517024,39.4630487724035,-60.8474361505734));
#184265=CARTESIAN_POINT('Ctrl Pts',(25.8308068264298,39.4504137803346,-60.8407180074614));
#184266=CARTESIAN_POINT('Ctrl Pts',(25.8769227933553,39.4377485444914,-60.834204548861));
#184267=CARTESIAN_POINT('Ctrl Pts',(25.9230504277369,39.4250553877985,-60.8278902493107));
#184268=CARTESIAN_POINT('Ctrl Pts',(26.0189121987724,39.3986766563304,-60.8147679648959));
#184269=CARTESIAN_POINT('Ctrl Pts',(26.1148365047503,39.3721740320321,-60.802503877652));
#184270=CARTESIAN_POINT('Ctrl Pts',(26.2108418493022,39.3455428505808,-60.7910366361297));
#184271=CARTESIAN_POINT('Ctrl Pts',(26.3373732051069,39.3104439765394,-60.7759232523495));
#184272=CARTESIAN_POINT('Ctrl Pts',(26.4640345619824,39.2751247126816,-60.7621958302966));
#184273=CARTESIAN_POINT('Ctrl Pts',(26.5907640035296,39.2396032095401,-60.7497269836428));
#184274=CARTESIAN_POINT('Ctrl Pts',(26.7373460877471,39.1985171296091,-60.7353048453615));
#184275=CARTESIAN_POINT('Ctrl Pts',(26.8840228587755,39.1572049156071,-60.722550892655));
#184276=CARTESIAN_POINT('Ctrl Pts',(27.0306967963677,39.1155727408901,-60.7113062733474));
#184277=CARTESIAN_POINT('Ctrl Pts',(27.0336145588422,39.1147445583301,-60.7110825858348));
#184278=CARTESIAN_POINT('Ctrl Pts',(27.0365323211635,39.1139163090821,-60.710859474163));
#184279=CARTESIAN_POINT('Ctrl Pts',(27.0394500838819,39.1130879917084,-60.7106369372409));
#184280=CARTESIAN_POINT('Ctrl Pts',(27.0975646374211,39.0965899762741,-60.7062045569802));
#184281=CARTESIAN_POINT('Ctrl Pts',(27.1556813189417,39.0800646342817,-60.7020077089736));
#184282=CARTESIAN_POINT('Ctrl Pts',(27.2138073132673,39.063498894174,-60.6980512411089));
#184283=CARTESIAN_POINT('Ctrl Pts',(27.3964586715723,39.0114437858338,-60.6856186928498));
#184284=CARTESIAN_POINT('Ctrl Pts',(27.5792042711961,38.9589865331188,-60.6755585565127));
#184285=CARTESIAN_POINT('Ctrl Pts',(27.761941720716,38.906196118852,-60.6679131829684));
#184286=CARTESIAN_POINT('Ctrl Pts',(27.8960426829491,38.8674561377017,-60.6623026638788));
#184287=CARTESIAN_POINT('Ctrl Pts',(28.0301318919162,38.8285192033564,-60.6579982788021));
#184288=CARTESIAN_POINT('Ctrl Pts',(28.1641720722495,38.7893376413634,-60.65501386678));
#184289=CARTESIAN_POINT('Ctrl Pts',(28.2739136266319,38.7572588609145,-60.6525704650074));
#184290=CARTESIAN_POINT('Ctrl Pts',(28.3836422506653,38.7250861587992,-60.6510040856624));
#184291=CARTESIAN_POINT('Ctrl Pts',(28.493364741833,38.6927858841118,-60.6503273734803));
#184292=CARTESIAN_POINT('Origin',(24.2,-73.08000002,-55.74995));
#184293=CARTESIAN_POINT('',(24.2,-66.6526716808631,-55.24995));
#184294=CARTESIAN_POINT('',(24.2,-73.08000002,-55.24995));
#184295=CARTESIAN_POINT('',(23.7,-67.0923340267327,-55.74995));
#184296=CARTESIAN_POINT('Ctrl Pts',(24.2,-66.6526716808631,-55.24995));
#184297=CARTESIAN_POINT('Ctrl Pts',(24.1759721551885,-66.6743340439622,
-55.24995));
#184298=CARTESIAN_POINT('Ctrl Pts',(24.152826179152,-66.6949988683232,-55.2516491172883));
#184299=CARTESIAN_POINT('Ctrl Pts',(24.13068348082,-66.7146565642086,-55.2547374293595));
#184300=CARTESIAN_POINT('Ctrl Pts',(24.1180297981078,-66.7258901655909,
-55.2565022784524));
#184301=CARTESIAN_POINT('Ctrl Pts',(24.1057033057649,-66.7367955085337,
-55.2587201954649));
#184302=CARTESIAN_POINT('Ctrl Pts',(24.0937224210386,-66.7473756878393,
-55.2613292670619));
#184303=CARTESIAN_POINT('Ctrl Pts',(24.0772492946111,-66.7619229132994,
-55.2649166120082));
#184304=CARTESIAN_POINT('Ctrl Pts',(24.0614340950303,-66.775851731569,-55.2692432542138));
#184305=CARTESIAN_POINT('Ctrl Pts',(24.0463294237835,-66.7891621442409,
-55.274133644209));
#184306=CARTESIAN_POINT('Ctrl Pts',(24.0387770881601,-66.7958173505768,
-55.2765788392066));
#184307=CARTESIAN_POINT('Ctrl Pts',(24.0314022714302,-66.8023179571051,
-55.279164741744));
#184308=CARTESIAN_POINT('Ctrl Pts',(24.0242106428603,-66.8086639704726,
-55.2818681998208));
#184309=CARTESIAN_POINT('Ctrl Pts',(24.0213602322104,-66.811179220518,-55.2829397186873));
#184310=CARTESIAN_POINT('Ctrl Pts',(24.018539123137,-66.8136696853031,-55.2840294773983));
#184311=CARTESIAN_POINT('Ctrl Pts',(24.0157447324672,-66.8161379878207,
-55.2851371841595));
#184312=CARTESIAN_POINT('Ctrl Pts',(24.0114888338122,-66.8198972493579,
-55.2868242380731));
#184313=CARTESIAN_POINT('Ctrl Pts',(24.0073073500582,-66.8235941097571,
-55.2885480177634));
#184314=CARTESIAN_POINT('Ctrl Pts',(24.0031907212466,-66.8272382341148,
-55.2903085862464));
#184315=CARTESIAN_POINT('Ctrl Pts',(23.9829089320758,-66.8451920903692,
-55.2989825474966));
#184316=CARTESIAN_POINT('Ctrl Pts',(23.9642328599911,-66.86178060286,-55.3085399422178));
#184317=CARTESIAN_POINT('Ctrl Pts',(23.9471249453662,-66.8769984520897,
-55.318559493563));
#184318=CARTESIAN_POINT('Ctrl Pts',(23.9412233074604,-66.8822480829084,
-55.3220158916872));
#184319=CARTESIAN_POINT('Ctrl Pts',(23.9355078950893,-66.8873348856796,
-55.3255272894897));
#184320=CARTESIAN_POINT('Ctrl Pts',(23.9299760697225,-66.8922594645355,
-55.3290764557181));
#184321=CARTESIAN_POINT('Ctrl Pts',(23.919192213749,-66.9018595414706,-55.3359952745339));
#184322=CARTESIAN_POINT('Ctrl Pts',(23.9091037294454,-66.9108412221197,
-55.3430586687082));
#184323=CARTESIAN_POINT('Ctrl Pts',(23.8996731398199,-66.9192045149494,
-55.3501525154962));
#184324=CARTESIAN_POINT('Ctrl Pts',(23.8949578450071,-66.9233861613642,
-55.3536994388901));
#184325=CARTESIAN_POINT('Ctrl Pts',(23.8904068208279,-66.9274132107852,
-55.3572541745423));
#184326=CARTESIAN_POINT('Ctrl Pts',(23.8860143747022,-66.9312856634615,
-55.3608037660014));
#184327=CARTESIAN_POINT('Ctrl Pts',(23.8838181516394,-66.9332218897997,
-55.3625785617309));
#184328=CARTESIAN_POINT('Ctrl Pts',(23.8816615756776,-66.9351194669366,
-55.3643520766352));
#184329=CARTESIAN_POINT('Ctrl Pts',(23.8795438764403,-66.9369783948365,
-55.366122790075));
#184330=CARTESIAN_POINT('Ctrl Pts',(23.8784850268217,-66.9379078587864,
-55.3670081467949));
#184331=CARTESIAN_POINT('Ctrl Pts',(23.8774358966177,-66.9388276604262,
-55.3678928035676));
#184332=CARTESIAN_POINT('Ctrl Pts',(23.8763963890696,-66.939737799748,-55.3687765744431));
#184333=CARTESIAN_POINT('Ctrl Pts',(23.8755708968128,-66.9404605582929,
-55.3694783933149));
#184334=CARTESIAN_POINT('Ctrl Pts',(23.8752370420761,-66.9407532450194,
-55.3697629895785));
#184335=CARTESIAN_POINT('Ctrl Pts',(23.8742375999357,-66.9416259151707,
-55.3706224726781));
#184336=CARTESIAN_POINT('Ctrl Pts',(23.8739784867836,-66.9418521616982,
-55.3708453003597));
#184337=CARTESIAN_POINT('Ctrl Pts',(23.8736747333741,-66.9421173022114,
-55.3711069295282));
#184338=CARTESIAN_POINT('Ctrl Pts',(23.8733064912044,-66.9424386456662,
-55.3714251723656));
#184339=CARTESIAN_POINT('Ctrl Pts',(23.8669822397958,-66.9479574508522,
-55.3768907270425));
#184340=CARTESIAN_POINT('Ctrl Pts',(23.8608071175581,-66.9533361614165,
-55.3825025454305));
#184341=CARTESIAN_POINT('Ctrl Pts',(23.854778934738,-66.9585783373303,-55.3882561842759));
#184342=CARTESIAN_POINT('Ctrl Pts',(23.8379273040769,-66.9732327058185,
-55.4043403342882));
#184343=CARTESIAN_POINT('Ctrl Pts',(23.8224506346135,-66.9866238435088,
-55.4213586770294));
#184344=CARTESIAN_POINT('Ctrl Pts',(23.8083326526315,-66.9988025045773,
-55.4391491120011));
#184345=CARTESIAN_POINT('Ctrl Pts',(23.793908545267,-67.0112452400215,-55.4573253035009));
#184346=CARTESIAN_POINT('Ctrl Pts',(23.780902068212,-67.0224228512157,-55.4763077982106));
#184347=CARTESIAN_POINT('Ctrl Pts',(23.7693045786636,-67.0323770023654,
-55.4959754807223));
#184348=CARTESIAN_POINT('Ctrl Pts',(23.7647881472762,-67.0362534654999,
-55.5036347019911));
#184349=CARTESIAN_POINT('Ctrl Pts',(23.7604855416912,-67.0399442097422,
-55.5113983533584));
#184350=CARTESIAN_POINT('Ctrl Pts',(23.7563969204059,-67.0434509476726,
-55.5192611609635));
#184351=CARTESIAN_POINT('Ctrl Pts',(23.7510293947303,-67.0480545792065,
-55.5295834233493));
#184352=CARTESIAN_POINT('Ctrl Pts',(23.7460378255205,-67.0523366189893,
-55.5400629061549));
#184353=CARTESIAN_POINT('Ctrl Pts',(23.7414232710247,-67.0562986848684,
-55.5506824062784));
#184354=CARTESIAN_POINT('Ctrl Pts',(23.7308438701964,-67.0653821799449,
-55.5750288406965));
#184355=CARTESIAN_POINT('Ctrl Pts',(23.7223346138157,-67.07270992344,-55.5998560569635));
#184356=CARTESIAN_POINT('Ctrl Pts',(23.7158399969348,-67.0783500466653,
-55.6249940165964));
#184357=CARTESIAN_POINT('Ctrl Pts',(23.7151405459333,-67.078957471231,-55.6277013003919));
#184358=CARTESIAN_POINT('Ctrl Pts',(23.7144644807411,-67.0795453050864,
-55.630412231224));
#184359=CARTESIAN_POINT('Ctrl Pts',(23.7138117462416,-67.0801136209466,
-55.6331266267316));
#184360=CARTESIAN_POINT('Ctrl Pts',(23.7090188656243,-67.0842866347413,
-55.6530578141074));
#184361=CARTESIAN_POINT('Ctrl Pts',(23.705503143361,-67.0873988103307,-55.6731086055997));
#184362=CARTESIAN_POINT('Ctrl Pts',(23.7032227806793,-67.089434092737,-55.6931075567179));
#184363=CARTESIAN_POINT('Ctrl Pts',(23.7010511586342,-67.0913723213252,
-55.712152844327));
#184364=CARTESIAN_POINT('Ctrl Pts',(23.7,-67.0923340254841,-55.7311508771076));
#184365=CARTESIAN_POINT('Ctrl Pts',(23.7,-67.0923340267327,-55.74995));
#184366=CARTESIAN_POINT('',(23.7,67.7009572055632,-55.74995));
#184367=CARTESIAN_POINT('Origin',(23.7,67.7009572055632,-55.24995));
#184368=CARTESIAN_POINT('',(23.7,-67.0923340267327,-60.42825533736));
#184369=CARTESIAN_POINT('',(23.7,-67.0923340267327,-55.24995));
#184370=CARTESIAN_POINT('Origin',(23.7000000338415,-65.5006105042907,-60.4353544159677));
#184371=CARTESIAN_POINT('',(23.7,-67.2147119299503,-176.84995));
#184372=CARTESIAN_POINT('Ctrl Pts',(23.6999999991391,-67.091907941908,-60.3927543614583));
#184373=CARTESIAN_POINT('Ctrl Pts',(23.7000444961003,-66.3339120499587,
-60.4123961703813));
#184374=CARTESIAN_POINT('Ctrl Pts',(23.0030676793154,-66.6324461755816,
-60.4045898193842));
#184375=CARTESIAN_POINT('Ctrl Pts',(23.6999999991382,-67.0981649919348,
-60.6366434264883));
#184376=CARTESIAN_POINT('Ctrl Pts',(23.7000445996745,-66.3350862497407,
-60.5213661743368));
#184377=CARTESIAN_POINT('Ctrl Pts',(23.0023333098335,-66.6369323384171,
-60.5671687383292));
#184378=CARTESIAN_POINT('Ctrl Pts',(23.6999999991466,-67.0398545336994,
-60.8767984170649));
#184379=CARTESIAN_POINT('Ctrl Pts',(23.7000436587852,-66.3247262225054,
-60.6279370962731));
#184380=CARTESIAN_POINT('Ctrl Pts',(23.0091746715062,-66.5951265090932,
-60.7272889592882));
#184381=CARTESIAN_POINT('Ctrl Pts',(23.6999999991637,-66.9227827756908,
-61.0939974638106));
#184382=CARTESIAN_POINT('Ctrl Pts',(23.7000418676227,-66.2856006592058,
-60.7504731406958));
#184383=CARTESIAN_POINT('Ctrl Pts',(23.0230090051523,-66.5111384208581,
-60.8720725995973));
#184384=CARTESIAN_POINT('',(23.0030142220336,-66.6327727106072,-60.42825533736));
#184385=CARTESIAN_POINT('Origin',(23.2,-67.0923340267327,-60.42825533736));
#184386=CARTESIAN_POINT('Origin',(23.2063851675584,-65.3975925798871,-60.4139429821593));
#184387=CARTESIAN_POINT('Origin',(0.,-12.9675000200281,-60.64995));
#184388=CARTESIAN_POINT('Origin',(0.,-12.9675000200281,-60.8508735991007));
#184389=CARTESIAN_POINT('Origin',(17.05,67.7009572055632,-55.24995));
#184390=CARTESIAN_POINT('',(17.05,-69.2968662511513,-171.871644662643));
#184391=CARTESIAN_POINT('',(17.05,-69.1790215814778,-60.42825533736));
#184392=CARTESIAN_POINT('Origin',(17.0499997344964,-67.70076355866,-60.4478804501376));
#184393=CARTESIAN_POINT('',(17.05,-69.1790215814778,-55.74995));
#184394=CARTESIAN_POINT('',(17.05,-69.1790215814778,-55.24995));
#184395=CARTESIAN_POINT('',(17.05,67.7009572055632,-55.74995));
#184396=CARTESIAN_POINT('Ctrl Pts',(17.0500000072448,-69.0016232241721,
-61.1207587448991));
#184397=CARTESIAN_POINT('Ctrl Pts',(17.0499351254479,-68.6669792326861,
-60.9382791396779));
#184398=CARTESIAN_POINT('Ctrl Pts',(17.4174322081753,-68.5782862263167,
-60.8898940315426));
#184399=CARTESIAN_POINT('Ctrl Pts',(17.0500000070135,-69.1279231312628,
-60.8888915170785));
#184400=CARTESIAN_POINT('Ctrl Pts',(17.0499377736316,-68.768366090799,-60.7724682610327));
#184401=CARTESIAN_POINT('Ctrl Pts',(17.4057007122192,-68.6661491518679,
-60.7353408116852));
#184402=CARTESIAN_POINT('Ctrl Pts',(17.0500000069009,-69.1898773189587,
-60.6289947788348));
#184403=CARTESIAN_POINT('Ctrl Pts',(17.0499390370914,-68.8203021885316,
-60.5773600099809));
#184404=CARTESIAN_POINT('Ctrl Pts',(17.3999941136478,-68.7092345420341,
-60.5620638496915));
#184405=CARTESIAN_POINT('Ctrl Pts',(17.0500000069233,-69.1775691162164,
-60.3615671969807));
#184406=CARTESIAN_POINT('Ctrl Pts',(17.0499387884128,-68.8100686727309,
-60.3786737910309));
#184407=CARTESIAN_POINT('Ctrl Pts',(17.4011286297274,-68.7006746954154,
-60.3838015812945));
#184408=CARTESIAN_POINT('',(17.4009870515814,-68.7017426890012,-60.42825533736));
#184409=CARTESIAN_POINT('Origin',(17.5775644535055,-67.3782391193926,-60.380625282891));
#184410=CARTESIAN_POINT('Origin',(17.55,-69.1790215814778,-60.42825533736));
#184411=CARTESIAN_POINT('Origin',(16.55,67.7009572055632,-55.74995));
#184412=CARTESIAN_POINT('',(16.55,-69.4815262104643,-55.24995));
#184413=CARTESIAN_POINT('Ctrl Pts',(17.05,-69.1790215814778,-55.74995));
#184414=CARTESIAN_POINT('Ctrl Pts',(17.05,-69.1790215814778,-55.6863354647393));
#184415=CARTESIAN_POINT('Ctrl Pts',(17.0376836641811,-69.1872430679557,
-55.62011998619));
#184416=CARTESIAN_POINT('Ctrl Pts',(16.9980239220187,-69.2119075273894,
-55.5253450968975));
#184417=CARTESIAN_POINT('Ctrl Pts',(16.9813062406437,-69.2221843854867,
-55.4945430062267));
#184418=CARTESIAN_POINT('Ctrl Pts',(16.9510291215394,-69.2406827300619,
-55.4508010486414));
#184419=CARTESIAN_POINT('Ctrl Pts',(16.9400731279519,-69.2473626878252,
-55.4366317733573));
#184420=CARTESIAN_POINT('Ctrl Pts',(16.9223801176293,-69.2581533888275,
-55.4161620627276));
#184421=CARTESIAN_POINT('Ctrl Pts',(16.9132191956801,-69.2637414304179,
-55.4061233109409));
#184422=CARTESIAN_POINT('Ctrl Pts',(16.9019928706252,-69.2705980216798,
-55.3947915321209));
#184423=CARTESIAN_POINT('Ctrl Pts',(16.8970676687462,-69.2736088199504,
-55.3900204673471));
#184424=CARTESIAN_POINT('Ctrl Pts',(16.8937590578697,-69.2756320763883,
-55.3868591776192));
#184425=CARTESIAN_POINT('Ctrl Pts',(16.8912710328977,-69.2771542353966,
-55.3845249666426));
#184426=CARTESIAN_POINT('Ctrl Pts',(16.8629500306956,-69.2944853013176,
-55.3581999174045));
#184427=CARTESIAN_POINT('Ctrl Pts',(16.8233316225938,-69.3198754749745,
-55.3266480832757));
#184428=CARTESIAN_POINT('Ctrl Pts',(16.7108981077624,-69.3878244053918,
-55.2724497512768));
#184429=CARTESIAN_POINT('Ctrl Pts',(16.6373202287544,-69.4303831621522,
-55.24995));
#184430=CARTESIAN_POINT('Ctrl Pts',(16.55,-69.4815262104643,-55.24995));
#184431=CARTESIAN_POINT('',(16.55,-73.08000002,-55.24995));
#184432=CARTESIAN_POINT('Origin',(41.5,-73.08000002,-55.24995));
#184433=CARTESIAN_POINT('',(16.05,-69.6255546658886,-55.24995));
#184434=CARTESIAN_POINT('Origin',(0.,-12.9675000200281,-55.24995));
#184435=CARTESIAN_POINT('',(16.05,-73.08000002,-55.24995));
#184436=CARTESIAN_POINT('Origin',(16.05,-73.08000002,-55.74995));
#184437=CARTESIAN_POINT('',(15.55,-69.8993466109593,-55.74995));
#184438=CARTESIAN_POINT('Ctrl Pts',(16.05,-69.6255546658886,-55.24995));
#184439=CARTESIAN_POINT('Ctrl Pts',(16.0288722037061,-69.6375247602604,
-55.24995));
#184440=CARTESIAN_POINT('Ctrl Pts',(16.0083301026716,-69.6490223109434,
-55.2512895581316));
#184441=CARTESIAN_POINT('Ctrl Pts',(15.9885162403179,-69.6600473179374,
-55.2537446520891));
#184442=CARTESIAN_POINT('Ctrl Pts',(15.9681617141798,-69.6713731659234,
-55.2562667385575));
#184443=CARTESIAN_POINT('Ctrl Pts',(15.9485754876161,-69.6822003296312,
-55.2599653874695));
#184444=CARTESIAN_POINT('Ctrl Pts',(15.9298569819113,-69.6925288090609,
-55.2645989361251));
#184445=CARTESIAN_POINT('Ctrl Pts',(15.9103217854581,-69.7033079213419,
-55.2694346470888));
#184446=CARTESIAN_POINT('Ctrl Pts',(15.8917314336212,-69.7135438847403,
-55.2752879340727));
#184447=CARTESIAN_POINT('Ctrl Pts',(15.8741431710191,-69.7232366992563,
-55.2818961829012));
#184448=CARTESIAN_POINT('Ctrl Pts',(15.8560955088269,-69.7331826868751,
-55.2886770369989));
#184449=CARTESIAN_POINT('Ctrl Pts',(15.8391024265034,-69.7425567813175,
-55.2962522526717));
#184450=CARTESIAN_POINT('Ctrl Pts',(15.8231746650905,-69.7513589825835,
-55.3043602027165));
#184451=CARTESIAN_POINT('Ctrl Pts',(15.8066197703906,-69.7605077581903,
-55.3127873919331));
#184452=CARTESIAN_POINT('Ctrl Pts',(15.7912151617321,-69.7690387190412,
-55.321789591021));
#184453=CARTESIAN_POINT('Ctrl Pts',(15.7769270004145,-69.776951865136,-55.3311049965711));
#184454=CARTESIAN_POINT('Ctrl Pts',(15.7738353234149,-69.7786641142653,
-55.3331206670581));
#184455=CARTESIAN_POINT('Ctrl Pts',(15.7707957734989,-69.7803474370327,
-55.3351511317179));
#184456=CARTESIAN_POINT('Ctrl Pts',(15.7678077818739,-69.782001833438,-55.3371939557934));
#184457=CARTESIAN_POINT('Ctrl Pts',(15.756555490458,-69.7882320217404,-55.3448868996478));
#184458=CARTESIAN_POINT('Ctrl Pts',(15.7460352862097,-69.7940519898752,
-55.3527538808861));
#184459=CARTESIAN_POINT('Ctrl Pts',(15.7362087545715,-69.7994617378423,
-55.3606749631784));
#184460=CARTESIAN_POINT('Ctrl Pts',(15.7312954887525,-69.8021666118259,
-55.3646355043245));
#184461=CARTESIAN_POINT('Ctrl Pts',(15.7265554551632,-69.8047689307675,
-55.3686098210218));
#184462=CARTESIAN_POINT('Ctrl Pts',(15.721982899875,-69.8072686946673,-55.3725844185997));
#184463=CARTESIAN_POINT('Ctrl Pts',(15.719696622231,-69.8085185766171,-55.3745717173886));
#184464=CARTESIAN_POINT('Ctrl Pts',(15.7174522181041,-69.8097428198065,
-55.3765590908577));
#184465=CARTESIAN_POINT('Ctrl Pts',(15.7152489034228,-69.8109414242354,
-55.3785449605345));
#184466=CARTESIAN_POINT('Ctrl Pts',(15.7139033590177,-69.8116734011504,
-55.3797577132364));
#184467=CARTESIAN_POINT('Ctrl Pts',(15.7130061596117,-69.812164167094,-55.3805748440141));
#184468=CARTESIAN_POINT('Ctrl Pts',(15.7117619226199,-69.8128381202302,
-55.3817177322528));
#184469=CARTESIAN_POINT('Ctrl Pts',(15.7109687347443,-69.813267758201,-55.382446311374));
#184470=CARTESIAN_POINT('Ctrl Pts',(15.7100347608739,-69.8137718421128,
-55.383307570602));
#184471=CARTESIAN_POINT('Ctrl Pts',(15.7087614611218,-69.8144603212408,
-55.3844965014748));
#184472=CARTESIAN_POINT('Ctrl Pts',(15.6900035624944,-69.8246028047116,
-55.4020115011831));
#184473=CARTESIAN_POINT('Ctrl Pts',(15.6727531453279,-69.8338363960813,
-55.4208270616741));
#184474=CARTESIAN_POINT('Ctrl Pts',(15.6571396559972,-69.84216109535,-55.4406592789784));
#184475=CARTESIAN_POINT('Ctrl Pts',(15.6413283311722,-69.8505912752681,
-55.460742786461));
#184476=CARTESIAN_POINT('Ctrl Pts',(15.6271956225887,-69.8580893843722,
-55.4818682723947));
#184477=CARTESIAN_POINT('Ctrl Pts',(15.6148225747989,-69.8646554226621,
-55.5037374727083));
#184478=CARTESIAN_POINT('Ctrl Pts',(15.6022021547712,-69.8713527346377,
-55.5260439002204));
#184479=CARTESIAN_POINT('Ctrl Pts',(15.5914123584404,-69.8770803337719,
-55.5491234737585));
#184480=CARTESIAN_POINT('Ctrl Pts',(15.5824851075871,-69.8818382200647,
-55.5726654113518));
#184481=CARTESIAN_POINT('Ctrl Pts',(15.573457165996,-69.8866497707038,-55.5964728791855));
#184482=CARTESIAN_POINT('Ctrl Pts',(15.5663337420152,-69.890469610296,-55.6207526467196));
#184483=CARTESIAN_POINT('Ctrl Pts',(15.5610961173292,-69.8932977388412,
-55.6451979426959));
#184484=CARTESIAN_POINT('Ctrl Pts',(15.5557670007162,-69.8961752697293,
-55.6700702542321));
#184485=CARTESIAN_POINT('Ctrl Pts',(15.5523898151382,-69.898026140128,-55.6951134072476));
#184486=CARTESIAN_POINT('Ctrl Pts',(15.5508961531647,-69.8988503500373,
-55.7200275991231));
#184487=CARTESIAN_POINT('Ctrl Pts',(15.5502965922522,-69.899181190652,-55.7300282390814));
#184488=CARTESIAN_POINT('Ctrl Pts',(15.55,-69.8993466109593,-55.7400084027481));
#184489=CARTESIAN_POINT('Ctrl Pts',(15.55,-69.8993466109593,-55.74995));
#184490=CARTESIAN_POINT('',(15.55,67.7009572055632,-55.74995));
#184491=CARTESIAN_POINT('Origin',(15.55,67.7009572055632,-55.24995));
#184492=CARTESIAN_POINT('',(15.55,-69.8993466109592,-60.4282553373601));
#184493=CARTESIAN_POINT('',(15.55,-69.8993466109593,-55.24995));
#184494=CARTESIAN_POINT('Origin',(15.5500003881169,-68.4591876509329,-60.4515855208539));
#184495=CARTESIAN_POINT('',(15.55,-70.015703322148,-176.84995));
#184496=CARTESIAN_POINT('Ctrl Pts',(15.5499999897346,-69.8979710840162,
-60.3623910423524));
#184497=CARTESIAN_POINT('Ctrl Pts',(15.5501315664229,-69.2493490991427,
-60.3919718313354));
#184498=CARTESIAN_POINT('Ctrl Pts',(14.9223321947707,-69.4149357692034,
-60.3843514923986));
#184499=CARTESIAN_POINT('Ctrl Pts',(15.5499999897191,-69.909794297014,-60.6262209796107));
#184500=CARTESIAN_POINT('Ctrl Pts',(15.5501319338923,-69.254225424885,-60.5374367820963));
#184501=CARTESIAN_POINT('Ctrl Pts',(14.9213859066283,-69.4230681799894,
-60.5602124639497));
#184502=CARTESIAN_POINT('Ctrl Pts',(15.5499999897966,-69.8505276805174,
-60.8861498986541));
#184503=CARTESIAN_POINT('Ctrl Pts',(15.5501300981793,-69.2303831032415,
-60.678769908775));
#184504=CARTESIAN_POINT('Ctrl Pts',(14.9261257169452,-69.3823033916894,
-60.7335097961699));
#184505=CARTESIAN_POINT('Ctrl Pts',(15.5499999899638,-69.7237798948102,
-61.1215831761309));
#184506=CARTESIAN_POINT('Ctrl Pts',(15.5501262723864,-69.1690548338264,
-60.822436019398));
#184507=CARTESIAN_POINT('Ctrl Pts',(14.9363515075123,-69.2951068303029,
-60.89043888838));
#184508=CARTESIAN_POINT('',(15.05,-69.3993466109593,-60.4282553373601));
#184509=CARTESIAN_POINT('Origin',(15.05,-69.8993466109592,-60.4282553373601));
#184510=CARTESIAN_POINT('',(14.9222139673106,-69.4159516070034,-60.4282553373601));
#184511=CARTESIAN_POINT('Origin',(15.05,-69.8993466109592,-60.4282553373601));
#184512=CARTESIAN_POINT('Origin',(15.0817285037655,-68.054728362522,-60.3659193157066));
#184513=CARTESIAN_POINT('Origin',(0.,-12.9675000200281,-60.64995));
#184514=CARTESIAN_POINT('Origin',(0.,-12.9675000200281,-60.8508735991007));
#184515=CARTESIAN_POINT('Origin',(8.9,67.7009572055632,-55.24995));
#184516=CARTESIAN_POINT('',(8.9,-71.2138732976838,-171.871644662643));
#184517=CARTESIAN_POINT('',(8.9,-71.0999148696911,-60.4282553373601));
#184518=CARTESIAN_POINT('Origin',(8.89999938777026,-69.7158521501157,-60.4580628686921));
#184519=CARTESIAN_POINT('',(8.89999999157093,-71.0999148696892,-55.8925850873042));
#184520=CARTESIAN_POINT('',(8.9,-71.0999148696911,-55.24995));
#184521=CARTESIAN_POINT('Ctrl Pts',(8.89999996628377,-71.0999148696861,
-55.8925850873112));
#184522=CARTESIAN_POINT('Ctrl Pts',(8.89999995709263,-71.1271912455156,
-55.9047800168435));
#184523=CARTESIAN_POINT('Ctrl Pts',(8.89999995405378,-71.1542893399126,
-55.9174976277303));
#184524=CARTESIAN_POINT('Ctrl Pts',(8.89999995711454,-71.1811814737311,
-55.9307199810309));
#184525=CARTESIAN_POINT('Ctrl Pts',(8.89999996594249,-71.2587447432654,
-55.9688563728791));
#184526=CARTESIAN_POINT('Ctrl Pts',(8.89999997989509,-71.334738576959,-56.0111644614647));
#184527=CARTESIAN_POINT('Ctrl Pts',(8.89999998822403,-71.4082909897899,
-56.0572656901885));
#184528=CARTESIAN_POINT('Ctrl Pts',(8.89999999429182,-71.4618752880493,
-56.0908512911903));
#184529=CARTESIAN_POINT('Ctrl Pts',(8.89999999762151,-71.5141639062427,
-56.1264488763495));
#184530=CARTESIAN_POINT('Ctrl Pts',(8.89999999894661,-71.5648287885728,
-56.1638971934456));
#184531=CARTESIAN_POINT('Ctrl Pts',(8.90000000021705,-71.6134037334432,
-56.1998007592839));
#184532=CARTESIAN_POINT('Ctrl Pts',(8.9,-71.6605183672425,-56.2373236964706));
#184533=CARTESIAN_POINT('Ctrl Pts',(8.9,-71.7061534805117,-56.276424902386));
#184534=CARTESIAN_POINT('Ctrl Pts',(8.9,-71.7586958576709,-56.3214444095464));
#184535=CARTESIAN_POINT('Ctrl Pts',(8.90000000000525,-71.8093442969672,
-56.3686312342461));
#184536=CARTESIAN_POINT('Ctrl Pts',(8.89999999994877,-71.8580831316161,
-56.4179650024181));
#184537=CARTESIAN_POINT('Ctrl Pts',(8.89999999986101,-71.9338178277761,
-56.4946241587122));
#184538=CARTESIAN_POINT('Ctrl Pts',(8.89999999955086,-72.0053843762005,
-56.5771518376463));
#184539=CARTESIAN_POINT('Ctrl Pts',(8.89999999953632,-72.0709679837606,
-56.6635131964722));
#184540=CARTESIAN_POINT('Ctrl Pts',(8.89999999953336,-72.0842871673865,
-56.6810520730174));
#184541=CARTESIAN_POINT('Ctrl Pts',(8.89999999954423,-72.0973597365653,
-56.6987489820034));
#184542=CARTESIAN_POINT('Ctrl Pts',(8.89999999957055,-72.1101707466964,
-56.7165867802331));
#184543=CARTESIAN_POINT('Ctrl Pts',(8.89999999961887,-72.1337005884473,
-56.7493492685329));
#184544=CARTESIAN_POINT('Ctrl Pts',(8.89999999972697,-72.1563957720432,
-56.7826109127347));
#184545=CARTESIAN_POINT('Ctrl Pts',(8.89999999983668,-72.1782434639423,
-56.8163461536645));
#184546=CARTESIAN_POINT('Ctrl Pts',(8.90000000003969,-72.2186712712155,
-56.8787711377284));
#184547=CARTESIAN_POINT('Ctrl Pts',(8.89999999999795,-72.2562052259125,
-56.9428012878312));
#184548=CARTESIAN_POINT('Ctrl Pts',(8.89999999999952,-72.2908444043654,
-57.0084360093222));
#184549=CARTESIAN_POINT('Ctrl Pts',(8.90000000000048,-72.3119017301615,
-57.0483356771464));
#184550=CARTESIAN_POINT('Ctrl Pts',(8.9,-72.3318884210686,-57.0888288165431));
#184551=CARTESIAN_POINT('Ctrl Pts',(8.9,-72.3507957900478,-57.1299193914404));
#184552=CARTESIAN_POINT('Ctrl Pts',(8.9,-72.3746230901592,-57.1817022418682));
#184553=CARTESIAN_POINT('Ctrl Pts',(8.89999999998365,-72.3967864402965,
-57.2345342704725));
#184554=CARTESIAN_POINT('Ctrl Pts',(8.89999999972024,-72.4171503424455,
-57.288197632296));
#184555=CARTESIAN_POINT('Ctrl Pts',(8.89999999952357,-72.4323543754486,
-57.3282636038496));
#184556=CARTESIAN_POINT('Ctrl Pts',(8.89999999921991,-72.4465562092313,
-57.3687924002643));
#184557=CARTESIAN_POINT('Ctrl Pts',(8.89999999918092,-72.4597162071225,
-57.4096844656319));
#184558=CARTESIAN_POINT('Ctrl Pts',(8.89999999916252,-72.4659246935418,
-57.428976097332));
#184559=CARTESIAN_POINT('Ctrl Pts',(8.89999999920801,-72.4718879323416,
-57.4482939264422));
#184560=CARTESIAN_POINT('Ctrl Pts',(8.89999999932168,-72.4776042453442,
-57.4676297862024));
#184561=CARTESIAN_POINT('Ctrl Pts',(8.90000000038932,-72.5312977767249,
-57.649252204767));
#184562=CARTESIAN_POINT('Ctrl Pts',(8.89999999999947,-72.5639591690373,
-57.8344657871011));
#184563=CARTESIAN_POINT('Ctrl Pts',(8.89999999999994,-72.5753897578169,
-58.0232925566211));
#184564=CARTESIAN_POINT('Ctrl Pts',(8.90000000000006,-72.5784617700065,
-58.0740404357435));
#184565=CARTESIAN_POINT('Ctrl Pts',(8.9,-72.58000002,-58.1250492743389));
#184566=CARTESIAN_POINT('Ctrl Pts',(8.9,-72.58000002,-58.1763194612681));
#184567=CARTESIAN_POINT('Ctrl Pts',(8.90000001675659,-70.928272917477,-61.1211126854555));
#184568=CARTESIAN_POINT('Ctrl Pts',(8.89988778396233,-70.5448235085214,
-60.918842206156));
#184569=CARTESIAN_POINT('Ctrl Pts',(9.32900358361251,-70.4903946571405,
-60.8901185898342));
#184570=CARTESIAN_POINT('Ctrl Pts',(8.90000001650961,-71.0511602413471,
-60.887714756578));
#184571=CARTESIAN_POINT('Ctrl Pts',(8.89989004681885,-70.6365947859941,
-60.7567344379851));
#184572=CARTESIAN_POINT('Ctrl Pts',(9.32267960676822,-70.5733355012344,
-60.7345408641471));
#184573=CARTESIAN_POINT('Ctrl Pts',(8.9000000163917,-71.110350340576,-60.6286014156989));
#184574=CARTESIAN_POINT('Ctrl Pts',(8.89989111303313,-70.682184857852,-60.5709595618158));
#184575=CARTESIAN_POINT('Ctrl Pts',(9.31966069353146,-70.6132825269153,
-60.5618033393074));
#184576=CARTESIAN_POINT('Ctrl Pts',(8.90000001641518,-71.0985729052349,
-60.3617033877878));
#184577=CARTESIAN_POINT('Ctrl Pts',(8.89989090319397,-70.6731622220975,
-60.3808238190959));
#184578=CARTESIAN_POINT('Ctrl Pts',(9.32026185019719,-70.6053339699646,
-60.3838922942772));
#184579=CARTESIAN_POINT('',(9.32018679685842,-70.6063261212332,-60.4282553373601));
#184580=CARTESIAN_POINT('Origin',(9.42949994728011,-69.1714755465159,-60.3396721918004));
#184581=CARTESIAN_POINT('Origin',(9.4,-71.0999148696911,-60.4282553373601));
#184582=CARTESIAN_POINT('Ctrl Pts',(8.9,-72.58000002,-58.1763194612681));
#184583=CARTESIAN_POINT('Ctrl Pts',(8.89999999999996,-73.0800000199999,
-58.1763194612681));
#184584=CARTESIAN_POINT('Ctrl Pts',(8.4,-73.08000002,-58.1763194612681));
#184585=CARTESIAN_POINT('Ctrl Pts',(8.9,-72.5800000128814,-57.9140108579591));
#184586=CARTESIAN_POINT('Ctrl Pts',(8.89999999999996,-73.0782816065607,
-57.8621442504892));
#184587=CARTESIAN_POINT('Ctrl Pts',(8.40172135040051,-73.08000002,-57.8616056776356));
#184588=CARTESIAN_POINT('Ctrl Pts',(8.9,-72.5397349720259,-57.6584337450815));
#184589=CARTESIAN_POINT('Ctrl Pts',(8.89999999999997,-73.0284577192567,
-57.5559934180811));
#184590=CARTESIAN_POINT('Ctrl Pts',(8.40340362484077,-73.0316819589995,
-57.5549684855522));
#184591=CARTESIAN_POINT('Ctrl Pts',(8.9,-72.3796429547841,-57.1609527205255));
#184592=CARTESIAN_POINT('Ctrl Pts',(8.89999999999997,-72.8336034512039,
-56.9611013895289));
#184593=CARTESIAN_POINT('Ctrl Pts',(8.40668695336401,-72.8395715451724,
-56.9580994114807));
#184594=CARTESIAN_POINT('Ctrl Pts',(8.9,-72.262073445265,-56.9281157265161));
#184595=CARTESIAN_POINT('Ctrl Pts',(8.89999999999995,-72.6915892789857,
-56.6830185073362));
#184596=CARTESIAN_POINT('Ctrl Pts',(8.40822820346396,-72.6984881279278,
-56.6787458682451));
#184597=CARTESIAN_POINT('Ctrl Pts',(8.9,-72.0341941498609,-56.6108404408522));
#184598=CARTESIAN_POINT('Ctrl Pts',(8.89999999999996,-72.4171612181699,
-56.3044762227344));
#184599=CARTESIAN_POINT('Ctrl Pts',(8.41033280652841,-72.4250329770282,
-56.2980850295082));
#184600=CARTESIAN_POINT('Ctrl Pts',(8.9,-71.9491494655935,-56.5101636182542));
#184601=CARTESIAN_POINT('Ctrl Pts',(8.9000000000003,-72.3149747479787,-56.1845060329552));
#184602=CARTESIAN_POINT('Ctrl Pts',(8.41100144942456,-72.322979355276,-56.1772949390326));
#184603=CARTESIAN_POINT('Ctrl Pts',(8.9,-71.7670066137261,-56.3257764465383));
#184604=CARTESIAN_POINT('Ctrl Pts',(8.89999999999963,-72.0963975739119,
-55.9649406347444));
#184605=CARTESIAN_POINT('Ctrl Pts',(8.41222718544652,-72.1044079319076,
-55.9560708595913));
#184606=CARTESIAN_POINT('Ctrl Pts',(8.9,-71.6692649365715,-56.2410779083558));
#184607=CARTESIAN_POINT('Ctrl Pts',(8.89999999999951,-71.9792314944188,
-55.8641264120645));
#184608=CARTESIAN_POINT('Ctrl Pts',(8.41279083164671,-71.9871179192065,
-55.8544512596825));
#184609=CARTESIAN_POINT('Ctrl Pts',(8.9,-71.3558986429072,-56.0096140831459));
#184610=CARTESIAN_POINT('Ctrl Pts',(8.90000000000086,-71.6041352856071,
-55.588933048404));
#184611=CARTESIAN_POINT('Ctrl Pts',(8.41433230457371,-71.6110783688472,
-55.5767456783554));
#184612=CARTESIAN_POINT('Ctrl Pts',(8.9,-71.1195373961099,-55.8869904035305));
#184613=CARTESIAN_POINT('Ctrl Pts',(8.89999999999818,-71.3214288330036,
-55.443108937543));
#184614=CARTESIAN_POINT('Ctrl Pts',(8.41515058995443,-71.3274449382984,
-55.429624391176));
#184615=CARTESIAN_POINT('Ctrl Pts',(8.9,-70.8760630000525,-55.8051600336001));
#184616=CARTESIAN_POINT('Ctrl Pts',(8.89999999999995,-71.0304294360218,
-55.3458650785795));
#184617=CARTESIAN_POINT('Ctrl Pts',(8.41569693570581,-71.0352755960629,
-55.3314460318215));
#184618=CARTESIAN_POINT('',(8.41560828703704,-71.0814003738044,-55.3473768767704));
#184619=CARTESIAN_POINT('Ctrl Pts',(8.9,-71.0999148696911,-55.8925850873));
#184620=CARTESIAN_POINT('Ctrl Pts',(8.9,-71.0917569396884,-55.8670436478413));
#184621=CARTESIAN_POINT('Ctrl Pts',(8.89879514641371,-71.0842969126188,
-55.8417769940206));
#184622=CARTESIAN_POINT('Ctrl Pts',(8.89633575766726,-71.0775620353416,
-55.8169812460787));
#184623=CARTESIAN_POINT('Ctrl Pts',(8.89546270726179,-71.0751712431799,
-55.8081790842302));
#184624=CARTESIAN_POINT('Ctrl Pts',(8.8944319555344,-71.0728715932264,-55.7994361429263));
#184625=CARTESIAN_POINT('Ctrl Pts',(8.89324259912972,-71.0706635285073,
-55.7907607345806));
#184626=CARTESIAN_POINT('Ctrl Pts',(8.89097270851189,-71.0664494297141,
-55.7742036891632));
#184627=CARTESIAN_POINT('Ctrl Pts',(8.88812453435926,-71.062569970447,-55.7578953071278));
#184628=CARTESIAN_POINT('Ctrl Pts',(8.88470313888677,-71.0590262147759,
-55.7419018510144));
#184629=CARTESIAN_POINT('Ctrl Pts',(8.88325156030962,-71.057522723041,-55.7351163862952));
#184630=CARTESIAN_POINT('Ctrl Pts',(8.88176022108365,-71.0561390037238,
-55.7286645371772));
#184631=CARTESIAN_POINT('Ctrl Pts',(8.88015840509708,-71.0547945234521,
-55.722195200418));
#184632=CARTESIAN_POINT('Ctrl Pts',(8.87860148389261,-71.0534877255043,
-55.7159071825286));
#184633=CARTESIAN_POINT('Ctrl Pts',(8.87694017157194,-71.0522180593377,
-55.7096025647674));
#184634=CARTESIAN_POINT('Ctrl Pts',(8.87507019836549,-71.0509326662682,
-55.7029762075288));
#184635=CARTESIAN_POINT('Ctrl Pts',(8.87432941318369,-71.0504234610371,
-55.7003511927774));
#184636=CARTESIAN_POINT('Ctrl Pts',(8.87355543624803,-71.0499120229146,
-55.6976758891632));
#184637=CARTESIAN_POINT('Ctrl Pts',(8.87273988365555,-71.0493960567217,
-55.6949322108189));
#184638=CARTESIAN_POINT('Ctrl Pts',(8.87072835501306,-71.0481234462425,
-55.6881650352544));
#184639=CARTESIAN_POINT('Ctrl Pts',(8.86859773578304,-71.0469083241857,
-55.6814343500413));
#184640=CARTESIAN_POINT('Ctrl Pts',(8.86634547526123,-71.045751189175,-55.674743166039));
#184641=CARTESIAN_POINT('Ctrl Pts',(8.85507553034525,-71.0399610739979,
-55.6412615708154));
#184642=CARTESIAN_POINT('Ctrl Pts',(8.84089085739564,-71.0356842930815,
-55.6091873630217));
#184643=CARTESIAN_POINT('Ctrl Pts',(8.82376193805604,-71.0328761747199,
-55.5790161842937));
#184644=CARTESIAN_POINT('Ctrl Pts',(8.81033080789415,-71.030674272634,-55.5553583562312));
#184645=CARTESIAN_POINT('Ctrl Pts',(8.79509006677787,-71.0293748193011,
-55.5328713397496));
#184646=CARTESIAN_POINT('Ctrl Pts',(8.77803915034933,-71.0289449158603,
-55.5118076651523));
#184647=CARTESIAN_POINT('Ctrl Pts',(8.77375593123921,-71.0288369233873,
-55.5065164343881));
#184648=CARTESIAN_POINT('Ctrl Pts',(8.76935125432371,-71.0287837954292,
-55.5013061479734));
#184649=CARTESIAN_POINT('Ctrl Pts',(8.76482428326351,-71.0287853916737,
-55.4961820802034));
#184650=CARTESIAN_POINT('Ctrl Pts',(8.74779107634948,-71.0287913977125,
-55.4769022338321));
#184651=CARTESIAN_POINT('Ctrl Pts',(8.72908197860236,-71.0295822993029,
-55.458973225983));
#184652=CARTESIAN_POINT('Ctrl Pts',(8.70888162163445,-71.0311233825918,
-55.4427172100486));
#184653=CARTESIAN_POINT('Ctrl Pts',(8.70741300418116,-71.031235423276,-55.4415353562447));
#184654=CARTESIAN_POINT('Ctrl Pts',(8.70593652454071,-71.0313514220976,
-55.4403623533746));
#184655=CARTESIAN_POINT('Ctrl Pts',(8.7044522630751,-71.0314713623944,-55.4391983289897));
#184656=CARTESIAN_POINT('Ctrl Pts',(8.69616488178655,-71.0321410496392,
-55.432698993037));
#184657=CARTESIAN_POINT('Ctrl Pts',(8.68749347126554,-71.0329463519757,
-55.4263738514522));
#184658=CARTESIAN_POINT('Ctrl Pts',(8.67858198159518,-71.0338775435445,
-55.4203637320546));
#184659=CARTESIAN_POINT('Ctrl Pts',(8.66968930617718,-71.0348067691487,
-55.4143663014338));
#184660=CARTESIAN_POINT('Ctrl Pts',(8.66055796015982,-71.0358612349136,
-55.4086829050489));
#184661=CARTESIAN_POINT('Ctrl Pts',(8.65135665870045,-71.0370157116539,
-55.4034110626757));
#184662=CARTESIAN_POINT('Ctrl Pts',(8.64203670453801,-71.0381850756127,
-55.3980712387946));
#184663=CARTESIAN_POINT('Ctrl Pts',(8.63264545478659,-71.0394568806338,
-55.3931538649237));
#184664=CARTESIAN_POINT('Ctrl Pts',(8.62337802331042,-71.0407910350239,
-55.3887122670778));
#184665=CARTESIAN_POINT('Ctrl Pts',(8.62073171866857,-71.0411720013104,
-55.3874439738051));
#184666=CARTESIAN_POINT('Ctrl Pts',(8.61809560649366,-71.0415579751156,
-55.3862141696892));
#184667=CARTESIAN_POINT('Ctrl Pts',(8.615474432557,-71.0419478523178,-55.3850233723615));
#184668=CARTESIAN_POINT('Ctrl Pts',(8.61241983732061,-71.0424021972309,
-55.3836356720665));
#184669=CARTESIAN_POINT('Ctrl Pts',(8.60934133814994,-71.0428683753267,
-55.3822808217115));
#184670=CARTESIAN_POINT('Ctrl Pts',(8.60623983960316,-71.0433462841332,
-55.3809601346928));
#184671=CARTESIAN_POINT('Ctrl Pts',(8.58930959822934,-71.0459550589972,
-55.3737508616046));
#184672=CARTESIAN_POINT('Ctrl Pts',(8.57166297875426,-71.0489168177501,
-55.367543437794));
#184673=CARTESIAN_POINT('Ctrl Pts',(8.55347665375656,-71.0522143880086,
-55.3624867791543));
#184674=CARTESIAN_POINT('Ctrl Pts',(8.53515596710212,-71.0555363209133,
-55.3573927616181));
#184675=CARTESIAN_POINT('Ctrl Pts',(8.51628826305535,-71.0591989361935,
-55.3534669775368));
#184676=CARTESIAN_POINT('Ctrl Pts',(8.49708344608809,-71.0631697725525,
-55.3508199238887));
#184677=CARTESIAN_POINT('Ctrl Pts',(8.47782643478517,-71.0671514007439,
-55.3481656761492));
#184678=CARTESIAN_POINT('Ctrl Pts',(8.45823131035549,-71.0714427669999,
-55.3467974390802));
#184679=CARTESIAN_POINT('Ctrl Pts',(8.43852743622952,-71.0759982761646,
-55.3467793842152));
#184680=CARTESIAN_POINT('Ctrl Pts',(8.43089942989955,-71.0777618609562,
-55.3467723945935));
#184681=CARTESIAN_POINT('Ctrl Pts',(8.42325524547048,-71.0795649100216,
-55.3469672331109));
#184682=CARTESIAN_POINT('Ctrl Pts',(8.41560847893818,-71.0814043465126,
-55.3473655849103));
#184683=CARTESIAN_POINT('Ctrl Pts',(8.4,-73.08000002,-58.1763194612681));
#184684=CARTESIAN_POINT('Ctrl Pts',(8.40035672389639,-73.08000002,-58.1110997784471));
#184685=CARTESIAN_POINT('Ctrl Pts',(8.40073754463678,-73.0779206981902,
-58.0450936526532));
#184686=CARTESIAN_POINT('Ctrl Pts',(8.40113458127941,-73.0735758450926,
-57.978552610913));
#184687=CARTESIAN_POINT('Ctrl Pts',(8.40152353070599,-73.0693194920526,
-57.9133669397449));
#184688=CARTESIAN_POINT('Ctrl Pts',(8.40192804222985,-73.0628889081674,
-57.8476679403423));
#184689=CARTESIAN_POINT('Ctrl Pts',(8.40234076967212,-73.0541584892345,
-57.7816841227729));
#184690=CARTESIAN_POINT('Ctrl Pts',(8.40275020169798,-73.045497778208,-57.7162271520608));
#184691=CARTESIAN_POINT('Ctrl Pts',(8.40316771887553,-73.0345737249397,
-57.6504899174073));
#184692=CARTESIAN_POINT('Ctrl Pts',(8.40358621253362,-73.0213140539565,
-57.5846872495408));
#184693=CARTESIAN_POINT('Ctrl Pts',(8.4040017342091,-73.0081485481076,-57.519351887165));
#184694=CARTESIAN_POINT('Ctrl Pts',(8.40441821842852,-72.9926804455084,
-57.4539520333922));
#184695=CARTESIAN_POINT('Ctrl Pts',(8.40482877076465,-72.974889733916,-57.3886895117376));
#184696=CARTESIAN_POINT('Ctrl Pts',(8.4050299722353,-72.966170949436,-57.3567059759489));
#184697=CARTESIAN_POINT('Ctrl Pts',(8.40522975001004,-72.9568951136423,
-57.3247552929955));
#184698=CARTESIAN_POINT('Ctrl Pts',(8.40542729839457,-72.94706438667,-57.2928604536989));
#184699=CARTESIAN_POINT('Ctrl Pts',(8.40550227634482,-72.9433332108387,
-57.2807550159361));
#184700=CARTESIAN_POINT('Ctrl Pts',(8.40557697894183,-72.9395187712762,
-57.2686466985916));
#184701=CARTESIAN_POINT('Ctrl Pts',(8.40565135799998,-72.9356205804985,
-57.2565359345658));
#184702=CARTESIAN_POINT('Ctrl Pts',(8.40619760549404,-72.9069918643403,
-57.1675932312636));
#184703=CARTESIAN_POINT('Ctrl Pts',(8.40672108609692,-72.8740822822173,
-57.0794847544457));
#184704=CARTESIAN_POINT('Ctrl Pts',(8.40720150496587,-72.8368274130977,
-56.9926068087741));
#184705=CARTESIAN_POINT('Ctrl Pts',(8.40745556118681,-72.8171262067712,
-56.94666381197));
#184706=CARTESIAN_POINT('Ctrl Pts',(8.40769757664703,-72.7962107080569,
-56.9010649498654));
#184707=CARTESIAN_POINT('Ctrl Pts',(8.40792456334921,-72.7740772741753,
-56.8558686291175));
#184708=CARTESIAN_POINT('Ctrl Pts',(8.40824535919252,-72.7427965272451,
-56.7919935576286));
#184709=CARTESIAN_POINT('Ctrl Pts',(8.40853569883156,-72.7091163079819,
-56.7289987036777));
#184710=CARTESIAN_POINT('Ctrl Pts',(8.40878697458908,-72.6731278697012,
-56.6671446660938));
#184711=CARTESIAN_POINT('Ctrl Pts',(8.40881559250486,-72.6690291293133,
-56.6601000802737));
#184712=CARTESIAN_POINT('Ctrl Pts',(8.40884370389039,-72.6649004993438,
-56.6530702685158));
#184713=CARTESIAN_POINT('Ctrl Pts',(8.40887129616344,-72.6607421532749,
-56.6460555971729));
#184714=CARTESIAN_POINT('Ctrl Pts',(8.40900622741974,-72.6404070812704,
-56.6117525727297));
#184715=CARTESIAN_POINT('Ctrl Pts',(8.40912875293662,-72.6193610983144,
-56.5778119325455));
#184716=CARTESIAN_POINT('Ctrl Pts',(8.40923748796417,-72.5976273704848,
-56.5442753574122));
#184717=CARTESIAN_POINT('Ctrl Pts',(8.40929185547795,-72.58676050657,-56.5275070698456));
#184718=CARTESIAN_POINT('Ctrl Pts',(8.40934277697055,-72.5757217691974,
-56.5108397496895));
#184719=CARTESIAN_POINT('Ctrl Pts',(8.40939008649233,-72.5645144644975,
-56.4942783667926));
#184720=CARTESIAN_POINT('Ctrl Pts',(8.40941709131399,-72.5581172054839,
-56.4848249380822));
#184721=CARTESIAN_POINT('Ctrl Pts',(8.40944431705732,-72.5512762083545,
-56.4748395208255));
#184722=CARTESIAN_POINT('Ctrl Pts',(8.40947678617871,-72.544654112667,-56.4652954501693));
#184723=CARTESIAN_POINT('Ctrl Pts',(8.40950119944023,-72.5396750141612,
-56.4581193430598));
#184724=CARTESIAN_POINT('Ctrl Pts',(8.40952858023405,-72.5348207940818,
-56.4511920813509));
#184725=CARTESIAN_POINT('Ctrl Pts',(8.40956111525206,-72.5303897605329,
-56.4449172192676));
#184726=CARTESIAN_POINT('Ctrl Pts',(8.40959563855584,-72.5256879368788,
-56.4382588867039));
#184727=CARTESIAN_POINT('Ctrl Pts',(8.40963023878015,-72.5209528390535,
-56.431610605939));
#184728=CARTESIAN_POINT('Ctrl Pts',(8.40966490858559,-72.5161841667267,
-56.424972354458));
#184729=CARTESIAN_POINT('Ctrl Pts',(8.40992896618708,-72.4798642577818,
-56.3744130639842));
#184730=CARTESIAN_POINT('Ctrl Pts',(8.41019734451649,-72.4415022725631,
-56.3243841045374));
#184731=CARTESIAN_POINT('Ctrl Pts',(8.41046552964781,-72.4011582747068,
-56.2751057922352));
#184732=CARTESIAN_POINT('Ctrl Pts',(8.41071616361799,-72.3634545574798,
-56.2290524596161));
#184733=CARTESIAN_POINT('Ctrl Pts',(8.41096663041762,-72.3240192051747,
-56.1836544928687));
#184734=CARTESIAN_POINT('Ctrl Pts',(8.41121299955242,-72.2829028029665,
-56.1391378648765));
#184735=CARTESIAN_POINT('Ctrl Pts',(8.4112764114403,-72.2723200297268,-56.1276799222031));
#184736=CARTESIAN_POINT('Ctrl Pts',(8.41133955045791,-72.2616259229582,
-56.1162806284349));
#184737=CARTESIAN_POINT('Ctrl Pts',(8.41140234650254,-72.2508214301511,
-56.1049444090467));
#184738=CARTESIAN_POINT('Ctrl Pts',(8.41147347283705,-72.2385836534875,
-56.0921043689301));
#184739=CARTESIAN_POINT('Ctrl Pts',(8.41154415246921,-72.226205355973,-56.0793464580293));
#184740=CARTESIAN_POINT('Ctrl Pts',(8.41161431743554,-72.2136936435918,
-56.066682899312));
#184741=CARTESIAN_POINT('Ctrl Pts',(8.41185965065156,-72.1699461896023,
-56.022404511554));
#184742=CARTESIAN_POINT('Ctrl Pts',(8.41209972464812,-72.124441480344,-55.979092815899));
#184743=CARTESIAN_POINT('Ctrl Pts',(8.41233324066691,-72.0772624573489,
-55.9369797476933));
#184744=CARTESIAN_POINT('Ctrl Pts',(8.41253881658477,-72.0357283861281,
-55.8999054917393));
#184745=CARTESIAN_POINT('Ctrl Pts',(8.41273931262493,-71.9928971384868,
-55.8637596924157));
#184746=CARTESIAN_POINT('Ctrl Pts',(8.4129339808891,-71.9488479037631,-55.8286752066144));
#184747=CARTESIAN_POINT('Ctrl Pts',(8.4130399900923,-71.9248603046815,-55.80956948129));
#184748=CARTESIAN_POINT('Ctrl Pts',(8.4131442757425,-71.9005112029568,-55.7907776395893));
#184749=CARTESIAN_POINT('Ctrl Pts',(8.41324670514547,-71.8758233350021,
-55.7723232379903));
#184750=CARTESIAN_POINT('Ctrl Pts',(8.4132660877491,-71.8711516768159,-55.7688311318085));
#184751=CARTESIAN_POINT('Ctrl Pts',(8.41328540470802,-71.8664677096972,
-55.7653509601608));
#184752=CARTESIAN_POINT('Ctrl Pts',(8.41330465595571,-71.8617714024201,
-55.7618827325735));
#184753=CARTESIAN_POINT('Ctrl Pts',(8.41363128196581,-71.7820915742357,
-55.7030391003416));
#184754=CARTESIAN_POINT('Ctrl Pts',(8.41393799526188,-71.6987858561321,
-55.647812970034));
#184755=CARTESIAN_POINT('Ctrl Pts',(8.41422246514108,-71.6125045136972,
-55.5966136090959));
#184756=CARTESIAN_POINT('Ctrl Pts',(8.41449855328811,-71.5287653986031,
-55.5469228062253));
#184757=CARTESIAN_POINT('Ctrl Pts',(8.41475369066292,-71.4422227019064,
-55.5010247736432));
#184758=CARTESIAN_POINT('Ctrl Pts',(8.41498549912693,-71.3534940238151,
-55.4593377991568));
#184759=CARTESIAN_POINT('Ctrl Pts',(8.41520278482016,-71.2703241861167,
-55.4202625083179));
#184760=CARTESIAN_POINT('Ctrl Pts',(8.41539957263635,-71.1852333264852,
-55.384887255107));
#184761=CARTESIAN_POINT('Ctrl Pts',(8.41557368114123,-71.0987580297025,
-55.3535961962895));
#184762=CARTESIAN_POINT('Ctrl Pts',(8.41558531806895,-71.0929782616274,
-55.3515047890378));
#184763=CARTESIAN_POINT('Ctrl Pts',(8.41559685359719,-71.0871923211226,
-55.3494316420719));
#184764=CARTESIAN_POINT('Ctrl Pts',(8.41560828703704,-71.0814003738044,
-55.3473768767704));
#184765=CARTESIAN_POINT('Ctrl Pts',(7.81557216061077,-73.08000002,-58.1565578346149));
#184766=CARTESIAN_POINT('Ctrl Pts',(7.88787222497771,-73.08000002,-56.0696654600803));
#184767=CARTESIAN_POINT('Ctrl Pts',(7.91297989639773,-71.1218111846181,
-55.3449495350315));
#184768=CARTESIAN_POINT('Ctrl Pts',(8.01154341310716,-73.08000002,-58.1633472285769));
#184769=CARTESIAN_POINT('Ctrl Pts',(8.08415144386654,-73.0800000199999,
-56.0574351382549));
#184770=CARTESIAN_POINT('Ctrl Pts',(8.10803398103684,-71.0978479138796,
-55.3428278238728));
#184771=CARTESIAN_POINT('Ctrl Pts',(8.20751459243696,-73.08000002,-58.1699994619965));
#184772=CARTESIAN_POINT('Ctrl Pts',(8.27957773899348,-73.080000019995,-56.0443052546218));
#184773=CARTESIAN_POINT('Ctrl Pts',(8.30261637241262,-71.0730051020405,
-55.3405756034005));
#184774=CARTESIAN_POINT('Ctrl Pts',(8.40348565123649,-73.08000002,-58.1764339313253));
#184775=CARTESIAN_POINT('Ctrl Pts',(8.47395476320647,-73.08000002,-56.0301952716572));
#184776=CARTESIAN_POINT('Ctrl Pts',(8.49667612020153,-71.0472900720475,
-55.3381835033849));
#184777=CARTESIAN_POINT('',(7.91618841388596,-71.1413938388782,-55.3523953317199));
#184778=CARTESIAN_POINT('Origin',(0.0693744628069737,-4.69854457220239,
-43.5232227885957));
#184779=CARTESIAN_POINT('Ctrl Pts',(7.91618834474436,-71.1413930828737,
-55.3523973277251));
#184780=CARTESIAN_POINT('Ctrl Pts',(7.91605153909874,-71.2034746521269,
-55.3759080424155));
#184781=CARTESIAN_POINT('Ctrl Pts',(7.91590005671631,-71.2659341313245,
-55.4019927616619));
#184782=CARTESIAN_POINT('Ctrl Pts',(7.91573324782657,-71.328557341725,-55.4307509004807));
#184783=CARTESIAN_POINT('Ctrl Pts',(7.91558128376081,-71.385607524595,-55.4569497661747));
#184784=CARTESIAN_POINT('Ctrl Pts',(7.91541659756771,-71.4427935588638,
-55.4853677620711));
#184785=CARTESIAN_POINT('Ctrl Pts',(7.9152386469442,-71.4999079010297,-55.5160892262258));
#184786=CARTESIAN_POINT('Ctrl Pts',(7.91506676331057,-71.5550750056455,
-55.545763282911));
#184787=CARTESIAN_POINT('Ctrl Pts',(7.91488250297984,-71.6101755625449,
-55.5775866415003));
#184788=CARTESIAN_POINT('Ctrl Pts',(7.91468535064406,-71.6649751653101,
-55.6116402864228));
#184789=CARTESIAN_POINT('Ctrl Pts',(7.91449742712847,-71.717209565496,-55.6440998596117));
#184790=CARTESIAN_POINT('Ctrl Pts',(7.91429778919425,-71.7691707021736,
-55.6785859971176));
#184791=CARTESIAN_POINT('Ctrl Pts',(7.91408598336362,-71.8206083105627,
-55.7151704742676));
#184792=CARTESIAN_POINT('Ctrl Pts',(7.91399247664347,-71.843316665843,-55.7313215615922));
#184793=CARTESIAN_POINT('Ctrl Pts',(7.9138965984125,-71.8659223339732,-55.7478816187245));
#184794=CARTESIAN_POINT('Ctrl Pts',(7.91379831004409,-71.888400490254,-55.7648567817402));
#184795=CARTESIAN_POINT('Ctrl Pts',(7.91375750815433,-71.8977317190606,
-55.7719035843405));
#184796=CARTESIAN_POINT('Ctrl Pts',(7.91371629392849,-71.9070408946849,
-55.7790218888929));
#184797=CARTESIAN_POINT('Ctrl Pts',(7.91367467121773,-71.9163247705886,
-55.7862110477586));
#184798=CARTESIAN_POINT('Ctrl Pts',(7.91344559186313,-71.9674205368459,
-55.8257780976412));
#184799=CARTESIAN_POINT('Ctrl Pts',(7.91320420359684,-72.0178756635473,
-55.8674802576463));
#184800=CARTESIAN_POINT('Ctrl Pts',(7.91295060237791,-72.0674131211372,
-55.9113042692579));
#184801=CARTESIAN_POINT('Ctrl Pts',(7.91278763230622,-72.0992470494138,
-55.9394666035865));
#184802=CARTESIAN_POINT('Ctrl Pts',(7.91261962316456,-72.1307026933166,
-55.9685044232441));
#184803=CARTESIAN_POINT('Ctrl Pts',(7.91244665070092,-72.1617142526647,
-55.9984055386534));
#184804=CARTESIAN_POINT('Ctrl Pts',(7.91233172832566,-72.1823182377497,
-56.0182717481853));
#184805=CARTESIAN_POINT('Ctrl Pts',(7.91221461584245,-72.2027263192037,
-56.038518895424));
#184806=CARTESIAN_POINT('Ctrl Pts',(7.91209534542699,-72.2229207324772,
-56.0591416827554));
#184807=CARTESIAN_POINT('Ctrl Pts',(7.9120350990377,-72.2331214220513,-56.0695587544905));
#184808=CARTESIAN_POINT('Ctrl Pts',(7.91197429303426,-72.2432690765559,
-56.08007323039));
#184809=CARTESIAN_POINT('Ctrl Pts',(7.91191298560901,-72.2533528906614,
-56.0906750808164));
#184810=CARTESIAN_POINT('Ctrl Pts',(7.91170698464258,-72.2872358247832,
-56.1262986847231));
#184811=CARTESIAN_POINT('Ctrl Pts',(7.91149455903653,-72.3204838435951,
-56.1630410022271));
#184812=CARTESIAN_POINT('Ctrl Pts',(7.91127619570105,-72.3529964672989,
-56.2008190342108));
#184813=CARTESIAN_POINT('Ctrl Pts',(7.91113867876851,-72.3734716824736,
-56.2246102034745));
#184814=CARTESIAN_POINT('Ctrl Pts',(7.91099882009844,-72.3936530793658,
-56.2488098609766));
#184815=CARTESIAN_POINT('Ctrl Pts',(7.9108566916282,-72.4135189243128,-56.2734059029323));
#184816=CARTESIAN_POINT('Ctrl Pts',(7.9106970878667,-72.4358273581791,-56.30102613136));
#184817=CARTESIAN_POINT('Ctrl Pts',(7.91053459989681,-72.4577411046642,
-56.3291500043599));
#184818=CARTESIAN_POINT('Ctrl Pts',(7.9103693134689,-72.4792240409969,-56.3577632330128));
#184819=CARTESIAN_POINT('Ctrl Pts',(7.91028667025495,-72.4899655091633,
-56.3720698473392));
#184820=CARTESIAN_POINT('Ctrl Pts',(7.91020332703685,-72.5005992083201,
-56.3864988690585));
#184821=CARTESIAN_POINT('Ctrl Pts',(7.91011929378563,-72.5111199845664,
-56.4010486482998));
#184822=CARTESIAN_POINT('Ctrl Pts',(7.91010814227553,-72.51251612884,-56.402979455542));
#184823=CARTESIAN_POINT('Ctrl Pts',(7.91009699085137,-72.513908771587,-56.4049102703791));
#184824=CARTESIAN_POINT('Ctrl Pts',(7.9100857447223,-72.515309674263,-56.4068575059994));
#184825=CARTESIAN_POINT('Ctrl Pts',(7.91002258730152,-72.5231770390477,
-56.4177930357892));
#184826=CARTESIAN_POINT('Ctrl Pts',(7.90995716291352,-72.531209313664,-56.4291218453457));
#184827=CARTESIAN_POINT('Ctrl Pts',(7.9098939454102,-72.5388590978003,-56.4400692573546));
#184828=CARTESIAN_POINT('Ctrl Pts',(7.9098835928595,-72.5401118327867,-56.4418620146129));
#184829=CARTESIAN_POINT('Ctrl Pts',(7.9098732997821,-72.541354412209,-56.4436444925833));
#184830=CARTESIAN_POINT('Ctrl Pts',(7.90986308615092,-72.5425845514597,
-56.4454132317544));
#184831=CARTESIAN_POINT('Ctrl Pts',(7.90984507450521,-72.5447538908436,
-56.4485323872007));
#184832=CARTESIAN_POINT('Ctrl Pts',(7.90982730837562,-72.5468849317012,
-56.4516090843173));
#184833=CARTESIAN_POINT('Ctrl Pts',(7.90980989769223,-72.5489653972306,
-56.4546242799526));
#184834=CARTESIAN_POINT('Ctrl Pts',(7.90943253237259,-72.5940581441442,
-56.5199766983186));
#184835=CARTESIAN_POINT('Ctrl Pts',(7.90901970086401,-72.6363853652346,
-56.586848561989));
#184836=CARTESIAN_POINT('Ctrl Pts',(7.9085826566518,-72.675894254675,-56.6550786162537));
#184837=CARTESIAN_POINT('Ctrl Pts',(7.90820073287228,-72.7104202453145,
-56.7147034310293));
#184838=CARTESIAN_POINT('Ctrl Pts',(7.90780032030306,-72.7427947088886,
-56.7753650383112));
#184839=CARTESIAN_POINT('Ctrl Pts',(7.90738899215006,-72.7730108753014,
-56.8369399773851));
#184840=CARTESIAN_POINT('Ctrl Pts',(7.90692956490218,-72.8067604012585,
-56.9057152474241));
#184841=CARTESIAN_POINT('Ctrl Pts',(7.90645485946628,-72.8379002618168,
-56.9759187116765));
#184842=CARTESIAN_POINT('Ctrl Pts',(7.90597814647801,-72.8662221236656,
-57.0468995536857));
#184843=CARTESIAN_POINT('Ctrl Pts',(7.90552849392276,-72.8929363057061,
-57.1138511949638));
#184844=CARTESIAN_POINT('Ctrl Pts',(7.90507706021611,-72.9171434174572,
-57.1814935793758));
#184845=CARTESIAN_POINT('Ctrl Pts',(7.90463487950093,-72.9387159615222,
-57.2492917775834));
#184846=CARTESIAN_POINT('Ctrl Pts',(7.90460826872894,-72.9400142136436,
-57.2533719247549));
#184847=CARTESIAN_POINT('Ctrl Pts',(7.9045816914238,-72.9413029388677,-57.2574526420199));
#184848=CARTESIAN_POINT('Ctrl Pts',(7.90455514997215,-72.9425821151501,
-57.2615338151869));
#184849=CARTESIAN_POINT('Ctrl Pts',(7.90449310528884,-72.9455723844232,
-57.2710741786905));
#184850=CARTESIAN_POINT('Ctrl Pts',(7.90443128316216,-72.9485108109217,
-57.2806123946304));
#184851=CARTESIAN_POINT('Ctrl Pts',(7.90436970799662,-72.9513975879421,
-57.2901480548786));
#184852=CARTESIAN_POINT('Ctrl Pts',(7.90394961648964,-72.9710923869453,
-57.3552043133363));
#184853=CARTESIAN_POINT('Ctrl Pts',(7.90353978491141,-72.9884844749361,
-57.420491090881));
#184854=CARTESIAN_POINT('Ctrl Pts',(7.90314750826272,-73.003568062194,-57.4858113326828));
#184855=CARTESIAN_POINT('Ctrl Pts',(7.90275224687669,-73.0187664167882,
-57.5516285802714));
#184856=CARTESIAN_POINT('Ctrl Pts',(7.90237480900421,-73.0316210069439,
-57.6174797935744));
#184857=CARTESIAN_POINT('Ctrl Pts',(7.90202267091283,-73.0421783087771,
-57.6831546116925));
#184858=CARTESIAN_POINT('Ctrl Pts',(7.90166792717642,-73.0528137293421,
-57.7493153904834));
#184859=CARTESIAN_POINT('Ctrl Pts',(7.90133885955718,-73.061117798216,-57.8152971347828));
#184860=CARTESIAN_POINT('Ctrl Pts',(7.90104311783998,-73.0671905619965,
-57.8808761274596));
#184861=CARTESIAN_POINT('Ctrl Pts',(7.900742514705,-73.0733631501847,-57.9475331110384));
#184862=CARTESIAN_POINT('Ctrl Pts',(7.90047634278182,-73.0772305249596,
-58.0137739762241));
#184863=CARTESIAN_POINT('Ctrl Pts',(7.90025263259021,-73.078951103751,-58.0793551407081));
#184864=CARTESIAN_POINT('Ctrl Pts',(7.90016113595277,-73.0796548140859,
-58.1061775933928));
#184865=CARTESIAN_POINT('Ctrl Pts',(7.90007674213687,-73.08000002,-58.1328895949801));
#184866=CARTESIAN_POINT('Ctrl Pts',(7.9,-73.08000002,-58.1594740865074));
#184867=CARTESIAN_POINT('Ctrl Pts',(7.9,-73.08000002,-58.1594740865074));
#184868=CARTESIAN_POINT('Ctrl Pts',(7.39999999999995,-73.0800000199999,
-58.1594740865073));
#184869=CARTESIAN_POINT('Ctrl Pts',(7.4,-72.58000002,-58.1594740865074));
#184870=CARTESIAN_POINT('Ctrl Pts',(7.9017604405896,-73.08000002,-57.8524302618023));
#184871=CARTESIAN_POINT('Ctrl Pts',(7.39999999999985,-73.0817635435305,
-57.8518911502672));
#184872=CARTESIAN_POINT('Ctrl Pts',(7.4,-72.5800000130548,-57.9035537157173));
#184873=CARTESIAN_POINT('Ctrl Pts',(7.90348019558611,-73.0339592231946,
-57.5530891712348));
#184874=CARTESIAN_POINT('Ctrl Pts',(7.40000000000007,-73.0373043377172,
-57.5520537815894));
#184875=CARTESIAN_POINT('Ctrl Pts',(7.4,-72.5416326919704,-57.6540534055839));
#184876=CARTESIAN_POINT('Ctrl Pts',(7.90599716341333,-72.896885176701,-57.1157587646024));
#184877=CARTESIAN_POINT('Ctrl Pts',(7.3999999999999,-72.9025581822962,-57.1135670536862));
#184878=CARTESIAN_POINT('Ctrl Pts',(7.4,-72.42740431593,-57.2895390365225));
#184879=CARTESIAN_POINT('Ctrl Pts',(7.90681948691283,-72.8397791179241,
-56.9730119912525));
#184880=CARTESIAN_POINT('Ctrl Pts',(7.39999999999985,-72.846103402619,-56.9702086770063));
#184881=CARTESIAN_POINT('Ctrl Pts',(7.4,-72.3798159344887,-57.1705597381646));
#184882=CARTESIAN_POINT('Ctrl Pts',(7.9083884819823,-72.7062368443098,-56.70087080336));
#184883=CARTESIAN_POINT('Ctrl Pts',(7.40000000000008,-72.7136696095191,
-56.6966550709085));
#184884=CARTESIAN_POINT('Ctrl Pts',(7.4,-72.2685307073729,-56.9437302645456));
#184885=CARTESIAN_POINT('Ctrl Pts',(7.90914169806791,-72.6294692039913,
-56.5703391604345));
#184886=CARTESIAN_POINT('Ctrl Pts',(7.39999999999996,-72.6373398680779,
-56.5653507289509));
#184887=CARTESIAN_POINT('Ctrl Pts',(7.4,-72.2045576741781,-56.8349322106875));
#184888=CARTESIAN_POINT('Ctrl Pts',(7.91058447423394,-72.4556998989282,
-56.3204873030743));
#184889=CARTESIAN_POINT('Ctrl Pts',(7.39999999999996,-72.4642201336178,
-56.3138046122562));
#184890=CARTESIAN_POINT('Ctrl Pts',(7.4,-72.0597499182548,-56.6266807792285));
#184891=CARTESIAN_POINT('Ctrl Pts',(7.91127644455456,-72.3580508393546,
-56.2007516828216));
#184892=CARTESIAN_POINT('Ctrl Pts',(7.39999999999996,-72.366765643856,-56.1931795440353));
#184893=CARTESIAN_POINT('Ctrl Pts',(7.4,-71.9783757021874,-56.5268811589555));
#184894=CARTESIAN_POINT('Ctrl Pts',(7.91254952666346,-72.1486549419682,
-55.9805984788111));
#184895=CARTESIAN_POINT('Ctrl Pts',(7.39999999999996,-72.1574857101496,
-55.9712111947932));
#184896=CARTESIAN_POINT('Ctrl Pts',(7.4,-71.8038791222482,-56.3433834633767));
#184897=CARTESIAN_POINT('Ctrl Pts',(7.91313676360239,-72.0363041630141,
-55.879119540041));
#184898=CARTESIAN_POINT('Ctrl Pts',(7.39999999999952,-72.0450577059424,
-55.8688410357779));
#184899=CARTESIAN_POINT('Ctrl Pts',(7.4,-71.710253472938,-56.2588007503857));
#184900=CARTESIAN_POINT('Ctrl Pts',(7.9147504864484,-71.6763659857377,-55.6003940631938));
#184901=CARTESIAN_POINT('Ctrl Pts',(7.40000000000084,-71.6842770741658,
-55.5873067274671));
#184902=CARTESIAN_POINT('Ctrl Pts',(7.4,-71.4103049905956,-56.0264829839341));
#184903=CARTESIAN_POINT('Ctrl Pts',(7.91562717321909,-71.4030569333749,
-55.449171357324));
#184904=CARTESIAN_POINT('Ctrl Pts',(7.40000000000019,-71.4100611802463,
-55.4345719679896));
#184905=CARTESIAN_POINT('Ctrl Pts',(7.4,-71.1825473819866,-55.9004387386915));
#184906=CARTESIAN_POINT('Ctrl Pts',(7.91623251645313,-71.1210872664424,
-55.3447940747887));
#184907=CARTESIAN_POINT('Ctrl Pts',(7.39999999999996,-71.1269094387434,
-55.3290689454198));
#184908=CARTESIAN_POINT('Ctrl Pts',(7.4,-70.9475727253686,-55.8134402200258));
#184909=CARTESIAN_POINT('',(7.40000000638209,-71.4493575166324,-56.0666111687524));
#184910=CARTESIAN_POINT('Ctrl Pts',(7.91618843693206,-71.1413940909408,
-55.352394666395));
#184911=CARTESIAN_POINT('Ctrl Pts',(7.89640718675846,-71.1458420666493,
-55.3533930281891));
#184912=CARTESIAN_POINT('Ctrl Pts',(7.87623144639825,-71.1506401421049,
-55.3558165327541));
#184913=CARTESIAN_POINT('Ctrl Pts',(7.8558979626605,-71.1557708852316,-55.3597440199642));
#184914=CARTESIAN_POINT('Ctrl Pts',(7.83950012223097,-71.1599085484163,
-55.3629113231863));
#184915=CARTESIAN_POINT('Ctrl Pts',(7.82300052698497,-71.1642623278572,
-55.3670559830725));
#184916=CARTESIAN_POINT('Ctrl Pts',(7.8065381012743,-71.1688178845881,-55.3722003240005));
#184917=CARTESIAN_POINT('Ctrl Pts',(7.78854780695949,-71.1737962400139,
-55.3778221083583));
#184918=CARTESIAN_POINT('Ctrl Pts',(7.7705985227141,-71.1790163264486,-55.384638034101));
#184919=CARTESIAN_POINT('Ctrl Pts',(7.7528637382243,-71.1844612784818,-55.3926687943192));
#184920=CARTESIAN_POINT('Ctrl Pts',(7.74067935838542,-71.1882021394895,
-55.3981861905384));
#184921=CARTESIAN_POINT('Ctrl Pts',(7.72858942076698,-71.1920513333967,
-55.4042803599328));
#184922=CARTESIAN_POINT('Ctrl Pts',(7.71666532190953,-71.195999024024,-55.4109499585248));
#184923=CARTESIAN_POINT('Ctrl Pts',(7.71368430355678,-71.1969859445748,
-55.4126173546145));
#184924=CARTESIAN_POINT('Ctrl Pts',(7.7107136939813,-71.1979790030223,-55.4143206650124));
#184925=CARTESIAN_POINT('Ctrl Pts',(7.70775465049132,-71.1989780231378,
-55.4160597890549));
#184926=CARTESIAN_POINT('Ctrl Pts',(7.69950783403543,-71.2017622794544,
-55.4209067055744));
#184927=CARTESIAN_POINT('Ctrl Pts',(7.69133583163375,-71.2045985436463,
-55.4260385615872));
#184928=CARTESIAN_POINT('Ctrl Pts',(7.68327221711032,-71.2074785661779,
-55.4314358850195));
#184929=CARTESIAN_POINT('Ctrl Pts',(7.66246480526368,-71.2149101980804,
-55.4453631791875));
#184930=CARTESIAN_POINT('Ctrl Pts',(7.64235304315307,-71.2226426260351,
-55.4610765570766));
#184931=CARTESIAN_POINT('Ctrl Pts',(7.62319591956619,-71.2306314343771,
-55.478378275891));
#184932=CARTESIAN_POINT('Ctrl Pts',(7.60671393753606,-71.2375046685,-55.4932639458245));
#184933=CARTESIAN_POINT('Ctrl Pts',(7.59094155712043,-71.2445660091722,
-55.5093204534968));
#184934=CARTESIAN_POINT('Ctrl Pts',(7.57601858380446,-71.2517900510317,
-55.526411754027));
#184935=CARTESIAN_POINT('Ctrl Pts',(7.56579096848368,-71.2567411234243,
-55.5381254550068));
#184936=CARTESIAN_POINT('Ctrl Pts',(7.555961737699,-71.2617687656666,-55.5503253156747));
#184937=CARTESIAN_POINT('Ctrl Pts',(7.54657201875478,-71.2668653200254,
-55.5629668564504));
#184938=CARTESIAN_POINT('Ctrl Pts',(7.54416897604539,-71.2681696442408,
-55.5662021143507));
#184939=CARTESIAN_POINT('Ctrl Pts',(7.54179496034111,-71.2694783484373,
-55.5694659659879));
#184940=CARTESIAN_POINT('Ctrl Pts',(7.53945105296537,-71.2707910522752,
-55.5727570060984));
#184941=CARTESIAN_POINT('Ctrl Pts',(7.53513871124294,-71.2732061765195,
-55.5788118910846));
#184942=CARTESIAN_POINT('Ctrl Pts',(7.5309232906607,-71.2756374896449,-55.5849635221776));
#184943=CARTESIAN_POINT('Ctrl Pts',(7.52680908600444,-71.2780824878212,
-55.5912018872169));
#184944=CARTESIAN_POINT('Ctrl Pts',(7.52498538384955,-71.2791662813647,
-55.5939671652513));
#184945=CARTESIAN_POINT('Ctrl Pts',(7.52291658093658,-71.2804108673737,
-55.5971588684365));
#184946=CARTESIAN_POINT('Ctrl Pts',(7.52107659255899,-71.2815341427215,
-55.6000507784099));
#184947=CARTESIAN_POINT('Ctrl Pts',(7.51981528719233,-71.2823041439028,
-55.6020331722195));
#184948=CARTESIAN_POINT('Ctrl Pts',(7.51866042720015,-71.2830169397287,
-55.6038735813195));
#184949=CARTESIAN_POINT('Ctrl Pts',(7.5177546815274,-71.283579827305,-55.6053281505645));
#184950=CARTESIAN_POINT('Ctrl Pts',(7.50884650286416,-71.2891159322487,
-55.6196341120529));
#184951=CARTESIAN_POINT('Ctrl Pts',(7.50024952653351,-71.2948630784978,
-55.6346931994416));
#184952=CARTESIAN_POINT('Ctrl Pts',(7.49204715080729,-71.3007868659789,
-55.6504666068426));
#184953=CARTESIAN_POINT('Ctrl Pts',(7.48063639476581,-71.3090277581357,
-55.6724098230282));
#184954=CARTESIAN_POINT('Ctrl Pts',(7.46999669255816,-71.3176307939435,
-55.6957377083987));
#184955=CARTESIAN_POINT('Ctrl Pts',(7.46034213011195,-71.326574450456,-55.7203187323114));
#184956=CARTESIAN_POINT('Ctrl Pts',(7.45322822633404,-71.333164527656,-55.7384311055911));
#184957=CARTESIAN_POINT('Ctrl Pts',(7.44664909626611,-71.3399387392636,
-55.7572206846394));
#184958=CARTESIAN_POINT('Ctrl Pts',(7.44067748575595,-71.3468921359277,
-55.7766331127628));
#184959=CARTESIAN_POINT('Ctrl Pts',(7.43854478555646,-71.3493754711063,
-55.7835660648133));
#184960=CARTESIAN_POINT('Ctrl Pts',(7.43648958483996,-71.3518816220817,
-55.7905782755251));
#184961=CARTESIAN_POINT('Ctrl Pts',(7.43451563366501,-71.3544095298621,
-55.7976646694261));
#184962=CARTESIAN_POINT('Ctrl Pts',(7.43334182825126,-71.3559127442656,
-55.8018785768573));
#184963=CARTESIAN_POINT('Ctrl Pts',(7.43219623109102,-71.3574242320433,
-55.8061199279847));
#184964=CARTESIAN_POINT('Ctrl Pts',(7.43107929389869,-71.3589437211669,
-55.8103877195221));
#184965=CARTESIAN_POINT('Ctrl Pts',(7.4236300003487,-71.3690777919146,-55.8388513002773));
#184966=CARTESIAN_POINT('Ctrl Pts',(7.41747275315307,-71.3795491841635,
-55.8684398208395));
#184967=CARTESIAN_POINT('Ctrl Pts',(7.41266945915069,-71.3903109707646,
-55.898939933161));
#184968=CARTESIAN_POINT('Ctrl Pts',(7.4076670564432,-71.4015188606843,-55.9307043524075));
#184969=CARTESIAN_POINT('Ctrl Pts',(7.40413342652849,-71.4130416748627,
-55.9634570188779));
#184970=CARTESIAN_POINT('Ctrl Pts',(7.4020940672613,-71.4248176732263,-55.996921242169));
#184971=CARTESIAN_POINT('Ctrl Pts',(7.40069675959774,-71.4328862333001,
-56.0198499219811));
#184972=CARTESIAN_POINT('Ctrl Pts',(7.4,-71.4410734654608,-56.0431118800405));
#184973=CARTESIAN_POINT('Ctrl Pts',(7.4,-71.4493575166339,-56.06661116875));
#184974=CARTESIAN_POINT('Ctrl Pts',(7.4,-72.58000002,-58.1594740865074));
#184975=CARTESIAN_POINT('Ctrl Pts',(7.4,-72.58000002,-58.0551776270551));
#184976=CARTESIAN_POINT('Ctrl Pts',(7.4,-72.5736287847411,-57.9519715312753));
#184977=CARTESIAN_POINT('Ctrl Pts',(7.4,-72.5609286762394,-57.8498358231105));
#184978=CARTESIAN_POINT('Ctrl Pts',(7.4,-72.5482285677376,-57.7477001149456));
#184979=CARTESIAN_POINT('Ctrl Pts',(7.39999999935597,-72.529198463361,-57.6466357793308));
#184980=CARTESIAN_POINT('Ctrl Pts',(7.40000000064314,-72.5039045953935,
-57.5466462680235));
#184981=CARTESIAN_POINT('Ctrl Pts',(7.40000000122792,-72.4924131270627,
-57.5012191983453));
#184982=CARTESIAN_POINT('Ctrl Pts',(7.40000000179748,-72.4796171505751,
-57.4560136230692));
#184983=CARTESIAN_POINT('Ctrl Pts',(7.40000000193861,-72.4655224562879,
-57.4110306599075));
#184984=CARTESIAN_POINT('Ctrl Pts',(7.40000000231984,-72.4274510918893,
-57.2895265855827));
#184985=CARTESIAN_POINT('Ctrl Pts',(7.4000000004226,-72.3798384459848,-57.1705512406855));
#184986=CARTESIAN_POINT('Ctrl Pts',(7.40000000013593,-72.3241837880397,
-57.0571398660674));
#184987=CARTESIAN_POINT('Ctrl Pts',(7.40000000006153,-72.3097383663643,
-57.0277034237349));
#184988=CARTESIAN_POINT('Ctrl Pts',(7.40000000003645,-72.2947325387356,
-56.9985778271777));
#184989=CARTESIAN_POINT('Ctrl Pts',(7.40000000002765,-72.279165204543,-56.9697637092872));
#184990=CARTESIAN_POINT('Ctrl Pts',(7.40000000000257,-72.2347715487634,
-56.8875939546328));
#184991=CARTESIAN_POINT('Ctrl Pts',(7.40000000007907,-72.18577952644,-56.8079051030792));
#184992=CARTESIAN_POINT('Ctrl Pts',(7.40000000044821,-72.1321711779399,
-56.7307944085666));
#184993=CARTESIAN_POINT('Ctrl Pts',(7.40000000085049,-72.0737492661551,
-56.6467598445757));
#184994=CARTESIAN_POINT('Ctrl Pts',(7.40000000144702,-72.0094938737862,
-56.5655636032011));
#184995=CARTESIAN_POINT('Ctrl Pts',(7.40000000089367,-71.941102656717,-56.4892360541651));
#184996=CARTESIAN_POINT('Ctrl Pts',(7.40000000083676,-71.9340690507475,
-56.4813862464333));
#184997=CARTESIAN_POINT('Ctrl Pts',(7.40000000077119,-71.9269917258042,
-56.4735878952506));
#184998=CARTESIAN_POINT('Ctrl Pts',(7.4000000007,-71.9198725431757,-56.465843179204));
#184999=CARTESIAN_POINT('Ctrl Pts',(7.40000000060499,-71.9103706657815,
-56.4555064107617));
#185000=CARTESIAN_POINT('Ctrl Pts',(7.40000000052617,-71.9007927917902,
-56.4452629042245));
#185001=CARTESIAN_POINT('Ctrl Pts',(7.40000000046129,-71.8911429761284,
-56.4351175107121));
#185002=CARTESIAN_POINT('Ctrl Pts',(7.39999999996768,-71.817727207018,-56.357931386775));
#185003=CARTESIAN_POINT('Ctrl Pts',(7.39999999939412,-71.7397944141584,
-56.285795401294));
#185004=CARTESIAN_POINT('Ctrl Pts',(7.40000000114364,-71.6572752456049,
-56.2186315211947));
#185005=CARTESIAN_POINT('Ctrl Pts',(7.40000000147217,-71.6417795999254,
-56.206019328092));
#185006=CARTESIAN_POINT('Ctrl Pts',(7.40000000193345,-71.6261221119199,
-56.1935825531786));
#185007=CARTESIAN_POINT('Ctrl Pts',(7.40000000264863,-71.6103021593138,
-56.1813208069962));
#185008=CARTESIAN_POINT('Ctrl Pts',(7.40000000499281,-71.558447829008,-56.1411294959033));
#185009=CARTESIAN_POINT('Ctrl Pts',(7.40000000927177,-71.5046891439978,
-56.1028356287388));
#185010=CARTESIAN_POINT('Ctrl Pts',(7.40000002552836,-71.4493575166295,
-56.0666111687568));
#185011=CARTESIAN_POINT('Origin',(7.4,67.7009572055632,-55.24995));
#185012=CARTESIAN_POINT('',(7.4,-71.449357516634,-60.42825533736));
#185013=CARTESIAN_POINT('',(7.4,-71.449357516634,-55.24995));
#185014=CARTESIAN_POINT('Origin',(7.4,-69.2744516168521,-60.2813964156253));
#185015=CARTESIAN_POINT('',(7.4,-71.5626363369615,-176.798439391084));
#185016=CARTESIAN_POINT('Ctrl Pts',(7.4,-71.449357516634,-60.42825533736));
#185017=CARTESIAN_POINT('Ctrl Pts',(7.39999999999997,-70.886896756869,-60.42825533736));
#185018=CARTESIAN_POINT('Ctrl Pts',(6.84141371258755,-70.9528017323285,
-60.42825533736));
#185019=CARTESIAN_POINT('Ctrl Pts',(7.4,-71.4493574998816,-60.6471383113761));
#185020=CARTESIAN_POINT('Ctrl Pts',(7.39999999999996,-70.8868967471692,
-60.5644399462782));
#185021=CARTESIAN_POINT('Ctrl Pts',(6.84141371452047,-70.9528017321005,
-60.574175588166));
#185022=CARTESIAN_POINT('Ctrl Pts',(7.4,-71.4018249198588,-60.8620307958147));
#185023=CARTESIAN_POINT('Ctrl Pts',(7.39999999999997,-70.85979500338,-60.6978441698658));
#185024=CARTESIAN_POINT('Ctrl Pts',(6.84320633698782,-70.9209010052172,
-60.7174412822399));
#185025=CARTESIAN_POINT('Ctrl Pts',(7.4,-71.3078420373655,-61.0621827299711));
#185026=CARTESIAN_POINT('Ctrl Pts',(7.39999999999996,-70.8042142666047,
-60.8257004209668));
#185027=CARTESIAN_POINT('Ctrl Pts',(6.84677576889373,-70.8578246683297,
-60.8508735991007));
#185028=CARTESIAN_POINT('',(6.9,-70.949357516634,-60.42825533736));
#185029=CARTESIAN_POINT('Origin',(6.9,-71.449357516634,-60.42825533736));
#185030=CARTESIAN_POINT('',(6.84141371258755,-70.9528017323285,-60.42825533736));
#185031=CARTESIAN_POINT('Origin',(6.9,-71.449357516634,-60.42825533736));
#185032=CARTESIAN_POINT('Origin',(6.92387266608663,-69.4955362780865,-60.3306855231676));
#185033=CARTESIAN_POINT('Origin',(0.,-12.9675000200281,-60.64995));
#185034=CARTESIAN_POINT('Origin',(0.,-12.9675000200281,-60.8508735991007));
#185035=CARTESIAN_POINT('Origin',(0.750000000000035,67.7009572055632,-55.24995));
#185036=CARTESIAN_POINT('',(0.749999999999964,-72.58000002,-174.689806803098));
#185037=CARTESIAN_POINT('',(0.749999999999965,-71.9542570083556,-176.344247731786));
#185038=CARTESIAN_POINT('Ctrl Pts',(0.749999999999964,-72.58000002,-174.689806803098));
#185039=CARTESIAN_POINT('Ctrl Pts',(0.749999999999964,-72.58000002,-174.831376286945));
#185040=CARTESIAN_POINT('Ctrl Pts',(0.750000000181377,-72.5681788618565,
-174.970941599173));
#185041=CARTESIAN_POINT('Ctrl Pts',(0.749999999141365,-72.5447649315039,
-175.108599805088));
#185042=CARTESIAN_POINT('Ctrl Pts',(0.749999998625103,-72.5331422713358,
-175.176933251143));
#185043=CARTESIAN_POINT('Ctrl Pts',(0.749999997778457,-72.5186622030691,
-175.244796569616));
#185044=CARTESIAN_POINT('Ctrl Pts',(0.749999996441189,-72.501348066122,
-175.312200510247));
#185045=CARTESIAN_POINT('Ctrl Pts',(0.749999994685787,-72.4786201957877,
-175.400680116672));
#185046=CARTESIAN_POINT('Ctrl Pts',(0.749999992058193,-72.4508191867992,
-175.488345833607));
#185047=CARTESIAN_POINT('Ctrl Pts',(0.749999988588697,-72.4183069147095,
-175.574298130555));
#185048=CARTESIAN_POINT('Ctrl Pts',(0.749999986546665,-72.3991712571463,
-175.624886834926));
#185049=CARTESIAN_POINT('Ctrl Pts',(0.749999987460588,-72.3784930874995,
-175.674621364589));
#185050=CARTESIAN_POINT('Ctrl Pts',(0.749999990785369,-72.3562980983165,
-175.723514264027));
#185051=CARTESIAN_POINT('Ctrl Pts',(0.749999992115961,-72.3474155677618,
-175.743081413602));
#185052=CARTESIAN_POINT('Ctrl Pts',(0.749999993758535,-72.3382895360991,
-175.762513592359));
#185053=CARTESIAN_POINT('Ctrl Pts',(0.749999995341682,-72.3289194940821,
-175.781810711456));
#185054=CARTESIAN_POINT('Ctrl Pts',(0.749999998527987,-72.3100609827057,
-175.820648844666));
#185055=CARTESIAN_POINT('Ctrl Pts',(0.749999999364237,-72.2901904086323,
-175.8590152493));
#185056=CARTESIAN_POINT('Ctrl Pts',(0.749999999592108,-72.2694003762988,
-175.896717968815));
#185057=CARTESIAN_POINT('Ctrl Pts',(0.749999999760363,-72.2540495109208,
-175.924556760134));
#185058=CARTESIAN_POINT('Ctrl Pts',(0.749999999832536,-72.2381324361931,
-175.952153763115));
#185059=CARTESIAN_POINT('Ctrl Pts',(0.749999998887563,-72.22169996255,-175.979441154676));
#185060=CARTESIAN_POINT('Ctrl Pts',(0.749999996495687,-72.1801067750972,
-176.048509854673));
#185061=CARTESIAN_POINT('Ctrl Pts',(0.749999993208358,-72.1348499287514,
-176.116013152083));
#185062=CARTESIAN_POINT('Ctrl Pts',(0.749999994093549,-72.0863465370719,
-176.181265394638));
#185063=CARTESIAN_POINT('Ctrl Pts',(0.749999994855056,-72.0446203524776,
-176.237400172511));
#185064=CARTESIAN_POINT('Ctrl Pts',(0.749999998190332,-72.0004927389814,
-176.291868658537));
#185065=CARTESIAN_POINT('Ctrl Pts',(0.749999999535633,-71.9542570083559,
-176.344247731786));
#185066=CARTESIAN_POINT('',(0.749999999999965,-71.9542570083556,-171.871644662643));
#185067=CARTESIAN_POINT('',(0.749999999999965,-71.8417317029411,-60.42825533736));
#185068=CARTESIAN_POINT('Origin',(0.749999999999965,-69.6146150315905,-60.2676349698354));
#185069=CARTESIAN_POINT('',(0.749999999999963,-71.8417317505524,-56.1920013490171));
#185070=CARTESIAN_POINT('',(0.749999999999965,-71.8417317029411,-55.24995));
#185071=CARTESIAN_POINT('',(0.749999999999964,-72.58000002,-57.9657868813819));
#185072=CARTESIAN_POINT('Ctrl Pts',(0.749999999999965,-71.8417319269066,
-56.1920012792715));
#185073=CARTESIAN_POINT('Ctrl Pts',(0.749999999999965,-71.8444758759865,
-56.1947266143563));
#185074=CARTESIAN_POINT('Ctrl Pts',(0.749999999999854,-71.8472142189877,
-56.1974588803415));
#185075=CARTESIAN_POINT('Ctrl Pts',(0.7499999999996,-71.849946925556,-56.2001980449111));
#185076=CARTESIAN_POINT('Ctrl Pts',(0.749999999995322,-71.8957971239686,
-56.2461565976726));
#185077=CARTESIAN_POINT('Ctrl Pts',(0.750000000361229,-71.9401028597197,
-56.2942420626375));
#185078=CARTESIAN_POINT('Ctrl Pts',(0.74999999895657,-71.9825277370108,
-56.3440358937271));
#185079=CARTESIAN_POINT('Ctrl Pts',(0.749999998672542,-71.9911062235932,
-56.3541044134062));
#185080=CARTESIAN_POINT('Ctrl Pts',(0.749999998292393,-71.9996079282015,
-56.3642426607221));
#185081=CARTESIAN_POINT('Ctrl Pts',(0.749999997746176,-72.0080302616703,
-56.3744470046658));
#185082=CARTESIAN_POINT('Ctrl Pts',(0.74999999604191,-72.0343090036282,
-56.4062858439066));
#185083=CARTESIAN_POINT('Ctrl Pts',(0.749999992814762,-72.0598149071135,
-56.4387765753063));
#185084=CARTESIAN_POINT('Ctrl Pts',(0.749999990764931,-72.0844669777911,
-56.471823595159));
#185085=CARTESIAN_POINT('Ctrl Pts',(0.7499999887151,-72.1091190484687,-56.5048706150116));
#185086=CARTESIAN_POINT('Ctrl Pts',(0.74999998878556,-72.1329172515315,
-56.5384738714876));
#185087=CARTESIAN_POINT('Ctrl Pts',(0.749999992523647,-72.1557838559918,
-56.5725357961293));
#185088=CARTESIAN_POINT('Ctrl Pts',(0.749999997741391,-72.1877018007307,
-56.6200805302109));
#185089=CARTESIAN_POINT('Ctrl Pts',(0.749999998819484,-72.2179714721241,
-56.6686674551481));
#185090=CARTESIAN_POINT('Ctrl Pts',(0.749999999429074,-72.2464142286222,
-56.7180788042008));
#185091=CARTESIAN_POINT('Ctrl Pts',(0.750000000419556,-72.2926289656526,
-56.7983640080259));
#185092=CARTESIAN_POINT('Ctrl Pts',(0.749999999999578,-72.3344223494519,
-56.8812169184766));
#185093=CARTESIAN_POINT('Ctrl Pts',(0.749999999999555,-72.3716419026412,
-56.9665912683872));
#185094=CARTESIAN_POINT('Ctrl Pts',(0.749999999999551,-72.3771587620865,
-56.9792458611572));
#185095=CARTESIAN_POINT('Ctrl Pts',(0.749999999999476,-72.3825752068175,
-56.9919557956391));
#185096=CARTESIAN_POINT('Ctrl Pts',(0.749999999999378,-72.3878908196252,
-57.0047208623372));
#185097=CARTESIAN_POINT('Ctrl Pts',(0.749999999999364,-72.3886377760633,
-57.0065146251825));
#185098=CARTESIAN_POINT('Ctrl Pts',(0.749999999999346,-72.389382748593,
-57.0083094879105));
#185099=CARTESIAN_POINT('Ctrl Pts',(0.749999999999324,-72.3901257364801,
-57.0101054509238));
#185100=CARTESIAN_POINT('Ctrl Pts',(0.749999999998099,-72.4318199510488,
-57.1108894186501));
#185101=CARTESIAN_POINT('Ctrl Pts',(0.749999999915445,-72.4672597866091,
-57.2155313871763));
#185102=CARTESIAN_POINT('Ctrl Pts',(0.749999999861768,-72.4953436211357,
-57.3206699820973));
#185103=CARTESIAN_POINT('Ctrl Pts',(0.749999999835408,-72.5091351036103,
-57.3723017166415));
#185104=CARTESIAN_POINT('Ctrl Pts',(0.749999999849788,-72.5212576085903,
-57.4242193465116));
#185105=CARTESIAN_POINT('Ctrl Pts',(0.749999999908996,-72.53169711994,-57.4764233217448));
#185106=CARTESIAN_POINT('Ctrl Pts',(0.75000000009092,-72.5637736078163,
-57.6368254825896));
#185107=CARTESIAN_POINT('Ctrl Pts',(0.749999999999964,-72.58000002,-57.7999242188348));
#185108=CARTESIAN_POINT('Ctrl Pts',(0.749999999999964,-72.58000002,-57.9657868813819));
#185109=CARTESIAN_POINT('',(0.749999999999964,-72.58000002,-174.687529226493));
#185110=CARTESIAN_POINT('Ctrl Pts',(0.749999999999965,-71.701161634982,
-61.0621827299711));
#185111=CARTESIAN_POINT('Ctrl Pts',(0.749999999999965,-71.2566817467534,
-60.8548714197835));
#185112=CARTESIAN_POINT('Ctrl Pts',(1.24035792914739,-71.2481103336038,
-60.8508735991007));
#185113=CARTESIAN_POINT('Ctrl Pts',(0.749999999999965,-71.7936527766986,
-60.8638797025928));
#185114=CARTESIAN_POINT('Ctrl Pts',(0.749999999999964,-71.3194598672011,
-60.7217601410268));
#185115=CARTESIAN_POINT('Ctrl Pts',(1.23971725581624,-71.3097847042778,
-60.7186716617645));
#185116=CARTESIAN_POINT('Ctrl Pts',(0.749999999999965,-71.8417316989903,
-60.6492890757558));
#185117=CARTESIAN_POINT('Ctrl Pts',(0.749999999999964,-71.3522348667501,
-60.5771488614746));
#185118=CARTESIAN_POINT('Ctrl Pts',(1.23938654221847,-71.3418443611191,
-60.5756111021815));
#185119=CARTESIAN_POINT('Ctrl Pts',(0.749999999999965,-71.8417317029411,
-60.42825533736));
#185120=CARTESIAN_POINT('Ctrl Pts',(0.749999999999964,-71.3522348691612,
-60.4282553373599));
#185121=CARTESIAN_POINT('Ctrl Pts',(1.2393865421354,-71.3418443611208,-60.42825533736));
#185122=CARTESIAN_POINT('',(1.2393865421354,-71.3418443611208,-60.42825533736));
#185123=CARTESIAN_POINT('Origin',(1.25481291792095,-69.8566648529799,-60.3211428649281));
#185124=CARTESIAN_POINT('Origin',(1.24999999999996,-71.8417317029411,-60.42825533736));
#185125=CARTESIAN_POINT('Ctrl Pts',(0.749999999999964,-72.58000002,-57.9657868813819));
#185126=CARTESIAN_POINT('Ctrl Pts',(0.749999999999964,-73.08000002,-57.9657868813819));
#185127=CARTESIAN_POINT('Ctrl Pts',(0.249999999999964,-73.08000002,-57.9657868813819));
#185128=CARTESIAN_POINT('Ctrl Pts',(0.749999999999964,-72.5800000140225,
-57.7459735178474));
#185129=CARTESIAN_POINT('Ctrl Pts',(0.749999999999964,-73.0799097169388,
-57.7020347823602));
#185130=CARTESIAN_POINT('Ctrl Pts',(0.250090304006367,-73.08000002,-57.7020110302663));
#185131=CARTESIAN_POINT('Ctrl Pts',(0.749999999999964,-72.5514958309333,
-57.5309525432158));
#185132=CARTESIAN_POINT('Ctrl Pts',(0.749999999999975,-73.0456227684187,
-57.4440313928443));
#185133=CARTESIAN_POINT('Ctrl Pts',(0.250178150913126,-73.0457949912512,
-57.4439860415223));
#185134=CARTESIAN_POINT('Ctrl Pts',(0.749999999999964,-72.4672504799085,
-57.2155332517716));
#185135=CARTESIAN_POINT('Ctrl Pts',(0.749999999999959,-72.9444091558477,
-57.0655786327141));
#185136=CARTESIAN_POINT('Ctrl Pts',(0.250306370454135,-72.9447005728246,
-57.0654831530319));
#185137=CARTESIAN_POINT('Ctrl Pts',(0.749999999999964,-72.4318183244811,
-57.1108895827629));
#185138=CARTESIAN_POINT('Ctrl Pts',(0.749999999999965,-72.9018554492066,
-56.9400333127282));
#185139=CARTESIAN_POINT('Ctrl Pts',(0.25034879630597,-72.9021819864826,
-56.9399108365871));
#185140=CARTESIAN_POINT('Ctrl Pts',(0.749999999999964,-72.3484316704448,
-56.9093219305338));
#185141=CARTESIAN_POINT('Ctrl Pts',(0.749999999999964,-72.8017292323873,
-56.6982147960383));
#185142=CARTESIAN_POINT('Ctrl Pts',(0.250430320614374,-72.8021179994285,
-56.6980298209841));
#185143=CARTESIAN_POINT('Ctrl Pts',(0.749999999999965,-72.300481803901,
-56.8120054092621));
#185144=CARTESIAN_POINT('Ctrl Pts',(0.749999999999975,-72.7441631076294,
-56.581469426742));
#185145=CARTESIAN_POINT('Ctrl Pts',(0.250469580226035,-72.744578160532,
-56.5812500750007));
#185146=CARTESIAN_POINT('Ctrl Pts',(0.749999999999965,-72.1382169632082,
-56.5302613678863));
#185147=CARTESIAN_POINT('Ctrl Pts',(0.74999999999994,-72.5493874743356,
-56.2435031793822));
#185148=CARTESIAN_POINT('Ctrl Pts',(0.250582991914968,-72.5498603521484,
-56.2431574556907));
#185149=CARTESIAN_POINT('Ctrl Pts',(0.749999999999965,-72.0032732927043,
-56.3539043654751));
#185150=CARTESIAN_POINT('Ctrl Pts',(0.749999999999422,-72.3874332788213,
-56.0319576106046));
#185151=CARTESIAN_POINT('Ctrl Pts',(0.250653625589273,-72.3879279481205,
-56.0315291953545));
#185152=CARTESIAN_POINT('Ctrl Pts',(0.749999999999965,-71.6966197023802,
-56.0464925782632));
#185153=CARTESIAN_POINT('Ctrl Pts',(0.750000000000507,-72.0194499168863,
-55.6632379181992));
#185154=CARTESIAN_POINT('Ctrl Pts',(0.250776334581247,-72.0199436379809,
-55.6626353009023));
#185155=CARTESIAN_POINT('Ctrl Pts',(0.749999999999965,-71.5244049571092,
-55.9134072123415));
#185156=CARTESIAN_POINT('Ctrl Pts',(0.749999999997373,-71.8128142650138,
-55.5036164406726));
#185157=CARTESIAN_POINT('Ctrl Pts',(0.250829232083772,-71.8132859417639,
-55.5029329728744));
#185158=CARTESIAN_POINT('Ctrl Pts',(0.749999999999965,-71.3337760574596,
-55.8029033796444));
#185159=CARTESIAN_POINT('Ctrl Pts',(0.749999999999965,-71.5840941797283,
-55.3710824677091));
#185160=CARTESIAN_POINT('Ctrl Pts',(0.250873059487692,-71.5845312649516,
-55.3703284570208));
#185161=CARTESIAN_POINT('',(0.250869887203108,-71.6009673739886,-55.3799259279409));
#185162=CARTESIAN_POINT('Ctrl Pts',(0.749999999999961,-71.841731660912,
-56.1920013789646));
#185163=CARTESIAN_POINT('Ctrl Pts',(0.749999996232492,-71.8203840101541,
-56.128102426568));
#185164=CARTESIAN_POINT('Ctrl Pts',(0.747131052735305,-71.8000607354501,
-56.0666787373699));
#185165=CARTESIAN_POINT('Ctrl Pts',(0.741078423025563,-71.7810191778214,
-56.0081419188211));
#185166=CARTESIAN_POINT('Ctrl Pts',(0.737825285209295,-71.770784814549,
-55.9766798358593));
#185167=CARTESIAN_POINT('Ctrl Pts',(0.733652115393616,-71.7609200326615,
-55.9460509739298));
#185168=CARTESIAN_POINT('Ctrl Pts',(0.728509395282827,-71.7514597327231,
-55.9163159881819));
#185169=CARTESIAN_POINT('Ctrl Pts',(0.722846494412134,-71.7410425333414,
-55.8835733397285));
#185170=CARTESIAN_POINT('Ctrl Pts',(0.716008517443964,-71.7311170853223,
-55.8519328895509));
#185171=CARTESIAN_POINT('Ctrl Pts',(0.707973883712583,-71.7217347566402,
-55.8215590914709));
#185172=CARTESIAN_POINT('Ctrl Pts',(0.705572376408577,-71.7189304308163,
-55.812480532276));
#185173=CARTESIAN_POINT('Ctrl Pts',(0.703064221368542,-71.716174534353,
-55.8035149179954));
#185174=CARTESIAN_POINT('Ctrl Pts',(0.70044952091513,-71.7134681966337,
-55.7946660664912));
#185175=CARTESIAN_POINT('Ctrl Pts',(0.69476821762457,-71.707587781013,-55.7754390039406));
#185176=CARTESIAN_POINT('Ctrl Pts',(0.688583995937285,-71.701942135274,
-55.7567665704553));
#185177=CARTESIAN_POINT('Ctrl Pts',(0.681909838458245,-71.6965464723651,
-55.7386975291575));
#185178=CARTESIAN_POINT('Ctrl Pts',(0.678572759718724,-71.6938486409106,
-55.7296630085086));
#185179=CARTESIAN_POINT('Ctrl Pts',(0.675113361509717,-71.6912133527727,
-55.7207792739838));
#185180=CARTESIAN_POINT('Ctrl Pts',(0.671534603530799,-71.6886427442802,
-55.7120524393633));
#185181=CARTESIAN_POINT('Ctrl Pts',(0.669745224541341,-71.6873574400339,
-55.7076890220531));
#185182=CARTESIAN_POINT('Ctrl Pts',(0.667926017606087,-71.6860883098401,
-55.7033648240785));
#185183=CARTESIAN_POINT('Ctrl Pts',(0.666077427506471,-71.6848356434166,
-55.6990805767485));
#185184=CARTESIAN_POINT('Ctrl Pts',(0.664935253287673,-71.6840616679993,
-55.6964335016354));
#185185=CARTESIAN_POINT('Ctrl Pts',(0.663995068024676,-71.6834353209859,
-55.6942867742518));
#185186=CARTESIAN_POINT('Ctrl Pts',(0.662863955044102,-71.6826935920275,
-55.691739575195));
#185187=CARTESIAN_POINT('Ctrl Pts',(0.662164380356346,-71.6822348449233,
-55.6901641746688));
#185188=CARTESIAN_POINT('Ctrl Pts',(0.661391294896625,-71.6817321390306,
-55.6884359887418));
#185189=CARTESIAN_POINT('Ctrl Pts',(0.660444402984383,-71.6811259913739,
-55.6863481504284));
#185190=CARTESIAN_POINT('Ctrl Pts',(0.650608220603443,-71.6748294132496,
-55.6646599744419));
#185191=CARTESIAN_POINT('Ctrl Pts',(0.639939411226591,-71.668891690002,
-55.6438739328685));
#185192=CARTESIAN_POINT('Ctrl Pts',(0.628369170664437,-71.6633099906125,
-55.6239326668601));
#185193=CARTESIAN_POINT('Ctrl Pts',(0.616621675343986,-71.6576427802286,
-55.6036859029437));
#185194=CARTESIAN_POINT('Ctrl Pts',(0.604083829173103,-71.652372581358,
-55.5845338609078));
#185195=CARTESIAN_POINT('Ctrl Pts',(0.590719085952487,-71.6474786056494,
-55.5664598731969));
#185196=CARTESIAN_POINT('Ctrl Pts',(0.57770892323427,-71.6427144721935,
-55.5488654071301));
#185197=CARTESIAN_POINT('Ctrl Pts',(0.563942592492347,-71.6383206108158,
-55.532342364749));
#185198=CARTESIAN_POINT('Ctrl Pts',(0.549514613866369,-71.6343052814187,
-55.5170103376903));
#185199=CARTESIAN_POINT('Ctrl Pts',(0.541878516611505,-71.6321801434087,
-55.5088957671903));
#185200=CARTESIAN_POINT('Ctrl Pts',(0.53405774216662,-71.6301608945464,
-55.5011144209525));
#185201=CARTESIAN_POINT('Ctrl Pts',(0.526071135343876,-71.6282476732945,
-55.4936805695738));
#185202=CARTESIAN_POINT('Ctrl Pts',(0.522626356583135,-71.6274224637807,
-55.4904742049801));
#185203=CARTESIAN_POINT('Ctrl Pts',(0.519393187313092,-71.6266733711271,
-55.4875523510514));
#185204=CARTESIAN_POINT('Ctrl Pts',(0.516052248208152,-71.6259220367257,
-55.4846129885499));
#185205=CARTESIAN_POINT('Ctrl Pts',(0.512850492195839,-71.6252020028186,
-55.4817960795116));
#185206=CARTESIAN_POINT('Ctrl Pts',(0.509549728098309,-71.6244799207866,
-55.4789630294608));
#185207=CARTESIAN_POINT('Ctrl Pts',(0.505845569683937,-71.623698353505,
-55.4758859675463));
#185208=CARTESIAN_POINT('Ctrl Pts',(0.504783854460946,-71.6234743345005,
-55.475003995689));
#185209=CARTESIAN_POINT('Ctrl Pts',(0.503688841818574,-71.6232455061024,
-55.4741022375036));
#185210=CARTESIAN_POINT('Ctrl Pts',(0.502552953881557,-71.6230107197811,
-55.4731760177748));
#185211=CARTESIAN_POINT('Ctrl Pts',(0.490275767922547,-71.6204730439836,
-55.4631650197884));
#185212=CARTESIAN_POINT('Ctrl Pts',(0.477525582018539,-71.6181363231932,
-55.4538148724768));
#185213=CARTESIAN_POINT('Ctrl Pts',(0.464337021242048,-71.6160065604269,
-55.4451889526195));
#185214=CARTESIAN_POINT('Ctrl Pts',(0.447262090742039,-71.6132492048798,
-55.4340211698296));
#185215=CARTESIAN_POINT('Ctrl Pts',(0.429665697481203,-71.6108662887343,
-55.4242021638032));
#185216=CARTESIAN_POINT('Ctrl Pts',(0.411688401881651,-71.6088670387269,
-55.4158238229682));
#185217=CARTESIAN_POINT('Ctrl Pts',(0.393843346884726,-71.6068824951599,
-55.4075071130295));
#185218=CARTESIAN_POINT('Ctrl Pts',(0.375623361038916,-71.6052759751029,
-55.4006101353856));
#185219=CARTESIAN_POINT('Ctrl Pts',(0.35717783270288,-71.6040442407152,
-55.3951748301981));
#185220=CARTESIAN_POINT('Ctrl Pts',(0.338866566196649,-71.6028214719104,
-55.3897790876626));
#185221=CARTESIAN_POINT('Ctrl Pts',(0.320333393067772,-71.6019680183095,
-55.3858239119413));
#185222=CARTESIAN_POINT('Ctrl Pts',(0.301730629650085,-71.6014689796738,
-55.3833008360601));
#185223=CARTESIAN_POINT('Ctrl Pts',(0.28479589526439,-71.6010146876659,
-55.3810039934392));
#185224=CARTESIAN_POINT('Ctrl Pts',(0.267803743668673,-71.6008539429058,
-55.3798933886721));
#185225=CARTESIAN_POINT('Ctrl Pts',(0.250869887203208,-71.6009673739965,
-55.3799259279328));
#185226=CARTESIAN_POINT('',(0.249999999999964,-73.08000002,-57.9657868813819));
#185227=CARTESIAN_POINT('Ctrl Pts',(0.249999999999963,-73.08000002,-57.9657868813819));
#185228=CARTESIAN_POINT('Ctrl Pts',(0.250042469931417,-73.080000019999,
-57.8920441993433));
#185229=CARTESIAN_POINT('Ctrl Pts',(0.250086371965619,-73.0772779883399,
-57.8175078453759));
#185230=CARTESIAN_POINT('Ctrl Pts',(0.250131098523594,-73.0716768447104,
-57.7424712607537));
#185231=CARTESIAN_POINT('Ctrl Pts',(0.250175351214089,-73.0661350438948,
-57.668229671293));
#185232=CARTESIAN_POINT('Ctrl Pts',(0.250220410087223,-73.0577743703455,
-57.5934988530362));
#185233=CARTESIAN_POINT('Ctrl Pts',(0.250265626043886,-73.0464826175312,
-57.5185941346588));
#185234=CARTESIAN_POINT('Ctrl Pts',(0.250310434748604,-73.0352925674925,
-57.4443640695335));
#185235=CARTESIAN_POINT('Ctrl Pts',(0.250355396587183,-73.0212236537723,
-57.3699637680883));
#185236=CARTESIAN_POINT('Ctrl Pts',(0.250399835547614,-73.0042119982681,
-57.2957233809505));
#185237=CARTESIAN_POINT('Ctrl Pts',(0.25044394534943,-72.9873263478039,
-57.2220328910844));
#185238=CARTESIAN_POINT('Ctrl Pts',(0.250487538732826,-72.9675411584413,
-57.1485005658174));
#185239=CARTESIAN_POINT('Ctrl Pts',(0.250529928559043,-72.9448431246011,
-57.0754636929159));
#185240=CARTESIAN_POINT('Ctrl Pts',(0.250572072640272,-72.9222766772416,
-57.0028502340045));
#185241=CARTESIAN_POINT('Ctrl Pts',(0.250613025749873,-72.8968309609008,
-56.9307271493267));
#185242=CARTESIAN_POINT('Ctrl Pts',(0.250652106105929,-72.8685441528253,
-56.8594307921769));
#185243=CARTESIAN_POINT('Ctrl Pts',(0.250691023114669,-72.8403755774027,
-56.7884324381607));
#185244=CARTESIAN_POINT('Ctrl Pts',(0.250728081651377,-72.8093896477869,
-56.7182545754342));
#185245=CARTESIAN_POINT('Ctrl Pts',(0.250762621939711,-72.7756755277479,
-56.6492244236476));
#185246=CARTESIAN_POINT('Ctrl Pts',(0.250797078194219,-72.7420434315326,
-56.5803622168345));
#185247=CARTESIAN_POINT('Ctrl Pts',(0.250829027144611,-72.7056965763661,
-56.5126427849829));
#185248=CARTESIAN_POINT('Ctrl Pts',(0.250857847047447,-72.6667732478891,
-56.4463762751986));
#185249=CARTESIAN_POINT('Ctrl Pts',(0.250886657396073,-72.6278628230513,
-56.3801317337086));
#185250=CARTESIAN_POINT('Ctrl Pts',(0.250912339577454,-72.586377932768,
-56.3153397478542));
#185251=CARTESIAN_POINT('Ctrl Pts',(0.250934324442956,-72.5425029977862,
-56.2522861365262));
#185252=CARTESIAN_POINT('Ctrl Pts',(0.250956333737572,-72.4985793099114,
-56.1891624613686));
#185253=CARTESIAN_POINT('Ctrl Pts',(0.250974636461275,-72.452260682586,
-56.1277815480868));
#185254=CARTESIAN_POINT('Ctrl Pts',(0.250988730474407,-72.4037731304877,
-56.0683976530279));
#185255=CARTESIAN_POINT('Ctrl Pts',(0.25100286048415,-72.3551617394526,
-56.0088620893836));
#185256=CARTESIAN_POINT('Ctrl Pts',(0.251012759433403,-72.3043708505095,
-55.9513341800841));
#185257=CARTESIAN_POINT('Ctrl Pts',(0.25101800459919,-72.2516623010505,
-55.8960303301876));
#185258=CARTESIAN_POINT('Ctrl Pts',(0.251023288789269,-72.1985615973934,
-55.8403150169303));
#185259=CARTESIAN_POINT('Ctrl Pts',(0.251023849052114,-72.1435151798975,
-55.7868573130842));
#185260=CARTESIAN_POINT('Ctrl Pts',(0.251019348764074,-72.086816969245,
-55.7358323645543));
#185261=CARTESIAN_POINT('Ctrl Pts',(0.251014826609809,-72.0298432704859,
-55.6845594934481));
#185262=CARTESIAN_POINT('Ctrl Pts',(0.251005194309946,-71.9712023416134,
-55.6357432440695));
#185263=CARTESIAN_POINT('Ctrl Pts',(0.25099021352996,-71.911209329447,-55.5895111537473));
#185264=CARTESIAN_POINT('Ctrl Pts',(0.25097507537099,-71.8505860671018,
-55.5427933771403));
#185265=CARTESIAN_POINT('Ctrl Pts',(0.250954475679539,-71.7885828358966,
-55.4987144045882));
#185266=CARTESIAN_POINT('Ctrl Pts',(0.250928276758545,-71.7255319930884,
-55.4573528781666));
#185267=CARTESIAN_POINT('Ctrl Pts',(0.250911195986817,-71.684425069125,
-55.4303866229051));
#185268=CARTESIAN_POINT('Ctrl Pts',(0.25089173745834,-71.6428729679957,
-55.4045743425418));
#185269=CARTESIAN_POINT('Ctrl Pts',(0.250869887203029,-71.6009673739763,
-55.3799259279683));
#185270=CARTESIAN_POINT('Origin',(0.249999999999964,-72.58000002,-57.9657868813819));
#185271=CARTESIAN_POINT('Origin',(0.249999999999964,-72.58000002,-55.24995));
#185272=CARTESIAN_POINT('',(0.249999999999962,-73.08000002,-174.689806803098));
#185273=CARTESIAN_POINT('Origin',(0.249999999999964,-72.58000002,-174.689806803098));
#185274=CARTESIAN_POINT('',(0.249999999999964,-73.08000002,-57.9678366169137));
#185275=CARTESIAN_POINT('Ctrl Pts',(0.249999999999964,-73.08000002,-174.689806803097));
#185276=CARTESIAN_POINT('Ctrl Pts',(0.749999999999964,-73.08000002,-174.689806803097));
#185277=CARTESIAN_POINT('Ctrl Pts',(0.749999999999964,-72.58000002,-174.689806803097));
#185278=CARTESIAN_POINT('Ctrl Pts',(0.250096721285987,-73.08000002,-174.944087763949));
#185279=CARTESIAN_POINT('Ctrl Pts',(0.749999999999963,-73.0799033011073,
-174.944063234271));
#185280=CARTESIAN_POINT('Ctrl Pts',(0.749999999999964,-72.5800000142362,
-174.901707787501));
#185281=CARTESIAN_POINT('Ctrl Pts',(0.25019084538922,-73.0481762528639,
-175.193013365813));
#185282=CARTESIAN_POINT('Ctrl Pts',(0.749999999999965,-73.047991321912,
-175.192966486363));
#185283=CARTESIAN_POINT('Ctrl Pts',(0.749999999999964,-72.5534802154039,
-175.109145968138));
#185284=CARTESIAN_POINT('Ctrl Pts',(0.250374112266224,-72.9229204323206,
-175.680308208816));
#185285=CARTESIAN_POINT('Ctrl Pts',(0.749999999999964,-72.9225699879354,
-175.680169902411));
#185286=CARTESIAN_POINT('Ctrl Pts',(0.749999999999964,-72.4491003622499,
-175.515225349862));
#185287=CARTESIAN_POINT('Ctrl Pts',(0.250463183534996,-72.8282888567225,
-175.918532203572));
#185288=CARTESIAN_POINT('Ctrl Pts',(0.750000000001369,-72.8278715101479,
-175.918330718485));
#185289=CARTESIAN_POINT('Ctrl Pts',(0.749999999999965,-72.3702407172373,
-175.713745513771));
#185290=CARTESIAN_POINT('Ctrl Pts',(0.25062659166413,-72.5862295913911,
-176.357642327882));
#185291=CARTESIAN_POINT('Ctrl Pts',(0.74999999999856,-72.5857133666792,
-176.357282462775));
#185292=CARTESIAN_POINT('Ctrl Pts',(0.749999999999965,-72.1685246628573,
-176.079670924798));
#185293=CARTESIAN_POINT('Ctrl Pts',(0.250703242845797,-72.4354180409157,
-176.564734305741));
#185294=CARTESIAN_POINT('Ctrl Pts',(0.749999999997952,-72.4348744309047,
-176.56428717754));
#185295=CARTESIAN_POINT('Ctrl Pts',(0.749999999999965,-72.0428483696925,
-176.252247715791));
#185296=CARTESIAN_POINT('Ctrl Pts',(0.250838284668646,-72.090128509306,
-176.930952892336));
#185297=CARTESIAN_POINT('Ctrl Pts',(0.750000000001977,-72.0895755229708,
-176.930319469104));
#185298=CARTESIAN_POINT('Ctrl Pts',(0.749999999999965,-71.7551070954922,
-176.557430126179));
#185299=CARTESIAN_POINT('Ctrl Pts',(0.250896921774036,-71.8966556096658,
-177.090711302921));
#185300=CARTESIAN_POINT('Ctrl Pts',(0.749999999997485,-71.8961205198801,
-177.08999030776));
#185301=CARTESIAN_POINT('Ctrl Pts',(0.749999999999965,-71.5938796749303,
-176.690562238895));
#185302=CARTESIAN_POINT('Ctrl Pts',(0.250946592270043,-71.6818193327012,
-177.226378685119));
#185303=CARTESIAN_POINT('Ctrl Pts',(0.749999999999965,-71.6813148644928,
-177.225579834422));
#185304=CARTESIAN_POINT('Ctrl Pts',(0.749999999999965,-71.414849447251,
-176.803618488051));
#185305=CARTESIAN_POINT('',(0.250942965994138,-71.6973962901444,-177.216474798299));
#185306=CARTESIAN_POINT('Ctrl Pts',(0.25094296599405,-71.6973962901389,
-177.216474798276));
#185307=CARTESIAN_POINT('Ctrl Pts',(0.250976479214862,-71.760322042129,
-177.176193884541));
#185308=CARTESIAN_POINT('Ctrl Pts',(0.251003803266757,-71.822289052444,
-177.133208560261));
#185309=CARTESIAN_POINT('Ctrl Pts',(0.251025052218208,-71.8829682618455,
-177.087581567843));
#185310=CARTESIAN_POINT('Ctrl Pts',(0.251046127790315,-71.9431523634545,
-177.0423268657));
#185311=CARTESIAN_POINT('Ctrl Pts',(0.251061226926392,-72.0020689462363,
-176.994473421731));
#185312=CARTESIAN_POINT('Ctrl Pts',(0.251070576134496,-72.0594007051876,
-176.944133320408));
#185313=CARTESIAN_POINT('Ctrl Pts',(0.25107986405914,-72.1163566581376,
-176.89412319522));
#185314=CARTESIAN_POINT('Ctrl Pts',(0.251083477423211,-72.1717478547756,
-176.841659032887));
#185315=CARTESIAN_POINT('Ctrl Pts',(0.251081751302264,-72.2252765394361,
-176.786900255691));
#185316=CARTESIAN_POINT('Ctrl Pts',(0.251080033711072,-72.2785407081389,
-176.732412073046));
#185317=CARTESIAN_POINT('Ctrl Pts',(0.251073029808676,-72.3299601210376,
-176.675652156158));
#185318=CARTESIAN_POINT('Ctrl Pts',(0.251061176284639,-72.3792640075592,
-176.616823910038));
#185319=CARTESIAN_POINT('Ctrl Pts',(0.251049362132091,-72.4284041311798,
-176.558191061989));
#185320=CARTESIAN_POINT('Ctrl Pts',(0.251032731334361,-72.4754422161327,
-176.497503982321));
#185321=CARTESIAN_POINT('Ctrl Pts',(0.251011812305099,-72.520141292388,
-176.435005426744));
#185322=CARTESIAN_POINT('Ctrl Pts',(0.250990240328152,-72.5662355652342,
-176.370556097707));
#185323=CARTESIAN_POINT('Ctrl Pts',(0.250964108948217,-72.6098417978143,
-176.30418078364));
#185324=CARTESIAN_POINT('Ctrl Pts',(0.250934089145355,-72.6507433908404,
-176.236184599534));
#185325=CARTESIAN_POINT('Ctrl Pts',(0.25090499157123,-72.6903884591434,
-176.170277304395));
#185326=CARTESIAN_POINT('Ctrl Pts',(0.25087224249439,-72.727492393518,-176.10284794613));
#185327=CARTESIAN_POINT('Ctrl Pts',(0.250836518310456,-72.7619035974977,
-176.034201619033));
#185328=CARTESIAN_POINT('Ctrl Pts',(0.250800722749006,-72.7963835556372,
-175.965418135428));
#185329=CARTESIAN_POINT('Ctrl Pts',(0.250761941597354,-72.8281597947364,
-175.895413450691));
#185330=CARTESIAN_POINT('Ctrl Pts',(0.250720899474743,-72.8571292191755,
-175.824512204359));
#185331=CARTESIAN_POINT('Ctrl Pts',(0.250679716181218,-72.8861982885607,
-175.753367081905));
#185332=CARTESIAN_POINT('Ctrl Pts',(0.250636257835567,-72.9124411218246,
-175.681319886333));
#185333=CARTESIAN_POINT('Ctrl Pts',(0.250591278953596,-72.9358055216485,
-175.608706599455));
#185334=CARTESIAN_POINT('Ctrl Pts',(0.250544145622038,-72.9602890560385,
-175.532615198869));
#185335=CARTESIAN_POINT('Ctrl Pts',(0.250495344354186,-72.981611464156,
-175.455902966511));
#185336=CARTESIAN_POINT('Ctrl Pts',(0.250445742789475,-72.9997735060265,
-175.378953996231));
#185337=CARTESIAN_POINT('Ctrl Pts',(0.250397681398313,-73.0173716000327,
-175.304394361233));
#185338=CARTESIAN_POINT('Ctrl Pts',(0.250348870046398,-73.0320031038598,
-175.229613064406));
#185339=CARTESIAN_POINT('Ctrl Pts',(0.250300073860922,-73.0437215355442,
-175.154946852542));
#185340=CARTESIAN_POINT('Ctrl Pts',(0.250248932094337,-73.0560032598656,
-175.076691514717));
#185341=CARTESIAN_POINT('Ctrl Pts',(0.250197808860602,-73.0650851592926,
-174.99856341985));
#185342=CARTESIAN_POINT('Ctrl Pts',(0.250147532330345,-73.0710841986421,
-174.920924864984));
#185343=CARTESIAN_POINT('Ctrl Pts',(0.250097255800088,-73.0770832379916,
-174.843286310117));
#185344=CARTESIAN_POINT('Ctrl Pts',(0.25004782720234,-73.0800000199989,
-174.766137816945));
#185345=CARTESIAN_POINT('Ctrl Pts',(0.249999999999961,-73.08000002,-174.689806803098));
#185346=CARTESIAN_POINT('Ctrl Pts',(0.250942965994174,-71.697396290156,
-177.216474798319));
#185347=CARTESIAN_POINT('Ctrl Pts',(0.270264526385401,-71.6972689123026,
-177.216513071422));
#185348=CARTESIAN_POINT('Ctrl Pts',(0.289719933294543,-71.6975397265544,
-177.214938644682));
#185349=CARTESIAN_POINT('Ctrl Pts',(0.30909956798559,-71.6982247726489,
-177.211737182828));
#185350=CARTESIAN_POINT('Ctrl Pts',(0.328957416411424,-71.698926723007,
-177.208456721393));
#185351=CARTESIAN_POINT('Ctrl Pts',(0.348735110265057,-71.7000636457951,
-177.203467956048));
#185352=CARTESIAN_POINT('Ctrl Pts',(0.368198254111624,-71.7016407715696,
-177.196808079087));
#185353=CARTESIAN_POINT('Ctrl Pts',(0.374482450132035,-71.7021499887646,
-177.194657759867));
#185354=CARTESIAN_POINT('Ctrl Pts',(0.380733825865396,-71.7027050024855,
-177.192333627024));
#185355=CARTESIAN_POINT('Ctrl Pts',(0.386944469709064,-71.7033057202149,
-177.189838046772));
#185356=CARTESIAN_POINT('Ctrl Pts',(0.401084223294227,-71.7046733724069,
-177.184156366947));
#185357=CARTESIAN_POINT('Ctrl Pts',(0.415014553244461,-71.7062782430979,
-177.177584716033));
#185358=CARTESIAN_POINT('Ctrl Pts',(0.428650066650391,-71.7081181561605,
-177.170155344181));
#185359=CARTESIAN_POINT('Ctrl Pts',(0.437491216212795,-71.7093111399582,
-177.165338203401));
#185360=CARTESIAN_POINT('Ctrl Pts',(0.446206744620982,-71.7106026105523,
-177.160161774));
#185361=CARTESIAN_POINT('Ctrl Pts',(0.454779260000809,-71.7119923408229,
-177.154633350333));
#185362=CARTESIAN_POINT('Ctrl Pts',(0.459427949347712,-71.7127459614369,
-177.151635405965));
#185363=CARTESIAN_POINT('Ctrl Pts',(0.46403489949683,-71.7135285745735,
-177.148533580525));
#185364=CARTESIAN_POINT('Ctrl Pts',(0.468589071742487,-71.7143385748615,
-177.1453352109));
#185365=CARTESIAN_POINT('Ctrl Pts',(0.473063010586619,-71.715134304921,
-177.142193188744));
#185366=CARTESIAN_POINT('Ctrl Pts',(0.477498484508432,-71.7159593880345,
-177.138948316893));
#185367=CARTESIAN_POINT('Ctrl Pts',(0.481883829164943,-71.716811182357,
-177.135612221786));
#185368=CARTESIAN_POINT('Ctrl Pts',(0.485757118468243,-71.7175635168019,
-177.132665666269));
#185369=CARTESIAN_POINT('Ctrl Pts',(0.489837937730701,-71.7183834985899,
-177.129457083549));
#185370=CARTESIAN_POINT('Ctrl Pts',(0.493835191553745,-71.7192185065134,
-177.126200136524));
#185371=CARTESIAN_POINT('Ctrl Pts',(0.498075833628816,-71.7201043571225,
-177.122744877689));
#185372=CARTESIAN_POINT('Ctrl Pts',(0.502221922901849,-71.7210071255079,
-177.11923531805));
#185373=CARTESIAN_POINT('Ctrl Pts',(0.505950388940999,-71.7218478956593,
-177.115981351614));
#185374=CARTESIAN_POINT('Ctrl Pts',(0.507713663755773,-71.7222455146311,
-177.114442478253));
#185375=CARTESIAN_POINT('Ctrl Pts',(0.509383932591482,-71.7226290411988,
-177.112961523303));
#185376=CARTESIAN_POINT('Ctrl Pts',(0.510928956307166,-71.7229891444007,
-177.111574477354));
#185377=CARTESIAN_POINT('Ctrl Pts',(0.525744610702608,-71.7264422723574,
-177.098273714909));
#185378=CARTESIAN_POINT('Ctrl Pts',(0.540145094113651,-71.7302846063745,
-177.083683222483));
#185379=CARTESIAN_POINT('Ctrl Pts',(0.553845466478309,-71.7344794501829,
-177.068004345852));
#185380=CARTESIAN_POINT('Ctrl Pts',(0.5557948104403,-71.7350763093946,-177.065773492363));
#185381=CARTESIAN_POINT('Ctrl Pts',(0.557729972543417,-71.7356802828448,
-177.06352068727));
#185382=CARTESIAN_POINT('Ctrl Pts',(0.55965012674352,-71.7362912430783,
-177.061246589637));
#185383=CARTESIAN_POINT('Ctrl Pts',(0.572987316213086,-71.7405349087129,
-177.045450946246));
#185384=CARTESIAN_POINT('Ctrl Pts',(0.585704230882826,-71.7451282375326,
-177.028575967441));
#185385=CARTESIAN_POINT('Ctrl Pts',(0.597763139675443,-71.7500808478573,
-177.010630935905));
#185386=CARTESIAN_POINT('Ctrl Pts',(0.610239883661992,-71.7552050636673,
-176.992064117948));
#185387=CARTESIAN_POINT('Ctrl Pts',(0.621956874734709,-71.7606986066875,
-176.97242882321));
#185388=CARTESIAN_POINT('Ctrl Pts',(0.632911144964776,-71.7665625189615,
-176.951783782017));
#185389=CARTESIAN_POINT('Ctrl Pts',(0.633369156063166,-71.7668076961248,
-176.950920588231));
#185390=CARTESIAN_POINT('Ctrl Pts',(0.633825564774752,-71.7670534314148,
-176.950056147609));
#185391=CARTESIAN_POINT('Ctrl Pts',(0.634280373130207,-71.7672997213183,
-176.949190468659));
#185392=CARTESIAN_POINT('Ctrl Pts',(0.639946612355886,-71.7703681291322,
-176.938405389707));
#185393=CARTESIAN_POINT('Ctrl Pts',(0.645400236066963,-71.7735423162463,
-176.927359520256));
#185394=CARTESIAN_POINT('Ctrl Pts',(0.650639754836452,-71.7768027187209,
-176.916069509228));
#185395=CARTESIAN_POINT('Ctrl Pts',(0.653259514221201,-71.7784329199583,
-176.910424503714));
#185396=CARTESIAN_POINT('Ctrl Pts',(0.655825527594471,-71.7800854028515,
-176.904718297703));
#185397=CARTESIAN_POINT('Ctrl Pts',(0.658336622015916,-71.7817616184398,
-176.898952175483));
#185398=CARTESIAN_POINT('Ctrl Pts',(0.65982011992222,-71.7827518887755,
-176.895545680622));
#185399=CARTESIAN_POINT('Ctrl Pts',(0.661488202284415,-71.7838900418682,
-176.891639326401));
#185400=CARTESIAN_POINT('Ctrl Pts',(0.662976735295404,-71.7849296832095,
-176.888079828907));
#185401=CARTESIAN_POINT('Ctrl Pts',(0.664007819551247,-71.7856498270093,
-176.885614218942));
#185402=CARTESIAN_POINT('Ctrl Pts',(0.664953887829225,-71.7863222897559,
-176.883316006929));
#185403=CARTESIAN_POINT('Ctrl Pts',(0.665704692784938,-71.7868612729392,
-176.881475844081));
#185404=CARTESIAN_POINT('Ctrl Pts',(0.673043534861993,-71.7921296351606,
-176.863488929597));
#185405=CARTESIAN_POINT('Ctrl Pts',(0.679883034351907,-71.7976623272424,
-176.844889471199));
#185406=CARTESIAN_POINT('Ctrl Pts',(0.686226766441959,-71.8034367538504,
-176.825696233573));
#185407=CARTESIAN_POINT('Ctrl Pts',(0.697394959541523,-71.8136026799144,
-176.791906379121));
#185408=CARTESIAN_POINT('Ctrl Pts',(0.707022095169632,-71.8244891229403,
-176.756302654074));
#185409=CARTESIAN_POINT('Ctrl Pts',(0.715145536483142,-71.8360319850039,
-176.7189895102));
#185410=CARTESIAN_POINT('Ctrl Pts',(0.723451411044401,-71.8478340724048,
-176.680838401508));
#185411=CARTESIAN_POINT('Ctrl Pts',(0.730185480967119,-71.8603223275583,
-176.640900304655));
#185412=CARTESIAN_POINT('Ctrl Pts',(0.735428754255368,-71.873409659994,
-176.599320597914));
#185413=CARTESIAN_POINT('Ctrl Pts',(0.740933102500712,-71.8871486416127,
-176.555670539399));
#185414=CARTESIAN_POINT('Ctrl Pts',(0.744794629914615,-71.9015477772457,
-176.510211301259));
#185415=CARTESIAN_POINT('Ctrl Pts',(0.747149609679553,-71.9164869468611,
-176.463147664823));
#185416=CARTESIAN_POINT('Ctrl Pts',(0.749080992754893,-71.9287389669356,
-176.424549494159));
#185417=CARTESIAN_POINT('Ctrl Pts',(0.749999999999965,-71.9413537743572,
-176.384872959276));
#185418=CARTESIAN_POINT('Ctrl Pts',(0.749999999999965,-71.9542570083556,
-176.344247731786));
#185419=CARTESIAN_POINT('Origin',(0.,-12.9675000200281,-177.84995));
#185420=CARTESIAN_POINT('',(23.9949152542395,-66.3200448697526,-177.84995));
#185421=CARTESIAN_POINT('Origin',(24.200000000006,-66.7760495265862,-177.84995));
#185422=CARTESIAN_POINT('',(24.4906779661044,-66.0942982743985,-177.84995));
#185423=CARTESIAN_POINT('Origin',(0.,-12.9675000200281,-177.84995));
#185424=CARTESIAN_POINT('Origin',(24.7000000000027,-66.5483734731538,-177.84995));
#185425=CARTESIAN_POINT('Ctrl Pts',(25.166383622031,-65.7775666303703,-177.581785882201));
#185426=CARTESIAN_POINT('Ctrl Pts',(24.9516549782085,-65.8798945343463,
-177.298823774072));
#185427=CARTESIAN_POINT('Ctrl Pts',(25.0407404589729,-66.228934721057,-177.2158679411));
#185428=CARTESIAN_POINT('Ctrl Pts',(24.9795558812766,-65.8665984929838,
-177.757245548006));
#185429=CARTESIAN_POINT('Ctrl Pts',(24.8039770572177,-65.9493003143299,
-177.391803085524));
#185430=CARTESIAN_POINT('Ctrl Pts',(24.9465334973015,-66.3187224932389,
-177.303592864513));
#185431=CARTESIAN_POINT('Ctrl Pts',(24.7362442762044,-65.9810957924573,
-177.84994999494));
#185432=CARTESIAN_POINT('Ctrl Pts',(24.6278738771108,-66.0310529650264,
-177.399536111675));
#185433=CARTESIAN_POINT('Ctrl Pts',(24.8237985595108,-66.4342348178924,
-177.34995));
#185434=CARTESIAN_POINT('Ctrl Pts',(24.4906779661017,-66.0942982743997,
-177.84995));
#185435=CARTESIAN_POINT('Ctrl Pts',(24.4906779661017,-66.0942982743998,
-177.34995));
#185436=CARTESIAN_POINT('Ctrl Pts',(24.7,-66.548373473155,-177.34995));
#185437=CARTESIAN_POINT('Ctrl Pts',(25.166383622031,-65.7775666303703,-177.581785882201));
#185438=CARTESIAN_POINT('Ctrl Pts',(25.1415920409418,-65.7893809392764,
-177.605068947741));
#185439=CARTESIAN_POINT('Ctrl Pts',(25.1158854587622,-65.8016057771408,
-177.626825178572));
#185440=CARTESIAN_POINT('Ctrl Pts',(25.0893171817991,-65.8142137722865,
-177.64711393097));
#185441=CARTESIAN_POINT('Ctrl Pts',(25.067740038687,-65.8244532212351,-177.663591225101));
#185442=CARTESIAN_POINT('Ctrl Pts',(25.0455930316585,-65.8349461067523,
-177.67910099763));
#185443=CARTESIAN_POINT('Ctrl Pts',(25.0228835124146,-65.845687478185,-177.693662139191));
#185444=CARTESIAN_POINT('Ctrl Pts',(25.0179522289245,-65.8480199250782,
-177.696824034263));
#185445=CARTESIAN_POINT('Ctrl Pts',(25.0129943890564,-65.8503641038013,
-177.699941201796));
#185446=CARTESIAN_POINT('Ctrl Pts',(25.008000291213,-65.8527245791014,-177.703019463535));
#185447=CARTESIAN_POINT('Ctrl Pts',(24.9863105885612,-65.8629762820078,
-177.7163885612));
#185448=CARTESIAN_POINT('Ctrl Pts',(24.9639883366338,-65.8735110172848,
-177.728985587561));
#185449=CARTESIAN_POINT('Ctrl Pts',(24.9412183470617,-65.8842397535242,
-177.740690014451));
#185450=CARTESIAN_POINT('Ctrl Pts',(24.9235937056763,-65.8925441108073,
-177.749749584984));
#185451=CARTESIAN_POINT('Ctrl Pts',(24.9057018486688,-65.9009642216675,
-177.758274996804));
#185452=CARTESIAN_POINT('Ctrl Pts',(24.8876387414352,-65.9094542954476,
-177.766228663939));
#185453=CARTESIAN_POINT('Ctrl Pts',(24.8749962615991,-65.9153965502981,
-177.77179548448));
#185454=CARTESIAN_POINT('Ctrl Pts',(24.8622705967981,-65.9213727527722,
-177.777082364443));
#185455=CARTESIAN_POINT('Ctrl Pts',(24.8494947047088,-65.9273672725666,
-177.782082032575));
#185456=CARTESIAN_POINT('Ctrl Pts',(24.8190218618827,-65.9416653003081,
-177.794007156872));
#185457=CARTESIAN_POINT('Ctrl Pts',(24.788219590087,-65.9560881393781,-177.804322161695));
#185458=CARTESIAN_POINT('Ctrl Pts',(24.7570997784996,-65.9706278171961,
-177.813083012314));
#185459=CARTESIAN_POINT('Ctrl Pts',(24.7258330121357,-65.9852361546556,
-177.821885233647));
#185460=CARTESIAN_POINT('Ctrl Pts',(24.6942450261371,-65.9999627695759,
-177.829118717227));
#185461=CARTESIAN_POINT('Ctrl Pts',(24.6623322245521,-66.0148059325099,
-177.834790172697));
#185462=CARTESIAN_POINT('Ctrl Pts',(24.6308159404476,-66.029464668716,-177.840391160168));
#185463=CARTESIAN_POINT('Ctrl Pts',(24.5989822036623,-66.0442373978369,
-177.844468742953));
#185464=CARTESIAN_POINT('Ctrl Pts',(24.5668222618469,-66.0591237512874,
-177.846979582025));
#185465=CARTESIAN_POINT('Ctrl Pts',(24.5416418773983,-66.0707793725903,
-177.848945502656));
#185466=CARTESIAN_POINT('Ctrl Pts',(24.5162613043884,-66.0825047291482,
-177.849949999473));
#185467=CARTESIAN_POINT('Ctrl Pts',(24.4906779661043,-66.0942982743985,
-177.84995));
#185468=CARTESIAN_POINT('Origin',(26.4569673975197,-68.4857751744904,-179.64995));
#185469=CARTESIAN_POINT('',(25.166383622031,-65.7775666303703,-179.39995));
#185470=CARTESIAN_POINT('',(25.166383622031,-65.7775666303703,-179.64995));
#185471=CARTESIAN_POINT('Origin',(26.4569673975197,-68.4857751744904,-179.39995));
#185472=CARTESIAN_POINT('Ctrl Pts',(1.23783545400211,-71.4544141842476,
-176.238260704663));
#185473=CARTESIAN_POINT('Ctrl Pts',(0.721132232531162,-71.4643985224633,
-176.261250303005));
#185474=CARTESIAN_POINT('Ctrl Pts',(0.748751140187461,-71.9810613292915,
-176.259802934377));
#185475=CARTESIAN_POINT('Ctrl Pts',(1.25321977150542,-71.4540136938127,
-176.572353761973));
#185476=CARTESIAN_POINT('Ctrl Pts',(0.81377284711986,-71.4627451452814,
-176.500715567558));
#185477=CARTESIAN_POINT('Ctrl Pts',(0.756542354171283,-71.895138681302,
-176.530753994678));
#185478=CARTESIAN_POINT('Ctrl Pts',(1.19860343374803,-71.4555315991133,
-176.926629115674));
#185479=CARTESIAN_POINT('Ctrl Pts',(0.841287188135883,-71.4620507681087,
-176.792597259361));
#185480=CARTESIAN_POINT('Ctrl Pts',(0.729058399664653,-71.8180309468073,
-176.770579193097));
#185481=CARTESIAN_POINT('Ctrl Pts',(0.965096742606605,-71.4595547413853,
-177.27331690312));
#185482=CARTESIAN_POINT('Ctrl Pts',(0.713294749850913,-71.4632595324917,
-177.074901556755));
#185483=CARTESIAN_POINT('Ctrl Pts',(0.611402945447152,-71.7550490002612,
-176.992319359077));
#185484=CARTESIAN_POINT('Ctrl Pts',(0.916779319039344,-71.4603417028127,
-177.331361977737));
#185485=CARTESIAN_POINT('Ctrl Pts',(0.685390263968729,-71.4635316607953,
-177.121001585987));
#185486=CARTESIAN_POINT('Ctrl Pts',(0.587057849709363,-71.7450124422729,
-177.02878681156));
#185487=CARTESIAN_POINT('Ctrl Pts',(0.807976114834587,-71.4619457720088,
-177.435774845394));
#185488=CARTESIAN_POINT('Ctrl Pts',(0.61920619489495,-71.4641477944332,
-177.203686314583));
#185489=CARTESIAN_POINT('Ctrl Pts',(0.532234779142866,-71.7275925135231,
-177.093698009026));
#185490=CARTESIAN_POINT('Ctrl Pts',(0.746606781238387,-71.4627719946713,
-177.482505016316));
#185491=CARTESIAN_POINT('Ctrl Pts',(0.580314974840451,-71.4644967134863,
-177.240847062286));
#185492=CARTESIAN_POINT('Ctrl Pts',(0.501311469386272,-71.7201585461063,
-177.122354454569));
#185493=CARTESIAN_POINT('Ctrl Pts',(0.521249492735721,-71.4653981046342,
-177.613426214874));
#185494=CARTESIAN_POINT('Ctrl Pts',(0.434920719988867,-71.4656764551474,
-177.343994523926));
#185495=CARTESIAN_POINT('Ctrl Pts',(0.387756225423206,-71.6999617297923,
-177.202103665492));
#185496=CARTESIAN_POINT('Ctrl Pts',(0.330983066508931,-71.4669014486956,
-177.656473197042));
#185497=CARTESIAN_POINT('Ctrl Pts',(0.304420776205656,-71.4665113043489,
-177.379037765856));
#185498=CARTESIAN_POINT('Ctrl Pts',(0.291876596246233,-71.6944798744154,
-177.227398366312));
#185499=CARTESIAN_POINT('Ctrl Pts',(0.141805636875531,-71.4673186419509,
-177.630934590095));
#185500=CARTESIAN_POINT('Ctrl Pts',(0.176963829132147,-71.4669036380682,
-177.358245566005));
#185501=CARTESIAN_POINT('Ctrl Pts',(0.196547809098401,-71.698807761693,
-177.212077768614));
#185502=CARTESIAN_POINT('',(0.249751305446096,-71.4669668918333,-177.637584354353));
#185503=CARTESIAN_POINT('Origin',(0.25188593198836,-71.966962335182,-177.637584354353));
#185504=CARTESIAN_POINT('',(1.23940677966098,-71.4543692372681,-176.344247731786));
#185505=CARTESIAN_POINT('Ctrl Pts',(1.23940677966098,-71.4543692372681,
-176.344247731786));
#185506=CARTESIAN_POINT('Ctrl Pts',(1.23940677966098,-71.4543692372681,
-176.517170194872));
#185507=CARTESIAN_POINT('Ctrl Pts',(1.22017060769392,-71.4547863693157,
-176.675572408682));
#185508=CARTESIAN_POINT('Ctrl Pts',(1.1624603379848,-71.4559523518045,-176.891395355483));
#185509=CARTESIAN_POINT('Ctrl Pts',(1.12639114428662,-71.4566677449925,
-176.993861735405));
#185510=CARTESIAN_POINT('Ctrl Pts',(1.07168494602295,-71.4576871945188,
-177.103876931726));
#185511=CARTESIAN_POINT('Ctrl Pts',(1.04117534582081,-71.4582351623851,
-177.156502301489));
#185512=CARTESIAN_POINT('Ctrl Pts',(1.02742339564269,-71.4584772975563,
-177.178545553874));
#185513=CARTESIAN_POINT('Ctrl Pts',(1.01810511453015,-71.4586402353632,
-177.193127616017));
#185514=CARTESIAN_POINT('Ctrl Pts',(1.01411410582161,-71.4587096452574,
-177.199252649036));
#185515=CARTESIAN_POINT('Ctrl Pts',(0.964139403507473,-71.4595713554461,
-177.273834478609));
#185516=CARTESIAN_POINT('Ctrl Pts',(0.890131256064229,-71.4607724720151,
-177.362452390043));
#185517=CARTESIAN_POINT('Ctrl Pts',(0.805059306817399,-71.4619677502115,
-177.434833509482));
#185518=CARTESIAN_POINT('Ctrl Pts',(0.745885964242655,-71.4627522175639,
-177.479479413109));
#185519=CARTESIAN_POINT('Ctrl Pts',(0.716981135486837,-71.463116020377,
-177.498882122092));
#185520=CARTESIAN_POINT('Ctrl Pts',(0.547198059716821,-71.4650984803593,
-177.598036775321));
#185521=CARTESIAN_POINT('Ctrl Pts',(0.40277284172198,-71.4663135982139,
-177.637660542527));
#185522=CARTESIAN_POINT('Ctrl Pts',(0.249751305446096,-71.4669668918333,
-177.637584354353));
#185523=CARTESIAN_POINT('Origin',(1.24999999999996,-71.9542570083556,-176.344247731786));
#185524=CARTESIAN_POINT('Origin',(1.24999999999996,-71.9542570083556,-179.64995));
#185525=CARTESIAN_POINT('',(1.23940677966098,-71.4543692372681,-179.64995));
#185526=CARTESIAN_POINT('Origin',(0.,-12.9675000200281,-171.871644662643));
#185527=CARTESIAN_POINT('Origin',(0.,-12.9675000200281,-171.871644662643));
#185528=CARTESIAN_POINT('Origin',(6.9,-71.5626363369615,-179.64995));
#185529=CARTESIAN_POINT('',(6.84152542372878,-71.066067385123,-176.485569595297));
#185530=CARTESIAN_POINT('Origin',(6.9,-71.5626363369615,-176.485569595297));
#185531=CARTESIAN_POINT('',(6.84152542372878,-71.066067385123,-179.64995));
#185532=CARTESIAN_POINT('Ctrl Pts',(7.86991817520074,-70.935718794764,-177.700825662764));
#185533=CARTESIAN_POINT('Ctrl Pts',(7.87530650495354,-70.9349872609141,
-177.368681451895));
#185534=CARTESIAN_POINT('Ctrl Pts',(7.91859121655422,-71.2381488509314,
-177.239961484007));
#185535=CARTESIAN_POINT('Ctrl Pts',(7.72465595207765,-70.9554399770617,
-177.698405110518));
#185536=CARTESIAN_POINT('Ctrl Pts',(7.7814869526158,-70.9477382671599,-177.362180852783));
#185537=CARTESIAN_POINT('Ctrl Pts',(7.84535391894273,-71.2544423085659,
-177.236091643156));
#185538=CARTESIAN_POINT('Ctrl Pts',(7.57909439591914,-70.9746058127342,
-177.660005031717));
#185539=CARTESIAN_POINT('Ctrl Pts',(7.68873678647519,-70.9601668953933,
-177.328725158091));
#185540=CARTESIAN_POINT('Ctrl Pts',(7.77193648886645,-71.274739088698,-177.212399058377));
#185541=CARTESIAN_POINT('Ctrl Pts',(7.32049271153216,-71.0078082615326,
-177.524965998388));
#185542=CARTESIAN_POINT('Ctrl Pts',(7.53187921075035,-70.98103712284,-177.221702886533));
#185543=CARTESIAN_POINT('Ctrl Pts',(7.64153051403658,-71.3201342851139,
-177.131947985374));
#185544=CARTESIAN_POINT('Ctrl Pts',(7.20559474882705,-71.0221114770482,
-177.427818678983));
#185545=CARTESIAN_POINT('Ctrl Pts',(7.46634030528468,-70.9896817811965,
-177.14630380948));
#185546=CARTESIAN_POINT('Ctrl Pts',(7.58359051438092,-71.3455846992379,
-177.074841178091));
#185547=CARTESIAN_POINT('Ctrl Pts',(7.0224958330043,-71.0445441888331,-177.19789774704));
#185548=CARTESIAN_POINT('Ctrl Pts',(7.3754100247025,-71.0018071186815,-176.974926941462));
#185549=CARTESIAN_POINT('Ctrl Pts',(7.49125858243999,-71.4004398176271,
-176.937641167035));
#185550=CARTESIAN_POINT('Ctrl Pts',(6.95330228061017,-71.0528136932555,
-177.064676392973));
#185551=CARTESIAN_POINT('Ctrl Pts',(7.35016748493995,-71.0052818262832,
-176.876651794266));
#185552=CARTESIAN_POINT('Ctrl Pts',(7.45636610731683,-71.4300660132009,
-176.85726439743));
#185553=CARTESIAN_POINT('Ctrl Pts',(6.86278910799687,-71.0635773642165,
-176.782076502575));
#185554=CARTESIAN_POINT('Ctrl Pts',(7.34226626007839,-71.0069144630253,
-176.677678014477));
#185555=CARTESIAN_POINT('Ctrl Pts',(7.41072271257901,-71.4935573295699,
-176.680998879949));
#185556=CARTESIAN_POINT('Ctrl Pts',(6.8415254209523,-71.06606738545,-176.633819401763));
#185557=CARTESIAN_POINT('Ctrl Pts',(7.36167840976143,-71.0048156182874,
-176.575906600101));
#185558=CARTESIAN_POINT('Ctrl Pts',(7.4,-71.5272255526701,-176.585813210379));
#185559=CARTESIAN_POINT('Ctrl Pts',(6.84152542372878,-71.066067385123,-176.485569595297));
#185560=CARTESIAN_POINT('Ctrl Pts',(7.40000000000002,-71.0003029749946,
-176.485569595297));
#185561=CARTESIAN_POINT('Ctrl Pts',(7.4,-71.5626363369615,-176.485569595297));
#185562=CARTESIAN_POINT('',(7.86991817520075,-70.935718794764,-177.700825662763));
#185563=CARTESIAN_POINT('Origin',(7.93718243310846,-71.4311736560866,-177.700825662763));
#185564=CARTESIAN_POINT('Ctrl Pts',(7.86991817520075,-70.935718794764,-177.700825662763));
#185565=CARTESIAN_POINT('Ctrl Pts',(7.84145915028903,-70.9395824669992,
-177.700351440663));
#185566=CARTESIAN_POINT('Ctrl Pts',(7.81325306985417,-70.9433890026599,
-177.698505055736));
#185567=CARTESIAN_POINT('Ctrl Pts',(7.78529419147432,-70.9471417642783,
-177.695385832037));
#185568=CARTESIAN_POINT('Ctrl Pts',(7.7769616359882,-70.9482601959259,-177.694456213038));
#185569=CARTESIAN_POINT('Ctrl Pts',(7.76865098308067,-70.9493738524319,
-177.693413186647));
#185570=CARTESIAN_POINT('Ctrl Pts',(7.76036198762536,-70.9504828203398,
-177.692258509338));
#185571=CARTESIAN_POINT('Ctrl Pts',(7.7317172038824,-70.9543151479204,-177.688268221013));
#185572=CARTESIAN_POINT('Ctrl Pts',(7.7033289936208,-70.9580918229642,-177.682948350417));
#185573=CARTESIAN_POINT('Ctrl Pts',(7.675186105217,-70.9618160028387,-177.676335993945));
#185574=CARTESIAN_POINT('Ctrl Pts',(7.66343218081142,-70.9633714127913,
-177.673574332207));
#185575=CARTESIAN_POINT('Ctrl Pts',(7.65172493394877,-70.964917145146,-177.670587723933));
#185576=CARTESIAN_POINT('Ctrl Pts',(7.64004659107783,-70.9664556187766,
-177.667371199649));
#185577=CARTESIAN_POINT('Ctrl Pts',(7.60920468562832,-70.9705186488466,
-177.65887652374));
#185578=CARTESIAN_POINT('Ctrl Pts',(7.57859346491502,-70.9745271017102,
-177.648778373647));
#185579=CARTESIAN_POINT('Ctrl Pts',(7.54854310099584,-70.9784389453262,
-177.637166030246));
#185580=CARTESIAN_POINT('Ctrl Pts',(7.52067144326505,-70.9820671731458,
-177.626395602919));
#185581=CARTESIAN_POINT('Ctrl Pts',(7.49328227206074,-70.9856123005526,
-177.614321694518));
#185582=CARTESIAN_POINT('Ctrl Pts',(7.46663887751155,-70.9890415496572,
-177.601070367657));
#185583=CARTESIAN_POINT('Ctrl Pts',(7.46098971645219,-70.9897686484685,
-177.598260707666));
#185584=CARTESIAN_POINT('Ctrl Pts',(7.45537399181972,-70.9904905521545,
-177.595398277761));
#185585=CARTESIAN_POINT('Ctrl Pts',(7.44979405295273,-70.9912069730377,
-177.59248453496));
#185586=CARTESIAN_POINT('Ctrl Pts',(7.44926963945517,-70.9912743036645,
-177.59221069575));
#185587=CARTESIAN_POINT('Ctrl Pts',(7.44874551143164,-70.9913415902563,
-177.591936395013));
#185588=CARTESIAN_POINT('Ctrl Pts',(7.44822167031192,-70.9914088326578,
-177.591661634332));
#185589=CARTESIAN_POINT('Ctrl Pts',(7.36341668565129,-71.0022947494199,
-177.547180446295));
#185590=CARTESIAN_POINT('Ctrl Pts',(7.28492054201756,-71.0121779828271,
-177.489997024811));
#185591=CARTESIAN_POINT('Ctrl Pts',(7.21521421994463,-71.0208423096966,
-177.423514614651));
#185592=CARTESIAN_POINT('Ctrl Pts',(7.17900585541714,-71.0253429216403,
-177.388980884135));
#185593=CARTESIAN_POINT('Ctrl Pts',(7.14516858273338,-71.0295147031061,
-177.35193750338));
#185594=CARTESIAN_POINT('Ctrl Pts',(7.11404633506787,-71.0333277050162,
-177.3128573618));
#185595=CARTESIAN_POINT('Ctrl Pts',(7.11356074608127,-71.033387197883,-177.312247608721));
#185596=CARTESIAN_POINT('Ctrl Pts',(7.11307579006788,-71.0334466073515,
-177.311637347152));
#185597=CARTESIAN_POINT('Ctrl Pts',(7.11259146723154,-71.0335059334348,
-177.311026578643));
#185598=CARTESIAN_POINT('Ctrl Pts',(7.05806005587485,-71.0401856412932,
-177.242258256468));
#185599=CARTESIAN_POINT('Ctrl Pts',(7.01156780675731,-71.0458068303084,
-177.167083119785));
#185600=CARTESIAN_POINT('Ctrl Pts',(6.97337953735775,-71.0503909874143,
-177.087652956309));
#185601=CARTESIAN_POINT('Ctrl Pts',(6.94786514373312,-71.0534537601107,
-177.034583977576));
#185602=CARTESIAN_POINT('Ctrl Pts',(6.92605814997056,-71.0560535184279,
-176.979614410751));
#185603=CARTESIAN_POINT('Ctrl Pts',(6.90804579110999,-71.058195517224,-176.923376416061));
#185604=CARTESIAN_POINT('Ctrl Pts',(6.90788807893848,-71.0582142720847,
-176.922884008801));
#185605=CARTESIAN_POINT('Ctrl Pts',(6.90773065840123,-71.0582329917957,
-176.922391517884));
#185606=CARTESIAN_POINT('Ctrl Pts',(6.90757352937676,-71.0582516763749,
-176.921898943596));
#185607=CARTESIAN_POINT('Ctrl Pts',(6.89200677785444,-71.0601027551398,
-176.873099674503));
#185608=CARTESIAN_POINT('Ctrl Pts',(6.87933106860591,-71.0616054747707,
-176.82359063585));
#185609=CARTESIAN_POINT('Ctrl Pts',(6.86938539001924,-71.0627821611452,
-176.773553029938));
#185610=CARTESIAN_POINT('Ctrl Pts',(6.85903549341787,-71.0640066710871,
-176.72148176674));
#185611=CARTESIAN_POINT('Ctrl Pts',(6.85164206564097,-71.0648780949575,
-176.668837206011));
#185612=CARTESIAN_POINT('Ctrl Pts',(6.84707944646843,-71.065414925157,-176.615812182358));
#185613=CARTESIAN_POINT('Ctrl Pts',(6.84336254226504,-71.0658522499368,
-176.572615736228));
#185614=CARTESIAN_POINT('Ctrl Pts',(6.84152542372878,-71.066067385123,-176.529166339213));
#185615=CARTESIAN_POINT('Ctrl Pts',(6.84152542372878,-71.066067385123,-176.485569595297));
#185616=CARTESIAN_POINT('Ctrl Pts',(7.91859121655416,-71.2381488509313,
-177.239961484006));
#185617=CARTESIAN_POINT('Ctrl Pts',(7.87530650495358,-70.9349872609141,
-177.368681451894));
#185618=CARTESIAN_POINT('Ctrl Pts',(7.86991817520098,-70.935718794764,-177.700825662763));
#185619=CARTESIAN_POINT('Ctrl Pts',(8.08517348178868,-71.21877443556,-177.241356202481));
#185620=CARTESIAN_POINT('Ctrl Pts',(8.04094447940713,-70.9124841487064,
-177.368907517599));
#185621=CARTESIAN_POINT('Ctrl Pts',(8.03499989482399,-70.9133068653807,
-177.703576433696));
#185622=CARTESIAN_POINT('Ctrl Pts',(8.25170137526425,-71.1987909763519,
-177.242846915875));
#185623=CARTESIAN_POINT('Ctrl Pts',(8.20613182703653,-70.889318969813,-177.369144269326));
#185624=CARTESIAN_POINT('Ctrl Pts',(8.19998119128136,-70.8901904062617,
-177.706427680957));
#185625=CARTESIAN_POINT('Ctrl Pts',(8.41817827172741,-71.1781985203567,
-177.244444626904));
#185626=CARTESIAN_POINT('Ctrl Pts',(8.3707824215504,-70.8655141261623,-177.369392503912));
#185627=CARTESIAN_POINT('Ctrl Pts',(8.36486199647703,-70.866369471684,-177.709383806605));
#185628=CARTESIAN_POINT('',(8.36486199647649,-70.8663694716841,-177.709383806605));
#185629=CARTESIAN_POINT('Origin',(0.0230368111365542,-14.1525797472871,
-185.975887612657));
#185630=CARTESIAN_POINT('Origin',(8.43635654345535,-71.3612316037495,-177.709383806605));
#185631=CARTESIAN_POINT('Ctrl Pts',(9.31194471985222,-70.7216281469411,
-176.521703250262));
#185632=CARTESIAN_POINT('Ctrl Pts',(8.86316466557432,-70.7927544609078,
-176.577904846168));
#185633=CARTESIAN_POINT('Ctrl Pts',(8.89511833477312,-71.2491795873182,
-176.583278767617));
#185634=CARTESIAN_POINT('Ctrl Pts',(9.33426782231391,-70.7179921647292,
-176.707671693767));
#185635=CARTESIAN_POINT('Ctrl Pts',(8.91524414222188,-70.7846676236483,
-176.691761787883));
#185636=CARTESIAN_POINT('Ctrl Pts',(8.90639454875205,-71.2042306696945,
-176.699592289102));
#185637=CARTESIAN_POINT('Ctrl Pts',(9.31861749655483,-70.7205733106781,
-176.894655311153));
#185638=CARTESIAN_POINT('Ctrl Pts',(8.93334931956903,-70.7817419161099,
-176.820727622377));
#185639=CARTESIAN_POINT('Ctrl Pts',(8.8985376639078,-71.1725272604627,-176.808271319893));
#185640=CARTESIAN_POINT('Ctrl Pts',(9.21240345628522,-70.7375942109218,
-177.194427742108));
#185641=CARTESIAN_POINT('Ctrl Pts',(8.89508753920652,-70.7873478881673,
-177.027386013335));
#185642=CARTESIAN_POINT('Ctrl Pts',(8.84506581279844,-71.1392355158483,
-176.976329963003));
#185643=CARTESIAN_POINT('Ctrl Pts',(9.14614340920233,-70.7481724076873,
-177.308522414764));
#185644=CARTESIAN_POINT('Ctrl Pts',(8.86032021978074,-70.7925702591893,
-177.107065661507));
#185645=CARTESIAN_POINT('Ctrl Pts',(8.81169873029936,-71.1320753660863,
-177.038360991276));
#185646=CARTESIAN_POINT('Ctrl Pts',(8.84766881369401,-70.7949534600523,
-177.640884592286));
#185647=CARTESIAN_POINT('Ctrl Pts',(8.68613018229932,-70.8186420493741,
-177.333034085865));
#185648=CARTESIAN_POINT('Ctrl Pts',(8.66138036999789,-71.1267167292917,
-177.215887692752));
#185649=CARTESIAN_POINT('Ctrl Pts',(8.52372344713472,-70.8442550810108,
-177.757261114079));
#185650=CARTESIAN_POINT('Ctrl Pts',(8.4669598281481,-70.8511504969647,-177.410277645602));
#185651=CARTESIAN_POINT('Ctrl Pts',(8.49812639039677,-71.1551635236587,
-177.272472653023));
#185652=CARTESIAN_POINT('Ctrl Pts',(8.2060354143041,-70.8890492358094,-177.693193871778));
#185653=CARTESIAN_POINT('Ctrl Pts',(8.27002543687626,-70.8792234239869,
-177.351033919866));
#185654=CARTESIAN_POINT('Ctrl Pts',(8.33823067532437,-71.1985789270941,
-177.232285602531));
#185655=CARTESIAN_POINT('',(9.32033898305081,-70.7202599648223,-176.681036188741));
#185656=CARTESIAN_POINT('Ctrl Pts',(9.32033898305081,-70.7202599648223,
-176.681036188741));
#185657=CARTESIAN_POINT('Ctrl Pts',(9.3203389830508,-70.7202599648223,-176.749135893056));
#185658=CARTESIAN_POINT('Ctrl Pts',(9.31498446872546,-70.7211248588454,
-176.815409677274));
#185659=CARTESIAN_POINT('Ctrl Pts',(9.30427471976772,-70.7228501785986,
-176.879857541395));
#185660=CARTESIAN_POINT('Ctrl Pts',(9.29891984528884,-70.7237128384752,
-176.912081473456));
#185661=CARTESIAN_POINT('Ctrl Pts',(9.29222613967396,-70.7247904651451,
-176.943848925492));
#185662=CARTESIAN_POINT('Ctrl Pts',(9.28419337855619,-70.7260816621493,
-176.975159897504));
#185663=CARTESIAN_POINT('Ctrl Pts',(9.27616061743841,-70.7273728591534,
-177.006470869516));
#185664=CARTESIAN_POINT('Ctrl Pts',(9.26728977127031,-70.7287973499507,
-177.035903622681));
#185665=CARTESIAN_POINT('Ctrl Pts',(9.25607761587008,-70.7305940089151,
-177.067723373468));
#185666=CARTESIAN_POINT('Ctrl Pts',(9.23365330506961,-70.7341873268439,
-177.131362875041));
#185667=CARTESIAN_POINT('Ctrl Pts',(9.20602077392941,-70.7386025493298,
-177.191198784361));
#185668=CARTESIAN_POINT('Ctrl Pts',(9.17317647543608,-70.74381725599,-177.247231101426));
#185669=CARTESIAN_POINT('Ctrl Pts',(9.14033217694275,-70.7490319626502,
-177.303263418491));
#185670=CARTESIAN_POINT('Ctrl Pts',(9.10348192879145,-70.7548571469264,
-177.354142742939));
#185671=CARTESIAN_POINT('Ctrl Pts',(9.05900346753984,-70.7618289474852,
-177.403917275858));
#185672=CARTESIAN_POINT('Ctrl Pts',(8.98900499154369,-70.7728008966113,
-177.48225050389));
#185673=CARTESIAN_POINT('Ctrl Pts',(8.90992354066234,-70.7850704087956,
-177.545955215629));
#185674=CARTESIAN_POINT('Ctrl Pts',(8.82049689367651,-70.7987098858838,
-177.595581650182));
#185675=CARTESIAN_POINT('Ctrl Pts',(8.79627650488861,-70.802404013407,-177.609022515736));
#185676=CARTESIAN_POINT('Ctrl Pts',(8.77129720830665,-70.8061983474297,
-177.621430672585));
#185677=CARTESIAN_POINT('Ctrl Pts',(8.74553383831428,-70.810093650353,-177.632817052588));
#185678=CARTESIAN_POINT('Ctrl Pts',(8.6246468180102,-70.8283712112355,-177.686244284778));
#185679=CARTESIAN_POINT('Ctrl Pts',(8.49776106948925,-70.8471690552384,
-177.711766536117));
#185680=CARTESIAN_POINT('Ctrl Pts',(8.36486199647649,-70.8663694716841,
-177.709383806605));
#185681=CARTESIAN_POINT('Origin',(9.4,-71.2138732976838,-176.681036188741));
#185682=CARTESIAN_POINT('Origin',(9.4,-71.2138732976838,-179.64995));
#185683=CARTESIAN_POINT('',(9.32033898305081,-70.7202599648223,-179.64995));
#185684=CARTESIAN_POINT('Origin',(0.,-12.9675000200281,-171.871644662643));
#185685=CARTESIAN_POINT('Origin',(0.,-12.9675000200281,-171.871644662643));
#185686=CARTESIAN_POINT('Origin',(15.05,-70.015703322148,-179.64995));
#185687=CARTESIAN_POINT('',(14.9224576271186,-69.53224397213,-176.84995));
#185688=CARTESIAN_POINT('Origin',(15.05,-70.015703322148,-176.84995));
#185689=CARTESIAN_POINT('',(14.9224576271186,-69.5322439721301,-179.64995));
#185690=CARTESIAN_POINT('Ctrl Pts',(16.0658981859834,-69.2181101857427,
-177.83843816103));
#185691=CARTESIAN_POINT('Ctrl Pts',(16.0005358602646,-69.2358256555765,
-177.36456142736));
#185692=CARTESIAN_POINT('Ctrl Pts',(16.1265631343295,-69.6989087749272,
-177.34368264398));
#185693=CARTESIAN_POINT('Ctrl Pts',(15.7646054310406,-69.3044096982964,
-177.889038147364));
#185694=CARTESIAN_POINT('Ctrl Pts',(15.8105690999498,-69.289401681716,-177.348580470172));
#185695=CARTESIAN_POINT('Ctrl Pts',(15.9746754260325,-69.785917294809,-177.368934418229));
#185696=CARTESIAN_POINT('Ctrl Pts',(15.4414114400423,-69.3932567531528,
-177.784709035369));
#185697=CARTESIAN_POINT('Ctrl Pts',(15.682807240394,-69.3252572316702,-177.238537996438));
#185698=CARTESIAN_POINT('Ctrl Pts',(15.8119354596535,-69.8753938355129,
-177.316789718218));
#185699=CARTESIAN_POINT('Ctrl Pts',(14.9965996919493,-69.5131029391016,
-177.344861768588));
#185700=CARTESIAN_POINT('Ctrl Pts',(15.549956079405,-69.3641921133352,-177.008091533137));
#185701=CARTESIAN_POINT('Ctrl Pts',(15.5879032634866,-69.9961227595722,
-177.097095005978));
#185702=CARTESIAN_POINT('Ctrl Pts',(14.879290383782,-69.5434999409872,-177.013244119206));
#185703=CARTESIAN_POINT('Ctrl Pts',(15.547119708319,-69.3663509905523,-176.898252015644));
#185704=CARTESIAN_POINT('Ctrl Pts',(15.5288419201426,-70.0267333379905,
-176.931492946677));
#185705=CARTESIAN_POINT('Ctrl Pts',(14.935107290865,-69.5289450233885,-176.686865358248));
#185706=CARTESIAN_POINT('Ctrl Pts',(15.5511428301757,-69.3646343509962,
-176.799766495381));
#185707=CARTESIAN_POINT('Ctrl Pts',(15.5569471014035,-70.0120745403484,
-176.768510892379));
#185708=CARTESIAN_POINT('',(15.9139830508475,-69.2613286645371,-177.84995));
#185709=CARTESIAN_POINT('Origin',(16.0500000000002,-69.7424724991055,-177.84995));
#185710=CARTESIAN_POINT('Ctrl Pts',(15.9139830508475,-69.2613286645371,
-177.84995));
#185711=CARTESIAN_POINT('Ctrl Pts',(15.7965712698714,-69.2945203862127,
-177.84995));
#185712=CARTESIAN_POINT('Ctrl Pts',(15.6837640763244,-69.3260183464345,
-177.829973206133));
#185713=CARTESIAN_POINT('Ctrl Pts',(15.5736771291949,-69.3564225197141,
-177.789235002346));
#185714=CARTESIAN_POINT('Ctrl Pts',(15.5622378038961,-69.3595818700064,
-177.78500182505));
#185715=CARTESIAN_POINT('Ctrl Pts',(15.5508278378011,-69.3627293657972,
-177.780544473358));
#185716=CARTESIAN_POINT('Ctrl Pts',(15.5394451078152,-69.3658656500816,
-177.77586206693));
#185717=CARTESIAN_POINT('Ctrl Pts',(15.4185200786613,-69.3991841307096,
-177.726118276597));
#185718=CARTESIAN_POINT('Ctrl Pts',(15.3111353387459,-69.4283571390207,
-177.654683080351));
#185719=CARTESIAN_POINT('Ctrl Pts',(15.2182598314156,-69.453379385614,-177.562452499716));
#185720=CARTESIAN_POINT('Ctrl Pts',(15.14774018584,-69.4723785815483,-177.492422541931));
#185721=CARTESIAN_POINT('Ctrl Pts',(15.0892668418245,-69.4879953157288,
-177.413800201241));
#185722=CARTESIAN_POINT('Ctrl Pts',(15.0422976393026,-69.5004928802211,
-177.325216521744));
#185723=CARTESIAN_POINT('Ctrl Pts',(15.0274076467375,-69.5044548091529,
-177.297134070728));
#185724=CARTESIAN_POINT('Ctrl Pts',(15.0136737030358,-69.5081028798345,
-177.268050513167));
#185725=CARTESIAN_POINT('Ctrl Pts',(15.0010782474499,-69.5114444474722,
-177.237922234316));
#185726=CARTESIAN_POINT('Ctrl Pts',(14.9647660441677,-69.5210780556028,
-177.151063590839));
#185727=CARTESIAN_POINT('Ctrl Pts',(14.9410265060011,-69.5273431954927,
-177.062202234145));
#185728=CARTESIAN_POINT('Ctrl Pts',(14.9298722292227,-69.5302873914005,
-176.971338164234));
#185729=CARTESIAN_POINT('Ctrl Pts',(14.9249529310265,-69.5315858509875,
-176.931264974005));
#185730=CARTESIAN_POINT('Ctrl Pts',(14.9224813123119,-69.5322377236921,
-176.890802252594));
#185731=CARTESIAN_POINT('Ctrl Pts',(14.9224576271186,-69.53224397213,-176.84995));
#185732=CARTESIAN_POINT('Origin',(0.,-12.9675000200281,-177.84995));
#185733=CARTESIAN_POINT('',(16.4097457627119,-69.1188156235219,-177.84995));
#185734=CARTESIAN_POINT('Origin',(0.,-12.9675000200281,-177.84995));
#185735=CARTESIAN_POINT('Origin',(16.55,-69.5987413979107,-177.84995));
#185736=CARTESIAN_POINT('Ctrl Pts',(17.3880466788383,-68.8236353260961,
-176.690807598274));
#185737=CARTESIAN_POINT('Ctrl Pts',(17.038994500873,-68.9322836414647,-176.752287790566));
#185738=CARTESIAN_POINT('Ctrl Pts',(17.0433452950906,-69.3023910050376,
-176.770445463412));
#185739=CARTESIAN_POINT('Ctrl Pts',(17.4191280954739,-68.8139047586067,
-176.874276825325));
#185740=CARTESIAN_POINT('Ctrl Pts',(17.0626089168816,-68.9251254936702,
-176.864255982328));
#185741=CARTESIAN_POINT('Ctrl Pts',(17.0589896637034,-69.292572888558,-176.862105468243));
#185742=CARTESIAN_POINT('Ctrl Pts',(17.394639930152,-68.8216149564082,-177.068700056101));
#185743=CARTESIAN_POINT('Ctrl Pts',(17.0432848595555,-68.9310044443038,
-176.986133124776));
#185744=CARTESIAN_POINT('Ctrl Pts',(17.0466665865239,-69.3003518068395,
-176.959226205544));
#185745=CARTESIAN_POINT('Ctrl Pts',(17.271522613636,-68.8597838444499,-177.362008470827));
#185746=CARTESIAN_POINT('Ctrl Pts',(16.9544868301422,-68.9577361986752,
-177.158772927448));
#185747=CARTESIAN_POINT('Ctrl Pts',(16.9846783298497,-69.3388689248328,
-177.105787340716));
#185748=CARTESIAN_POINT('Ctrl Pts',(17.1958580434816,-68.8831664553272,
-177.473129011102));
#185749=CARTESIAN_POINT('Ctrl Pts',(16.8998209438857,-68.9741481933376,
-177.221234746742));
#185750=CARTESIAN_POINT('Ctrl Pts',(16.9465808939194,-69.3624640417944,
-177.161324454504));
#185751=CARTESIAN_POINT('Ctrl Pts',(17.0115440055365,-68.9395167543114,
-177.65527913718));
#185752=CARTESIAN_POINT('Ctrl Pts',(16.7731937352441,-69.0119018737478,
-177.313591442829));
#185753=CARTESIAN_POINT('Ctrl Pts',(16.8537504063022,-69.4193302850168,
-177.252399550336));
#185754=CARTESIAN_POINT('Ctrl Pts',(16.901371584146,-68.9729353808306,-177.727810792065));
#185755=CARTESIAN_POINT('Ctrl Pts',(16.6994218041251,-69.0337699903486,
-177.343918516311));
#185756=CARTESIAN_POINT('Ctrl Pts',(16.7982523396534,-69.4530549873958,
-177.288688678996));
#185757=CARTESIAN_POINT('Ctrl Pts',(16.618372268784,-69.0576898916785,-177.843950929236));
#185758=CARTESIAN_POINT('Ctrl Pts',(16.521465396758,-69.0861983475692,-177.375991886255));
#185759=CARTESIAN_POINT('Ctrl Pts',(16.6556481050719,-69.5385895805552,
-177.346851666338));
#185760=CARTESIAN_POINT('Ctrl Pts',(16.4326032723997,-69.1124772258283,
-177.866548824772));
#185761=CARTESIAN_POINT('Ctrl Pts',(16.4142810526698,-69.1175007347054,
-177.359511295888));
#185762=CARTESIAN_POINT('Ctrl Pts',(16.5619959483196,-69.5938880549685,
-177.358242713103));
#185763=CARTESIAN_POINT('Ctrl Pts',(16.2582586240097,-69.1628382672821,
-177.837630803223));
#185764=CARTESIAN_POINT('Ctrl Pts',(16.3327830474041,-69.141293341008,-177.320021141446));
#185765=CARTESIAN_POINT('Ctrl Pts',(16.4740613080989,-69.6447181033276,
-177.343862647942));
#185766=CARTESIAN_POINT('',(17.4012711864406,-68.8194987407181,-176.84995));
#185767=CARTESIAN_POINT('Ctrl Pts',(17.4012711864406,-68.8194987407181,
-176.84995));
#185768=CARTESIAN_POINT('Ctrl Pts',(17.4012711797275,-68.8194987428096,
-176.887694684675));
#185769=CARTESIAN_POINT('Ctrl Pts',(17.3991058038741,-68.8201748588276,
-176.925251096234));
#185770=CARTESIAN_POINT('Ctrl Pts',(17.3948976591097,-68.8214863041692,
-176.962447012708));
#185771=CARTESIAN_POINT('Ctrl Pts',(17.3906053585138,-68.8228239762163,
-177.000386785074));
#185772=CARTESIAN_POINT('Ctrl Pts',(17.3841876175728,-68.8248226995135,
-177.037952567699));
#185773=CARTESIAN_POINT('Ctrl Pts',(17.3757224555706,-68.8274555088436,
-177.074968429999));
#185774=CARTESIAN_POINT('Ctrl Pts',(17.3672590966796,-68.8300877573754,
-177.11197640778));
#185775=CARTESIAN_POINT('Ctrl Pts',(17.356748909814,-68.83335391904,-177.148435801524));
#185776=CARTESIAN_POINT('Ctrl Pts',(17.3442218215212,-68.837241948804,-177.184161144092));
#185777=CARTESIAN_POINT('Ctrl Pts',(17.3378147381211,-68.839230513934,-177.202433167405));
#185778=CARTESIAN_POINT('Ctrl Pts',(17.3308793073379,-68.8413819840089,
-177.22051291325));
#185779=CARTESIAN_POINT('Ctrl Pts',(17.3234150119904,-68.8436961361599,
-177.238373157981));
#185780=CARTESIAN_POINT('Ctrl Pts',(17.323216781765,-68.8437575933882,-177.238847474735));
#185781=CARTESIAN_POINT('Ctrl Pts',(17.3230181873272,-68.8438191626283,
-177.239321615502));
#185782=CARTESIAN_POINT('Ctrl Pts',(17.3228192288394,-68.8438808438229,
-177.23979557955));
#185783=CARTESIAN_POINT('Ctrl Pts',(17.2882744024223,-68.8545904455369,
-177.322089157366));
#185784=CARTESIAN_POINT('Ctrl Pts',(17.2426551334793,-68.8686994417092,
-177.39942640593));
#185785=CARTESIAN_POINT('Ctrl Pts',(17.1883023464386,-68.8854065190396,
-177.46904491663));
#185786=CARTESIAN_POINT('Ctrl Pts',(17.1624825557959,-68.8933430621758,
-177.502116548629));
#185787=CARTESIAN_POINT('Ctrl Pts',(17.1346920798654,-68.9018658361706,
-177.533445664936));
#185788=CARTESIAN_POINT('Ctrl Pts',(17.1051831298931,-68.9108884594798,
-177.562732114831));
#185789=CARTESIAN_POINT('Ctrl Pts',(17.104688915706,-68.9110395698531,-177.5632226026));
#185790=CARTESIAN_POINT('Ctrl Pts',(17.1041942190907,-68.9111908205538,
-177.563712518466));
#185791=CARTESIAN_POINT('Ctrl Pts',(17.1036990412529,-68.9113422111695,
-177.564201860987));
#185792=CARTESIAN_POINT('Ctrl Pts',(17.0462278720981,-68.928912859572,-177.620995773435));
#185793=CARTESIAN_POINT('Ctrl Pts',(16.9816775189014,-68.9485450280233,
-177.670649891561));
#185794=CARTESIAN_POINT('Ctrl Pts',(16.9125398584853,-68.9694257059557,
-177.71172930656));
#185795=CARTESIAN_POINT('Ctrl Pts',(16.8713991530569,-68.9818508562253,
-177.736173814828));
#185796=CARTESIAN_POINT('Ctrl Pts',(16.8286352683534,-68.9947177370481,
-177.757582237901));
#185797=CARTESIAN_POINT('Ctrl Pts',(16.7847809634131,-69.007852694924,-177.775654990622));
#185798=CARTESIAN_POINT('Ctrl Pts',(16.78433889104,-69.007985101583,-177.775837172615));
#185799=CARTESIAN_POINT('Ctrl Pts',(16.7838967203631,-69.008117531739,-177.776019010763));
#185800=CARTESIAN_POINT('Ctrl Pts',(16.7834544517973,-69.0082499852543,
-177.776200504879));
#185801=CARTESIAN_POINT('Ctrl Pts',(16.7449698092193,-69.0197756205531,
-177.791993479437));
#185802=CARTESIAN_POINT('Ctrl Pts',(16.7054466746898,-69.0315662591249,
-177.805303057386));
#185803=CARTESIAN_POINT('Ctrl Pts',(16.6651986963193,-69.0435261398608,
-177.816095296664));
#185804=CARTESIAN_POINT('Ctrl Pts',(16.6237252999668,-69.0558501594554,
-177.827216123976));
#185805=CARTESIAN_POINT('Ctrl Pts',(16.5814808439821,-69.0683543171783,
-177.835664557351));
#185806=CARTESIAN_POINT('Ctrl Pts',(16.5387947985051,-69.0809368867563,
-177.841347934728));
#185807=CARTESIAN_POINT('Ctrl Pts',(16.4988275773256,-69.0927180282443,
-177.84666931782));
#185808=CARTESIAN_POINT('Ctrl Pts',(16.458472065883,-69.1045682551433,-177.849566394706));
#185809=CARTESIAN_POINT('Ctrl Pts',(16.4180055598673,-69.1164010707451,
-177.849914459328));
#185810=CARTESIAN_POINT('Ctrl Pts',(16.4152527710431,-69.1172060140366,
-177.849938136895));
#185811=CARTESIAN_POINT('Ctrl Pts',(16.41249947515,-69.1180108744162,-177.849949999677));
#185812=CARTESIAN_POINT('Ctrl Pts',(16.4097457627119,-69.1188156235219,
-177.84995));
#185813=CARTESIAN_POINT('Origin',(17.55,-69.2968662511513,-176.84995));
#185814=CARTESIAN_POINT('Origin',(17.55,-69.2968662511513,-179.64995));
#185815=CARTESIAN_POINT('',(17.4012711864406,-68.8194987407181,-179.64995));
#185816=CARTESIAN_POINT('Origin',(0.,-12.9675000200281,-171.871644662643));
#185817=CARTESIAN_POINT('Origin',(0.,-12.9675000200281,-171.871644662643));
#185818=CARTESIAN_POINT('Origin',(23.2,-67.2147119299503,-179.64995));
#185819=CARTESIAN_POINT('',(23.0033898305085,-66.7549897951205,-176.84995));
#185820=CARTESIAN_POINT('Origin',(23.2,-67.2147119299503,-176.84995));
#185821=CARTESIAN_POINT('',(23.0033898305085,-66.7549897951205,-179.64995));
#185822=CARTESIAN_POINT('Ctrl Pts',(23.9949152542395,-66.3200448697526,
-177.84995));
#185823=CARTESIAN_POINT('Ctrl Pts',(23.9949152542386,-66.320044869753,-177.34995));
#185824=CARTESIAN_POINT('Ctrl Pts',(24.2000000000011,-66.7760495265879,
-177.34995));
#185825=CARTESIAN_POINT('Ctrl Pts',(23.8703538324233,-66.3760654545035,
-177.849949984965));
#185826=CARTESIAN_POINT('Ctrl Pts',(23.9206657457682,-66.3534380400361,
-177.323497139763));
#185827=CARTESIAN_POINT('Ctrl Pts',(24.1371859654851,-66.8325498277328,
-177.34995));
#185828=CARTESIAN_POINT('Ctrl Pts',(23.7477652296632,-66.4306666697135,
-177.82675752222));
#185829=CARTESIAN_POINT('Ctrl Pts',(23.85857311611,-66.3812761568117,-177.28202856183));
#185830=CARTESIAN_POINT('Ctrl Pts',(24.0753687900163,-66.8876168115863,
-177.338353763422));
#185831=CARTESIAN_POINT('Ctrl Pts',(23.5124556672824,-66.534569849442,-177.732855161513));
#185832=CARTESIAN_POINT('Ctrl Pts',(23.7605684693856,-66.4255018631538,
-177.182659406882));
#185833=CARTESIAN_POINT('Ctrl Pts',(23.9567084144264,-66.9924080535444,
-177.291402578445));
#185834=CARTESIAN_POINT('Ctrl Pts',(23.4045112120254,-66.5817650498296,
-177.66401934989));
#185835=CARTESIAN_POINT('Ctrl Pts',(23.728650188117,-66.4401283754592,-177.126465197113));
#185836=CARTESIAN_POINT('Ctrl Pts',(23.9022748831747,-67.0400066306863,
-177.256984676403));
#185837=CARTESIAN_POINT('Ctrl Pts',(23.2160104726183,-66.6636583322845,
-177.482533676026));
#185838=CARTESIAN_POINT('Ctrl Pts',(23.6923095199098,-66.4575908379652,
-177.01948600884));
#185839=CARTESIAN_POINT('Ctrl Pts',(23.8072189577995,-67.1225998569154,
-177.166241836555));
#185840=CARTESIAN_POINT('Ctrl Pts',(23.1390036429345,-66.6968206283899,
-177.372560789955));
#185841=CARTESIAN_POINT('Ctrl Pts',(23.6901782519314,-66.4593985440301,
-176.972463316884));
#185842=CARTESIAN_POINT('Ctrl Pts',(23.7683864506384,-67.1560455904002,
-177.111255395708));
#185843=CARTESIAN_POINT('Ctrl Pts',(23.0321233068433,-66.742723669979,-177.12454316851));
#185844=CARTESIAN_POINT('Ctrl Pts',(23.6945043498585,-66.4589699067553,
-176.898771091495));
#185845=CARTESIAN_POINT('Ctrl Pts',(23.7144895325829,-67.2023409665867,
-176.987246583524));
#185846=CARTESIAN_POINT('Ctrl Pts',(23.0033898412675,-66.7549897905191,
-176.989728313577));
#185847=CARTESIAN_POINT('Ctrl Pts',(23.6999999982817,-66.4570693060762,
-176.874118380146));
#185848=CARTESIAN_POINT('Ctrl Pts',(23.7,-67.2147119253083,-176.919839157335));
#185849=CARTESIAN_POINT('Ctrl Pts',(23.0033898305084,-66.7549897951205,
-176.84995));
#185850=CARTESIAN_POINT('Ctrl Pts',(23.6999999999999,-66.45706930551,-176.84995));
#185851=CARTESIAN_POINT('Ctrl Pts',(23.7,-67.2147119299503,-176.84995));
#185852=CARTESIAN_POINT('Ctrl Pts',(23.9949152542395,-66.3200448697526,
-177.84995));
#185853=CARTESIAN_POINT('Ctrl Pts',(23.9428551887954,-66.3434585018855,
-177.849949993716));
#185854=CARTESIAN_POINT('Ctrl Pts',(23.8912891629463,-66.3665571088583,
-177.845903065055));
#185855=CARTESIAN_POINT('Ctrl Pts',(23.8403424606449,-66.3892926538624,
-177.83781160242));
#185856=CARTESIAN_POINT('Ctrl Pts',(23.7898936124082,-66.411806025831,-177.829799210017));
#185857=CARTESIAN_POINT('Ctrl Pts',(23.740051601186,-66.4339635775751,-177.817820923569));
#185858=CARTESIAN_POINT('Ctrl Pts',(23.6909420374968,-66.4557157061558,
-177.801828391251));
#185859=CARTESIAN_POINT('Ctrl Pts',(23.6705352998632,-66.4647544747291,
-177.795182935934));
#185860=CARTESIAN_POINT('Ctrl Pts',(23.6502551185154,-66.4737231883062,
-177.78784373804));
#185861=CARTESIAN_POINT('Ctrl Pts',(23.6301109846052,-66.4826180228466,
-177.779804722709));
#185862=CARTESIAN_POINT('Ctrl Pts',(23.6296825902114,-66.4828071844789,
-177.779633761321));
#185863=CARTESIAN_POINT('Ctrl Pts',(23.6292543206867,-66.4829962847601,
-177.77946250822));
#185864=CARTESIAN_POINT('Ctrl Pts',(23.628826176177,-66.4831853236384,-177.779290963367));
#185865=CARTESIAN_POINT('Ctrl Pts',(23.549083605048,-66.5183941044447,-177.747340471676));
#185866=CARTESIAN_POINT('Ctrl Pts',(23.4738664381757,-66.5513895428365,
-177.705344056631));
#185867=CARTESIAN_POINT('Ctrl Pts',(23.4044230513637,-66.5817044397988,
-177.653364341203));
#185868=CARTESIAN_POINT('Ctrl Pts',(23.3717123604556,-66.5959840029072,
-177.628879757676));
#185869=CARTESIAN_POINT('Ctrl Pts',(23.340282339806,-66.6096689890179,-177.60218062655));
#185870=CARTESIAN_POINT('Ctrl Pts',(23.3102608826734,-66.6227116735265,
-177.57327646271));
#185871=CARTESIAN_POINT('Ctrl Pts',(23.3097552045839,-66.6229313630558,
-177.572789604185));
#185872=CARTESIAN_POINT('Ctrl Pts',(23.3092500282568,-66.6231508261632,
-177.572302197161));
#185873=CARTESIAN_POINT('Ctrl Pts',(23.3087453546535,-66.6233700624812,
-177.571814242488));
#185874=CARTESIAN_POINT('Ctrl Pts',(23.2428791470159,-66.6519831398302,
-177.508130064148));
#185875=CARTESIAN_POINT('Ctrl Pts',(23.1855484931327,-66.6767452815919,
-177.435089847604));
#185876=CARTESIAN_POINT('Ctrl Pts',(23.1388722340366,-66.696846286165,-177.354542469168));
#185877=CARTESIAN_POINT('Ctrl Pts',(23.1191486795936,-66.7053401814714,
-177.320506309574));
#185878=CARTESIAN_POINT('Ctrl Pts',(23.101326993937,-66.7130020216598,-177.285129627946));
#185879=CARTESIAN_POINT('Ctrl Pts',(23.0855644128598,-66.7197717463455,
-177.248551496375));
#185880=CARTESIAN_POINT('Ctrl Pts',(23.0853517691174,-66.7198630727333,
-177.248058042242));
#185881=CARTESIAN_POINT('Ctrl Pts',(23.0851395181392,-66.7199542292592,
-177.24756442059));
#185882=CARTESIAN_POINT('Ctrl Pts',(23.0849276601637,-66.7200452158304,
-177.247070631801));
#185883=CARTESIAN_POINT('Ctrl Pts',(23.0685067964827,-66.7270974784524,
-177.208797640755));
#185884=CARTESIAN_POINT('Ctrl Pts',(23.0544044796133,-66.7331469401741,
-177.169412579499));
#185885=CARTESIAN_POINT('Ctrl Pts',(23.0427873419503,-66.7381263973539,
-177.129172865924));
#185886=CARTESIAN_POINT('Ctrl Pts',(23.0313107069201,-66.7430456308483,
-177.08941982866));
#185887=CARTESIAN_POINT('Ctrl Pts',(23.022259763421,-66.746920485885,-177.048833228896));
#185888=CARTESIAN_POINT('Ctrl Pts',(23.015750900502,-66.7497052241091,-177.007676413085));
#185889=CARTESIAN_POINT('Ctrl Pts',(23.0093646056923,-66.7524375230511,
-176.967294619449));
#185890=CARTESIAN_POINT('Ctrl Pts',(23.0054256948345,-66.7541203250939,
-176.926364378225));
#185891=CARTESIAN_POINT('Ctrl Pts',(23.0039983429948,-66.7547299427615,
-176.88514146636));
#185892=CARTESIAN_POINT('Ctrl Pts',(23.0035929213886,-66.7549030971072,
-176.873432608967));
#185893=CARTESIAN_POINT('Ctrl Pts',(23.0033898314129,-66.7549897947337,
-176.861700158874));
#185894=CARTESIAN_POINT('Ctrl Pts',(23.0033898305084,-66.7549897951205,
-176.84995));
#185895=CARTESIAN_POINT('Origin',(44.5079524583208,31.5404524382925,-171.64995));
#185896=CARTESIAN_POINT('',(44.5079524583208,28.7904524382925,-179.64995));
#185897=CARTESIAN_POINT('',(44.5079524583208,28.7904524382925,-171.64995));
#185898=CARTESIAN_POINT('Origin',(44.5079524583208,31.5404524382925,-179.64995));
#185899=CARTESIAN_POINT('Origin',(44.5079524583208,-57.4754524783487,-171.64995));
#185900=CARTESIAN_POINT('',(44.5079524583208,-60.2254524783487,-179.64995));
#185901=CARTESIAN_POINT('',(44.5079524583208,-60.2254524783487,-171.64995));
#185902=CARTESIAN_POINT('Origin',(44.5079524583208,-57.4754524783487,-179.64995));
#185903=CARTESIAN_POINT('Origin',(26.4569673975197,-68.4857751744904,-179.39995));
#185904=CARTESIAN_POINT('',(25.0588349740736,-65.5518825850269,-179.64995));
#185905=CARTESIAN_POINT('Origin',(25.0588349740736,-65.5518825850269,-179.39995));
#185906=CARTESIAN_POINT('',(26.0046548193995,-65.2674039510802,-179.64995));
#185907=CARTESIAN_POINT('Origin',(26.4569673975197,-68.4857751744904,-179.64995));
#185908=CARTESIAN_POINT('Origin',(26.0046548193995,-65.2674039510803,-179.39995));
#185909=CARTESIAN_POINT('Origin',(51.7734815964994,-61.6458315265255,-179.39995));
#185910=CARTESIAN_POINT('',(44.5938155824071,-62.6548677810304,-179.64995));
#185911=CARTESIAN_POINT('',(26.0046548193995,-65.2674039510802,-179.64995));
#185912=CARTESIAN_POINT('Origin',(44.5938155824071,-62.6548677810303,-179.39995));
#185913=CARTESIAN_POINT('Origin',(44.2110895547669,-59.9316305919911,-179.39995));
#185914=CARTESIAN_POINT('',(46.0960584892725,-61.9339772442841,-179.64995));
#185915=CARTESIAN_POINT('Origin',(44.2110895547669,-59.9316305919911,-179.64995));
#185916=CARTESIAN_POINT('Origin',(46.0960584892725,-61.9339772442841,-179.39995));
#185917=CARTESIAN_POINT('Origin',(0.,-12.9675000200281,-179.39995));
#185918=CARTESIAN_POINT('',(48.9664772242561,-59.0635585093003,-179.64995));
#185919=CARTESIAN_POINT('Origin',(0.,-12.9675000200281,-179.64995));
#185920=CARTESIAN_POINT('Origin',(48.9664772242561,-59.0635585093003,-179.39995));
#185921=CARTESIAN_POINT('Origin',(46.9641305719631,-57.1785895747948,-179.39995));
#185922=CARTESIAN_POINT('',(49.6873677610024,-57.561315602435,-179.64995));
#185923=CARTESIAN_POINT('Origin',(46.9641305719631,-57.1785895747948,-179.64995));
#185924=CARTESIAN_POINT('Origin',(49.6873677610024,-57.561315602435,-179.39995));
#185925=CARTESIAN_POINT('Origin',(50.3220654694669,-53.04520674476,-179.39995));
#185926=CARTESIAN_POINT('',(52.2574626216431,-39.2741404473771,-179.64995));
#185927=CARTESIAN_POINT('',(49.6873677610024,-57.561315602435,-179.64995));
#185928=CARTESIAN_POINT('Origin',(52.2574626216431,-39.2741404473771,-179.39995));
#185929=CARTESIAN_POINT('Origin',(57.4563699825363,-40.0047992274175,-179.39995));
#185930=CARTESIAN_POINT('',(52.7060401808306,-37.7694319701137,-179.64995));
#185931=CARTESIAN_POINT('Origin',(57.4563699825363,-40.0047992274175,-179.64995));
#185932=CARTESIAN_POINT('Origin',(52.7060401808306,-37.7694319701137,-179.39995));
#185933=CARTESIAN_POINT('Origin',(0.,-12.9675000200281,-179.39995));
#185934=CARTESIAN_POINT('',(52.7060401808306,11.8344319300573,-179.64995));
#185935=CARTESIAN_POINT('Origin',(0.,-12.9675000200281,-179.64995));
#185936=CARTESIAN_POINT('Origin',(52.7060401808306,11.8344319300573,-179.39995));
#185937=CARTESIAN_POINT('Origin',(57.4563699825364,14.0697991873612,-179.39995));
#185938=CARTESIAN_POINT('',(52.2574626216432,13.3391404073208,-179.64995));
#185939=CARTESIAN_POINT('Origin',(57.4563699825364,14.0697991873612,-179.64995));
#185940=CARTESIAN_POINT('Origin',(52.2574626216431,13.3391404073208,-179.39995));
#185941=CARTESIAN_POINT('Origin',(61.3785689046687,-51.5609030735669,-179.39995));
#185942=CARTESIAN_POINT('',(49.6873677610025,31.6263155623787,-179.64995));
#185943=CARTESIAN_POINT('',(52.2574626216432,13.3391404073208,-179.64995));
#185944=CARTESIAN_POINT('Origin',(49.6873677610024,31.6263155623787,-179.39995));
#185945=CARTESIAN_POINT('Origin',(46.9641305719631,31.2435895347386,-179.39995));
#185946=CARTESIAN_POINT('',(48.9664772242561,33.1285584692441,-179.64995));
#185947=CARTESIAN_POINT('Origin',(46.9641305719631,31.2435895347386,-179.64995));
#185948=CARTESIAN_POINT('Origin',(48.9664772242561,33.1285584692441,-179.39995));
#185949=CARTESIAN_POINT('Origin',(0.,-12.9675000200281,-179.39995));
#185950=CARTESIAN_POINT('',(46.0960584892724,35.9989772042278,-179.64995));
#185951=CARTESIAN_POINT('Origin',(0.,-12.9675000200281,-179.64995));
#185952=CARTESIAN_POINT('Origin',(46.0960584892724,35.9989772042278,-179.39995));
#185953=CARTESIAN_POINT('Origin',(44.2110895547669,33.9966305519348,-179.39995));
#185954=CARTESIAN_POINT('',(44.593815582407,36.7198677409741,-179.64995));
#185955=CARTESIAN_POINT('Origin',(44.2110895547669,33.9966305519348,-179.64995));
#185956=CARTESIAN_POINT('Origin',(44.593815582407,36.7198677409741,-179.39995));
#185957=CARTESIAN_POINT('Origin',(62.8299850317005,34.1569412647963,-179.39995));
#185958=CARTESIAN_POINT('',(26.3066404273498,39.2899626016146,-179.64995));
#185959=CARTESIAN_POINT('',(44.593815582407,36.7198677409741,-179.64995));
#185960=CARTESIAN_POINT('Origin',(26.3066404273498,39.2899626016146,-179.39995));
#185961=CARTESIAN_POINT('Origin',(27.0372992073901,44.4888699625078,-179.39995));
#185962=CARTESIAN_POINT('',(24.8019319500862,39.7385401608021,-179.64995));
#185963=CARTESIAN_POINT('Origin',(27.0372992073901,44.4888699625078,-179.64995));
#185964=CARTESIAN_POINT('',(24.9083780099579,39.9647463418357,-179.39995));
#185965=CARTESIAN_POINT('Origin',(24.8019319500862,39.7385401608021,-179.39995));
#185966=CARTESIAN_POINT('Origin',(27.0372992073901,44.4888699625078,-179.39995));
#185967=CARTESIAN_POINT('Origin',(27.0372992073901,44.4888699625078,-179.64995));
#185968=CARTESIAN_POINT('',(24.9083780099579,39.9647463418357,-177.84995));
#185969=CARTESIAN_POINT('',(24.9083780099579,39.9647463418357,-179.64995));
#185970=CARTESIAN_POINT('Origin',(27.0372992073901,44.4888699625078,-177.84995));
#185971=CARTESIAN_POINT('Origin',(45.6308101826775,37.3314983336592,-177.84995));
#185972=CARTESIAN_POINT('',(26.4110202530699,40.0326636531708,-177.34995));
#185973=CARTESIAN_POINT('Origin',(26.4110202530699,40.0326636531708,-177.84995));
#185974=CARTESIAN_POINT('',(-42.7876488459256,49.7579023686377,-177.34995));
#185975=CARTESIAN_POINT('Origin',(27.0372992073901,44.4888699625078,-177.84995));
#185976=CARTESIAN_POINT('',(25.121270129701,40.4171587039029,-177.34995));
#185977=CARTESIAN_POINT('Origin',(25.121270129701,40.4171587039029,-177.84995));
#185978=CARTESIAN_POINT('Origin',(27.0372992073901,44.4888699625078,-177.34995));
#185979=CARTESIAN_POINT('Origin',(38.5,58.91999998,-174.34995));
#185980=CARTESIAN_POINT('',(41.5,58.91999998,-174.34995));
#185981=CARTESIAN_POINT('',(41.5,58.91999998,-174.34995));
#185982=CARTESIAN_POINT('',(38.5,58.91999998,-177.34995));
#185983=CARTESIAN_POINT('',(38.5,58.91999998,-177.34995));
#185984=CARTESIAN_POINT('Origin',(38.5,58.91999998,-174.34995));
#185985=CARTESIAN_POINT('Origin',(41.5,58.91999998,-92.34995));
#185986=CARTESIAN_POINT('',(41.5,58.91999998,-95.34995));
#185987=CARTESIAN_POINT('',(41.5,58.91999998,-92.34995));
#185988=CARTESIAN_POINT('',(41.5,58.91999998,-95.34995));
#185989=CARTESIAN_POINT('Origin',(37.,58.91999998,-91.84995));
#185990=CARTESIAN_POINT('',(37.,46.41999998,-92.34995));
#185991=CARTESIAN_POINT('Origin',(37.,46.41999998,-91.84995));
#185992=CARTESIAN_POINT('',(37.,46.41999998,-92.34995));
#185993=CARTESIAN_POINT('Origin',(60.,29.41999998,-91.34995));
#185994=CARTESIAN_POINT('',(37.5,29.41999998,-92.34995));
#185995=CARTESIAN_POINT('Origin',(31.,-9.33460238845303,-91.84995));
#185996=CARTESIAN_POINT('',(31.,46.41999998,-92.34995));
#185997=CARTESIAN_POINT('Origin',(31.,46.41999998,-91.84995));
#185998=CARTESIAN_POINT('',(31.,29.41999998,-92.34995));
#185999=CARTESIAN_POINT('Origin',(30.,46.41999998,-91.84995));
#186000=CARTESIAN_POINT('',(30.,47.41999998,-92.34995));
#186001=CARTESIAN_POINT('Origin',(30.,47.41999998,-91.84995));
#186002=CARTESIAN_POINT('Origin',(30.,46.41999998,-92.34995));
#186003=CARTESIAN_POINT('Origin',(-41.5,47.41999998,-91.84995));
#186004=CARTESIAN_POINT('',(29.5,47.41999998,-92.34995));
#186005=CARTESIAN_POINT('Origin',(29.5,47.41999998,-91.84995));
#186006=CARTESIAN_POINT('',(-41.5,47.41999998,-92.34995));
#186007=CARTESIAN_POINT('Origin',(29.5,46.41999998,-91.84995));
#186008=CARTESIAN_POINT('',(28.5,46.41999998,-92.34995));
#186009=CARTESIAN_POINT('Origin',(28.5,46.41999998,-91.84995));
#186010=CARTESIAN_POINT('Origin',(29.5,46.41999998,-92.34995));
#186011=CARTESIAN_POINT('Origin',(28.5,58.91999998,-91.84995));
#186012=CARTESIAN_POINT('',(28.5,46.41999998,-92.34995));
#186013=CARTESIAN_POINT('Origin',(60.,29.41999998,-91.34995));
#186014=CARTESIAN_POINT('',(29.,29.41999998,-92.34995));
#186015=CARTESIAN_POINT('Origin',(22.5,-9.33460238845303,-91.84995));
#186016=CARTESIAN_POINT('',(22.5,46.41999998,-92.34995));
#186017=CARTESIAN_POINT('Origin',(22.5,46.41999998,-91.84995));
#186018=CARTESIAN_POINT('',(22.5,29.41999998,-92.34995));
#186019=CARTESIAN_POINT('Origin',(21.5,46.41999998,-91.84995));
#186020=CARTESIAN_POINT('',(21.5,47.41999998,-92.34995));
#186021=CARTESIAN_POINT('Origin',(21.5,47.41999998,-91.84995));
#186022=CARTESIAN_POINT('Origin',(21.5,46.41999998,-92.34995));
#186023=CARTESIAN_POINT('Origin',(-41.5,47.41999998,-91.84995));
#186024=CARTESIAN_POINT('',(21.,47.41999998,-92.34995));
#186025=CARTESIAN_POINT('Origin',(21.,47.41999998,-91.84995));
#186026=CARTESIAN_POINT('',(-41.5,47.41999998,-92.34995));
#186027=CARTESIAN_POINT('Origin',(21.,46.41999998,-91.84995));
#186028=CARTESIAN_POINT('',(20.,46.41999998,-92.34995));
#186029=CARTESIAN_POINT('Origin',(20.,46.41999998,-91.84995));
#186030=CARTESIAN_POINT('Origin',(21.,46.41999998,-92.34995));
#186031=CARTESIAN_POINT('Origin',(20.,58.91999998,-91.84995));
#186032=CARTESIAN_POINT('',(20.,46.41999998,-92.34995));
#186033=CARTESIAN_POINT('Origin',(60.,29.41999998,-91.34995));
#186034=CARTESIAN_POINT('',(17.5283605562717,29.41999998,-92.34995));
#186035=CARTESIAN_POINT('',(20.5,29.41999998,-92.34995));
#186036=CARTESIAN_POINT('Origin',(17.5283605562717,29.41999998,-91.34995));
#186037=CARTESIAN_POINT('Ctrl Pts',(17.5283605562717,28.4199999800001,-91.34995));
#186038=CARTESIAN_POINT('Ctrl Pts',(17.5283605562716,28.41999998,-92.34995));
#186039=CARTESIAN_POINT('Ctrl Pts',(17.5283605562717,29.4199999800001,-92.34995));
#186040=CARTESIAN_POINT('Ctrl Pts',(16.8748117549663,28.4199999800001,-91.2778699709694));
#186041=CARTESIAN_POINT('Ctrl Pts',(16.8501904102942,28.3452044605545,-92.3499500000001));
#186042=CARTESIAN_POINT('Ctrl Pts',(16.9294484484718,29.4199999819522,-92.34995));
#186043=CARTESIAN_POINT('Ctrl Pts',(16.233134779349,28.4803469141606,-91.2065756291954));
#186044=CARTESIAN_POINT('Ctrl Pts',(16.1934854928648,28.3221299458475,-92.34995));
#186045=CARTESIAN_POINT('Ctrl Pts',(16.3387077693293,29.4682775272991,-92.34995));
#186046=CARTESIAN_POINT('Ctrl Pts',(14.9727946058278,28.7108958947333,-91.0656179778369));
#186047=CARTESIAN_POINT('Ctrl Pts',(14.8701093399109,28.3452025116243,-92.34995));
#186048=CARTESIAN_POINT('Ctrl Pts',(15.1723882243972,29.6527167118161,-92.34995));
#186049=CARTESIAN_POINT('Ctrl Pts',(14.3539522178783,28.8809201843631,-90.9959326732687));
#186050=CARTESIAN_POINT('Ctrl Pts',(14.194875318369,28.3987342821361,-92.3499499999805));
#186051=CARTESIAN_POINT('Ctrl Pts',(14.5966754937866,29.7887243470281,-92.34995));
#186052=CARTESIAN_POINT('Ctrl Pts',(13.7480613600421,29.1125253108927,-90.92733173826));
#186053=CARTESIAN_POINT('Ctrl Pts',(13.5420441920761,28.4819485757734,-92.3499500000002));
#186054=CARTESIAN_POINT('Ctrl Pts',(14.0295223410746,29.9740202447142,-92.34995));
#186055=CARTESIAN_POINT('',(14.0295223410747,29.9740202447141,-92.34995));
#186056=CARTESIAN_POINT('Origin',(14.0295223410747,29.9740202447144,-91.34995));
#186057=CARTESIAN_POINT('Ctrl Pts',(14.0295223410747,29.9740202447141,-92.34995));
#186058=CARTESIAN_POINT('Ctrl Pts',(14.5967291533814,29.7887068092282,-92.34995));
#186059=CARTESIAN_POINT('Ctrl Pts',(15.1723882243932,29.6527167117912,-92.34995));
#186060=CARTESIAN_POINT('Ctrl Pts',(16.3387077693334,29.4682775273239,-92.34995));
#186061=CARTESIAN_POINT('Ctrl Pts',(16.9293976390415,29.4199999800001,-92.34995));
#186062=CARTESIAN_POINT('Ctrl Pts',(17.5283605562717,29.41999998,-92.34995));
#186063=CARTESIAN_POINT('Origin',(1.1373643128445E-15,-12.9675000200281,
-91.34995));
#186064=CARTESIAN_POINT('Origin',(1.1373643128445E-15,-12.9675000200281,
-92.34995));
#186065=CARTESIAN_POINT('Origin',(14.,-9.33460238845303,-91.84995));
#186066=CARTESIAN_POINT('',(14.,46.41999998,-92.34995));
#186067=CARTESIAN_POINT('Origin',(14.,46.41999998,-91.84995));
#186068=CARTESIAN_POINT('',(14.,30.1434227231235,-92.34995));
#186069=CARTESIAN_POINT('Origin',(13.,46.41999998,-91.84995));
#186070=CARTESIAN_POINT('',(13.,47.41999998,-92.34995));
#186071=CARTESIAN_POINT('Origin',(13.,47.41999998,-91.84995));
#186072=CARTESIAN_POINT('Origin',(13.,46.41999998,-92.34995));
#186073=CARTESIAN_POINT('Origin',(-41.5,47.41999998,-91.84995));
#186074=CARTESIAN_POINT('',(12.5,47.41999998,-92.34995));
#186075=CARTESIAN_POINT('Origin',(12.5,47.41999998,-91.84995));
#186076=CARTESIAN_POINT('',(-41.5,47.41999998,-92.34995));
#186077=CARTESIAN_POINT('Origin',(12.5,46.41999998,-91.84995));
#186078=CARTESIAN_POINT('',(11.5,46.41999998,-92.34995));
#186079=CARTESIAN_POINT('Origin',(11.5,46.41999998,-91.84995));
#186080=CARTESIAN_POINT('Origin',(12.5,46.41999998,-92.34995));
#186081=CARTESIAN_POINT('Origin',(11.5,58.91999998,-91.84995));
#186082=CARTESIAN_POINT('',(11.5,46.41999998,-92.34995));
#186083=CARTESIAN_POINT('Origin',(1.1373643128445E-15,-12.9675000200281,
-91.34995));
#186084=CARTESIAN_POINT('Origin',(1.1373643128445E-15,-12.9675000200281,
-92.34995));
#186085=CARTESIAN_POINT('Origin',(5.5,-9.33460238845303,-91.84995));
#186086=CARTESIAN_POINT('',(5.5,46.41999998,-92.34995));
#186087=CARTESIAN_POINT('Origin',(5.5,46.41999998,-91.84995));
#186088=CARTESIAN_POINT('',(5.5,31.9301798728793,-92.34995));
#186089=CARTESIAN_POINT('Origin',(4.5,46.41999998,-91.84995));
#186090=CARTESIAN_POINT('',(4.5,47.41999998,-92.34995));
#186091=CARTESIAN_POINT('Origin',(4.5,47.41999998,-91.84995));
#186092=CARTESIAN_POINT('Origin',(4.5,46.41999998,-92.34995));
#186093=CARTESIAN_POINT('Origin',(-41.5,47.41999998,-91.84995));
#186094=CARTESIAN_POINT('',(4.,47.41999998,-92.34995));
#186095=CARTESIAN_POINT('Origin',(4.,47.41999998,-91.84995));
#186096=CARTESIAN_POINT('',(-41.5,47.41999998,-92.34995));
#186097=CARTESIAN_POINT('Origin',(4.,46.41999998,-91.84995));
#186098=CARTESIAN_POINT('',(3.,46.41999998,-92.34995));
#186099=CARTESIAN_POINT('Origin',(3.,46.41999998,-91.84995));
#186100=CARTESIAN_POINT('Origin',(4.,46.41999998,-92.34995));
#186101=CARTESIAN_POINT('Origin',(3.,58.91999998,-91.84995));
#186102=CARTESIAN_POINT('',(3.,32.1080106234021,-92.34995));
#186103=CARTESIAN_POINT('Origin',(3.,32.1080106234021,-91.84995));
#186104=CARTESIAN_POINT('',(3.,46.41999998,-92.34995));
#186105=CARTESIAN_POINT('Origin',(38.5,58.91999998,-95.34995));
#186106=CARTESIAN_POINT('',(38.5,58.91999998,-92.34995));
#186107=CARTESIAN_POINT('Origin',(38.5,58.91999998,-95.34995));
#186108=CARTESIAN_POINT('',(38.5,58.91999998,-92.34995));
#186109=CARTESIAN_POINT('Origin',(-41.5,47.41999998,-91.84995));
#186110=CARTESIAN_POINT('',(38.,47.41999998,-92.34995));
#186111=CARTESIAN_POINT('Origin',(38.,47.41999998,-91.84995));
#186112=CARTESIAN_POINT('',(-41.5,47.41999998,-92.34995));
#186113=CARTESIAN_POINT('Origin',(38.,46.41999998,-91.84995));
#186114=CARTESIAN_POINT('Origin',(38.,46.41999998,-92.34995));
#186115=CARTESIAN_POINT('Ctrl Pts',(2.9730852099506,31.3045898136069,-90.7567930161436));
#186116=CARTESIAN_POINT('Ctrl Pts',(3.50093046722966,31.2817579610315,-90.7398891378361));
#186117=CARTESIAN_POINT('Ctrl Pts',(3.49999922403526,31.7061080469582,-91.0538938313493));
#186118=CARTESIAN_POINT('Ctrl Pts',(2.96831480394843,31.1636040483254,-90.9411472609555));
#186119=CARTESIAN_POINT('Ctrl Pts',(3.50094375794647,31.1316900065056,-90.9272767748672));
#186120=CARTESIAN_POINT('Ctrl Pts',(3.49999921701682,31.6355825669373,-91.1459119172329));
#186121=CARTESIAN_POINT('Ctrl Pts',(2.96597720456975,31.0948501016434,-91.1829665694402));
#186122=CARTESIAN_POINT('Ctrl Pts',(3.50095025048169,31.0578808190773,-91.1768644172926));
#186123=CARTESIAN_POINT('Ctrl Pts',(3.49999921357759,31.6011902598928,-91.2666067024717));
#186124=CARTESIAN_POINT('Ctrl Pts',(2.9666837372529,31.1156607402492,-91.4988149931348));
#186125=CARTESIAN_POINT('Ctrl Pts',(3.50094827348241,31.0802559450011,-91.5041387140221));
#186126=CARTESIAN_POINT('Ctrl Pts',(3.49999921461707,31.6116002328841,-91.4242502749333));
#186127=CARTESIAN_POINT('Ctrl Pts',(2.96723234610694,31.1318174446344,-91.5823694312293));
#186128=CARTESIAN_POINT('Ctrl Pts',(3.50094674031663,31.0976044869907,-91.5905362019412));
#186129=CARTESIAN_POINT('Ctrl Pts',(3.49999921542421,31.6196822275484,-91.4659533973627));
#186130=CARTESIAN_POINT('Ctrl Pts',(2.96900087342029,31.1839643938508,-91.7412472447188));
#186131=CARTESIAN_POINT('Ctrl Pts',(3.50094181368991,31.1534426029942,-91.7542039764945));
#186132=CARTESIAN_POINT('Ctrl Pts',(3.49999921802616,31.6457674414273,-91.5452519327685));
#186133=CARTESIAN_POINT('Ctrl Pts',(2.97020720291435,31.2195539123312,-91.8165845933835));
#186134=CARTESIAN_POINT('Ctrl Pts',(3.50093846494821,31.1914250734018,-91.8313961753176));
#186135=CARTESIAN_POINT('Ctrl Pts',(3.49999921980099,31.6635702854767,-91.582854393305));
#186136=CARTESIAN_POINT('Ctrl Pts',(2.97327686342368,31.3102833845102,-91.9588329995341));
#186137=CARTESIAN_POINT('Ctrl Pts',(3.50092999134622,31.2877769651877,-91.976055099741));
#186138=CARTESIAN_POINT('Ctrl Pts',(3.49999922431731,31.7089557758124,-91.6538544608224));
#186139=CARTESIAN_POINT('Ctrl Pts',(2.97508200188551,31.363705231644,-92.0229770344444));
#186140=CARTESIAN_POINT('Ctrl Pts',(3.50092503769121,31.3442016959818,-92.0406579023939));
#186141=CARTESIAN_POINT('Ctrl Pts',(3.4999992269732,31.735679025568,-91.6858710465136));
#186142=CARTESIAN_POINT('Ctrl Pts',(2.97918951587053,31.4855444640944,-92.1370301830535));
#186143=CARTESIAN_POINT('Ctrl Pts',(3.50091385025873,31.4720404315998,-92.154150157461));
#186144=CARTESIAN_POINT('Ctrl Pts',(3.49999923301664,31.7966270247391,-91.7428001834818));
#186145=CARTESIAN_POINT('Ctrl Pts',(2.98150917200635,31.5544802723793,-92.1869191253344));
#186146=CARTESIAN_POINT('Ctrl Pts',(3.5009075812992,31.5438634599872,-92.2030139201566));
#186147=CARTESIAN_POINT('Ctrl Pts',(3.49999923642963,31.8311111796843,-91.7677027010548));
#186148=CARTESIAN_POINT('Ctrl Pts',(2.99080944970468,31.8316005441471,-92.3387964507699));
#186149=CARTESIAN_POINT('Ctrl Pts',(3.50088278313963,31.8290484154313,-92.3480335721559));
#186150=CARTESIAN_POINT('Ctrl Pts',(3.49999925011377,31.9697383525658,-91.8435168239899));
#186151=CARTESIAN_POINT('Ctrl Pts',(2.99906263916586,32.0790639346103,-92.3785629445754));
#186152=CARTESIAN_POINT('Ctrl Pts',(3.50086123689989,32.0791891259729,-92.3794444887817));
#186153=CARTESIAN_POINT('Ctrl Pts',(3.49999926225773,32.0935311034211,-91.8633729799761));
#186154=CARTESIAN_POINT('Ctrl Pts',(3.00656307387834,32.3061821416724,-92.3288442122165));
#186155=CARTESIAN_POINT('Ctrl Pts',(3.50084207052921,32.3047067774897,-92.3225109654136));
#186156=CARTESIAN_POINT('Ctrl Pts',(3.49999927329452,32.2071461725455,-91.8385626593203));
#186157=CARTESIAN_POINT('',(2.96960200166493,31.2017108282785,-90.9273317382593));
#186158=CARTESIAN_POINT('Origin',(3.,31.6538440087773,-91.1386408691297));
#186159=CARTESIAN_POINT('',(2.96642827403755,31.1080789525293,-91.3499500965915));
#186160=CARTESIAN_POINT('Ctrl Pts',(2.96642827403755,31.1080789525293,-91.3499500965915));
#186161=CARTESIAN_POINT('Ctrl Pts',(2.96642678046511,31.1080459325444,-91.3718155306746));
#186162=CARTESIAN_POINT('Ctrl Pts',(2.96644996804348,31.1087378443562,-91.3937457112765));
#186163=CARTESIAN_POINT('Ctrl Pts',(2.9664988473075,31.1101841867365,-91.4156969915003));
#186164=CARTESIAN_POINT('Ctrl Pts',(2.96658204510027,31.1126460178633,-91.4530604440709));
#186165=CARTESIAN_POINT('Ctrl Pts',(2.96673926306768,31.1172834424333,-91.4908103834415));
#186166=CARTESIAN_POINT('Ctrl Pts',(2.96697200208073,31.1241452740858,-91.5285793415084));
#186167=CARTESIAN_POINT('Ctrl Pts',(2.96718969499616,31.1305635024613,-91.563906614262));
#186168=CARTESIAN_POINT('Ctrl Pts',(2.96747346980304,31.1389281132673,-91.5992509320773));
#186169=CARTESIAN_POINT('Ctrl Pts',(2.96782515711633,31.1492971045932,-91.6342689486014));
#186170=CARTESIAN_POINT('Ctrl Pts',(2.96791760205605,31.1520227098165,-91.6434738255027));
#186171=CARTESIAN_POINT('Ctrl Pts',(2.9680147424783,31.1548868999422,-91.6526558966934));
#186172=CARTESIAN_POINT('Ctrl Pts',(2.96811661795246,31.1578909187456,-91.6618083381375));
#186173=CARTESIAN_POINT('Ctrl Pts',(2.96834122380717,31.1645139083954,-91.6819868153449));
#186174=CARTESIAN_POINT('Ctrl Pts',(2.96858796167743,31.1717904982887,-91.7020221689901));
#186175=CARTESIAN_POINT('Ctrl Pts',(2.96885783449233,31.1797517323839,-91.7219119918425));
#186176=CARTESIAN_POINT('Ctrl Pts',(2.9693297949791,31.1936745423575,-91.7566958231767));
#186177=CARTESIAN_POINT('Ctrl Pts',(2.96987110529427,31.2096497893136,-91.7909173348017));
#186178=CARTESIAN_POINT('Ctrl Pts',(2.97048317220471,31.2277257567495,-91.8244266948797));
#186179=CARTESIAN_POINT('Ctrl Pts',(2.97087397256257,31.2392671330634,-91.8458221823448));
#186180=CARTESIAN_POINT('Ctrl Pts',(2.97129358683363,31.2516639907196,-91.8669277438773));
#186181=CARTESIAN_POINT('Ctrl Pts',(2.97174203316901,31.2649186484207,-91.8877087964588));
#186182=CARTESIAN_POINT('Ctrl Pts',(2.97188629124988,31.269182461795,-91.8943937318173));
#186183=CARTESIAN_POINT('Ctrl Pts',(2.97203290085651,31.2735163747235,-91.9010157806221));
#186184=CARTESIAN_POINT('Ctrl Pts',(2.97218246192385,31.2779381969121,-91.9076009010963));
#186185=CARTESIAN_POINT('Ctrl Pts',(2.97279243835603,31.2959723509214,-91.9344579459385));
#186186=CARTESIAN_POINT('Ctrl Pts',(2.97345013747225,31.3154282321948,-91.9606258130146));
#186187=CARTESIAN_POINT('Ctrl Pts',(2.97415449702867,31.3362801043901,-91.9859303053176));
#186188=CARTESIAN_POINT('Ctrl Pts',(2.97474456601411,31.3537485165932,-92.0071288479712));
#186189=CARTESIAN_POINT('Ctrl Pts',(2.97536733810749,31.3721953750359,-92.0277208595378));
#186190=CARTESIAN_POINT('Ctrl Pts',(2.97602129399163,31.3915791216418,-92.0476150004765));
#186191=CARTESIAN_POINT('Ctrl Pts',(2.97609144185887,31.3936583574381,-92.0497489847272));
#186192=CARTESIAN_POINT('Ctrl Pts',(2.97618040919332,31.3962956170435,-92.0524293242319));
#186193=CARTESIAN_POINT('Ctrl Pts',(2.97625004760575,31.3983599125,-92.0545074783175));
#186194=CARTESIAN_POINT('Ctrl Pts',(2.9762813755989,31.3992885699988,-92.0554423703501));
#186195=CARTESIAN_POINT('Ctrl Pts',(2.97630876917177,31.4001005898352,-92.0562560290692));
#186196=CARTESIAN_POINT('Ctrl Pts',(2.97632867593465,31.4006906176559,-92.0568461220599));
#186197=CARTESIAN_POINT('Ctrl Pts',(2.97658533779428,31.4082979638933,-92.0644543085469));
#186198=CARTESIAN_POINT('Ctrl Pts',(2.97685413045719,31.4162673444773,-92.072180195945));
#186199=CARTESIAN_POINT('Ctrl Pts',(2.97713591686397,31.4246248429328,-92.0800036140342));
#186200=CARTESIAN_POINT('Ctrl Pts',(2.97762383390965,31.4390959666555,-92.0935499702442));
#186201=CARTESIAN_POINT('Ctrl Pts',(2.97815174851592,31.45476186078,-92.107390661295));
#186202=CARTESIAN_POINT('Ctrl Pts',(2.97872268282718,31.4717153663622,-92.1213593491614));
#186203=CARTESIAN_POINT('Ctrl Pts',(2.9792693842564,31.4879492930143,-92.1347351464646));
#186204=CARTESIAN_POINT('Ctrl Pts',(2.97985554597519,31.5053642854582,-92.1482285118527));
#186205=CARTESIAN_POINT('Ctrl Pts',(2.98048308745592,31.5240210210283,-92.1616525687454));
#186206=CARTESIAN_POINT('Ctrl Pts',(2.98107284624726,31.5415544816169,-92.1742683970388));
#186207=CARTESIAN_POINT('Ctrl Pts',(2.98169916121911,31.5601849324601,-92.1868230399458));
#186208=CARTESIAN_POINT('Ctrl Pts',(2.98236279914083,31.5799391110566,-92.1991231155207));
#186209=CARTESIAN_POINT('Ctrl Pts',(2.9828721293334,31.5951000885405,-92.2085632027373));
#186210=CARTESIAN_POINT('Ctrl Pts',(2.98340343022638,31.6109225867108,-92.217852654633));
#186211=CARTESIAN_POINT('Ctrl Pts',(2.98395662917302,31.6274066594453,-92.2268868429956));
#186212=CARTESIAN_POINT('Ctrl Pts',(2.98435229799388,31.6391966920572,-92.2333484363853));
#186213=CARTESIAN_POINT('Ctrl Pts',(2.98476048602021,31.6513647799655,-92.2396977532999));
#186214=CARTESIAN_POINT('Ctrl Pts',(2.98518137990977,31.6639171754063,-92.2459029934989));
#186215=CARTESIAN_POINT('Ctrl Pts',(2.98601398420453,31.6887480855549,-92.2581780817527));
#186216=CARTESIAN_POINT('Ctrl Pts',(2.98689570726584,31.7150655813268,-92.2698795468468));
#186217=CARTESIAN_POINT('Ctrl Pts',(2.98782458083186,31.7428170652605,-92.2807176036799));
#186218=CARTESIAN_POINT('Ctrl Pts',(2.98873306176462,31.7699592888437,-92.2913177201448));
#186219=CARTESIAN_POINT('Ctrl Pts',(2.98968665019425,31.7984733669073,-92.3010917718003));
#186220=CARTESIAN_POINT('Ctrl Pts',(2.99068186466826,31.8282616120353,-92.3097564908611));
#186221=CARTESIAN_POINT('Ctrl Pts',(2.99107431360402,31.8400081906916,-92.3131733018732));
#186222=CARTESIAN_POINT('Ctrl Pts',(2.99147321684361,31.8519523538066,-92.3164174876833));
#186223=CARTESIAN_POINT('Ctrl Pts',(2.99187828661466,31.8640859130555,-92.3194712210215));
#186224=CARTESIAN_POINT('Ctrl Pts',(2.99279119518676,31.8914314002778,-92.3263534411737));
#186225=CARTESIAN_POINT('Ctrl Pts',(2.99373551476277,31.919741474585,-92.332271745838));
#186226=CARTESIAN_POINT('Ctrl Pts',(2.99471042887811,31.9489972704144,-92.3370248940461));
#186227=CARTESIAN_POINT('Ctrl Pts',(2.99563020838728,31.9765985545735,-92.3415092360585));
#186228=CARTESIAN_POINT('Ctrl Pts',(2.9965772290768,32.0050418930296,-92.3449564431487));
#186229=CARTESIAN_POINT('Ctrl Pts',(2.99754983431874,32.0342833809711,-92.3471621364646));
#186230=CARTESIAN_POINT('Ctrl Pts',(2.99834977367418,32.0583336492687,-92.3489762546837));
#186231=CARTESIAN_POINT('Ctrl Pts',(2.9991670082457,32.0829234978557,-92.34995));
#186232=CARTESIAN_POINT('Ctrl Pts',(3.,32.1080106234021,-92.34995));
#186233=CARTESIAN_POINT('Origin',(2.99219087770694,31.868484915383,-91.2979036528092));
#186234=CARTESIAN_POINT('Ctrl Pts',(3.5,31.6538440087773,-91.1386408691297));
#186235=CARTESIAN_POINT('Ctrl Pts',(3.5,31.1724436113174,-90.9136534008893));
#186236=CARTESIAN_POINT('Ctrl Pts',(2.96960200166493,31.2017108282785,-90.9273317382593));
#186237=CARTESIAN_POINT('Ctrl Pts',(3.5,36.338906312512,-81.114123180147));
#186238=CARTESIAN_POINT('Ctrl Pts',(3.50000000000001,35.8447898541155,-80.9243218897256));
#186239=CARTESIAN_POINT('Ctrl Pts',(2.97277930784816,35.8865598281193,-80.9028133775132));
#186240=CARTESIAN_POINT('Ctrl Pts',(3.5,41.0213995348936,-71.0884053145847));
#186241=CARTESIAN_POINT('Ctrl Pts',(3.49999999995192,40.5360321489106,-70.8854859061211));
#186242=CARTESIAN_POINT('Ctrl Pts',(2.97501738453455,40.5689313038002,-70.8770956617078));
#186243=CARTESIAN_POINT('Ctrl Pts',(3.5,45.7028119503364,-61.0621827299711));
#186244=CARTESIAN_POINT('Ctrl Pts',(3.5,45.2282873890496,-60.8406192095206));
#186245=CARTESIAN_POINT('Ctrl Pts',(2.97685902995381,45.2502493063675,-60.8508735991007));
#186246=CARTESIAN_POINT('',(2.97685902995381,45.2502493063675,-60.8508735991007));
#186247=CARTESIAN_POINT('Origin',(3.,45.7028119503364,-61.0621827299711));
#186248=CARTESIAN_POINT('Ctrl Pts',(2.97685902995381,45.2502493063675,-60.8508735991007));
#186249=CARTESIAN_POINT('Ctrl Pts',(2.97608222207012,43.2756646801029,-65.079944115883));
#186250=CARTESIAN_POINT('Ctrl Pts',(2.9752678572138,41.3885517362141,-69.1211703991517));
#186251=CARTESIAN_POINT('Ctrl Pts',(2.97440329692527,39.5888778999211,-72.974536173095));
#186252=CARTESIAN_POINT('Ctrl Pts',(2.97345929524181,37.6238383836545,-77.1819741342009));
#186253=CARTESIAN_POINT('Ctrl Pts',(2.97245555482809,35.7630454531903,-81.1654419117765));
#186254=CARTESIAN_POINT('Ctrl Pts',(2.97139650992555,34.0065114235406,-84.9249450806595));
#186255=CARTESIAN_POINT('Ctrl Pts',(2.97081378910475,33.0400094848007,-86.9935455404804));
#186256=CARTESIAN_POINT('Ctrl Pts',(2.97021467020169,32.1050734276472,-88.9943398821521));
#186257=CARTESIAN_POINT('Ctrl Pts',(2.96960200166741,31.2017108282783,-90.9273317382593));
#186258=CARTESIAN_POINT('Ctrl Pts',(3.5,45.7028119503364,-61.0621827299711));
#186259=CARTESIAN_POINT('Ctrl Pts',(3.50000000000001,45.2282873890497,-60.8406192095206));
#186260=CARTESIAN_POINT('Ctrl Pts',(2.97685902995381,45.2502493063675,-60.8508735991007));
#186261=CARTESIAN_POINT('Ctrl Pts',(3.5,45.7953890262578,-60.8639095446885));
#186262=CARTESIAN_POINT('Ctrl Pts',(3.49999999999858,45.287151661289,-60.7107288313437));
#186263=CARTESIAN_POINT('Ctrl Pts',(2.97532164922327,45.3120457868827,-60.7186918897092));
#186264=CARTESIAN_POINT('Ctrl Pts',(3.5,45.8435334327792,-60.6493041067215));
#186265=CARTESIAN_POINT('Ctrl Pts',(3.50000000000077,45.317377912702,-60.5716465029093));
#186266=CARTESIAN_POINT('Ctrl Pts',(2.97452770132487,45.3441826962796,-60.5756208725641));
#186267=CARTESIAN_POINT('Ctrl Pts',(3.5,45.8435334367418,-60.42825533736));
#186268=CARTESIAN_POINT('Ctrl Pts',(3.5,45.3173779148743,-60.42825533736));
#186269=CARTESIAN_POINT('Ctrl Pts',(2.97452770112504,45.3441826962898,-60.42825533736));
#186270=CARTESIAN_POINT('',(2.97452770112504,45.3441826962898,-60.42825533736));
#186271=CARTESIAN_POINT('Origin',(3.01136102441785,43.8634705376828,-60.3227888586894));
#186272=CARTESIAN_POINT('Origin',(3.,45.8435334367418,-60.42825533736));
#186273=CARTESIAN_POINT('Origin',(24.7,67.7009572055632,-55.74995));
#186274=CARTESIAN_POINT('',(24.8935146892254,-66.4063101061761,-55.2889163081141));
#186275=CARTESIAN_POINT('Ctrl Pts',(25.2,-66.3526821257161,-55.74995));
#186276=CARTESIAN_POINT('Ctrl Pts',(25.2,-66.352682125716,-55.721081183649));
#186277=CARTESIAN_POINT('Ctrl Pts',(25.1974331879958,-66.3531312596204,
-55.6919499699875));
#186278=CARTESIAN_POINT('Ctrl Pts',(25.1922799898092,-66.3540329524655,
-55.6630004684243));
#186279=CARTESIAN_POINT('Ctrl Pts',(25.1889659954452,-66.3546128263415,
-55.644383197839));
#186280=CARTESIAN_POINT('Ctrl Pts',(25.1845828022603,-66.3553797857692,
-55.6258420559621));
#186281=CARTESIAN_POINT('Ctrl Pts',(25.1791300982028,-66.3563338853502,
-55.6075053780511));
#186282=CARTESIAN_POINT('Ctrl Pts',(25.1715115231656,-66.3576669632459,
-55.5818851802329));
#186283=CARTESIAN_POINT('Ctrl Pts',(25.1618029424538,-66.3593657447479,
-55.5566554601816));
#186284=CARTESIAN_POINT('Ctrl Pts',(25.150005285251,-66.3614300672704,-55.5321823974089));
#186285=CARTESIAN_POINT('Ctrl Pts',(25.145622779736,-66.362196906371,-55.5230913269764));
#186286=CARTESIAN_POINT('Ctrl Pts',(25.1409521535631,-66.3630141600543,
-55.5141052166639));
#186287=CARTESIAN_POINT('Ctrl Pts',(25.1359942361077,-66.3638816831983,
-55.5052447720227));
#186288=CARTESIAN_POINT('Ctrl Pts',(25.1334491307288,-66.3643270189345,
-55.5006963370159));
#186289=CARTESIAN_POINT('Ctrl Pts',(25.1306700660852,-66.3648132922397,
-55.4959068094754));
#186290=CARTESIAN_POINT('Ctrl Pts',(25.1278462777817,-66.3653073850614,
-55.4912277069156));
#186291=CARTESIAN_POINT('Ctrl Pts',(25.1249297654731,-66.365817702281,-55.4863949578771));
#186292=CARTESIAN_POINT('Ctrl Pts',(25.121965606198,-66.3663363501209,-55.4816803024046));
#186293=CARTESIAN_POINT('Ctrl Pts',(25.1192114572054,-66.3668182376422,
-55.4774411221205));
#186294=CARTESIAN_POINT('Ctrl Pts',(25.1182394326667,-66.3669883106836,
-55.4759449840135));
#186295=CARTESIAN_POINT('Ctrl Pts',(25.1172939855352,-66.3671537316268,
-55.4745077921305));
#186296=CARTESIAN_POINT('Ctrl Pts',(25.1163876444297,-66.3673123079502,
-55.4731444191925));
#186297=CARTESIAN_POINT('Ctrl Pts',(25.1055064504905,-66.3692161162602,
-55.4567762711959));
#186298=CARTESIAN_POINT('Ctrl Pts',(25.0932998315912,-66.3713519177965,
-55.4405626004351));
#186299=CARTESIAN_POINT('Ctrl Pts',(25.0797034238071,-66.3737309494593,
-55.4247364723726));
#186300=CARTESIAN_POINT('Ctrl Pts',(25.0666803568155,-66.376009660808,-55.4095777091722));
#186301=CARTESIAN_POINT('Ctrl Pts',(25.0523821103081,-66.3785115442445,
-55.3947744975832));
#186302=CARTESIAN_POINT('Ctrl Pts',(25.0367814521774,-66.381241342281,-55.3805688465406));
#186303=CARTESIAN_POINT('Ctrl Pts',(25.0215171215312,-66.3839122898447,
-55.3666694486599));
#186304=CARTESIAN_POINT('Ctrl Pts',(25.0050057348895,-66.386801465097,-55.3533420190667));
#186305=CARTESIAN_POINT('Ctrl Pts',(24.9872529759462,-66.3899078520514,
-55.3408505682589));
#186306=CARTESIAN_POINT('Ctrl Pts',(24.9700316183068,-66.3929212541304,
-55.3287330296565));
#186307=CARTESIAN_POINT('Ctrl Pts',(24.9516419793518,-66.3961390786697,
-55.3174021413002));
#186308=CARTESIAN_POINT('Ctrl Pts',(24.9321210832928,-66.3995548271715,
-55.307135300076));
#186309=CARTESIAN_POINT('Ctrl Pts',(24.919703751785,-66.4017276004585,-55.3006045152886));
#186310=CARTESIAN_POINT('Ctrl Pts',(24.9068293227691,-66.403980347188,-55.2945050041632));
#186311=CARTESIAN_POINT('Ctrl Pts',(24.8935146892254,-66.4063101061761,
-55.2889163081141));
#186312=CARTESIAN_POINT('',(24.7,-66.4710859610356,-55.24995));
#186313=CARTESIAN_POINT('Ctrl Pts',(24.8935146892254,-66.4063101061761,
-55.2889163081141));
#186314=CARTESIAN_POINT('Ctrl Pts',(24.8743436827644,-66.4096645924202,
-55.2808694529217));
#186315=CARTESIAN_POINT('Ctrl Pts',(24.8548198692694,-66.4139932223095,
-55.2740625582484));
#186316=CARTESIAN_POINT('Ctrl Pts',(24.8350955380933,-66.4193328230275,
-55.2685172310238));
#186317=CARTESIAN_POINT('Ctrl Pts',(24.8153425491825,-66.4246801817201,
-55.2629638469218));
#186318=CARTESIAN_POINT('Ctrl Pts',(24.7953888759615,-66.4310416706885,
-55.2586755730986));
#186319=CARTESIAN_POINT('Ctrl Pts',(24.7753941434843,-66.4384223361908,
-55.2556332240216));
#186320=CARTESIAN_POINT('Ctrl Pts',(24.7553495325246,-66.445821413362,-55.252583285558));
#186321=CARTESIAN_POINT('Ctrl Pts',(24.7352640798756,-66.4542449394322,
-55.2507853224051));
#186322=CARTESIAN_POINT('Ctrl Pts',(24.7152989762785,-66.4636628855439,
-55.2501811880231));
#186323=CARTESIAN_POINT('Ctrl Pts',(24.7101905706034,-66.4660726245733,
-55.2500266101373));
#186324=CARTESIAN_POINT('Ctrl Pts',(24.7050900275942,-66.4685472800516,
-55.24995));
#186325=CARTESIAN_POINT('Ctrl Pts',(24.7,-66.4710859610356,-55.24995));
#186326=CARTESIAN_POINT('',(24.7,-73.08000002,-55.24995));
#186327=CARTESIAN_POINT('Origin',(41.5,-73.08000002,-55.24995));
#186328=CARTESIAN_POINT('',(24.2743783673579,-66.6190816475223,-55.24995));
#186329=CARTESIAN_POINT('Origin',(25.30491873532,-68.8967968514054,-55.24995));
#186330=CARTESIAN_POINT('Origin',(0.,-12.9675000200281,-55.24995));
#186331=CARTESIAN_POINT('Origin',(0.,-12.9675000200281,-60.64995));
#186332=CARTESIAN_POINT('',(43.0192624284939,-63.3317132462777,-60.64995));
#186333=CARTESIAN_POINT('',(4.6996065532056,-66.6842487255793,-60.64995));
#186334=CARTESIAN_POINT('',(50.3642132262497,-55.9867624485218,-60.64995));
#186335=CARTESIAN_POINT('',(53.7167487055513,-17.6671065732338,-60.64995));
#186336=CARTESIAN_POINT('',(49.7860373924393,-57.2266645253997,-60.64995));
#186337=CARTESIAN_POINT('Origin',(48.3718238300662,-55.8124509630266,-60.64995));
#186338=CARTESIAN_POINT('',(44.2591645053717,-62.7535374124673,-60.64995));
#186339=CARTESIAN_POINT('',(47.0226009489055,-59.9901009689335,-60.64995));
#186340=CARTESIAN_POINT('Origin',(42.8449509429986,-61.3393238500942,-60.64995));
#186341=CARTESIAN_POINT('Origin',(0.,-12.9675000200281,-60.64995));
#186342=CARTESIAN_POINT('',(50.3642132262496,30.0517624084658,-60.64995));
#186343=CARTESIAN_POINT('',(53.7167487055517,-8.26789346682159,-60.64995));
#186344=CARTESIAN_POINT('',(43.019262428494,37.3967132062212,-60.64995));
#186345=CARTESIAN_POINT('',(4.69960655320655,40.7492486855235,-60.64995));
#186346=CARTESIAN_POINT('',(44.2591645053719,36.8185373724109,-60.64995));
#186347=CARTESIAN_POINT('Origin',(42.8449509429988,35.4043238100378,-60.64995));
#186348=CARTESIAN_POINT('',(49.7860373924392,31.2916644853436,-60.64995));
#186349=CARTESIAN_POINT('',(47.0226009489055,34.0551009288773,-60.64995));
#186350=CARTESIAN_POINT('Origin',(48.3718238300661,29.8774509229704,-60.64995));
#186351=CARTESIAN_POINT('Origin',(53.7167487055513,-17.6671065732338,-59.64995));
#186352=CARTESIAN_POINT('',(52.6206164493,-41.6696688386047,-59.64995));
#186353=CARTESIAN_POINT('',(52.9858497431864,-37.4950331867729,-59.64995));
#186354=CARTESIAN_POINT('Origin',(51.6244217512083,-41.5825130958571,-59.64995));
#186355=CARTESIAN_POINT('Origin',(52.8810286821225,-44.43000002,-52.64995));
#186356=CARTESIAN_POINT('',(52.3810286821225,-44.43000002,-55.74995));
#186357=CARTESIAN_POINT('Origin',(52.8810286821225,-44.43000002,-55.74995));
#186358=CARTESIAN_POINT('',(52.3829313330767,-44.3864221486262,-55.74995));
#186359=CARTESIAN_POINT('',(52.3829313330767,-44.3864221486262,-52.64995));
#186360=CARTESIAN_POINT('Origin',(52.8810286821225,-44.43000002,-55.74995));
#186361=CARTESIAN_POINT('Ctrl Pts',(52.8810286821225,-44.93000002,-55.74995));
#186362=CARTESIAN_POINT('Ctrl Pts',(52.3353744315879,-44.93000002,-55.74995));
#186363=CARTESIAN_POINT('Ctrl Pts',(52.3829313330767,-44.3864221486262,
-55.74995));
#186364=CARTESIAN_POINT('Ctrl Pts',(52.8810286821171,-44.93000002,-55.6186826543063));
#186365=CARTESIAN_POINT('Ctrl Pts',(52.3353744315888,-44.9300000200045,
-55.6317784220498));
#186366=CARTESIAN_POINT('Ctrl Pts',(52.3829313330709,-44.3864221486917,
-55.4874153086129));
#186367=CARTESIAN_POINT('Ctrl Pts',(52.8715997552662,-44.9838865835627,
-55.4889566552507));
#186368=CARTESIAN_POINT('Ctrl Pts',(52.3317239990966,-44.9717246542945,
-55.5133819370972));
#186369=CARTESIAN_POINT('Ctrl Pts',(52.3735024062205,-44.4941952757516,
-55.2279633105015));
#186370=CARTESIAN_POINT('Ctrl Pts',(52.8392079364393,-45.1690066752507,
-55.3038365635627));
#186371=CARTESIAN_POINT('Ctrl Pts',(52.317584547802,-45.1333393221421,-55.3274496218433));
#186372=CARTESIAN_POINT('Ctrl Pts',(52.3411105873933,-44.8644354591276,
-54.8577231271254));
#186373=CARTESIAN_POINT('Ctrl Pts',(52.8165088278734,-45.2987326743059,
-55.24995));
#186374=CARTESIAN_POINT('Ctrl Pts',(52.3071965192496,-45.252075031829,-55.2615708605687));
#186375=CARTESIAN_POINT('Ctrl Pts',(52.3184114788294,-45.1238874572391,
-54.7499500000658));
#186376=CARTESIAN_POINT('Ctrl Pts',(52.7935400185966,-45.43000002,-55.24995));
#186377=CARTESIAN_POINT('Ctrl Pts',(52.2954426695507,-45.3864221486261,
-55.2499499999999));
#186378=CARTESIAN_POINT('Ctrl Pts',(52.2954426695508,-45.3864221486262,
-54.74995));
#186379=CARTESIAN_POINT('',(52.2954426695508,-45.3864221486261,-54.74995));
#186380=CARTESIAN_POINT('Origin',(52.7935400185966,-45.43000002,-54.74995));
#186381=CARTESIAN_POINT('Ctrl Pts',(52.2954426695508,-45.3864221486261,
-54.74995));
#186382=CARTESIAN_POINT('Ctrl Pts',(52.3184114788294,-45.123887457239,-54.7499500000658));
#186383=CARTESIAN_POINT('Ctrl Pts',(52.3411105873933,-44.8644354591276,
-54.8577231271254));
#186384=CARTESIAN_POINT('Ctrl Pts',(52.3573064968069,-44.6793153674396,
-55.0428432188135));
#186385=CARTESIAN_POINT('Ctrl Pts',(52.3735024062205,-44.4941952757516,
-55.2279633105015));
#186386=CARTESIAN_POINT('Ctrl Pts',(52.3829313330709,-44.3864221486917,
-55.4874153086129));
#186387=CARTESIAN_POINT('Ctrl Pts',(52.3829313330767,-44.3864221486262,
-55.74995));
#186388=CARTESIAN_POINT('Origin',(53.4839470922323,-37.5386110581466,-54.74995));
#186389=CARTESIAN_POINT('',(52.2516983377878,-45.8864221486262,-54.74995));
#186390=CARTESIAN_POINT('Origin',(52.7497956868337,-45.93000002,-54.74995));
#186391=CARTESIAN_POINT('',(52.9858497431864,-37.4950331867729,-54.74995));
#186392=CARTESIAN_POINT('Ctrl Pts',(52.7497956868337,-45.93000002,-55.24995));
#186393=CARTESIAN_POINT('Ctrl Pts',(52.2516983377878,-45.8864221486262,
-55.24995));
#186394=CARTESIAN_POINT('Ctrl Pts',(52.2516983377878,-45.8864221486262,
-54.74995));
#186395=CARTESIAN_POINT('Ctrl Pts',(52.7268268775569,-46.0612673656941,
-55.24995));
#186396=CARTESIAN_POINT('Ctrl Pts',(52.2402778440398,-46.0169589895406,
-55.2386587236919));
#186397=CARTESIAN_POINT('Ctrl Pts',(52.2287295285091,-46.1489568400132,
-54.7499500000658));
#186398=CARTESIAN_POINT('Ctrl Pts',(52.704127768991,-46.1909933647493,-55.3038365635627));
#186399=CARTESIAN_POINT('Ctrl Pts',(52.227884321682,-46.1586175982532,-55.2822894538777));
#186400=CARTESIAN_POINT('Ctrl Pts',(52.2060304199453,-46.4084088381247,
-54.8577231271255));
#186401=CARTESIAN_POINT('Ctrl Pts',(52.6717359501641,-46.3761134564373,
-55.4889566552507));
#186402=CARTESIAN_POINT('Ctrl Pts',(52.2097524154255,-46.3658662351156,
-55.4680441063688));
#186403=CARTESIAN_POINT('Ctrl Pts',(52.1736386011181,-46.7786490215007,
-55.2279633105015));
#186404=CARTESIAN_POINT('Ctrl Pts',(52.6623070233132,-46.43000002,-55.6186826543062));
#186405=CARTESIAN_POINT('Ctrl Pts',(52.2041414362981,-46.4300000199443,
-55.6078478088784));
#186406=CARTESIAN_POINT('Ctrl Pts',(52.1642096742676,-46.8864221485606,
-55.487415308613));
#186407=CARTESIAN_POINT('Ctrl Pts',(52.6623070233078,-46.43000002,-55.74995));
#186408=CARTESIAN_POINT('Ctrl Pts',(52.2041414362991,-46.43000002,-55.74995));
#186409=CARTESIAN_POINT('Ctrl Pts',(52.1642096742619,-46.8864221486262,
-55.74995));
#186410=CARTESIAN_POINT('',(52.1642096742619,-46.8864221486262,-55.74995));
#186411=CARTESIAN_POINT('Origin',(52.6623070233078,-46.93000002,-55.74995));
#186412=CARTESIAN_POINT('Ctrl Pts',(52.1642096742619,-46.8864221486262,
-55.74995));
#186413=CARTESIAN_POINT('Ctrl Pts',(52.1642096742676,-46.8864221485606,
-55.487415308613));
#186414=CARTESIAN_POINT('Ctrl Pts',(52.1736386011181,-46.7786490215007,
-55.2279633105015));
#186415=CARTESIAN_POINT('Ctrl Pts',(52.1898345105317,-46.5935289298127,
-55.0428432188135));
#186416=CARTESIAN_POINT('Ctrl Pts',(52.2060304199453,-46.4084088381247,
-54.8577231271255));
#186417=CARTESIAN_POINT('Ctrl Pts',(52.2287295285091,-46.1489568400132,
-54.7499500000658));
#186418=CARTESIAN_POINT('Ctrl Pts',(52.2516983377878,-45.8864221486262,
-54.74995));
#186419=CARTESIAN_POINT('Origin',(52.6623070233078,-46.93000002,-52.64995));
#186420=CARTESIAN_POINT('',(52.1642096742619,-46.8864221486262,-52.64995));
#186421=CARTESIAN_POINT('Origin',(53.7167487055513,-17.6671065732338,-59.64995));
#186422=CARTESIAN_POINT('',(52.9858497431864,-37.4950331867729,-59.64995));
#186423=CARTESIAN_POINT('Origin',(52.1679960743864,-52.58000002,-55.2499500000008));
#186424=CARTESIAN_POINT('',(51.6698987253405,-52.5364221486262,-55.74995));
#186425=CARTESIAN_POINT('Origin',(52.1679960743864,-52.58000002,-55.74995));
#186426=CARTESIAN_POINT('',(51.6698987253405,-52.5364221486262,-52.64995));
#186427=CARTESIAN_POINT('Ctrl Pts',(52.1679960743864,-53.08000002,-55.74995));
#186428=CARTESIAN_POINT('Ctrl Pts',(51.6223418238518,-53.08000002,-55.74995));
#186429=CARTESIAN_POINT('Ctrl Pts',(51.6698987253405,-52.5364221486262,
-55.74995));
#186430=CARTESIAN_POINT('Ctrl Pts',(52.1679960743809,-53.08000002,-55.6186826543066));
#186431=CARTESIAN_POINT('Ctrl Pts',(51.6223418238527,-53.0800000200045,
-55.6317784220505));
#186432=CARTESIAN_POINT('Ctrl Pts',(51.6698987253348,-52.5364221486917,
-55.4874153086129));
#186433=CARTESIAN_POINT('Ctrl Pts',(52.1585671475301,-53.1338865835632,
-55.4889566552503));
#186434=CARTESIAN_POINT('Ctrl Pts',(51.6186913913614,-53.1217246542964,
-55.5133819370962));
#186435=CARTESIAN_POINT('Ctrl Pts',(51.6604697984843,-52.6441952757516,
-55.2279633105015));
#186436=CARTESIAN_POINT('Ctrl Pts',(52.1261753287031,-53.3190066752503,
-55.3038365635632));
#186437=CARTESIAN_POINT('Ctrl Pts',(51.6045519400649,-53.2833393221403,
-55.327449621844));
#186438=CARTESIAN_POINT('Ctrl Pts',(51.6280779796571,-53.0144354591276,
-54.8577231271254));
#186439=CARTESIAN_POINT('Ctrl Pts',(52.1034762201372,-53.4487326743062,
-55.24995));
#186440=CARTESIAN_POINT('Ctrl Pts',(51.5941639115132,-53.4020750318305,
-55.2615708605685));
#186441=CARTESIAN_POINT('Ctrl Pts',(51.6053788710933,-53.2738874572391,
-54.7499500000658));
#186442=CARTESIAN_POINT('Ctrl Pts',(52.0805074108605,-53.58000002,-55.24995));
#186443=CARTESIAN_POINT('Ctrl Pts',(51.5824100618146,-53.5364221486261,
-55.2499499999999));
#186444=CARTESIAN_POINT('Ctrl Pts',(51.5824100618146,-53.5364221486262,
-54.74995));
#186445=CARTESIAN_POINT('',(51.5824100618146,-53.5364221486262,-54.74995));
#186446=CARTESIAN_POINT('Origin',(52.0805074108605,-53.58000002,-54.74995));
#186447=CARTESIAN_POINT('Ctrl Pts',(51.5824100618146,-53.5364221486262,
-54.74995));
#186448=CARTESIAN_POINT('Ctrl Pts',(51.6053788710933,-53.2738874572391,
-54.7499500000658));
#186449=CARTESIAN_POINT('Ctrl Pts',(51.6280779796571,-53.0144354591276,
-54.8577231271254));
#186450=CARTESIAN_POINT('Ctrl Pts',(51.6442738890707,-52.8293153674396,
-55.0428432188135));
#186451=CARTESIAN_POINT('Ctrl Pts',(51.6604697984843,-52.6441952757516,
-55.2279633105015));
#186452=CARTESIAN_POINT('Ctrl Pts',(51.6698987253348,-52.5364221486917,
-55.4874153086129));
#186453=CARTESIAN_POINT('Ctrl Pts',(51.6698987253405,-52.5364221486262,
-55.74995));
#186454=CARTESIAN_POINT('Origin',(53.4839470922323,-37.5386110581466,-54.74995));
#186455=CARTESIAN_POINT('',(51.5386657300517,-54.0364221486261,-54.74995));
#186456=CARTESIAN_POINT('Origin',(52.0367630790975,-54.08000002,-54.74995));
#186457=CARTESIAN_POINT('',(52.9858497431864,-37.4950331867729,-54.74995));
#186458=CARTESIAN_POINT('Ctrl Pts',(52.0367630790975,-54.08000002,-55.24995));
#186459=CARTESIAN_POINT('Ctrl Pts',(51.5386657300516,-54.0364221486262,
-55.24995));
#186460=CARTESIAN_POINT('Ctrl Pts',(51.5386657300517,-54.0364221486262,
-54.74995));
#186461=CARTESIAN_POINT('Ctrl Pts',(52.0137942698207,-54.2112673656937,
-55.24995));
#186462=CARTESIAN_POINT('Ctrl Pts',(51.5272452363036,-54.1669589895393,
-55.2386587236848));
#186463=CARTESIAN_POINT('Ctrl Pts',(51.5156969207731,-54.2989568400126,
-54.7499500000658));
#186464=CARTESIAN_POINT('Ctrl Pts',(51.9910951612549,-54.3409933647497,
-55.3038365635632));
#186465=CARTESIAN_POINT('Ctrl Pts',(51.5148517139458,-54.308617598254,-55.2822894538766));
#186466=CARTESIAN_POINT('Ctrl Pts',(51.4929978122091,-54.5584088381255,
-54.8577231271254));
#186467=CARTESIAN_POINT('Ctrl Pts',(51.958703342428,-54.5261134564368,-55.4889566552503));
#186468=CARTESIAN_POINT('Ctrl Pts',(51.4967198076894,-54.5158662351146,
-55.4680441063697));
#186469=CARTESIAN_POINT('Ctrl Pts',(51.460605993382,-54.9286490214999,-55.2279633105015));
#186470=CARTESIAN_POINT('Ctrl Pts',(51.9492744155771,-54.58000002,-55.6186826543065));
#186471=CARTESIAN_POINT('Ctrl Pts',(51.491108828562,-54.5800000199489,-55.6078478088776));
#186472=CARTESIAN_POINT('Ctrl Pts',(51.4511770665315,-55.0364221485606,
-55.4874153086129));
#186473=CARTESIAN_POINT('Ctrl Pts',(51.9492744155716,-54.58000002,-55.74995));
#186474=CARTESIAN_POINT('Ctrl Pts',(51.491108828563,-54.58000002,-55.74995));
#186475=CARTESIAN_POINT('Ctrl Pts',(51.4511770665258,-55.0364221486262,
-55.74995));
#186476=CARTESIAN_POINT('',(51.4511770665258,-55.0364221486262,-55.74995));
#186477=CARTESIAN_POINT('Origin',(51.9492744155716,-55.08000002,-55.74995));
#186478=CARTESIAN_POINT('Ctrl Pts',(51.4511770665258,-55.0364221486262,
-55.74995));
#186479=CARTESIAN_POINT('Ctrl Pts',(51.4511770665315,-55.0364221485606,
-55.4874153086129));
#186480=CARTESIAN_POINT('Ctrl Pts',(51.460605993382,-54.9286490214999,-55.2279633105015));
#186481=CARTESIAN_POINT('Ctrl Pts',(51.4768019027956,-54.7435289298127,
-55.0428432188135));
#186482=CARTESIAN_POINT('Ctrl Pts',(51.4929978122091,-54.5584088381255,
-54.8577231271254));
#186483=CARTESIAN_POINT('Ctrl Pts',(51.5156969207731,-54.2989568400126,
-54.7499500000658));
#186484=CARTESIAN_POINT('Ctrl Pts',(51.5386657300517,-54.0364221486262,
-54.74995));
#186485=CARTESIAN_POINT('Origin',(51.9492744155716,-55.08000002,-52.64995));
#186486=CARTESIAN_POINT('',(51.4511770665258,-55.0364221486262,-52.64995));
#186487=CARTESIAN_POINT('Origin',(53.7167487055513,-17.6671065732338,-59.64995));
#186488=CARTESIAN_POINT('',(51.3604079243415,-56.0739181912695,-59.64995));
#186489=CARTESIAN_POINT('',(52.9858497431864,-37.4950331867729,-59.64995));
#186490=CARTESIAN_POINT('Origin',(50.3642132262497,-55.9867624485218,-59.64995));
#186491=CARTESIAN_POINT('Ctrl Pts',(53.4093483797613,-38.0856391317044,
-55.3542421110299));
#186492=CARTESIAN_POINT('Ctrl Pts',(52.9364314216307,-38.0597244105783,
-55.3342259538136));
#186493=CARTESIAN_POINT('Ctrl Pts',(52.9112502355242,-38.3477094636814,
-54.9585223635782));
#186494=CARTESIAN_POINT('Ctrl Pts',(53.3880736387225,-38.2072248331335,
-55.448153047952));
#186495=CARTESIAN_POINT('Ctrl Pts',(52.9247563553463,-38.1931762538392,
-55.4246794702588));
#186496=CARTESIAN_POINT('Ctrl Pts',(52.889976625843,-38.5908679349475,-55.1463344612842));
#186497=CARTESIAN_POINT('Ctrl Pts',(53.375339024416,-38.2800034869308,-55.5963379967406));
#186498=CARTESIAN_POINT('Ctrl Pts',(52.9171601694683,-38.2800041317283,
-55.5832548498195));
#186499=CARTESIAN_POINT('Ctrl Pts',(52.87724039479,-38.7364437219894,-55.4427310705271));
#186500=CARTESIAN_POINT('Ctrl Pts',(53.3753396310656,-38.2800000198762,
-55.7499609770277));
#186501=CARTESIAN_POINT('Ctrl Pts',(52.9171605282557,-38.2800000198531,
-55.7499619127669));
#186502=CARTESIAN_POINT('Ctrl Pts',(52.8772410016055,-38.736436786057,-55.7499719536926));
#186503=CARTESIAN_POINT('',(52.9112495105562,-38.347717747534,-54.9585476429427));
#186504=CARTESIAN_POINT('Origin',(53.4093468596021,-38.3912956189078,-54.9585476429427));
#186505=CARTESIAN_POINT('',(52.877242281998,-38.7364221486262,-55.74995));
#186506=CARTESIAN_POINT('Origin',(52.954126623731,-37.8576301013555,-55.6904184160469));
#186507=CARTESIAN_POINT('Origin',(53.3753396310439,-38.78000002,-55.74995));
#186508=CARTESIAN_POINT('Origin',(53.3753396310439,-38.78000002,-55.2499500000007));
#186509=CARTESIAN_POINT('',(52.877242281998,-38.7364221486262,-52.64995));
#186510=CARTESIAN_POINT('Ctrl Pts',(52.903095448475,-38.4409191036023,-60.08258062683));
#186511=CARTESIAN_POINT('Ctrl Pts',(52.8907789702838,-38.5816970935142,
-60.5786901973488));
#186512=CARTESIAN_POINT('Ctrl Pts',(52.4648996019023,-38.6266655296175,
-60.866265313415));
#186513=CARTESIAN_POINT('Ctrl Pts',(52.8569709369232,-38.9681246830787,
-59.9318336272105));
#186514=CARTESIAN_POINT('Ctrl Pts',(52.8442212423788,-39.1138543585791,
-60.5019204415683));
#186515=CARTESIAN_POINT('Ctrl Pts',(52.3309754745585,-39.1170130132287,
-60.7908684306025));
#186516=CARTESIAN_POINT('Ctrl Pts',(52.8102637225239,-39.5019905865797,
-59.8278758615346));
#186517=CARTESIAN_POINT('Ctrl Pts',(52.7984570004479,-39.6369420374376,
-60.4756484953684));
#186518=CARTESIAN_POINT('Ctrl Pts',(52.1936254351686,-39.6095793654924,
-60.7389129305601));
#186519=CARTESIAN_POINT('Ctrl Pts',(52.7160699755127,-40.5786300415107,
-59.6865014144928));
#186520=CARTESIAN_POINT('Ctrl Pts',(52.7078841622538,-40.6721943151964,
-60.4973085875933));
#186521=CARTESIAN_POINT('Ctrl Pts',(51.9132529272684,-40.5953951229239,
-60.6682257074536));
#186522=CARTESIAN_POINT('Ctrl Pts',(52.6685584273161,-41.1216895223836,
-59.6499500020974));
#186523=CARTESIAN_POINT('Ctrl Pts',(52.662477767809,-41.1911917785403,-60.5526719649898));
#186524=CARTESIAN_POINT('Ctrl Pts',(51.7702028983306,-41.0887654988916,
-60.64995));
#186525=CARTESIAN_POINT('Ctrl Pts',(52.6206164493,-41.6696688386047,-59.64995));
#186526=CARTESIAN_POINT('Ctrl Pts',(52.6206164493,-41.6696688386047,-60.64995));
#186527=CARTESIAN_POINT('Ctrl Pts',(51.6244217512083,-41.5825130958571,
-60.64995));
#186528=CARTESIAN_POINT('Ctrl Pts',(52.6206164493,-41.6696688386047,-59.64995));
#186529=CARTESIAN_POINT('Ctrl Pts',(52.647177193844,-41.3660781392669,-59.649950001162));
#186530=CARTESIAN_POINT('Ctrl Pts',(52.6736027803761,-41.0640322847493,
-59.6612277190034));
#186531=CARTESIAN_POINT('Ctrl Pts',(52.6998985433583,-40.763470321929,-59.6832689389187));
#186532=CARTESIAN_POINT('Ctrl Pts',(52.7166476389893,-40.5720272722755,
-59.6973081018224));
#186533=CARTESIAN_POINT('Ctrl Pts',(52.7333441220441,-40.3811856094009,
-59.7157148983376));
#186534=CARTESIAN_POINT('Ctrl Pts',(52.7499897489645,-40.1909252438875,
-59.7383666003327));
#186535=CARTESIAN_POINT('Ctrl Pts',(52.7543856861046,-40.1406794579502,
-59.7443486795034));
#186536=CARTESIAN_POINT('Ctrl Pts',(52.7587779570344,-40.0904755740926,
-59.7506312543479));
#186537=CARTESIAN_POINT('Ctrl Pts',(52.7631665715902,-40.0403134816151,
-59.7572129455377));
#186538=CARTESIAN_POINT('Ctrl Pts',(52.7801318002604,-39.8464000361233,
-59.7826560311971));
#186539=CARTESIAN_POINT('Ctrl Pts',(52.7970456659898,-39.6530737072156,
-59.8124579292866));
#186540=CARTESIAN_POINT('Ctrl Pts',(52.8138987094321,-39.4604424150672,
-59.8472750881764));
#186541=CARTESIAN_POINT('Ctrl Pts',(52.8286848633259,-39.2914357937869,
-59.877822203969));
#186542=CARTESIAN_POINT('Ctrl Pts',(52.8434252414643,-39.1229522134604,
-59.9121898106578));
#186543=CARTESIAN_POINT('Ctrl Pts',(52.8581158408277,-38.9550379662969,
-59.9506823384307));
#186544=CARTESIAN_POINT('Ctrl Pts',(52.8645007938109,-38.882057651007,-59.9674122875603));
#186545=CARTESIAN_POINT('Ctrl Pts',(52.8708763604388,-38.8091846968994,
-59.9849220508816));
#186546=CARTESIAN_POINT('Ctrl Pts',(52.877242268511,-38.7364221474456,-60.003239652154));
#186547=CARTESIAN_POINT('Origin',(52.6819919725962,20.76999998,-52.64995));
#186548=CARTESIAN_POINT('',(52.1838946235503,20.7264221086262,-55.74995));
#186549=CARTESIAN_POINT('',(52.1838946235503,20.7264221086262,-52.64995));
#186550=CARTESIAN_POINT('Origin',(52.6819919725962,20.76999998,-55.74995));
#186551=CARTESIAN_POINT('Ctrl Pts',(52.6819919725962,20.26999998,-55.74995));
#186552=CARTESIAN_POINT('Ctrl Pts',(52.2238263855875,20.26999998,-55.74995));
#186553=CARTESIAN_POINT('Ctrl Pts',(52.1838946235503,20.7264221086262,-55.74995));
#186554=CARTESIAN_POINT('Ctrl Pts',(52.6819919726017,20.26999998,-55.6186826543063));
#186555=CARTESIAN_POINT('Ctrl Pts',(52.2238263855902,20.2699999799516,-55.6078478088784));
#186556=CARTESIAN_POINT('Ctrl Pts',(52.1838946235561,20.7264221085606,-55.487415308613));
#186557=CARTESIAN_POINT('Ctrl Pts',(52.6914208994525,20.2161134164373,-55.4889566552507));
#186558=CARTESIAN_POINT('Ctrl Pts',(52.229437364714,20.2058661951152,-55.4680441063689));
#186559=CARTESIAN_POINT('Ctrl Pts',(52.1933235504066,20.6186489815003,-55.2279633105015));
#186560=CARTESIAN_POINT('Ctrl Pts',(52.7238127182794,20.0309933247493,-55.3038365635627));
#186561=CARTESIAN_POINT('Ctrl Pts',(52.2475692709704,19.9986175582537,-55.2822894538776));
#186562=CARTESIAN_POINT('Ctrl Pts',(52.2257153692336,20.2484087981252,-54.8577231271255));
#186563=CARTESIAN_POINT('Ctrl Pts',(52.746511826845,19.901267325694,-55.24995));
#186564=CARTESIAN_POINT('Ctrl Pts',(52.2599627933277,19.8569589495402,-55.2386587236914));
#186565=CARTESIAN_POINT('Ctrl Pts',(52.2484144777976,19.9889568000129,-54.7499500000658));
#186566=CARTESIAN_POINT('Ctrl Pts',(52.7694806361221,19.76999998,-55.24995));
#186567=CARTESIAN_POINT('Ctrl Pts',(52.2713832870762,19.7264221086262,-55.2499499999999));
#186568=CARTESIAN_POINT('Ctrl Pts',(52.2713832870762,19.7264221086262,-54.74995));
#186569=CARTESIAN_POINT('',(52.2713832870762,19.7264221086262,-54.74995));
#186570=CARTESIAN_POINT('Origin',(52.7694806361221,19.76999998,-54.74995));
#186571=CARTESIAN_POINT('Ctrl Pts',(52.2713832870762,19.7264221086262,-54.74995));
#186572=CARTESIAN_POINT('Ctrl Pts',(52.2484144777976,19.9889568000129,-54.7499500000658));
#186573=CARTESIAN_POINT('Ctrl Pts',(52.2257153692336,20.2484087981252,-54.8577231271255));
#186574=CARTESIAN_POINT('Ctrl Pts',(52.2095194598201,20.4335288898127,-55.0428432188135));
#186575=CARTESIAN_POINT('Ctrl Pts',(52.1933235504066,20.6186489815003,-55.2279633105015));
#186576=CARTESIAN_POINT('Ctrl Pts',(52.1838946235561,20.7264221085606,-55.487415308613));
#186577=CARTESIAN_POINT('Ctrl Pts',(52.1838946235503,20.7264221086262,-55.74995));
#186578=CARTESIAN_POINT('Origin',(51.7633389850707,31.2702516755049,-54.74995));
#186579=CARTESIAN_POINT('',(52.3151276188392,19.2264221086262,-54.74995));
#186580=CARTESIAN_POINT('Origin',(52.8132249678851,19.26999998,-54.74995));
#186581=CARTESIAN_POINT('',(51.2652416360248,31.226673804131,-54.74995));
#186582=CARTESIAN_POINT('Ctrl Pts',(52.8132511574963,19.2700238915803,-55.2499499996828));
#186583=CARTESIAN_POINT('Ctrl Pts',(52.3151257340121,19.2264436522985,-55.2499781675605));
#186584=CARTESIAN_POINT('Ctrl Pts',(52.3151238928183,19.2264646972402,-54.7499500009454));
#186585=CARTESIAN_POINT('Ctrl Pts',(52.8362215618991,19.1387494339943,-55.2499434816102));
#186586=CARTESIAN_POINT('Ctrl Pts',(52.3268796769205,19.0920954701104,-55.26159490362));
#186587=CARTESIAN_POINT('Ctrl Pts',(52.3380939732538,18.9639154764634,-54.7499383449302));
#186588=CARTESIAN_POINT('Ctrl Pts',(52.8589226187611,19.0090137328179,-55.3038301720458));
#186589=CARTESIAN_POINT('Ctrl Pts',(52.3372676751065,18.9733601075009,-55.3274735569165));
#186590=CARTESIAN_POINT('Ctrl Pts',(52.3607946609107,18.7044454292369,-54.8577131170158));
#186591=CARTESIAN_POINT('Ctrl Pts',(52.8913167201329,18.823882239107,-55.4889602509492));
#186592=CARTESIAN_POINT('Ctrl Pts',(52.3514067244284,18.8117500342473,-55.5134049012176));
#186593=CARTESIAN_POINT('Ctrl Pts',(52.39318823128,18.3341852256424,-55.2279733206111));
#186594=CARTESIAN_POINT('Ctrl Pts',(52.9007459593775,18.7699941513777,-55.6186959323247));
#186595=CARTESIAN_POINT('Ctrl Pts',(52.3550567877969,18.7700296190381,-55.6318003689065));
#186596=CARTESIAN_POINT('Ctrl Pts',(52.4026173020516,18.2264104535562,-55.4874433678369));
#186597=CARTESIAN_POINT('Ctrl Pts',(52.9007449425538,18.7699999794923,-55.7499712944291));
#186598=CARTESIAN_POINT('Ctrl Pts',(52.3550563912364,18.770034151741,-55.7499691665881));
#186599=CARTESIAN_POINT('Ctrl Pts',(52.4026162822824,18.2264221095716,-55.749992588614));
#186600=CARTESIAN_POINT('',(52.4026162823651,18.2264221086262,-55.74995));
#186601=CARTESIAN_POINT('Origin',(52.900713631411,18.26999998,-55.74995));
#186602=CARTESIAN_POINT('Ctrl Pts',(52.4026162823651,18.2264221086262,-55.74995));
#186603=CARTESIAN_POINT('Ctrl Pts',(52.4026162823594,18.2264221086918,-55.4874153086129));
#186604=CARTESIAN_POINT('Ctrl Pts',(52.3931873555089,18.334195235752,-55.2279633105015));
#186605=CARTESIAN_POINT('Ctrl Pts',(52.3769914460954,18.5193153274396,-55.0428432188135));
#186606=CARTESIAN_POINT('Ctrl Pts',(52.3607955366818,18.7044354191273,-54.8577231271254));
#186607=CARTESIAN_POINT('Ctrl Pts',(52.3380964281178,18.9638874172394,-54.7499500000658));
#186608=CARTESIAN_POINT('Ctrl Pts',(52.3151276188392,19.2264221086262,-54.74995));
#186609=CARTESIAN_POINT('Origin',(52.900713631411,18.26999998,-52.64995));
#186610=CARTESIAN_POINT('',(52.4026162823651,18.2264221086262,-52.64995));
#186611=CARTESIAN_POINT('Origin',(53.7167487055517,-8.26789346682159,-59.64995));
#186612=CARTESIAN_POINT('',(52.6206164493001,15.7346687985483,-59.64995));
#186613=CARTESIAN_POINT('',(51.2652416360248,31.226673804131,-59.64995));
#186614=CARTESIAN_POINT('Origin',(51.6244217512084,15.6475130558006,-59.64995));
#186615=CARTESIAN_POINT('Ctrl Pts',(52.6206164493001,15.7346687985483,-59.64995));
#186616=CARTESIAN_POINT('Ctrl Pts',(52.6206164493002,15.7346687985482,-60.64995));
#186617=CARTESIAN_POINT('Ctrl Pts',(51.6244217512084,15.6475130558006,-60.64995));
#186618=CARTESIAN_POINT('Ctrl Pts',(52.6699713539896,15.1705396565499,-59.6499500021592));
#186619=CARTESIAN_POINT('Ctrl Pts',(52.6636514122595,15.2427769209991,-60.5499446302911));
#186620=CARTESIAN_POINT('Ctrl Pts',(51.7744992817202,15.1392139958173,-60.64995));
#186621=CARTESIAN_POINT('Ctrl Pts',(52.7188714030742,14.6116095379051,-59.6886254732604));
#186622=CARTESIAN_POINT('Ctrl Pts',(52.7104450878319,14.7079227618566,-60.4941916839025));
#186623=CARTESIAN_POINT('Ctrl Pts',(51.921686259274,14.6313008059217,-60.6692877368673));
#186624=CARTESIAN_POINT('Ctrl Pts',(52.8157906892286,13.5038170280144,-59.8384384618772));
#186625=CARTESIAN_POINT('Ctrl Pts',(52.8037229951722,13.64175140224,-60.4769182500017));
#186626=CARTESIAN_POINT('Ctrl Pts',(52.209973495227,13.6164898397673,-60.7441942307015));
#186627=CARTESIAN_POINT('Ctrl Pts',(52.8638414531199,12.954594283549,-59.9484723594913));
#186628=CARTESIAN_POINT('Ctrl Pts',(52.850859560631,13.1029779936029,-60.5072438893719));
#186629=CARTESIAN_POINT('Ctrl Pts',(52.3511088881553,13.109439201609,-60.799180633384));
#186630=CARTESIAN_POINT('Ctrl Pts',(52.9112495105564,12.4127177074772,-60.1097730249189));
#186631=CARTESIAN_POINT('Ctrl Pts',(52.8987763848902,12.5552861862208,-60.5923862926586));
#186632=CARTESIAN_POINT('Ctrl Pts',(52.4885489491165,12.6049688303995,-60.8798615124595));
#186633=CARTESIAN_POINT('Ctrl Pts',(52.8969272285826,12.5764221083876,-60.0627241236307));
#186634=CARTESIAN_POINT('Ctrl Pts',(52.8810850690579,12.757498700804,-60.0124953264531));
#186635=CARTESIAN_POINT('Ctrl Pts',(52.8651783101952,12.9393136629288,-59.9676531117601));
#186636=CARTESIAN_POINT('Ctrl Pts',(52.8492129207352,13.1217989910806,-59.9276740961144));
#186637=CARTESIAN_POINT('Ctrl Pts',(52.8424237249517,13.1993998929284,-59.9106732352752));
#186638=CARTESIAN_POINT('Ctrl Pts',(52.8356239352222,13.2771218944127,-59.8945524608647));
#186639=CARTESIAN_POINT('Ctrl Pts',(52.8288140636152,13.354959116562,-59.879274237381));
#186640=CARTESIAN_POINT('Ctrl Pts',(52.8084063492457,13.5882204595985,-59.8334887014819));
#186641=CARTESIAN_POINT('Ctrl Pts',(52.7879062369248,13.822537779029,-59.7953375078724));
#186642=CARTESIAN_POINT('Ctrl Pts',(52.7673307740641,14.0577163898014,-59.7635551171396));
#186643=CARTESIAN_POINT('Ctrl Pts',(52.7648947458015,14.0855603195582,-59.7597922466466));
#186644=CARTESIAN_POINT('Ctrl Pts',(52.7624575809797,14.1134172399927,-59.7561214184401));
#186645=CARTESIAN_POINT('Ctrl Pts',(52.7600192757781,14.1412871946384,-59.7525428773024));
#186646=CARTESIAN_POINT('Ctrl Pts',(52.7305287650649,14.4783652583484,-59.7092615826992));
#186647=CARTESIAN_POINT('Ctrl Pts',(52.7008776982777,14.8172785115573,-59.6793561042855));
#186648=CARTESIAN_POINT('Ctrl Pts',(52.6710582492637,15.1581163818755,-59.6634323280937));
#186649=CARTESIAN_POINT('Ctrl Pts',(52.6542978767187,15.3496883214269,-59.6544821821278));
#186650=CARTESIAN_POINT('Ctrl Pts',(52.6374843263043,15.5418680821543,-59.6499500007379));
#186651=CARTESIAN_POINT('Ctrl Pts',(52.6206164493001,15.7346687985482,-59.64995));
#186652=CARTESIAN_POINT('Origin',(53.3950245803324,12.61999998,-55.24995));
#186653=CARTESIAN_POINT('',(52.8969272312866,12.5764221086262,-55.74995));
#186654=CARTESIAN_POINT('Origin',(53.3950245803325,12.61999998,-55.74995));
#186655=CARTESIAN_POINT('',(52.8969272312866,12.5764221086262,-52.64995));
#186656=CARTESIAN_POINT('Ctrl Pts',(53.3950245803324,12.11999998,-55.74995));
#186657=CARTESIAN_POINT('Ctrl Pts',(52.9368589933237,12.11999998,-55.74995));
#186658=CARTESIAN_POINT('Ctrl Pts',(52.8969272312866,12.5764221086262,-55.74995));
#186659=CARTESIAN_POINT('Ctrl Pts',(53.3950245803365,12.11999998,-55.6530085475485));
#186660=CARTESIAN_POINT('Ctrl Pts',(52.9368589933258,12.1199999799653,-55.6451138110298));
#186661=CARTESIAN_POINT('Ctrl Pts',(52.8969272312908,12.5764221085778,-55.5560711921817));
#186662=CARTESIAN_POINT('Ctrl Pts',(53.4000464934415,12.0912996152796,-55.5568836545521));
#186663=CARTESIAN_POINT('Ctrl Pts',(52.9398152308639,12.0862100303001,-55.5412722521129));
#186664=CARTESIAN_POINT('Ctrl Pts',(52.9019494572905,12.5190178027248,-55.3638118539785));
#186665=CARTESIAN_POINT('Ctrl Pts',(53.4093468596023,12.0381477794255,-55.4758105868621));
#186666=CARTESIAN_POINT('Ctrl Pts',(52.9450883668941,12.0259378096709,-55.4571865884902));
#186667=CARTESIAN_POINT('Ctrl Pts',(52.9112495105564,12.4127177074772,-55.2016711737242));
#186668=CARTESIAN_POINT('',(52.9112495105564,12.4127177074773,-55.2016711737242));
#186669=CARTESIAN_POINT('Origin',(53.4093468596018,12.4562955788561,-55.2016711737319));
#186670=CARTESIAN_POINT('Origin',(52.9691152015747,11.7513098326049,-55.69773241533));
#186671=CARTESIAN_POINT('Origin',(53.7167487055517,-8.26789346682159,-59.64995));
#186672=CARTESIAN_POINT('',(51.3604079243413,30.1389181512134,-59.64995));
#186673=CARTESIAN_POINT('',(51.2652416360248,31.226673804131,-59.64995));
#186674=CARTESIAN_POINT('Origin',(50.3642132262496,30.0517624084658,-59.64995));
#186675=CARTESIAN_POINT('Origin',(51.9689593648599,28.91999998,-52.64995));
#186676=CARTESIAN_POINT('',(51.4708620158141,28.8764221086262,-55.74995));
#186677=CARTESIAN_POINT('',(51.4708620158141,28.8764221086262,-52.64995));
#186678=CARTESIAN_POINT('Origin',(51.9689593648599,28.91999998,-55.74995));
#186679=CARTESIAN_POINT('Ctrl Pts',(51.9689593648599,28.41999998,-55.74995));
#186680=CARTESIAN_POINT('Ctrl Pts',(51.5107937778512,28.41999998,-55.74995));
#186681=CARTESIAN_POINT('Ctrl Pts',(51.4708620158141,28.8764221086262,-55.74995));
#186682=CARTESIAN_POINT('Ctrl Pts',(51.9689593648654,28.41999998,-55.6186826543062));
#186683=CARTESIAN_POINT('Ctrl Pts',(51.5107937778567,28.4199999799462,-55.6078478088784));
#186684=CARTESIAN_POINT('Ctrl Pts',(51.4708620158198,28.8764221085606,-55.4874153086129));
#186685=CARTESIAN_POINT('Ctrl Pts',(51.9783882917162,28.3661134164373,-55.4889566552507));
#186686=CARTESIAN_POINT('Ctrl Pts',(51.5164047569777,28.3558661951151,-55.4680441063688));
#186687=CARTESIAN_POINT('Ctrl Pts',(51.4802909426703,28.7686489815003,-55.2279633105015));
#186688=CARTESIAN_POINT('Ctrl Pts',(52.0107801105432,28.1809933247493,-55.3038365635627));
#186689=CARTESIAN_POINT('Ctrl Pts',(51.5345366632341,28.1486175582537,-55.2822894538777));
#186690=CARTESIAN_POINT('Ctrl Pts',(51.5126827614974,28.3984087981251,-54.8577231271254));
#186691=CARTESIAN_POINT('Ctrl Pts',(52.033479219109,28.0512673256941,-55.24995));
#186692=CARTESIAN_POINT('Ctrl Pts',(51.5469301855916,28.0069589495408,-55.2386587236988));
#186693=CARTESIAN_POINT('Ctrl Pts',(51.5353818700614,28.1389568000129,-54.7499500000658));
#186694=CARTESIAN_POINT('Ctrl Pts',(52.0564480283858,27.91999998,-55.24995));
#186695=CARTESIAN_POINT('Ctrl Pts',(51.5583506793399,27.8764221086261,-55.24995));
#186696=CARTESIAN_POINT('Ctrl Pts',(51.55835067934,27.8764221086262,-54.74995));
#186697=CARTESIAN_POINT('',(51.55835067934,27.8764221086262,-54.74995));
#186698=CARTESIAN_POINT('Ctrl Pts',(51.55835067934,27.8764221086262,-54.74995));
#186699=CARTESIAN_POINT('Ctrl Pts',(51.5353818700614,28.1389568000129,-54.7499500000658));
#186700=CARTESIAN_POINT('Ctrl Pts',(51.5126827614974,28.3984087981251,-54.8577231271254));
#186701=CARTESIAN_POINT('Ctrl Pts',(51.4964868520838,28.5835288898127,-55.0428432188135));
#186702=CARTESIAN_POINT('Ctrl Pts',(51.4802909426703,28.7686489815003,-55.2279633105015));
#186703=CARTESIAN_POINT('Ctrl Pts',(51.4708620158198,28.8764221085606,-55.4874153086129));
#186704=CARTESIAN_POINT('Ctrl Pts',(51.4708620158141,28.8764221086262,-55.74995));
#186705=CARTESIAN_POINT('Origin',(52.0564480283858,27.91999998,-54.74995));
#186706=CARTESIAN_POINT('Origin',(51.7633389850707,31.2702516755049,-54.74995));
#186707=CARTESIAN_POINT('',(51.6020950111029,27.3764221086262,-54.74995));
#186708=CARTESIAN_POINT('',(51.2652416360248,31.226673804131,-54.74995));
#186709=CARTESIAN_POINT('Origin',(52.1001923601488,27.41999998,-54.74995));
#186710=CARTESIAN_POINT('Ctrl Pts',(52.1002185497626,27.4200238915827,-55.2499499996828));
#186711=CARTESIAN_POINT('Ctrl Pts',(51.6020931262756,27.3764436523005,-55.2499781675633));
#186712=CARTESIAN_POINT('Ctrl Pts',(51.6020912850816,27.3764646972444,-54.7499500009454));
#186713=CARTESIAN_POINT('Ctrl Pts',(52.1231889541655,27.288749433996,-55.2499434816096));
#186714=CARTESIAN_POINT('Ctrl Pts',(51.6138470691841,27.2420954701119,-55.2615949036223));
#186715=CARTESIAN_POINT('Ctrl Pts',(51.6250613655174,27.1139154764662,-54.7499383449291));
#186716=CARTESIAN_POINT('Ctrl Pts',(52.1458900110277,27.1590137328186,-55.3038301720452));
#186717=CARTESIAN_POINT('Ctrl Pts',(51.6242350673701,27.1233601075035,-55.327473556918));
#186718=CARTESIAN_POINT('Ctrl Pts',(51.6477620531743,26.8544454292379,-54.8577131170148));
#186719=CARTESIAN_POINT('Ctrl Pts',(52.1782841123997,26.9738822391066,-55.4889602509496));
#186720=CARTESIAN_POINT('Ctrl Pts',(51.6383741166919,26.9617500342493,-55.5134049012208));
#186721=CARTESIAN_POINT('Ctrl Pts',(51.6801556235438,26.4841852256414,-55.2279733206121));
#186722=CARTESIAN_POINT('Ctrl Pts',(52.1877133516444,26.9199941513771,-55.618695932326));
#186723=CARTESIAN_POINT('Ctrl Pts',(51.6420241800604,26.920029619041,-55.631800368908));
#186724=CARTESIAN_POINT('Ctrl Pts',(51.6895846943154,26.376410453555,-55.4874433678397));
#186725=CARTESIAN_POINT('Ctrl Pts',(52.1877123348205,26.9199999794923,-55.7499712944312));
#186726=CARTESIAN_POINT('Ctrl Pts',(51.6420237834999,26.9200341517443,-55.7499691665899));
#186727=CARTESIAN_POINT('Ctrl Pts',(51.6895836745461,26.3764221095716,-55.7499925886182));
#186728=CARTESIAN_POINT('',(51.6895836746288,26.3764221086262,-55.74995));
#186729=CARTESIAN_POINT('Ctrl Pts',(51.6895836746288,26.3764221086262,-55.74995));
#186730=CARTESIAN_POINT('Ctrl Pts',(51.6895836746231,26.3764221086917,-55.4874153086129));
#186731=CARTESIAN_POINT('Ctrl Pts',(51.6801547477726,26.484195235752,-55.2279633105015));
#186732=CARTESIAN_POINT('Ctrl Pts',(51.6639588383591,26.6693153274396,-55.0428432188135));
#186733=CARTESIAN_POINT('Ctrl Pts',(51.6477629289455,26.8544354191273,-54.8577231271254));
#186734=CARTESIAN_POINT('Ctrl Pts',(51.6250638203816,27.1138874172394,-54.7499500000658));
#186735=CARTESIAN_POINT('Ctrl Pts',(51.6020950111029,27.3764221086262,-54.74995));
#186736=CARTESIAN_POINT('Origin',(52.1876810236747,26.41999998,-55.74995));
#186737=CARTESIAN_POINT('Origin',(52.1876810236747,26.41999998,-52.64995));
#186738=CARTESIAN_POINT('',(51.6895836746288,26.3764221086262,-52.64995));
#186739=CARTESIAN_POINT('Origin',(53.7167487055517,-8.26789346682159,-59.64995));
#186740=CARTESIAN_POINT('',(51.2652416360248,31.226673804131,-59.64995));
#186741=CARTESIAN_POINT('Origin',(47.0226009489055,34.0551009288773,-59.64995));
#186742=CARTESIAN_POINT('',(50.4931441736257,31.9987712665301,-59.64995));
#186743=CARTESIAN_POINT('Origin',(49.7860373924392,31.2916644853435,-59.64995));
#186744=CARTESIAN_POINT('',(44.9662712865584,37.5256441535974,-59.64995));
#186745=CARTESIAN_POINT('Origin',(44.2591645053719,36.8185373724109,-59.64995));
#186746=CARTESIAN_POINT('',(44.1941738241593,38.2977416159964,-59.64995));
#186747=CARTESIAN_POINT('Origin',(37.,39.4290601878171,-92.34995));
#186748=CARTESIAN_POINT('',(36.9564221286262,38.9309628387712,-55.74995));
#186749=CARTESIAN_POINT('Origin',(37.,39.4290601878171,-55.74995));
#186750=CARTESIAN_POINT('',(36.9564221286262,38.9309628387712,-52.64995));
#186751=CARTESIAN_POINT('Ctrl Pts',(37.5,39.4290601878171,-55.74995));
#186752=CARTESIAN_POINT('Ctrl Pts',(37.5000000000001,38.8834059372824,-55.74995));
#186753=CARTESIAN_POINT('Ctrl Pts',(36.9564221286262,38.9309628387712,-55.74995));
#186754=CARTESIAN_POINT('Ctrl Pts',(37.5,39.4290601878116,-55.6186826543065));
#186755=CARTESIAN_POINT('Ctrl Pts',(37.5000000000036,38.8834059372834,-55.6317784220504));
#186756=CARTESIAN_POINT('Ctrl Pts',(36.9564221286917,38.9309628387654,-55.487415308613));
#186757=CARTESIAN_POINT('Ctrl Pts',(37.5538865635632,39.4196312609607,-55.4889566552503));
#186758=CARTESIAN_POINT('Ctrl Pts',(37.5417246342956,38.879755504792,-55.5133819370962));
#186759=CARTESIAN_POINT('Ctrl Pts',(37.0641952557516,38.9215339119149,-55.2279633105015));
#186760=CARTESIAN_POINT('Ctrl Pts',(37.7390066552503,39.3872394421337,-55.3038365635632));
#186761=CARTESIAN_POINT('Ctrl Pts',(37.7033393021412,38.8656160534955,-55.3274496218441));
#186762=CARTESIAN_POINT('Ctrl Pts',(37.4344354391277,38.8891420930878,-54.8577231271255));
#186763=CARTESIAN_POINT('Ctrl Pts',(37.8687326543062,39.3645403335679,-55.24995));
#186764=CARTESIAN_POINT('Ctrl Pts',(37.8220750118298,38.855228024944,-55.2615708605686));
#186765=CARTESIAN_POINT('Ctrl Pts',(37.6938874372391,38.8664429845239,-54.7499500000658));
#186766=CARTESIAN_POINT('Ctrl Pts',(38.,39.3415715242911,-55.24995));
#186767=CARTESIAN_POINT('Ctrl Pts',(37.9564221286261,38.8434741752452,-55.2499499999999));
#186768=CARTESIAN_POINT('Ctrl Pts',(37.9564221286262,38.8434741752452,-54.74995));
#186769=CARTESIAN_POINT('',(37.9564221286262,38.8434741752452,-54.74995));
#186770=CARTESIAN_POINT('Origin',(38.,39.3415715242911,-54.74995));
#186771=CARTESIAN_POINT('Ctrl Pts',(37.9564221286262,38.8434741752452,-54.74995));
#186772=CARTESIAN_POINT('Ctrl Pts',(37.6938874372391,38.8664429845239,-54.7499500000658));
#186773=CARTESIAN_POINT('Ctrl Pts',(37.4344354391277,38.8891420930878,-54.8577231271255));
#186774=CARTESIAN_POINT('Ctrl Pts',(37.2493153474397,38.9053380025014,-55.0428432188135));
#186775=CARTESIAN_POINT('Ctrl Pts',(37.0641952557516,38.9215339119149,-55.2279633105015));
#186776=CARTESIAN_POINT('Ctrl Pts',(36.9564221286917,38.9309628387654,-55.487415308613));
#186777=CARTESIAN_POINT('Ctrl Pts',(36.9564221286262,38.9309628387712,-55.74995));
#186778=CARTESIAN_POINT('Origin',(3.70444879364117,42.3420434642203,-54.74995));
#186779=CARTESIAN_POINT('',(38.4564221286262,38.7997298434823,-54.74995));
#186780=CARTESIAN_POINT('Origin',(38.5,39.2978271925282,-54.74995));
#186781=CARTESIAN_POINT('',(38.,38.8396616055195,-54.74995));
#186782=CARTESIAN_POINT('Ctrl Pts',(38.5,39.2978271925282,-55.24995));
#186783=CARTESIAN_POINT('Ctrl Pts',(38.4564221286261,38.7997298434823,-55.2499499999999));
#186784=CARTESIAN_POINT('Ctrl Pts',(38.4564221286262,38.7997298434823,-54.74995));
#186785=CARTESIAN_POINT('Ctrl Pts',(38.6312673456941,39.2748583832512,-55.24995));
#186786=CARTESIAN_POINT('Ctrl Pts',(38.5869589695399,38.788309349734,-55.2386587236917));
#186787=CARTESIAN_POINT('Ctrl Pts',(38.7189568200132,38.7767610342036,-54.7499500000658));
#186788=CARTESIAN_POINT('Ctrl Pts',(38.7609933447493,39.2521592746855,-55.3038365635627));
#186789=CARTESIAN_POINT('Ctrl Pts',(38.7286175782541,38.7759158273764,-55.2822894538767));
#186790=CARTESIAN_POINT('Ctrl Pts',(38.9784088181247,38.7540619256397,-54.8577231271255));
#186791=CARTESIAN_POINT('Ctrl Pts',(38.9461134364373,39.2197674558585,-55.4889566552507));
#186792=CARTESIAN_POINT('Ctrl Pts',(38.9358662151147,38.7577839211201,-55.4680441063697));
#186793=CARTESIAN_POINT('Ctrl Pts',(39.3486490015007,38.7216701068126,-55.2279633105015));
#186794=CARTESIAN_POINT('Ctrl Pts',(39.,39.2103385290077,-55.6186826543063));
#186795=CARTESIAN_POINT('Ctrl Pts',(38.9999999999489,38.7521729419962,-55.6078478088777));
#186796=CARTESIAN_POINT('Ctrl Pts',(39.4564221285606,38.7122411799621,-55.487415308613));
#186797=CARTESIAN_POINT('Ctrl Pts',(39.,39.2103385290022,-55.74995));
#186798=CARTESIAN_POINT('Ctrl Pts',(39.,38.7521729419935,-55.74995));
#186799=CARTESIAN_POINT('Ctrl Pts',(39.4564221286262,38.7122411799564,-55.74995));
#186800=CARTESIAN_POINT('',(39.4564221286262,38.7122411799564,-55.74995));
#186801=CARTESIAN_POINT('Origin',(39.5,39.2103385290022,-55.74995));
#186802=CARTESIAN_POINT('Ctrl Pts',(39.4564221286262,38.7122411799564,-55.74995));
#186803=CARTESIAN_POINT('Ctrl Pts',(39.4564221285606,38.7122411799621,-55.487415308613));
#186804=CARTESIAN_POINT('Ctrl Pts',(39.3486490015007,38.7216701068126,-55.2279633105015));
#186805=CARTESIAN_POINT('Ctrl Pts',(39.1635289098127,38.7378660162261,-55.0428432188135));
#186806=CARTESIAN_POINT('Ctrl Pts',(38.9784088181247,38.7540619256397,-54.8577231271255));
#186807=CARTESIAN_POINT('Ctrl Pts',(38.7189568200132,38.7767610342036,-54.7499500000658));
#186808=CARTESIAN_POINT('Ctrl Pts',(38.4564221286262,38.7997298434823,-54.74995));
#186809=CARTESIAN_POINT('Origin',(39.5,39.2103385290023,-129.34995));
#186810=CARTESIAN_POINT('',(39.4564221286262,38.7122411799564,-55.74995));
#186811=CARTESIAN_POINT('Origin',(4.69960655320655,40.7492486855235,-59.64995));
#186812=CARTESIAN_POINT('',(43.1064181712417,38.392907904313,-59.64995));
#186813=CARTESIAN_POINT('',(24.5275331667447,40.0183497231583,-59.64995));
#186814=CARTESIAN_POINT('Origin',(43.019262428494,37.3967132062212,-59.64995));
#186815=CARTESIAN_POINT('Ctrl Pts',(25.3802177275058,39.9437494905281,-60.1097730249189));
#186816=CARTESIAN_POINT('Ctrl Pts',(25.5227862062494,39.9312763648619,-60.5923862926587));
#186817=CARTESIAN_POINT('Ctrl Pts',(25.572468850428,39.5210489290882,-60.8798615124595));
#186818=CARTESIAN_POINT('Ctrl Pts',(25.9036128690389,39.8979583490994,-59.9539737371434));
#186819=CARTESIAN_POINT('Ctrl Pts',(26.0512576071349,39.8850411082851,-60.5102318318317));
#186820=CARTESIAN_POINT('Ctrl Pts',(26.059719336348,39.3883003271754,-60.8019346414671));
#186821=CARTESIAN_POINT('Ctrl Pts',(26.4338688782163,39.8515669595299,-59.8461489023585));
#186822=CARTESIAN_POINT('Ctrl Pts',(26.5712796028832,39.8395450788764,-60.4792397999495));
#186823=CARTESIAN_POINT('Ctrl Pts',(26.5494003841727,39.2520983829515,-60.748049450926));
#186824=CARTESIAN_POINT('Ctrl Pts',(27.5031785292772,39.7580144872632,-59.6965141185183));
#186825=CARTESIAN_POINT('Ctrl Pts',(27.601298997848,39.7494300586015,-60.4901498725136));
#186826=CARTESIAN_POINT('Ctrl Pts',(27.529498834359,38.9740545371747,-60.6732320595124));
#186827=CARTESIAN_POINT('Ctrl Pts',(28.0425516254864,39.710825455934,-59.6557090289434));
#186828=CARTESIAN_POINT('Ctrl Pts',(28.1179039179461,39.7042329845701,-60.5392590138154));
#186829=CARTESIAN_POINT('Ctrl Pts',(28.0200529940657,38.8321810243987,-60.6528294999755));
#186830=CARTESIAN_POINT('Ctrl Pts',(28.5867228014573,39.663216647019,-59.6505032458185));
#186831=CARTESIAN_POINT('Ctrl Pts',(28.5960141520618,39.6624037591722,-60.6291816703115));
#186832=CARTESIAN_POINT('Ctrl Pts',(28.5109323535812,38.6876131939284,-60.6502266229092));
#186833=CARTESIAN_POINT('',(25.3802177275058,39.9437494905281,-60.1097730249189));
#186834=CARTESIAN_POINT('Ctrl Pts',(28.4564221286157,39.6746164786217,-59.6524466674074));
#186835=CARTESIAN_POINT('Ctrl Pts',(28.1317998821407,39.7030172440177,-59.6590182799319));
#186836=CARTESIAN_POINT('Ctrl Pts',(27.8089020756387,39.7312671410707,-59.6781506934664));
#186837=CARTESIAN_POINT('Ctrl Pts',(27.4876982951917,39.7593688309396,-59.7096215394412));
#186838=CARTESIAN_POINT('Ctrl Pts',(27.3141484358393,39.7745524764045,-59.7266255762088));
#186839=CARTESIAN_POINT('Ctrl Pts',(27.1410937670796,39.7896927982219,-59.7472310046323));
#186840=CARTESIAN_POINT('Ctrl Pts',(26.9685328542776,39.8047899206072,-59.7713974032318));
#186841=CARTESIAN_POINT('Ctrl Pts',(26.9471826335434,39.8066578227303,-59.7743874079558));
#186842=CARTESIAN_POINT('Ctrl Pts',(26.9258394639526,39.8085251079323,-59.7774303163423));
#186843=CARTESIAN_POINT('Ctrl Pts',(26.904503506364,39.8103917621319,-59.7805271013239));
#186844=CARTESIAN_POINT('Ctrl Pts',(26.5372951385086,39.8425183277728,-59.8338251712117));
#186845=CARTESIAN_POINT('Ctrl Pts',(26.172250803663,39.874455574155,-59.9028698737259));
#186846=CARTESIAN_POINT('Ctrl Pts',(25.8100560257878,39.9061435120092,-59.9926952104099));
#186847=CARTESIAN_POINT('Ctrl Pts',(25.6663124460363,39.9187194460103,-60.0283440276653));
#186848=CARTESIAN_POINT('Ctrl Pts',(25.5230181721596,39.9312560704744,-60.0672655467143));
#186849=CARTESIAN_POINT('Ctrl Pts',(25.3802177275058,39.9437494905281,-60.1097730249189));
#186850=CARTESIAN_POINT('Origin',(25.2930619847582,38.9475547924363,-60.1097730249189));
#186851=CARTESIAN_POINT('Origin',(28.5,40.1727138277873,-52.64995));
#186852=CARTESIAN_POINT('',(28.4564221286262,39.6746164787415,-55.74995));
#186853=CARTESIAN_POINT('Origin',(28.5,40.1727138277873,-55.74995));
#186854=CARTESIAN_POINT('',(28.4564221286262,39.6746164787415,-52.64995));
#186855=CARTESIAN_POINT('Ctrl Pts',(29.,40.1727138277873,-55.74995));
#186856=CARTESIAN_POINT('Ctrl Pts',(29.,39.6270595772528,-55.74995));
#186857=CARTESIAN_POINT('Ctrl Pts',(28.4564221286262,39.6746164787415,-55.74995));
#186858=CARTESIAN_POINT('Ctrl Pts',(29.,40.1727138277819,-55.6186826543062));
#186859=CARTESIAN_POINT('Ctrl Pts',(29.0000000000046,39.6270595772536,-55.6317784220498));
#186860=CARTESIAN_POINT('Ctrl Pts',(28.4564221286917,39.6746164787358,-55.487415308613));
#186861=CARTESIAN_POINT('Ctrl Pts',(29.0538865635627,40.163284900931,-55.4889566552507));
#186862=CARTESIAN_POINT('Ctrl Pts',(29.0417246342951,39.6234091447624,-55.5133819370971));
#186863=CARTESIAN_POINT('Ctrl Pts',(28.5641952557521,39.6651875518853,-55.2279633105015));
#186864=CARTESIAN_POINT('Ctrl Pts',(29.2390066552507,40.1308930821041,-55.3038365635627));
#186865=CARTESIAN_POINT('Ctrl Pts',(29.2033393021417,39.6092696934658,-55.3274496218431));
#186866=CARTESIAN_POINT('Ctrl Pts',(28.9344354391272,39.6327957330582,-54.8577231271255));
#186867=CARTESIAN_POINT('Ctrl Pts',(29.368732654306,40.1081939735386,-55.24995));
#186868=CARTESIAN_POINT('Ctrl Pts',(29.3220750118295,39.5988816649146,-55.2615708605689));
#186869=CARTESIAN_POINT('Ctrl Pts',(29.1938874372395,39.6100966244942,-54.7499500000658));
#186870=CARTESIAN_POINT('Ctrl Pts',(29.5,40.0852251642615,-55.24995));
#186871=CARTESIAN_POINT('Ctrl Pts',(29.4564221286262,39.5871278152156,-55.24995));
#186872=CARTESIAN_POINT('Ctrl Pts',(29.4564221286262,39.5871278152156,-54.74995));
#186873=CARTESIAN_POINT('',(29.4564221286262,39.5871278152156,-54.74995));
#186874=CARTESIAN_POINT('Ctrl Pts',(29.4564221286262,39.5871278152156,-54.74995));
#186875=CARTESIAN_POINT('Ctrl Pts',(29.1938874372394,39.6100966244942,-54.7499500000658));
#186876=CARTESIAN_POINT('Ctrl Pts',(28.9344354391271,39.6327957330582,-54.8577231271255));
#186877=CARTESIAN_POINT('Ctrl Pts',(28.7493153474396,39.6489916424717,-55.0428432188135));
#186878=CARTESIAN_POINT('Ctrl Pts',(28.5641952557521,39.6651875518853,-55.2279633105015));
#186879=CARTESIAN_POINT('Ctrl Pts',(28.4564221286917,39.6746164787358,-55.487415308613));
#186880=CARTESIAN_POINT('Ctrl Pts',(28.4564221286262,39.6746164787415,-55.74995));
#186881=CARTESIAN_POINT('Origin',(29.5,40.0852251642615,-54.74995));
#186882=CARTESIAN_POINT('Origin',(3.70444879364117,42.3420434642203,-54.74995));
#186883=CARTESIAN_POINT('',(29.9564221286262,39.5433834834526,-54.74995));
#186884=CARTESIAN_POINT('',(29.5,39.5833152454898,-54.74995));
#186885=CARTESIAN_POINT('Origin',(30.,40.0414808324985,-54.74995));
#186886=CARTESIAN_POINT('Ctrl Pts',(30.,40.0414808324985,-55.24995));
#186887=CARTESIAN_POINT('Ctrl Pts',(29.9564221286262,39.5433834834526,-55.24995));
#186888=CARTESIAN_POINT('Ctrl Pts',(29.9564221286262,39.5433834834526,-54.74995));
#186889=CARTESIAN_POINT('Ctrl Pts',(30.131267345694,40.0185120232214,-55.24995));
#186890=CARTESIAN_POINT('Ctrl Pts',(30.0869589695403,39.5319629897042,-55.2386587236916));
#186891=CARTESIAN_POINT('Ctrl Pts',(30.218956820013,39.520414674174,-54.7499500000658));
#186892=CARTESIAN_POINT('Ctrl Pts',(30.2609933447492,39.9958129146559,-55.3038365635627));
#186893=CARTESIAN_POINT('Ctrl Pts',(30.2286175782536,39.5195694673468,-55.2822894538777));
#186894=CARTESIAN_POINT('Ctrl Pts',(30.4784088181251,39.4977155656101,-54.8577231271254));
#186895=CARTESIAN_POINT('Ctrl Pts',(30.4461134364373,39.9634210958289,-55.4889566552508));
#186896=CARTESIAN_POINT('Ctrl Pts',(30.4358662151152,39.5014375610904,-55.4680441063689));
#186897=CARTESIAN_POINT('Ctrl Pts',(30.8486490015003,39.4653237467829,-55.2279633105015));
#186898=CARTESIAN_POINT('Ctrl Pts',(30.5,39.9539921689781,-55.6186826543063));
#186899=CARTESIAN_POINT('Ctrl Pts',(30.4999999999484,39.4958265819666,-55.6078478088783));
#186900=CARTESIAN_POINT('Ctrl Pts',(30.9564221285606,39.4558948199325,-55.4874153086129));
#186901=CARTESIAN_POINT('Ctrl Pts',(30.5,39.9539921689726,-55.74995));
#186902=CARTESIAN_POINT('Ctrl Pts',(30.5,39.4958265819639,-55.74995));
#186903=CARTESIAN_POINT('Ctrl Pts',(30.9564221286262,39.4558948199267,-55.74995));
#186904=CARTESIAN_POINT('',(30.9564221286262,39.4558948199267,-55.74995));
#186905=CARTESIAN_POINT('Ctrl Pts',(30.9564221286262,39.4558948199267,-55.74995));
#186906=CARTESIAN_POINT('Ctrl Pts',(30.9564221285606,39.4558948199325,-55.4874153086129));
#186907=CARTESIAN_POINT('Ctrl Pts',(30.8486490015003,39.4653237467829,-55.2279633105015));
#186908=CARTESIAN_POINT('Ctrl Pts',(30.6635289098127,39.4815196561965,-55.0428432188135));
#186909=CARTESIAN_POINT('Ctrl Pts',(30.4784088181251,39.4977155656101,-54.8577231271254));
#186910=CARTESIAN_POINT('Ctrl Pts',(30.218956820013,39.520414674174,-54.7499500000658));
#186911=CARTESIAN_POINT('Ctrl Pts',(29.9564221286262,39.5433834834526,-54.74995));
#186912=CARTESIAN_POINT('Origin',(31.,39.9539921689726,-55.74995));
#186913=CARTESIAN_POINT('Origin',(31.,39.9539921689726,-52.64995));
#186914=CARTESIAN_POINT('',(30.9564221286262,39.4558948199267,-52.64995));
#186915=CARTESIAN_POINT('Origin',(4.69960655320655,40.7492486855235,-59.64995));
#186916=CARTESIAN_POINT('',(24.5275331667447,40.0183497231583,-59.64995));
#186917=CARTESIAN_POINT('Ctrl Pts',(25.572468850428,39.5210489290882,-60.8798615124595));
#186918=CARTESIAN_POINT('Ctrl Pts',(25.5227862062494,39.9312763648619,-60.5923862926587));
#186919=CARTESIAN_POINT('Ctrl Pts',(25.3802177275058,39.943749490528,-60.1097730249189));
#186920=CARTESIAN_POINT('Ctrl Pts',(25.2694477113958,39.6036052974814,-60.9283242463865));
#186921=CARTESIAN_POINT('Ctrl Pts',(25.2414738675095,39.9482243711148,-60.6373384822398));
#186922=CARTESIAN_POINT('Ctrl Pts',(25.1089972874034,39.9674782043536,-60.2066542280814));
#186923=CARTESIAN_POINT('Ctrl Pts',(24.9650212889786,39.6997861053784,-60.9766079791613));
#186924=CARTESIAN_POINT('Ctrl Pts',(24.9493186357974,39.9900159541718,-60.6937268873635));
#186925=CARTESIAN_POINT('Ctrl Pts',(24.8422602775208,40.0127575956439,-60.3032659617329));
#186926=CARTESIAN_POINT('Ctrl Pts',(24.3438778196125,39.9224728282123,-61.0507205920708));
#186927=CARTESIAN_POINT('Ctrl Pts',(24.3665512677474,40.1299777240875,-60.7838744940585));
#186928=CARTESIAN_POINT('Ctrl Pts',(24.3096510677746,40.1491089179394,-60.4514911807313));
#186929=CARTESIAN_POINT('Ctrl Pts',(24.0238031468177,40.0506166841414,-61.0754935252291));
#186930=CARTESIAN_POINT('Ctrl Pts',(24.0669512606426,40.2300655352922,-60.8169267274199));
#186931=CARTESIAN_POINT('Ctrl Pts',(24.0409609718932,40.24165543605,-60.5010370503254));
#186932=CARTESIAN_POINT('Ctrl Pts',(23.7057274034393,40.1924568448808,-61.0754935261973));
#186933=CARTESIAN_POINT('Ctrl Pts',(23.7796330855957,40.3581899105084,-60.8169267287601));
#186934=CARTESIAN_POINT('Ctrl Pts',(23.7796330855957,40.3581899105085,-60.5010370523946));
#186935=CARTESIAN_POINT('',(23.7796330855957,40.3581899105085,-60.5010370523947));
#186936=CARTESIAN_POINT('Origin',(23.372360414466,39.4448832964128,-60.5010370523947));
#186937=CARTESIAN_POINT('Ctrl Pts',(25.3802177275058,39.943749490528,-60.1097730249189));
#186938=CARTESIAN_POINT('Ctrl Pts',(25.3377363135767,39.9474661326574,-60.1249475836356));
#186939=CARTESIAN_POINT('Ctrl Pts',(25.2979927848269,39.9514798686665,-60.1391717405498));
#186940=CARTESIAN_POINT('Ctrl Pts',(25.2609589409308,39.9556072078286,-60.1523839922766));
#186941=CARTESIAN_POINT('Ctrl Pts',(25.2220309924076,39.9599456407197,-60.166271987715));
#186942=CARTESIAN_POINT('Ctrl Pts',(25.1860970996603,39.9644092678141,-60.1790428287426));
#186943=CARTESIAN_POINT('Ctrl Pts',(25.1531400482302,39.9688089768955,-60.1906788704549));
#186944=CARTESIAN_POINT('Ctrl Pts',(25.1171272460509,39.9736166233906,-60.2033937964009));
#186945=CARTESIAN_POINT('Ctrl Pts',(25.0846688996706,39.9783471985322,-60.214754833184));
#186946=CARTESIAN_POINT('Ctrl Pts',(25.0557488187266,39.9827921994797,-60.2247897604492));
#186947=CARTESIAN_POINT('Ctrl Pts',(25.0404115499051,39.9851495294808,-60.230111611981));
#186948=CARTESIAN_POINT('Ctrl Pts',(25.0260697403982,39.9874272035645,-60.2350611282861));
#186949=CARTESIAN_POINT('Ctrl Pts',(25.0127218112758,39.9895989300769,-60.2396456694191));
#186950=CARTESIAN_POINT('Ctrl Pts',(25.0067601800825,39.9905688957099,-60.2416932786905));
#186951=CARTESIAN_POINT('Ctrl Pts',(25.0009985443053,39.9915174894833,-60.2436742905531));
#186952=CARTESIAN_POINT('Ctrl Pts',(24.9954346520016,39.9924429351662,-60.2455817846297));
#186953=CARTESIAN_POINT('Ctrl Pts',(24.9926527058498,39.9929056580077,-60.246535531668));
#186954=CARTESIAN_POINT('Ctrl Pts',(24.9899201612054,39.9933626023715,-60.2474707707647));
#186955=CARTESIAN_POINT('Ctrl Pts',(24.9872369808442,39.9938135212305,-60.2483875019273));
#186956=CARTESIAN_POINT('Ctrl Pts',(24.9845538004829,39.9942644400894,-60.2493042330899));
#186957=CARTESIAN_POINT('Ctrl Pts',(24.9839661492007,39.9943620659877,-60.2495059770713));
#186958=CARTESIAN_POINT('Ctrl Pts',(24.9793354964283,39.9951479630991,-60.2510821716195));
#186959=CARTESIAN_POINT('Ctrl Pts',(24.9279712430605,40.003865312539,-60.2685656799095));
#186960=CARTESIAN_POINT('Ctrl Pts',(24.8784655257637,40.0130996371524,-60.2850161933571));
#186961=CARTESIAN_POINT('Ctrl Pts',(24.8308013791055,40.0226898926197,-60.3003979240438));
#186962=CARTESIAN_POINT('Ctrl Pts',(24.8097123058818,40.0269331155444,-60.3072035938712));
#186963=CARTESIAN_POINT('Ctrl Pts',(24.788983882997,40.031246087386,-60.3138007330426));
#186964=CARTESIAN_POINT('Ctrl Pts',(24.7686152583926,40.0356152269098,-60.3201893531102));
#186965=CARTESIAN_POINT('Ctrl Pts',(24.7200988895179,40.0460221536866,-60.3354065144951));
#186966=CARTESIAN_POINT('Ctrl Pts',(24.6736205664744,40.0567475976147,-60.3494274338396));
#186967=CARTESIAN_POINT('Ctrl Pts',(24.6291674207005,40.067616735454,-60.3622788776091));
#186968=CARTESIAN_POINT('Ctrl Pts',(24.6203828382536,40.0697646337818,-60.3648185081659));
#186969=CARTESIAN_POINT('Ctrl Pts',(24.6116773469398,40.071918181481,-60.3673126301496));
#186970=CARTESIAN_POINT('Ctrl Pts',(24.6030508521459,40.0740760877997,-60.3697616771469));
#186971=CARTESIAN_POINT('Ctrl Pts',(24.597473538032,40.0754712455845,-60.3713450670069));
#186972=CARTESIAN_POINT('Ctrl Pts',(24.5930293483899,40.0765902002605,-60.3725999802461));
#186973=CARTESIAN_POINT('Ctrl Pts',(24.5872536899646,40.0780546948281,-60.3742211678561));
#186974=CARTESIAN_POINT('Ctrl Pts',(24.5852952247151,40.0785512895898,-60.3747708955864));
#186975=CARTESIAN_POINT('Ctrl Pts',(24.5831836712054,40.0790878901403,-60.3753624736458));
#186976=CARTESIAN_POINT('Ctrl Pts',(24.5808229576604,40.0796897628148,-60.376021988692));
#186977=CARTESIAN_POINT('Ctrl Pts',(24.5791995774519,40.0801036496203,-60.3764755141421));
#186978=CARTESIAN_POINT('Ctrl Pts',(24.5775771985916,40.0805181359584,-60.3769279325757));
#186979=CARTESIAN_POINT('Ctrl Pts',(24.5759558187269,40.0809332193942,-60.377379242392));
#186980=CARTESIAN_POINT('Ctrl Pts',(24.5180765447908,40.095750677295,-60.3934898929903));
#186981=CARTESIAN_POINT('Ctrl Pts',(24.4613393330448,40.1113972696723,-60.4080863642803));
#186982=CARTESIAN_POINT('Ctrl Pts',(24.405783193626,40.1277441546784,-60.4211041690535));
#186983=CARTESIAN_POINT('Ctrl Pts',(24.3457160996731,40.1454183467258,-60.4351789717766));
#186984=CARTESIAN_POINT('Ctrl Pts',(24.2870296504741,40.1639110071772,-60.4474085751543));
#186985=CARTESIAN_POINT('Ctrl Pts',(24.2297431097138,40.1830806284349,-60.4577626719886));
#186986=CARTESIAN_POINT('Ctrl Pts',(24.1695508319587,40.2032225876436,-60.4686419581922));
#186987=CARTESIAN_POINT('Ctrl Pts',(24.1109038743736,40.2241118573122,-60.4774512669829));
#186988=CARTESIAN_POINT('Ctrl Pts',(24.0537946101968,40.24560866413,-60.4842026045568));
#186989=CARTESIAN_POINT('Ctrl Pts',(23.9916402035452,40.2690045402969,-60.4915503683052));
#186990=CARTESIAN_POINT('Ctrl Pts',(23.9313070653885,40.2931197928505,-60.4964610838971));
#186991=CARTESIAN_POINT('Ctrl Pts',(23.8727530525808,40.317805125582,-60.4989952734271));
#186992=CARTESIAN_POINT('Ctrl Pts',(23.8412002274789,40.3311072367254,-60.5003608645315));
#186993=CARTESIAN_POINT('Ctrl Pts',(23.8101634964631,40.3445754224573,-60.5010370523947));
#186994=CARTESIAN_POINT('Ctrl Pts',(23.7796330855957,40.3581899105085,-60.5010370523947));
#186995=CARTESIAN_POINT('Origin',(47.0226009489055,-59.9901009689335,-59.64995));
#186996=CARTESIAN_POINT('',(44.9662712865582,-63.4606441936539,-59.64995));
#186997=CARTESIAN_POINT('Origin',(44.2591645053717,-62.7535374124673,-59.64995));
#186998=CARTESIAN_POINT('',(50.4931441736259,-57.9337713065862,-59.64995));
#186999=CARTESIAN_POINT('Origin',(49.7860373924393,-57.2266645253997,-59.64995));
#187000=CARTESIAN_POINT('',(51.265241636025,-57.1616738441871,-59.64995));
#187001=CARTESIAN_POINT('Origin',(33.85,-65.63964951798,-52.64995));
#187002=CARTESIAN_POINT('',(33.8064221286261,-65.1415521689341,-55.74995));
#187003=CARTESIAN_POINT('',(33.8064221286261,-65.1415521689341,-52.64995));
#187004=CARTESIAN_POINT('Origin',(33.85,-65.63964951798,-55.74995));
#187005=CARTESIAN_POINT('Ctrl Pts',(33.35,-65.63964951798,-55.74995));
#187006=CARTESIAN_POINT('Ctrl Pts',(33.3499999999999,-65.1814839309712,
-55.74995));
#187007=CARTESIAN_POINT('Ctrl Pts',(33.8064221286261,-65.1415521689341,
-55.74995));
#187008=CARTESIAN_POINT('Ctrl Pts',(33.35,-65.6396495179854,-55.6186826543062));
#187009=CARTESIAN_POINT('Ctrl Pts',(33.3499999999488,-65.1814839309712,
-55.607847808877));
#187010=CARTESIAN_POINT('Ctrl Pts',(33.8064221285606,-65.1415521689398,
-55.487415308613));
#187011=CARTESIAN_POINT('Ctrl Pts',(33.2961134364373,-65.6490784448363,
-55.4889566552507));
#187012=CARTESIAN_POINT('Ctrl Pts',(33.2858662151155,-65.1870949100978,
-55.4680441063706));
#187013=CARTESIAN_POINT('Ctrl Pts',(33.6986490015007,-65.1509810957903,
-55.2279633105015));
#187014=CARTESIAN_POINT('Ctrl Pts',(33.1109933447493,-65.6814702636632,
-55.3038365635628));
#187015=CARTESIAN_POINT('Ctrl Pts',(33.0786175782532,-65.2052268163542,
-55.2822894538758));
#187016=CARTESIAN_POINT('Ctrl Pts',(33.3284088181247,-65.1833729146174,
-54.8577231271255));
#187017=CARTESIAN_POINT('Ctrl Pts',(32.981267345694,-65.704169372229,-55.24995));
#187018=CARTESIAN_POINT('Ctrl Pts',(32.9369589695398,-65.2176203387053,
-55.2386587236917));
#187019=CARTESIAN_POINT('Ctrl Pts',(33.0689568200132,-65.2060720231813,
-54.7499500000659));
#187020=CARTESIAN_POINT('Ctrl Pts',(32.85,-65.7271381815059,-55.24995));
#187021=CARTESIAN_POINT('Ctrl Pts',(32.8064221286261,-65.22904083246,-55.24995));
#187022=CARTESIAN_POINT('Ctrl Pts',(32.8064221286262,-65.22904083246,-54.74995));
#187023=CARTESIAN_POINT('',(32.8064221286262,-65.22904083246,-54.74995));
#187024=CARTESIAN_POINT('Origin',(32.85,-65.7271381815059,-54.74995));
#187025=CARTESIAN_POINT('Ctrl Pts',(32.8064221286262,-65.22904083246,-54.74995));
#187026=CARTESIAN_POINT('Ctrl Pts',(33.0689568200132,-65.2060720231813,
-54.7499500000659));
#187027=CARTESIAN_POINT('Ctrl Pts',(33.3284088181247,-65.1833729146174,
-54.8577231271255));
#187028=CARTESIAN_POINT('Ctrl Pts',(33.5135289098127,-65.1671770052039,
-55.0428432188135));
#187029=CARTESIAN_POINT('Ctrl Pts',(33.6986490015007,-65.1509810957903,
-55.2279633105015));
#187030=CARTESIAN_POINT('Ctrl Pts',(33.8064221285606,-65.1415521689398,
-55.487415308613));
#187031=CARTESIAN_POINT('Ctrl Pts',(33.8064221286261,-65.1415521689341,
-55.74995));
#187032=CARTESIAN_POINT('Origin',(44.2377516955329,-64.7308390050988,-54.74995));
#187033=CARTESIAN_POINT('',(32.3064221286262,-65.2727851642229,-54.74995));
#187034=CARTESIAN_POINT('Origin',(32.35,-65.7708825132688,-54.74995));
#187035=CARTESIAN_POINT('',(44.1941738241591,-64.2327416560529,-54.74995));
#187036=CARTESIAN_POINT('Ctrl Pts',(32.350023911586,-65.7709087028862,-55.2499499996829));
#187037=CARTESIAN_POINT('Ctrl Pts',(32.3064436723035,-65.2727832793954,
-55.2499781675672));
#187038=CARTESIAN_POINT('Ctrl Pts',(32.3064647172502,-65.2727814382011,
-54.7499500009454));
#187039=CARTESIAN_POINT('Ctrl Pts',(32.2187494539986,-65.7938791072894,
-55.2499434816087));
#187040=CARTESIAN_POINT('Ctrl Pts',(32.1720954901142,-65.2845372222937,
-55.2615949036257));
#187041=CARTESIAN_POINT('Ctrl Pts',(32.0439154964703,-65.2957515186369,
-54.7499383449276));
#187042=CARTESIAN_POINT('Ctrl Pts',(32.089013752819,-65.8165801641519,-55.3038301720448));
#187043=CARTESIAN_POINT('Ctrl Pts',(32.0533601275064,-65.2949252204907,
-55.327473556922));
#187044=CARTESIAN_POINT('Ctrl Pts',(31.7844454492387,-65.3184522062943,
-54.8577131170134));
#187045=CARTESIAN_POINT('Ctrl Pts',(31.9038822591064,-65.8489742655241,
-55.4889602509496));
#187046=CARTESIAN_POINT('Ctrl Pts',(31.891750054253,-65.3090642698107,-55.5134049012229));
#187047=CARTESIAN_POINT('Ctrl Pts',(31.4141852456405,-65.3508457766639,
-55.2279733206136));
#187048=CARTESIAN_POINT('Ctrl Pts',(31.8499941713763,-65.8584035047689,
-55.6186959323283));
#187049=CARTESIAN_POINT('Ctrl Pts',(31.8500296390451,-65.3127143331746,
-55.6318003689116));
#187050=CARTESIAN_POINT('Ctrl Pts',(31.3064104735534,-65.3602748474356,
-55.4874433678435));
#187051=CARTESIAN_POINT('Ctrl Pts',(31.8499999994923,-65.8584024879449,
-55.7499712944341));
#187052=CARTESIAN_POINT('Ctrl Pts',(31.850034171749,-65.3127139366194,-55.7499691665926));
#187053=CARTESIAN_POINT('Ctrl Pts',(31.3064221295715,-65.3602738276662,
-55.7499925886241));
#187054=CARTESIAN_POINT('',(31.3064221286262,-65.3602738277489,-55.74995));
#187055=CARTESIAN_POINT('Origin',(31.35,-65.8583711767947,-55.74995));
#187056=CARTESIAN_POINT('Ctrl Pts',(31.3064221286262,-65.3602738277489,
-55.74995));
#187057=CARTESIAN_POINT('Ctrl Pts',(31.3064221286917,-65.3602738277431,
-55.4874153086129));
#187058=CARTESIAN_POINT('Ctrl Pts',(31.4141952557525,-65.3508449008926,
-55.2279633105016));
#187059=CARTESIAN_POINT('Ctrl Pts',(31.5993153474396,-65.3346489914791,
-55.0428432188135));
#187060=CARTESIAN_POINT('Ctrl Pts',(31.7844354391267,-65.3184530820656,
-54.8577231271254));
#187061=CARTESIAN_POINT('Ctrl Pts',(32.0438874372397,-65.2957539735015,
-54.7499500000659));
#187062=CARTESIAN_POINT('Ctrl Pts',(32.3064221286262,-65.2727851642229,
-54.74995));
#187063=CARTESIAN_POINT('Origin',(31.35,-65.8583711767947,-52.64995));
#187064=CARTESIAN_POINT('',(31.3064221286262,-65.3602738277489,-52.64995));
#187065=CARTESIAN_POINT('Origin',(4.6996065532056,-66.6842487255793,-59.64995));
#187066=CARTESIAN_POINT('',(28.7021688185769,-65.588116469328,-59.64995));
#187067=CARTESIAN_POINT('',(44.1941738241591,-64.2327416560529,-59.64995));
#187068=CARTESIAN_POINT('Origin',(28.6150130758292,-64.5919217712362,-59.64995));
#187069=CARTESIAN_POINT('Ctrl Pts',(28.7021688185769,-65.588116469328,-59.64995));
#187070=CARTESIAN_POINT('Ctrl Pts',(28.7021688185769,-65.588116469328,-60.64995));
#187071=CARTESIAN_POINT('Ctrl Pts',(28.6150130758292,-64.5919217712362,
-60.64995));
#187072=CARTESIAN_POINT('Ctrl Pts',(28.1296330247306,-65.6382068607523,
-59.649950002333));
#187073=CARTESIAN_POINT('Ctrl Pts',(28.2033028175763,-65.6317615890315,
-60.5485267380177));
#187074=CARTESIAN_POINT('Ctrl Pts',(28.0991390263463,-64.7442358506513,
-60.64995));
#187075=CARTESIAN_POINT('Ctrl Pts',(27.5637794550765,-65.6877126333127,
-59.6897495968387));
#187076=CARTESIAN_POINT('Ctrl Pts',(27.6612478839793,-65.6791852507322,
-60.4928259381272));
#187077=CARTESIAN_POINT('Ctrl Pts',(27.584859681119,-64.89321892758,-60.6698497986403));
#187078=CARTESIAN_POINT('Ctrl Pts',(26.4448676457179,-65.7856047321169,
-59.8430005124393));
#187079=CARTESIAN_POINT('Ctrl Pts',(26.5839609508645,-65.7734356447442,
-60.477600868097));
#187080=CARTESIAN_POINT('Ctrl Pts',(26.5596543334024,-65.1843117452004,
-60.7464752559987));
#187081=CARTESIAN_POINT('Ctrl Pts',(25.8914156146746,-65.8340255106386,
-59.9553384305595));
#187082=CARTESIAN_POINT('Ctrl Pts',(26.0406038710994,-65.8209732294689,
-60.5097186566584));
#187083=CARTESIAN_POINT('Ctrl Pts',(26.0485518825385,-65.3264611076661,
-60.802611641644));
#187084=CARTESIAN_POINT('Ctrl Pts',(25.3471476467368,-65.8816427877534,
-60.1196878110938));
#187085=CARTESIAN_POINT('Ctrl Pts',(25.4903329393053,-65.86911569787,-60.5974971539929));
#187086=CARTESIAN_POINT('Ctrl Pts',(25.5416884892005,-65.4644312001072,
-60.8848189055469));
#187087=CARTESIAN_POINT('Ctrl Pts',(25.6564221266688,-65.8545847543119,
-60.0322609860537));
#187088=CARTESIAN_POINT('Ctrl Pts',(25.7808509976504,-65.8436986122353,
-59.9993769765733));
#187089=CARTESIAN_POINT('Ctrl Pts',(25.9056363008897,-65.8327812988126,
-59.9689324054821));
#187090=CARTESIAN_POINT('Ctrl Pts',(26.0307566852339,-65.8218346938133,
-59.9407811370796));
#187091=CARTESIAN_POINT('Ctrl Pts',(26.252037221755,-65.80247517346,-59.8909944631614));
#187092=CARTESIAN_POINT('Ctrl Pts',(26.4743884950002,-65.7830219799129,
-59.8484921029725));
#187093=CARTESIAN_POINT('Ctrl Pts',(26.6976513564849,-65.7634890172034,
-59.812264924346));
#187094=CARTESIAN_POINT('Ctrl Pts',(26.7996931166677,-65.7545615230236,
-59.7957073784607));
#187095=CARTESIAN_POINT('Ctrl Pts',(26.9019251840858,-65.7456173770713,
-59.7804614113611));
#187096=CARTESIAN_POINT('Ctrl Pts',(27.0043315823481,-65.7366579782249,
-59.7664341473284));
#187097=CARTESIAN_POINT('Ctrl Pts',(27.0579416473936,-65.7319677053213,
-59.7590908313837));
#187098=CARTESIAN_POINT('Ctrl Pts',(27.1116030957325,-65.7272729367138,
-59.7520917680714));
#187099=CARTESIAN_POINT('Ctrl Pts',(27.1653166053581,-65.7225736127227,
-59.7454407818489));
#187100=CARTESIAN_POINT('Ctrl Pts',(27.4668119230827,-65.696196185709,-59.7081086242909));
#187101=CARTESIAN_POINT('Ctrl Pts',(27.7698631240487,-65.6696826439597,
-59.6814497127403));
#187102=CARTESIAN_POINT('Ctrl Pts',(28.0745495814197,-65.6430260356534,
-59.665944037988));
#187103=CARTESIAN_POINT('Ctrl Pts',(28.2829846777418,-65.6247903294528,
-59.655336652158));
#187104=CARTESIAN_POINT('Ctrl Pts',(28.4921848717869,-65.6064876841945,
-59.6499500008557));
#187105=CARTESIAN_POINT('Ctrl Pts',(28.7021688185769,-65.588116469328,-59.64995));
#187106=CARTESIAN_POINT('Origin',(25.7,-66.3526821257161,-52.64995));
#187107=CARTESIAN_POINT('',(25.6564221286262,-65.8545847766702,-55.74995));
#187108=CARTESIAN_POINT('',(25.6564221286262,-65.8545847766702,-52.64995));
#187109=CARTESIAN_POINT('Origin',(25.7,-66.3526821257161,-55.74995));
#187110=CARTESIAN_POINT('Ctrl Pts',(25.2,-66.3526821257161,-55.74995));
#187111=CARTESIAN_POINT('Ctrl Pts',(25.2,-65.8945165387074,-55.74995));
#187112=CARTESIAN_POINT('Ctrl Pts',(25.6564221286262,-65.8545847766702,
-55.74995));
#187113=CARTESIAN_POINT('Ctrl Pts',(25.2,-66.3526821257202,-55.6520807487743));
#187114=CARTESIAN_POINT('Ctrl Pts',(25.1999999999616,-65.8945165387115,
-55.6441589529833));
#187115=CARTESIAN_POINT('Ctrl Pts',(25.6564221285773,-65.8545847766745,
-55.5542114975488));
#187116=CARTESIAN_POINT('Ctrl Pts',(25.1705210566577,-66.3578402724271,
-55.5545751632329));
#187117=CARTESIAN_POINT('Ctrl Pts',(25.1652351487286,-65.8975580690824,
-55.5387129880067));
#187118=CARTESIAN_POINT('Ctrl Pts',(25.5974642419416,-65.8597429233806,
-55.3592003264656));
#187119=CARTESIAN_POINT('Ctrl Pts',(25.062254236699,-66.3767845111906,-55.391713681917));
#187120=CARTESIAN_POINT('Ctrl Pts',(25.0420941082282,-65.9083315141418,
-55.3693682972756));
#187121=CARTESIAN_POINT('Ctrl Pts',(25.3809306020242,-65.8786871621453,
-55.033477363834));
#187122=CARTESIAN_POINT('Ctrl Pts',(24.9837596261582,-66.3905192883359,
-55.3267957976874));
#187123=CARTESIAN_POINT('Ctrl Pts',(24.9535760611327,-65.9160758397827,
-55.3059410651653));
#187124=CARTESIAN_POINT('Ctrl Pts',(25.2239370702218,-65.892422316425,-54.9036397860402));
#187125=CARTESIAN_POINT('Ctrl Pts',(24.8935146892254,-66.4063101061761,
-55.2889163081141));
#187126=CARTESIAN_POINT('Ctrl Pts',(24.8576734148988,-65.9244662341272,
-55.273872259957));
#187127=CARTESIAN_POINT('Ctrl Pts',(25.043451507077,-65.9082127571302,-54.8278826162281));
#187128=CARTESIAN_POINT('',(25.043451507077,-65.9082127571302,-54.8278826162281));
#187129=CARTESIAN_POINT('Origin',(25.0870293784509,-66.4063101061761,-54.8278826162281));
#187130=CARTESIAN_POINT('Ctrl Pts',(25.043451507077,-65.9082127571302,-54.8278826162281));
#187131=CARTESIAN_POINT('Ctrl Pts',(25.0742713040834,-65.90551637428,-54.8408189450663));
#187132=CARTESIAN_POINT('Ctrl Pts',(25.104915072702,-65.9028353919181,-54.8555499531048));
#187133=CARTESIAN_POINT('Ctrl Pts',(25.1350929986057,-65.9001951655129,
-54.8720618327809));
#187134=CARTESIAN_POINT('Ctrl Pts',(25.1657431004607,-65.8975136290646,
-54.8888320639594));
#187135=CARTESIAN_POINT('Ctrl Pts',(25.1959121242359,-65.8948741814946,
-54.9074392518001));
#187136=CARTESIAN_POINT('Ctrl Pts',(25.2252929736523,-65.892303690246,-54.9278152010716));
#187137=CARTESIAN_POINT('Ctrl Pts',(25.2553889373856,-65.8896706346014,
-54.9486870901588));
#187138=CARTESIAN_POINT('Ctrl Pts',(25.2846571909018,-65.8871099942175,
-54.9714147499623));
#187139=CARTESIAN_POINT('Ctrl Pts',(25.3127736146752,-65.8846501258785,
-54.9958704922167));
#187140=CARTESIAN_POINT('Ctrl Pts',(25.3411372062356,-65.88216863316,-55.0205412216878));
#187141=CARTESIAN_POINT('Ctrl Pts',(25.3683278367126,-65.8797897612392,
-55.0469701419947));
#187142=CARTESIAN_POINT('Ctrl Pts',(25.3940301284273,-65.8775411020875,
-55.0749758606088));
#187143=CARTESIAN_POINT('Ctrl Pts',(25.4197097931075,-65.8752944225448,
-55.1029569243646));
#187144=CARTESIAN_POINT('Ctrl Pts',(25.4439029560561,-65.873177795052,-55.1325114406684));
#187145=CARTESIAN_POINT('Ctrl Pts',(25.4663241567112,-65.871216194172,-55.1634160027496));
#187146=CARTESIAN_POINT('Ctrl Pts',(25.4741688835925,-65.8705298695015,
-55.1742288870657));
#187147=CARTESIAN_POINT('Ctrl Pts',(25.4817970097154,-65.8698624949418,
-55.1852066986187));
#187148=CARTESIAN_POINT('Ctrl Pts',(25.4891974219829,-65.869215042763,-55.1963388451498));
#187149=CARTESIAN_POINT('Ctrl Pts',(25.510338242743,-65.8673654606088,-55.228140142967));
#187150=CARTESIAN_POINT('Ctrl Pts',(25.5295950731415,-65.8656807062535,
-55.2611692657123));
#187151=CARTESIAN_POINT('Ctrl Pts',(25.5468557307134,-65.864170594391,-55.295083999148));
#187152=CARTESIAN_POINT('Ctrl Pts',(25.5641515040968,-65.862657410293,-55.3290677301512));
#187153=CARTESIAN_POINT('Ctrl Pts',(25.5794427196934,-65.8613196022768,
-55.363939731283));
#187154=CARTESIAN_POINT('Ctrl Pts',(25.5926659905796,-65.8601627159795,
-55.3993402855053));
#187155=CARTESIAN_POINT('Ctrl Pts',(25.6056853291763,-65.8590236714457,
-55.4341948843334));
#187156=CARTESIAN_POINT('Ctrl Pts',(25.6166999804352,-65.8580600143278,
-55.4695609780295));
#187157=CARTESIAN_POINT('Ctrl Pts',(25.6256992872677,-65.8572726770004,
-55.5050939643816));
#187158=CARTESIAN_POINT('Ctrl Pts',(25.6345695399044,-65.8564966304521,
-55.5401173913793));
#187159=CARTESIAN_POINT('Ctrl Pts',(25.641481865841,-65.855891880294,-55.5753022272925));
#187160=CARTESIAN_POINT('Ctrl Pts',(25.6464749038184,-65.8554550460744,
-55.6103291116175));
#187161=CARTESIAN_POINT('Ctrl Pts',(25.6513699614093,-65.8550267840279,
-55.6446686493459));
#187162=CARTESIAN_POINT('Ctrl Pts',(25.6544204578572,-65.8547599001706,
-55.6788558270728));
#187163=CARTESIAN_POINT('Ctrl Pts',(25.6557087574904,-65.8546471885575,
-55.7126093508298));
#187164=CARTESIAN_POINT('Ctrl Pts',(25.6561862637138,-65.8546054121762,
-55.7251200410772));
#187165=CARTESIAN_POINT('Ctrl Pts',(25.6564221286231,-65.8545847766705,
-55.7375713926724));
#187166=CARTESIAN_POINT('Ctrl Pts',(25.6564221286262,-65.8545847766702,
-55.74995));
#187167=CARTESIAN_POINT('Origin',(4.6996065532056,-66.6842487255793,-59.64995));
#187168=CARTESIAN_POINT('',(43.1064181712415,-64.3279079443695,-59.64995));
#187169=CARTESIAN_POINT('',(44.1941738241591,-64.2327416560529,-59.64995));
#187170=CARTESIAN_POINT('Origin',(43.0192624284939,-63.3317132462777,-59.64995));
#187171=CARTESIAN_POINT('Origin',(42.,-64.9266169102438,-52.64995));
#187172=CARTESIAN_POINT('',(41.9564221286262,-64.428519561198,-55.74995));
#187173=CARTESIAN_POINT('Origin',(42.,-64.9266169102438,-55.74995));
#187174=CARTESIAN_POINT('',(41.9564221286262,-64.428519561198,-52.64995));
#187175=CARTESIAN_POINT('Ctrl Pts',(41.5,-64.9266169102438,-55.74995));
#187176=CARTESIAN_POINT('Ctrl Pts',(41.5,-64.4684513232351,-55.74995));
#187177=CARTESIAN_POINT('Ctrl Pts',(41.9564221286262,-64.428519561198,-55.74995));
#187178=CARTESIAN_POINT('Ctrl Pts',(41.5,-64.9266169102493,-55.6186826543063));
#187179=CARTESIAN_POINT('Ctrl Pts',(41.4999999999489,-64.4684513232351,
-55.6078478088783));
#187180=CARTESIAN_POINT('Ctrl Pts',(41.9564221285606,-64.4285195612037,
-55.487415308613));
#187181=CARTESIAN_POINT('Ctrl Pts',(41.4461134364372,-64.9360458371002,
-55.4889566552508));
#187182=CARTESIAN_POINT('Ctrl Pts',(41.4358662151155,-64.4740623023634,
-55.4680441063688));
#187183=CARTESIAN_POINT('Ctrl Pts',(41.8486490015007,-64.4379484880542,
-55.2279633105015));
#187184=CARTESIAN_POINT('Ctrl Pts',(41.2609933447493,-64.9684376559271,
-55.3038365635627));
#187185=CARTESIAN_POINT('Ctrl Pts',(41.2286175782531,-64.4921942086162,
-55.2822894538775));
#187186=CARTESIAN_POINT('Ctrl Pts',(41.4784088181247,-64.4703403068813,
-54.8577231271255));
#187187=CARTESIAN_POINT('Ctrl Pts',(41.1312673456941,-64.991136764493,-55.24995));
#187188=CARTESIAN_POINT('Ctrl Pts',(41.0869589695398,-64.5045877309693,
-55.2386587236917));
#187189=CARTESIAN_POINT('Ctrl Pts',(41.2189568200132,-64.4930394154452,
-54.7499500000659));
#187190=CARTESIAN_POINT('Ctrl Pts',(41.,-65.0141055737697,-55.24995));
#187191=CARTESIAN_POINT('Ctrl Pts',(40.9564221286262,-64.5160082247238,
-55.24995));
#187192=CARTESIAN_POINT('Ctrl Pts',(40.9564221286262,-64.5160082247239,
-54.74995));
#187193=CARTESIAN_POINT('',(40.9564221286262,-64.5160082247239,-54.74995));
#187194=CARTESIAN_POINT('Origin',(41.,-65.0141055737697,-54.74995));
#187195=CARTESIAN_POINT('Ctrl Pts',(40.9564221286262,-64.5160082247239,
-54.74995));
#187196=CARTESIAN_POINT('Ctrl Pts',(41.2189568200132,-64.4930394154452,
-54.7499500000659));
#187197=CARTESIAN_POINT('Ctrl Pts',(41.4784088181247,-64.4703403068813,
-54.8577231271255));
#187198=CARTESIAN_POINT('Ctrl Pts',(41.6635289098127,-64.4541443974678,
-55.0428432188135));
#187199=CARTESIAN_POINT('Ctrl Pts',(41.8486490015007,-64.4379484880542,
-55.2279633105015));
#187200=CARTESIAN_POINT('Ctrl Pts',(41.9564221285606,-64.4285195612037,
-55.487415308613));
#187201=CARTESIAN_POINT('Ctrl Pts',(41.9564221286262,-64.428519561198,-55.74995));
#187202=CARTESIAN_POINT('Origin',(44.2377516955329,-64.7308390050988,-54.74995));
#187203=CARTESIAN_POINT('',(40.4564221286262,-64.5597525564868,-54.74995));
#187204=CARTESIAN_POINT('Origin',(40.5,-65.0578499055327,-54.74995));
#187205=CARTESIAN_POINT('',(44.1941738241591,-64.2327416560529,-54.74995));
#187206=CARTESIAN_POINT('Ctrl Pts',(40.5000239115806,-65.0578760951442,
-55.2499499996828));
#187207=CARTESIAN_POINT('Ctrl Pts',(40.4564436722986,-64.5597506716597,
-55.2499781675608));
#187208=CARTESIAN_POINT('Ctrl Pts',(40.4564647172406,-64.5597488304658,
-54.7499500009454));
#187209=CARTESIAN_POINT('Ctrl Pts',(40.3687494539948,-65.080846499547,-55.2499434816101));
#187210=CARTESIAN_POINT('Ctrl Pts',(40.3220954901096,-64.571504614558,-55.2615949036203));
#187211=CARTESIAN_POINT('Ctrl Pts',(40.1939154964641,-64.5827189109014,
-54.7499383449302));
#187212=CARTESIAN_POINT('Ctrl Pts',(40.2390137528174,-65.1035475564089,
-55.3038301720462));
#187213=CARTESIAN_POINT('Ctrl Pts',(40.2033601275017,-64.581892612755,-55.3274735569167));
#187214=CARTESIAN_POINT('Ctrl Pts',(39.9344454492365,-64.6054195985583,
-54.8577131170157));
#187215=CARTESIAN_POINT('Ctrl Pts',(40.0538822591073,-65.1359416577808,
-55.4889602509488));
#187216=CARTESIAN_POINT('Ctrl Pts',(40.0417500542473,-64.5960316620751,
-55.5134049012177));
#187217=CARTESIAN_POINT('Ctrl Pts',(39.5641852456427,-64.6378131689275,
-55.2279733206113));
#187218=CARTESIAN_POINT('Ctrl Pts',(39.9999941713776,-65.1453708970254,
-55.6186959323252));
#187219=CARTESIAN_POINT('Ctrl Pts',(40.0000296390384,-64.5996817254391,
-55.6318003689066));
#187220=CARTESIAN_POINT('Ctrl Pts',(39.456410473556,-64.6472422396993,-55.4874433678372));
#187221=CARTESIAN_POINT('Ctrl Pts',(39.9999999994923,-65.1453698802017,
-55.7499712944293));
#187222=CARTESIAN_POINT('Ctrl Pts',(40.0000341717414,-64.5996813288839,
-55.7499691665883));
#187223=CARTESIAN_POINT('Ctrl Pts',(39.4564221295715,-64.64724121993,-55.7499925886145));
#187224=CARTESIAN_POINT('',(39.4564221286262,-64.6472412200127,-55.74995));
#187225=CARTESIAN_POINT('Origin',(39.5,-65.1453385690586,-55.74995));
#187226=CARTESIAN_POINT('Ctrl Pts',(39.4564221286262,-64.6472412200127,
-55.74995));
#187227=CARTESIAN_POINT('Ctrl Pts',(39.4564221286917,-64.647241220007,-55.4874153086129));
#187228=CARTESIAN_POINT('Ctrl Pts',(39.5641952557525,-64.6378122931564,
-55.2279633105016));
#187229=CARTESIAN_POINT('Ctrl Pts',(39.7493153474396,-64.6216163837429,
-55.0428432188135));
#187230=CARTESIAN_POINT('Ctrl Pts',(39.9344354391268,-64.6054204743294,
-54.8577231271254));
#187231=CARTESIAN_POINT('Ctrl Pts',(40.1938874372398,-64.5827213657654,
-54.7499500000659));
#187232=CARTESIAN_POINT('Ctrl Pts',(40.4564221286262,-64.5597525564868,
-54.74995));
#187233=CARTESIAN_POINT('Origin',(39.5,-65.1453385690586,-52.64995));
#187234=CARTESIAN_POINT('',(39.4564221286262,-64.6472412200127,-52.64995));
#187235=CARTESIAN_POINT('Origin',(4.6996065532056,-66.6842487255793,-59.64995));
#187236=CARTESIAN_POINT('',(44.1941738241591,-64.2327416560529,-59.64995));
#187237=CARTESIAN_POINT('Ctrl Pts',(53.7823432375846,11.067884690566,-55.2526734204115));
#187238=CARTESIAN_POINT('Ctrl Pts',(53.3054454943535,10.8575310968505,-55.2747187747876));
#187239=CARTESIAN_POINT('Ctrl Pts',(53.3256899305368,10.8121330655672,-54.7553968408231));
#187240=CARTESIAN_POINT('Ctrl Pts',(53.8861362179292,10.9515071084652,-55.2648699557477));
#187241=CARTESIAN_POINT('Ctrl Pts',(53.3650311600591,10.7244739426765,-55.3417466734359));
#187242=CARTESIAN_POINT('Ctrl Pts',(53.4285862862346,10.5813885818665,-54.7797862992586));
#187243=CARTESIAN_POINT('Ctrl Pts',(53.9838097653667,10.83974934456,-55.3179449795228));
#187244=CARTESIAN_POINT('Ctrl Pts',(53.3983781597441,10.6502596450882,-55.4540676493459));
#187245=CARTESIAN_POINT('Ctrl Pts',(53.5254458539065,10.3597364405483,-54.885939939012));
#187246=CARTESIAN_POINT('Ctrl Pts',(54.0930825652429,10.7133083132261,-55.4526385853652));
#187247=CARTESIAN_POINT('Ctrl Pts',(53.4176451441909,10.6111056725941,-55.596678279911));
#187248=CARTESIAN_POINT('Ctrl Pts',(53.633790842791,10.1090015716016,-55.1553271807471));
#187249=CARTESIAN_POINT('Ctrl Pts',(54.1219468150851,10.6796458924645,-55.5047178594674));
#187250=CARTESIAN_POINT('Ctrl Pts',(53.4186534680994,10.6106295502708,-55.6378844781733));
#187251=CARTESIAN_POINT('Ctrl Pts',(53.6624100137865,10.0422483461928,-55.2594857136242));
#187252=CARTESIAN_POINT('Ctrl Pts',(54.1624914359772,10.6322531187842,-55.6228534833935));
#187253=CARTESIAN_POINT('Ctrl Pts',(53.4178589543304,10.6154785181549,-55.7046481866627));
#187254=CARTESIAN_POINT('Ctrl Pts',(53.702610379063,9.94826762670561,-55.4957569720976));
#187255=CARTESIAN_POINT('Ctrl Pts',(54.172917586547,10.61999998,-55.685050712911));
#187256=CARTESIAN_POINT('Ctrl Pts',(53.4163125940233,10.619999979359,-55.7271468411276));
#187257=CARTESIAN_POINT('Ctrl Pts',(53.7129480039811,9.9239694167493,-55.6201514218302));
#187258=CARTESIAN_POINT('Ctrl Pts',(54.1729175880533,10.61999998,-55.74995));
#187259=CARTESIAN_POINT('Ctrl Pts',(53.4163125938068,10.61999998,-55.74995));
#187260=CARTESIAN_POINT('Ctrl Pts',(53.7129480054761,9.92396941324122,-55.74995));
#187261=CARTESIAN_POINT('',(53.3256899305368,10.8121330655672,-54.7553968408231));
#187262=CARTESIAN_POINT('Origin',(53.7823432375846,11.015769401132,-54.7553968408231));
#187263=CARTESIAN_POINT('',(53.7129480054761,9.92396941324122,-55.74995));
#187264=CARTESIAN_POINT('Ctrl Pts',(53.7129480054761,9.92396941324122,-55.74995));
#187265=CARTESIAN_POINT('Ctrl Pts',(53.7129480048637,9.92396941467835,-55.6967763512781));
#187266=CARTESIAN_POINT('Ctrl Pts',(53.7112147843802,9.92804334268761,-55.6443923193454));
#187267=CARTESIAN_POINT('Ctrl Pts',(53.7077550226655,9.93615769838508,-55.5927930680038));
#187268=CARTESIAN_POINT('Ctrl Pts',(53.7070427178468,9.93782830322472,-55.582169678763));
#187269=CARTESIAN_POINT('Ctrl Pts',(53.7062571614758,9.93967032838863,-55.57157960177));
#187270=CARTESIAN_POINT('Ctrl Pts',(53.7053983076824,9.94168372171603,-55.5610228702942));
#187271=CARTESIAN_POINT('Ctrl Pts',(53.7036268526,9.9458365075222,-55.5392487618595));
#187272=CARTESIAN_POINT('Ctrl Pts',(53.7015273912866,9.9507562630614,-55.5174450002407));
#187273=CARTESIAN_POINT('Ctrl Pts',(53.6991098272624,9.95641828381884,-55.4957961558367));
#187274=CARTESIAN_POINT('Ctrl Pts',(53.6966689320685,9.96213494700362,-55.473938385069));
#187275=CARTESIAN_POINT('Ctrl Pts',(53.693903757809,9.96860827125173,-55.452238612997));
#187276=CARTESIAN_POINT('Ctrl Pts',(53.6908450504304,9.9757648499092,-55.4308742653829));
#187277=CARTESIAN_POINT('Ctrl Pts',(53.6883304010962,9.98164847443693,-55.4133100345323));
#187278=CARTESIAN_POINT('Ctrl Pts',(53.6856177574555,9.98799296192938,-55.3959722863425));
#187279=CARTESIAN_POINT('Ctrl Pts',(53.6827342900112,9.99473409341425,-55.3789529390801));
#187280=CARTESIAN_POINT('Ctrl Pts',(53.6826591797317,9.99490969042721,-55.3785096089732));
#187281=CARTESIAN_POINT('Ctrl Pts',(53.6825839300607,9.9950856114844,-55.378066355819));
#187282=CARTESIAN_POINT('Ctrl Pts',(53.682508540985,9.99526185660251,-55.3776231795372));
#187283=CARTESIAN_POINT('Ctrl Pts',(53.6757958049232,10.0109549387852,-55.3381622180861));
#187284=CARTESIAN_POINT('Ctrl Pts',(53.6681180133557,10.0288871912831,-55.3001692589446));
#187285=CARTESIAN_POINT('Ctrl Pts',(53.6594755760649,10.0490364743368,-55.2635974761426));
#187286=CARTESIAN_POINT('Ctrl Pts',(53.6554675883568,10.0583808382114,-55.2466370689097));
#187287=CARTESIAN_POINT('Ctrl Pts',(53.6512518906864,10.0682025695934,-55.2299827533854));
#187288=CARTESIAN_POINT('Ctrl Pts',(53.6468273042282,10.07850218353,-55.2136321846475));
#187289=CARTESIAN_POINT('Ctrl Pts',(53.6421181547434,10.0894642072407,-55.1962300447914));
#187290=CARTESIAN_POINT('Ctrl Pts',(53.637124495453,10.1010789815322,-55.1790043701209));
#187291=CARTESIAN_POINT('Ctrl Pts',(53.6318875227673,10.1132475345242,-55.1621368610288));
#187292=CARTESIAN_POINT('Ctrl Pts',(53.626579315431,10.1255816073064,-55.1450399157357));
#187293=CARTESIAN_POINT('Ctrl Pts',(53.6210211374223,10.1384845723914,-55.1283110733852));
#187294=CARTESIAN_POINT('Ctrl Pts',(53.6152735870561,10.1518130379855,-55.1121076745932));
#187295=CARTESIAN_POINT('Ctrl Pts',(53.609746478553,10.1646303028765,-55.0965257418503));
#187296=CARTESIAN_POINT('Ctrl Pts',(53.604044430579,10.1778406037002,-55.0814294938097));
#187297=CARTESIAN_POINT('Ctrl Pts',(53.5982359111103,10.1912837029229,-55.0669307798463));
#187298=CARTESIAN_POINT('Ctrl Pts',(53.5980491569954,10.1917159222018,-55.0664646206972));
#187299=CARTESIAN_POINT('Ctrl Pts',(53.5978622041318,10.1921485874913,-55.065998854503));
#187300=CARTESIAN_POINT('Ctrl Pts',(53.5976750524344,10.1925816989101,-55.0655334806687));
#187301=CARTESIAN_POINT('Ctrl Pts',(53.5876493716261,10.2157833951786,-55.0406034929458));
#187302=CARTESIAN_POINT('Ctrl Pts',(53.5771573605076,10.2400161971565,-55.0171039053591));
#187303=CARTESIAN_POINT('Ctrl Pts',(53.5662062859971,10.2652563708093,-54.9949777152844));
#187304=CARTESIAN_POINT('Ctrl Pts',(53.5578688397943,10.2844726212124,-54.9781322523811));
#187305=CARTESIAN_POINT('Ctrl Pts',(53.5492649777567,10.3042735113455,-54.9620836922876));
#187306=CARTESIAN_POINT('Ctrl Pts',(53.5403934613312,10.3246581340979,-54.9468240992755));
#187307=CARTESIAN_POINT('Ctrl Pts',(53.5325206041197,10.3427480768479,-54.9332822659373));
#187308=CARTESIAN_POINT('Ctrl Pts',(53.5243691543248,10.3614533780027,-54.9202518509527));
#187309=CARTESIAN_POINT('Ctrl Pts',(53.5160082521778,10.3806116918597,-54.9078854214808));
#187310=CARTESIAN_POINT('Ctrl Pts',(53.5133554582639,10.3866903491033,-54.9039617313978));
#187311=CARTESIAN_POINT('Ctrl Pts',(53.5106816795215,10.3928143899775,-54.9001045739724));
#187312=CARTESIAN_POINT('Ctrl Pts',(53.5079893939122,10.3989780408986,-54.8963179394496));
#187313=CARTESIAN_POINT('Ctrl Pts',(53.499437108409,10.4185574281069,-54.8842893569607));
#187314=CARTESIAN_POINT('Ctrl Pts',(53.4907041389291,10.4385224734264,-54.8729481962707));
#187315=CARTESIAN_POINT('Ctrl Pts',(53.4818760853353,10.458675248751,-54.8623971539524));
#187316=CARTESIAN_POINT('Ctrl Pts',(53.479166060809,10.464861721774,-54.8591582085658));
#187317=CARTESIAN_POINT('Ctrl Pts',(53.4764471557122,10.4710657164826,-54.8559933977348));
#187318=CARTESIAN_POINT('Ctrl Pts',(53.4737220448059,10.4772810900949,-54.8529048290228));
#187319=CARTESIAN_POINT('Ctrl Pts',(53.4607634882216,10.5068366837629,-54.8382179433156));
#187320=CARTESIAN_POINT('Ctrl Pts',(53.4475736911319,10.536857104021,-54.8251456815363));
#187321=CARTESIAN_POINT('Ctrl Pts',(53.4341586380481,10.5673216564299,-54.8136257598735));
#187322=CARTESIAN_POINT('Ctrl Pts',(53.420641509875,10.5980180135051,-54.8020181831695));
#187323=CARTESIAN_POINT('Ctrl Pts',(53.406895419264,10.6291659382345,-54.7919864990641));
#187324=CARTESIAN_POINT('Ctrl Pts',(53.3929173025913,10.6607631354219,-54.7835158564423));
#187325=CARTESIAN_POINT('Ctrl Pts',(53.379019678782,10.6921783804239,-54.7750939919424));
#187326=CARTESIAN_POINT('Ctrl Pts',(53.3648924224103,10.7240383998955,-54.7682151279967));
#187327=CARTESIAN_POINT('Ctrl Pts',(53.3505275116743,10.756349667385,-54.7629146804316));
#187328=CARTESIAN_POINT('Ctrl Pts',(53.3423264209277,10.7747965371003,-54.7598885946954));
#187329=CARTESIAN_POINT('Ctrl Pts',(53.3340477989169,10.7933905939691,-54.7573779011054));
#187330=CARTESIAN_POINT('Ctrl Pts',(53.3256899305368,10.8121330655672,-54.7553968408231));
#187331=CARTESIAN_POINT('Origin',(54.1729175880533,10.11999998,-55.74995));
#187332=CARTESIAN_POINT('Origin',(54.1729175880533,10.11999998,-55.24995));
#187333=CARTESIAN_POINT('',(53.7129480054761,9.92396941324122,-55.24995));
#187334=CARTESIAN_POINT('Origin',(0.,-12.9675000200281,-60.42825533736));
#187335=CARTESIAN_POINT('Origin',(0.,-12.9675000200281,-60.42825533736));
#187336=CARTESIAN_POINT('Origin',(56.2465221147258,4.46999998000001,-55.24995));
#187337=CARTESIAN_POINT('',(55.7689460407313,4.32194224278905,-55.74995));
#187338=CARTESIAN_POINT('',(55.7689460407313,4.32194224278906,-55.24995));
#187339=CARTESIAN_POINT('Origin',(56.2465221147258,4.46999998000001,-55.74995));
#187340=CARTESIAN_POINT('Ctrl Pts',(56.2518760188067,3.96334729621203,-55.8294468689166));
#187341=CARTESIAN_POINT('Ctrl Pts',(55.8813420564174,3.95911837961328,-55.8475485519145));
#187342=CARTESIAN_POINT('Ctrl Pts',(55.7730598430189,4.30872548228013,-55.9090619298413));
#187343=CARTESIAN_POINT('Ctrl Pts',(56.2421124760699,3.97898568412623,-55.7377933134847));
#187344=CARTESIAN_POINT('Ctrl Pts',(55.8742327966825,3.9826937870183,-55.7356483282311));
#187345=CARTESIAN_POINT('Ctrl Pts',(55.7633830612446,4.33978792174147,-55.7256225368045));
#187346=CARTESIAN_POINT('Ctrl Pts',(56.2498472169413,3.96666903650799,-55.6406903017816));
#187347=CARTESIAN_POINT('Ctrl Pts',(55.8800704582515,3.96340574722032,-55.6138694439694));
#187348=CARTESIAN_POINT('Ctrl Pts',(55.7710496378194,4.31531871748535,-55.5312554109142));
#187349=CARTESIAN_POINT('Ctrl Pts',(56.2881583747582,3.90468933699336,-55.494132859849));
#187350=CARTESIAN_POINT('Ctrl Pts',(55.9066278983059,3.87472424751448,-55.4413052836556));
#187351=CARTESIAN_POINT('Ctrl Pts',(55.8090161453349,4.19224220492976,-55.2379754767005));
#187352=CARTESIAN_POINT('Ctrl Pts',(56.3116282654917,3.86659531774519,-55.4385935578195));
#187353=CARTESIAN_POINT('Ctrl Pts',(55.9229328254989,3.82012971028789,-55.3788565241339));
#187354=CARTESIAN_POINT('Ctrl Pts',(55.832275617124,4.11659879830721,-55.1268557913785));
#187355=CARTESIAN_POINT('Ctrl Pts',(56.3681986096508,3.77376027759107,-55.34750757013));
#187356=CARTESIAN_POINT('Ctrl Pts',(55.9604473236213,3.69364022912991,-55.2864718145835));
#187357=CARTESIAN_POINT('Ctrl Pts',(55.888335440433,3.9323045563208,-54.9446837986715));
#187358=CARTESIAN_POINT('Ctrl Pts',(56.4017509144347,3.71825300770064,-55.3112107227452));
#187359=CARTESIAN_POINT('Ctrl Pts',(55.9821791809102,3.61993921542383,-55.2561026101603));
#187360=CARTESIAN_POINT('Ctrl Pts',(55.9215848671782,3.82212901679781,-54.8721313715614));
#187361=CARTESIAN_POINT('Ctrl Pts',(56.4868459075913,3.57562280381526,-55.2530405928642));
#187362=CARTESIAN_POINT('Ctrl Pts',(56.0342869816528,3.44212912761038,-55.2238841518077));
#187363=CARTESIAN_POINT('Ctrl Pts',(56.005908358045,3.53910658458787,-54.7559557018408));
#187364=CARTESIAN_POINT('Ctrl Pts',(56.5418624571477,3.48194475398672,-55.2416519066958));
#187365=CARTESIAN_POINT('Ctrl Pts',(56.0654069380446,3.33499954426141,-55.2402241631574));
#187366=CARTESIAN_POINT('Ctrl Pts',(56.0604196755096,3.35329673808427,-54.7333414930262));
#187367=CARTESIAN_POINT('Ctrl Pts',(56.592425919442,3.39399197445088,-55.2560492201736));
#187368=CARTESIAN_POINT('Ctrl Pts',(56.0890816376392,3.25347227784392,-55.2795842141493));
#187369=CARTESIAN_POINT('Ctrl Pts',(56.110520856671,3.17891193839818,-54.7622758815643));
#187370=CARTESIAN_POINT('',(56.066723956657,3.33043300908072,-54.74995));
#187371=CARTESIAN_POINT('Ctrl Pts',(56.0667239566569,3.33043300908083,-54.74995));
#187372=CARTESIAN_POINT('Ctrl Pts',(56.054810110711,3.3714179800412,-54.7499500048111));
#187373=CARTESIAN_POINT('Ctrl Pts',(56.0428719096527,3.41230937921189,-54.7525736247989));
#187374=CARTESIAN_POINT('Ctrl Pts',(56.0309991957517,3.45281789175017,-54.7576881483825));
#187375=CARTESIAN_POINT('Ctrl Pts',(56.0183308037643,3.49604117835013,-54.7631454338967));
#187376=CARTESIAN_POINT('Ctrl Pts',(56.0057365602009,3.53882993079309,-54.7714383768922));
#187377=CARTESIAN_POINT('Ctrl Pts',(55.9933214348628,3.58084263808004,-54.7824678791719));
#187378=CARTESIAN_POINT('Ctrl Pts',(55.9809063095247,3.62285534536699,-54.7934973814515));
#187379=CARTESIAN_POINT('Ctrl Pts',(55.9686698102716,3.66409363256126,-54.8072637702972));
#187380=CARTESIAN_POINT('Ctrl Pts',(55.9567198801064,3.70420224798085,-54.8237268632943));
#187381=CARTESIAN_POINT('Ctrl Pts',(55.9565878111619,3.70464552274758,-54.8239088110787));
#187382=CARTESIAN_POINT('Ctrl Pts',(55.9564557655643,3.70508869905399,-54.8240911044694));
#187383=CARTESIAN_POINT('Ctrl Pts',(55.9563237434519,3.70553177648158,-54.8242737432782));
#187384=CARTESIAN_POINT('Ctrl Pts',(55.9343635745757,3.77923196927894,-54.8546533441933));
#187385=CARTESIAN_POINT('Ctrl Pts',(55.9131570004002,3.84984800741946,-54.8944556864574));
#187386=CARTESIAN_POINT('Ctrl Pts',(55.8935222184455,3.91485853316083,-54.9422511775329));
#187387=CARTESIAN_POINT('Ctrl Pts',(55.8818370634331,3.95354794017741,-54.970695482308));
#187388=CARTESIAN_POINT('Ctrl Pts',(55.8707083955309,3.99025269895495,-55.0019703122245));
#187389=CARTESIAN_POINT('Ctrl Pts',(55.8603061323666,4.02444969307579,-55.0357720069019));
#187390=CARTESIAN_POINT('Ctrl Pts',(55.8601552265094,4.02494578961079,-55.0362623688194));
#187391=CARTESIAN_POINT('Ctrl Pts',(55.8600044604701,4.02544140270094,-55.0367533059883));
#187392=CARTESIAN_POINT('Ctrl Pts',(55.859853834661,4.02593653113584,-55.0372448169564));
#187393=CARTESIAN_POINT('Ctrl Pts',(55.8409688317124,4.0880142189489,-55.0988689578539));
#187394=CARTESIAN_POINT('Ctrl Pts',(55.8242867117939,4.14247853961686,-55.1695258968661));
#187395=CARTESIAN_POINT('Ctrl Pts',(55.8106050241011,4.1869905311094,-55.2464345690386));
#187396=CARTESIAN_POINT('Ctrl Pts',(55.8040947258896,4.20817112995892,-55.2830308137518));
#187397=CARTESIAN_POINT('Ctrl Pts',(55.7982636966349,4.22709855295217,-55.3210433783436));
#187398=CARTESIAN_POINT('Ctrl Pts',(55.7931974644892,4.24352182478376,-55.3601764970326));
#187399=CARTESIAN_POINT('Ctrl Pts',(55.7931360049005,4.24372105914634,-55.3606512295973));
#187400=CARTESIAN_POINT('Ctrl Pts',(55.7930746570768,4.24391992824448,-55.3611261391855));
#187401=CARTESIAN_POINT('Ctrl Pts',(55.7930134210752,4.24411843191566,-55.3616012250647));
#187402=CARTESIAN_POINT('Ctrl Pts',(55.7885029443904,4.25873967037657,-55.3965947538371));
#187403=CARTESIAN_POINT('Ctrl Pts',(55.7846130556769,4.27133328431391,-55.4324278680426));
#187404=CARTESIAN_POINT('Ctrl Pts',(55.7813486835249,4.28189251196921,-55.4689029452562));
#187405=CARTESIAN_POINT('Ctrl Pts',(55.7780780325758,4.2924720495779,-55.5054481797902));
#187406=CARTESIAN_POINT('Ctrl Pts',(55.775435211876,4.30100963982806,-55.5426389688294));
#187407=CARTESIAN_POINT('Ctrl Pts',(55.7734395025711,4.30745180750473,-55.5802948673857));
#187408=CARTESIAN_POINT('Ctrl Pts',(55.7714984886898,4.31371741785941,-55.6169187492451));
#187409=CARTESIAN_POINT('Ctrl Pts',(55.7701695736421,4.31800094942098,-55.6539836247096));
#187410=CARTESIAN_POINT('Ctrl Pts',(55.7694848260442,4.32020701122525,-55.6913249513655));
#187411=CARTESIAN_POINT('Ctrl Pts',(55.7691277073319,4.32135754604051,-55.7107996987557));
#187412=CARTESIAN_POINT('Ctrl Pts',(55.7689460418115,4.32194223930484,-55.7303495724289));
#187413=CARTESIAN_POINT('Ctrl Pts',(55.7689460407313,4.32194224278906,-55.74995));
#187414=CARTESIAN_POINT('Origin',(56.5468500449175,3.46999998000001,-54.74995));
#187415=CARTESIAN_POINT('Origin',(0.,-12.9675000200281,-54.74995));
#187416=CARTESIAN_POINT('',(56.208463007634,2.83467839222654,-54.74995));
#187417=CARTESIAN_POINT('Origin',(0.,-12.9675000200281,-54.74995));
#187418=CARTESIAN_POINT('Origin',(56.6898028749653,2.96999998000001,-54.74995));
#187419=CARTESIAN_POINT('Ctrl Pts',(56.6516106473573,3.03773716318841,-55.2548395864932));
#187420=CARTESIAN_POINT('Ctrl Pts',(56.1862233638146,2.91063352623763,-55.2365176478553));
#187421=CARTESIAN_POINT('Ctrl Pts',(56.1704852303868,2.96901219974452,-54.7588470687756));
#187422=CARTESIAN_POINT('Ctrl Pts',(56.7365664636558,2.88838457711559,-55.2329986037404));
#187423=CARTESIAN_POINT('Ctrl Pts',(56.2378094923969,2.72675510356031,-55.2554023668191));
#187424=CARTESIAN_POINT('Ctrl Pts',(56.2547381424865,2.67276304505858,-54.7151058664062));
#187425=CARTESIAN_POINT('Ctrl Pts',(56.8232758616439,2.72973218222745,-55.2852577349349));
#187426=CARTESIAN_POINT('Ctrl Pts',(56.272540084895,2.60245677689778,-55.3631060048095));
#187427=CARTESIAN_POINT('Ctrl Pts',(56.3408153301335,2.35776462627681,-54.8196810538982));
#187428=CARTESIAN_POINT('Ctrl Pts',(56.9409610884963,2.51006427970322,-55.5006989132498));
#187429=CARTESIAN_POINT('Ctrl Pts',(56.3106636954826,2.47176602276538,-55.5888533041906));
#187430=CARTESIAN_POINT('Ctrl Pts',(56.4576103865826,1.92173897553581,-55.2509470312754));
#187431=CARTESIAN_POINT('Ctrl Pts',(56.9713444184252,2.4511633015209,-55.6620201884579));
#187432=CARTESIAN_POINT('Ctrl Pts',(56.3132427996389,2.46728529949762,-55.6970341949502));
#187433=CARTESIAN_POINT('Ctrl Pts',(56.4877712558399,1.80479876584888,-55.5739123475053));
#187434=CARTESIAN_POINT('Ctrl Pts',(56.9587711759279,2.47540554332925,-55.8218687400276));
#187435=CARTESIAN_POINT('Ctrl Pts',(56.3116760352399,2.47109535466139,-55.7946188306712));
#187436=CARTESIAN_POINT('Ctrl Pts',(56.4752909911635,1.85292504817076,-55.8939326223247));
#187437=CARTESIAN_POINT('',(56.4778207328943,1.8431691585182,-55.74995));
#187438=CARTESIAN_POINT('Ctrl Pts',(56.4778207328944,1.84316915851821,-55.74995));
#187439=CARTESIAN_POINT('Ctrl Pts',(56.4778064569306,1.84322359733619,-55.6560313317286));
#187440=CARTESIAN_POINT('Ctrl Pts',(56.4743371862811,1.85647090128218,-55.5635633305672));
#187441=CARTESIAN_POINT('Ctrl Pts',(56.4675209933656,1.88238984882649,-55.4737762830553));
#187442=CARTESIAN_POINT('Ctrl Pts',(56.4646552786549,1.89328688624677,-55.4360273422497));
#187443=CARTESIAN_POINT('Ctrl Pts',(56.4611973335471,1.90642358799506,-55.3987522848102));
#187444=CARTESIAN_POINT('Ctrl Pts',(56.4571525729354,1.92176052606978,-55.362042538798));
#187445=CARTESIAN_POINT('Ctrl Pts',(56.4466430200751,1.96161068702785,-55.2666591395701));
#187446=CARTESIAN_POINT('Ctrl Pts',(56.4329085143679,2.01353490739002,-55.1807492293272));
#187447=CARTESIAN_POINT('Ctrl Pts',(56.4157876207897,2.07773388906235,-55.1040867013627));
#187448=CARTESIAN_POINT('Ctrl Pts',(56.4106465751013,2.09701149840069,-55.0810665501625));
#187449=CARTESIAN_POINT('Ctrl Pts',(56.4051998459472,2.11739579758647,-55.0588802123864));
#187450=CARTESIAN_POINT('Ctrl Pts',(56.3994421718616,2.1388919699916,-55.0375215661014));
#187451=CARTESIAN_POINT('Ctrl Pts',(56.3745100863326,2.23197546186361,-54.9450335947364));
#187452=CARTESIAN_POINT('Ctrl Pts',(56.3453168238088,2.34004445713371,-54.8734764439432));
#187453=CARTESIAN_POINT('Ctrl Pts',(56.3124317677987,2.46007868339493,-54.8240658663659));
#187454=CARTESIAN_POINT('Ctrl Pts',(56.2795467117886,2.58011290965614,-54.7746552887886));
#187455=CARTESIAN_POINT('Ctrl Pts',(56.2449231123173,2.70498953592612,-54.74995));
#187456=CARTESIAN_POINT('Ctrl Pts',(56.2084630076341,2.83467839222655,-54.74995));
#187457=CARTESIAN_POINT('Origin',(56.9614672388491,1.96999998000001,-55.74995));
#187458=CARTESIAN_POINT('Origin',(56.9614672388491,1.96999998000001,-55.24995));
#187459=CARTESIAN_POINT('',(56.4778207328943,1.84316915851819,-55.24995));
#187460=CARTESIAN_POINT('Origin',(0.,-12.9675000200281,-60.42825533736));
#187461=CARTESIAN_POINT('Origin',(0.,-12.9675000200281,-60.42825533736));
#187462=CARTESIAN_POINT('Origin',(58.1504944089282,-3.68000001999999,-55.24995));
#187463=CARTESIAN_POINT('',(57.6567521511579,-3.75885801193397,-55.9233081330105));
#187464=CARTESIAN_POINT('',(57.6567521511579,-3.75885801193397,-55.24995));
#187465=CARTESIAN_POINT('Origin',(58.1504944089282,-3.68000001999999,-55.9233081330105));
#187466=CARTESIAN_POINT('Ctrl Pts',(58.1878043152552,-4.18472849816432,
-56.0217471588075));
#187467=CARTESIAN_POINT('Ctrl Pts',(57.7288017309817,-4.21869464918518,
-56.0268087650182));
#187468=CARTESIAN_POINT('Ctrl Pts',(57.6580782481123,-3.7670747753154,-56.0829545312913));
#187469=CARTESIAN_POINT('Ctrl Pts',(58.1423490001074,-4.17368834353939,
-55.9044937172376));
#187470=CARTESIAN_POINT('Ctrl Pts',(57.7207276063559,-4.16605409632374,
-55.912529187981));
#187471=CARTESIAN_POINT('Ctrl Pts',(57.6545081941398,-3.74493084812172,
-55.8965040979149));
#187472=CARTESIAN_POINT('Ctrl Pts',(58.11010891456,-4.18155527439172,-55.7954042268261));
#187473=CARTESIAN_POINT('Ctrl Pts',(57.7177405846301,-4.14730583030866,
-55.7833549220629));
#187474=CARTESIAN_POINT('Ctrl Pts',(57.6570350940306,-3.76040655228401,
-55.7095218572218));
#187475=CARTESIAN_POINT('Ctrl Pts',(58.0758010551818,-4.23492939420442,
-55.626523645907));
#187476=CARTESIAN_POINT('Ctrl Pts',(57.7231513907377,-4.18465995709919,
-55.5758965119262));
#187477=CARTESIAN_POINT('Ctrl Pts',(57.6738297434981,-3.86630826885906,
-55.4091279774612));
#187478=CARTESIAN_POINT('Ctrl Pts',(58.0682346046872,-4.2681708265488,-55.5642771712915));
#187479=CARTESIAN_POINT('Ctrl Pts',(57.7282596126722,-4.21904460184081,
-55.4959409277901));
#187480=CARTESIAN_POINT('Ctrl Pts',(57.6842607125848,-3.93233117446903,
-55.2948627293281));
#187481=CARTESIAN_POINT('Ctrl Pts',(58.0615640318237,-4.41832044615007,
-55.3857650708271));
#187482=CARTESIAN_POINT('Ctrl Pts',(57.7539337512875,-4.39250111928527,
-55.26869173567));
#187483=CARTESIAN_POINT('Ctrl Pts',(57.730526224235,-4.2306772427365,-54.9612377069699));
#187484=CARTESIAN_POINT('Ctrl Pts',(58.0893322115688,-4.58139785886709,
-55.3288487124944));
#187485=CARTESIAN_POINT('Ctrl Pts',(57.7860859134861,-4.61172772721033,
-55.1905959772978));
#187486=CARTESIAN_POINT('Ctrl Pts',(57.7793092684043,-4.5547357307314,-54.8442406125823));
#187487=CARTESIAN_POINT('Ctrl Pts',(58.132482042408,-4.74154412477497,-55.3691052207555));
#187488=CARTESIAN_POINT('Ctrl Pts',(57.8139022478951,-4.80923291831809,
-55.2499722576169));
#187489=CARTESIAN_POINT('Ctrl Pts',(57.8236816674951,-4.87324703899737,
-54.9084895606105));
#187490=CARTESIAN_POINT('',(57.8012193907064,-4.71406478367238,-54.8923577774473));
#187491=CARTESIAN_POINT('Origin',(58.2961987903268,-4.64338668274023,-54.8923577774473));
#187492=CARTESIAN_POINT('Ctrl Pts',(57.8012193907064,-4.71406478367238,
-54.8923577774473));
#187493=CARTESIAN_POINT('Ctrl Pts',(57.7836536578014,-4.59104682177848,
-54.8901832085045));
#187494=CARTESIAN_POINT('Ctrl Pts',(57.7662856874572,-4.47225223324713,
-54.9123724001228));
#187495=CARTESIAN_POINT('Ctrl Pts',(57.7495807450161,-4.36017290714565,
-54.9578152376692));
#187496=CARTESIAN_POINT('Ctrl Pts',(57.7482218313389,-4.35105547799513,
-54.9615119216709));
#187497=CARTESIAN_POINT('Ctrl Pts',(57.7468673329787,-4.34198248231328,
-54.9653624866117));
#187498=CARTESIAN_POINT('Ctrl Pts',(57.745517514559,-4.33295525906636,-54.9693663348943));
#187499=CARTESIAN_POINT('Ctrl Pts',(57.7365460375155,-4.27295642889168,
-54.9959776423346));
#187500=CARTESIAN_POINT('Ctrl Pts',(57.7280596798513,-4.2168386440149,-55.0284329935762));
#187501=CARTESIAN_POINT('Ctrl Pts',(57.7200923014674,-4.16459703502482,
-55.0667323886189));
#187502=CARTESIAN_POINT('Ctrl Pts',(57.7121249230835,-4.11235542603474,
-55.1050317836617));
#187503=CARTESIAN_POINT('Ctrl Pts',(57.70446832363,-4.06264749225641,-55.1506834849025));
#187504=CARTESIAN_POINT('Ctrl Pts',(57.6977762772175,-4.01949639254467,
-55.1991627051508));
#187505=CARTESIAN_POINT('Ctrl Pts',(57.6910842308049,-3.97634529283294,
-55.2476419253992));
#187506=CARTESIAN_POINT('Ctrl Pts',(57.6851484738385,-3.93838586919532,
-55.2999617303345));
#187507=CARTESIAN_POINT('Ctrl Pts',(57.6799997155797,-3.90561340277092,
-55.3561221199568));
#187508=CARTESIAN_POINT('Ctrl Pts',(57.6774253364502,-3.88922716955872,
-55.384202314768));
#187509=CARTESIAN_POINT('Ctrl Pts',(57.67504757604,-3.87413769627492,-55.4132426557509));
#187510=CARTESIAN_POINT('Ctrl Pts',(57.6728694851827,-3.8603445037118,-55.4432431429055));
#187511=CARTESIAN_POINT('Ctrl Pts',(57.6706913943255,-3.84655131114868,
-55.4732436300601));
#187512=CARTESIAN_POINT('Ctrl Pts',(57.6686282628525,-3.83352020962757,
-55.5057266054656));
#187513=CARTESIAN_POINT('Ctrl Pts',(57.6669367487985,-3.82285337494814,
-55.5361250428846));
#187514=CARTESIAN_POINT('Ctrl Pts',(57.6616870217134,-3.7897481395564,-55.6304686280757));
#187515=CARTESIAN_POINT('Ctrl Pts',(57.6584496886985,-3.76948979078947,
-55.7293075756491));
#187516=CARTESIAN_POINT('Ctrl Pts',(57.6572653615991,-3.76207187814138,
-55.8326418856047));
#187517=CARTESIAN_POINT('Ctrl Pts',(57.6569232810199,-3.75992929113468,
-55.8624889275369));
#187518=CARTESIAN_POINT('Ctrl Pts',(57.656752151158,-3.75885801193395,-55.8927110100055));
#187519=CARTESIAN_POINT('Ctrl Pts',(57.656752151158,-3.75885801193396,-55.9233081330105));
#187520=CARTESIAN_POINT('Ctrl Pts',(58.1110275345658,-4.66169335137012,
-55.3564444847807));
#187521=CARTESIAN_POINT('Ctrl Pts',(57.8003896508712,-4.70825387307828,
-55.2306628708486));
#187522=CARTESIAN_POINT('Ctrl Pts',(57.8012193907063,-4.71406478367217,
-54.8923577774473));
#187523=CARTESIAN_POINT('Ctrl Pts',(58.13138502781,-4.82819068711566,-55.3579993904125));
#187524=CARTESIAN_POINT('Ctrl Pts',(57.8239228782473,-4.87294575633325,
-55.2309062620395));
#187525=CARTESIAN_POINT('Ctrl Pts',(57.8247681406176,-4.8789835624615,-54.8952730204543));
#187526=CARTESIAN_POINT('Ctrl Pts',(58.1511322005955,-4.99473857781996,
-55.3594494677196));
#187527=CARTESIAN_POINT('Ctrl Pts',(57.8468132839757,-5.03816723372008,
-55.2311383656919));
#187528=CARTESIAN_POINT('Ctrl Pts',(57.8476108954267,-5.04400181406656,
-54.8980841413334));
#187529=CARTESIAN_POINT('Ctrl Pts',(58.1702690071153,-5.16134039100007,
-55.3608055405081));
#187530=CARTESIAN_POINT('Ctrl Pts',(57.8690388195133,-5.20383266421771,
-55.2313599550618));
#187531=CARTESIAN_POINT('Ctrl Pts',(57.8697476022662,-5.20911947359366,
-54.9007953984755));
#187532=CARTESIAN_POINT('',(57.8697476022662,-5.20911947359366,-54.9007953984755));
#187533=CARTESIAN_POINT('Origin',(58.3653138416346,-5.14268076199931,-54.9007953984755));
#187534=CARTESIAN_POINT('Origin',(1.16314418724182,-12.9460285170553,-46.7095980005158));
#187535=CARTESIAN_POINT('Ctrl Pts',(58.1702690071154,-5.16134039100007,
-55.3608055405082));
#187536=CARTESIAN_POINT('Ctrl Pts',(57.8690388195133,-5.20383266421795,
-55.2313599550619));
#187537=CARTESIAN_POINT('Ctrl Pts',(57.8697476022663,-5.20911947359449,
-54.9007953984755));
#187538=CARTESIAN_POINT('Ctrl Pts',(58.1863681399526,-5.2347113163298,-55.3646554087878));
#187539=CARTESIAN_POINT('Ctrl Pts',(57.8816711167897,-5.29795553030126,
-55.2377699288153));
#187540=CARTESIAN_POINT('Ctrl Pts',(57.8892576239528,-5.35464469293038,
-54.9031849800101));
#187541=CARTESIAN_POINT('Ctrl Pts',(58.206532806921,-5.30826342386473,-55.3884755439432));
#187542=CARTESIAN_POINT('Ctrl Pts',(57.8939857420187,-5.39104663027327,
-55.2713483619941));
#187543=CARTESIAN_POINT('Ctrl Pts',(57.9082088324435,-5.50047055831863,
-54.9417550134773));
#187544=CARTESIAN_POINT('Ctrl Pts',(58.2517768983759,-5.43880935502387,
-55.4693790307482));
#187545=CARTESIAN_POINT('Ctrl Pts',(57.9146461968408,-5.54837256073304,
-55.3788933751119));
#187546=CARTESIAN_POINT('Ctrl Pts',(57.9410017896518,-5.75934555612452,
-55.0773466647676));
#187547=CARTESIAN_POINT('Ctrl Pts',(58.2772082041435,-5.49676306934017,
-55.5268083141558));
#187548=CARTESIAN_POINT('Ctrl Pts',(57.9231956882672,-5.61406051834577,
-55.4547002829484));
#187549=CARTESIAN_POINT('Ctrl Pts',(57.9551095363294,-5.87426883806545,
-55.1748695369358));
#187550=CARTESIAN_POINT('Ctrl Pts',(58.3321412809957,-5.58904289089475,
-55.6647824032721));
#187551=CARTESIAN_POINT('Ctrl Pts',(57.9351757774934,-5.70509939430376,
-55.6270222213536));
#187552=CARTESIAN_POINT('Ctrl Pts',(57.9772132186836,-6.05726143051376,
-55.4055720426652));
#187553=CARTESIAN_POINT('Ctrl Pts',(58.3618432600141,-5.62384585378313,
-55.7455542887996));
#187554=CARTESIAN_POINT('Ctrl Pts',(57.9385982402169,-5.73028333208738,
-55.725786817627));
#187555=CARTESIAN_POINT('Ctrl Pts',(57.9853419314568,-6.12627634754757,
-55.5391049776385));
#187556=CARTESIAN_POINT('Ctrl Pts',(58.4256102669737,-5.66935462867838,
-55.922812372103));
#187557=CARTESIAN_POINT('Ctrl Pts',(57.9401928503808,-5.73799842569994,
-55.9259333604635));
#187558=CARTESIAN_POINT('Ctrl Pts',(57.9959179918116,-6.21652108864807,
-55.822399360329));
#187559=CARTESIAN_POINT('Ctrl Pts',(58.4594118188674,-5.68000001999999,
-56.0184103401194));
#187560=CARTESIAN_POINT('Ctrl Pts',(57.9381116944449,-5.71846326962249,
-56.0282143296095));
#187561=CARTESIAN_POINT('Ctrl Pts',(57.9983536021903,-6.2376310994186,-55.9707502487912));
#187562=CARTESIAN_POINT('Ctrl Pts',(58.4950211556756,-5.68000001999999,
-56.1192785199305));
#187563=CARTESIAN_POINT('Ctrl Pts',(57.9336485918015,-5.68000002,-56.1192785199305));
#187564=CARTESIAN_POINT('Ctrl Pts',(57.9983536018174,-6.23763109620483,
-56.1192785199305));
#187565=CARTESIAN_POINT('',(57.9983536018174,-6.23763109620483,-56.1192785199305));
#187566=CARTESIAN_POINT('Origin',(58.4950211556756,-6.18000001999999,-56.1192785199305));
#187567=CARTESIAN_POINT('Ctrl Pts',(57.9983536018174,-6.23763109620483,
-56.1192785199305));
#187568=CARTESIAN_POINT('Ctrl Pts',(57.9983536018174,-6.23763109620483,
-56.0644455264786));
#187569=CARTESIAN_POINT('Ctrl Pts',(57.9980221190057,-6.23475814249574,
-56.0098560074896));
#187570=CARTESIAN_POINT('Ctrl Pts',(57.9973433490653,-6.22891039019457,
-55.9557040569575));
#187571=CARTESIAN_POINT('Ctrl Pts',(57.9966909788379,-6.22329007722613,
-55.9036582632633));
#187572=CARTESIAN_POINT('Ctrl Pts',(57.9957178277956,-6.21492191913588,
-55.8520157782166));
#187573=CARTESIAN_POINT('Ctrl Pts',(57.9944044945626,-6.20366890587323,
-55.8009488806203));
#187574=CARTESIAN_POINT('Ctrl Pts',(57.9933769792934,-6.1948648623442,-55.7609955651095));
#187575=CARTESIAN_POINT('Ctrl Pts',(57.9921411410287,-6.1842941397813,-55.7213944424274));
#187576=CARTESIAN_POINT('Ctrl Pts',(57.9906851268661,-6.17186945082616,
-55.682233037996));
#187577=CARTESIAN_POINT('Ctrl Pts',(57.9906667712501,-6.17171281579784,
-55.6817393397059));
#187578=CARTESIAN_POINT('Ctrl Pts',(57.9906483809945,-6.17155588913671,
-55.681245721757));
#187579=CARTESIAN_POINT('Ctrl Pts',(57.9906299560812,-6.17139867071413,
-55.6807521844164));
#187580=CARTESIAN_POINT('Ctrl Pts',(57.9875046150389,-6.14473036685059,
-55.5970355082689));
#187581=CARTESIAN_POINT('Ctrl Pts',(57.9833865494891,-6.10971202599363,
-55.5161284707291));
#187582=CARTESIAN_POINT('Ctrl Pts',(57.9782530724075,-6.06658854500581,
-55.4400802261805));
#187583=CARTESIAN_POINT('Ctrl Pts',(57.9747553923278,-6.03720648329143,
-55.3882649700043));
#187584=CARTESIAN_POINT('Ctrl Pts',(57.9707862300964,-6.00406098349663,
-55.3387057443247));
#187585=CARTESIAN_POINT('Ctrl Pts',(57.9663371613776,-5.96722056379155,
-55.2920615727606));
#187586=CARTESIAN_POINT('Ctrl Pts',(57.9662786111709,-5.96673574004027,
-55.2914477306162));
#187587=CARTESIAN_POINT('Ctrl Pts',(57.9662199779913,-5.96625027756548,
-55.2908343949051));
#187588=CARTESIAN_POINT('Ctrl Pts',(57.9661612618222,-5.96576417654625,
-55.290221567164));
#187589=CARTESIAN_POINT('Ctrl Pts',(57.9589421887773,-5.90599871813124,
-55.2148752308583));
#187590=CARTESIAN_POINT('Ctrl Pts',(57.9504117107839,-5.83617450509476,
-55.1470534422411));
#187591=CARTESIAN_POINT('Ctrl Pts',(57.9407769623022,-5.75872949143219,
-55.0901422818071));
#187592=CARTESIAN_POINT('Ctrl Pts',(57.9357443409793,-5.7182768083291,-55.0604152660938));
#187593=CARTESIAN_POINT('Ctrl Pts',(57.9304104809609,-5.6757454289285,-55.0336657755819));
#187594=CARTESIAN_POINT('Ctrl Pts',(57.9248052326105,-5.6314864592146,-55.0103806480697));
#187595=CARTESIAN_POINT('Ctrl Pts',(57.9247386150578,-5.63096044786509,
-55.0101039077518));
#187596=CARTESIAN_POINT('Ctrl Pts',(57.9246719532792,-5.63043414597654,
-55.0098276317697));
#187597=CARTESIAN_POINT('Ctrl Pts',(57.9246052474285,-5.62990755498805,
-55.0095518217286));
#187598=CARTESIAN_POINT('Ctrl Pts',(57.9212703682262,-5.6035812685004,-54.9957630286864));
#187599=CARTESIAN_POINT('Ctrl Pts',(57.9178139721908,-5.57645251025445,
-54.9831217176357));
#187600=CARTESIAN_POINT('Ctrl Pts',(57.9142675773715,-5.54877950578547,
-54.971764271749));
#187601=CARTESIAN_POINT('Ctrl Pts',(57.913512817463,-5.54289001085152,-54.9693471283525));
#187602=CARTESIAN_POINT('Ctrl Pts',(57.9127539957423,-5.53697595914941,
-54.9669879747414));
#187603=CARTESIAN_POINT('Ctrl Pts',(57.91199143806,-5.5310399789474,-54.9646878564231));
#187604=CARTESIAN_POINT('Ctrl Pts',(57.9086784919242,-5.50525100176252,
-54.9546949493021));
#187605=CARTESIAN_POINT('Ctrl Pts',(57.9052948080902,-5.47904671417077,
-54.9458177116981));
#187606=CARTESIAN_POINT('Ctrl Pts',(57.9018664479803,-5.45263506176634,
-54.9381157197596));
#187607=CARTESIAN_POINT('Ctrl Pts',(57.9006211279107,-5.4430412735538,-54.9353180424943));
#187608=CARTESIAN_POINT('Ctrl Pts',(57.8993701409321,-5.43342183598718,
-54.9326755439205));
#187609=CARTESIAN_POINT('Ctrl Pts',(57.8981140995163,-5.42378169739113,
-54.9301886689187));
#187610=CARTESIAN_POINT('Ctrl Pts',(57.8944762323973,-5.39586100721126,
-54.9229859440048));
#187611=CARTESIAN_POINT('Ctrl Pts',(57.8907870927057,-5.36769806591993,
-54.9170666561105));
#187612=CARTESIAN_POINT('Ctrl Pts',(57.8870439982321,-5.33928354730464,
-54.9124555883763));
#187613=CARTESIAN_POINT('Ctrl Pts',(57.8834098871839,-5.31169634191586,
-54.9079787758577));
#187614=CARTESIAN_POINT('Ctrl Pts',(57.8797247293363,-5.28387052582338,
-54.9047349097721));
#187615=CARTESIAN_POINT('Ctrl Pts',(57.8759849933551,-5.25579526938749,
-54.902794710981));
#187616=CARTESIAN_POINT('Ctrl Pts',(57.8739226319616,-5.24031253871396,
-54.9017247447849));
#187617=CARTESIAN_POINT('Ctrl Pts',(57.8718436840546,-5.22475414416982,
-54.9010521259368));
#187618=CARTESIAN_POINT('Ctrl Pts',(57.8697476022663,-5.20911947359449,
-54.9007953984755));
#187619=CARTESIAN_POINT('Origin',(58.4950211556756,-6.18000001999999,-55.24995));
#187620=CARTESIAN_POINT('',(57.9983536018174,-6.23763109620483,-55.24995));
#187621=CARTESIAN_POINT('Origin',(0.,-12.9675000200281,-60.42825533736));
#187622=CARTESIAN_POINT('Origin',(0.,-12.9675000200281,-60.42825533736));
#187623=CARTESIAN_POINT('Origin',(58.8765127194474,-11.83000002,-55.24995));
#187624=CARTESIAN_POINT('',(58.376606009879,-11.839658266657,-56.2580153373943));
#187625=CARTESIAN_POINT('',(58.376606009879,-11.839658266657,-55.24995));
#187626=CARTESIAN_POINT('Origin',(58.8765127194474,-11.83000002,-56.2580153373923));
#187627=CARTESIAN_POINT('Ctrl Pts',(58.9204693868563,-12.3332405111934,
-56.3968205615773));
#187628=CARTESIAN_POINT('Ctrl Pts',(58.3858773874524,-12.3801702023644,
-56.3925855609961));
#187629=CARTESIAN_POINT('Ctrl Pts',(58.3767427611297,-11.8450339177556,
-56.4300980462111));
#187630=CARTESIAN_POINT('Ctrl Pts',(58.8276762845464,-12.3201365847109,
-56.1030402216339));
#187631=CARTESIAN_POINT('Ctrl Pts',(58.3841915353992,-12.2706483349671,
-56.1428486906975));
#187632=CARTESIAN_POINT('Ctrl Pts',(58.3760938044882,-11.8191230277002,
-56.0766739558416));
#187633=CARTESIAN_POINT('Ctrl Pts',(58.7434563338895,-12.3445753573015,
-55.8427359981275));
#187634=CARTESIAN_POINT('Ctrl Pts',(58.3834159308919,-12.231047346678,-55.8250036101692));
#187635=CARTESIAN_POINT('Ctrl Pts',(58.377497118127,-11.8677221198328,-55.6935276731622));
#187636=CARTESIAN_POINT('Ctrl Pts',(58.6765740898316,-12.4686431832956,
-55.6084324108456));
#187637=CARTESIAN_POINT('Ctrl Pts',(58.3844523423634,-12.3662466486663,
-55.5259929392754));
#187638=CARTESIAN_POINT('Ctrl Pts',(58.3812774173441,-12.1139782222975,
-55.3274681950692));
#187639=CARTESIAN_POINT('Ctrl Pts',(58.6664450477116,-12.4930003730007,
-55.5718694403823));
#187640=CARTESIAN_POINT('Ctrl Pts',(58.3846738120602,-12.3941454433015,
-55.4797853161406));
#187641=CARTESIAN_POINT('Ctrl Pts',(58.3819739476742,-12.162324552265,-55.2693146819956));
#187642=CARTESIAN_POINT('Ctrl Pts',(58.6488234778106,-12.5478651152317,
-55.5067647140881));
#187643=CARTESIAN_POINT('Ctrl Pts',(58.3851684019452,-12.4603487355267,
-55.3968754406393));
#187644=CARTESIAN_POINT('Ctrl Pts',(58.3833741817178,-12.2712209921738,
-55.1646750530484));
#187645=CARTESIAN_POINT('Ctrl Pts',(58.6412804318072,-12.5788151444312,
-55.4780148049617));
#187646=CARTESIAN_POINT('Ctrl Pts',(58.3854452700191,-12.4992609451243,
-55.359601343505));
#187647=CARTESIAN_POINT('Ctrl Pts',(58.3840852347027,-12.3326490346772,
-55.1178342268099));
#187648=CARTESIAN_POINT('Ctrl Pts',(58.6189489342569,-12.7021410587872,
-55.3911723350316));
#187649=CARTESIAN_POINT('Ctrl Pts',(58.3864295862247,-12.6569413001418,
-55.2474388094329));
#187650=CARTESIAN_POINT('Ctrl Pts',(58.386474193177,-12.5774201145556,-54.9754185610577));
#187651=CARTESIAN_POINT('Ctrl Pts',(58.6136591241034,-12.8116339481853,
-55.3668837279628));
#187652=CARTESIAN_POINT('Ctrl Pts',(58.3870807295506,-12.8069198757032,
-55.212974677113));
#187653=CARTESIAN_POINT('Ctrl Pts',(58.3876968043474,-12.7947167262509,
-54.9337374850759));
#187654=CARTESIAN_POINT('Ctrl Pts',(58.6208473456642,-12.9180978208483,
-55.3950294078271));
#187655=CARTESIAN_POINT('Ctrl Pts',(58.3871216621357,-12.9488461390236,
-55.2514801948388));
#187656=CARTESIAN_POINT('Ctrl Pts',(58.3874545650717,-13.0060107626915,
-54.9810563880024));
#187657=CARTESIAN_POINT('',(58.3873384184922,-12.8301367871357,-54.9623589764041));
#187658=CARTESIAN_POINT('Origin',(58.8873370347925,-12.8289604802815,-54.9623589764042));
#187659=CARTESIAN_POINT('Ctrl Pts',(58.3873384184922,-12.8301367871357,
-54.9623589764041));
#187660=CARTESIAN_POINT('Ctrl Pts',(58.3871582402025,-12.7535505671015,
-54.962337964741));
#187661=CARTESIAN_POINT('Ctrl Pts',(58.3866696814845,-12.6418858505425,
-54.9772287565121));
#187662=CARTESIAN_POINT('Ctrl Pts',(58.3857822010939,-12.5172370713889,
-55.0207153881268));
#187663=CARTESIAN_POINT('Ctrl Pts',(58.3853403721938,-12.46502197154,-55.0449483819363));
#187664=CARTESIAN_POINT('Ctrl Pts',(58.3850328759368,-12.4304798696505,
-55.0623472369148));
#187665=CARTESIAN_POINT('Ctrl Pts',(58.384863102533,-12.4123661419375,-55.0722395517767));
#187666=CARTESIAN_POINT('Ctrl Pts',(58.3840791937441,-12.3322340243949,
-55.1190986956505));
#187667=CARTESIAN_POINT('Ctrl Pts',(58.3830530216899,-12.2434331788292,
-55.1861910548624));
#187668=CARTESIAN_POINT('Ctrl Pts',(58.3818235406729,-12.1527075458442,
-55.283472900429));
#187669=CARTESIAN_POINT('Ctrl Pts',(58.381213203161,-12.1105634443595,-55.3368656798338));
#187670=CARTESIAN_POINT('Ctrl Pts',(58.380953857786,-12.0931913982438,-55.3607665545691));
#187671=CARTESIAN_POINT('Ctrl Pts',(58.380781592723,-12.0817633019031,-55.376926749946));
#187672=CARTESIAN_POINT('Ctrl Pts',(58.3806842527656,-12.0753758242722,
-55.3862403887367));
#187673=CARTESIAN_POINT('Ctrl Pts',(58.378245228469,-11.9166221344459,-55.6233775609728));
#187674=CARTESIAN_POINT('Ctrl Pts',(58.3766060098791,-11.8396582666571,
-55.9115738855532));
#187675=CARTESIAN_POINT('Ctrl Pts',(58.376606009879,-11.839658266657,-56.2580153373943));
#187676=CARTESIAN_POINT('Ctrl Pts',(58.6177174583935,-12.8294802501408,
-55.3834349955049));
#187677=CARTESIAN_POINT('Ctrl Pts',(58.3873382434228,-12.8300623725117,
-55.2359199480943));
#187678=CARTESIAN_POINT('Ctrl Pts',(58.3873384184922,-12.8301367871357,
-54.9623589764042));
#187679=CARTESIAN_POINT('Ctrl Pts',(58.6180560895148,-12.9967778686933,
-55.3834453150663));
#187680=CARTESIAN_POINT('Ctrl Pts',(58.3877303689834,-12.9966482737698,
-55.2359230050539));
#187681=CARTESIAN_POINT('Ctrl Pts',(58.3877301336919,-12.9966384589807,
-54.9624046566442));
#187682=CARTESIAN_POINT('Ctrl Pts',(58.617779029823,-13.1640733250721,-55.3834369075807));
#187683=CARTESIAN_POINT('Ctrl Pts',(58.3874094466061,-13.1632604597666,
-55.2359205049346));
#187684=CARTESIAN_POINT('Ctrl Pts',(58.3874096419063,-13.1631387418538,
-54.9623672844226));
#187685=CARTESIAN_POINT('Ctrl Pts',(58.6168862797194,-13.3313694061421,
-55.3834096347596));
#187686=CARTESIAN_POINT('Ctrl Pts',(58.3863757263072,-13.3298338968439,
-55.2359124429047));
#187687=CARTESIAN_POINT('Ctrl Pts',(58.3863769436068,-13.3296376352283,
-54.9622468511542));
#187688=CARTESIAN_POINT('',(58.3863769436068,-13.3296376352283,-54.9622468511542));
#187689=CARTESIAN_POINT('Origin',(58.8863673263393,-13.3327387922841,-54.9622468511542));
#187690=CARTESIAN_POINT('Origin',(0.783669006986427,-12.9675005471716,-48.2446834721308));
#187691=CARTESIAN_POINT('Ctrl Pts',(58.6186775397123,-13.2733227804916,
-55.388616176824));
#187692=CARTESIAN_POINT('Ctrl Pts',(58.3866003242463,-13.2520322171712,
-55.2428270583313));
#187693=CARTESIAN_POINT('Ctrl Pts',(58.386962112441,-13.2144813034654,-54.9704131764568));
#187694=CARTESIAN_POINT('Ctrl Pts',(58.6137221237977,-13.3676448320215,
-55.3717404151163));
#187695=CARTESIAN_POINT('Ctrl Pts',(58.3859840071227,-13.3780470899907,
-55.2199040746864));
#187696=CARTESIAN_POINT('Ctrl Pts',(58.3862324741917,-13.4016008615142,
-54.9423444295408));
#187697=CARTESIAN_POINT('Ctrl Pts',(58.6187510133404,-13.4663403062683,
-55.3964780242175));
#187698=CARTESIAN_POINT('Ctrl Pts',(58.3848758374799,-13.5124773652813,
-55.2543020165157));
#187699=CARTESIAN_POINT('Ctrl Pts',(58.3843307468424,-13.5974054698093,
-54.9846201136219));
#187700=CARTESIAN_POINT('Ctrl Pts',(58.6445475220142,-13.6142160529627,
-55.4999871066229));
#187701=CARTESIAN_POINT('Ctrl Pts',(58.3829825750198,-13.7025676579945,
-55.3887162988093));
#187702=CARTESIAN_POINT('Ctrl Pts',(58.3803445916225,-13.8907847695389,
-55.1547197684422));
#187703=CARTESIAN_POINT('Ctrl Pts',(58.661975771747,-13.6701810246484,-55.5666033099607));
#187704=CARTESIAN_POINT('Ctrl Pts',(58.3821783788648,-13.7708664553361,
-55.4756510335785));
#187705=CARTESIAN_POINT('Ctrl Pts',(58.3784002394851,-14.0018188962434,
-55.2630243475737));
#187706=CARTESIAN_POINT('Ctrl Pts',(58.70763761142,-13.7560113852979,-55.728182562924));
#187707=CARTESIAN_POINT('Ctrl Pts',(58.3811768765057,-13.8615861427662,
-55.675458539348));
#187708=CARTESIAN_POINT('Ctrl Pts',(58.3751345491859,-14.1721158329694,
-55.515820517695));
#187709=CARTESIAN_POINT('Ctrl Pts',(58.7355603527933,-13.7855764942266,
-55.8218098030616));
#187710=CARTESIAN_POINT('Ctrl Pts',(58.3810006665601,-13.8831469670814,
-55.7888512930239));
#187711=CARTESIAN_POINT('Ctrl Pts',(58.3738438065525,-14.2307829272749,
-55.6580807676195));
#187712=CARTESIAN_POINT('Ctrl Pts',(58.8069643993684,-13.8272064381204,
-56.0513753893604));
#187713=CARTESIAN_POINT('Ctrl Pts',(58.3813803134092,-13.8862762339219,
-56.0506342944055));
#187714=CARTESIAN_POINT('Ctrl Pts',(58.3720039090521,-14.3134065083042,
-55.9886327543262));
#187715=CARTESIAN_POINT('Ctrl Pts',(58.8522139297507,-13.8331326129651,
-56.1908063572759));
#187716=CARTESIAN_POINT('Ctrl Pts',(58.3821759711571,-13.8532144093832,
-56.2013060500146));
#187717=CARTESIAN_POINT('Ctrl Pts',(58.3717055999094,-14.3251897822734,
-56.1779359856761));
#187718=CARTESIAN_POINT('Ctrl Pts',(58.9012188893463,-13.828579144379,-56.3461607940094));
#187719=CARTESIAN_POINT('Ctrl Pts',(58.3832944048987,-13.7981222944649,
-56.3451627200497));
#187720=CARTESIAN_POINT('Ctrl Pts',(58.3719245331925,-14.3161844310707,
-56.3703692758833));
#187721=CARTESIAN_POINT('',(58.3718694303385,-14.3184313509278,-56.2531111209796));
#187722=CARTESIAN_POINT('Origin',(58.871735578318,-14.33000002,-56.2531111209796));
#187723=CARTESIAN_POINT('Ctrl Pts',(58.3718694303385,-14.3184313509278,
-56.2531111209796));
#187724=CARTESIAN_POINT('Ctrl Pts',(58.3718694303385,-14.3184313509278,
-56.1315282681123));
#187725=CARTESIAN_POINT('Ctrl Pts',(58.3720934589562,-14.3089057630787,
-56.0113829394871));
#187726=CARTESIAN_POINT('Ctrl Pts',(58.372602521148,-14.2863749805017,-55.8932001781189));
#187727=CARTESIAN_POINT('Ctrl Pts',(58.3727280602367,-14.2808186968923,
-55.8640552987669));
#187728=CARTESIAN_POINT('Ctrl Pts',(58.3728706983335,-14.274471486997,-55.8350297744669));
#187729=CARTESIAN_POINT('Ctrl Pts',(58.3730308041295,-14.2672811529287,
-55.8061314796515));
#187730=CARTESIAN_POINT('Ctrl Pts',(58.3735850259137,-14.2423911122432,
-55.7060972215946));
#187731=CARTESIAN_POINT('Ctrl Pts',(58.3743558983076,-14.2072301125135,
-55.6079785795892));
#187732=CARTESIAN_POINT('Ctrl Pts',(58.3753143408088,-14.1603251811705,
-55.5154726363337));
#187733=CARTESIAN_POINT('Ctrl Pts',(58.3757555226855,-14.138734313063,-55.4728911089164));
#187734=CARTESIAN_POINT('Ctrl Pts',(58.3762357928548,-14.114655053344,-55.431498836353));
#187735=CARTESIAN_POINT('Ctrl Pts',(58.3767484727564,-14.0879436829683,
-55.3916564088811));
#187736=CARTESIAN_POINT('Ctrl Pts',(58.3783749205468,-14.0032033816892,
-55.2652585767906));
#187737=CARTESIAN_POINT('Ctrl Pts',(58.3803191831255,-13.8924014500595,
-55.1564962213834));
#187738=CARTESIAN_POINT('Ctrl Pts',(58.382091437956,-13.7622047346492,-55.0806296262956));
#187739=CARTESIAN_POINT('Ctrl Pts',(58.3829775653712,-13.6971063769441,
-55.0426963287517));
#187740=CARTESIAN_POINT('Ctrl Pts',(58.3838281227637,-13.6263468744968,
-55.0125723550395));
#187741=CARTESIAN_POINT('Ctrl Pts',(58.3845593996408,-13.5534863365101,
-54.9925162587396));
#187742=CARTESIAN_POINT('Ctrl Pts',(58.385290676518,-13.4806257985234,-54.9724601624396));
#187743=CARTESIAN_POINT('Ctrl Pts',(58.3859030562338,-13.4060410952294,
-54.9621915864083));
#187744=CARTESIAN_POINT('Ctrl Pts',(58.3863769436069,-13.3296376352283,
-54.9622468511542));
#187745=CARTESIAN_POINT('Origin',(58.871735578318,-14.33000002,-55.24995));
#187746=CARTESIAN_POINT('',(58.3718694303385,-14.3184313509278,-55.24995));
#187747=CARTESIAN_POINT('Origin',(0.,-12.9675000200281,-60.42825533736));
#187748=CARTESIAN_POINT('Origin',(0.,-12.9675000200281,-60.42825533736));
#187749=CARTESIAN_POINT('Origin',(58.4684744114614,-19.98000002,-55.24995));
#187750=CARTESIAN_POINT('',(57.9720322598041,-19.92045852138,-56.1088024963483));
#187751=CARTESIAN_POINT('',(57.9720322598041,-19.92045852138,-55.24995));
#187752=CARTESIAN_POINT('Origin',(58.4684744114614,-19.98000002,-56.108802496345));
#187753=CARTESIAN_POINT('Ctrl Pts',(58.4684744114589,-20.48000002,-56.1088024963516));
#187754=CARTESIAN_POINT('Ctrl Pts',(57.9049228508699,-20.4800000199972,
-56.108802496352));
#187755=CARTESIAN_POINT('Ctrl Pts',(57.9720322598041,-19.92045852138,-56.1088024963483));
#187756=CARTESIAN_POINT('Ctrl Pts',(58.4330292345976,-20.4800000200005,
-56.0085121468718));
#187757=CARTESIAN_POINT('Ctrl Pts',(57.9095337666328,-20.4415553517815,
-56.0186397573414));
#187758=CARTESIAN_POINT('Ctrl Pts',(57.972032259745,-19.920458521873,-55.9596727479179));
#187759=CARTESIAN_POINT('Ctrl Pts',(58.4001436082512,-20.4906502319919,
-55.9155728413271));
#187760=CARTESIAN_POINT('Ctrl Pts',(57.9116095949012,-20.4226888878798,
-55.9192309942947));
#187761=CARTESIAN_POINT('Ctrl Pts',(57.9695132223445,-19.9415780781022,
-55.8143395431684));
#187762=CARTESIAN_POINT('Ctrl Pts',(58.336964041887,-20.5362234599901,-55.7404218332007));
#187763=CARTESIAN_POINT('Ctrl Pts',(57.9099756200818,-20.4304312900862,
-55.7217019778744));
#187764=CARTESIAN_POINT('Ctrl Pts',(57.9585693859923,-20.0319506515215,
-55.5325899309841));
#187765=CARTESIAN_POINT('Ctrl Pts',(58.3075894202415,-20.5708407676795,
-55.6609201576627));
#187766=CARTESIAN_POINT('Ctrl Pts',(57.9064908388997,-20.4553081180622,
-55.624563633487));
#187767=CARTESIAN_POINT('Ctrl Pts',(57.9502161720285,-20.1005973934661,
-55.4004673410398));
#187768=CARTESIAN_POINT('Ctrl Pts',(58.2664303444063,-20.6399469122455,
-55.5584001983321));
#187769=CARTESIAN_POINT('Ctrl Pts',(57.8972223460235,-20.5236291209351,
-55.4954672167701));
#187770=CARTESIAN_POINT('Ctrl Pts',(57.9331286547812,-20.2376361665866,
-55.2282616560402));
#187771=CARTESIAN_POINT('Ctrl Pts',(58.252990069642,-20.6662757908246,-55.526584865508));
#187772=CARTESIAN_POINT('Ctrl Pts',(57.8934574975699,-20.5515587218466,
-55.4548005580757));
#187773=CARTESIAN_POINT('Ctrl Pts',(57.9265619920107,-20.2898468150981,
-55.1744487967193));
#187774=CARTESIAN_POINT('Ctrl Pts',(58.2277581334007,-20.7227877352239,
-55.4712423952938));
#187775=CARTESIAN_POINT('Ctrl Pts',(57.8849360912282,-20.614784763174,-55.3832820627753));
#187776=CARTESIAN_POINT('Ctrl Pts',(57.9122860844342,-20.4019110441904,
-55.0807659948788));
#187777=CARTESIAN_POINT('Ctrl Pts',(58.2157933021909,-20.7532073937065,
-55.4472489303381));
#187778=CARTESIAN_POINT('Ctrl Pts',(57.8801540568373,-20.6502674204662,
-55.3516348732274));
#187779=CARTESIAN_POINT('Ctrl Pts',(57.9045197753069,-20.4622337862451,
-55.0401096877444));
#187780=CARTESIAN_POINT('Ctrl Pts',(58.1812959053717,-20.8514432878938,
-55.3865915677339));
#187781=CARTESIAN_POINT('Ctrl Pts',(57.8642971460945,-20.7674694003889,
-55.2713260639177));
#187782=CARTESIAN_POINT('Ctrl Pts',(57.8790836561167,-20.6570373864694,
-54.9381051588475));
#187783=CARTESIAN_POINT('Ctrl Pts',(58.1608566910152,-20.9243786591062,
-55.3628734830557));
#187784=CARTESIAN_POINT('Ctrl Pts',(57.851773276413,-20.8594120817092,-55.2377696368355));
#187785=CARTESIAN_POINT('Ctrl Pts',(57.8597273248566,-20.8016654950799,
-54.8995711242948));
#187786=CARTESIAN_POINT('Ctrl Pts',(58.1440639002148,-20.9985364556096,
-55.3589167601806));
#187787=CARTESIAN_POINT('Ctrl Pts',(57.838673217243,-20.9542432701794,-55.2310547627909));
#187788=CARTESIAN_POINT('Ctrl Pts',(57.8394345625603,-20.9487258492222,
-54.8970741880307));
#187789=CARTESIAN_POINT('',(57.8394345625603,-20.9487258492221,-54.8970741880307));
#187790=CARTESIAN_POINT('Origin',(58.3347412169172,-21.017072891219,-54.8970741880307));
#187791=CARTESIAN_POINT('Ctrl Pts',(57.8394345625603,-20.9487258492221,
-54.8970741880307));
#187792=CARTESIAN_POINT('Ctrl Pts',(57.8483315717593,-20.8842497909848,
-54.8981689263708));
#187793=CARTESIAN_POINT('Ctrl Pts',(57.8570330166362,-20.8203546606247,
-54.9061845094689));
#187794=CARTESIAN_POINT('Ctrl Pts',(57.8654251279068,-20.7580154570746,
-54.9205228428019));
#187795=CARTESIAN_POINT('Ctrl Pts',(57.8742541462857,-20.6924307721091,
-54.9356076533388));
#187796=CARTESIAN_POINT('Ctrl Pts',(57.8827409478669,-20.6285669203539,
-54.9576909614068));
#187797=CARTESIAN_POINT('Ctrl Pts',(57.8907523071727,-20.5675574167704,
-54.9861327822005));
#187798=CARTESIAN_POINT('Ctrl Pts',(57.8925393734123,-20.5539482376052,
-54.9924772008932));
#187799=CARTESIAN_POINT('Ctrl Pts',(57.8943027736333,-20.5404811271438,
-54.9991382130752));
#187800=CARTESIAN_POINT('Ctrl Pts',(57.8960410108923,-20.5271687639928,
-55.0061090485496));
#187801=CARTESIAN_POINT('Ctrl Pts',(57.8961104580828,-20.5266368997638,
-55.0063875519222));
#187802=CARTESIAN_POINT('Ctrl Pts',(57.8961798575478,-20.5261053444105,
-55.0066665020562));
#187803=CARTESIAN_POINT('Ctrl Pts',(57.8962492093382,-20.5255740977204,
-55.0069458987164));
#187804=CARTESIAN_POINT('Ctrl Pts',(57.9046540977693,-20.4611912009517,
-55.0408065639478));
#187805=CARTESIAN_POINT('Ctrl Pts',(57.9123517927205,-20.4013952311835,
-55.0812026657775));
#187806=CARTESIAN_POINT('Ctrl Pts',(57.9194238609353,-20.3458803213664,
-55.1276091020937));
#187807=CARTESIAN_POINT('Ctrl Pts',(57.9194970031007,-20.3453061639072,
-55.1280890560674));
#187808=CARTESIAN_POINT('Ctrl Pts',(57.9195700843622,-20.3447324149112,
-55.1285697353016));
#187809=CARTESIAN_POINT('Ctrl Pts',(57.9196431043984,-20.3441590772921,
-55.1290511360631));
#187810=CARTESIAN_POINT('Ctrl Pts',(57.9261585705981,-20.2930010380225,
-55.1720057900754));
#187811=CARTESIAN_POINT('Ctrl Pts',(57.9321919519941,-20.2450759632038,
-55.2207529417662));
#187812=CARTESIAN_POINT('Ctrl Pts',(57.9375117382139,-20.2024766659963,
-55.2726481082499));
#187813=CARTESIAN_POINT('Ctrl Pts',(57.9379542983799,-20.1989327732039,
-55.2769653369019));
#187814=CARTESIAN_POINT('Ctrl Pts',(57.9383919237743,-20.1954257087606,
-55.2813043482889));
#187815=CARTESIAN_POINT('Ctrl Pts',(57.938824483381,-20.1919566596153,-55.2856636195628));
#187816=CARTESIAN_POINT('Ctrl Pts',(57.938884960972,-20.1914716403672,-55.2862731037146));
#187817=CARTESIAN_POINT('Ctrl Pts',(57.9389453520762,-20.1909872680675,
-55.2868830674044));
#187818=CARTESIAN_POINT('Ctrl Pts',(57.9390056567172,-20.1905035428319,
-55.2874935092313));
#187819=CARTESIAN_POINT('Ctrl Pts',(57.9476291333811,-20.121331532001,-55.3747858097982));
#187820=CARTESIAN_POINT('Ctrl Pts',(57.9544934737034,-20.0653204626869,
-55.4719393844623));
#187821=CARTESIAN_POINT('Ctrl Pts',(57.9596779034763,-20.022713941091,-55.5751875387868));
#187822=CARTESIAN_POINT('Ctrl Pts',(57.9612949610576,-20.0094246881208,
-55.6073913139397));
#187823=CARTESIAN_POINT('Ctrl Pts',(57.9627485647956,-19.997439611234,-55.640188380711));
#187824=CARTESIAN_POINT('Ctrl Pts',(57.964041058706,-19.9867663918423,-55.6734654024398));
#187825=CARTESIAN_POINT('Ctrl Pts',(57.9640600250566,-19.9866097705855,
-55.6739537170499));
#187826=CARTESIAN_POINT('Ctrl Pts',(57.9640789558543,-19.9864534391018,
-55.6744420834266));
#187827=CARTESIAN_POINT('Ctrl Pts',(57.964097851118,-19.9862973972617,-55.6749305015429));
#187828=CARTESIAN_POINT('Ctrl Pts',(57.9681300897667,-19.9529981564453,
-55.7791586525505));
#187829=CARTESIAN_POINT('Ctrl Pts',(57.9705461679584,-19.9328724060776,
-55.885764707647));
#187830=CARTESIAN_POINT('Ctrl Pts',(57.9715251367094,-19.9246984926926,
-55.9945278474385));
#187831=CARTESIAN_POINT('Ctrl Pts',(57.9718656735483,-19.9218551755562,
-56.0323613899058));
#187832=CARTESIAN_POINT('Ctrl Pts',(57.9720322597889,-19.9204585215068,
-56.0704559927497));
#187833=CARTESIAN_POINT('Ctrl Pts',(57.9720322598041,-19.92045852138,-56.1088024963483));
#187834=CARTESIAN_POINT('Ctrl Pts',(58.1440639002148,-20.9985364556095,
-55.3589167601806));
#187835=CARTESIAN_POINT('Ctrl Pts',(57.8386732172432,-20.9542432701794,
-55.231054762791));
#187836=CARTESIAN_POINT('Ctrl Pts',(57.8394345625603,-20.9487258492223,
-54.8970741880307));
#187837=CARTESIAN_POINT('Ctrl Pts',(58.124377168252,-21.1650956023415,-55.357473843553));
#187838=CARTESIAN_POINT('Ctrl Pts',(57.8158059697175,-21.1198442176536,
-55.2308230742677));
#187839=CARTESIAN_POINT('Ctrl Pts',(57.8166617235658,-21.1137591610236,
-54.8942721021231));
#187840=CARTESIAN_POINT('Ctrl Pts',(58.1040803997663,-21.3315995267041,
-55.3559321998119));
#187841=CARTESIAN_POINT('Ctrl Pts',(57.7922771725925,-21.2849855841189,
-55.2305804544121));
#187842=CARTESIAN_POINT('Ctrl Pts',(57.7931832180155,-21.2786902591483,
-54.8913683748515));
#187843=CARTESIAN_POINT('Ctrl Pts',(58.0831736437665,-21.4980516416408,
-55.3542805420642));
#187844=CARTESIAN_POINT('Ctrl Pts',(57.7681097820422,-21.4495803068845,
-55.2303260732311));
#187845=CARTESIAN_POINT('Ctrl Pts',(57.7689991024637,-21.4435190710235,
-54.8883584020537));
#187846=CARTESIAN_POINT('',(57.7689991024637,-21.4435190710235,-54.8883584020537));
#187847=CARTESIAN_POINT('Origin',(58.2637025843942,-21.516103263282,-54.8883584020538));
#187848=CARTESIAN_POINT('Origin',(1.20679687888321,-12.9924344910764,-46.5556728739474));
#187849=CARTESIAN_POINT('Ctrl Pts',(58.0831736437665,-21.4980516416407,
-55.3542805420643));
#187850=CARTESIAN_POINT('Ctrl Pts',(57.7681097820422,-21.4495803068843,
-55.2303260732311));
#187851=CARTESIAN_POINT('Ctrl Pts',(57.7689991024638,-21.4435190710229,
-54.8883584020538));
#187852=CARTESIAN_POINT('Ctrl Pts',(58.0674311963076,-21.5630475770342,
-55.3506990738629));
#187853=CARTESIAN_POINT('Ctrl Pts',(57.7561082976292,-21.5312836766001,
-55.2240269539558));
#187854=CARTESIAN_POINT('Ctrl Pts',(57.7500908600563,-21.5723897392102,
-54.8860050875463));
#187855=CARTESIAN_POINT('Ctrl Pts',(58.0543804972822,-21.6287810566872,
-55.3623310903062));
#187856=CARTESIAN_POINT('Ctrl Pts',(57.7435735661121,-21.6157110452939,
-55.2378962877635));
#187857=CARTESIAN_POINT('Ctrl Pts',(57.7304928612488,-21.702757912867,-54.9116382623115));
#187858=CARTESIAN_POINT('Ctrl Pts',(58.0368385085867,-21.7483268550824,
-55.4143541528288));
#187859=CARTESIAN_POINT('Ctrl Pts',(57.720944678806,-21.7667785312353,-55.3041336540307));
#187860=CARTESIAN_POINT('Ctrl Pts',(57.6941246628956,-21.9398194436421,
-55.0150801896028));
#187861=CARTESIAN_POINT('Ctrl Pts',(58.0322828839583,-21.8027029130102,
-55.4549704742887));
#187862=CARTESIAN_POINT('Ctrl Pts',(57.7106605173207,-21.8347350541072,
-55.3571283178239));
#187863=CARTESIAN_POINT('Ctrl Pts',(57.6771952780886,-22.0476481665544,
-55.0933432841215));
#187864=CARTESIAN_POINT('Ctrl Pts',(58.0344578164564,-21.8906114651791,
-55.5576238485917));
#187865=CARTESIAN_POINT('Ctrl Pts',(57.695076042676,-21.9376161761805,-55.488705776954));
#187866=CARTESIAN_POINT('Ctrl Pts',(57.6494812249724,-22.2219724523816,
-55.2860232465006));
#187867=CARTESIAN_POINT('Ctrl Pts',(58.0412481050148,-21.9247947465257,
-55.6203478572209));
#187868=CARTESIAN_POINT('Ctrl Pts',(57.689647002784,-21.9734580917706,-55.5692031110363));
#187869=CARTESIAN_POINT('Ctrl Pts',(57.6385084201743,-22.2897585279143,
-55.4017143890713));
#187870=CARTESIAN_POINT('Ctrl Pts',(58.0678405993018,-21.9693186886025,
-55.7585030512593));
#187871=CARTESIAN_POINT('Ctrl Pts',(57.6849292160892,-22.0058199931385,
-55.7382976471412));
#187872=CARTESIAN_POINT('Ctrl Pts',(57.6241589914286,-22.3780503291714,
-55.6490268368888));
#187873=CARTESIAN_POINT('Ctrl Pts',(58.0878569699436,-21.9800000199996,
-55.8347456438184));
#187874=CARTESIAN_POINT('Ctrl Pts',(57.6857286259381,-22.0018252542719,
-55.8292768225565));
#187875=CARTESIAN_POINT('Ctrl Pts',(57.6206785404325,-22.3992316104322,
-55.7821117710573));
#187876=CARTESIAN_POINT('Ctrl Pts',(58.1141118834632,-21.98000002,-55.9136064684135));
#187877=CARTESIAN_POINT('Ctrl Pts',(57.6893011240825,-21.9800000200013,
-55.9136064684131));
#187878=CARTESIAN_POINT('Ctrl Pts',(57.6206785412152,-22.3992316056509,
-55.9136064684106));
#187879=CARTESIAN_POINT('',(57.6206785412152,-22.3992316056509,-55.9136064684106));
#187880=CARTESIAN_POINT('Origin',(58.1141118834647,-22.48000002,-55.9136064684106));
#187881=CARTESIAN_POINT('Ctrl Pts',(57.6206785412152,-22.3992316056509,
-55.9136064684106));
#187882=CARTESIAN_POINT('Ctrl Pts',(57.6206785412152,-22.3992316056506,
-55.8712576139305));
#187883=CARTESIAN_POINT('Ctrl Pts',(57.6210388568449,-22.3970387396972,
-55.8289927265007));
#187884=CARTESIAN_POINT('Ctrl Pts',(57.6217580713774,-22.3926459443346,
-55.7870504595467));
#187885=CARTESIAN_POINT('Ctrl Pts',(57.6224751991257,-22.3882658945648,
-55.7452298870977));
#187886=CARTESIAN_POINT('Ctrl Pts',(57.6235491311395,-22.3816988155787,
-55.7037286574053));
#187887=CARTESIAN_POINT('Ctrl Pts',(57.6249866999783,-22.3728877575665,
-55.6627754268272));
#187888=CARTESIAN_POINT('Ctrl Pts',(57.6263702144474,-22.364408006253,-55.6233620884624));
#187889=CARTESIAN_POINT('Ctrl Pts',(57.6280905589435,-22.353849749917,-55.5844551760951));
#187890=CARTESIAN_POINT('Ctrl Pts',(57.6301613121382,-22.341116023378,-55.5462695907389));
#187891=CARTESIAN_POINT('Ctrl Pts',(57.6305151022056,-22.3389404546126,
-55.5397455487364));
#187892=CARTESIAN_POINT('Ctrl Pts',(57.6308791385552,-22.3367012727077,
-55.533242612179));
#187893=CARTESIAN_POINT('Ctrl Pts',(57.6312535111585,-22.3343978551758,
-55.5267619228708));
#187894=CARTESIAN_POINT('Ctrl Pts',(57.631280295686,-22.3342330569249,-55.5262982612688));
#187895=CARTESIAN_POINT('Ctrl Pts',(57.6313071321696,-22.3340679357285,
-55.525834729741));
#187896=CARTESIAN_POINT('Ctrl Pts',(57.6313340206222,-22.3339024914829,
-55.525371328865));
#187897=CARTESIAN_POINT('Ctrl Pts',(57.6359864322556,-22.305276272468,-55.4451907525303));
#187898=CARTESIAN_POINT('Ctrl Pts',(57.6422382498633,-22.2666955115386,
-55.3683025756002));
#187899=CARTESIAN_POINT('Ctrl Pts',(57.6498495152222,-22.2192637924304,
-55.2978189119911));
#187900=CARTESIAN_POINT('Ctrl Pts',(57.6538973328718,-22.1940386898093,
-55.2603343408838));
#187901=CARTESIAN_POINT('Ctrl Pts',(57.6583296672911,-22.166310049833,-55.2246619070089));
#187902=CARTESIAN_POINT('Ctrl Pts',(57.6631104665851,-22.1362429894798,
-55.1912758544359));
#187903=CARTESIAN_POINT('Ctrl Pts',(57.6631864482776,-22.1357651308643,
-55.1907452467652));
#187904=CARTESIAN_POINT('Ctrl Pts',(57.663262518071,-22.1352866810589,-55.1902152153126));
#187905=CARTESIAN_POINT('Ctrl Pts',(57.6633386758179,-22.1348076407421,
-55.1896857620266));
#187906=CARTESIAN_POINT('Ctrl Pts',(57.6719065247416,-22.0809149610449,
-55.1301215555118));
#187907=CARTESIAN_POINT('Ctrl Pts',(57.6816602960296,-22.0190502353779,
-55.0773873317807));
#187908=CARTESIAN_POINT('Ctrl Pts',(57.6921719467781,-21.9515533423725,
-55.0335672587661));
#187909=CARTESIAN_POINT('Ctrl Pts',(57.6985643073562,-21.9105070321098,
-55.0069193312453));
#187910=CARTESIAN_POINT('Ctrl Pts',(57.705236739167,-21.867379079,-54.9835681411996));
#187911=CARTESIAN_POINT('Ctrl Pts',(57.7120915003347,-21.8227047516213,
-54.9639818384176));
#187912=CARTESIAN_POINT('Ctrl Pts',(57.7121639633474,-21.8222324906232,
-54.9637747878039));
#187913=CARTESIAN_POINT('Ctrl Pts',(57.7122364434107,-21.8217600784835,
-54.9635681670512));
#187914=CARTESIAN_POINT('Ctrl Pts',(57.7123089404443,-21.8212875156173,
-54.9633619764799));
#187915=CARTESIAN_POINT('Ctrl Pts',(57.7175256896612,-21.7872827868695,
-54.9485248935223));
#187916=CARTESIAN_POINT('Ctrl Pts',(57.7228431420999,-21.7524063113003,
-54.935873883604));
#187917=CARTESIAN_POINT('Ctrl Pts',(57.7282261110468,-21.716879990905,-54.9253981395351));
#187918=CARTESIAN_POINT('Ctrl Pts',(57.7336334907217,-21.6811925654856,
-54.9148748899834));
#187919=CARTESIAN_POINT('Ctrl Pts',(57.7391071704681,-21.6448481995524,
-54.9065464760172));
#187920=CARTESIAN_POINT('Ctrl Pts',(57.7446130540746,-21.6080564477772,
-54.9004521188838));
#187921=CARTESIAN_POINT('Ctrl Pts',(57.7499689591833,-21.5722668914811,
-54.8945237700776));
#187922=CARTESIAN_POINT('Ctrl Pts',(57.7553555069844,-21.5360528976765,
-54.8907094534876));
#187923=CARTESIAN_POINT('Ctrl Pts',(57.7607401663574,-21.49960966879,-54.8890935200766));
#187924=CARTESIAN_POINT('Ctrl Pts',(57.7634952382929,-21.4809634165034,
-54.8882667244556));
#187925=CARTESIAN_POINT('Ctrl Pts',(57.7662497818651,-21.4622572897838,
-54.8880162223889));
#187926=CARTESIAN_POINT('Ctrl Pts',(57.7689991024637,-21.4435190710235,
-54.8883584020538));
#187927=CARTESIAN_POINT('Origin',(58.1141118834647,-22.48000002,-55.24995));
#187928=CARTESIAN_POINT('',(57.6206785412152,-22.3992316056509,-55.24995));
#187929=CARTESIAN_POINT('Origin',(0.,-12.9675000200281,-60.42825533736));
#187930=CARTESIAN_POINT('Origin',(0.,-12.9675000200281,-60.42825533736));
#187931=CARTESIAN_POINT('Origin',(56.9019881023868,-28.13000002,-55.24995));
#187932=CARTESIAN_POINT('',(56.418846619879,-28.0012587761031,-55.74995));
#187933=CARTESIAN_POINT('',(56.418846619879,-28.0012587761031,-55.24995));
#187934=CARTESIAN_POINT('Origin',(56.9019881023868,-28.13000002,-55.74995));
#187935=CARTESIAN_POINT('Ctrl Pts',(56.9019881023868,-28.63000002,-55.74995));
#187936=CARTESIAN_POINT('Ctrl Pts',(56.2513078496445,-28.6300000199999,
-55.74995));
#187937=CARTESIAN_POINT('Ctrl Pts',(56.418846619879,-28.0012587761031,-55.74995));
#187938=CARTESIAN_POINT('Ctrl Pts',(56.9019880961229,-28.63000002,-55.6833917541491));
#187939=CARTESIAN_POINT('Ctrl Pts',(56.2513078484208,-28.6300000235388,
-55.7066092661189));
#187940=CARTESIAN_POINT('Ctrl Pts',(56.4188466136678,-28.0012587994123,
-55.6168335059946));
#187941=CARTESIAN_POINT('Ctrl Pts',(56.8947679354133,-28.6435819282218,
-55.6165654527396));
#187942=CARTESIAN_POINT('Ctrl Pts',(56.2500205046201,-28.6336048267405,
-55.662915181482));
#187943=CARTESIAN_POINT('Ctrl Pts',(56.4116877572674,-28.0281919581543,
-55.4831809085995));
#187944=CARTESIAN_POINT('Ctrl Pts',(56.8671374536179,-28.6951410554417,
-55.4944276362032));
#187945=CARTESIAN_POINT('Ctrl Pts',(56.2435792593614,-28.6535512137473,
-55.5706051556274));
#187946=CARTESIAN_POINT('Ctrl Pts',(56.3842918802123,-28.1304346451459,
-55.2389052692862));
#187947=CARTESIAN_POINT('Ctrl Pts',(56.8466599215264,-28.733218160043,-55.438805637664));
#187948=CARTESIAN_POINT('Ctrl Pts',(56.2384193392041,-28.6700167701719,
-55.5221237308774));
#187949=CARTESIAN_POINT('Ctrl Pts',(56.3639882171558,-28.2059422564823,
-55.1276612780425));
#187950=CARTESIAN_POINT('Ctrl Pts',(56.7960439448031,-28.8262229205127,
-55.3474998385745));
#187951=CARTESIAN_POINT('Ctrl Pts',(56.2221065093684,-28.7248002564605,
-55.4263976661905));
#187952=CARTESIAN_POINT('Ctrl Pts',(56.313802009893,-28.3903724090483,-54.9450496744345));
#187953=CARTESIAN_POINT('Ctrl Pts',(56.7654715266632,-28.8819195410099,
-55.3110999839041));
#187954=CARTESIAN_POINT('Ctrl Pts',(56.2109691262328,-28.7630648267862,
-55.3789982403422));
#187955=CARTESIAN_POINT('Ctrl Pts',(56.2834891741183,-28.5008198383441,
-54.8722499675113));
#187956=CARTESIAN_POINT('Ctrl Pts',(56.6991996177705,-29.0010091208419,
-55.2626158142325));
#187957=CARTESIAN_POINT('Ctrl Pts',(56.1824656282838,-28.8623399510796,
-55.300226361809));
#187958=CARTESIAN_POINT('Ctrl Pts',(56.2177799652687,-28.7369766748766,
-54.7752816287617));
#187959=CARTESIAN_POINT('Ctrl Pts',(56.6626879858136,-29.0658450537332,
-55.24995));
#187960=CARTESIAN_POINT('Ctrl Pts',(56.1650303807126,-28.9235240815735,
-55.2679072059029));
#187961=CARTESIAN_POINT('Ctrl Pts',(56.1815764992065,-28.8655539935311,
-54.749950013458));
#187962=CARTESIAN_POINT('Ctrl Pts',(56.6260651114328,-29.1300000200001,
-55.24995));
#187963=CARTESIAN_POINT('Ctrl Pts',(56.1452664265556,-28.9927680098115,
-55.24995));
#187964=CARTESIAN_POINT('Ctrl Pts',(56.1452664265556,-28.9927680098115,
-54.74995));
#187965=CARTESIAN_POINT('',(56.1452664265556,-28.9927680098114,-54.74995));
#187966=CARTESIAN_POINT('Ctrl Pts',(56.1452664265556,-28.9927680098114,
-54.74995));
#187967=CARTESIAN_POINT('Ctrl Pts',(56.157135481805,-28.951184226649,-54.7499500043992));
#187968=CARTESIAN_POINT('Ctrl Pts',(56.168934149989,-28.9096618081524,-54.7526528441348));
#187969=CARTESIAN_POINT('Ctrl Pts',(56.1805785937552,-28.8685154650404,
-54.7579280669059));
#187970=CARTESIAN_POINT('Ctrl Pts',(56.1927137076009,-28.825635309661,-54.7634255754322));
#187971=CARTESIAN_POINT('Ctrl Pts',(56.204681702463,-28.7831622366754,-54.7717167436038));
#187972=CARTESIAN_POINT('Ctrl Pts',(56.2163892898622,-28.7414427179697,
-54.7827110993106));
#187973=CARTESIAN_POINT('Ctrl Pts',(56.2280968772615,-28.699723199264,-54.7937054550173));
#187974=CARTESIAN_POINT('Ctrl Pts',(56.239544464813,-28.6587557436148,-54.8074032739245));
#187975=CARTESIAN_POINT('Ctrl Pts',(56.2506343384323,-28.6188990877768,
-54.8237679977477));
#187976=CARTESIAN_POINT('Ctrl Pts',(56.2507584702878,-28.618452961805,-54.823951172381));
#187977=CARTESIAN_POINT('Ctrl Pts',(56.2508825687622,-28.618006934334,-54.8241346982876));
#187978=CARTESIAN_POINT('Ctrl Pts',(56.2510066337442,-28.6175610058129,
-54.824318575259));
#187979=CARTESIAN_POINT('Ctrl Pts',(56.2715808747849,-28.543610720002,-54.8548117012852));
#187980=CARTESIAN_POINT('Ctrl Pts',(56.2911418613678,-28.4727130044645,
-54.8948321838621));
#187981=CARTESIAN_POINT('Ctrl Pts',(56.3090294712616,-28.4074824207886,
-54.9428936399917));
#187982=CARTESIAN_POINT('Ctrl Pts',(56.3196152133162,-28.3688794918917,
-54.9713360188438));
#187983=CARTESIAN_POINT('Ctrl Pts',(56.3296151020253,-28.3322606012602,
-55.0025940679603));
#187984=CARTESIAN_POINT('Ctrl Pts',(56.3388945722868,-28.2981593218029,
-55.0363576523063));
#187985=CARTESIAN_POINT('Ctrl Pts',(56.339029993733,-28.2976616592801,-55.036850386621));
#187986=CARTESIAN_POINT('Ctrl Pts',(56.3391652743153,-28.297164488402,-55.0373436962489));
#187987=CARTESIAN_POINT('Ctrl Pts',(56.3393004137533,-28.2966678103585,
-55.037837579714));
#187988=CARTESIAN_POINT('Ctrl Pts',(56.3561267590158,-28.2348259352745,
-55.0993314990782));
#187989=CARTESIAN_POINT('Ctrl Pts',(56.3707655818743,-28.1806225233929,
-55.1697303039634));
#187990=CARTESIAN_POINT('Ctrl Pts',(56.3826877315525,-28.1363072821715,
-55.2462670316364));
#187991=CARTESIAN_POINT('Ctrl Pts',(56.3884405285137,-28.1149238411049,
-55.2831983121737));
#187992=CARTESIAN_POINT('Ctrl Pts',(56.3935608278327,-28.0958424992937,
-55.3215595430154));
#187993=CARTESIAN_POINT('Ctrl Pts',(56.397989272594,-28.0793153399122,-55.3610440111482));
#187994=CARTESIAN_POINT('Ctrl Pts',(56.3980423761537,-28.0791171549869,
-55.3615174879381));
#187995=CARTESIAN_POINT('Ctrl Pts',(56.3980953812291,-28.0789193343635,
-55.3619911356046));
#187996=CARTESIAN_POINT('Ctrl Pts',(56.3981482877874,-28.0787218781893,
-55.3624649534454));
#187997=CARTESIAN_POINT('Ctrl Pts',(56.4020846045284,-28.0640308820639,
-55.3977176169507));
#187998=CARTESIAN_POINT('Ctrl Pts',(56.4054635861547,-28.0514021107091,
-55.4337954284409));
#187999=CARTESIAN_POINT('Ctrl Pts',(56.4082873243379,-28.0408381674741,
-55.4705044074015));
#188000=CARTESIAN_POINT('Ctrl Pts',(56.4111187646799,-28.030245409539,-55.5073135154709));
#188001=CARTESIAN_POINT('Ctrl Pts',(56.4133919882818,-28.0217284962734,
-55.5447583433603));
#188002=CARTESIAN_POINT('Ctrl Pts',(56.4150963311521,-28.0153374570685,
-55.5826612239241));
#188003=CARTESIAN_POINT('Ctrl Pts',(56.4167572958903,-28.0091090795838,
-55.6195994182211));
#188004=CARTESIAN_POINT('Ctrl Pts',(56.4178779761682,-28.0048996781119,
-55.6569736701745));
#188005=CARTESIAN_POINT('Ctrl Pts',(56.4184359903581,-28.0028025535954,
-55.6946207896264));
#188006=CARTESIAN_POINT('Ctrl Pts',(56.4187084931304,-28.0017784358308,
-55.7130055271623));
#188007=CARTESIAN_POINT('Ctrl Pts',(56.4188466190161,-28.0012587793416,
-55.7314552635405));
#188008=CARTESIAN_POINT('Ctrl Pts',(56.418846619879,-28.0012587761031,-55.74995));
#188009=CARTESIAN_POINT('Origin',(56.6260651114328,-29.13000002,-54.74995));
#188010=CARTESIAN_POINT('Origin',(0.,-12.9675000200281,-54.74995));
#188011=CARTESIAN_POINT('',(56.0013925566522,-29.4885226266656,-54.74995));
#188012=CARTESIAN_POINT('Origin',(0.,-12.9675000200281,-54.74995));
#188013=CARTESIAN_POINT('Origin',(56.4809591809864,-29.63000002,-54.74995));
#188014=CARTESIAN_POINT('Ctrl Pts',(56.4809591809864,-29.63000002,-55.24995));
#188015=CARTESIAN_POINT('Ctrl Pts',(56.0013925566522,-29.4885226266655,
-55.2499499999999));
#188016=CARTESIAN_POINT('Ctrl Pts',(56.0013925566522,-29.4885226266656,
-54.74995));
#188017=CARTESIAN_POINT('Ctrl Pts',(56.4430235619105,-29.6942952977694,
-55.24995));
#188018=CARTESIAN_POINT('Ctrl Pts',(55.9815963325889,-29.5556259878439,
-55.2320894585059));
#188019=CARTESIAN_POINT('Ctrl Pts',(55.9637778607192,-29.6160253486821,
-54.7499500197391));
#188020=CARTESIAN_POINT('Ctrl Pts',(56.4048920758008,-29.7580863098899,
-55.2623271401185));
#188021=CARTESIAN_POINT('Ctrl Pts',(55.9595264494602,-29.6302973578872,
-55.2276198610214));
#188022=CARTESIAN_POINT('Ctrl Pts',(55.9259713199402,-29.7425201026704,
-54.7747042862246));
#188023=CARTESIAN_POINT('Ctrl Pts',(56.3324398513309,-29.877933435243,-55.3109611929186));
#188024=CARTESIAN_POINT('Ctrl Pts',(55.9152124797534,-29.7792875750423,
-55.2543206061649));
#188025=CARTESIAN_POINT('Ctrl Pts',(55.8541342694537,-29.9801791700519,
-54.8719723798496));
#188026=CARTESIAN_POINT('Ctrl Pts',(56.2987519266105,-29.9329514036474,
-55.3468561181883));
#188027=CARTESIAN_POINT('Ctrl Pts',(55.8932648786607,-29.8526235485765,
-55.2844345178149));
#188028=CARTESIAN_POINT('Ctrl Pts',(55.8207323820705,-30.0892808127342,
-54.9437622390698));
#188029=CARTESIAN_POINT('Ctrl Pts',(56.2123326186624,-30.0729950473548,
-55.4838442327376));
#188030=CARTESIAN_POINT('Ctrl Pts',(55.8363250868006,-30.0417896984651,
-55.4221362713026));
#188031=CARTESIAN_POINT('Ctrl Pts',(55.7350468385274,-30.3669899517508,
-55.2177384600888));
#188032=CARTESIAN_POINT('Ctrl Pts',(56.1762739146114,-30.1300000200003,
-55.614004390749));
#188033=CARTESIAN_POINT('Ctrl Pts',(55.8093485438182,-30.1300000005986,
-55.5818806132723));
#188034=CARTESIAN_POINT('Ctrl Pts',(55.699294301712,-30.4800318342627,-55.4780587856325));
#188035=CARTESIAN_POINT('Ctrl Pts',(56.1762739063772,-30.1300000200003,
-55.74995));
#188036=CARTESIAN_POINT('Ctrl Pts',(55.8093485379488,-30.1300000200003,
-55.7499499999999));
#188037=CARTESIAN_POINT('Ctrl Pts',(55.6992942935022,-30.4800318603742,
-55.74995));
#188038=CARTESIAN_POINT('',(55.6992942935022,-30.4800318603739,-55.74995));
#188039=CARTESIAN_POINT('Ctrl Pts',(55.6992942935022,-30.4800318603742,
-55.74995));
#188040=CARTESIAN_POINT('Ctrl Pts',(55.6992942945104,-30.4800318571677,
-55.7165618050259));
#188041=CARTESIAN_POINT('Ctrl Pts',(55.6998330297483,-30.4783285093804,
-55.6833050175431));
#188042=CARTESIAN_POINT('Ctrl Pts',(55.7008904740051,-30.4749766534797,
-55.6502628336504));
#188043=CARTESIAN_POINT('Ctrl Pts',(55.7022012337469,-30.4708218455575,
-55.6093052473247));
#188044=CARTESIAN_POINT('Ctrl Pts',(55.704311824946,-30.4641251495371,-55.5686774361727));
#188045=CARTESIAN_POINT('Ctrl Pts',(55.7071988207748,-30.4549435229948,
-55.5285389205525));
#188046=CARTESIAN_POINT('Ctrl Pts',(55.7078054138863,-30.4530143510309,
-55.520105327806));
#188047=CARTESIAN_POINT('Ctrl Pts',(55.7084463261485,-30.4509753351475,
-55.5116934444067));
#188048=CARTESIAN_POINT('Ctrl Pts',(55.7091214061603,-30.4488267863995,
-55.5033049359167));
#188049=CARTESIAN_POINT('Ctrl Pts',(55.7110654210346,-30.4426396520572,
-55.4791487099962));
#188050=CARTESIAN_POINT('Ctrl Pts',(55.7132913748237,-30.4355486844701,
-55.4551844602832));
#188051=CARTESIAN_POINT('Ctrl Pts',(55.7157933833999,-30.4275683986656,
-55.4314477302124));
#188052=CARTESIAN_POINT('Ctrl Pts',(55.718295391976,-30.4195881128611,-55.4077110001416));
#188053=CARTESIAN_POINT('Ctrl Pts',(55.7210734551748,-30.4107185086403,
-55.3842017897311));
#188054=CARTESIAN_POINT('Ctrl Pts',(55.724121621672,-30.4009740809159,-55.3609556432104));
#188055=CARTESIAN_POINT('Ctrl Pts',(55.7281858436682,-30.3879815106165,
-55.3299607811827));
#188056=CARTESIAN_POINT('Ctrl Pts',(55.7326675876837,-30.373634015077,-55.2999843610343));
#188057=CARTESIAN_POINT('Ctrl Pts',(55.7375386580734,-30.3580127797202,
-55.2709916628686));
#188058=CARTESIAN_POINT('Ctrl Pts',(55.7422761695128,-30.3428198600378,
-55.2427939099668));
#188059=CARTESIAN_POINT('Ctrl Pts',(55.7473822073897,-30.3264213210404,
-55.2155261265394));
#188060=CARTESIAN_POINT('Ctrl Pts',(55.7528459976329,-30.3088429857846,
-55.1891766996987));
#188061=CARTESIAN_POINT('Ctrl Pts',(55.7585408389563,-30.2905213032979,
-55.1617130164057));
#188062=CARTESIAN_POINT('Ctrl Pts',(55.7646244097769,-30.2709177421356,
-55.1352460408554));
#188063=CARTESIAN_POINT('Ctrl Pts',(55.7710988761824,-30.2500142965945,
-55.1097968023626));
#188064=CARTESIAN_POINT('Ctrl Pts',(55.7772054795241,-30.230298532793,-55.0857935262488));
#188065=CARTESIAN_POINT('Ctrl Pts',(55.7836600583737,-30.2094256741772,
-55.0626953151138));
#188066=CARTESIAN_POINT('Ctrl Pts',(55.7904742625662,-30.1873473542624,
-55.0405578359032));
#188067=CARTESIAN_POINT('Ctrl Pts',(55.7908847516535,-30.186017351648,-55.0392242695204));
#188068=CARTESIAN_POINT('Ctrl Pts',(55.7912965483067,-30.1846829658094,
-55.0378942024439));
#188069=CARTESIAN_POINT('Ctrl Pts',(55.7917096560192,-30.1833441828804,
-55.0365676519554));
#188070=CARTESIAN_POINT('Ctrl Pts',(55.7918632993036,-30.1828462618782,
-55.0360742804503));
#188071=CARTESIAN_POINT('Ctrl Pts',(55.7920170835031,-30.1823478636952,
-55.0355815185873));
#188072=CARTESIAN_POINT('Ctrl Pts',(55.792171008419,-30.1818489888761,-55.0350893667936));
#188073=CARTESIAN_POINT('Ctrl Pts',(55.800290879717,-30.1555322662012,-55.0091272982118));
#188074=CARTESIAN_POINT('Ctrl Pts',(55.8087607420851,-30.1280129936589,
-54.9848694510044));
#188075=CARTESIAN_POINT('Ctrl Pts',(55.8175466321019,-30.0993860830431,
-54.9622897882634));
#188076=CARTESIAN_POINT('Ctrl Pts',(55.8264122965254,-30.0704992448839,
-54.9395051059746));
#188077=CARTESIAN_POINT('Ctrl Pts',(55.8355999692742,-30.0404839357451,
-54.9184288364593));
#188078=CARTESIAN_POINT('Ctrl Pts',(55.845084553161,-30.0094041347627,-54.8990745550387));
#188079=CARTESIAN_POINT('Ctrl Pts',(55.854533149884,-29.9784422592366,-54.8797937091743));
#188080=CARTESIAN_POINT('Ctrl Pts',(55.8642766342982,-29.946423293465,-54.8622214688159));
#188081=CARTESIAN_POINT('Ctrl Pts',(55.8742965418741,-29.913387106528,-54.8464163971206));
#188082=CARTESIAN_POINT('Ctrl Pts',(55.8793448400683,-29.8967425894409,
-54.8384533780713));
#188083=CARTESIAN_POINT('Ctrl Pts',(55.8844633853516,-29.8798395511654,
-54.8309396845163));
#188084=CARTESIAN_POINT('Ctrl Pts',(55.889650155579,-29.862681631768,-54.8238876164085));
#188085=CARTESIAN_POINT('Ctrl Pts',(55.8897844414451,-29.8622374119616,
-54.8237050378419));
#188086=CARTESIAN_POINT('Ctrl Pts',(55.8899187507015,-29.8617930951974,
-54.8235227993659));
#188087=CARTESIAN_POINT('Ctrl Pts',(55.8900530833078,-29.861348681574,-54.8233409008622));
#188088=CARTESIAN_POINT('Ctrl Pts',(55.8995504810642,-29.8299283654799,
-54.8104805649473));
#188089=CARTESIAN_POINT('Ctrl Pts',(55.9091201713665,-29.7981698989578,
-54.7993661329088));
#188090=CARTESIAN_POINT('Ctrl Pts',(55.9187569872376,-29.7660885799508,
-54.7899280455082));
#188091=CARTESIAN_POINT('Ctrl Pts',(55.9284529762139,-29.7338102714721,
-54.7804320052583));
#188092=CARTESIAN_POINT('Ctrl Pts',(55.938217108462,-29.7012045233227,-54.7726328698961));
#188093=CARTESIAN_POINT('Ctrl Pts',(55.9480481282842,-29.6682706672262,
-54.7665101842522));
#188094=CARTESIAN_POINT('Ctrl Pts',(55.9578188295005,-29.6355388780897,
-54.7604250645851));
#188095=CARTESIAN_POINT('Ctrl Pts',(55.9676557893865,-29.6024823867339,
-54.7559958377295));
#188096=CARTESIAN_POINT('Ctrl Pts',(55.9775588733957,-29.5690936714574,
-54.7532529199582));
#188097=CARTESIAN_POINT('Ctrl Pts',(55.9854615290049,-29.5424494949745,
-54.7510640730807));
#188098=CARTESIAN_POINT('Ctrl Pts',(55.9934063510512,-29.5155935075394,
-54.7499500041909));
#188099=CARTESIAN_POINT('Ctrl Pts',(56.0013925566522,-29.4885226266656,
-54.74995));
#188100=CARTESIAN_POINT('Origin',(56.1762739063772,-30.63000002,-55.74995));
#188101=CARTESIAN_POINT('Origin',(56.1762739063772,-30.63000002,-55.24995));
#188102=CARTESIAN_POINT('',(55.6992942935022,-30.4800318603739,-55.24995));
#188103=CARTESIAN_POINT('Origin',(0.,-12.9675000200281,-60.42825533736));
#188104=CARTESIAN_POINT('Origin',(0.,-12.9675000200281,-60.42825533736));
#188105=CARTESIAN_POINT('Origin',(54.076473627675,-36.28000002,-55.24995));
#188106=CARTESIAN_POINT('',(53.6173229282256,-36.0820590308261,-55.74995));
#188107=CARTESIAN_POINT('Origin',(54.076473627675,-36.28000002,-55.74995));
#188108=CARTESIAN_POINT('',(53.6173229282256,-36.0820590308261,-55.24995));
#188109=CARTESIAN_POINT('Ctrl Pts',(54.076473627675,-36.78000002,-55.74995));
#188110=CARTESIAN_POINT('Ctrl Pts',(53.3164388612999,-36.78000002,-55.7499499999999));
#188111=CARTESIAN_POINT('Ctrl Pts',(53.6173229282256,-36.0820590308261,
-55.74995));
#188112=CARTESIAN_POINT('Ctrl Pts',(54.07647361027,-36.78000002,-55.6425914202082));
#188113=CARTESIAN_POINT('Ctrl Pts',(53.3164388632929,-36.7800000140484,
-55.7160682965194));
#188114=CARTESIAN_POINT('Ctrl Pts',(53.6173229109667,-36.0820590708605,
-55.5352328299022));
#188115=CARTESIAN_POINT('Ctrl Pts',(54.0462927577141,-36.8151341090744,
-55.5384961709319));
#188116=CARTESIAN_POINT('Ctrl Pts',(53.3223470981189,-36.7637806572682,
-55.672084159207));
#188117=CARTESIAN_POINT('Ctrl Pts',(53.587398316273,-36.1517305970246,-55.3270423559178));
#188118=CARTESIAN_POINT('Ctrl Pts',(53.939326192416,-36.9379861363991,-55.370688163807));
#188119=CARTESIAN_POINT('Ctrl Pts',(53.3111802821853,-36.783202746029,-55.5229519438579));
#188120=CARTESIAN_POINT('Ctrl Pts',(53.481339980492,-36.3953483985127,-54.9914263135601));
#188121=CARTESIAN_POINT('Ctrl Pts',(53.8654589377065,-37.0221914881654,
-55.3103188190833));
#188122=CARTESIAN_POINT('Ctrl Pts',(53.293833750711,-36.8201344622738,-55.429912748872));
#188123=CARTESIAN_POINT('Ctrl Pts',(53.4080974646291,-36.562334686105,-54.8706857163843));
#188124=CARTESIAN_POINT('Ctrl Pts',(53.7823432375794,-37.1153847305999,
-55.2778252214766));
#188125=CARTESIAN_POINT('Ctrl Pts',(53.2549772028899,-36.9057059891941,
-55.3509337052243));
#188126=CARTESIAN_POINT('Ctrl Pts',(53.3256899305316,-36.747133105635,-54.8057004429533));
#188127=CARTESIAN_POINT('',(53.3256899305366,-36.7471331056238,-54.8057004429536));
#188128=CARTESIAN_POINT('Origin',(53.7823432375799,-36.9507694411988,-54.8057004429536));
#188129=CARTESIAN_POINT('Ctrl Pts',(53.3256899305362,-36.7471331056248,
-54.8057004429569));
#188130=CARTESIAN_POINT('Ctrl Pts',(53.3365047080717,-36.7228810294277,
-54.8142288048715));
#188131=CARTESIAN_POINT('Ctrl Pts',(53.347033550176,-36.6992232138251,-54.8236117045923));
#188132=CARTESIAN_POINT('Ctrl Pts',(53.3573294859536,-36.6760484250078,
-54.833842030096));
#188133=CARTESIAN_POINT('Ctrl Pts',(53.3676295626462,-36.6528643155391,
-54.8440764701269));
#188134=CARTESIAN_POINT('Ctrl Pts',(53.3776967400546,-36.6301631323027,
-54.855159268536));
#188135=CARTESIAN_POINT('Ctrl Pts',(53.3875763712775,-36.6078483738899,
-54.8671326577126));
#188136=CARTESIAN_POINT('Ctrl Pts',(53.3972846011521,-36.5859207533766,
-54.8788983210135));
#188137=CARTESIAN_POINT('Ctrl Pts',(53.406811903452,-36.5643658402485,-54.891524208438));
#188138=CARTESIAN_POINT('Ctrl Pts',(53.4161912134876,-36.5431130768774,
-54.9050940181005));
#188139=CARTESIAN_POINT('Ctrl Pts',(53.4247320031921,-36.5237603332428,
-54.9174506722911));
#188140=CARTESIAN_POINT('Ctrl Pts',(53.4331500860381,-36.5046580712458,
-54.9305905504039));
#188141=CARTESIAN_POINT('Ctrl Pts',(53.4414609284995,-36.4857733835863,
-54.9446070495014));
#188142=CARTESIAN_POINT('Ctrl Pts',(53.4509986505366,-36.4641008633228,
-54.9606927198705));
#188143=CARTESIAN_POINT('Ctrl Pts',(53.4601425635063,-36.4432889157824,
-54.9775073786436));
#188144=CARTESIAN_POINT('Ctrl Pts',(53.4689373117184,-36.4232432529379,
-54.9950729719853));
#188145=CARTESIAN_POINT('Ctrl Pts',(53.4776988122795,-36.4032733706824,
-55.0125721603883));
#188146=CARTESIAN_POINT('Ctrl Pts',(53.4861139520167,-36.3840635594153,
-55.0308169094228));
#188147=CARTESIAN_POINT('Ctrl Pts',(53.4942155666396,-36.3655444879779,
-55.0498730291534));
#188148=CARTESIAN_POINT('Ctrl Pts',(53.5021531960704,-36.3474002620039,
-55.0685434329988));
#188149=CARTESIAN_POINT('Ctrl Pts',(53.509789997807,-36.3299187504364,-55.0879929870304));
#188150=CARTESIAN_POINT('Ctrl Pts',(53.5171438153628,-36.3130633064965,
-55.1083215416835));
#188151=CARTESIAN_POINT('Ctrl Pts',(53.5230683586813,-36.2994838551412,
-55.1246990764445));
#188152=CARTESIAN_POINT('Ctrl Pts',(53.5288090292654,-36.2863111840396,
-55.1416478579265));
#188153=CARTESIAN_POINT('Ctrl Pts',(53.5343678189769,-36.2735425514815,
-55.1592369940626));
#188154=CARTESIAN_POINT('Ctrl Pts',(53.5344871593642,-36.2732684246241,
-55.1596146112107));
#188155=CARTESIAN_POINT('Ctrl Pts',(53.5346064010008,-36.272994519867,-55.1599924902182));
#188156=CARTESIAN_POINT('Ctrl Pts',(53.534725543904,-36.2727208371876,-55.1603706315252));
#188157=CARTESIAN_POINT('Ctrl Pts',(53.5416014628259,-36.2569261917407,
-55.1821937439223));
#188158=CARTESIAN_POINT('Ctrl Pts',(53.5480238717073,-36.2421576554038,
-55.2044892728991));
#188159=CARTESIAN_POINT('Ctrl Pts',(53.5540298412575,-36.2283345422306,
-55.2272840027525));
#188160=CARTESIAN_POINT('Ctrl Pts',(53.5600584943761,-36.2144592214114,
-55.2501648245862));
#188161=CARTESIAN_POINT('Ctrl Pts',(53.5656676548917,-36.2015362223129,
-55.2735491895684));
#188162=CARTESIAN_POINT('Ctrl Pts',(53.5708774015945,-36.1895232328314,
-55.2974947075211));
#188163=CARTESIAN_POINT('Ctrl Pts',(53.5760229208745,-36.1776583433246,
-55.3211450174732));
#188164=CARTESIAN_POINT('Ctrl Pts',(53.5807788918407,-36.1666809556098,
-55.3453432833983));
#188165=CARTESIAN_POINT('Ctrl Pts',(53.5851464697891,-36.1565918414746,
-55.3701663329474));
#188166=CARTESIAN_POINT('Ctrl Pts',(53.5890231720465,-36.1476366512055,
-55.3921994994665));
#188167=CARTESIAN_POINT('Ctrl Pts',(53.5925937005088,-36.139381680042,-55.4147254208055));
#188168=CARTESIAN_POINT('Ctrl Pts',(53.5958456670774,-36.1318578925515,
-55.4378070838457));
#188169=CARTESIAN_POINT('Ctrl Pts',(53.6001803589108,-36.1218290993573,
-55.4685736659031));
#188170=CARTESIAN_POINT('Ctrl Pts',(53.6038427283339,-36.1133454971332,
-55.4995748163826));
#188171=CARTESIAN_POINT('Ctrl Pts',(53.6068550156883,-36.1063621989411,
-55.5307884996878));
#188172=CARTESIAN_POINT('Ctrl Pts',(53.6098729740293,-36.0993657538655,
-55.5620609464382));
#188173=CARTESIAN_POINT('Ctrl Pts',(53.6122384934281,-36.0938750177308,
-55.5935474015465));
#188174=CARTESIAN_POINT('Ctrl Pts',(53.6139551145697,-36.0898877949595,
-55.6252487013041));
#188175=CARTESIAN_POINT('Ctrl Pts',(53.6156514736902,-36.0859476351017,
-55.6565758169199));
#188176=CARTESIAN_POINT('Ctrl Pts',(53.6167142276579,-36.0834755230399,
-55.6881133687363));
#188177=CARTESIAN_POINT('Ctrl Pts',(53.6171273211733,-36.0825142809585,
-55.7198748365422));
#188178=CARTESIAN_POINT('Ctrl Pts',(53.6172574163426,-36.0822115578542,
-55.7298774470373));
#188179=CARTESIAN_POINT('Ctrl Pts',(53.617322927418,-36.0820590326995,-55.7399023232672));
#188180=CARTESIAN_POINT('Ctrl Pts',(53.6173229282256,-36.0820590308261,
-55.74995));
#188181=CARTESIAN_POINT('Origin',(24.5275331667447,40.0183497231583,-52.64995));
#188182=CARTESIAN_POINT('',(25.3802177275058,39.9437494905281,-52.64995));
#188183=CARTESIAN_POINT('',(25.3802177275058,39.9437494905281,-52.64995));
#188184=CARTESIAN_POINT('',(43.1064181712417,38.392907904313,-52.64995));
#188185=CARTESIAN_POINT('',(24.5275331667447,40.0183497231583,-52.64995));
#188186=CARTESIAN_POINT('',(43.1064181712417,38.392907904313,-52.64995));
#188187=CARTESIAN_POINT('Origin',(42.8449509429988,35.4043238100378,-59.64995));
#188188=CARTESIAN_POINT('Origin',(42.8449509429988,35.4043238100378,-59.64995));
#188189=CARTESIAN_POINT('Origin',(44.1941738241593,38.2977416159964,-52.64995));
#188190=CARTESIAN_POINT('',(50.4931441736257,31.9987712665301,-52.64995));
#188191=CARTESIAN_POINT('',(50.4931441736257,31.9987712665301,-52.64995));
#188192=CARTESIAN_POINT('',(44.9662712865584,37.5256441535974,-52.64995));
#188193=CARTESIAN_POINT('',(44.9662712865584,37.5256441535974,-52.64995));
#188194=CARTESIAN_POINT('',(44.1941738241593,38.2977416159964,-52.64995));
#188195=CARTESIAN_POINT('Origin',(42.8449509429988,35.4043238100378,-52.64995));
#188196=CARTESIAN_POINT('Origin',(42.8449509429988,35.4043238100378,-52.64995));
#188197=CARTESIAN_POINT('Origin',(48.3718238300661,29.8774509229704,-59.64995));
#188198=CARTESIAN_POINT('Origin',(48.3718238300661,29.8774509229704,-59.64995));
#188199=CARTESIAN_POINT('Origin',(51.2652416360248,31.226673804131,-52.64995));
#188200=CARTESIAN_POINT('',(51.3604079243413,30.1389181512134,-52.64995));
#188201=CARTESIAN_POINT('',(51.3604079243413,30.1389181512134,-52.64995));
#188202=CARTESIAN_POINT('',(52.9112495105564,12.4127177074772,-52.64995));
#188203=CARTESIAN_POINT('',(51.2652416360248,31.226673804131,-52.64995));
#188204=CARTESIAN_POINT('',(52.9112495105564,12.4127177074773,-55.24995));
#188205=CARTESIAN_POINT('Origin',(48.3718238300661,29.8774509229704,-52.64995));
#188206=CARTESIAN_POINT('Origin',(48.3718238300661,29.8774509229704,-52.64995));
#188207=CARTESIAN_POINT('Ctrl Pts',(53.0821522164592,11.4835005182672,-54.749226640207));
#188208=CARTESIAN_POINT('Ctrl Pts',(53.0814553265489,11.4833027557155,-55.24995));
#188209=CARTESIAN_POINT('Ctrl Pts',(53.5631588418786,11.61999998,-55.24995));
#188210=CARTESIAN_POINT('Ctrl Pts',(53.0314894680352,11.6620294726881,-54.7492424048586));
#188211=CARTESIAN_POINT('Ctrl Pts',(53.0524992546297,11.5855117152954,-55.2284093535366));
#188212=CARTESIAN_POINT('Ctrl Pts',(53.5175339525391,11.7003881248737,-55.24995));
#188213=CARTESIAN_POINT('Ctrl Pts',(52.9910538795555,11.8458000768038,-54.7896174675006));
#188214=CARTESIAN_POINT('Ctrl Pts',(53.0226612146944,11.6989200777954,-55.238154595146));
#188215=CARTESIAN_POINT('Ctrl Pts',(53.481213741953,11.782936109662,-55.2701189042654));
#188216=CARTESIAN_POINT('Ctrl Pts',(52.9359085954001,12.1689324824227,-54.9449932254243));
#188217=CARTESIAN_POINT('Ctrl Pts',(52.9757607799671,11.8899765016028,-55.3144933675901));
#188218=CARTESIAN_POINT('Ctrl Pts',(53.4315945187188,11.9282552364233,-55.3477500998626));
#188219=CARTESIAN_POINT('Ctrl Pts',(52.9200762514753,12.3116974252973,-55.0618112506234));
#188220=CARTESIAN_POINT('Ctrl Pts',(52.9570824697211,11.9716603673777,-55.3811270199801));
#188221=CARTESIAN_POINT('Ctrl Pts',(53.4173436672944,11.9924457375215,-55.4061007701193));
#188222=CARTESIAN_POINT('Ctrl Pts',(52.9111992844441,12.4132973608818,-55.2012882697194));
#188223=CARTESIAN_POINT('Ctrl Pts',(52.9444394937624,12.0259207443505,-55.4571605585729));
#188224=CARTESIAN_POINT('Ctrl Pts',(53.4093468596018,12.0381477794281,-55.475810586866));
#188225=CARTESIAN_POINT('',(53.0821517130856,11.4835003754205,-54.74995));
#188226=CARTESIAN_POINT('Origin',(53.5631588418786,11.61999998,-54.74995));
#188227=CARTESIAN_POINT('Ctrl Pts',(53.0821517130856,11.4835003754205,-54.74995));
#188228=CARTESIAN_POINT('Ctrl Pts',(53.0564462519378,11.5740831291147,-54.74995));
#188229=CARTESIAN_POINT('Ctrl Pts',(53.0341440975299,11.6624073741825,-54.7594183008898));
#188230=CARTESIAN_POINT('Ctrl Pts',(53.0051082177742,11.79112063162,-54.7878232035592));
#188231=CARTESIAN_POINT('Ctrl Pts',(52.9916948966,11.8545354170554,-54.8055762677276));
#188232=CARTESIAN_POINT('Ctrl Pts',(52.9798127489238,11.9164774315466,-54.8286552511465));
#188233=CARTESIAN_POINT('Ctrl Pts',(52.9722178731516,11.9574389462162,-54.8452247777036));
#188234=CARTESIAN_POINT('Ctrl Pts',(52.9687758404164,11.9766401182258,-54.8535781982143));
#188235=CARTESIAN_POINT('Ctrl Pts',(52.9357472552443,12.1679591460758,-54.943500910384));
#188236=CARTESIAN_POINT('Ctrl Pts',(52.9205204470379,12.3067504185984,-55.0562014313995));
#188237=CARTESIAN_POINT('Ctrl Pts',(52.9112495105564,12.4127177074773,-55.2016711737242));
#188238=CARTESIAN_POINT('Origin',(57.8922230010151,12.8484964212155,-54.74995));
#188239=CARTESIAN_POINT('',(53.275786978871,10.927944819865,-54.74995));
#188240=CARTESIAN_POINT('Origin',(53.7374305810854,11.11999998,-54.74995));
#188241=CARTESIAN_POINT('Origin',(57.8922230010151,12.8484964212155,-54.74995));
#188242=CARTESIAN_POINT('Ctrl Pts',(53.3256899305368,10.8121330655672,-54.7553968408231));
#188243=CARTESIAN_POINT('Ctrl Pts',(53.3054454943535,10.8575310968505,-55.2747187747876));
#188244=CARTESIAN_POINT('Ctrl Pts',(53.7823432375846,11.067884690566,-55.2526734204115));
#188245=CARTESIAN_POINT('Ctrl Pts',(53.3086079255675,10.8504393631076,-54.7517837407593));
#188246=CARTESIAN_POINT('Ctrl Pts',(53.2957533879043,10.880281535778,-55.2650191833929));
#188247=CARTESIAN_POINT('Ctrl Pts',(53.7669694165083,11.0851225427625,-55.2508668691012));
#188248=CARTESIAN_POINT('Ctrl Pts',(53.2919715007789,10.8890420328302,-54.7499500043796));
#188249=CARTESIAN_POINT('Ctrl Pts',(53.2858304006402,10.9038034191885,-55.2567197573796));
#188250=CARTESIAN_POINT('Ctrl Pts',(53.7519966717624,11.1024937011227,-55.24995));
#188251=CARTESIAN_POINT('Ctrl Pts',(53.275786978871,10.927944819865,-54.74995));
#188252=CARTESIAN_POINT('Ctrl Pts',(53.275786978871,10.927944819865,-55.24995));
#188253=CARTESIAN_POINT('Ctrl Pts',(53.7374305810854,11.11999998,-55.24995));
#188254=CARTESIAN_POINT('Origin',(53.6412833044364,11.0802639242609,-56.1025073833426));
#188255=CARTESIAN_POINT('Origin',(0.,-12.9675000200281,-55.24995));
#188256=CARTESIAN_POINT('',(53.3256899305366,-36.7471331056238,-52.64995));
#188257=CARTESIAN_POINT('',(53.3256899305368,10.8121330655672,-52.64995));
#188258=CARTESIAN_POINT('Origin',(0.,-12.9675000200281,-52.64995));
#188259=CARTESIAN_POINT('',(53.3256899305366,-36.7471331056238,-55.24995));
#188260=CARTESIAN_POINT('',(53.3256899305368,10.8121330655672,-55.24995));
#188261=CARTESIAN_POINT('Origin',(57.8922230010151,12.8484964212155,-55.24995));
#188262=CARTESIAN_POINT('Origin',(57.8922230010151,12.8484964212155,-52.64995));
#188263=CARTESIAN_POINT('Ctrl Pts',(53.1795531264094,-37.1129448598586,
-54.74995));
#188264=CARTESIAN_POINT('Ctrl Pts',(53.1795531264094,-37.1129448598586,
-55.24995));
#188265=CARTESIAN_POINT('Ctrl Pts',(53.65082011387,-37.28000002,-55.24995));
#188266=CARTESIAN_POINT('Ctrl Pts',(53.2245914375472,-36.9858906030954,
-54.74995002559));
#188267=CARTESIAN_POINT('Ctrl Pts',(53.2071047405196,-37.0352210513017,
-55.2694186883497));
#188268=CARTESIAN_POINT('Ctrl Pts',(53.6913582052585,-37.222820517008,-55.24995));
#188269=CARTESIAN_POINT('Ctrl Pts',(53.2735999108999,-36.8639446739783,
-54.7690447340998));
#188270=CARTESIAN_POINT('Ctrl Pts',(53.233451048998,-36.9645829953838,-55.3049428618926));
#188271=CARTESIAN_POINT('Ctrl Pts',(53.7354566371443,-37.1679561903806,
-55.2594951814958));
#188272=CARTESIAN_POINT('Ctrl Pts',(53.3256899305359,-36.7471331056253,
-54.8057004429567));
#188273=CARTESIAN_POINT('Ctrl Pts',(53.2549772028919,-36.90570598919,-55.3509337052282));
#188274=CARTESIAN_POINT('Ctrl Pts',(53.7823432375838,-37.115384730595,-55.2778252214784));
#188275=CARTESIAN_POINT('',(53.1795531264094,-37.1129448598587,-54.74995));
#188276=CARTESIAN_POINT('Origin',(53.65082011387,-37.28000002,-54.74995));
#188277=CARTESIAN_POINT('Ctrl Pts',(53.1795531264094,-37.1129448598586,
-54.74995));
#188278=CARTESIAN_POINT('Ctrl Pts',(53.203745009962,-37.044698921971,-54.7499500137454));
#188279=CARTESIAN_POINT('Ctrl Pts',(53.229115357639,-36.9778304553021,-54.7554548649733));
#188280=CARTESIAN_POINT('Ctrl Pts',(53.2555724802121,-36.9122732840969,
-54.7662993117297));
#188281=CARTESIAN_POINT('Ctrl Pts',(53.2781697189556,-36.8562803829422,
-54.7755616399258));
#188282=CARTESIAN_POINT('Ctrl Pts',(53.301560005639,-36.8012443229208,-54.7887202323916));
#188283=CARTESIAN_POINT('Ctrl Pts',(53.3256899305359,-36.7471331056253,
-54.8057004429567));
#188284=CARTESIAN_POINT('Origin',(57.8922230010149,-38.7834964612722,-54.74995));
#188285=CARTESIAN_POINT('',(53.0181298732915,-37.6685004154142,-54.74995));
#188286=CARTESIAN_POINT('Origin',(53.5055391860638,-37.78000002,-54.74995));
#188287=CARTESIAN_POINT('Origin',(57.8922230010149,-38.7834964612722,-54.74995));
#188288=CARTESIAN_POINT('Ctrl Pts',(52.9112495105562,-38.347717747534,-54.9585476429427));
#188289=CARTESIAN_POINT('Ctrl Pts',(52.9364447521332,-38.0597348185281,
-55.3342330819689));
#188290=CARTESIAN_POINT('Ctrl Pts',(53.4093468596021,-38.0856478194539,
-55.3542488214713));
#188291=CARTESIAN_POINT('Ctrl Pts',(52.9283556128915,-38.1521941031454,
-54.8226237570584));
#188292=CARTESIAN_POINT('Ctrl Pts',(52.9572784319432,-37.9516014512281,
-55.2598937783695));
#188293=CARTESIAN_POINT('Ctrl Pts',(53.4247544927353,-37.9975926380036,
-55.2862331725394));
#188294=CARTESIAN_POINT('Ctrl Pts',(52.9626456126999,-37.9110442829472,
-54.7499500131212));
#188295=CARTESIAN_POINT('Ctrl Pts',(52.9868771633111,-37.8051184700684,
-55.2259980552998));
#188296=CARTESIAN_POINT('Ctrl Pts',(53.4555105552472,-37.889347597856,-55.24995));
#188297=CARTESIAN_POINT('Ctrl Pts',(53.0181298732915,-37.6685004154142,
-54.74995));
#188298=CARTESIAN_POINT('Ctrl Pts',(53.0181298732915,-37.6685004154141,
-55.2499499999999));
#188299=CARTESIAN_POINT('Ctrl Pts',(53.5055391860638,-37.78000002,-55.24995));
#188300=CARTESIAN_POINT('Ctrl Pts',(52.9112495105562,-38.347717747534,-54.9585476429427));
#188301=CARTESIAN_POINT('Ctrl Pts',(52.9138167203455,-38.3183744053704,
-54.9381487773268));
#188302=CARTESIAN_POINT('Ctrl Pts',(52.9167587015664,-38.288135817498,-54.9192611255627));
#188303=CARTESIAN_POINT('Ctrl Pts',(52.920093649339,-38.2570537209009,-54.901824465559));
#188304=CARTESIAN_POINT('Ctrl Pts',(52.9223677590233,-38.2358587572315,
-54.8899343611017));
#188305=CARTESIAN_POINT('Ctrl Pts',(52.9248248159382,-38.2142707844826,
-54.8787197886081));
#188306=CARTESIAN_POINT('Ctrl Pts',(52.9274736531865,-38.1922987278826,
-54.8681728665638));
#188307=CARTESIAN_POINT('Ctrl Pts',(52.9299589939906,-38.1716828713013,
-54.8582769411983));
#188308=CARTESIAN_POINT('Ctrl Pts',(52.9326383429721,-38.1505275158821,
-54.8488776493919));
#188309=CARTESIAN_POINT('Ctrl Pts',(52.9354970235834,-38.1290543071062,
-54.8400916455875));
#188310=CARTESIAN_POINT('Ctrl Pts',(52.9379577126515,-38.1105706437396,
-54.832528847761));
#188311=CARTESIAN_POINT('Ctrl Pts',(52.9405510514482,-38.0918525526911,
-54.8254200347525));
#188312=CARTESIAN_POINT('Ctrl Pts',(52.9432599418087,-38.0730559676527,
-54.8188132901669));
#188313=CARTESIAN_POINT('Ctrl Pts',(52.9456302208742,-38.0566089557442,
-54.8130323886545));
#188314=CARTESIAN_POINT('Ctrl Pts',(52.9480888658684,-38.0401021278493,
-54.8076355026166));
#188315=CARTESIAN_POINT('Ctrl Pts',(52.9506198739619,-38.0236452379292,
-54.8026387626986));
#188316=CARTESIAN_POINT('Ctrl Pts',(52.9513690438644,-38.0187740537363,
-54.8011597444501));
#188317=CARTESIAN_POINT('Ctrl Pts',(52.9521257433548,-38.0138993081238,
-54.7997132372211));
#188318=CARTESIAN_POINT('Ctrl Pts',(52.952890638887,-38.0090171068857,-54.7982978559824));
#188319=CARTESIAN_POINT('Ctrl Pts',(52.9583778797083,-37.9739929594029,
-54.7881441325221));
#188320=CARTESIAN_POINT('Ctrl Pts',(52.964275682584,-37.9386530390232,-54.7796085808392));
#188321=CARTESIAN_POINT('Ctrl Pts',(52.9706104876299,-37.9030233239771,
-54.7726555501025));
#188322=CARTESIAN_POINT('Ctrl Pts',(52.976957882613,-37.8673227976168,-54.7656887007527));
#188323=CARTESIAN_POINT('Ctrl Pts',(52.9837439516238,-37.8313305401564,
-54.7603105161544));
#188324=CARTESIAN_POINT('Ctrl Pts',(52.9910089773631,-37.7950582648799,
-54.75653337115));
#188325=CARTESIAN_POINT('Ctrl Pts',(52.9981747631865,-37.7592814672075,
-54.7528078217717));
#188326=CARTESIAN_POINT('Ctrl Pts',(53.0058064655273,-37.7232314999343,
-54.750639790985));
#188327=CARTESIAN_POINT('Ctrl Pts',(53.0139568096317,-37.6869169823467,
-54.7500895663837));
#188328=CARTESIAN_POINT('Ctrl Pts',(53.0153329135287,-37.6807856400957,
-54.7499966664756));
#188329=CARTESIAN_POINT('Ctrl Pts',(53.0167238361879,-37.6746467652684,
-54.7499500003325));
#188330=CARTESIAN_POINT('Ctrl Pts',(53.0181298732915,-37.6685004154142,
-54.74995));
#188331=CARTESIAN_POINT('Origin',(3.,45.8435334367418,-55.24995));
#188332=CARTESIAN_POINT('',(2.97452770112504,45.3441826962898,-56.3263223051814));
#188333=CARTESIAN_POINT('',(2.97452770112504,45.3441826962898,-55.24995));
#188334=CARTESIAN_POINT('Origin',(3.,45.8435334367418,-56.3263223051791));
#188335=CARTESIAN_POINT('Ctrl Pts',(3.5,45.8435334367382,-56.3263223051844));
#188336=CARTESIAN_POINT('Ctrl Pts',(3.49999999999616,45.3173779148746,-56.3263223051846));
#188337=CARTESIAN_POINT('Ctrl Pts',(2.97452770112504,45.3441826962898,-56.3263223051814));
#188338=CARTESIAN_POINT('Ctrl Pts',(3.50000000000048,45.8043701107064,-56.199422183327));
#188339=CARTESIAN_POINT('Ctrl Pts',(3.46044927957146,45.3193954300817,-56.2062114458595));
#188340=CARTESIAN_POINT('Ctrl Pts',(2.97452768320356,45.344182697204,-56.1669325210571));
#188341=CARTESIAN_POINT('Ctrl Pts',(3.50768789429957,45.7667515939358,-56.0829442465191));
#188342=CARTESIAN_POINT('Ctrl Pts',(3.43677818882601,45.3204789931111,-56.08184534982));
#188343=CARTESIAN_POINT('Ctrl Pts',(2.98977292660286,45.3434149603554,-56.0100642332945));
#188344=CARTESIAN_POINT('Ctrl Pts',(3.54526290572092,45.6961797895947,-55.8659417020081));
#188345=CARTESIAN_POINT('Ctrl Pts',(3.43477708310906,45.3200587327755,-55.8400245162723));
#188346=CARTESIAN_POINT('Ctrl Pts',(3.06428488995232,45.339546776353,-55.7037165501142));
#188347=CARTESIAN_POINT('Ctrl Pts',(3.57574585639141,45.6630233017381,-55.7649226433931));
#188348=CARTESIAN_POINT('Ctrl Pts',(3.45484122335623,45.3186462559097,-55.719311149436));
#188349=CARTESIAN_POINT('Ctrl Pts',(3.12473312373466,45.3363910645469,-55.5532476192867));
#188350=CARTESIAN_POINT('Ctrl Pts',(3.64122647661092,45.619502323306,-55.6349498078453));
#188351=CARTESIAN_POINT('Ctrl Pts',(3.52210194558877,45.3142897117584,-55.5588309593355));
#188352=CARTESIAN_POINT('Ctrl Pts',(3.2545824170552,45.329238556454,-55.3542910788838));
#188353=CARTESIAN_POINT('Ctrl Pts',(3.66673217579536,45.6057722112868,-55.5945395207919));
#188354=CARTESIAN_POINT('Ctrl Pts',(3.55052601940426,45.3124719950673,-55.508240833463));
#188355=CARTESIAN_POINT('Ctrl Pts',(3.30516068386241,45.3264035474275,-55.2914116693877));
#188356=CARTESIAN_POINT('Ctrl Pts',(3.72301031701685,45.5810344345382,-55.523890140111));
#188357=CARTESIAN_POINT('Ctrl Pts',(3.61713920495136,45.3082025597939,-55.418990846134));
#188358=CARTESIAN_POINT('Ctrl Pts',(3.4167612791713,45.3199688102369,-55.1805611737224));
#188359=CARTESIAN_POINT('Ctrl Pts',(3.75395740734289,45.5698505794225,-55.4931090773944));
#188360=CARTESIAN_POINT('Ctrl Pts',(3.65544514044212,45.3057432608012,-55.3793555355223));
#188361=CARTESIAN_POINT('Ctrl Pts',(3.47812992567118,45.3163517222977,-55.1317622002044));
#188362=CARTESIAN_POINT('Ctrl Pts',(3.85643479923312,45.5394893320724,-55.41516737719));
#188363=CARTESIAN_POINT('Ctrl Pts',(3.78526119814061,45.2973112081201,-55.2791383019779));
#188364=CARTESIAN_POINT('Ctrl Pts',(3.68134449873891,45.3039876967517,-55.0081141730616));
#188365=CARTESIAN_POINT('Ctrl Pts',(3.93416970441317,45.5245403614249,-55.3854368917647));
#188366=CARTESIAN_POINT('Ctrl Pts',(3.88948584507308,45.2904098439472,-55.2390222324484));
#188367=CARTESIAN_POINT('Ctrl Pts',(3.83550338599137,45.2941065762735,-54.961052531036));
#188368=CARTESIAN_POINT('Ctrl Pts',(4.01487932239363,45.5159631499936,-55.3828830175977));
#188369=CARTESIAN_POINT('Ctrl Pts',(3.99772850678843,45.282979186916,-55.2358129028005));
#188370=CARTESIAN_POINT('Ctrl Pts',(3.99554290592259,45.2831291022416,-54.9597685279837));
#188371=CARTESIAN_POINT('',(3.99554290592262,45.2831291022416,-54.9597685279837));
#188372=CARTESIAN_POINT('Ctrl Pts',(3.99554290592259,45.2831291022416,-54.9597685279837));
#188373=CARTESIAN_POINT('Ctrl Pts',(3.94364694050733,45.286688764336,-54.9601848912546));
#188374=CARTESIAN_POINT('Ctrl Pts',(3.89225569970065,45.2901408601658,-54.9654203274222));
#188375=CARTESIAN_POINT('Ctrl Pts',(3.84188163699711,45.2934612214904,-54.975154634361));
#188376=CARTESIAN_POINT('Ctrl Pts',(3.78940342464469,45.2969202759588,-54.9852955481412));
#188377=CARTESIAN_POINT('Ctrl Pts',(3.73803006365291,45.3002363143349,-55.000318715847));
#188378=CARTESIAN_POINT('Ctrl Pts',(3.68833368154415,45.3033833815734,-55.0198046066567));
#188379=CARTESIAN_POINT('Ctrl Pts',(3.63901329264086,45.3065066387104,-55.039143070989));
#188380=CARTESIAN_POINT('Ctrl Pts',(3.59134547691614,45.3094634363256,-55.0628761864957));
#188381=CARTESIAN_POINT('Ctrl Pts',(3.54586890420049,45.3122303325377,-55.0905475013328));
#188382=CARTESIAN_POINT('Ctrl Pts',(3.54528805073115,45.3122656729596,-55.0909009356016));
#188383=CARTESIAN_POINT('Ctrl Pts',(3.5447076792751,45.3123009754724,-55.0912549191843));
#188384=CARTESIAN_POINT('Ctrl Pts',(3.54412778939157,45.3123362401396,-55.0916094513196));
#188385=CARTESIAN_POINT('Ctrl Pts',(3.47701183225151,45.3164177424284,-55.1326426961998));
#188386=CARTESIAN_POINT('Ctrl Pts',(3.41622114944533,45.3199999518618,-55.181103831794));
#188387=CARTESIAN_POINT('Ctrl Pts',(3.36096258887421,45.3231860861595,-55.2359880590722));
#188388=CARTESIAN_POINT('Ctrl Pts',(3.36038241673501,45.3232195381049,-55.2365643010014));
#188389=CARTESIAN_POINT('Ctrl Pts',(3.35980281684021,45.3232529482704,-55.2371413403593));
#188390=CARTESIAN_POINT('Ctrl Pts',(3.35922379149642,45.3232863165813,-55.2377191725326));
#188391=CARTESIAN_POINT('Ctrl Pts',(3.30734351853634,45.3262760943051,-55.2894925382371));
#188392=CARTESIAN_POINT('Ctrl Pts',(3.26003938774549,45.328931962174,-55.3476821319182));
#188393=CARTESIAN_POINT('Ctrl Pts',(3.21898968010886,45.3311986016838,-55.4089811023496));
#188394=CARTESIAN_POINT('Ctrl Pts',(3.21640175023779,45.331341499269,-55.4128456228488));
#188395=CARTESIAN_POINT('Ctrl Pts',(3.21383866111205,45.3314828508092,-55.4167225044094));
#188396=CARTESIAN_POINT('Ctrl Pts',(3.21130082579067,45.3316226428383,-55.4206109203385));
#188397=CARTESIAN_POINT('Ctrl Pts',(3.21085284159181,45.3316473192307,-55.4212973119574));
#188398=CARTESIAN_POINT('Ctrl Pts',(3.21040556228037,45.3316719521366,-55.4219841720788));
#188399=CARTESIAN_POINT('Ctrl Pts',(3.20995898742772,45.3316965416118,-55.4226714985032));
#188400=CARTESIAN_POINT('Ctrl Pts',(3.1542985362487,45.3347613386447,-55.5083388813912));
#188401=CARTESIAN_POINT('Ctrl Pts',(3.10954127961328,45.337153729465,-55.6013158854463));
#188402=CARTESIAN_POINT('Ctrl Pts',(3.07484642277082,45.338981720226,-55.6975623037683));
#188403=CARTESIAN_POINT('Ctrl Pts',(3.05597305038916,45.3399761140204,-55.7499186083825));
#188404=CARTESIAN_POINT('Ctrl Pts',(3.04007792774143,45.34080344662,-55.8032432879277));
#188405=CARTESIAN_POINT('Ctrl Pts',(3.0270298121595,45.3414808214313,-55.8568906140328));
#188406=CARTESIAN_POINT('Ctrl Pts',(3.0269130014781,45.3414868854957,-55.8573708811394));
#188407=CARTESIAN_POINT('Ctrl Pts',(3.0267964073689,45.3414929380841,-55.8578511838465));
#188408=CARTESIAN_POINT('Ctrl Pts',(3.02668002962044,45.3414989792089,-55.8583315221214));
#188409=CARTESIAN_POINT('Ctrl Pts',(2.99362945634284,45.343214621947,-55.9947446729407));
#188410=CARTESIAN_POINT('Ctrl Pts',(2.97802127132288,45.3440061056745,-56.1340253984927));
#188411=CARTESIAN_POINT('Ctrl Pts',(2.9750567785663,45.3441559820078,-56.275384513425));
#188412=CARTESIAN_POINT('Ctrl Pts',(2.97470131764747,45.3441739531022,-56.2923343409352));
#188413=CARTESIAN_POINT('Ctrl Pts',(2.97452770112514,45.3441826962898,-56.3093140568108));
#188414=CARTESIAN_POINT('Ctrl Pts',(2.97452770112504,45.3441826962898,-56.3263223051814));
#188415=CARTESIAN_POINT('Origin',(4.02975864478749,45.7819570116602,-54.9597685279843));
#188416=CARTESIAN_POINT('Ctrl Pts',(4.49412912371062,45.2467848220336,-54.955514051414));
#188417=CARTESIAN_POINT('Ctrl Pts',(4.49662538953713,45.2465921108978,-55.2355242600995));
#188418=CARTESIAN_POINT('Ctrl Pts',(4.51630724703493,45.4845441383302,-55.3818234144886));
#188419=CARTESIAN_POINT('Ctrl Pts',(4.32798628668273,45.2596110100493,-54.9570167865889));
#188420=CARTESIAN_POINT('Ctrl Pts',(4.33057507588361,45.2594183143523,-55.2356268020846));
#188421=CARTESIAN_POINT('Ctrl Pts',(4.34919298261046,45.4956321595243,-55.3822130600194));
#188422=CARTESIAN_POINT('Ctrl Pts',(4.16179087919831,45.271725776299,-54.9584347299645));
#188423=CARTESIAN_POINT('Ctrl Pts',(4.16425328466829,45.2715506006274,-55.2357229472724));
#188424=CARTESIAN_POINT('Ctrl Pts',(4.18205130859575,45.5061051687682,-55.3825645302384));
#188425=CARTESIAN_POINT('Ctrl Pts',(3.9955429059226,45.2831291022416,-54.9597685279837));
#188426=CARTESIAN_POINT('Ctrl Pts',(3.99772850678838,45.2829791869159,-55.2358129028006));
#188427=CARTESIAN_POINT('Ctrl Pts',(4.01487932239355,45.5159631499936,-55.3828830175977));
#188428=CARTESIAN_POINT('',(4.49412912371054,45.2467848220337,-54.955514051414));
#188429=CARTESIAN_POINT('Origin',(0.000537877572094891,-12.1619648097437,
-48.139312741498));
#188430=CARTESIAN_POINT('Origin',(4.53261449406992,45.7453014980519,-54.955514051414));
#188431=CARTESIAN_POINT('Ctrl Pts',(4.47139039164512,45.4906548448225,-55.3863604038316));
#188432=CARTESIAN_POINT('Ctrl Pts',(4.43672341851431,45.2509948349534,-55.2414357815079));
#188433=CARTESIAN_POINT('Ctrl Pts',(4.40504871546121,45.2535845867532,-54.9609750843566));
#188434=CARTESIAN_POINT('Ctrl Pts',(4.55693219186144,45.4776416184101,-55.3719745613438));
#188435=CARTESIAN_POINT('Ctrl Pts',(4.55013513142212,45.2423482358409,-55.2221823835831));
#188436=CARTESIAN_POINT('Ctrl Pts',(4.57467261000343,45.2407903510215,-54.9401638606375));
#188437=CARTESIAN_POINT('Ctrl Pts',(4.64632152753948,45.4720450292502,-55.3906024673539));
#188438=CARTESIAN_POINT('Ctrl Pts',(4.67148999584471,45.2327453727894,-55.2479506024289));
#188439=CARTESIAN_POINT('Ctrl Pts',(4.75204967627739,45.2264957449184,-54.9756360521502));
#188440=CARTESIAN_POINT('Ctrl Pts',(4.78526231654569,45.4785391935409,-55.4758941943565));
#188441=CARTESIAN_POINT('Ctrl Pts',(4.85155529671713,45.2181899234016,-55.3600111127249));
#188442=CARTESIAN_POINT('Ctrl Pts',(5.02768780679811,45.2032674062285,-55.1236362709704));
#188443=CARTESIAN_POINT('Ctrl Pts',(4.83987531604392,45.4877168692796,-55.5336384447089));
#188444=CARTESIAN_POINT('Ctrl Pts',(4.91960725641842,45.2125663061104,-55.4362681462788));
#188445=CARTESIAN_POINT('Ctrl Pts',(5.13603339661033,45.193728067178,-55.2216356337625));
#188446=CARTESIAN_POINT('Ctrl Pts',(4.92459268013903,45.5188916935313,-55.6761597789111));
#188447=CARTESIAN_POINT('Ctrl Pts',(5.01304731809969,45.2048811773774,-55.6156547787452));
#188448=CARTESIAN_POINT('Ctrl Pts',(5.30411094495532,45.178640871319,-55.4541550621106));
#188449=CARTESIAN_POINT('Ctrl Pts',(4.95452456181636,45.5407314582523,-55.7600334675643));
#188450=CARTESIAN_POINT('Ctrl Pts',(5.03798355387793,45.2028686588532,-55.7195028114066));
#188451=CARTESIAN_POINT('Ctrl Pts',(5.3635004865346,45.1731436419375,-55.5870891782066));
#188452=CARTESIAN_POINT('Ctrl Pts',(4.99613220506374,45.6005437839053,-55.9629949137757));
#188453=CARTESIAN_POINT('Ctrl Pts',(5.04892271004841,45.2022954662183,-55.9561269088791));
#188454=CARTESIAN_POINT('Ctrl Pts',(5.44607043400786,45.165473055749,-55.8925951196528));
#188455=CARTESIAN_POINT('Ctrl Pts',(5.00281283901272,45.6402645497958,-56.0837699876345));
#188456=CARTESIAN_POINT('Ctrl Pts',(5.02368213791864,45.2047138612132,-56.0903086587098));
#188457=CARTESIAN_POINT('Ctrl Pts',(5.45934494047938,45.1642043041266,-56.0648075138964));
#188458=CARTESIAN_POINT('Ctrl Pts',(4.99898645253333,45.6858523253613,-56.217596972311));
#188459=CARTESIAN_POINT('Ctrl Pts',(4.97691572104403,45.208981116778,-56.2185887282702));
#188460=CARTESIAN_POINT('Ctrl Pts',(5.45177805579375,45.1649222445519,-56.2401344498715));
#188461=CARTESIAN_POINT('',(5.4533007853959,45.1647773033082,-56.1488993661993));
#188462=CARTESIAN_POINT('Ctrl Pts',(5.4533007853959,45.1647773033082,-56.1488993661993));
#188463=CARTESIAN_POINT('Ctrl Pts',(5.4533007853959,45.1647773033082,-56.0055674620926));
#188464=CARTESIAN_POINT('Ctrl Pts',(5.43788134491899,45.1662336319389,-55.8645506073504));
#188465=CARTESIAN_POINT('Ctrl Pts',(5.3637535993023,45.1731199385278,-55.5890146236025));
#188466=CARTESIAN_POINT('Ctrl Pts',(5.30482297007121,45.1785752810591,-55.4563513172782));
#188467=CARTESIAN_POINT('Ctrl Pts',(5.13740816361988,45.1936060305266,-55.2236271337424));
#188468=CARTESIAN_POINT('Ctrl Pts',(5.02927744515326,45.2031302456007,-55.1252272506259));
#188469=CARTESIAN_POINT('Ctrl Pts',(4.8419870330226,45.2189180089433,-55.0241597383142));
#188470=CARTESIAN_POINT('Ctrl Pts',(4.77441476074195,45.2245089469405,-54.9977644123794));
#188471=CARTESIAN_POINT('Ctrl Pts',(4.63647895825164,45.2356614644569,-54.9633053694043));
#188472=CARTESIAN_POINT('Ctrl Pts',(4.56605684297844,45.2412320189915,-54.9548634767888));
#188473=CARTESIAN_POINT('Ctrl Pts',(4.49412912371054,45.2467848220337,-54.955514051414));
#188474=CARTESIAN_POINT('Origin',(5.5,45.6625917098448,-56.1488993661993));
#188475=CARTESIAN_POINT('Origin',(5.5,45.6625917098448,-55.24995));
#188476=CARTESIAN_POINT('',(5.4533007853959,45.1647773033082,-55.24995));
#188477=CARTESIAN_POINT('Origin',(0.,-12.9675000200281,-60.42825533736));
#188478=CARTESIAN_POINT('Origin',(0.,-12.9675000200281,-60.42825533736));
#188479=CARTESIAN_POINT('Origin',(11.5,44.7861808691872,-55.24995));
#188480=CARTESIAN_POINT('',(11.402356187646,44.2958078622741,-55.9012688372262));
#188481=CARTESIAN_POINT('',(11.402356187646,44.2958078622741,-55.24995));
#188482=CARTESIAN_POINT('Origin',(11.5,44.7861808691872,-55.9012688372262));
#188483=CARTESIAN_POINT('Ctrl Pts',(12.0063585556897,44.8133988368639,-55.994729193492));
#188484=CARTESIAN_POINT('Ctrl Pts',(12.0432961608807,44.166306685066,-55.9714168634058));
#188485=CARTESIAN_POINT('Ctrl Pts',(11.4137787144181,44.2935713409156,-56.0670761670352));
#188486=CARTESIAN_POINT('Ctrl Pts',(11.9806229374089,44.7620399676921,-55.807622827858));
#188487=CARTESIAN_POINT('Ctrl Pts',(11.9479581346228,44.1860579521207,-55.8533126924881));
#188488=CARTESIAN_POINT('Ctrl Pts',(11.3625533696003,44.3036045439701,-55.7375862930343));
#188489=CARTESIAN_POINT('Ctrl Pts',(12.0342088179099,44.7020611377846,-55.618213877133));
#188490=CARTESIAN_POINT('Ctrl Pts',(11.9394256397489,44.1869658481102,-55.6416294054125));
#188491=CARTESIAN_POINT('Ctrl Pts',(11.4688213961376,44.2829757401497,-55.3880964587751));
#188492=CARTESIAN_POINT('Ctrl Pts',(12.2561025511723,44.5772902436325,-55.3546719045028));
#188493=CARTESIAN_POINT('Ctrl Pts',(12.1283065348885,44.1458422480371,-55.3228555036694));
#188494=CARTESIAN_POINT('Ctrl Pts',(11.9092544880125,44.1929801108985,-54.9017249097375));
#188495=CARTESIAN_POINT('Ctrl Pts',(12.4220919977125,44.5119954318218,-55.2820851549404));
#188496=CARTESIAN_POINT('Ctrl Pts',(12.3105489858414,44.1068007671422,-55.2078316060723));
#188497=CARTESIAN_POINT('Ctrl Pts',(12.2388210327084,44.124039351436,-54.76829873255));
#188498=CARTESIAN_POINT('Ctrl Pts',(12.5881212157209,44.4526104250917,-55.3021722916518));
#188499=CARTESIAN_POINT('Ctrl Pts',(12.5143053198889,44.0622780980818,-55.2189585580228));
#188500=CARTESIAN_POINT('Ctrl Pts',(12.5685011226759,44.0511648497893,-54.8168105684966));
#188501=CARTESIAN_POINT('',(12.4042000461459,44.0871753139748,-54.8084491013776));
#188502=CARTESIAN_POINT('Ctrl Pts',(12.4042000461459,44.0871753139748,-54.8084491013776));
#188503=CARTESIAN_POINT('Ctrl Pts',(12.3367608750176,44.101837196892,-54.8105480223147));
#188504=CARTESIAN_POINT('Ctrl Pts',(12.2704278259804,44.1161334117608,-54.8196434921937));
#188505=CARTESIAN_POINT('Ctrl Pts',(12.139979885891,44.1440180229867,-54.8518275298353));
#188506=CARTESIAN_POINT('Ctrl Pts',(12.0748636121213,44.1578169517408,-54.8753942762821));
#188507=CARTESIAN_POINT('Ctrl Pts',(11.8888586925018,44.1969229345987,-54.9642150903431));
#188508=CARTESIAN_POINT('Ctrl Pts',(11.7804034422216,44.2193085174476,-55.0453048135951));
#188509=CARTESIAN_POINT('Ctrl Pts',(11.5963788422947,44.2569088778311,-55.249379574632));
#188510=CARTESIAN_POINT('Ctrl Pts',(11.5252471488681,44.2712224279124,-55.366778251881));
#188511=CARTESIAN_POINT('Ctrl Pts',(11.4269419773585,44.2909287600296,-55.6267443723887));
#188512=CARTESIAN_POINT('Ctrl Pts',(11.402356187646,44.2958078622742,-55.7615802140858));
#188513=CARTESIAN_POINT('Ctrl Pts',(11.402356187646,44.2958078622741,-55.9012688372262));
#188514=CARTESIAN_POINT('Origin',(12.5104231251106,44.5757617009068,-54.8084491013774));
#188515=CARTESIAN_POINT('Ctrl Pts',(12.8921600942007,43.978899026433,-54.7926966592038));
#188516=CARTESIAN_POINT('Ctrl Pts',(12.9056883239205,43.9758363551094,-55.2210744412794));
#188517=CARTESIAN_POINT('Ctrl Pts',(13.0012809038513,44.3884784473357,-55.2865609247418));
#188518=CARTESIAN_POINT('Ctrl Pts',(12.7296669706488,44.015686029617,-54.798137418056));
#188519=CARTESIAN_POINT('Ctrl Pts',(12.743502264335,44.012594228669,-55.2216770608656));
#188520=CARTESIAN_POINT('Ctrl Pts',(12.8359967737338,44.4202801831072,-55.2911600797832));
#188521=CARTESIAN_POINT('Ctrl Pts',(12.5670134373343,44.0517782170206,-54.8033818322122));
#188522=CARTESIAN_POINT('Ctrl Pts',(12.5803648873612,44.0488388411796,-55.2222478741758));
#188523=CARTESIAN_POINT('Ctrl Pts',(12.6706421628547,44.4514812651211,-55.2954855956284));
#188524=CARTESIAN_POINT('Ctrl Pts',(12.4042000461459,44.0871753139748,-54.8084491013774));
#188525=CARTESIAN_POINT('Ctrl Pts',(12.4164090892806,44.0845209580867,-55.2227904669344));
#188526=CARTESIAN_POINT('Ctrl Pts',(12.5052115625551,44.4820814550629,-55.2995670619066));
#188527=CARTESIAN_POINT('',(12.8921600942007,43.978899026433,-54.7926966592038));
#188528=CARTESIAN_POINT('Origin',(0.36005249046184,-9.26137067386744,-40.4793207392961));
#188529=CARTESIAN_POINT('Origin',(13.0025618077027,44.4665581918916,-54.7926966592038));
#188530=CARTESIAN_POINT('Ctrl Pts',(13.0012809038513,44.3884784473357,-55.2865609247418));
#188531=CARTESIAN_POINT('Ctrl Pts',(12.9056883239205,43.9758363551094,-55.2210744412793));
#188532=CARTESIAN_POINT('Ctrl Pts',(12.8921600942007,43.978899026433,-54.7926966592038));
#188533=CARTESIAN_POINT('Ctrl Pts',(13.0654243459864,44.3636027691474,-55.2827944545873));
#188534=CARTESIAN_POINT('Ctrl Pts',(12.9784387965694,43.9593348061506,-55.2098637836594));
#188535=CARTESIAN_POINT('Ctrl Pts',(13.0193597758081,43.9501021457404,-54.7884376491597));
#188536=CARTESIAN_POINT('Ctrl Pts',(13.1299983077116,44.3395152672781,-55.2921354075477));
#188537=CARTESIAN_POINT('Ctrl Pts',(13.0552570243808,43.9418365181403,-55.2141810151918));
#188538=CARTESIAN_POINT('Ctrl Pts',(13.1474090807614,43.9206427834081,-54.8097712354121));
#188539=CARTESIAN_POINT('Ctrl Pts',(13.2502943581078,44.2958064353142,-55.3361304655099));
#188540=CARTESIAN_POINT('Ctrl Pts',(13.2011715416027,43.9084021006501,-55.25643129776));
#188541=CARTESIAN_POINT('Ctrl Pts',(13.3859583749986,43.8649843137035,-54.9019989045167));
#188542=CARTESIAN_POINT('Ctrl Pts',(13.3058135696287,44.2762488685004,-55.3707576859229));
#188543=CARTESIAN_POINT('Ctrl Pts',(13.2704159548698,43.8924342454859,-55.2940831522118));
#188544=CARTESIAN_POINT('Ctrl Pts',(13.496053992198,43.8388872267122,-54.9728361666051));
#188545=CARTESIAN_POINT('Ctrl Pts',(13.3986038888631,44.2453125071312,-55.4597899571993));
#188546=CARTESIAN_POINT('Ctrl Pts',(13.3860573147077,43.8656515577332,-55.3967868701307));
#188547=CARTESIAN_POINT('Ctrl Pts',(13.6800589131788,43.7948562869374,-55.1530004401584));
#188548=CARTESIAN_POINT('Ctrl Pts',(13.4362889542451,44.2338103823362,-55.514828855807));
#188549=CARTESIAN_POINT('Ctrl Pts',(13.4334072964209,43.8546223828157,-55.46277372953));
#188550=CARTESIAN_POINT('Ctrl Pts',(13.7547890917519,43.7767382792428,-55.2636104102621));
#188551=CARTESIAN_POINT('Ctrl Pts',(13.4867061057231,44.2229131048268,-55.6353022097904));
#188552=CARTESIAN_POINT('Ctrl Pts',(13.4931806941864,43.8407149886408,-55.6082533108594));
#188553=CARTESIAN_POINT('Ctrl Pts',(13.8547672339164,43.7524103115038,-55.5042410247415));
#188554=CARTESIAN_POINT('Ctrl Pts',(13.5,44.2234307110673,-55.7021231738994));
#188555=CARTESIAN_POINT('Ctrl Pts',(13.5063795391634,43.8376645208725,-55.6900657479952));
#188556=CARTESIAN_POINT('Ctrl Pts',(13.8811292609786,43.7459411266109,-55.6370500544614));
#188557=CARTESIAN_POINT('Ctrl Pts',(13.5,44.2316053598055,-55.7692503840715));
#188558=CARTESIAN_POINT('Ctrl Pts',(13.5,43.83922597116,-55.7692503840715));
#188559=CARTESIAN_POINT('Ctrl Pts',(13.8811292719168,43.7459411239336,-55.7692503840715));
#188560=CARTESIAN_POINT('',(13.8811292719168,43.7459411239337,-55.7692503840715));
#188561=CARTESIAN_POINT('Ctrl Pts',(13.8811292719168,43.7459411239336,-55.7692503840715));
#188562=CARTESIAN_POINT('Ctrl Pts',(13.8811292682097,43.745941124841,-55.7244458157436));
#188563=CARTESIAN_POINT('Ctrl Pts',(13.878105549578,43.7466831296689,-55.679736138466));
#188564=CARTESIAN_POINT('Ctrl Pts',(13.8722047277525,43.7481272051964,-55.6355346293339));
#188565=CARTESIAN_POINT('Ctrl Pts',(13.8662038608382,43.7495957642058,-55.590583708673));
#188566=CARTESIAN_POINT('Ctrl Pts',(13.8572273197945,43.7517904587082,-55.5461569097345));
#188567=CARTESIAN_POINT('Ctrl Pts',(13.8453776205413,43.7546819864356,-55.5026858819466));
#188568=CARTESIAN_POINT('Ctrl Pts',(13.8344632356934,43.7573452815743,-55.462646087107));
#188569=CARTESIAN_POINT('Ctrl Pts',(13.8211106222446,43.7605999346755,-55.4234162320198));
#188570=CARTESIAN_POINT('Ctrl Pts',(13.8053642538662,43.7644316776827,-55.3853473456883));
#188571=CARTESIAN_POINT('Ctrl Pts',(13.8051683359555,43.7644793526174,-55.3848736887475));
#188572=CARTESIAN_POINT('Ctrl Pts',(13.8049720511568,43.7645271159922,-55.3844002212373));
#188573=CARTESIAN_POINT('Ctrl Pts',(13.8047753996222,43.7645749677634,-55.3839269439647));
#188574=CARTESIAN_POINT('Ctrl Pts',(13.7718577708332,43.7725849069898,-55.3047047522695));
#188575=CARTESIAN_POINT('Ctrl Pts',(13.728178051487,43.7831849346504,-55.2296008411665));
#188576=CARTESIAN_POINT('Ctrl Pts',(13.6758172364472,43.7957998172932,-55.1617614773765));
#188577=CARTESIAN_POINT('Ctrl Pts',(13.6492141753589,43.8022090852412,-55.127294199934));
#188578=CARTESIAN_POINT('Ctrl Pts',(13.6203708268795,43.8091382966098,-55.0947027771945));
#188579=CARTESIAN_POINT('Ctrl Pts',(13.5895638615798,43.8165110245856,-55.0644031256242));
#188580=CARTESIAN_POINT('Ctrl Pts',(13.5890610147607,43.8166313659687,-55.0639085594356));
#188581=CARTESIAN_POINT('Ctrl Pts',(13.5885576424949,43.8167518260625,-55.0634146006456));
#188582=CARTESIAN_POINT('Ctrl Pts',(13.5880537459902,43.8168724045334,-55.0629212511039));
#188583=CARTESIAN_POINT('Ctrl Pts',(13.5330913533177,43.8300244728729,-55.0091092659332));
#188584=CARTESIAN_POINT('Ctrl Pts',(13.4715943783219,43.8446517471115,-54.9620890033291));
#188585=CARTESIAN_POINT('Ctrl Pts',(13.4054646975447,43.8602521578852,-54.9231113264467));
#188586=CARTESIAN_POINT('Ctrl Pts',(13.3615129962558,43.8706206427509,-54.8972056334033));
#188587=CARTESIAN_POINT('Ctrl Pts',(13.3155161569027,43.8814186797025,-54.8748524249676));
#188588=CARTESIAN_POINT('Ctrl Pts',(13.2680436044718,43.8924962435662,-54.8564136580933));
#188589=CARTESIAN_POINT('Ctrl Pts',(13.2675902582944,43.8926020304046,-54.8562375743555));
#188590=CARTESIAN_POINT('Ctrl Pts',(13.267136793244,43.89270783907,-54.8560618534164));
#188591=CARTESIAN_POINT('Ctrl Pts',(13.2666832096553,43.8928136694707,-54.8558864954404));
#188592=CARTESIAN_POINT('Ctrl Pts',(13.2297963270863,43.9014201395016,-54.8416258184039));
#188593=CARTESIAN_POINT('Ctrl Pts',(13.1921658567097,43.9101602729064,-54.82976688078));
#188594=CARTESIAN_POINT('Ctrl Pts',(13.1539812007031,43.9189886853961,-54.8202850097806));
#188595=CARTESIAN_POINT('Ctrl Pts',(13.1156262419325,43.9278564724202,-54.8107608498357));
#188596=CARTESIAN_POINT('Ctrl Pts',(13.0767111408946,43.9368135671448,-54.8036348844097));
#188597=CARTESIAN_POINT('Ctrl Pts',(13.037416426663,43.9458157565233,-54.7989332461647));
#188598=CARTESIAN_POINT('Ctrl Pts',(12.9988139657374,43.9546593547151,-54.7943144364803));
#188599=CARTESIAN_POINT('Ctrl Pts',(12.9598441948041,43.9635466980804,-54.7920353122774));
#188600=CARTESIAN_POINT('Ctrl Pts',(12.9206817922385,43.9724341406896,-54.7921703301218));
#188601=CARTESIAN_POINT('Ctrl Pts',(12.9111849603394,43.9745893340114,-54.7922030717742));
#188602=CARTESIAN_POINT('Ctrl Pts',(12.9016768542622,43.976744516291,-54.7923780107907));
#188603=CARTESIAN_POINT('Ctrl Pts',(12.8921600942007,43.978899026433,-54.7926966592038));
#188604=CARTESIAN_POINT('Origin',(14.,44.2316053598044,-55.7692503840718));
#188605=CARTESIAN_POINT('Origin',(14.,44.2316053598056,-55.24995));
#188606=CARTESIAN_POINT('',(13.8811292719168,43.7459411239336,-55.24995));
#188607=CARTESIAN_POINT('Origin',(0.,-12.9675000200281,-60.42825533736));
#188608=CARTESIAN_POINT('Origin',(0.,-12.9675000200281,-60.42825533736));
#188609=CARTESIAN_POINT('Origin',(20.,42.4196614549321,-55.24995));
#188610=CARTESIAN_POINT('',(19.8301846741669,41.9493820112901,-55.74995));
#188611=CARTESIAN_POINT('Origin',(20.,42.4196614549321,-55.74995));
#188612=CARTESIAN_POINT('',(19.8301846741669,41.9493820112901,-55.24995));
#188613=CARTESIAN_POINT('Ctrl Pts',(20.5,42.4196614549321,-55.74995));
#188614=CARTESIAN_POINT('Ctrl Pts',(20.5,41.7075153736088,-55.7499499999999));
#188615=CARTESIAN_POINT('Ctrl Pts',(19.8301846741669,41.9493820112901,-55.74995));
#188616=CARTESIAN_POINT('Ctrl Pts',(20.5,42.4196614460347,-55.6824493590803));
#188617=CARTESIAN_POINT('Ctrl Pts',(20.4999999995541,41.7075153734334,-55.7174757167052));
#188618=CARTESIAN_POINT('Ctrl Pts',(19.8301846986023,41.9493820024666,-55.6149487156912));
#188619=CARTESIAN_POINT('Ctrl Pts',(20.514053798786,42.4095322277552,-55.614564639731));
#188620=CARTESIAN_POINT('Ctrl Pts',(20.4987004734351,41.7075927453749,-55.6840485748926));
#188621=CARTESIAN_POINT('Ctrl Pts',(19.8580536242861,41.939338788612,-55.4791792828035));
#188622=CARTESIAN_POINT('Ctrl Pts',(20.5667184545259,42.3713246265636,-55.4916091232479));
#188623=CARTESIAN_POINT('Ctrl Pts',(20.5049952302095,41.704035376344,-55.6029041515887));
#188624=CARTESIAN_POINT('Ctrl Pts',(19.9624885940201,41.9014556000366,-55.2332682431543));
#188625=CARTESIAN_POINT('Ctrl Pts',(20.6054777681041,42.3431217478432,-55.4359504896237));
#188626=CARTESIAN_POINT('Ctrl Pts',(20.5131880407467,41.7002281457635,-55.5554275272938));
#188627=CARTESIAN_POINT('Ctrl Pts',(20.0393490386551,41.8734921844523,-55.1219509819824));
#188628=CARTESIAN_POINT('Ctrl Pts',(20.6991000803093,42.274341317199,-55.3453480693239));
#188629=CARTESIAN_POINT('Ctrl Pts',(20.5562936263709,41.682844191329,-55.4545960701533));
#188630=CARTESIAN_POINT('Ctrl Pts',(20.2250038078484,41.8052957533979,-54.9407461359128));
#188631=CARTESIAN_POINT('Ctrl Pts',(20.7546446997872,42.233248744276,-55.3096493999238));
#188632=CARTESIAN_POINT('Ctrl Pts',(20.5906196334233,41.6694809696074,-55.401758477076));
#188633=CARTESIAN_POINT('Ctrl Pts',(20.3351498160899,41.7645520870248,-54.8693487992283));
#188634=CARTESIAN_POINT('Ctrl Pts',(20.8729715384853,42.1447441871192,-55.2621717596744));
#188635=CARTESIAN_POINT('Ctrl Pts',(20.6877494411454,41.6322368154735,-55.3113977742726));
#188636=CARTESIAN_POINT('Ctrl Pts',(20.569794123189,41.6767990021169,-54.774393519968));
#188637=CARTESIAN_POINT('Ctrl Pts',(20.936865425116,42.0964926027484,-55.24995));
#188638=CARTESIAN_POINT('Ctrl Pts',(20.7498635250281,41.608586604298,-55.2730231656551));
#188639=CARTESIAN_POINT('Ctrl Pts',(20.6965038706024,41.6289544421905,-54.7499500128377));
#188640=CARTESIAN_POINT('Ctrl Pts',(21.,42.0482945870964,-55.24995));
#188641=CARTESIAN_POINT('Ctrl Pts',(20.8216939078753,41.5811683327377,-55.2499499999999));
#188642=CARTESIAN_POINT('Ctrl Pts',(20.8216939078753,41.5811683327377,-54.74995));
#188643=CARTESIAN_POINT('',(20.8216939078753,41.5811683327377,-54.74995));
#188644=CARTESIAN_POINT('Ctrl Pts',(20.8216939078753,41.5811683327377,-54.74995));
#188645=CARTESIAN_POINT('Ctrl Pts',(20.7819408740053,41.5963424062421,-54.7499500040765));
#188646=CARTESIAN_POINT('Ctrl Pts',(20.7422583702479,41.6114370651536,-54.7524107511961));
#188647=CARTESIAN_POINT('Ctrl Pts',(20.7028910580564,41.6263644244518,-54.7572302478587));
#188648=CARTESIAN_POINT('Ctrl Pts',(20.6627696815177,41.6415777110541,-54.7621420599578));
#188649=CARTESIAN_POINT('Ctrl Pts',(20.6229744854673,41.6566176734327,-54.769503891898));
#188650=CARTESIAN_POINT('Ctrl Pts',(20.5837549178884,41.671393724625,-54.7792610196498));
#188651=CARTESIAN_POINT('Ctrl Pts',(20.5448758646516,41.686041486352,-54.7889334335166));
#188652=CARTESIAN_POINT('Ctrl Pts',(20.5065612917292,41.7004303395793,-54.8009599654576));
#188653=CARTESIAN_POINT('Ctrl Pts',(20.4690629498568,41.7144677618964,-54.8153366743303));
#188654=CARTESIAN_POINT('Ctrl Pts',(20.4635146440735,41.7165447580391,-54.8174638717742));
#188655=CARTESIAN_POINT('Ctrl Pts',(20.4579842421571,41.7186140458698,-54.8196426059304));
#188656=CARTESIAN_POINT('Ctrl Pts',(20.452472600707,41.7206753085659,-54.8218729523577));
#188657=CARTESIAN_POINT('Ctrl Pts',(20.4520370571492,41.7208381946492,-54.8220491998562));
#188658=CARTESIAN_POINT('Ctrl Pts',(20.4516016002718,41.7210010421259,-54.8222257818663));
#188659=CARTESIAN_POINT('Ctrl Pts',(20.451166230457,41.7211638508663,-54.8224026982642));
#188660=CARTESIAN_POINT('Ctrl Pts',(20.3795793872688,41.747934112313,-54.8514926489224));
#188661=CARTESIAN_POINT('Ctrl Pts',(20.3107136334647,41.7735197491871,-54.8894829736804));
#188662=CARTESIAN_POINT('Ctrl Pts',(20.2468906651867,41.7971168064876,-54.9352464330092));
#188663=CARTESIAN_POINT('Ctrl Pts',(20.2064337192117,41.8120748207908,-54.9642555789586));
#188664=CARTESIAN_POINT('Ctrl Pts',(20.1680024696355,41.8262340118394,-54.9963875370291));
#188665=CARTESIAN_POINT('Ctrl Pts',(20.1321785809257,41.8393931763607,-55.0313510893754));
#188666=CARTESIAN_POINT('Ctrl Pts',(20.1316789419887,41.8395767083895,-55.0318387291252));
#188667=CARTESIAN_POINT('Ctrl Pts',(20.1311797709301,41.8397600607401,-55.0323269633832));
#188668=CARTESIAN_POINT('Ctrl Pts',(20.1306810690887,41.839943232968,-55.0328157906737));
#188669=CARTESIAN_POINT('Ctrl Pts',(20.0684907293821,41.8627856252234,-55.093774729926));
#188670=CARTESIAN_POINT('Ctrl Pts',(20.0135863047548,41.8828310295748,-55.1639774211747));
#188671=CARTESIAN_POINT('Ctrl Pts',(19.9685212499206,41.8992323516663,-55.2406426510358));
#188672=CARTESIAN_POINT('Ctrl Pts',(19.9467038340058,41.9071727495408,-55.2777587094149));
#188673=CARTESIAN_POINT('Ctrl Pts',(19.9271921606274,41.9142591786556,-55.3163901520181));
#188674=CARTESIAN_POINT('Ctrl Pts',(19.9102738131902,41.9203962134609,-55.3562250735781));
#188675=CARTESIAN_POINT('Ctrl Pts',(19.9100688061412,41.9204705786079,-55.356707770824));
#188676=CARTESIAN_POINT('Ctrl Pts',(19.9098641753246,41.9205448062603,-55.3571906629275));
#188677=CARTESIAN_POINT('Ctrl Pts',(19.9096599209391,41.9206188963538,-55.3576737490625));
#188678=CARTESIAN_POINT('Ctrl Pts',(19.8950560556066,41.9259162207946,-55.3922136432421));
#188679=CARTESIAN_POINT('Ctrl Pts',(19.8824223932141,41.9304937150683,-55.4276284386807));
#188680=CARTESIAN_POINT('Ctrl Pts',(19.8717730238587,41.934349206398,-55.4637108040147));
#188681=CARTESIAN_POINT('Ctrl Pts',(19.8611060292098,41.9382110787783,-55.4998528876529));
#188682=CARTESIAN_POINT('Ctrl Pts',(19.8524296011668,41.9413486539406,-55.5366659074257));
#188683=CARTESIAN_POINT('Ctrl Pts',(19.8458033807233,41.9437431691666,-55.5739608322421));
#188684=CARTESIAN_POINT('Ctrl Pts',(19.8393763220395,41.9460657133694,-55.6101347978451));
#188685=CARTESIAN_POINT('Ctrl Pts',(19.8348780094478,41.9476892093276,-55.6467631869937));
#188686=CARTESIAN_POINT('Ctrl Pts',(19.832407933269,41.9485802658015,-55.6836754313746));
#188687=CARTESIAN_POINT('Ctrl Pts',(19.8309355210528,41.9491114244956,-55.7056788173516));
#188688=CARTESIAN_POINT('Ctrl Pts',(19.8301846781792,41.9493820098413,-55.727783032076));
#188689=CARTESIAN_POINT('Ctrl Pts',(19.8301846741669,41.9493820112901,-55.74995));
#188690=CARTESIAN_POINT('Origin',(21.,42.0482945870964,-54.74995));
#188691=CARTESIAN_POINT('Origin',(0.,-12.9675000200281,-54.74995));
#188692=CARTESIAN_POINT('',(21.3174485247294,41.3893444859658,-54.74995));
#188693=CARTESIAN_POINT('Origin',(0.,-12.9675000200281,-54.74995));
#188694=CARTESIAN_POINT('Origin',(21.5,41.8548280612684,-54.74995));
#188695=CARTESIAN_POINT('Ctrl Pts',(21.4248453217881,41.9155375404332,-55.2558060812404));
#188696=CARTESIAN_POINT('Ctrl Pts',(21.2373195046609,41.4189578841863,-55.287441243185));
#188697=CARTESIAN_POINT('Ctrl Pts',(21.16696734776,41.4480708968741,-54.7603378535211));
#188698=CARTESIAN_POINT('Ctrl Pts',(21.5755391452687,41.7984791341951,-55.2320625140271));
#188699=CARTESIAN_POINT('Ctrl Pts',(21.3763896092289,41.3649167149439,-55.2050098024457));
#188700=CARTESIAN_POINT('Ctrl Pts',(21.4662789569412,41.3318824788528,-54.7124836923955));
#188701=CARTESIAN_POINT('Ctrl Pts',(21.7343014022012,41.6710710097369,-55.2811995739867));
#188702=CARTESIAN_POINT('Ctrl Pts',(21.5979757909207,41.2778556958534,-55.2005038282256));
#188703=CARTESIAN_POINT('Ctrl Pts',(21.7817024793388,41.2055241661255,-54.8106147759211));
#188704=CARTESIAN_POINT('Ctrl Pts',(21.9601498093564,41.4868864651448,-55.4991545802739));
#188705=CARTESIAN_POINT('Ctrl Pts',(21.9275787592104,41.1463611545831,-55.4234682828707));
#188706=CARTESIAN_POINT('Ctrl Pts',(22.2307370972024,41.022808583346,-55.2471700554705));
#188707=CARTESIAN_POINT('Ctrl Pts',(22.022056389361,41.4349102113225,-55.664992125143));
#188708=CARTESIAN_POINT('Ctrl Pts',(22.0359917549909,41.102279443332,-55.6402740406839));
#188709=CARTESIAN_POINT('Ctrl Pts',(22.3539243365364,40.9712467786474,-55.5796280897733));
#188710=CARTESIAN_POINT('Ctrl Pts',(21.9927742364993,41.4593862584412,-55.8338983075843));
#188711=CARTESIAN_POINT('Ctrl Pts',(21.9870900777401,41.1221165139417,-55.8584680429781));
#188712=CARTESIAN_POINT('Ctrl Pts',(22.2956640008395,40.9955277705935,-55.9182451071506));
#188713=CARTESIAN_POINT('',(22.3089577584378,40.9899884313956,-55.74995));
#188714=CARTESIAN_POINT('Ctrl Pts',(22.3089577584378,40.9899884313956,-55.74995));
#188715=CARTESIAN_POINT('Ctrl Pts',(22.3089183239675,40.9900047357485,-55.6813689895721));
#188716=CARTESIAN_POINT('Ctrl Pts',(22.302201262956,40.9927833854558,-55.6142067014708));
#188717=CARTESIAN_POINT('Ctrl Pts',(22.2754057040688,41.0038504086268,-55.4827195699211));
#188718=CARTESIAN_POINT('Ctrl Pts',(22.2547133491493,41.0123915139066,-55.4169521642664));
#188719=CARTESIAN_POINT('Ctrl Pts',(22.2024041852375,41.0339277820542,-55.2940250464356));
#188720=CARTESIAN_POINT('Ctrl Pts',(22.1708638248328,41.0468920147473,-55.2362766810164));
#188721=CARTESIAN_POINT('Ctrl Pts',(22.0969884151167,41.0771560766471,-55.1282103371706));
#188722=CARTESIAN_POINT('Ctrl Pts',(22.0534159784586,41.094959425968,-55.0766846507022));
#188723=CARTESIAN_POINT('Ctrl Pts',(21.9138847547741,41.1517377505672,-54.9404994200361));
#188724=CARTESIAN_POINT('Ctrl Pts',(21.8055277290851,41.1955447566139,-54.8700273400709));
#188725=CARTESIAN_POINT('Ctrl Pts',(21.568431879825,41.290395306512,-54.7739654680142));
#188726=CARTESIAN_POINT('Ctrl Pts',(21.4452658848218,41.3392175880729,-54.74995));
#188727=CARTESIAN_POINT('Ctrl Pts',(21.3174485247294,41.3893444859658,-54.74995));
#188728=CARTESIAN_POINT('Origin',(22.5,41.4520521304013,-55.74995));
#188729=CARTESIAN_POINT('Origin',(22.5,41.4520521304013,-55.24995));
#188730=CARTESIAN_POINT('',(22.3089577584378,40.9899884313956,-55.24995));
#188731=CARTESIAN_POINT('Origin',(0.,-12.9675000200281,-60.5010370523947));
#188732=CARTESIAN_POINT('Origin',(0.,-12.9675000200281,-60.5010370523947));
#188733=CARTESIAN_POINT('Origin',(25.8159964412441,44.9247229809868,-55.24995));
#188734=CARTESIAN_POINT('',(23.7796330855957,40.3581899105085,-52.64995));
#188735=CARTESIAN_POINT('',(23.7796330855957,40.3581899105085,-55.24995));
#188736=CARTESIAN_POINT('Origin',(25.8159964412441,44.9247229809868,-52.64995));
#188737=CARTESIAN_POINT('Origin',(0.,-12.9675000200281,-54.74995));
#188738=CARTESIAN_POINT('',(23.9945234557419,-66.1968434349636,-54.74995));
#188739=CARTESIAN_POINT('Origin',(24.2,-66.6526716808631,-54.74995));
#188740=CARTESIAN_POINT('',(24.0682702937655,-66.1635386067456,-54.74995));
#188741=CARTESIAN_POINT('Origin',(24.2743783673579,-66.6190816475223,-54.74995));
#188742=CARTESIAN_POINT('Origin',(0.,-12.9675000200281,-54.74995));
#188743=CARTESIAN_POINT('Ctrl Pts',(24.2,-66.6526716808631,-55.24995));
#188744=CARTESIAN_POINT('Ctrl Pts',(23.9945234557419,-66.1968434349636,
-55.24995));
#188745=CARTESIAN_POINT('Ctrl Pts',(23.9945234557419,-66.1968434349636,
-54.74995));
#188746=CARTESIAN_POINT('Ctrl Pts',(24.1371955572435,-66.7092931820382,
-55.24995));
#188747=CARTESIAN_POINT('Ctrl Pts',(23.9202432240961,-66.2303271978257,
-55.2764502978682));
#188748=CARTESIAN_POINT('Ctrl Pts',(23.8699830688991,-66.2529832826787,
-54.7499500150097));
#188749=CARTESIAN_POINT('Ctrl Pts',(24.0753940809144,-66.764472406879,-55.2615406660682));
#188750=CARTESIAN_POINT('Ctrl Pts',(23.8581370153758,-66.2582349963978,
-55.3179716549212));
#188751=CARTESIAN_POINT('Ctrl Pts',(23.7474276190468,-66.3076948875735,
-54.7731313367517));
#188752=CARTESIAN_POINT('Ctrl Pts',(23.9567432347527,-66.8694948932304,
-55.3084792096817));
#188753=CARTESIAN_POINT('Ctrl Pts',(23.7601274312421,-66.3025641007665,
-55.4174636561498));
#188754=CARTESIAN_POINT('Ctrl Pts',(23.5121407959317,-66.4118256516783,
-54.867008414748));
#188755=CARTESIAN_POINT('Ctrl Pts',(23.902316841733,-66.9171958169871,-55.3428841126209));
#188756=CARTESIAN_POINT('Ctrl Pts',(23.7282344734586,-66.3172128520127,
-55.4737170925055));
#188757=CARTESIAN_POINT('Ctrl Pts',(23.4042122584794,-66.4591215590598,
-54.9358182281615));
#188758=CARTESIAN_POINT('Ctrl Pts',(23.8072473920369,-66.9999887868491,
-55.4336221821879));
#188759=CARTESIAN_POINT('Ctrl Pts',(23.6919934707232,-66.3346728811278,
-55.5807863787511));
#188760=CARTESIAN_POINT('Ctrl Pts',(23.2156877780054,-66.5412115519831,
-55.117294361456));
#188761=CARTESIAN_POINT('Ctrl Pts',(23.7684105820677,-67.0335141101085,
-55.4886013829516));
#188762=CARTESIAN_POINT('Ctrl Pts',(23.6899497583265,-66.3364476351196,
-55.6278104638636));
#188763=CARTESIAN_POINT('Ctrl Pts',(23.138673673191,-66.5744522205999,-55.227252767375));
#188764=CARTESIAN_POINT('Ctrl Pts',(23.7144942998795,-67.079931038232,-55.6126301527277));
#188765=CARTESIAN_POINT('Ctrl Pts',(23.6944387661923,-66.3359499016387,
-55.7013955638849));
#188766=CARTESIAN_POINT('Ctrl Pts',(23.0317566828166,-66.6204750325317,
-55.4753103039836));
#188767=CARTESIAN_POINT('Ctrl Pts',(23.7,-67.0923340220896,-55.6800435061715));
#188768=CARTESIAN_POINT('Ctrl Pts',(23.6999999982635,-66.3340176139022,
-55.7259208430489));
#188769=CARTESIAN_POINT('Ctrl Pts',(23.0030142327697,-66.6327727060053,
-55.6101370134438));
#188770=CARTESIAN_POINT('Ctrl Pts',(23.7,-67.0923340267327,-55.74995));
#188771=CARTESIAN_POINT('Ctrl Pts',(23.6999999999999,-66.3340176133293,
-55.74995));
#188772=CARTESIAN_POINT('Ctrl Pts',(23.0030142220336,-66.6327727106072,
-55.74995));
#188773=CARTESIAN_POINT('',(23.0030142220336,-66.6327727106072,-55.74995));
#188774=CARTESIAN_POINT('Origin',(23.2,-67.0923340267327,-55.74995));
#188775=CARTESIAN_POINT('Ctrl Pts',(23.0030142220336,-66.6327727106072,
-55.74995));
#188776=CARTESIAN_POINT('Ctrl Pts',(23.0030142252181,-66.6327727092422,
-55.7084794961837));
#188777=CARTESIAN_POINT('Ctrl Pts',(23.0055473075491,-66.6316889244747,
-55.6672305708313));
#188778=CARTESIAN_POINT('Ctrl Pts',(23.01056277729,-66.6295393332012,-55.6264611420265));
#188779=CARTESIAN_POINT('Ctrl Pts',(23.0156442349954,-66.62736146,-55.5851553144879));
#188780=CARTESIAN_POINT('Ctrl Pts',(23.0232736525723,-66.6240896154022,
-55.5443421797598));
#188781=CARTESIAN_POINT('Ctrl Pts',(23.0333489722999,-66.6197635354292,
-55.5042845968465));
#188782=CARTESIAN_POINT('Ctrl Pts',(23.0435966387888,-66.6153634542441,
-55.4635417955116));
#188783=CARTESIAN_POINT('Ctrl Pts',(23.0563743830217,-66.6098728426923,
-55.4235811788327));
#188784=CARTESIAN_POINT('Ctrl Pts',(23.0715270926204,-66.6033540441774,
-55.3846656949085));
#188785=CARTESIAN_POINT('Ctrl Pts',(23.075698862771,-66.6015593203436,-55.373951673553));
#188786=CARTESIAN_POINT('Ctrl Pts',(23.08005038839,-66.5996867754406,-55.3633167653533));
#188787=CARTESIAN_POINT('Ctrl Pts',(23.0845778500673,-66.5977379631867,
-55.3527661917799));
#188788=CARTESIAN_POINT('Ctrl Pts',(23.084790216786,-66.5976465515099,-55.3522713028445));
#188789=CARTESIAN_POINT('Ctrl Pts',(23.0850029782865,-66.5975549687209,
-55.3517765816014));
#188790=CARTESIAN_POINT('Ctrl Pts',(23.0852161343291,-66.5974632149135,
-55.3512820284305));
#188791=CARTESIAN_POINT('Ctrl Pts',(23.1225303099352,-66.5814011899272,
-55.2647076876707));
#188792=CARTESIAN_POINT('Ctrl Pts',(23.1713738964051,-66.5603327052685,
-55.1848774594373));
#188793=CARTESIAN_POINT('Ctrl Pts',(23.2296539151218,-66.5350590387655,
-55.1136222625289));
#188794=CARTESIAN_POINT('Ctrl Pts',(23.2542820784798,-66.5243788090573,
-55.0835110053912));
#188795=CARTESIAN_POINT('Ctrl Pts',(23.2805947528019,-66.5129478823946,
-55.0549311560842));
#188796=CARTESIAN_POINT('Ctrl Pts',(23.3084314920874,-66.5008277482104,
-55.0280211962633));
#188797=CARTESIAN_POINT('Ctrl Pts',(23.3089371697075,-66.5006075758495,
-55.0275323543663));
#188798=CARTESIAN_POINT('Ctrl Pts',(23.3094433520675,-66.5003871752661,
-55.0270440618915));
#188799=CARTESIAN_POINT('Ctrl Pts',(23.3099500382032,-66.5001665468298,
-55.0265563196877));
#188800=CARTESIAN_POINT('Ctrl Pts',(23.3737418241067,-66.4723894260785,
-54.9651495748625));
#188801=CARTESIAN_POINT('Ctrl Pts',(23.4438814283176,-66.4417108192607,
-54.9137085371825));
#188802=CARTESIAN_POINT('Ctrl Pts',(23.5191429186078,-66.4085890914668,
-54.8723032869094));
#188803=CARTESIAN_POINT('Ctrl Pts',(23.5545073851334,-66.3930255910721,
-54.8528474592129));
#188804=CARTESIAN_POINT('Ctrl Pts',(23.59100222619,-66.3769228800036,-54.8356069181236));
#188805=CARTESIAN_POINT('Ctrl Pts',(23.6284978920678,-66.3603295348338,
-54.8205860088575));
#188806=CARTESIAN_POINT('Ctrl Pts',(23.6289267193329,-66.360139761465,-54.8204142189909));
#188807=CARTESIAN_POINT('Ctrl Pts',(23.6293556721511,-66.359949926291,-54.8202427216662));
#188808=CARTESIAN_POINT('Ctrl Pts',(23.629784750377,-66.3597600293637,-54.8200715168436));
#188809=CARTESIAN_POINT('Ctrl Pts',(23.67833901584,-66.3382713933413,-54.8006980695174));
#188810=CARTESIAN_POINT('Ctrl Pts',(23.7276801213795,-66.3163541582091,
-54.7853871133686));
#188811=CARTESIAN_POINT('Ctrl Pts',(23.7776797138642,-66.2940596674702,
-54.7740684617324));
#188812=CARTESIAN_POINT('Ctrl Pts',(23.8282083296008,-66.2715292887288,
-54.7626300525221));
#188813=CARTESIAN_POINT('Ctrl Pts',(23.8794098794649,-66.2486134489516,
-54.7552688611601));
#188814=CARTESIAN_POINT('Ctrl Pts',(23.93115878902,-66.2253609159868,-54.7519649331453));
#188815=CARTESIAN_POINT('Ctrl Pts',(23.9521926643963,-66.2159096853277,
-54.7506220176963));
#188816=CARTESIAN_POINT('Ctrl Pts',(23.9733170103899,-66.2064027967323,
-54.7499500025558));
#188817=CARTESIAN_POINT('Ctrl Pts',(23.9945234557419,-66.1968434349636,
-54.74995));
#188818=CARTESIAN_POINT('Origin',(23.2,-67.0923340267327,-55.24995));
#188819=CARTESIAN_POINT('',(23.0030142220336,-66.6327727106072,-55.24995));
#188820=CARTESIAN_POINT('Origin',(0.,-12.9675000200281,-60.42825533736));
#188821=CARTESIAN_POINT('Origin',(0.,-12.9675000200281,-60.42825533736));
#188822=CARTESIAN_POINT('Origin',(17.55,-69.1790215814778,-55.24995));
#188823=CARTESIAN_POINT('',(17.4009870515814,-68.7017426890012,-55.74995));
#188824=CARTESIAN_POINT('',(17.4009870515814,-68.7017426890012,-55.24995));
#188825=CARTESIAN_POINT('Origin',(17.55,-69.1790215814778,-55.74995));
#188826=CARTESIAN_POINT('Ctrl Pts',(17.0433420738134,-69.1844099825972,
-55.8294677650393));
#188827=CARTESIAN_POINT('Ctrl Pts',(17.0390945871937,-68.8146441411288,
-55.8476657194646));
#188828=CARTESIAN_POINT('Ctrl Pts',(17.3877596852339,-68.7058888483382,
-55.909104778956));
#188829=CARTESIAN_POINT('Ctrl Pts',(17.0589933399128,-69.1745693542014,
-55.7377938248974));
#188830=CARTESIAN_POINT('Ctrl Pts',(17.0627281269977,-68.8074648626002,
-55.7356378606241));
#188831=CARTESIAN_POINT('Ctrl Pts',(17.4188481420652,-68.6961356562758,
-55.7256234362817));
#188832=CARTESIAN_POINT('Ctrl Pts',(17.0466637029569,-69.1823667222349,
-55.6406520746839));
#188833=CARTESIAN_POINT('Ctrl Pts',(17.0433869297458,-68.8133616424342,
-55.6136877993486));
#188834=CARTESIAN_POINT('Ctrl Pts',(17.3943527552328,-68.7038643204319,
-55.5311773838691));
#188835=CARTESIAN_POINT('Ctrl Pts',(16.9846573898727,-69.2209669761278,
-55.4940755209577));
#188836=CARTESIAN_POINT('Ctrl Pts',(16.9545279172638,-68.8401687966803,
-55.4409633820653));
#188837=CARTESIAN_POINT('Ctrl Pts',(17.2712219065013,-68.7421173320939,
-55.237857759257));
#188838=CARTESIAN_POINT('Ctrl Pts',(16.9465498226589,-69.2446125343844,
-55.438535909464));
#188839=CARTESIAN_POINT('Ctrl Pts',(16.8998247159699,-68.8566269554238,
-55.378474281339));
#188840=CARTESIAN_POINT('Ctrl Pts',(17.1955506950046,-68.7655509085055,
-55.1267370897427));
#188841=CARTESIAN_POINT('Ctrl Pts',(16.8537040849283,-69.3015957225698,
-55.3474653979614));
#188842=CARTESIAN_POINT('Ctrl Pts',(16.7731194206628,-68.894483990695,-55.286087043994));
#188843=CARTESIAN_POINT('Ctrl Pts',(17.0112333722604,-68.8220198533602,
-54.9445960314883));
#188844=CARTESIAN_POINT('Ctrl Pts',(16.7982009500299,-69.3353877920995,
-55.3111829565324));
#188845=CARTESIAN_POINT('Ctrl Pts',(16.6993048554918,-68.9164109459874,
-55.2557565295156));
#188846=CARTESIAN_POINT('Ctrl Pts',(16.9010650546211,-68.8555068833233,
-54.8720727600904));
#188847=CARTESIAN_POINT('Ctrl Pts',(16.6555913240634,-69.4210909343955,
-55.2530368583418));
#188848=CARTESIAN_POINT('Ctrl Pts',(16.5212476377685,-68.9689791681947,
-55.223696330687));
#188849=CARTESIAN_POINT('Ctrl Pts',(16.6180815577824,-68.9404329890533,
-54.7559465968208));
#188850=CARTESIAN_POINT('Ctrl Pts',(16.5619443816715,-69.4764948536126,
-55.2416586756739));
#188851=CARTESIAN_POINT('Ctrl Pts',(16.4140091296541,-69.0003625620744,
-55.2402085606976));
#188852=CARTESIAN_POINT('Ctrl Pts',(16.4323327263914,-68.9953280686919,
-54.7333548544426));
#188853=CARTESIAN_POINT('Ctrl Pts',(16.474021195344,-69.527420504419,-55.2560439941876));
#188854=CARTESIAN_POINT('Ctrl Pts',(16.3324809063319,-69.0242130218807,
-55.279736482239));
#188855=CARTESIAN_POINT('Ctrl Pts',(16.2580067759255,-69.0457880333801,
-54.7622666492363));
#188856=CARTESIAN_POINT('',(16.4094778178732,-69.001678821881,-54.74995));
#188857=CARTESIAN_POINT('Origin',(16.55,-69.4815262104644,-54.74995));
#188858=CARTESIAN_POINT('Ctrl Pts',(16.4094778178732,-69.001678821881,-54.74995));
#188859=CARTESIAN_POINT('Ctrl Pts',(16.4504095598616,-68.9896920572568,
-54.7499500048056));
#188860=CARTESIAN_POINT('Ctrl Pts',(16.4912475287743,-68.9776812452657,
-54.7525666780149));
#188861=CARTESIAN_POINT('Ctrl Pts',(16.5317041745654,-68.965736321318,-54.757667934043));
#188862=CARTESIAN_POINT('Ctrl Pts',(16.5749366447118,-68.9529718284177,
-54.7631191990857));
#188863=CARTESIAN_POINT('Ctrl Pts',(16.6177350648204,-68.9402821612408,
-54.7714073705121));
#188864=CARTESIAN_POINT('Ctrl Pts',(16.6597585620131,-68.9277728443736,
-54.7824337221977));
#188865=CARTESIAN_POINT('Ctrl Pts',(16.7017820592057,-68.9152635275064,
-54.7934600738833));
#188866=CARTESIAN_POINT('Ctrl Pts',(16.7430322683556,-68.9029340622973,
-54.8072249335998));
#188867=CARTESIAN_POINT('Ctrl Pts',(16.7831545131606,-68.8908929861314,
-54.8236888710244));
#188868=CARTESIAN_POINT('Ctrl Pts',(16.7835975596796,-68.890760023559,-54.8238706726708));
#188869=CARTESIAN_POINT('Ctrl Pts',(16.7840405080022,-68.8906270844636,
-54.8240528195673));
#188870=CARTESIAN_POINT('Ctrl Pts',(16.7844833577117,-68.8904941689839,
-54.8242353115275));
#188871=CARTESIAN_POINT('Ctrl Pts',(16.8581304439983,-68.8683899706623,
-54.8545842106013));
#188872=CARTESIAN_POINT('Ctrl Pts',(16.9287006566087,-68.8470438209497,
-54.8943416412344));
#188873=CARTESIAN_POINT('Ctrl Pts',(16.9936792242012,-68.827277340243,-54.9420858838147));
#188874=CARTESIAN_POINT('Ctrl Pts',(17.0324101749556,-68.8154953847583,
-54.9705441890173));
#188875=CARTESIAN_POINT('Ctrl Pts',(17.0691551792512,-68.8042744590648,
-55.001839638253));
#188876=CARTESIAN_POINT('Ctrl Pts',(17.1033900455892,-68.7937859900155,
-55.0356687800906));
#188877=CARTESIAN_POINT('Ctrl Pts',(17.103886172442,-68.7936339926019,-55.0361590272412));
#188878=CARTESIAN_POINT('Ctrl Pts',(17.1043818163765,-68.7934821358841,
-55.0366498500402));
#188879=CARTESIAN_POINT('Ctrl Pts',(17.1048769761793,-68.7933304202781,
-55.0371412470353));
#188880=CARTESIAN_POINT('Ctrl Pts',(17.1669690008274,-68.7743055941547,
-55.0987614233149));
#188881=CARTESIAN_POINT('Ctrl Pts',(17.2214535479527,-68.7574981762718,
-55.1694239623163));
#188882=CARTESIAN_POINT('Ctrl Pts',(17.2659841189481,-68.743713328347,-55.2463463516036));
#188883=CARTESIAN_POINT('Ctrl Pts',(17.2871667241191,-68.7371560580402,
-55.2829373174201));
#188884=CARTESIAN_POINT('Ctrl Pts',(17.3060972390717,-68.7312826257116,
-55.3209455236334));
#188885=CARTESIAN_POINT('Ctrl Pts',(17.322524151481,-68.7261792841162,-55.3600753258131));
#188886=CARTESIAN_POINT('Ctrl Pts',(17.3227235277485,-68.7261173439796,
-55.3605502509672));
#188887=CARTESIAN_POINT('Ctrl Pts',(17.3229225385083,-68.7260555164805,
-55.3610253536613));
#188888=CARTESIAN_POINT('Ctrl Pts',(17.3231211835968,-68.7259938016769,
-55.3615006331605));
#188889=CARTESIAN_POINT('Ctrl Pts',(17.3377397858477,-68.7214521129136,
-55.3964771936486));
#188890=CARTESIAN_POINT('Ctrl Pts',(17.3503329508714,-68.7175347662069,
-55.4322944098897));
#188891=CARTESIAN_POINT('Ctrl Pts',(17.3608936617493,-68.7142467873541,
-55.4687543689716));
#188892=CARTESIAN_POINT('Ctrl Pts',(17.3714744037537,-68.7109525719968,
-55.5052834838196));
#188893=CARTESIAN_POINT('Ctrl Pts',(17.3800152474177,-68.70829001851,-55.5424589028239));
#188894=CARTESIAN_POINT('Ctrl Pts',(17.3864625050711,-68.7062785938727,
-55.5800999366542));
#188895=CARTESIAN_POINT('Ctrl Pts',(17.3927323721603,-68.7043225117965,
-55.616705310893));
#188896=CARTESIAN_POINT('Ctrl Pts',(17.3970223360455,-68.7029821923561,
-55.6537520599019));
#188897=CARTESIAN_POINT('Ctrl Pts',(17.399236871165,-68.7022899564979,-55.6910754862818));
#188898=CARTESIAN_POINT('Ctrl Pts',(17.4003972743764,-68.7019272290316,
-55.7106327393816));
#188899=CARTESIAN_POINT('Ctrl Pts',(17.4009870480798,-68.7017426900946,
-55.730265892737));
#188900=CARTESIAN_POINT('Ctrl Pts',(17.4009870515814,-68.7017426890013,
-55.74995));
#188901=CARTESIAN_POINT('Origin',(0.,-12.9675000200281,-54.74995));
#188902=CARTESIAN_POINT('',(15.913723201019,-69.1444843653509,-54.74995));
#188903=CARTESIAN_POINT('Origin',(16.05,-69.6255546658886,-54.74995));
#188904=CARTESIAN_POINT('Origin',(0.,-12.9675000200281,-54.74995));
#188905=CARTESIAN_POINT('Ctrl Pts',(16.0943918791427,-69.6003138753269,
-55.2520324188857));
#188906=CARTESIAN_POINT('Ctrl Pts',(15.9626541784119,-69.1297266675286,
-55.2398173309746));
#188907=CARTESIAN_POINT('Ctrl Pts',(16.0017964545034,-69.1194462603403,
-54.7532354575004));
#188908=CARTESIAN_POINT('Ctrl Pts',(15.9520563039833,-69.6815449359842,
-55.238583696008));
#188909=CARTESIAN_POINT('Ctrl Pts',(15.7933965067921,-69.1775635977428,
-55.2661930138944));
#188910=CARTESIAN_POINT('Ctrl Pts',(15.7194486319347,-69.2000152527435,
-54.7262790994806));
#188911=CARTESIAN_POINT('Ctrl Pts',(15.8040804369175,-69.7629913547991,
-55.2908208908606));
#188912=CARTESIAN_POINT('Ctrl Pts',(15.6782147462389,-69.2100275662615,
-55.3690735314078));
#188913=CARTESIAN_POINT('Ctrl Pts',(15.4256393014046,-69.2808712212567,
-54.8307953991629));
#188914=CARTESIAN_POINT('Ctrl Pts',(15.5957850814026,-69.8754701070241,
-55.4950681095302));
#188915=CARTESIAN_POINT('Ctrl Pts',(15.5548552071343,-69.2462930289052,
-55.5833321666787));
#188916=CARTESIAN_POINT('Ctrl Pts',(15.0121582713081,-69.3925053704125,
-55.2396491450935));
#188917=CARTESIAN_POINT('Ctrl Pts',(15.5374042125397,-69.9059409697286,
-55.6453900516724));
#188918=CARTESIAN_POINT('Ctrl Pts',(15.5478910318033,-69.2494990492648,
-55.6859501835156));
#188919=CARTESIAN_POINT('Ctrl Pts',(14.89623691968,-69.4227546427598,-55.5406072672281));
#188920=CARTESIAN_POINT('Ctrl Pts',(15.5523010752554,-69.89814066138,-55.797007806289));
#188921=CARTESIAN_POINT('Ctrl Pts',(15.55041942508,-69.2484839021119,-55.7792669100244));
#188922=CARTESIAN_POINT('Ctrl Pts',(14.92581406719,-69.4150115966434,-55.8441656371953));
#188923=CARTESIAN_POINT('',(14.9222139673106,-69.4159516070034,-55.74995));
#188924=CARTESIAN_POINT('Origin',(15.05,-69.8993466109593,-55.74995));
#188925=CARTESIAN_POINT('Ctrl Pts',(14.9222139673106,-69.4159516070035,
-55.74995));
#188926=CARTESIAN_POINT('Ctrl Pts',(14.9222684167837,-69.4159372132218,
-55.6560401405972));
#188927=CARTESIAN_POINT('Ctrl Pts',(14.9355158903724,-69.4124399177686,
-55.563575015399));
#188928=CARTESIAN_POINT('Ctrl Pts',(14.9614297127064,-69.4055703024629,
-55.4737974919486));
#188929=CARTESIAN_POINT('Ctrl Pts',(14.9723367261448,-69.4026789117027,
-55.4360105286005));
#188930=CARTESIAN_POINT('Ctrl Pts',(14.985487454912,-69.3991894720854,-55.3986996822186));
#188931=CARTESIAN_POINT('Ctrl Pts',(15.0008419271996,-69.3951076046889,
-55.3619576246799));
#188932=CARTESIAN_POINT('Ctrl Pts',(15.0407650708988,-69.3844943465073,
-55.2664246480044));
#188933=CARTESIAN_POINT('Ctrl Pts',(15.0928106079671,-69.3706175165969,
-55.180386190476));
#188934=CARTESIAN_POINT('Ctrl Pts',(15.1571532348986,-69.3533214831149,
-55.1036416590134));
#188935=CARTESIAN_POINT('Ctrl Pts',(15.1763510453595,-69.348160892254,-55.0807435114059));
#188936=CARTESIAN_POINT('Ctrl Pts',(15.1966434942269,-69.3426955736518,
-55.0586727438326));
#188937=CARTESIAN_POINT('Ctrl Pts',(15.2180349745493,-69.3369205223421,
-55.037424028165));
#188938=CARTESIAN_POINT('Ctrl Pts',(15.3111212994845,-69.3117900360626,
-54.9449589522898));
#188939=CARTESIAN_POINT('Ctrl Pts',(15.4192055462156,-69.2823626792043,
-54.8734147542759));
#188940=CARTESIAN_POINT('Ctrl Pts',(15.5392134434446,-69.249228865297,-54.8240288525655));
#188941=CARTESIAN_POINT('Ctrl Pts',(15.6592213406736,-69.2160950513897,
-54.7746429508552));
#188942=CARTESIAN_POINT('Ctrl Pts',(15.7840680515859,-69.1812128616152,
-54.74995));
#188943=CARTESIAN_POINT('Ctrl Pts',(15.913723201019,-69.1444843653509,-54.74995));
#188944=CARTESIAN_POINT('Origin',(15.05,-69.8993466109593,-55.24995));
#188945=CARTESIAN_POINT('',(14.9222139673106,-69.4159516070034,-55.24995));
#188946=CARTESIAN_POINT('Origin',(0.,-12.9675000200281,-60.42825533736));
#188947=CARTESIAN_POINT('Origin',(0.,-12.9675000200281,-60.42825533736));
#188948=CARTESIAN_POINT('Origin',(9.4,-71.0999148696911,-55.24995));
#188949=CARTESIAN_POINT('',(9.32018679685842,-70.6063261212332,-55.8925850873));
#188950=CARTESIAN_POINT('',(9.32018679685842,-70.6063261212332,-55.24995));
#188951=CARTESIAN_POINT('Origin',(9.4,-71.0999148696911,-55.8925850873));
#188952=CARTESIAN_POINT('Ctrl Pts',(8.9,-71.0999148696911,-55.8925850873));
#188953=CARTESIAN_POINT('Ctrl Pts',(8.89999999999995,-70.674270243298,-55.8925850872999));
#188954=CARTESIAN_POINT('Ctrl Pts',(9.32018679685842,-70.6063261212332,
-55.8925850873));
#188955=CARTESIAN_POINT('Ctrl Pts',(8.9,-71.0753963340341,-55.8158206410579));
#188956=CARTESIAN_POINT('Ctrl Pts',(8.92045674363156,-70.670962391591,-55.8099505084873));
#188957=CARTESIAN_POINT('Ctrl Pts',(9.32018679646957,-70.606326121296,-55.7609765242912));
#188958=CARTESIAN_POINT('Ctrl Pts',(8.88914819160783,-71.0574685211989,
-55.7424878932553));
#188959=CARTESIAN_POINT('Ctrl Pts',(8.92288173642606,-70.6704214883702,
-55.7222104842267));
#188960=CARTESIAN_POINT('Ctrl Pts',(9.29866745626329,-70.6098198655576,
-55.6301334688925));
#188961=CARTESIAN_POINT('Ctrl Pts',(8.84354256567003,-71.0340357122248,
-55.606998619986));
#188962=CARTESIAN_POINT('Ctrl Pts',(8.88787909971282,-70.6754793338957,
-55.5563944136962));
#188963=CARTESIAN_POINT('Ctrl Pts',(9.20823066610786,-70.6243360556297,
-55.3829240249879));
#188964=CARTESIAN_POINT('Ctrl Pts',(8.80933590722104,-71.0287732217429,
-55.5465658668829));
#188965=CARTESIAN_POINT('Ctrl Pts',(8.8515542998134,-70.6809070626089,-55.4791108159719));
#188966=CARTESIAN_POINT('Ctrl Pts',(9.14039822217997,-70.6351795268323,
-55.2697323706429));
#188967=CARTESIAN_POINT('Ctrl Pts',(8.72031210976081,-71.028802992332,-55.4457995958176));
#188968=CARTESIAN_POINT('Ctrl Pts',(8.74741150404566,-70.6964574226719,
-55.3507681953891));
#188969=CARTESIAN_POINT('Ctrl Pts',(8.96386239650929,-70.6628838067398,
-55.0780797399289));
#188970=CARTESIAN_POINT('Ctrl Pts',(8.66589931539796,-71.0341559413013,
-55.4063653507054));
#188971=CARTESIAN_POINT('Ctrl Pts',(8.67980906181995,-70.7065384951403,
-55.2998814604829));
#188972=CARTESIAN_POINT('Ctrl Pts',(8.85596081453515,-70.679599541712,-55.0012953993776));
#188973=CARTESIAN_POINT('Ctrl Pts',(8.54658037248409,-71.0525391488741,
-55.3555557927535));
#188974=CARTESIAN_POINT('Ctrl Pts',(8.53037007175229,-70.7286009969626,
-55.2361886195966));
#188975=CARTESIAN_POINT('Ctrl Pts',(8.61934915026951,-70.7154116132197,
-54.8994528680703));
#188976=CARTESIAN_POINT('Ctrl Pts',(8.48132333269991,-71.0655965765405,
-55.3439422058851));
#188977=CARTESIAN_POINT('Ctrl Pts',(8.44749087161535,-70.7407315090392,
-55.2227831389152));
#188978=CARTESIAN_POINT('Ctrl Pts',(8.48994814797731,-70.7346037655486,
-54.8739206038906));
#188979=CARTESIAN_POINT('Ctrl Pts',(8.41560835021371,-71.0814043774774,
-55.3473655916161));
#188980=CARTESIAN_POINT('Ctrl Pts',(8.36589323739407,-70.7525502203441,
-55.2292031667485));
#188981=CARTESIAN_POINT('Ctrl Pts',(8.35962920986983,-70.7534564084689,
-54.8763024037294));
#188982=CARTESIAN_POINT('',(8.35962920986979,-70.7534564084689,-54.8763024037297));
#188983=CARTESIAN_POINT('Origin',(8.4312167004274,-71.248305103724,-54.8763024037297));
#188984=CARTESIAN_POINT('Ctrl Pts',(8.35962920986984,-70.7534564084689,
-54.8763024037297));
#188985=CARTESIAN_POINT('Ctrl Pts',(8.4266932097628,-70.7437545672695,-54.8750766952757));
#188986=CARTESIAN_POINT('Ctrl Pts',(8.49356141096506,-70.7339558949385,
-54.8812481493054));
#188987=CARTESIAN_POINT('Ctrl Pts',(8.55878406018679,-70.724290971257,-54.8944764365469));
#188988=CARTESIAN_POINT('Ctrl Pts',(8.62027176255571,-70.715179505258,-54.9069472116298));
#188989=CARTESIAN_POINT('Ctrl Pts',(8.68029576330459,-70.7061871116828,
-54.9256889700024));
#188990=CARTESIAN_POINT('Ctrl Pts',(8.73765415640112,-70.6975057024889,
-54.9503761135537));
#188991=CARTESIAN_POINT('Ctrl Pts',(8.73812533670876,-70.6974343875717,
-54.950578910307));
#188992=CARTESIAN_POINT('Ctrl Pts',(8.7385963482321,-70.6973630921029,-54.9507821155763));
#188993=CARTESIAN_POINT('Ctrl Pts',(8.7390671903714,-70.697291816191,-54.9509857288995));
#188994=CARTESIAN_POINT('Ctrl Pts',(8.81806341257938,-70.6853333967864,
-54.985147249244));
#188995=CARTESIAN_POINT('Ctrl Pts',(8.89230145001324,-70.673924118985,-55.030799607521));
#188996=CARTESIAN_POINT('Ctrl Pts',(8.95909820842037,-70.6635530304581,
-55.0858633072555));
#188997=CARTESIAN_POINT('Ctrl Pts',(8.99202329694071,-70.658440970892,-55.1130050014223));
#188998=CARTESIAN_POINT('Ctrl Pts',(9.02314073107693,-70.6535810854978,
-55.1424341547092));
#188999=CARTESIAN_POINT('Ctrl Pts',(9.05213028602996,-70.6490316704449,
-55.1739060774789));
#189000=CARTESIAN_POINT('Ctrl Pts',(9.05261593139239,-70.6489554567077,
-55.1744333085235));
#189001=CARTESIAN_POINT('Ctrl Pts',(9.05310095531287,-70.6488793344915,
-55.1749610621635));
#189002=CARTESIAN_POINT('Ctrl Pts',(9.05358535746146,-70.6488033038874,
-55.1754893372344));
#189003=CARTESIAN_POINT('Ctrl Pts',(9.10207551699106,-70.6411924042821,
-55.2283713125429));
#189004=CARTESIAN_POINT('Ctrl Pts',(9.14429186553919,-70.634506376804,-55.2864243412893));
#189005=CARTESIAN_POINT('Ctrl Pts',(9.17994788064258,-70.6288295105427,
-55.3485029540396));
#189006=CARTESIAN_POINT('Ctrl Pts',(9.20880098471937,-70.6242357495015,
-55.3987374143245));
#189007=CARTESIAN_POINT('Ctrl Pts',(9.23335776597275,-70.6203028545583,
-55.4516091557793));
#189008=CARTESIAN_POINT('Ctrl Pts',(9.25344901950571,-70.6170779672838,
-55.5065287627148));
#189009=CARTESIAN_POINT('Ctrl Pts',(9.25361952044245,-70.6170505998375,
-55.506994828429));
#189010=CARTESIAN_POINT('Ctrl Pts',(9.25378968425506,-70.6170232859403,
-55.5074609965585));
#189011=CARTESIAN_POINT('Ctrl Pts',(9.25395951106862,-70.6169960255762,
-55.5079272667724));
#189012=CARTESIAN_POINT('Ctrl Pts',(9.26917261736367,-70.6145540388982,
-55.5496958083666));
#189013=CARTESIAN_POINT('Ctrl Pts',(9.28164780823389,-70.6125470433612,
-55.5921779695173));
#189014=CARTESIAN_POINT('Ctrl Pts',(9.29152034880348,-70.6109563835461,
-55.6352174890367));
#189015=CARTESIAN_POINT('Ctrl Pts',(9.30173630321663,-70.609310393029,-55.6797541274304));
#189016=CARTESIAN_POINT('Ctrl Pts',(9.30916540444182,-70.6081101941254,
-55.7248883638107));
#189017=CARTESIAN_POINT('Ctrl Pts',(9.31390296845355,-70.6073438342246,
-55.7704597578364));
#189018=CARTESIAN_POINT('Ctrl Pts',(9.31810307746836,-70.606664414354,-55.8108612853706));
#189019=CARTESIAN_POINT('Ctrl Pts',(9.32018679673735,-70.6063261212527,
-55.8516070077995));
#189020=CARTESIAN_POINT('Ctrl Pts',(9.32018679685842,-70.6063261212332,
-55.8925850873));
#189021=CARTESIAN_POINT('Ctrl Pts',(8.41560835021369,-71.0814043774777,
-55.3473655916165));
#189022=CARTESIAN_POINT('Ctrl Pts',(8.36589323739404,-70.752550220344,-55.2292031667489));
#189023=CARTESIAN_POINT('Ctrl Pts',(8.35962920986988,-70.7534564084689,
-54.8763024037297));
#189024=CARTESIAN_POINT('Ctrl Pts',(8.24918690883785,-71.102010310254,-55.3491521481271));
#189025=CARTESIAN_POINT('Ctrl Pts',(8.2013544983267,-70.7763714724242,-55.2294679275358));
#189026=CARTESIAN_POINT('Ctrl Pts',(8.19486187074245,-70.7772925435282,
-54.8793138184774));
#189027=CARTESIAN_POINT('Ctrl Pts',(8.08271475024063,-71.1220068981801,
-55.3508246944299));
#189028=CARTESIAN_POINT('Ctrl Pts',(8.03626733023182,-70.7995543826982,
-55.2297202388378));
#189029=CARTESIAN_POINT('Ctrl Pts',(8.02999374674379,-70.8004238120746,
-54.8822160506073));
#189030=CARTESIAN_POINT('Ctrl Pts',(7.91618843693366,-71.141394090941,-55.3523946663951));
#189031=CARTESIAN_POINT('Ctrl Pts',(7.87072047725699,-70.8220758845274,
-55.2299609924931));
#189032=CARTESIAN_POINT('Ctrl Pts',(7.86502491569137,-70.8228501557662,
-54.8850140141151));
#189033=CARTESIAN_POINT('',(7.86502491569136,-70.8228501557662,-54.8850140141151));
#189034=CARTESIAN_POINT('Origin',(7.93237687386467,-71.3182931027643,-54.8850140141151));
#189035=CARTESIAN_POINT('Origin',(0.0280298706655902,-14.2420762575896,
-46.3192185165476));
#189036=CARTESIAN_POINT('Ctrl Pts',(7.91618843693208,-71.1413940909409,
-55.352394666395));
#189037=CARTESIAN_POINT('Ctrl Pts',(7.87072047725574,-70.8220758845275,
-55.2299609924928));
#189038=CARTESIAN_POINT('Ctrl Pts',(7.86502491569091,-70.8228501557662,
-54.8850140141151));
#189039=CARTESIAN_POINT('Ctrl Pts',(7.844285602846,-71.157562039706,-55.3560236134997));
#189040=CARTESIAN_POINT('Ctrl Pts',(7.77985413280654,-70.8344428879727,
-55.236521459352));
#189041=CARTESIAN_POINT('Ctrl Pts',(7.72241706825884,-70.8422366821738,
-54.8874327557878));
#189042=CARTESIAN_POINT('Ctrl Pts',(7.77219443565847,-71.177222127411,-55.3781864762555));
#189043=CARTESIAN_POINT('Ctrl Pts',(7.69016530757976,-70.8464897855799,
-55.2681271844367));
#189044=CARTESIAN_POINT('Ctrl Pts',(7.5794821547774,-70.8610938450093,-54.9239881329105));
#189045=CARTESIAN_POINT('Ctrl Pts',(7.64331486532417,-71.2207339188645,
-55.4539331018544));
#189046=CARTESIAN_POINT('Ctrl Pts',(7.53737924067218,-70.8668804541439,
-55.3692852810369));
#189047=CARTESIAN_POINT('Ctrl Pts',(7.32391158111293,-70.8939799308472,
-55.0534925677837));
#189048=CARTESIAN_POINT('Ctrl Pts',(7.58567352642291,-71.2449041853563,
-55.5078568245776));
#189049=CARTESIAN_POINT('Ctrl Pts',(7.47303212720142,-70.8754018535837,
-55.4405214339084));
#189050=CARTESIAN_POINT('Ctrl Pts',(7.20960774580809,-70.9082476913312,
-55.1469663768362));
#189051=CARTESIAN_POINT('Ctrl Pts',(7.49322857950783,-71.2966779191941,
-55.6376571876191));
#189052=CARTESIAN_POINT('Ctrl Pts',(7.38267219174721,-70.8874980297502,
-55.6027965247728));
#189053=CARTESIAN_POINT('Ctrl Pts',(7.02628770602923,-70.9307639518508,
-55.3693141862512));
#189054=CARTESIAN_POINT('Ctrl Pts',(7.45777202258463,-71.3246266217341,
-55.7141753031788));
#189055=CARTESIAN_POINT('Ctrl Pts',(7.35664509914443,-70.8910885028411,
-55.6963616877968));
#189056=CARTESIAN_POINT('Ctrl Pts',(6.95597670016225,-70.9391888126349,
-55.4992549495758));
#189057=CARTESIAN_POINT('Ctrl Pts',(7.41125924474539,-71.38419243799,-55.8811540356734));
#189058=CARTESIAN_POINT('Ctrl Pts',(7.34624804767826,-70.8930407983775,
-55.8848711139694));
#189059=CARTESIAN_POINT('Ctrl Pts',(6.86374100295758,-70.950181682438,-55.7748476118441));
#189060=CARTESIAN_POINT('Ctrl Pts',(7.4,-71.4160375965177,-55.9720928529598));
#189061=CARTESIAN_POINT('Ctrl Pts',(7.36384050363832,-70.8911630457611,
-55.9819410866112));
#189062=CARTESIAN_POINT('Ctrl Pts',(6.84141371299613,-70.9528017322803,
-55.9212771125469));
#189063=CARTESIAN_POINT('Ctrl Pts',(7.4,-71.4493575166339,-56.06661116875));
#189064=CARTESIAN_POINT('Ctrl Pts',(7.3999999999998,-70.8868967568689,-56.06661116875));
#189065=CARTESIAN_POINT('Ctrl Pts',(6.84141371258755,-70.9528017323285,
-56.0666111687498));
#189066=CARTESIAN_POINT('',(6.84141371258755,-70.9528017323285,-56.0666111687498));
#189067=CARTESIAN_POINT('',(6.9,-70.949357516634,-56.0666111687498));
#189068=CARTESIAN_POINT('Origin',(6.9,-71.449357516634,-56.0666111687498));
#189069=CARTESIAN_POINT('Origin',(6.9,-71.449357516634,-56.0666111687498));
#189070=CARTESIAN_POINT('Ctrl Pts',(6.84141371258755,-70.9528017323285,
-56.0666111687498));
#189071=CARTESIAN_POINT('Ctrl Pts',(6.84141371272281,-70.9528017323125,
-56.0185004951022));
#189072=CARTESIAN_POINT('Ctrl Pts',(6.84385625486988,-70.9525150960356,
-55.9705185340177));
#189073=CARTESIAN_POINT('Ctrl Pts',(6.8487439595216,-70.951938515923,-55.9228849154069));
#189074=CARTESIAN_POINT('Ctrl Pts',(6.85371160739849,-70.9513525052747,
-55.8744722020329));
#189075=CARTESIAN_POINT('Ctrl Pts',(6.86120476133719,-70.9504670347036,
-55.8264180258316));
#189076=CARTESIAN_POINT('Ctrl Pts',(6.87128050874745,-70.9492722819139,
-55.7789472465282));
#189077=CARTESIAN_POINT('Ctrl Pts',(6.88084558986923,-70.9481380824459,
-55.7338824154578));
#189078=CARTESIAN_POINT('Ctrl Pts',(6.89273836925604,-70.9467251353176,
-55.6893423359324));
#189079=CARTESIAN_POINT('Ctrl Pts',(6.90705554696957,-70.9450193012211,
-55.6455309032989));
#189080=CARTESIAN_POINT('Ctrl Pts',(6.9078199210414,-70.9449282291272,-55.6431918722535));
#189081=CARTESIAN_POINT('Ctrl Pts',(6.90859121688159,-70.9448363208197,
-55.6408549230079));
#189082=CARTESIAN_POINT('Ctrl Pts',(6.90936945309023,-70.944743573674,-55.638520088397));
#189083=CARTESIAN_POINT('Ctrl Pts',(6.90953264041296,-70.9447241256476,
-55.6380305000112));
#189084=CARTESIAN_POINT('Ctrl Pts',(6.90969612810931,-70.9447046413087,
-55.6375410188016));
#189085=CARTESIAN_POINT('Ctrl Pts',(6.90985991625218,-70.9446851206452,
-55.6370516451987));
#189086=CARTESIAN_POINT('Ctrl Pts',(6.93890470840672,-70.9412234926851,
-55.5502703047937));
#189087=CARTESIAN_POINT('Ctrl Pts',(6.97755496303265,-70.9365992546703,
-55.4665613054823));
#189088=CARTESIAN_POINT('Ctrl Pts',(7.02515534568111,-70.9308292795786,
-55.388637952601));
#189089=CARTESIAN_POINT('Ctrl Pts',(7.052652463843,-70.9274961616905,-55.3436242883712));
#189090=CARTESIAN_POINT('Ctrl Pts',(7.08313672341692,-70.92378064339,-55.3005419198593));
#189091=CARTESIAN_POINT('Ctrl Pts',(7.11648530834342,-70.9196854249332,
-55.2599212236758));
#189092=CARTESIAN_POINT('Ctrl Pts',(7.11697272521332,-70.9196255699628,
-55.2593275189465));
#189093=CARTESIAN_POINT('Ctrl Pts',(7.11746075366589,-70.9195656339149,
-55.2587343401393));
#189094=CARTESIAN_POINT('Ctrl Pts',(7.11794939330103,-70.9195056167998,
-55.2581416889457));
#189095=CARTESIAN_POINT('Ctrl Pts',(7.17766958662853,-70.9121704899281,
-55.1857094887866));
#189096=CARTESIAN_POINT('Ctrl Pts',(7.24707274855584,-70.9035491680659,
-55.1207030262999));
#189097=CARTESIAN_POINT('Ctrl Pts',(7.32365993963188,-70.8938669826863,
-55.0662525944808));
#189098=CARTESIAN_POINT('Ctrl Pts',(7.36395975880566,-70.8887722623484,
-55.0376010337509));
#189099=CARTESIAN_POINT('Ctrl Pts',(7.40624788203792,-70.8833838941673,
-55.011872736897));
#189100=CARTESIAN_POINT('Ctrl Pts',(7.450155212976,-70.8777352422905,-54.9895263260323));
#189101=CARTESIAN_POINT('Ctrl Pts',(7.45066930715087,-70.8776691043822,
-54.989264680439));
#189102=CARTESIAN_POINT('Ctrl Pts',(7.45118359869241,-70.877602933957,-54.9890035107279));
#189103=CARTESIAN_POINT('Ctrl Pts',(7.45169808724107,-70.8775367310404,
-54.9887428173532));
#189104=CARTESIAN_POINT('Ctrl Pts',(7.48702485166254,-70.8729909839197,
-54.9708426066328));
#189105=CARTESIAN_POINT('Ctrl Pts',(7.52340553096597,-70.8682741670682,
-54.9551443604244));
#189106=CARTESIAN_POINT('Ctrl Pts',(7.5606036934083,-70.8634146986663,-54.9417107539087));
#189107=CARTESIAN_POINT('Ctrl Pts',(7.59755058615544,-70.8585880554651,
-54.9283678899994));
#189108=CARTESIAN_POINT('Ctrl Pts',(7.63530511490774,-70.8536205390166,
-54.9172587967144));
#189109=CARTESIAN_POINT('Ctrl Pts',(7.67365359691508,-70.8485368945066,
-54.9084923483496));
#189110=CARTESIAN_POINT('Ctrl Pts',(7.71043547056373,-70.8436609265346,
-54.9000840260582));
#189111=CARTESIAN_POINT('Ctrl Pts',(7.74776474509213,-70.8386779998652,
-54.8938307755624));
#189112=CARTESIAN_POINT('Ctrl Pts',(7.78545391476942,-70.8336090347271,
-54.8898753244176));
#189113=CARTESIAN_POINT('Ctrl Pts',(7.81182391853935,-70.8300624288733,
-54.887107811562));
#189114=CARTESIAN_POINT('Ctrl Pts',(7.83837014274921,-70.8264736832847,
-54.8854661001065));
#189115=CARTESIAN_POINT('Ctrl Pts',(7.86502491569091,-70.8228501557662,
-54.8850140141151));
#189116=CARTESIAN_POINT('Origin',(6.9,-71.449357516634,-55.24995));
#189117=CARTESIAN_POINT('',(6.84141371258755,-70.9528017323285,-55.24995));
#189118=CARTESIAN_POINT('Origin',(0.,-12.9675000200281,-60.42825533736));
#189119=CARTESIAN_POINT('Origin',(0.,-12.9675000200281,-60.42825533736));
#189120=CARTESIAN_POINT('Origin',(1.24999999999996,-71.8417317029411,-55.24995));
#189121=CARTESIAN_POINT('',(1.2393865421354,-71.3418443611208,-56.1920015047684));
#189122=CARTESIAN_POINT('',(1.2393865421354,-71.3418443611208,-55.24995));
#189123=CARTESIAN_POINT('Origin',(1.24999999999996,-71.8417317029411,-56.1920015047684));
#189124=CARTESIAN_POINT('Ctrl Pts',(0.74992832526643,-71.8476124042683,
-56.2095834390661));
#189125=CARTESIAN_POINT('Ctrl Pts',(0.744108865482373,-71.351962221307,
-56.2095867879049));
#189126=CARTESIAN_POINT('Ctrl Pts',(1.23964458126955,-71.341839523454,-56.2153597573814));
#189127=CARTESIAN_POINT('Ctrl Pts',(0.751776125714688,-71.7713204575019,
-55.9817509371667));
#189128=CARTESIAN_POINT('Ctrl Pts',(0.816837216474583,-71.3505250778188,
-55.9987951501326));
#189129=CARTESIAN_POINT('Ctrl Pts',(1.24327926489108,-71.3417496291435,
-55.9137659627895));
#189130=CARTESIAN_POINT('Ctrl Pts',(0.718072267663703,-71.7066743634015,
-55.7785946996364));
#189131=CARTESIAN_POINT('Ctrl Pts',(0.824825378281954,-71.350036513351,
-55.7487495717777));
#189132=CARTESIAN_POINT('Ctrl Pts',(1.17639466159895,-71.3434192147202,
-55.6016397278362));
#189133=CARTESIAN_POINT('Ctrl Pts',(0.584670453989408,-71.6422004184537,
-55.5485996630821));
#189134=CARTESIAN_POINT('Ctrl Pts',(0.68043710643303,-71.3513071664449,
-55.4568954173326));
#189135=CARTESIAN_POINT('Ctrl Pts',(0.911756750913512,-71.34794523375,-55.2318343014585));
#189136=CARTESIAN_POINT('Ctrl Pts',(0.529612862082923,-71.6265518657637,
-55.4878844649265));
#189137=CARTESIAN_POINT('Ctrl Pts',(0.61348963780591,-71.3519450763092,
-55.3771436564239));
#189138=CARTESIAN_POINT('Ctrl Pts',(0.802538014423018,-71.3496280189885,
-55.1308312312545));
#189139=CARTESIAN_POINT('Ctrl Pts',(0.395598613078437,-71.6049256773685,
-55.4002431537929));
#189140=CARTESIAN_POINT('Ctrl Pts',(0.442382077620753,-71.3532818922767,
-55.2625191895523));
#189141=CARTESIAN_POINT('Ctrl Pts',(0.53669485310282,-71.3526926510771,
-54.9837531096389));
#189142=CARTESIAN_POINT('Ctrl Pts',(0.318989062465326,-71.5999429306173,
-55.3774294426603));
#189143=CARTESIAN_POINT('Ctrl Pts',(0.339989995154795,-71.3539406609335,
-55.2314667911085));
#189144=CARTESIAN_POINT('Ctrl Pts',(0.3847301999498,-71.3539511178465,-54.9445588028));
#189145=CARTESIAN_POINT('Ctrl Pts',(0.238798012754718,-71.6010945930311,
-55.3801419188632));
#189146=CARTESIAN_POINT('Ctrl Pts',(0.233742017347619,-71.3543709520858,
-55.2351306094688));
#189147=CARTESIAN_POINT('Ctrl Pts',(0.225655240690842,-71.354563899099,
-54.9490093924302));
#189148=CARTESIAN_POINT('',(0.249602310815417,-71.3544665017672,-54.9489505784606));
#189149=CARTESIAN_POINT('Ctrl Pts',(0.249602310815417,-71.3544665017672,
-54.9489505784606));
#189150=CARTESIAN_POINT('Ctrl Pts',(0.324383151711637,-71.3541468161967,
-54.9489131643343));
#189151=CARTESIAN_POINT('Ctrl Pts',(0.433588595141249,-71.35346461301,-54.9628114661091));
#189152=CARTESIAN_POINT('Ctrl Pts',(0.538344474802224,-71.3525282945736,
-54.9976414023299));
#189153=CARTESIAN_POINT('Ctrl Pts',(0.607192878775931,-71.3518528742047,
-55.0255128341318));
#189154=CARTESIAN_POINT('Ctrl Pts',(0.642806300227351,-71.3514701198547,
-55.0427102506267));
#189155=CARTESIAN_POINT('Ctrl Pts',(0.73806134014663,-71.3503695531929,
-55.0956639309939));
#189156=CARTESIAN_POINT('Ctrl Pts',(0.8263152279403,-71.3491952833432,-55.1589825749407));
#189157=CARTESIAN_POINT('Ctrl Pts',(0.917026830650857,-71.3478072668677,
-55.2509930124761));
#189158=CARTESIAN_POINT('Ctrl Pts',(0.953278076391069,-71.3472187265559,
-55.2943129184764));
#189159=CARTESIAN_POINT('Ctrl Pts',(0.97686221842195,-71.346828857815,-55.3240566027749));
#189160=CARTESIAN_POINT('Ctrl Pts',(0.989578654400162,-71.3466143523215,
-55.3410674841052));
#189161=CARTESIAN_POINT('Ctrl Pts',(1.15945421218685,-71.3437057224535,
-55.5795506821725));
#189162=CARTESIAN_POINT('Ctrl Pts',(1.23938654213546,-71.3418443611209,
-55.8585192145883));
#189163=CARTESIAN_POINT('Ctrl Pts',(1.2393865421354,-71.3418443611208,-56.1920015047684));
#189164=CARTESIAN_POINT('Origin',(0.251739774406202,-71.8544619329957,-54.9489505784606));
#189165=CARTESIAN_POINT('Origin',(0.,-12.9675000200281,-55.24995));
#189166=CARTESIAN_POINT('',(24.0682702937655,-66.1635386067456,-52.64995));
#189167=CARTESIAN_POINT('Origin',(0.,-12.9675000200281,-52.64995));
#189168=CARTESIAN_POINT('Origin',(8.64724958304919E-13,-13.7566898295974,
-48.2080483433929));
#189169=CARTESIAN_POINT('',(24.0682702937655,-66.1635386067456,-55.24995));
#189170=CARTESIAN_POINT('Origin',(52.9858497431864,-37.4950331867729,-52.64995));
#189171=CARTESIAN_POINT('',(52.9112495105562,-38.347717747534,-52.64995));
#189172=CARTESIAN_POINT('',(52.9112495105562,-38.347717747534,-52.64995));
#189173=CARTESIAN_POINT('',(51.3604079243415,-56.0739181912695,-52.64995));
#189174=CARTESIAN_POINT('',(52.9858497431864,-37.4950331867729,-52.64995));
#189175=CARTESIAN_POINT('',(51.3604079243415,-56.0739181912695,-52.64995));
#189176=CARTESIAN_POINT('Origin',(48.3718238300662,-55.8124509630266,-59.64995));
#189177=CARTESIAN_POINT('Origin',(48.3718238300662,-55.8124509630266,-59.64995));
#189178=CARTESIAN_POINT('Origin',(51.265241636025,-57.1616738441871,-52.64995));
#189179=CARTESIAN_POINT('',(44.9662712865582,-63.4606441936539,-52.64995));
#189180=CARTESIAN_POINT('',(44.9662712865582,-63.4606441936539,-52.64995));
#189181=CARTESIAN_POINT('',(50.4931441736259,-57.9337713065862,-52.64995));
#189182=CARTESIAN_POINT('',(50.4931441736259,-57.9337713065862,-52.64995));
#189183=CARTESIAN_POINT('',(51.265241636025,-57.1616738441871,-52.64995));
#189184=CARTESIAN_POINT('Origin',(48.3718238300662,-55.8124509630266,-52.64995));
#189185=CARTESIAN_POINT('Origin',(48.3718238300662,-55.8124509630266,-52.64995));
#189186=CARTESIAN_POINT('Origin',(42.8449509429986,-61.3393238500942,-59.64995));
#189187=CARTESIAN_POINT('Origin',(42.8449509429986,-61.3393238500942,-59.64995));
#189188=CARTESIAN_POINT('Origin',(44.1941738241591,-64.2327416560529,-52.64995));
#189189=CARTESIAN_POINT('',(43.1064181712415,-64.3279079443695,-52.64995));
#189190=CARTESIAN_POINT('',(43.1064181712415,-64.3279079443695,-52.64995));
#189191=CARTESIAN_POINT('',(25.043451507077,-65.9082127571302,-52.64995));
#189192=CARTESIAN_POINT('',(44.1941738241591,-64.2327416560529,-52.64995));
#189193=CARTESIAN_POINT('',(25.043451507077,-65.9082127571302,-55.24995));
#189194=CARTESIAN_POINT('Origin',(42.8449509429986,-61.3393238500942,-52.64995));
#189195=CARTESIAN_POINT('Origin',(42.8449509429986,-61.3393238500942,-52.64995));
#189196=CARTESIAN_POINT('Ctrl Pts',(24.579016252936,-65.9859437829616,-54.74995));
#189197=CARTESIAN_POINT('Ctrl Pts',(24.579016252936,-65.9859437829616,-55.24995));
#189198=CARTESIAN_POINT('Ctrl Pts',(24.7,-66.4710859610356,-55.24995));
#189199=CARTESIAN_POINT('Ctrl Pts',(24.7361092859404,-65.946768249212,-54.749950009163));
#189200=CARTESIAN_POINT('Ctrl Pts',(24.67310951117,-65.9624790000681,-55.2343403176332));
#189201=CARTESIAN_POINT('Ctrl Pts',(24.7654791450057,-66.4384278647148,
-55.24995));
#189202=CARTESIAN_POINT('Ctrl Pts',(24.8931309886626,-65.9213640983868,
-54.7753029040978));
#189203=CARTESIAN_POINT('Ctrl Pts',(24.7709452774937,-65.9414368141194,
-55.24317591549));
#189204=CARTESIAN_POINT('Ctrl Pts',(24.8308799729202,-66.4172697443503,
-55.2626259569449));
#189205=CARTESIAN_POINT('Ctrl Pts',(25.043451507077,-65.9082127571302,-54.8278826162281));
#189206=CARTESIAN_POINT('Ctrl Pts',(24.8576734148988,-65.9244662341272,
-55.273872259957));
#189207=CARTESIAN_POINT('Ctrl Pts',(24.8935146892254,-66.4063101061761,
-55.2889163081141));
#189208=CARTESIAN_POINT('',(24.579016252936,-65.9859437829616,-54.74995));
#189209=CARTESIAN_POINT('Origin',(24.7,-66.4710859610356,-54.74995));
#189210=CARTESIAN_POINT('Ctrl Pts',(24.579016252936,-65.9859437829616,-54.74995));
#189211=CARTESIAN_POINT('Ctrl Pts',(24.6281997735959,-65.9736784989023,
-54.7499500028688));
#189212=CARTESIAN_POINT('Ctrl Pts',(24.6769571248861,-65.9628648823717,
-54.7524316796293));
#189213=CARTESIAN_POINT('Ctrl Pts',(24.7252054215613,-65.9533744504568,
-54.757346690394));
#189214=CARTESIAN_POINT('Ctrl Pts',(24.7738214860051,-65.9438116786831,
-54.7622991653318));
#189215=CARTESIAN_POINT('Ctrl Pts',(24.8219213290088,-65.935592502924,-54.7697220721195));
#189216=CARTESIAN_POINT('Ctrl Pts',(24.8694314110454,-65.9286135012,-54.7796095236809));
#189217=CARTESIAN_POINT('Ctrl Pts',(24.9169285718598,-65.9216363975412,
-54.7894942861719));
#189218=CARTESIAN_POINT('Ctrl Pts',(24.9638369024156,-65.9158989677116,
-54.801842144168));
#189219=CARTESIAN_POINT('Ctrl Pts',(25.0100848485165,-65.9113231861505,
-54.8166923677705));
#189220=CARTESIAN_POINT('Ctrl Pts',(25.021245893932,-65.9102189099584,-54.8202761814105));
#189221=CARTESIAN_POINT('Ctrl Pts',(25.0323684634138,-65.9091823978081,
-54.8240059448895));
#189222=CARTESIAN_POINT('Ctrl Pts',(25.043451507077,-65.9082127571302,-54.8278826162281));
#189223=CARTESIAN_POINT('Origin',(25.30491873532,-68.8967968514054,-54.74995));
#189224=CARTESIAN_POINT('Origin',(25.30491873532,-68.8967968514054,-54.74995));
#189225=CARTESIAN_POINT('Origin',(25.30491873532,-68.8967968514054,-55.24995));
#189226=CARTESIAN_POINT('Origin',(25.30491873532,-68.8967968514054,-52.64995));
#189227=CARTESIAN_POINT('Ctrl Pts',(0.250869887203161,-71.6009673739963,
-55.3799259279347));
#189228=CARTESIAN_POINT('Ctrl Pts',(0.249744175923989,-71.3544658952986,
-55.234934426789));
#189229=CARTESIAN_POINT('Ctrl Pts',(0.249602310815494,-71.3544665017672,
-54.948950578461));
#189230=CARTESIAN_POINT('Ctrl Pts',(0.0835826979643991,-71.6015824809948,
-55.3799500715247));
#189231=CARTESIAN_POINT('Ctrl Pts',(0.0832191858260445,-71.355178188438,
-55.2349402623292));
#189232=CARTESIAN_POINT('Ctrl Pts',(0.0831608417598922,-71.3551780334291,
-54.9490338518609));
#189233=CARTESIAN_POINT('Ctrl Pts',(-0.0836629414004135,-71.6015821858332,
-55.3799500598782));
#189234=CARTESIAN_POINT('Ctrl Pts',(-0.0832990585829135,-71.3551778467503,
-55.2349402595226));
#189235=CARTESIAN_POINT('Ctrl Pts',(-0.0832406798117105,-71.3551776921241,
-54.9490338120093));
#189236=CARTESIAN_POINT('Ctrl Pts',(-0.250869887202844,-71.6009673739968,
-55.3799259279345));
#189237=CARTESIAN_POINT('Ctrl Pts',(-0.249744175923751,-71.3544658952987,
-55.2349344267889));
#189238=CARTESIAN_POINT('Ctrl Pts',(-0.249602310815417,-71.3544665017672,
-54.9489505784605));
#189239=CARTESIAN_POINT('Origin',(-6.81954492876002E-12,-3.47778663927897,
-52.706487452645));
#189240=CARTESIAN_POINT('Ctrl Pts',(-0.252999996541928,-73.08000002,-57.9657930806539));
#189241=CARTESIAN_POINT('Ctrl Pts',(-0.256592825118373,-73.0800000199999,
-56.2374226811825));
#189242=CARTESIAN_POINT('Ctrl Pts',(-0.25839495935019,-71.5847761540179,
-55.3704858385599));
#189243=CARTESIAN_POINT('Ctrl Pts',(-0.084333524296533,-73.08000002,-57.9654424673068));
#189244=CARTESIAN_POINT('Ctrl Pts',(-0.0855465369638168,-73.0800000199968,
-56.2375896397646));
#189245=CARTESIAN_POINT('Ctrl Pts',(-0.0861369317764507,-71.585454968994,
-55.3705213407165));
#189246=CARTESIAN_POINT('Ctrl Pts',(0.0843331399670236,-73.08000002,-57.9654424664997));
#189247=CARTESIAN_POINT('Ctrl Pts',(0.0855461472403026,-73.0800000199999,
-56.2375896401512));
#189248=CARTESIAN_POINT('Ctrl Pts',(0.0861365392586797,-71.5854549705621,
-55.3705213407996));
#189249=CARTESIAN_POINT('Ctrl Pts',(0.253000003458008,-73.08000002,-57.9657930806683));
#189250=CARTESIAN_POINT('Ctrl Pts',(0.256592832132617,-73.08000002,-56.2374226811757));
#189251=CARTESIAN_POINT('Ctrl Pts',(0.25839496641364,-71.5847761539902,
-55.3704858385584));
#189252=CARTESIAN_POINT('Origin',(1.31216565391057E-11,-73.08000002,-179.672570889095));
#189253=CARTESIAN_POINT('Origin',(-3.54807775957937E-14,-73.08000002,3.11172719585489E-30));
#189254=CARTESIAN_POINT('Origin',(1.0476064460363E-11,-73.08000002,-65.1484573036958));
#189255=CARTESIAN_POINT('Ctrl Pts',(0.253000177461644,-73.08000002,-174.689799914929));
#189256=CARTESIAN_POINT('Ctrl Pts',(0.256818808114103,-73.0800000199999,
-176.343172927719));
#189257=CARTESIAN_POINT('Ctrl Pts',(0.258858142486708,-71.6821458347228,
-177.226154478591));
#189258=CARTESIAN_POINT('Ctrl Pts',(0.0843234703769069,-73.08000002,-174.69018949069));
#189259=CARTESIAN_POINT('Ctrl Pts',(0.0856112439477064,-73.0800000199999,
-176.343045073677));
#189260=CARTESIAN_POINT('Ctrl Pts',(0.0862809304106464,-71.6828245492958,
-177.226124337495));
#189261=CARTESIAN_POINT('Ctrl Pts',(-0.0843431922589527,-73.08000002,-174.690189444595));
#189262=CARTESIAN_POINT('Ctrl Pts',(-0.0856312602925202,-73.0800000199957,
-176.343045088817));
#189263=CARTESIAN_POINT('Ctrl Pts',(-0.0863011085778896,-71.6828244689879,
-177.226124341061));
#189264=CARTESIAN_POINT('Ctrl Pts',(-0.252999822559396,-73.08000002,-174.689799915749));
#189265=CARTESIAN_POINT('Ctrl Pts',(-0.25681844785831,-73.0800000199999,
-176.34317292745));
#189266=CARTESIAN_POINT('Ctrl Pts',(-0.258857779373677,-71.6821458361509,
-177.226154478528));
#189267=CARTESIAN_POINT('Origin',(-1.05821948426232E-11,-3.44156790446887,
-179.298801253201));
#189268=CARTESIAN_POINT('Ctrl Pts',(0.24975130544611,-71.4669668918333,
-177.637584354353));
#189269=CARTESIAN_POINT('Ctrl Pts',(0.249886372443607,-71.4669663151929,
-177.363982952545));
#189270=CARTESIAN_POINT('Ctrl Pts',(0.250942965994211,-71.697396290156,
-177.216474798318));
#189271=CARTESIAN_POINT('Ctrl Pts',(0.0832106206914701,-71.467677902645,
-177.637501435082));
#189272=CARTESIAN_POINT('Ctrl Pts',(0.0832664445309527,-71.4676780488509,
-177.363977402067));
#189273=CARTESIAN_POINT('Ctrl Pts',(0.0836071881580228,-71.698010936898,
-177.216456047988));
#189274=CARTESIAN_POINT('Ctrl Pts',(-0.0832902307503821,-71.4676775627664,
-177.637501474743));
#189275=CARTESIAN_POINT('Ctrl Pts',(-0.0833460872557474,-71.4676777086203,
-177.363977404876));
#189276=CARTESIAN_POINT('Ctrl Pts',(-0.0836871780041486,-71.6980106428669,
-177.216456057091));
#189277=CARTESIAN_POINT('Ctrl Pts',(-0.249751305446095,-71.4669668918333,
-177.637584354353));
#189278=CARTESIAN_POINT('Ctrl Pts',(-0.249886372443348,-71.4669663151928,
-177.363982952544));
#189279=CARTESIAN_POINT('Ctrl Pts',(-0.250942965993822,-71.6973962901568,
-177.216474798318));
#189280=CARTESIAN_POINT('Origin',(1.46650053212127E-12,-13.7527233284612,
-184.368315095325));
#189281=CARTESIAN_POINT('Origin',(0.,-12.9675000200281,-179.64995));
#189282=CARTESIAN_POINT('Origin',(0.,-12.9675000200281,-179.39995));
#189283=CARTESIAN_POINT('Origin',(0.,-12.9675000200281,-179.39995));
#189284=CARTESIAN_POINT('Origin',(0.,-12.9675000200281,-179.64995));
#189285=CARTESIAN_POINT('Origin',(50.5696324866523,-53.08000002,-179.64995));
#189286=CARTESIAN_POINT('Origin',(0.,-12.9675000200281,-179.64995));
#189287=CARTESIAN_POINT('Origin',(0.,-12.9675000200281,-179.39995));
#189288=CARTESIAN_POINT('Origin',(0.,-12.9675000200281,-179.39995));
#189289=CARTESIAN_POINT('Origin',(0.,-12.9675000200281,-179.64995));
#189290=CARTESIAN_POINT('Origin',(0.,-12.9675000200281,-177.84995));
#189291=CARTESIAN_POINT('Origin',(0.,-12.9675000200281,-177.84995));
#189292=CARTESIAN_POINT('Origin',(0.,-12.9675000200281,-177.34995));
#189293=CARTESIAN_POINT('Origin',(-41.5,58.91999998,-177.34995));
#189294=CARTESIAN_POINT('',(-41.5,58.91999998,-177.34995));
#189295=CARTESIAN_POINT('Origin',(0.,58.91999998,0.));
#189296=CARTESIAN_POINT('',(-41.5,58.91999998,-92.34995));
#189297=CARTESIAN_POINT('Origin',(-41.5,58.91999998,-92.34995));
#189298=CARTESIAN_POINT('Origin',(1.1373643128445E-15,-12.9675000200281,
-92.34995));
#189299=CARTESIAN_POINT('Origin',(1.1373643128445E-15,-12.9675000200281,
-91.34995));
#189300=CARTESIAN_POINT('Origin',(1.1373643128445E-15,-12.9675000200281,
-90.9273317382593));
#189301=CARTESIAN_POINT('Origin',(0.,-12.9675000200281,-60.64995));
#189302=CARTESIAN_POINT('Origin',(0.,-12.9675000200281,-60.8508735991007));
#189303=CARTESIAN_POINT('Origin',(0.,-12.9675000200281,-60.42825533736));
#189304=CARTESIAN_POINT('Origin',(0.,-12.9675000200281,-60.42825533736));
#189305=CARTESIAN_POINT('Origin',(0.,-12.9675000200281,-55.24995));
#189306=CARTESIAN_POINT('Origin',(0.,-12.9675000200281,-52.64995));
#189307=CARTESIAN_POINT('Origin',(57.8922230010149,-38.7834964612722,-55.24995));
#189308=CARTESIAN_POINT('Origin',(57.8922230010149,-38.7834964612722,-52.64995));
#189309=CARTESIAN_POINT('Origin',(80.1225000199719,-131.7,-52.64995));
#189310=CARTESIAN_POINT('Origin',(47.392180948596,37.1573950045021,-220.195349461621));
#189311=CARTESIAN_POINT('',(47.392180948596,37.1573950045021,-221.195349461621));
#189312=CARTESIAN_POINT('',(47.392180948596,37.1573950045021,-223.85005));
#189313=CARTESIAN_POINT('',(47.392180948596,37.1573950045021,-220.195349461621));
#189314=CARTESIAN_POINT('',(48.892180948596,38.0234204082866,-223.85005));
#189315=CARTESIAN_POINT('Ctrl Pts',(47.392180948596,37.1573950045022,-223.85005));
#189316=CARTESIAN_POINT('Ctrl Pts',(48.142180948596,37.5904077063944,-223.417037298108));
#189317=CARTESIAN_POINT('Ctrl Pts',(48.8921809485959,38.0234204082866,-223.85005));
#189318=CARTESIAN_POINT('',(48.892180948596,38.0234204082866,-221.195349461621));
#189319=CARTESIAN_POINT('',(48.892180948596,38.0234204082866,-220.195349461621));
#189320=CARTESIAN_POINT('Ctrl Pts',(48.8921809485959,38.0234204082865,-221.195349461621));
#189321=CARTESIAN_POINT('Ctrl Pts',(48.142180948596,37.5904077063944,-220.945349461621));
#189322=CARTESIAN_POINT('Ctrl Pts',(47.3921809485961,37.1573950045022,-221.195349461621));
#189323=CARTESIAN_POINT('Origin',(47.392180948596,35.4253441969333,-220.195349461621));
#189324=CARTESIAN_POINT('',(47.392180948596,35.4253441969333,-221.195349461621));
#189325=CARTESIAN_POINT('',(47.392180948596,35.4253441969333,-223.85005));
#189326=CARTESIAN_POINT('',(47.392180948596,35.4253441969333,-220.195349461621));
#189327=CARTESIAN_POINT('Ctrl Pts',(47.392180948596,35.4253441969333,-223.85005));
#189328=CARTESIAN_POINT('Ctrl Pts',(47.392180948596,36.2913696007178,-223.417037298108));
#189329=CARTESIAN_POINT('Ctrl Pts',(47.392180948596,37.1573950045023,-223.85005));
#189330=CARTESIAN_POINT('Ctrl Pts',(47.392180948596,37.1573950045021,-221.195349461621));
#189331=CARTESIAN_POINT('Ctrl Pts',(47.392180948596,36.2913696007177,-220.945349461621));
#189332=CARTESIAN_POINT('Ctrl Pts',(47.392180948596,35.4253441969334,-221.195349461621));
#189333=CARTESIAN_POINT('Origin',(48.892180948596,34.5593187931488,-220.195349461621));
#189334=CARTESIAN_POINT('',(48.892180948596,34.5593187931488,-221.195349461621));
#189335=CARTESIAN_POINT('',(48.892180948596,34.5593187931488,-223.85005));
#189336=CARTESIAN_POINT('',(48.892180948596,34.5593187931488,-220.195349461621));
#189337=CARTESIAN_POINT('Ctrl Pts',(48.892180948596,34.5593187931488,-223.85005));
#189338=CARTESIAN_POINT('Ctrl Pts',(48.142180948596,34.9923314950411,-223.417037298108));
#189339=CARTESIAN_POINT('Ctrl Pts',(47.392180948596,35.4253441969333,-223.85005));
#189340=CARTESIAN_POINT('Ctrl Pts',(47.3921809485957,35.4253441969335,-221.195349461621));
#189341=CARTESIAN_POINT('Ctrl Pts',(48.1421809485959,34.9923314950412,-220.945349461621));
#189342=CARTESIAN_POINT('Ctrl Pts',(48.8921809485959,34.5593187931489,-221.195349461621));
#189343=CARTESIAN_POINT('Origin',(50.392180948596,35.4253441969333,-220.195349461621));
#189344=CARTESIAN_POINT('',(50.392180948596,35.4253441969323,-221.19534946162));
#189345=CARTESIAN_POINT('',(50.392180948596,35.4253441969333,-223.85005));
#189346=CARTESIAN_POINT('',(50.392180948596,35.4253441969333,-220.195349461621));
#189347=CARTESIAN_POINT('Ctrl Pts',(50.392180948596,35.4253441969333,-223.85005));
#189348=CARTESIAN_POINT('Ctrl Pts',(49.642180948596,34.9923314950411,-223.417037298108));
#189349=CARTESIAN_POINT('Ctrl Pts',(48.8921809485959,34.5593187931488,-223.85005));
#189350=CARTESIAN_POINT('Ctrl Pts',(48.8921809485957,34.5593187931487,-221.195349461621));
#189351=CARTESIAN_POINT('Ctrl Pts',(49.6421809485957,34.9923314950409,-220.945349461621));
#189352=CARTESIAN_POINT('Ctrl Pts',(50.3921809485954,35.425344196933,-221.195349461621));
#189353=CARTESIAN_POINT('Origin',(50.392180948596,37.1573950045021,-220.195349461621));
#189354=CARTESIAN_POINT('',(50.392180948596,37.1573950045021,-221.195349461621));
#189355=CARTESIAN_POINT('',(50.392180948596,37.1573950045021,-223.85005));
#189356=CARTESIAN_POINT('',(50.392180948596,37.1573950045021,-220.195349461621));
#189357=CARTESIAN_POINT('Ctrl Pts',(50.392180948596,37.1573950045021,-223.85005));
#189358=CARTESIAN_POINT('Ctrl Pts',(50.392180948596,36.2913696007177,-223.417037298108));
#189359=CARTESIAN_POINT('Ctrl Pts',(50.392180948596,35.4253441969334,-223.85005));
#189360=CARTESIAN_POINT('Ctrl Pts',(50.392180948596,35.4253441969324,-221.195349461621));
#189361=CARTESIAN_POINT('Ctrl Pts',(50.392180948596,36.2913696007174,-220.945349461621));
#189362=CARTESIAN_POINT('Ctrl Pts',(50.392180948596,37.1573950045021,-221.195349461621));
#189363=CARTESIAN_POINT('Origin',(48.892180948596,38.0234204082866,-220.195349461621));
#189364=CARTESIAN_POINT('Ctrl Pts',(48.892180948596,38.0234204082866,-223.85005));
#189365=CARTESIAN_POINT('Ctrl Pts',(49.642180948596,37.5904077063944,-223.417037298108));
#189366=CARTESIAN_POINT('Ctrl Pts',(50.3921809485959,37.1573950045022,-223.85005));
#189367=CARTESIAN_POINT('Ctrl Pts',(50.392180948596,37.1573950045022,-221.195349461621));
#189368=CARTESIAN_POINT('Ctrl Pts',(49.642180948596,37.5904077063944,-220.945349461621));
#189369=CARTESIAN_POINT('Ctrl Pts',(48.892180948596,38.0234204082866,-221.195349461621));
#189370=CARTESIAN_POINT('Origin',(48.892180948596,36.2913696007177,-221.35005));
#189371=CARTESIAN_POINT('',(48.892180948596,36.2913696007177,-220.195349461621));
#189372=CARTESIAN_POINT('',(48.892180948596,34.2913696007177,-221.35005));
#189373=CARTESIAN_POINT('Origin',(48.892180948596,36.2913696007177,-223.85005));
#189374=CARTESIAN_POINT('Origin',(48.892180948596,36.2913696007177,-223.85005));
#189375=CARTESIAN_POINT('Origin',(48.892180948596,36.2913696007177,-223.85005));
#189376=CARTESIAN_POINT('Origin',(48.892180948596,36.2913696007177,-223.85005));
#189377=CARTESIAN_POINT('Origin',(48.892180948596,36.2913696007177,-223.85005));
#189378=CARTESIAN_POINT('Origin',(48.892180948596,36.2913696007177,-223.85005));
#189379=CARTESIAN_POINT('Origin',(48.892180948596,36.2913696007177,-223.85005));
#189380=CARTESIAN_POINT('Origin',(48.892180948596,36.2913696007177,-223.85005));
#189381=CARTESIAN_POINT('Origin',(48.892180948596,36.2913696007177,-223.85005));
#189382=CARTESIAN_POINT('Origin',(48.892180948596,36.2913696007177,-223.85005));
#189383=CARTESIAN_POINT('Origin',(48.892180948596,36.2913696007177,-223.85005));
#189384=CARTESIAN_POINT('Origin',(48.892180948596,36.2913696007177,-223.85005));
#189385=CARTESIAN_POINT('Origin',(48.892180948596,36.2913696007177,-223.60005));
#189386=CARTESIAN_POINT('',(48.892180948596,33.2913696007177,-223.85005));
#189387=CARTESIAN_POINT('Origin',(48.892180948596,36.2913696007177,-223.85005));
#189388=CARTESIAN_POINT('',(48.892180948596,33.0413696007177,-223.60005));
#189389=CARTESIAN_POINT('Origin',(48.892180948596,33.2913696007177,-223.60005));
#189390=CARTESIAN_POINT('',(48.892180948596,39.5413696007177,-223.60005));
#189391=CARTESIAN_POINT('Origin',(48.892180948596,36.2913696007177,-223.60005));
#189392=CARTESIAN_POINT('Origin',(48.892180948596,36.2913696007177,-223.60005));
#189393=CARTESIAN_POINT('Origin',(48.892180948596,36.2913696007177,-218.35005));
#189394=CARTESIAN_POINT('',(48.892180948596,39.5413696007177,-218.35005));
#189395=CARTESIAN_POINT('Origin',(48.892180948596,36.2913696007177,-218.35005));
#189396=CARTESIAN_POINT('Origin',(48.892180948596,36.2913696007177,-223.85005));
#189397=CARTESIAN_POINT('Origin',(48.892180948596,36.2913696007177,-223.85005));
#189398=CARTESIAN_POINT('',(48.892180948596,39.5413696007177,-223.85005));
#189399=CARTESIAN_POINT('Origin',(44.5079524583208,-57.4754524783487,-39.8944822890418));
#189400=CARTESIAN_POINT('',(46.5079524583208,-57.4754524783487,-40.4194822890418));
#189401=CARTESIAN_POINT('Origin',(44.5079524583208,-57.4754524783487,-40.4194822890418));
#189402=CARTESIAN_POINT('',(45.9829524583208,-57.4754524783487,-39.8944822890418));
#189403=CARTESIAN_POINT('',(45.9829524583208,-57.4754524783487,-39.8944822890418));
#189404=CARTESIAN_POINT('Origin',(44.5079524583208,-57.4754524783487,-39.8944822890418));
#189405=CARTESIAN_POINT('Origin',(44.5079524583208,-57.4754524783487,-39.8944822890418));
#189406=CARTESIAN_POINT('Origin',(44.5079524583208,-57.4754524783487,-39.8944822890418));
#189407=CARTESIAN_POINT('',(46.5079524583208,-57.4754524783487,-55.24995));
#189408=CARTESIAN_POINT('Origin',(44.5079524583208,-57.4754524783487,-55.24995));
#189409=CARTESIAN_POINT('',(46.5079524583208,-57.4754524783487,-39.8944822890418));
#189410=CARTESIAN_POINT('Origin',(0.,45.41999998,-55.24995));
#189411=CARTESIAN_POINT('',(47.0079524583208,-57.4754524783487,-55.24995));
#189412=CARTESIAN_POINT('Origin',(44.5079524583208,-57.4754524783487,-55.24995));
#189413=CARTESIAN_POINT('Origin',(44.5079524583208,-57.4754524783487,-48.1788821881345));
#189414=CARTESIAN_POINT('',(47.0079524583208,-57.4754524783487,-179.64995));
#189415=CARTESIAN_POINT('Origin',(44.5079524583208,-57.4754524783487,-179.64995));
#189416=CARTESIAN_POINT('',(47.0079524583208,-57.4754524783487,-48.1788821881345));
#189417=CARTESIAN_POINT('Origin',(44.5079524583208,-57.4754524783487,-179.64995));
#189418=CARTESIAN_POINT('Ctrl Pts',(-52.1258919562643,38.67266339879,-228.35005));
#189419=CARTESIAN_POINT('Ctrl Pts',(-51.7302447133037,38.3813101134616,
-228.35005));
#189420=CARTESIAN_POINT('Ctrl Pts',(-51.7233397168138,38.3762252975093,
-227.858776203219));
#189421=CARTESIAN_POINT('Ctrl Pts',(-52.0466039743291,38.878041220954,-228.35005));
#189422=CARTESIAN_POINT('Ctrl Pts',(-51.6128088111955,38.5425689461205,
-228.410692739194));
#189423=CARTESIAN_POINT('Ctrl Pts',(-51.6174495896917,38.5200202664566,
-227.858776175692));
#189424=CARTESIAN_POINT('Ctrl Pts',(-51.9333069568917,39.0542288907298,
-228.338384512236));
#189425=CARTESIAN_POINT('Ctrl Pts',(-51.5043449566927,38.6663650434491,
-228.441452922891));
#189426=CARTESIAN_POINT('Ctrl Pts',(-51.5002798258237,38.6559630716119,
-227.854887707304));
#189427=CARTESIAN_POINT('Ctrl Pts',(-51.6439737530735,39.342374196026,-228.3384118607));
#189428=CARTESIAN_POINT('Ctrl Pts',(-51.2577525408945,38.9120667908531,
-228.441337182113));
#189429=CARTESIAN_POINT('Ctrl Pts',(-51.247332174135,38.9079983209904,-227.854896823446));
#189430=CARTESIAN_POINT('Ctrl Pts',(-51.4685984426326,39.4543128793957,
-228.35005));
#189431=CARTESIAN_POINT('Ctrl Pts',(-51.1344983277446,39.0193462915006,
-228.410782960183));
#189432=CARTESIAN_POINT('Ctrl Pts',(-51.1119650116918,39.023887086559,-227.858776175352));
#189433=CARTESIAN_POINT('Ctrl Pts',(-51.2626335243565,39.533036088795,-228.35005));
#189434=CARTESIAN_POINT('Ctrl Pts',(-50.9726066716339,39.136415486161,-228.35005));
#189435=CARTESIAN_POINT('Ctrl Pts',(-50.9675450051224,39.1294935022024,
-227.858776203219));
#189436=CARTESIAN_POINT('',(-52.1258919562641,38.6726633987897,-228.35005));
#189437=CARTESIAN_POINT('',(-51.7233397168138,38.3762252975093,-227.858776203219));
#189438=CARTESIAN_POINT('Origin',(-52.1258919562641,38.6726633987897,-227.85005));
#189439=CARTESIAN_POINT('',(-51.2626335243563,39.5330360887948,-228.35005));
#189440=CARTESIAN_POINT('Ctrl Pts',(-52.1258919562641,38.6726633987897,
-228.35005));
#189441=CARTESIAN_POINT('Ctrl Pts',(-52.0466039743291,38.878041220954,-228.35005));
#189442=CARTESIAN_POINT('Ctrl Pts',(-51.9333069568917,39.0542288907298,
-228.338384512236));
#189443=CARTESIAN_POINT('Ctrl Pts',(-51.6439737530735,39.342374196026,-228.3384118607));
#189444=CARTESIAN_POINT('Ctrl Pts',(-51.4685984426326,39.4543128793957,
-228.35005));
#189445=CARTESIAN_POINT('Ctrl Pts',(-51.2626335243563,39.5330360887948,
-228.35005));
#189446=CARTESIAN_POINT('',(-50.9675450051224,39.1294935022024,-227.858776203219));
#189447=CARTESIAN_POINT('Origin',(-51.2626335243564,39.5330360887949,-227.85005));
#189448=CARTESIAN_POINT('Ctrl Pts',(-50.9675450051224,39.1294935022024,
-227.858776203219));
#189449=CARTESIAN_POINT('Ctrl Pts',(-51.1119650120529,39.0238870864862,
-227.858776184197));
#189450=CARTESIAN_POINT('Ctrl Pts',(-51.2473321742961,38.9079983210533,
-227.854896832514));
#189451=CARTESIAN_POINT('Ctrl Pts',(-51.5002798258866,38.6559630717727,
-227.854887716373));
#189452=CARTESIAN_POINT('Ctrl Pts',(-51.6174495896174,38.520020266818,-227.858776184536));
#189453=CARTESIAN_POINT('Ctrl Pts',(-51.7233397168138,38.3762252975093,
-227.858776203219));
#189454=CARTESIAN_POINT('Origin',(-48.1334350484927,-61.7961505568785,-227.85005));
#189455=CARTESIAN_POINT('',(-48.1334350484927,-57.7802512760377,-228.35005));
#189456=CARTESIAN_POINT('Origin',(-48.1334350484927,-61.7961505568785,-228.35005));
#189457=CARTESIAN_POINT('',(-48.1334350484927,-58.2801751236159,-227.858776203219));
#189458=CARTESIAN_POINT('Origin',(-48.1334350484927,-57.7802512760377,-227.85005));
#189459=CARTESIAN_POINT('',(-48.1334350484927,-65.3121259901411,-227.858776203219));
#189460=CARTESIAN_POINT('Origin',(-48.1334350484927,-61.7961505568785,-227.858776203219));
#189461=CARTESIAN_POINT('Origin',(-48.1334350484927,-61.7961505568785,-227.858776203219));
#189462=CARTESIAN_POINT('Ctrl Pts',(-54.3075179287798,-60.4058635314347,
-219.986910060041));
#189463=CARTESIAN_POINT('Ctrl Pts',(-53.9849086976504,-60.7491038125482,
-220.006959754302));
#189464=CARTESIAN_POINT('Ctrl Pts',(-54.2123842387114,-60.9809369188682,
-220.34872120014));
#189465=CARTESIAN_POINT('Ctrl Pts',(-54.4118428785764,-60.5120824447637,
-219.845412347007));
#189466=CARTESIAN_POINT('Ctrl Pts',(-54.0902539551932,-60.8227589927709,
-219.884871134182));
#189467=CARTESIAN_POINT('Ctrl Pts',(-54.2905773520916,-61.0606279145824,
-220.207250076519));
#189468=CARTESIAN_POINT('Ctrl Pts',(-54.5038491541938,-60.6290451815934,
-219.706184350974));
#189469=CARTESIAN_POINT('Ctrl Pts',(-54.1883692315684,-60.9105945733191,
-219.759116870628));
#189470=CARTESIAN_POINT('Ctrl Pts',(-54.359483942211,-61.1484321661822,
-220.068048613768));
#189471=CARTESIAN_POINT('Ctrl Pts',(-54.6622597796057,-60.8851359437949,
-219.432400986523));
#189472=CARTESIAN_POINT('Ctrl Pts',(-54.3601921871582,-61.1113013655168,
-219.509518223974));
#189473=CARTESIAN_POINT('Ctrl Pts',(-54.4780017311477,-61.3407746536632,
-219.794316977736));
#189474=CARTESIAN_POINT('Ctrl Pts',(-54.7291280292794,-61.0257268060043,
-219.296601153239));
#189475=CARTESIAN_POINT('Ctrl Pts',(-54.4358335264202,-61.2248747082992,
-219.383842189251));
#189476=CARTESIAN_POINT('Ctrl Pts',(-54.5279586596326,-61.446412888813,
-219.65854206581));
#189477=CARTESIAN_POINT('Ctrl Pts',(-54.8292130354716,-61.3244815513707,
-219.038012931782));
#189478=CARTESIAN_POINT('Ctrl Pts',(-54.5543689314778,-61.4719546649741,
-219.14339871115));
#189479=CARTESIAN_POINT('Ctrl Pts',(-54.6025429402354,-61.6709815877615,
-219.399995666978));
#189480=CARTESIAN_POINT('Ctrl Pts',(-54.8629184699328,-61.4823979173529,
-218.91503263841));
#189481=CARTESIAN_POINT('Ctrl Pts',(-54.5990060222798,-61.6050459038155,
-219.027646728977));
#189482=CARTESIAN_POINT('Ctrl Pts',(-54.6275380455226,-61.7897249373759,
-219.277032330244));
#189483=CARTESIAN_POINT('Ctrl Pts',(-54.8898067560436,-61.8191471195152,
-218.684386523561));
#189484=CARTESIAN_POINT('Ctrl Pts',(-54.6493563799718,-61.8922244718457,
-218.810400243034));
#189485=CARTESIAN_POINT('Ctrl Pts',(-54.647034139304,-62.0430255579662,
-219.046408327256));
#189486=CARTESIAN_POINT('Ctrl Pts',(-54.8823609599705,-61.9966926518129,
-218.577969748942));
#189487=CARTESIAN_POINT('Ctrl Pts',(-54.6555291975718,-62.0456431176188,
-218.709001772434));
#189488=CARTESIAN_POINT('Ctrl Pts',(-54.6410642456133,-62.1766218791827,
-218.939992225722));
#189489=CARTESIAN_POINT('Ctrl Pts',(-54.848380895554,-62.1772035872432,
-218.488025452359));
#189490=CARTESIAN_POINT('Ctrl Pts',(-54.6359260398381,-62.2035651560494,
-218.622717457036));
#189491=CARTESIAN_POINT('Ctrl Pts',(-54.6151554910244,-62.3124799546862,
-218.850050000001));
#189492=CARTESIAN_POINT('',(-54.8483808955536,-62.1772035872456,-218.488025452358));
#189493=CARTESIAN_POINT('',(-54.615155491024,-62.3124799546881,-218.85005));
#189494=CARTESIAN_POINT('Origin',(-55.1063041457817,-62.4061442430845,-218.85005));
#189495=CARTESIAN_POINT('',(-54.3075179287798,-60.4058635314347,-219.986910060041));
#189496=CARTESIAN_POINT('Ctrl Pts',(-54.848380895554,-62.1772035872432,
-218.488025452359));
#189497=CARTESIAN_POINT('Ctrl Pts',(-54.8595780951869,-62.1177211520375,
-218.517664132037));
#189498=CARTESIAN_POINT('Ctrl Pts',(-54.8678564354561,-62.0587810758137,
-218.548979039057));
#189499=CARTESIAN_POINT('Ctrl Pts',(-54.8734777099623,-62.0004951202735,
-218.581727253403));
#189500=CARTESIAN_POINT('Ctrl Pts',(-54.8794967639978,-61.938084662374,
-218.616792837108));
#189501=CARTESIAN_POINT('Ctrl Pts',(-54.8824693653365,-61.8764235088643,
-218.653502177912));
#189502=CARTESIAN_POINT('Ctrl Pts',(-54.8826645527091,-61.8156518057411,
-218.691591283871));
#189503=CARTESIAN_POINT('Ctrl Pts',(-54.8828436018076,-61.7599047637286,
-218.726531147015));
#189504=CARTESIAN_POINT('Ctrl Pts',(-54.8806845561614,-61.7049057976097,
-218.762632937314));
#189505=CARTESIAN_POINT('Ctrl Pts',(-54.8763620068721,-61.6507727587229,
-218.799709864555));
#189506=CARTESIAN_POINT('Ctrl Pts',(-54.8763424593423,-61.6505279570743,
-218.799877534671));
#189507=CARTESIAN_POINT('Ctrl Pts',(-54.8763228688493,-61.6502831758786,
-218.800045222108));
#189508=CARTESIAN_POINT('Ctrl Pts',(-54.8763032354027,-61.6500384151225,
-218.800212926867));
#189509=CARTESIAN_POINT('Ctrl Pts',(-54.8628119724682,-61.4818493143656,
-218.915452449409));
#189510=CARTESIAN_POINT('Ctrl Pts',(-54.8291146403181,-61.3241894585148,
-219.038266143607));
#189511=CARTESIAN_POINT('Ctrl Pts',(-54.7791703042592,-61.1751043200491,
-219.167307118481));
#189512=CARTESIAN_POINT('Ctrl Pts',(-54.7790856375892,-61.174851587843,
-219.167525871407));
#189513=CARTESIAN_POINT('Ctrl Pts',(-54.7790009228209,-61.1745988809923,
-219.167744642781));
#189514=CARTESIAN_POINT('Ctrl Pts',(-54.7789161599765,-61.1743461995148,
-219.167963432577));
#189515=CARTESIAN_POINT('Ctrl Pts',(-54.7321821211911,-61.0350301342545,
-219.28859330143));
#189516=CARTESIAN_POINT('Ctrl Pts',(-54.6708383603461,-60.9034276385766,
-219.414819506217));
#189517=CARTESIAN_POINT('Ctrl Pts',(-54.5985282010653,-60.7825291661754,
-219.542285530591));
#189518=CARTESIAN_POINT('Ctrl Pts',(-54.5934244574704,-60.7739959972504,
-219.55128224574));
#189519=CARTESIAN_POINT('Ctrl Pts',(-54.5882660645263,-60.7655161587595,
-219.560285146215));
#189520=CARTESIAN_POINT('Ctrl Pts',(-54.5830542956885,-60.757090705388,
-219.569292703597));
#189521=CARTESIAN_POINT('Ctrl Pts',(-54.5829701683847,-60.7569547034476,
-219.569438101741));
#189522=CARTESIAN_POINT('Ctrl Pts',(-54.5828860266502,-60.7568187140274,
-219.569583502502));
#189523=CARTESIAN_POINT('Ctrl Pts',(-54.5828018704853,-60.7566827371269,
-219.569728905881));
#189524=CARTESIAN_POINT('Ctrl Pts',(-54.5036381576416,-60.62877248456,-219.706506423312));
#189525=CARTESIAN_POINT('Ctrl Pts',(-54.4117181269149,-60.5119554283026,
-219.845581549818));
#189526=CARTESIAN_POINT('Ctrl Pts',(-54.3075179287798,-60.4058635314347,
-219.986910060041));
#189527=CARTESIAN_POINT('',(-54.2123842387114,-60.9809369188682,-220.34872120014));
#189528=CARTESIAN_POINT('Origin',(-54.5692758093764,-60.630753528645,-220.34872120014));
#189529=CARTESIAN_POINT('Ctrl Pts',(-54.2123842387114,-60.9809369188682,
-220.34872120014));
#189530=CARTESIAN_POINT('Ctrl Pts',(-54.2905773520916,-61.0606279145824,
-220.207250076519));
#189531=CARTESIAN_POINT('Ctrl Pts',(-54.359483942211,-61.1484321661822,
-220.068048613768));
#189532=CARTESIAN_POINT('Ctrl Pts',(-54.4780017311477,-61.3407746536632,
-219.794316977736));
#189533=CARTESIAN_POINT('Ctrl Pts',(-54.5279586596326,-61.446412888813,
-219.65854206581));
#189534=CARTESIAN_POINT('Ctrl Pts',(-54.6025429402354,-61.6709815877615,
-219.399995666978));
#189535=CARTESIAN_POINT('Ctrl Pts',(-54.6275380455226,-61.7897249373759,
-219.277032330244));
#189536=CARTESIAN_POINT('Ctrl Pts',(-54.647034139304,-62.0430255579662,
-219.046408327256));
#189537=CARTESIAN_POINT('Ctrl Pts',(-54.6410642456133,-62.1766218791827,
-218.939992225722));
#189538=CARTESIAN_POINT('Ctrl Pts',(-54.615155491024,-62.3124799546881,
-218.85005));
#189539=CARTESIAN_POINT('Ctrl Pts',(-54.2123842387114,-60.9809369188682,
-220.34872120014));
#189540=CARTESIAN_POINT('Ctrl Pts',(-53.9849086976503,-60.7491038125481,
-220.006959754301));
#189541=CARTESIAN_POINT('Ctrl Pts',(-54.3075179287798,-60.4058635314347,
-219.986910060041));
#189542=CARTESIAN_POINT('Ctrl Pts',(-52.433041068884,-59.1675083087135,
-222.763182656182));
#189543=CARTESIAN_POINT('Ctrl Pts',(-52.2079291156962,-58.9380840675622,
-222.419842682816));
#189544=CARTESIAN_POINT('Ctrl Pts',(-52.5270340116508,-58.593055911284,
-222.401810820094));
#189545=CARTESIAN_POINT('Ctrl Pts',(-50.6562579911382,-57.3566888322572,
-225.181485677498));
#189546=CARTESIAN_POINT('Ctrl Pts',(-50.428037288823,-57.124096290766,-224.842059161051));
#189547=CARTESIAN_POINT('Ctrl Pts',(-50.7503363279055,-56.7819842883116,
-224.820210504335));
#189548=CARTESIAN_POINT('Ctrl Pts',(-48.8796513269547,-55.5460491487752,
-227.60005));
#189549=CARTESIAN_POINT('Ctrl Pts',(-48.6520074870279,-55.3140445196239,
-227.259140997287));
#189550=CARTESIAN_POINT('Ctrl Pts',(-48.9740484537045,-54.9709070690089,
-227.238815650979));
#189551=CARTESIAN_POINT('',(-48.8796513269546,-55.5460491487752,-227.60005));
#189552=CARTESIAN_POINT('',(-48.9740484537045,-54.9709070690089,-227.238815650979));
#189553=CARTESIAN_POINT('Origin',(-49.2365428976196,-55.195865758552,-227.60005));
#189554=CARTESIAN_POINT('Ctrl Pts',(-48.8796513269547,-55.5460491487752,
-227.60005));
#189555=CARTESIAN_POINT('Ctrl Pts',(-50.6562583519279,-57.3566891999582,
-225.181485185797));
#189556=CARTESIAN_POINT('Ctrl Pts',(-52.4330406746144,-59.1675079068912,
-222.763183190988));
#189557=CARTESIAN_POINT('Ctrl Pts',(-54.2123842387114,-60.9809369188682,
-220.34872120014));
#189558=CARTESIAN_POINT('Ctrl Pts',(-54.3075179287797,-60.4058635314346,
-219.98691006004));
#189559=CARTESIAN_POINT('Ctrl Pts',(-53.9280885484023,-60.0195458200305,
-220.501536611982));
#189560=CARTESIAN_POINT('Ctrl Pts',(-53.5487761278274,-59.6334370507339,
-221.016322062621));
#189561=CARTESIAN_POINT('Ctrl Pts',(-53.1695953219721,-59.247391120128,
-221.531234538341));
#189562=CARTESIAN_POINT('Ctrl Pts',(-52.822845399714,-58.8943632390786,
-222.002107162083));
#189563=CARTESIAN_POINT('Ctrl Pts',(-52.4762070166413,-58.5413872899351,
-222.473086011508));
#189564=CARTESIAN_POINT('Ctrl Pts',(-52.1296859830356,-58.1883927825386,
-222.944146711797));
#189565=CARTESIAN_POINT('Ctrl Pts',(-51.8076614103319,-57.8603523625148,
-223.381906922627));
#189566=CARTESIAN_POINT('Ctrl Pts',(-51.4857387604864,-57.532295845902,
-223.81973782087));
#189567=CARTESIAN_POINT('Ctrl Pts',(-51.1639046996426,-57.204208016568,
-224.257619844239));
#189568=CARTESIAN_POINT('Ctrl Pts',(-50.9738908938116,-57.0105019279858,
-224.516149440352));
#189569=CARTESIAN_POINT('Ctrl Pts',(-50.7839075752795,-56.8167857278758,
-224.774696857818));
#189570=CARTESIAN_POINT('Ctrl Pts',(-50.5939477257631,-56.6230638244338,
-225.033258070589));
#189571=CARTESIAN_POINT('Ctrl Pts',(-50.2918176133923,-56.314950185659,
-225.444498279865));
#189572=CARTESIAN_POINT('Ctrl Pts',(-49.9897484304673,-56.006819869112,
-225.85577338675));
#189573=CARTESIAN_POINT('Ctrl Pts',(-49.6876934835399,-55.6987203846147,
-226.26706719271));
#189574=CARTESIAN_POINT('Ctrl Pts',(-49.4498154301899,-55.4560820621642,
-226.590974385465));
#189575=CARTESIAN_POINT('Ctrl Pts',(-49.211945725251,-55.2134636586754,
-226.914893175522));
#189576=CARTESIAN_POINT('Ctrl Pts',(-48.9740484537044,-54.9709070690088,
-227.238815650979));
#189577=CARTESIAN_POINT('Origin',(-55.1063041457817,-62.4061442430845,-218.85005));
#189578=CARTESIAN_POINT('',(-55.1063041458243,-62.4061442430364,-218.35005));
#189579=CARTESIAN_POINT('Origin',(-55.1063041458054,-62.4061442430575,-218.85005));
#189580=CARTESIAN_POINT('Origin',(-55.1063041457932,-62.4061442430715,-218.85005));
#189581=CARTESIAN_POINT('Ctrl Pts',(-47.09240585629,-55.1677510010868,-228.462945982586));
#189582=CARTESIAN_POINT('Ctrl Pts',(-47.2381429264814,-55.2254222593817,
-228.322991735478));
#189583=CARTESIAN_POINT('Ctrl Pts',(-47.4171327932804,-55.3325755327477,
-228.334859743751));
#189584=CARTESIAN_POINT('Ctrl Pts',(-47.2344276267258,-54.917085392156,
-228.523519253622));
#189585=CARTESIAN_POINT('Ctrl Pts',(-47.3356274805824,-55.0226067438265,
-228.38397647119));
#189586=CARTESIAN_POINT('Ctrl Pts',(-47.4809019204392,-55.1586334957497,
-228.371096678113));
#189587=CARTESIAN_POINT('Ctrl Pts',(-47.4670751686631,-54.738003414354,
-228.471361175594));
#189588=CARTESIAN_POINT('Ctrl Pts',(-47.5256804778557,-54.8863412485756,
-228.335161447142));
#189589=CARTESIAN_POINT('Ctrl Pts',(-47.6309431060146,-55.0605826721568,
-228.339785024153));
#189590=CARTESIAN_POINT('Ctrl Pts',(-47.8754484729887,-54.5910305088289,
-228.271269171667));
#189591=CARTESIAN_POINT('Ctrl Pts',(-47.8504418710462,-54.8033124018473,
-228.155509466566));
#189592=CARTESIAN_POINT('Ctrl Pts',(-47.9276993204187,-55.0230946822617,
-228.219783397522));
#189593=CARTESIAN_POINT('Ctrl Pts',(-48.0443924842659,-54.5757186289002,
-228.159050207984));
#189594=CARTESIAN_POINT('Ctrl Pts',(-47.9863174736057,-54.8118823401931,
-228.052588015267));
#189595=CARTESIAN_POINT('Ctrl Pts',(-48.0594981945084,-55.0442134699009,
-228.152500861763));
#189596=CARTESIAN_POINT('Ctrl Pts',(-48.3554209171899,-54.6057538752492,
-227.91548473754));
#189597=CARTESIAN_POINT('Ctrl Pts',(-48.2285289945118,-54.8818438998474,
-227.834638886779));
#189598=CARTESIAN_POINT('Ctrl Pts',(-48.3137201093166,-55.1299765132312,
-228.006463242484));
#189599=CARTESIAN_POINT('Ctrl Pts',(-48.4988095574202,-54.650729797923,
-227.78342703208));
#189600=CARTESIAN_POINT('Ctrl Pts',(-48.3367798591397,-54.9456151314884,
-227.716732009813));
#189601=CARTESIAN_POINT('Ctrl Pts',(-48.4371064446681,-55.1945753847142,
-227.927285297474));
#189602=CARTESIAN_POINT('Ctrl Pts',(-48.8101521013542,-54.8085677819245,
-227.459055716783));
#189603=CARTESIAN_POINT('Ctrl Pts',(-48.5612091036401,-55.1417548970017,
-227.432331867016));
#189604=CARTESIAN_POINT('Ctrl Pts',(-48.7169768560648,-55.3833010737937,
-227.732785637971));
#189605=CARTESIAN_POINT('Ctrl Pts',(-48.962196654591,-54.9393505733203,
-227.26705029275));
#189606=CARTESIAN_POINT('Ctrl Pts',(-48.6555172039462,-55.293056012404,
-227.269754320687));
#189607=CARTESIAN_POINT('Ctrl Pts',(-48.8643360818247,-55.5187090833383,
-227.617637443069));
#189608=CARTESIAN_POINT('Ctrl Pts',(-49.0890536832928,-55.1029800540788,
-227.073013622619));
#189609=CARTESIAN_POINT('Ctrl Pts',(-48.7110565412925,-55.4558374114165,
-227.127899351983));
#189610=CARTESIAN_POINT('Ctrl Pts',(-48.9981163054993,-55.6756001905466,
-227.501240761046));
#189611=CARTESIAN_POINT('',(-47.4910910659473,-55.2017568268661,-228.35005));
#189612=CARTESIAN_POINT('',(-47.2343490658922,-54.9709330687352,-228.488381729218));
#189613=CARTESIAN_POINT('Origin',(-47.4910910659474,-55.2017568268662,-228.85005));
#189614=CARTESIAN_POINT('Ctrl Pts',(-47.4910910659473,-55.2017568268661,
-228.35005));
#189615=CARTESIAN_POINT('Ctrl Pts',(-47.5089077383994,-55.1802048283969,
-228.35005));
#189616=CARTESIAN_POINT('Ctrl Pts',(-47.5286070144591,-55.1606954806881,
-228.348498778758));
#189617=CARTESIAN_POINT('Ctrl Pts',(-47.5498778530217,-55.1432566637227,
-228.345450688067));
#189618=CARTESIAN_POINT('Ctrl Pts',(-47.571248428113,-55.1257360781397,
-228.342388305228));
#189619=CARTESIAN_POINT('Ctrl Pts',(-47.5942048306929,-55.1103059835697,
-228.337815232383));
#189620=CARTESIAN_POINT('Ctrl Pts',(-47.6184440641068,-55.0969824475394,
-228.331836254939));
#189621=CARTESIAN_POINT('Ctrl Pts',(-47.6427626834775,-55.0836152755725,
-228.325837695735));
#189622=CARTESIAN_POINT('Ctrl Pts',(-47.6683721101493,-55.0723689149521,
-228.318424429409));
#189623=CARTESIAN_POINT('Ctrl Pts',(-47.694986021396,-55.0632403004126,
-228.309747053101));
#189624=CARTESIAN_POINT('Ctrl Pts',(-47.7218011327211,-55.0540426739213,
-228.301004076183));
#189625=CARTESIAN_POINT('Ctrl Pts',(-47.7496356054836,-55.0469952960427,
-228.29097833533));
#189626=CARTESIAN_POINT('Ctrl Pts',(-47.7782226616637,-55.0420694341252,
-228.279862071304));
#189627=CARTESIAN_POINT('Ctrl Pts',(-47.7866984206837,-55.0406089683005,
-228.276566216897));
#189628=CARTESIAN_POINT('Ctrl Pts',(-47.7952405287646,-55.0393348075036,
-228.273174722161));
#189629=CARTESIAN_POINT('Ctrl Pts',(-47.8038425343185,-55.0382457107992,
-228.269693122561));
#189630=CARTESIAN_POINT('Ctrl Pts',(-47.8373355981116,-55.0340051665251,
-228.256137046974));
#189631=CARTESIAN_POINT('Ctrl Pts',(-47.8714478407728,-55.0324380445811,
-228.241273865974));
#189632=CARTESIAN_POINT('Ctrl Pts',(-47.9058935132037,-55.0332769093997,
-228.225382280215));
#189633=CARTESIAN_POINT('Ctrl Pts',(-47.941344924102,-55.0341402672405,
-228.209026694831));
#189634=CARTESIAN_POINT('Ctrl Pts',(-47.9771500135531,-55.0375516776966,
-228.191582014499));
#189635=CARTESIAN_POINT('Ctrl Pts',(-48.0130258818976,-55.0431915097372,
-228.173311683241));
#189636=CARTESIAN_POINT('Ctrl Pts',(-48.0505695742846,-55.049093530483,
-228.154191987238));
#189637=CARTESIAN_POINT('Ctrl Pts',(-48.0881912505395,-55.0574355196171,
-228.134168324689));
#189638=CARTESIAN_POINT('Ctrl Pts',(-48.1255900814225,-55.0678282154976,
-228.113495063768));
#189639=CARTESIAN_POINT('Ctrl Pts',(-48.1459525590084,-55.0734867088762,
-228.102239128697));
#189640=CARTESIAN_POINT('Ctrl Pts',(-48.166249328711,-55.0797527784695,
-228.09078978545));
#189641=CARTESIAN_POINT('Ctrl Pts',(-48.1864338070466,-55.0865616605034,
-228.079182315661));
#189642=CARTESIAN_POINT('Ctrl Pts',(-48.2254371008043,-55.0997187419852,
-228.056752726625));
#189643=CARTESIAN_POINT('Ctrl Pts',(-48.2640817812442,-55.1149286557663,
-228.03370656281));
#189644=CARTESIAN_POINT('Ctrl Pts',(-48.3022877633549,-55.1319614950397,
-228.010221319788));
#189645=CARTESIAN_POINT('Ctrl Pts',(-48.3417574665396,-55.1495577214256,
-227.985959266568));
#189646=CARTESIAN_POINT('Ctrl Pts',(-48.3807595496667,-55.1690988911915,
-227.961228118431));
#189647=CARTESIAN_POINT('Ctrl Pts',(-48.4191997560302,-55.1903373681973,
-227.936167758128));
#189648=CARTESIAN_POINT('Ctrl Pts',(-48.4593464424128,-55.2125186870885,
-227.909994890682));
#189649=CARTESIAN_POINT('Ctrl Pts',(-48.4988808327079,-55.2365507915592,
-227.883462342538));
#189650=CARTESIAN_POINT('Ctrl Pts',(-48.5376800280217,-55.2621668115556,
-227.856677877223));
#189651=CARTESIAN_POINT('Ctrl Pts',(-48.5429562511707,-55.2656502816791,
-227.853035512612));
#189652=CARTESIAN_POINT('Ctrl Pts',(-48.5482188485838,-55.2691630721293,
-227.849388422952));
#189653=CARTESIAN_POINT('Ctrl Pts',(-48.5534674817022,-55.2727045407243,
-227.845736819723));
#189654=CARTESIAN_POINT('Ctrl Pts',(-48.5900388830808,-55.2973807690938,
-227.820293195764));
#189655=CARTESIAN_POINT('Ctrl Pts',(-48.6257862712802,-55.3233531933449,
-227.794749601736));
#189656=CARTESIAN_POINT('Ctrl Pts',(-48.6607701121414,-55.3505444605623,
-227.769136578206));
#189657=CARTESIAN_POINT('Ctrl Pts',(-48.6963360307854,-55.378188149016,
-227.743097393008));
#189658=CARTESIAN_POINT('Ctrl Pts',(-48.731113046917,-55.4070913174802,
-227.71698545506));
#189659=CARTESIAN_POINT('Ctrl Pts',(-48.765131866684,-55.4372048986578,
-227.690804458223));
#189660=CARTESIAN_POINT('Ctrl Pts',(-48.7994856980231,-55.4676150332795,
-227.664365635366));
#189661=CARTESIAN_POINT('Ctrl Pts',(-48.8330664766557,-55.4992593903386,
-227.637855322385));
#189662=CARTESIAN_POINT('Ctrl Pts',(-48.8658695253829,-55.5321230557835,
-227.611264277926));
#189663=CARTESIAN_POINT('Ctrl Pts',(-48.8704788993216,-55.5367409473793,
-227.607527793908));
#189664=CARTESIAN_POINT('Ctrl Pts',(-48.8750728571358,-55.5413829729072,
-227.603789710314));
#189665=CARTESIAN_POINT('Ctrl Pts',(-48.8796513269546,-55.5460491487752,
-227.60005));
#189666=CARTESIAN_POINT('Ctrl Pts',(-48.9740484537045,-54.9709070690089,
-227.238815650979));
#189667=CARTESIAN_POINT('Ctrl Pts',(-48.8729000175802,-54.8677776014257,
-227.376540018855));
#189668=CARTESIAN_POINT('Ctrl Pts',(-48.7582616773652,-54.7822614512576,
-227.513117602665));
#189669=CARTESIAN_POINT('Ctrl Pts',(-48.4988095574202,-54.650729797923,
-227.78342703208));
#189670=CARTESIAN_POINT('Ctrl Pts',(-48.3554209171899,-54.6057538752492,
-227.91548473754));
#189671=CARTESIAN_POINT('Ctrl Pts',(-48.0443924842659,-54.5757186289002,
-228.159050207984));
#189672=CARTESIAN_POINT('Ctrl Pts',(-47.8754484729887,-54.5910305088289,
-228.271269171667));
#189673=CARTESIAN_POINT('Ctrl Pts',(-47.5351373860507,-54.7135079300998,
-228.438012508273));
#189674=CARTESIAN_POINT('Ctrl Pts',(-47.3678237910099,-54.8223730605885,
-228.488444249231));
#189675=CARTESIAN_POINT('Ctrl Pts',(-47.2343490658922,-54.9709330687352,
-228.488381729218));
#189676=CARTESIAN_POINT('Origin',(-53.1417095267163,-62.031487089538,-218.85005));
#189677=CARTESIAN_POINT('',(-54.6082148364463,-63.3913996516292,-218.35005));
#189678=CARTESIAN_POINT('',(-54.2415885090138,-63.0514215111064,-218.85005));
#189679=CARTESIAN_POINT('Origin',(-54.6082148364463,-63.3913996516292,-218.85005));
#189680=CARTESIAN_POINT('Origin',(-53.1417095267163,-62.031487089538,-218.35005));
#189681=CARTESIAN_POINT('Origin',(-53.1417095267163,-62.031487089538,-218.85005));
#189682=CARTESIAN_POINT('Ctrl Pts',(-47.4910910659474,-55.2017568268662,
-228.35005));
#189683=CARTESIAN_POINT('Ctrl Pts',(-47.3421114593162,-55.0678167910323,
-228.35005));
#189684=CARTESIAN_POINT('Ctrl Pts',(-47.2343490658922,-54.9709330687353,
-228.488381729218));
#189685=CARTESIAN_POINT('Ctrl Pts',(-46.5610878289829,-56.2361862677858,
-228.35005));
#189686=CARTESIAN_POINT('Ctrl Pts',(-46.4160092042075,-56.0984512122452,
-228.350050000212));
#189687=CARTESIAN_POINT('Ctrl Pts',(-46.3105395613661,-55.9991515869664,
-228.487948838892));
#189688=CARTESIAN_POINT('Ctrl Pts',(-45.5947854895852,-57.2325158021754,
-228.35005));
#189689=CARTESIAN_POINT('Ctrl Pts',(-45.4531166269507,-57.091545569762,
-228.350050000038));
#189690=CARTESIAN_POINT('Ctrl Pts',(-45.350506384691,-56.9893433179289,
-228.48772415168));
#189691=CARTESIAN_POINT('Ctrl Pts',(-43.5860475125547,-59.145141081541,
-228.35005));
#189692=CARTESIAN_POINT('Ctrl Pts',(-43.4520711334389,-58.9967304277239,
-228.350049999962));
#189693=CARTESIAN_POINT('Ctrl Pts',(-43.3550620161755,-58.8891661040005,
-228.487824007409));
#189694=CARTESIAN_POINT('Ctrl Pts',(-42.5429028274419,-60.0607223439083,
-228.35005));
#189695=CARTESIAN_POINT('Ctrl Pts',(-42.4124726432155,-59.9088386926303,
-228.35005000027));
#189696=CARTESIAN_POINT('Ctrl Pts',(-42.3185849747264,-59.7984761650306,
-228.488134585451));
#189697=CARTESIAN_POINT('Ctrl Pts',(-41.4636310035132,-60.9383233439605,
-228.35005));
#189698=CARTESIAN_POINT('Ctrl Pts',(-41.3371131727634,-60.7827319875555,
-228.35005));
#189699=CARTESIAN_POINT('Ctrl Pts',(-41.2456587371609,-60.6702615191614,
-228.488620962447));
#189700=CARTESIAN_POINT('',(-41.4636310035131,-60.9383233439604,-228.35005));
#189701=CARTESIAN_POINT('',(-41.2456587371609,-60.6702615191614,-228.488620962447));
#189702=CARTESIAN_POINT('Origin',(-41.4636310035131,-60.9383233439605,-228.85005));
#189703=CARTESIAN_POINT('Ctrl Pts',(-41.4636310035131,-60.9383233439604,
-228.35005));
#189704=CARTESIAN_POINT('Ctrl Pts',(-42.5429085052274,-60.0607177270638,
-228.35005));
#189705=CARTESIAN_POINT('Ctrl Pts',(-43.5860475125577,-59.1451410815382,
-228.35005));
#189706=CARTESIAN_POINT('Ctrl Pts',(-44.5904165010271,-58.1888284418133,
-228.35005));
#189707=CARTESIAN_POINT('Ctrl Pts',(-45.5947854894966,-57.2325158020884,
-228.35005));
#189708=CARTESIAN_POINT('Ctrl Pts',(-46.5610786115705,-56.2361965201832,
-228.35005));
#189709=CARTESIAN_POINT('Ctrl Pts',(-47.4910910659473,-55.2017568268661,
-228.35005));
#189710=CARTESIAN_POINT('Ctrl Pts',(-47.2343490658922,-54.9709330687352,
-228.488381729218));
#189711=CARTESIAN_POINT('Ctrl Pts',(-46.310539561368,-55.9991515869682,
-228.48794883889));
#189712=CARTESIAN_POINT('Ctrl Pts',(-45.3505063846929,-56.9893433179308,
-228.487724151677));
#189713=CARTESIAN_POINT('Ctrl Pts',(-43.3550620161773,-58.8891661040025,
-228.487824007406));
#189714=CARTESIAN_POINT('Ctrl Pts',(-42.3185849747281,-59.7984761650326,
-228.488134585449));
#189715=CARTESIAN_POINT('Ctrl Pts',(-41.2456587371609,-60.6702615191614,
-228.488620962447));
#189716=CARTESIAN_POINT('Origin',(-0.127542579976414,-12.8706479699377,
-218.85005));
#189717=CARTESIAN_POINT('',(-49.6055526500885,-68.3000311480131,-218.35005));
#189718=CARTESIAN_POINT('',(-49.2725916132775,-67.9270204940557,-218.85005));
#189719=CARTESIAN_POINT('Origin',(-49.6055526500885,-68.3000311480131,-218.85005));
#189720=CARTESIAN_POINT('Origin',(-0.127542579976414,-12.8706479699377,
-218.35005));
#189721=CARTESIAN_POINT('Origin',(-0.127542579976414,-12.8706479699377,
-218.85005));
#189722=CARTESIAN_POINT('Ctrl Pts',(-41.3169485390149,-62.5017525488808,
-227.074161006174));
#189723=CARTESIAN_POINT('Ctrl Pts',(-41.6737883368886,-62.1442676134989,
-227.135099137228));
#189724=CARTESIAN_POINT('Ctrl Pts',(-41.8830720182286,-62.4278907679969,
-227.501554844865));
#189725=CARTESIAN_POINT('Ctrl Pts',(-41.1560049633168,-62.3716221357798,
-227.26702335738));
#189726=CARTESIAN_POINT('Ctrl Pts',(-41.511713989187,-62.0831419564948,
-227.276651470545));
#189727=CARTESIAN_POINT('Ctrl Pts',(-41.7288940022276,-62.291150852776,
-227.617227833887));
#189728=CARTESIAN_POINT('Ctrl Pts',(-41.0290389449415,-62.2181773292494,
-227.457737962392));
#189729=CARTESIAN_POINT('Ctrl Pts',(-41.36324217846,-61.9848792214323,-227.438029208627));
#189730=CARTESIAN_POINT('Ctrl Pts',(-41.5972134010529,-62.1423580722077,
-227.731615003921));
#189731=CARTESIAN_POINT('Ctrl Pts',(-40.8795052413922,-61.9086867290375,
-227.779669319346));
#189732=CARTESIAN_POINT('Ctrl Pts',(-41.1743549655657,-61.7587852725776,
-227.719332117853));
#189733=CARTESIAN_POINT('Ctrl Pts',(-41.4166557380291,-61.8634089393353,
-227.924695300817));
#189734=CARTESIAN_POINT('Ctrl Pts',(-40.83755717967,-61.7643747830512,-227.9134383294));
#189735=CARTESIAN_POINT('Ctrl Pts',(-41.1129123325295,-61.6488546563462,
-227.83820193251));
#189736=CARTESIAN_POINT('Ctrl Pts',(-41.3546304032729,-61.7388485235333,
-228.004924872379));
#189737=CARTESIAN_POINT('Ctrl Pts',(-40.8167874720303,-61.4561982274081,
-228.157939415417));
#189738=CARTESIAN_POINT('Ctrl Pts',(-41.0510076565582,-61.4074592210291,
-228.055814452642));
#189739=CARTESIAN_POINT('Ctrl Pts',(-41.2770779346333,-61.4865010709279,
-228.151579714695));
#189740=CARTESIAN_POINT('Ctrl Pts',(-40.8377574579089,-61.2894729474496,
-228.270955921441));
#189741=CARTESIAN_POINT('Ctrl Pts',(-41.0474958312304,-61.2728289507257,
-228.158745887246));
#189742=CARTESIAN_POINT('Ctrl Pts',(-41.2608207422257,-61.3563705227572,
-228.219373496776));
#189743=CARTESIAN_POINT('Ctrl Pts',(-41.0018595517499,-60.8897708053906,
-228.472378638458));
#189744=CARTESIAN_POINT('Ctrl Pts',(-41.1456365144707,-60.9545865414107,
-228.33766271302));
#189745=CARTESIAN_POINT('Ctrl Pts',(-41.312673756006,-61.0669702905819,
-228.340237378046));
#189746=CARTESIAN_POINT('Ctrl Pts',(-41.1915219835726,-60.6688302795396,
-228.523150593266));
#189747=CARTESIAN_POINT('Ctrl Pts',(-41.2921564536673,-60.7745584980989,
-228.383687823478));
#189748=CARTESIAN_POINT('Ctrl Pts',(-41.4201823771292,-60.9267119894641,
-228.37074419579));
#189749=CARTESIAN_POINT('Ctrl Pts',(-41.4493760765003,-60.5376437416951,
-228.463541011148));
#189750=CARTESIAN_POINT('Ctrl Pts',(-41.5006225893106,-60.6869549447557,
-228.322209460736));
#189751=CARTESIAN_POINT('Ctrl Pts',(-41.6002487944716,-60.8719910741376,
-228.335067908123));
#189752=CARTESIAN_POINT('',(-41.7563078823353,-62.3074742642099,-227.60005));
#189753=CARTESIAN_POINT('',(-41.1874522920715,-62.3844144545142,-227.238927571877));
#189754=CARTESIAN_POINT('Origin',(-41.3994163116703,-62.6576576544332,-227.60005));
#189755=CARTESIAN_POINT('Ctrl Pts',(-41.7563078823353,-62.3074742642099,
-227.60005));
#189756=CARTESIAN_POINT('Ctrl Pts',(-41.7235734346169,-62.2741127491088,
-227.626724054627));
#189757=CARTESIAN_POINT('Ctrl Pts',(-41.6921357158834,-62.2400471989624,
-227.653311433456));
#189758=CARTESIAN_POINT('Ctrl Pts',(-41.6620056207862,-62.2052910952259,
-227.67982091917));
#189759=CARTESIAN_POINT('Ctrl Pts',(-41.6307102746536,-62.1691908342363,
-227.707355632504));
#189760=CARTESIAN_POINT('Ctrl Pts',(-41.6008254854847,-62.1323457352978,
-227.73480764522));
#189761=CARTESIAN_POINT('Ctrl Pts',(-41.5724052856148,-62.0947298672639,
-227.762174519856));
#189762=CARTESIAN_POINT('Ctrl Pts',(-41.5459110186549,-62.0596630889099,
-227.787686841577));
#189763=CARTESIAN_POINT('Ctrl Pts',(-41.5206901179788,-62.0239259257339,
-227.81312595281));
#189764=CARTESIAN_POINT('Ctrl Pts',(-41.4968179503685,-61.9874663713984,
-227.838464695241));
#189765=CARTESIAN_POINT('Ctrl Pts',(-41.4950826242579,-61.9848160374341,
-227.840306630254));
#189766=CARTESIAN_POINT('Ctrl Pts',(-41.4933544377594,-61.9821618738057,
-227.842148020231));
#189767=CARTESIAN_POINT('Ctrl Pts',(-41.4916334256868,-61.9795038547827,
-227.843988847451));
#189768=CARTESIAN_POINT('Ctrl Pts',(-41.4653523060016,-61.9389139500517,
-227.872099632527));
#189769=CARTESIAN_POINT('Ctrl Pts',(-41.4406731366018,-61.8973165619484,
-227.900153206132));
#189770=CARTESIAN_POINT('Ctrl Pts',(-41.4180385765043,-61.8549835530777,
-227.927912489062));
#189771=CARTESIAN_POINT('Ctrl Pts',(-41.3964658547037,-61.8146364811921,
-227.954369521382));
#189772=CARTESIAN_POINT('Ctrl Pts',(-41.3767507922726,-61.7736208112622,
-227.980559137109));
#189773=CARTESIAN_POINT('Ctrl Pts',(-41.359264822195,-61.7321834942838,
-228.006233157985));
#189774=CARTESIAN_POINT('Ctrl Pts',(-41.3425707322791,-61.6926227325739,
-228.030744489705));
#189775=CARTESIAN_POINT('Ctrl Pts',(-41.3279087531751,-61.652677312538,
-228.05478569363));
#189776=CARTESIAN_POINT('Ctrl Pts',(-41.3155859261546,-61.6125780064951,
-228.078102621503));
#189777=CARTESIAN_POINT('Ctrl Pts',(-41.3044314784935,-61.5762806852913,
-228.099208772807));
#189778=CARTESIAN_POINT('Ctrl Pts',(-41.2951200838481,-61.5396758565221,
-228.119813195706));
#189779=CARTESIAN_POINT('Ctrl Pts',(-41.2880440076531,-61.5030587469111,
-228.13969080728));
#189780=CARTESIAN_POINT('Ctrl Pts',(-41.2811808243614,-61.4675433103978,
-228.158970375204));
#189781=CARTESIAN_POINT('Ctrl Pts',(-41.2764209319513,-61.4320158754815,
-228.177566170525));
#189782=CARTESIAN_POINT('Ctrl Pts',(-41.2741059440455,-61.3967618102316,
-228.195230844135));
#189783=CARTESIAN_POINT('Ctrl Pts',(-41.2718932011152,-61.3630647945998,
-228.212115330464));
#189784=CARTESIAN_POINT('Ctrl Pts',(-41.2719145388887,-61.3296171684738,
-228.228148884212));
#189785=CARTESIAN_POINT('Ctrl Pts',(-41.2744473106528,-61.2966887064693,
-228.243078764507));
#189786=CARTESIAN_POINT('Ctrl Pts',(-41.2760291667021,-61.2761230607388,
-228.252403300493));
#189787=CARTESIAN_POINT('Ctrl Pts',(-41.2785902266755,-61.2557603463957,
-228.261296602549));
#189788=CARTESIAN_POINT('Ctrl Pts',(-41.2821925706481,-61.2356716714283,
-228.269690042848));
#189789=CARTESIAN_POINT('Ctrl Pts',(-41.2875991018068,-61.2055218445455,
-228.282287228693));
#189790=CARTESIAN_POINT('Ctrl Pts',(-41.2954370433597,-61.1763140509013,
-228.293669306206));
#189791=CARTESIAN_POINT('Ctrl Pts',(-41.3057207923416,-61.1483324005503,
-228.303616281046));
#189792=CARTESIAN_POINT('Ctrl Pts',(-41.3155679856567,-61.1215385998879,
-228.313140996627));
#189793=CARTESIAN_POINT('Ctrl Pts',(-41.3276572099933,-61.0958695700185,
-228.321349528454));
#189794=CARTESIAN_POINT('Ctrl Pts',(-41.3419742882173,-61.0716010662815,
-228.328085190812));
#189795=CARTESIAN_POINT('Ctrl Pts',(-41.3562413419726,-61.0474173577093,
-228.334797318485));
#189796=CARTESIAN_POINT('Ctrl Pts',(-41.372720286929,-61.0246248189081,
-228.340046421585));
#189797=CARTESIAN_POINT('Ctrl Pts',(-41.3913766316035,-61.0035164026252,
-228.343720453028));
#189798=CARTESIAN_POINT('Ctrl Pts',(-41.4099793999867,-60.9824686043616,
-228.347383933585));
#189799=CARTESIAN_POINT('Ctrl Pts',(-41.430746593826,-60.9630957469574,
-228.349481090787));
#189800=CARTESIAN_POINT('Ctrl Pts',(-41.4536304454056,-60.9457015839643,
-228.349949039638));
#189801=CARTESIAN_POINT('Ctrl Pts',(-41.4569202857835,-60.9432009551014,
-228.350016313148));
#189802=CARTESIAN_POINT('Ctrl Pts',(-41.4602538570071,-60.9407412364663,
-228.35005));
#189803=CARTESIAN_POINT('Ctrl Pts',(-41.4636310035131,-60.9383233439604,
-228.35005));
#189804=CARTESIAN_POINT('Ctrl Pts',(-41.2456587371609,-60.6702615191614,
-228.488620962447));
#189805=CARTESIAN_POINT('Ctrl Pts',(-41.0908117131772,-60.7960794826395,
-228.488691139081));
#189806=CARTESIAN_POINT('Ctrl Pts',(-40.9745092027764,-60.9563878290671,
-228.438808185622));
#189807=CARTESIAN_POINT('Ctrl Pts',(-40.8377574579089,-61.2894729474496,
-228.270955921441));
#189808=CARTESIAN_POINT('Ctrl Pts',(-40.8167874720303,-61.4561982274081,
-228.157939415417));
#189809=CARTESIAN_POINT('Ctrl Pts',(-40.83755717967,-61.7643747830512,-227.9134383294));
#189810=CARTESIAN_POINT('Ctrl Pts',(-40.8795052413922,-61.9086867290375,
-227.779669319346));
#189811=CARTESIAN_POINT('Ctrl Pts',(-41.0041166610166,-62.1665955625474,
-227.511393188551));
#189812=CARTESIAN_POINT('Ctrl Pts',(-41.0866968731953,-62.2817278482174,
-227.375764657105));
#189813=CARTESIAN_POINT('Ctrl Pts',(-41.1874522920715,-62.3844144545142,
-227.238927571877));
#189814=CARTESIAN_POINT('Origin',(-48.2737085028446,-66.8079885321834,-218.85005));
#189815=CARTESIAN_POINT('',(-49.0417551583074,-68.6546353135231,-218.35005));
#189816=CARTESIAN_POINT('',(-48.8497434944417,-68.1929736181882,-218.85005));
#189817=CARTESIAN_POINT('Origin',(-49.0417551583074,-68.6546353135231,-218.85005));
#189818=CARTESIAN_POINT('Origin',(-48.2737085028446,-66.8079885321834,-218.35005));
#189819=CARTESIAN_POINT('Origin',(-48.2737085028446,-66.8079885321834,-218.85005));
#189820=CARTESIAN_POINT('Ctrl Pts',(-41.7563078823354,-62.3074742642099,
-227.60005));
#189821=CARTESIAN_POINT('Ctrl Pts',(-41.533590072875,-62.0804900295131,
-227.265723268608));
#189822=CARTESIAN_POINT('Ctrl Pts',(-41.1874522920715,-62.3844144545142,
-227.238927571877));
#189823=CARTESIAN_POINT('Ctrl Pts',(-43.5663090949841,-64.1521482085568,
-225.141881592783));
#189824=CARTESIAN_POINT('Ctrl Pts',(-43.3439332486946,-63.9255124877361,
-224.807072796208));
#189825=CARTESIAN_POINT('Ctrl Pts',(-42.9977586927641,-64.2294190860942,
-224.780329817623));
#189826=CARTESIAN_POINT('Ctrl Pts',(-45.3784193710744,-65.9989716179707,
-222.686835360681));
#189827=CARTESIAN_POINT('Ctrl Pts',(-45.1633560000594,-65.7797884513162,
-222.341036594742));
#189828=CARTESIAN_POINT('Ctrl Pts',(-44.8096404055398,-66.0773673148437,
-222.324535970207));
#189829=CARTESIAN_POINT('Ctrl Pts',(-47.2030337908495,-67.8585387028531,
-220.250747695207));
#189830=CARTESIAN_POINT('Ctrl Pts',(-46.9799636370447,-67.6311953742356,
-219.91012892279));
#189831=CARTESIAN_POINT('Ctrl Pts',(-46.6323854374629,-67.9411854921914,
-219.886423382228));
#189832=CARTESIAN_POINT('',(-47.2030337908494,-67.858538702853,-220.250747695207));
#189833=CARTESIAN_POINT('',(-46.6323854374629,-67.9411854921913,-219.886423382228));
#189834=CARTESIAN_POINT('Origin',(-46.8461422201844,-68.2087220930763,-220.250747695207));
#189835=CARTESIAN_POINT('Ctrl Pts',(-47.2030337908494,-67.858538702853,
-220.250747695207));
#189836=CARTESIAN_POINT('Ctrl Pts',(-45.378411470404,-65.9989635659536,
-222.68684590906));
#189837=CARTESIAN_POINT('Ctrl Pts',(-43.5663164045416,-64.1521556581376,
-225.14187166565));
#189838=CARTESIAN_POINT('Ctrl Pts',(-41.7563078823354,-62.3074742642099,
-227.60005));
#189839=CARTESIAN_POINT('Ctrl Pts',(-41.1874522920715,-62.3844144545142,
-227.238927571877));
#189840=CARTESIAN_POINT('Ctrl Pts',(-42.9977586927641,-64.2294190860942,
-224.780329817623));
#189841=CARTESIAN_POINT('Ctrl Pts',(-44.8096404055398,-66.0773673148437,
-222.324535970207));
#189842=CARTESIAN_POINT('Ctrl Pts',(-46.6323854374629,-67.9411854921913,
-219.886423382228));
#189843=CARTESIAN_POINT('Ctrl Pts',(-49.0417551583074,-68.6546353135231,
-218.35005));
#189844=CARTESIAN_POINT('Ctrl Pts',(-48.8497434944417,-68.1929736181882,
-218.35005));
#189845=CARTESIAN_POINT('Ctrl Pts',(-48.8497434944417,-68.1929736181882,
-218.85005));
#189846=CARTESIAN_POINT('Ctrl Pts',(-48.8914370751605,-68.6805168842225,
-218.35005));
#189847=CARTESIAN_POINT('Ctrl Pts',(-48.7557592223196,-68.232063046543,
-218.382837715704));
#189848=CARTESIAN_POINT('Ctrl Pts',(-48.7287312757308,-68.2433043207298,
-218.85004996112));
#189849=CARTESIAN_POINT('Ctrl Pts',(-48.7342750095003,-68.6918682705249,
-218.342169793108));
#189850=CARTESIAN_POINT('Ctrl Pts',(-48.6402644556944,-68.2689304282727,
-218.402170544444));
#189851=CARTESIAN_POINT('Ctrl Pts',(-48.6040131804169,-68.2768832027127,
-218.836912439222));
#189852=CARTESIAN_POINT('Ctrl Pts',(-48.5701931618903,-68.6892604152372,
-218.333619302448));
#189853=CARTESIAN_POINT('Ctrl Pts',(-48.5093251395215,-68.2897551158004,
-218.412348259396));
#189854=CARTESIAN_POINT('Ctrl Pts',(-48.4757604447939,-68.2943179077776,
-218.82266550408));
#189855=CARTESIAN_POINT('',(-48.5701931618903,-68.6892604152372,-218.333619302448));
#189856=CARTESIAN_POINT('',(-48.4757604447939,-68.2943179077777,-218.82266550408));
#189857=CARTESIAN_POINT('Origin',(-48.5431110921104,-68.7897610329756,-218.82266550408));
#189858=CARTESIAN_POINT('Ctrl Pts',(-48.5701931618903,-68.6892604152372,
-218.333619302448));
#189859=CARTESIAN_POINT('Ctrl Pts',(-48.7342750095003,-68.6918682705249,
-218.342169793108));
#189860=CARTESIAN_POINT('Ctrl Pts',(-48.8914370751605,-68.6805168842225,
-218.35005));
#189861=CARTESIAN_POINT('Ctrl Pts',(-49.0417551583074,-68.6546353135231,
-218.35005));
#189862=CARTESIAN_POINT('Ctrl Pts',(-48.8497434944417,-68.1929736181882,
-218.85005));
#189863=CARTESIAN_POINT('Ctrl Pts',(-48.7287312757308,-68.2433043207298,
-218.85004996112));
#189864=CARTESIAN_POINT('Ctrl Pts',(-48.6040131804169,-68.2768832027127,
-218.836912439222));
#189865=CARTESIAN_POINT('Ctrl Pts',(-48.4757604447939,-68.2943179077777,
-218.82266550408));
#189866=CARTESIAN_POINT('Ctrl Pts',(-48.3245605310988,-68.5271120961852,
-218.457629631481));
#189867=CARTESIAN_POINT('Ctrl Pts',(-48.3620966736425,-68.3097367575389,
-218.591561281049));
#189868=CARTESIAN_POINT('Ctrl Pts',(-48.4757880438389,-68.2943141599182,
-218.822721620273));
#189869=CARTESIAN_POINT('Ctrl Pts',(-47.9776226084146,-68.5733796207044,
-218.632054575151));
#189870=CARTESIAN_POINT('Ctrl Pts',(-48.0565913810317,-68.3304993120465,
-218.760316454659));
#189871=CARTESIAN_POINT('Ctrl Pts',(-48.2145407189483,-68.3298331219756,
-218.997206525336));
#189872=CARTESIAN_POINT('Ctrl Pts',(-47.649067081485,-68.5245197011584,
-218.86174158345));
#189873=CARTESIAN_POINT('Ctrl Pts',(-47.775376539589,-68.2571434268353,
-218.980794630082));
#189874=CARTESIAN_POINT('Ctrl Pts',(-47.9672967132033,-68.2939483901744,
-219.226826228492));
#189875=CARTESIAN_POINT('Ctrl Pts',(-47.0472977798015,-68.2996159355387,
-219.380401121619));
#189876=CARTESIAN_POINT('Ctrl Pts',(-47.2783353223672,-67.9981939744083,
-219.464723226566));
#189877=CARTESIAN_POINT('Ctrl Pts',(-47.5147244105,-68.1266034179018,-219.745199430154));
#189878=CARTESIAN_POINT('Ctrl Pts',(-46.777719874766,-68.1088664499766,
-219.677867280655));
#189879=CARTESIAN_POINT('Ctrl Pts',(-47.0707096179741,-67.7884048023075,
-219.740938168961));
#189880=CARTESIAN_POINT('Ctrl Pts',(-47.3121561538429,-67.9841014827788,
-220.042431566437));
#189881=CARTESIAN_POINT('Ctrl Pts',(-46.5633692293693,-67.867058771901,
-219.981377366936));
#189882=CARTESIAN_POINT('Ctrl Pts',(-46.9321463856559,-67.5557234715507,
-219.993833370428));
#189883=CARTESIAN_POINT('Ctrl Pts',(-47.1512692652038,-67.8031102433352,
-220.345690853212));
#189884=CARTESIAN_POINT('',(-48.3245605310987,-68.5271120961857,-218.45762963148));
#189885=CARTESIAN_POINT('Origin',(-48.5431110921103,-68.7897610329758,-218.82266550408));
#189886=CARTESIAN_POINT('',(-48.2737085028434,-68.3079885321834,-218.970433100048));
#189887=CARTESIAN_POINT('Origin',(-48.3025662442039,-65.8964824566508,-221.193464878497));
#189888=CARTESIAN_POINT('Ctrl Pts',(-48.2737085028434,-68.3079885321834,
-218.970433100048));
#189889=CARTESIAN_POINT('Ctrl Pts',(-48.2200078753576,-68.3079885321833,
-219.013078180332));
#189890=CARTESIAN_POINT('Ctrl Pts',(-48.1671265874068,-68.3051041946007,
-219.057745077571));
#189891=CARTESIAN_POINT('Ctrl Pts',(-48.1153121427422,-68.2996019516411,
-219.104050254264));
#189892=CARTESIAN_POINT('Ctrl Pts',(-48.0624290103477,-68.2939862233479,
-219.15131048846));
#189893=CARTESIAN_POINT('Ctrl Pts',(-48.0106569899895,-68.2856439945604,
-219.200277279003));
#189894=CARTESIAN_POINT('Ctrl Pts',(-47.9602041194346,-68.274861056155,
-219.250542863839));
#189895=CARTESIAN_POINT('Ctrl Pts',(-47.9081697144589,-68.2637401074826,
-219.302384112294));
#189896=CARTESIAN_POINT('Ctrl Pts',(-47.857538280142,-68.2500235216982,
-219.355606857271));
#189897=CARTESIAN_POINT('Ctrl Pts',(-47.8084827582267,-68.2340197403078,
-219.409763776065));
#189898=CARTESIAN_POINT('Ctrl Pts',(-47.7899076849436,-68.2279598432661,
-219.430270514066));
#189899=CARTESIAN_POINT('Ctrl Pts',(-47.7715580265398,-68.2215719219543,
-219.450911192888));
#189900=CARTESIAN_POINT('Ctrl Pts',(-47.7534412888826,-68.2148723319608,
-219.471661526933));
#189901=CARTESIAN_POINT('Ctrl Pts',(-47.7036959697479,-68.1964764569085,
-219.528638230396));
#189902=CARTESIAN_POINT('Ctrl Pts',(-47.6555204296105,-68.1756653808065,
-219.586645968365));
#189903=CARTESIAN_POINT('Ctrl Pts',(-47.6089704551965,-68.1526532963566,
-219.645524393526));
#189904=CARTESIAN_POINT('Ctrl Pts',(-47.5600388327744,-68.1284638388622,
-219.707415230311));
#189905=CARTESIAN_POINT('Ctrl Pts',(-47.5129023330372,-68.1018424910022,
-219.770268127841));
#189906=CARTESIAN_POINT('Ctrl Pts',(-47.4676123806305,-68.0729822245595,
-219.833896846445));
#189907=CARTESIAN_POINT('Ctrl Pts',(-47.4192068535602,-68.0421366101503,
-219.901902695363));
#189908=CARTESIAN_POINT('Ctrl Pts',(-47.3729092787754,-68.008733452613,
-219.97079477694));
#189909=CARTESIAN_POINT('Ctrl Pts',(-47.3287869283299,-67.9729448481097,
-220.040345711594));
#189910=CARTESIAN_POINT('Ctrl Pts',(-47.2846645778844,-67.9371562436065,
-220.109896646248));
#189911=CARTESIAN_POINT('Ctrl Pts',(-47.242716187926,-67.8989812635678,
-220.18010643398));
#189912=CARTESIAN_POINT('Ctrl Pts',(-47.2030337908494,-67.858538702853,
-220.250747695207));
#189913=CARTESIAN_POINT('Ctrl Pts',(-46.6323854374629,-67.9411854921913,
-219.886423382228));
#189914=CARTESIAN_POINT('Ctrl Pts',(-46.8345979831289,-68.1479546277646,
-219.615942902677));
#189915=CARTESIAN_POINT('Ctrl Pts',(-47.0804817541895,-68.3120180317859,
-219.351800153137));
#189916=CARTESIAN_POINT('Ctrl Pts',(-47.649067081485,-68.5245197011584,
-218.86174158345));
#189917=CARTESIAN_POINT('Ctrl Pts',(-47.9776226084146,-68.5733796207044,
-218.632054575151));
#189918=CARTESIAN_POINT('Ctrl Pts',(-48.3245605310987,-68.5271120961857,
-218.45762963148));
#189919=CARTESIAN_POINT('Origin',(-48.5431110921103,-68.7897610329758,-218.82266550408));
#189920=CARTESIAN_POINT('Origin',(-48.5431110921103,-68.7897610329758,-218.82266550408));
#189921=CARTESIAN_POINT('Ctrl Pts',(-49.9821530185534,29.7903768266301,
-227.087737588405));
#189922=CARTESIAN_POINT('Ctrl Pts',(-49.6198764783311,30.1429190036325,
-227.149984230661));
#189923=CARTESIAN_POINT('Ctrl Pts',(-49.9128620056376,30.3690936660469,
-227.499383229701));
#189924=CARTESIAN_POINT('Ctrl Pts',(-49.8651657433229,29.6382362842524,
-227.284518486594));
#189925=CARTESIAN_POINT('Ctrl Pts',(-49.5705461543588,29.9918313989471,
-227.291056067445));
#189926=CARTESIAN_POINT('Ctrl Pts',(-49.7889944489624,30.2238041797745,
-227.61742149242));
#189927=CARTESIAN_POINT('Ctrl Pts',(-49.7229062924001,29.5201055635575,
-227.47950311892));
#189928=CARTESIAN_POINT('Ctrl Pts',(-49.4843813968511,29.8539883550855,
-227.45309706292));
#189929=CARTESIAN_POINT('Ctrl Pts',(-49.6516188678455,30.100801435488,-227.73438694973));
#189930=CARTESIAN_POINT('Ctrl Pts',(-49.4273244905926,29.3876439546323,
-227.809457307428));
#189931=CARTESIAN_POINT('Ctrl Pts',(-49.274698524826,29.6835679295866,-227.737356551705));
#189932=CARTESIAN_POINT('Ctrl Pts',(-49.3886234115437,29.9359477677008,
-227.932297012233));
#189933=CARTESIAN_POINT('Ctrl Pts',(-49.2917843161281,29.3546860495185,
-227.942284411928));
#189934=CARTESIAN_POINT('Ctrl Pts',(-49.1736791703851,29.6317476033538,
-227.854117706657));
#189935=CARTESIAN_POINT('Ctrl Pts',(-49.2735381356863,29.8826576832388,
-228.011965974601));
#189936=CARTESIAN_POINT('Ctrl Pts',(-49.0688864384257,29.3512758295993,
-228.126445026147));
#189937=CARTESIAN_POINT('Ctrl Pts',(-49.0005354215612,29.5971993197923,
-228.017792073831));
#189938=CARTESIAN_POINT('Ctrl Pts',(-49.094353778077,29.8357918748608,-228.122426020868));
#189939=CARTESIAN_POINT('Ctrl Pts',(-48.9919998081944,29.3580678656198,
-228.184587230454));
#189940=CARTESIAN_POINT('Ctrl Pts',(-48.9405355047191,29.5928733395382,
-228.06937023996));
#189941=CARTESIAN_POINT('Ctrl Pts',(-49.034125806983,29.8260226021538,-228.157300396488));
#189942=CARTESIAN_POINT('Ctrl Pts',(-48.8359253199892,29.3900316449823,
-228.290207259017));
#189943=CARTESIAN_POINT('Ctrl Pts',(-48.8180798673065,29.6014212406182,
-228.162864494856));
#189944=CARTESIAN_POINT('Ctrl Pts',(-48.9154714515405,29.8207826964393,
-228.220654439149));
#189945=CARTESIAN_POINT('Ctrl Pts',(-48.7550774165302,29.4157509526954,
-228.33866597543));
#189946=CARTESIAN_POINT('Ctrl Pts',(-48.7540839008066,29.6143499072788,
-228.205991351778));
#189947=CARTESIAN_POINT('Ctrl Pts',(-48.8558242941532,29.8254233230326,
-228.249722296701));
#189948=CARTESIAN_POINT('Ctrl Pts',(-48.4543941551331,29.5520514607806,
-228.490868066449));
#189949=CARTESIAN_POINT('Ctrl Pts',(-48.5190268257732,29.6989473079643,
-228.339039615738));
#189950=CARTESIAN_POINT('Ctrl Pts',(-48.6420470598464,29.8753114465513,
-228.341027466389));
#189951=CARTESIAN_POINT('Ctrl Pts',(-48.2384142358766,29.739665517712,-228.538258948111));
#189952=CARTESIAN_POINT('Ctrl Pts',(-48.3453525961707,29.8434973019672,
-228.381204030932));
#189953=CARTESIAN_POINT('Ctrl Pts',(-48.5063911947406,29.9830169918788,
-228.369471344765));
#189954=CARTESIAN_POINT('Ctrl Pts',(-48.1067814994714,29.9754013777531,
-228.482341346825));
#189955=CARTESIAN_POINT('Ctrl Pts',(-48.2558206399642,30.0319935302987,
-228.324194018));
#189956=CARTESIAN_POINT('Ctrl Pts',(-48.4474782994608,30.1465062177761,
-228.335958788446));
#189957=CARTESIAN_POINT('',(-48.2384287873563,29.7860380279371,-228.505869818703));
#189958=CARTESIAN_POINT('',(-48.515339402069,30.020261242545,-228.35005));
#189959=CARTESIAN_POINT('Origin',(-48.515339402069,30.020261242545,-228.85005));
#189960=CARTESIAN_POINT('',(-49.8755750290351,29.6684593880862,-227.255950349386));
#189961=CARTESIAN_POINT('Ctrl Pts',(-48.2384287873563,29.7860380279371,
-228.505869818703));
#189962=CARTESIAN_POINT('Ctrl Pts',(-48.3622865299896,29.6395743915966,
-228.505892074711));
#189963=CARTESIAN_POINT('Ctrl Pts',(-48.5176958943746,29.5233566169732,
-228.458825520971));
#189964=CARTESIAN_POINT('Ctrl Pts',(-48.7550774165302,29.4157509526954,
-228.33866597543));
#189965=CARTESIAN_POINT('Ctrl Pts',(-48.8359253199892,29.3900316449823,
-228.290207259017));
#189966=CARTESIAN_POINT('Ctrl Pts',(-48.9919998081944,29.3580678656198,
-228.184587230454));
#189967=CARTESIAN_POINT('Ctrl Pts',(-49.0688864384257,29.3512758295993,
-228.126445026147));
#189968=CARTESIAN_POINT('Ctrl Pts',(-49.2917843161281,29.3546860495185,
-227.942284411928));
#189969=CARTESIAN_POINT('Ctrl Pts',(-49.4273244905926,29.3876439546323,
-227.809457307428));
#189970=CARTESIAN_POINT('Ctrl Pts',(-49.6736426587655,29.4980286287366,
-227.534495483671));
#189971=CARTESIAN_POINT('Ctrl Pts',(-49.7814123210161,29.5740686437592,
-227.395733267867));
#189972=CARTESIAN_POINT('Ctrl Pts',(-49.8755750290351,29.6684593880862,
-227.255950349386));
#189973=CARTESIAN_POINT('',(-49.8031531494471,30.2499539750197,-227.60005));
#189974=CARTESIAN_POINT('Origin',(-50.1572979707234,29.8969930061248,-227.60005));
#189975=CARTESIAN_POINT('Ctrl Pts',(-49.8031531494471,30.2499539750196,
-227.60005));
#189976=CARTESIAN_POINT('Ctrl Pts',(-49.7734448823229,30.2201460645754,
-227.626521883971));
#189977=CARTESIAN_POINT('Ctrl Pts',(-49.7429857046469,30.191563965602,-227.652920536918));
#189978=CARTESIAN_POINT('Ctrl Pts',(-49.7117854125283,30.1642213555141,
-227.679257545219));
#189979=CARTESIAN_POINT('Ctrl Pts',(-49.6808651108338,30.137124117135,-227.70535820605));
#189980=CARTESIAN_POINT('Ctrl Pts',(-49.6492168074017,30.1112443498472,
-227.731399362287));
#189981=CARTESIAN_POINT('Ctrl Pts',(-49.6168148938523,30.0866303917786,
-227.757381347539));
#189982=CARTESIAN_POINT('Ctrl Pts',(-49.5852289197423,30.0626362581879,
-227.782709058886));
#189983=CARTESIAN_POINT('Ctrl Pts',(-49.5529265342257,30.0398452627543,
-227.807981431008));
#189984=CARTESIAN_POINT('Ctrl Pts',(-49.5198536003906,30.0183324962131,
-227.833174321558));
#189985=CARTESIAN_POINT('Ctrl Pts',(-49.5126382797592,30.0136391869035,
-227.838670501119));
#189986=CARTESIAN_POINT('Ctrl Pts',(-49.5053861763458,30.0090068233215,
-227.844162774479));
#189987=CARTESIAN_POINT('Ctrl Pts',(-49.4980965508085,30.0044363617929,
-227.849650666463));
#189988=CARTESIAN_POINT('Ctrl Pts',(-49.4649798247165,29.9836727818563,
-227.874582127582));
#189989=CARTESIAN_POINT('Ctrl Pts',(-49.4313422743447,29.9643338165172,
-227.899219369963));
#189990=CARTESIAN_POINT('Ctrl Pts',(-49.3972404504349,29.9465778326619,
-227.923525661612));
#189991=CARTESIAN_POINT('Ctrl Pts',(-49.3639866371966,29.929263387178,-227.947227528266));
#189992=CARTESIAN_POINT('Ctrl Pts',(-49.3302909420142,29.9134545841207,
-227.970615436086));
#189993=CARTESIAN_POINT('Ctrl Pts',(-49.2961839213851,29.8993200737892,
-227.993617660293));
#189994=CARTESIAN_POINT('Ctrl Pts',(-49.2635064665614,29.8857779990406,
-228.01565576648));
#189995=CARTESIAN_POINT('Ctrl Pts',(-49.2304509638959,29.8737732842517,
-228.0373403047));
#189996=CARTESIAN_POINT('Ctrl Pts',(-49.1970304416516,29.8634680481683,
-228.058564819369));
#189997=CARTESIAN_POINT('Ctrl Pts',(-49.1827533566865,29.8590657013087,
-228.067631829067));
#189998=CARTESIAN_POINT('Ctrl Pts',(-49.1684095214318,29.8549736373304,
-228.076614292399));
#189999=CARTESIAN_POINT('Ctrl Pts',(-49.1539994837212,29.8512049615201,
-228.085501029504));
#190000=CARTESIAN_POINT('Ctrl Pts',(-49.1169547854528,29.8415166136428,
-228.10834666678));
#190001=CARTESIAN_POINT('Ctrl Pts',(-49.0797216134608,29.834075936904,-228.130440543945));
#190002=CARTESIAN_POINT('Ctrl Pts',(-49.0426240763788,29.8292022975051,
-228.151491221325));
#190003=CARTESIAN_POINT('Ctrl Pts',(-49.0199091815933,29.8262181585332,
-228.164380592412));
#190004=CARTESIAN_POINT('Ctrl Pts',(-48.9972457051912,29.8241958719105,
-228.176878325889));
#190005=CARTESIAN_POINT('Ctrl Pts',(-48.9747142044139,29.8232026173048,
-228.188913138851));
#190006=CARTESIAN_POINT('Ctrl Pts',(-48.9493717776647,29.822085448842,-228.202449359493));
#190007=CARTESIAN_POINT('Ctrl Pts',(-48.9239814908925,29.8222824170942,
-228.215521988452));
#190008=CARTESIAN_POINT('Ctrl Pts',(-48.8988128289049,29.8239088085271,
-228.227919221305));
#190009=CARTESIAN_POINT('Ctrl Pts',(-48.8739511938202,29.825515359973,-228.240165223074));
#190010=CARTESIAN_POINT('Ctrl Pts',(-48.849306086085,29.8285163971193,-228.251751617269));
#190011=CARTESIAN_POINT('Ctrl Pts',(-48.8251655012992,29.8329948799433,
-228.262505936811));
#190012=CARTESIAN_POINT('Ctrl Pts',(-48.8165309820697,29.8345967278856,
-228.266352503898));
#190013=CARTESIAN_POINT('Ctrl Pts',(-48.8079612516762,29.8363873459285,
-228.270092960664));
#190014=CARTESIAN_POINT('Ctrl Pts',(-48.799470260208,29.8383697609083,-228.273720624));
#190015=CARTESIAN_POINT('Ctrl Pts',(-48.7738910424793,29.8443418107669,
-228.284649005056));
#190016=CARTESIAN_POINT('Ctrl Pts',(-48.7489150276425,29.8521574393405,
-228.294624127528));
#190017=CARTESIAN_POINT('Ctrl Pts',(-48.7247444939762,29.8617843087228,
-228.3034703766));
#190018=CARTESIAN_POINT('Ctrl Pts',(-48.7007470557507,29.8713422360112,
-228.312253273932));
#190019=CARTESIAN_POINT('Ctrl Pts',(-48.67754399401,29.88268516539,-228.319922927921));
#190020=CARTESIAN_POINT('Ctrl Pts',(-48.6553561292837,29.8957586681485,
-228.326347457397));
#190021=CARTESIAN_POINT('Ctrl Pts',(-48.6332362468861,29.9087921144539,
-228.332752302488));
#190022=CARTESIAN_POINT('Ctrl Pts',(-48.6121258098598,29.9235450873337,
-228.337919283806));
#190023=CARTESIAN_POINT('Ctrl Pts',(-48.5922600597141,29.9399472673055,
-228.341763936109));
#190024=CARTESIAN_POINT('Ctrl Pts',(-48.5724227307226,29.956325981318,-228.345603088017));
#190025=CARTESIAN_POINT('Ctrl Pts',(-48.5538270410762,29.974348677228,-228.348123494146));
#190026=CARTESIAN_POINT('Ctrl Pts',(-48.5367163511529,29.9939362403649,
-228.349291389838));
#190027=CARTESIAN_POINT('Ctrl Pts',(-48.5293054173971,30.0024199504604,
-228.349797225526));
#190028=CARTESIAN_POINT('Ctrl Pts',(-48.5221731256271,30.0111971448433,
-228.35005));
#190029=CARTESIAN_POINT('Ctrl Pts',(-48.515339402069,30.020261242545,-228.35005));
#190030=CARTESIAN_POINT('Ctrl Pts',(-49.7445598344273,30.1911641344867,
-227.687068118445));
#190031=CARTESIAN_POINT('Ctrl Pts',(-49.5079616707949,29.9537724063299,
-227.367376825119));
#190032=CARTESIAN_POINT('Ctrl Pts',(-49.8170070935167,29.6096338345331,
-227.342971407313));
#190033=CARTESIAN_POINT('Ctrl Pts',(-51.3768241225023,31.8289031354474,
-225.262929889291));
#190034=CARTESIAN_POINT('Ctrl Pts',(-51.1414011469561,31.5926905373472,
-224.940062144777));
#190035=CARTESIAN_POINT('Ctrl Pts',(-51.4500767842084,31.2466813577455,
-224.918633333245));
#190036=CARTESIAN_POINT('Ctrl Pts',(-53.0099479863855,33.4675045952855,
-222.839953095868));
#190037=CARTESIAN_POINT('Ctrl Pts',(-52.7769579711113,33.2337331174656,
-222.511152157197));
#190038=CARTESIAN_POINT('Ctrl Pts',(-53.0845220861009,32.8841489423223,
-222.495325263031));
#190039=CARTESIAN_POINT('Ctrl Pts',(-54.6462557747613,35.1093006586908,
-220.421288892634));
#190040=CARTESIAN_POINT('Ctrl Pts',(-54.4073852385165,34.8696289362572,
-220.0969923867));
#190041=CARTESIAN_POINT('Ctrl Pts',(-54.7232341443935,34.5239834253819,
-220.076050819216));
#190042=CARTESIAN_POINT('',(-54.5875190481084,35.0503669255136,-220.508112862707));
#190043=CARTESIAN_POINT('',(-54.6643562096698,34.4651804296884,-220.162900223157));
#190044=CARTESIAN_POINT('Origin',(-54.9416638693848,34.6974059566189,-220.508112862707));
#190045=CARTESIAN_POINT('Ctrl Pts',(-54.5875190481084,35.0503669255136,
-220.508112862707));
#190046=CARTESIAN_POINT('Ctrl Pts',(-52.990443779671,33.4479349702851,-222.86899632084));
#190047=CARTESIAN_POINT('Ctrl Pts',(-51.3963761190905,31.8485207106117,
-225.233951400128));
#190048=CARTESIAN_POINT('Ctrl Pts',(-49.8031531494471,30.2499539750197,
-227.60005));
#190049=CARTESIAN_POINT('Ctrl Pts',(-49.8755750290351,29.6684593880862,
-227.255950349386));
#190050=CARTESIAN_POINT('Ctrl Pts',(-50.3041362735325,30.098058504813,-226.619758552752));
#190051=CARTESIAN_POINT('Ctrl Pts',(-50.7327920588234,30.5277322534597,
-225.983640132402));
#190052=CARTESIAN_POINT('Ctrl Pts',(-51.161601590644,30.9574566332008,-225.347649411111));
#190053=CARTESIAN_POINT('Ctrl Pts',(-51.6179083782284,31.4147369329968,
-224.670876015395));
#190054=CARTESIAN_POINT('Ctrl Pts',(-52.0743881629137,31.8720749432885,
-223.994247221146));
#190055=CARTESIAN_POINT('Ctrl Pts',(-52.5310972104373,32.3295031544124,
-223.317828485869));
#190056=CARTESIAN_POINT('Ctrl Pts',(-53.024051994686,32.8232341771425,-222.587727224425));
#190057=CARTESIAN_POINT('Ctrl Pts',(-53.5172714088493,33.3170716250959,
-221.857870686764));
#190058=CARTESIAN_POINT('Ctrl Pts',(-54.0108369280568,33.8111131722922,
-221.128341184644));
#190059=CARTESIAN_POINT('Ctrl Pts',(-54.2286056520954,34.0290919272257,
-220.806461509823));
#190060=CARTESIAN_POINT('Ctrl Pts',(-54.4464421227249,34.2471109897794,
-220.484645499357));
#190061=CARTESIAN_POINT('Ctrl Pts',(-54.6643562096698,34.4651804296884,
-220.162900223157));
#190062=CARTESIAN_POINT('Ctrl Pts',(-42.6824807550636,35.9538445605081,
-228.35005));
#190063=CARTESIAN_POINT('Ctrl Pts',(-42.5405392130025,35.7913421132894,
-228.35005));
#190064=CARTESIAN_POINT('Ctrl Pts',(-42.4431629103415,35.679860391633,-228.507034483728));
#190065=CARTESIAN_POINT('Ctrl Pts',(-43.7299304472252,35.0389252651105,
-228.35005));
#190066=CARTESIAN_POINT('Ctrl Pts',(-43.5839578161182,34.8805832623425,
-228.350049999846));
#190067=CARTESIAN_POINT('Ctrl Pts',(-43.4842614434386,34.7712285271383,
-228.506443516651));
#190068=CARTESIAN_POINT('Ctrl Pts',(-44.7400658047431,34.0873590008399,
-228.35005));
#190069=CARTESIAN_POINT('Ctrl Pts',(-44.590423195572,33.9329609873047,-228.350049999904));
#190070=CARTESIAN_POINT('Ctrl Pts',(-44.4876418177359,33.826550002353,-228.506035020985));
#190071=CARTESIAN_POINT('Ctrl Pts',(-46.6832166107726,32.108381759188,-228.35005));
#190072=CARTESIAN_POINT('Ctrl Pts',(-46.5261142282933,31.9620046547715,
-228.350050000096));
#190073=CARTESIAN_POINT('Ctrl Pts',(-46.4180861418825,31.8610058543969,
-228.505671567324));
#190074=CARTESIAN_POINT('Ctrl Pts',(-47.617275666974,31.0819979338032,-228.35005));
#190075=CARTESIAN_POINT('Ctrl Pts',(-47.4568224915956,30.9392657163356,
-228.350050000173));
#190076=CARTESIAN_POINT('Ctrl Pts',(-47.3461759565219,30.8411406013281,
-228.505709331207));
#190077=CARTESIAN_POINT('Ctrl Pts',(-48.515339402069,30.020261242545,-228.35005));
#190078=CARTESIAN_POINT('Ctrl Pts',(-48.3513278433713,29.8815330303712,
-228.35005));
#190079=CARTESIAN_POINT('Ctrl Pts',(-48.2384287873563,29.7860380279371,
-228.505869818703));
#190080=CARTESIAN_POINT('',(-42.4431629103415,35.679860391633,-228.507034483728));
#190081=CARTESIAN_POINT('',(-42.6824807550636,35.9538445605081,-228.35005));
#190082=CARTESIAN_POINT('Origin',(-42.6824807550636,35.9538445605081,-228.85005));
#190083=CARTESIAN_POINT('Ctrl Pts',(-42.4431629103415,35.679860391633,-228.507034483728));
#190084=CARTESIAN_POINT('Ctrl Pts',(-42.7614810097597,35.402044258979,-228.506853794282));
#190085=CARTESIAN_POINT('Ctrl Pts',(-43.076290124364,35.1208529422878,-228.506690163061));
#190086=CARTESIAN_POINT('Ctrl Pts',(-43.3875670018904,34.8362478331756,
-228.50654485622));
#190087=CARTESIAN_POINT('Ctrl Pts',(-43.7001585717382,34.5504406811923,
-228.506398935668));
#190088=CARTESIAN_POINT('Ctrl Pts',(-44.0091888390155,34.2611903638572,
-228.506271494611));
#190089=CARTESIAN_POINT('Ctrl Pts',(-44.3146116172886,33.9684109762988,
-228.506163815315));
#190090=CARTESIAN_POINT('Ctrl Pts',(-44.4471552006037,33.8413542146283,
-228.506117085992));
#190091=CARTESIAN_POINT('Ctrl Pts',(-44.579019031032,33.7136322786005,-228.506074078358));
#190092=CARTESIAN_POINT('Ctrl Pts',(-44.7101974035188,33.5852357646224,
-228.506034897212));
#190093=CARTESIAN_POINT('Ctrl Pts',(-44.9602123734819,33.3405227835339,
-228.505960221236));
#190094=CARTESIAN_POINT('Ctrl Pts',(-45.2077386206811,33.0933602183811,
-228.505899445037));
#190095=CARTESIAN_POINT('Ctrl Pts',(-45.4528639798092,32.843777928375,-228.505853294154));
#190096=CARTESIAN_POINT('Ctrl Pts',(-45.7541910954216,32.5369720074249,
-228.505796561907));
#190097=CARTESIAN_POINT('Ctrl Pts',(-46.0518578739747,32.22654482337,-228.505761221002));
#190098=CARTESIAN_POINT('Ctrl Pts',(-46.3459620452366,31.9125632804965,
-228.505744327283));
#190099=CARTESIAN_POINT('Ctrl Pts',(-46.6359601710032,31.6029652949666,
-228.505727669421));
#190100=CARTESIAN_POINT('Ctrl Pts',(-46.9224947730646,31.2899106893207,
-228.505728947252));
#190101=CARTESIAN_POINT('Ctrl Pts',(-47.205610866628,30.9734514217353,-228.50574533822));
#190102=CARTESIAN_POINT('Ctrl Pts',(-47.4798027284841,30.6669674112761,
-228.505761212521));
#190103=CARTESIAN_POINT('Ctrl Pts',(-47.7507883244766,30.3572892892455,
-228.5057912622));
#190104=CARTESIAN_POINT('Ctrl Pts',(-48.0185596969337,30.0444638109572,
-228.505832923288));
#190105=CARTESIAN_POINT('Ctrl Pts',(-48.0920923646595,29.9585588400857,
-228.505844363835));
#190106=CARTESIAN_POINT('Ctrl Pts',(-48.165382347877,29.8724165560943,-228.505856680005));
#190107=CARTESIAN_POINT('Ctrl Pts',(-48.2384287873562,29.786038027937,-228.505869818702));
#190108=CARTESIAN_POINT('Ctrl Pts',(-48.515339402069,30.020261242545,-228.35005));
#190109=CARTESIAN_POINT('Ctrl Pts',(-47.6172684110892,31.0820065120798,
-228.35005));
#190110=CARTESIAN_POINT('Ctrl Pts',(-46.6832166107701,32.1083817591879,
-228.35005));
#190111=CARTESIAN_POINT('Ctrl Pts',(-45.7116412077571,33.0978703800133,
-228.35005));
#190112=CARTESIAN_POINT('Ctrl Pts',(-44.7400658047442,34.0873590008387,
-228.35005));
#190113=CARTESIAN_POINT('Ctrl Pts',(-43.7299213057923,35.0389332497409,
-228.35005));
#190114=CARTESIAN_POINT('Ctrl Pts',(-42.6824807550636,35.9538445605081,
-228.35005));
#190115=CARTESIAN_POINT('Ctrl Pts',(-55.2146353748417,36.257836765148,-218.504776656654));
#190116=CARTESIAN_POINT('Ctrl Pts',(-55.018269151756,36.2900558272771,-218.637811171833));
#190117=CARTESIAN_POINT('Ctrl Pts',(-54.9968660030027,36.3988348033229,
-218.849954951747));
#190118=CARTESIAN_POINT('Ctrl Pts',(-55.2870795674723,35.8851781565843,
-218.703954005327));
#190119=CARTESIAN_POINT('Ctrl Pts',(-55.0614326261131,35.9588010119757,
-218.832425369537));
#190120=CARTESIAN_POINT('Ctrl Pts',(-55.0521021372359,36.1181036739044,
-219.049315831024));
#190121=CARTESIAN_POINT('Ctrl Pts',(-55.2466620625291,35.5359310914311,
-218.973388048176));
#190122=CARTESIAN_POINT('Ctrl Pts',(-54.9920018853069,35.6566773356509,
-219.093930954104));
#190123=CARTESIAN_POINT('Ctrl Pts',(-55.0225064544177,35.8553343499258,
-219.318743015259));
#190124=CARTESIAN_POINT('Ctrl Pts',(-55.0420621792248,34.9357811050992,
-219.543206859613));
#190125=CARTESIAN_POINT('Ctrl Pts',(-54.7478058041436,35.1574653296577,
-219.62907206067));
#190126=CARTESIAN_POINT('Ctrl Pts',(-54.8701701172644,35.4039199531623,
-219.888552047862));
#190127=CARTESIAN_POINT('Ctrl Pts',(-54.8753705653332,34.6763452196008,
-219.851342245784));
#190128=CARTESIAN_POINT('Ctrl Pts',(-54.5592271140415,34.9538518370352,
-219.918109540735));
#190129=CARTESIAN_POINT('Ctrl Pts',(-54.7455508540625,35.2089287796778,
-220.196631257502));
#190130=CARTESIAN_POINT('Ctrl Pts',(-54.6643562096698,34.4651804296883,
-220.162900223157));
#190131=CARTESIAN_POINT('Ctrl Pts',(-54.3487296401403,34.8107766034666,
-220.183958003048));
#190132=CARTESIAN_POINT('Ctrl Pts',(-54.5875190481085,35.0503669255137,
-220.508112862707));
#190133=CARTESIAN_POINT('',(-54.9968660030035,36.3988348033192,-218.84995495175));
#190134=CARTESIAN_POINT('',(-55.2146353748417,36.257836765148,-218.504776656654));
#190135=CARTESIAN_POINT('Origin',(-55.4874598092474,36.4953631270242,-218.849954951747));
#190136=CARTESIAN_POINT('Ctrl Pts',(-54.9968660030035,36.3988348033192,
-218.84995495175));
#190137=CARTESIAN_POINT('Ctrl Pts',(-55.0521021372359,36.1181036739044,
-219.049315831024));
#190138=CARTESIAN_POINT('Ctrl Pts',(-55.0225064544177,35.8553343499258,
-219.318743015259));
#190139=CARTESIAN_POINT('Ctrl Pts',(-54.8701701172644,35.4039199531623,
-219.888552047862));
#190140=CARTESIAN_POINT('Ctrl Pts',(-54.7455508540625,35.2089287796778,
-220.196631257502));
#190141=CARTESIAN_POINT('Ctrl Pts',(-54.5875190481084,35.0503669255136,
-220.508112862707));
#190142=CARTESIAN_POINT('Ctrl Pts',(-54.6643562096698,34.4651804296884,
-220.162900223157));
#190143=CARTESIAN_POINT('Ctrl Pts',(-54.8753705653332,34.6763452196008,
-219.851342245784));
#190144=CARTESIAN_POINT('Ctrl Pts',(-55.0420621792248,34.9357811050992,
-219.543206859613));
#190145=CARTESIAN_POINT('Ctrl Pts',(-55.2466620625291,35.5359310914311,
-218.973388048176));
#190146=CARTESIAN_POINT('Ctrl Pts',(-55.2870795674723,35.8851781565843,
-218.703954005327));
#190147=CARTESIAN_POINT('Ctrl Pts',(-55.2146353748417,36.257836765148,-218.504776656654));
#190148=CARTESIAN_POINT('Ctrl Pts',(-42.6314390030157,35.5442154791813,
-228.483430065205));
#190149=CARTESIAN_POINT('Ctrl Pts',(-42.6895757642938,35.6923542175536,
-228.324885333136));
#190150=CARTESIAN_POINT('Ctrl Pts',(-42.8067874347039,35.8824975081984,
-228.335962498089));
#190151=CARTESIAN_POINT('Ctrl Pts',(-42.3959770663564,35.6815375109877,
-228.539447094234));
#190152=CARTESIAN_POINT('Ctrl Pts',(-42.5018122545368,35.7869463556559,
-228.38104135445));
#190153=CARTESIAN_POINT('Ctrl Pts',(-42.645165635708,35.9461794675295,-228.36947199979));
#190154=CARTESIAN_POINT('Ctrl Pts',(-42.2127692669972,35.8992424363046,
-228.49209590616));
#190155=CARTESIAN_POINT('Ctrl Pts',(-42.3616279932723,35.9623936460538,
-228.337833952227));
#190156=CARTESIAN_POINT('Ctrl Pts',(-42.5415988206105,36.0845090848309,
-228.341008503893));
#190157=CARTESIAN_POINT('Ctrl Pts',(-42.0435120014734,36.2819711039298,
-228.300199623458));
#190158=CARTESIAN_POINT('Ctrl Pts',(-42.2573880832737,36.263076259625,-228.168110622012));
#190159=CARTESIAN_POINT('Ctrl Pts',(-42.4817768757597,36.3581540306266,
-228.225845771006));
#190160=CARTESIAN_POINT('Ctrl Pts',(-42.0144214928843,36.4424407209236,
-228.190025881898));
#190161=CARTESIAN_POINT('Ctrl Pts',(-42.252716826051,36.390518917248,-228.068439552117));
#190162=CARTESIAN_POINT('Ctrl Pts',(-42.4902323852614,36.4811949763934,
-228.15975250057));
#190163=CARTESIAN_POINT('Ctrl Pts',(-42.0186496945452,36.7395078303233,
-227.945638225626));
#190164=CARTESIAN_POINT('Ctrl Pts',(-42.298164022469,36.6184786186142,-227.853003287225));
#190165=CARTESIAN_POINT('Ctrl Pts',(-42.5524035821008,36.7205098054508,
-228.013154749775));
#190166=CARTESIAN_POINT('Ctrl Pts',(-42.0508817378213,36.875278360935,-227.812856844476));
#190167=CARTESIAN_POINT('Ctrl Pts',(-42.3494090109542,36.7193110047082,
-227.736210930231));
#190168=CARTESIAN_POINT('Ctrl Pts',(-42.6050823582478,36.8359013839835,
-227.933511896208));
#190169=CARTESIAN_POINT('Ctrl Pts',(-42.1814227629516,37.1709308823785,
-227.48240945426));
#190170=CARTESIAN_POINT('Ctrl Pts',(-42.5181628534428,36.9279710066237,
-227.45166684362));
#190171=CARTESIAN_POINT('Ctrl Pts',(-42.7681359376673,37.099160688942,-227.735306122663));
#190172=CARTESIAN_POINT('Ctrl Pts',(-42.2982676358245,37.3130407532213,
-227.28653339185));
#190173=CARTESIAN_POINT('Ctrl Pts',(-42.6548022753341,37.0131169679292,
-227.289212613848));
#190174=CARTESIAN_POINT('Ctrl Pts',(-42.8898428091843,37.236452809997,-227.617810159066));
#190175=CARTESIAN_POINT('Ctrl Pts',(-42.449568951912,37.4293929451652,-227.088404778768));
#190176=CARTESIAN_POINT('Ctrl Pts',(-42.8047936666804,37.0608530872242,
-227.147939763718));
#190177=CARTESIAN_POINT('Ctrl Pts',(-43.034057629565,37.3598991263913,-227.498955015399));
#190178=CARTESIAN_POINT('',(-42.3284659498332,37.323247286775,-227.257657541791));
#190179=CARTESIAN_POINT('',(-42.9157357330403,37.2503223096489,-227.60005));
#190180=CARTESIAN_POINT('Origin',(-42.561590911764,37.6032832785437,-227.60005));
#190181=CARTESIAN_POINT('Ctrl Pts',(-42.3284659498332,37.323247286775,-227.257657541791));
#190182=CARTESIAN_POINT('Ctrl Pts',(-42.2348212547173,37.2293572270255,
-227.398208277735));
#190183=CARTESIAN_POINT('Ctrl Pts',(-42.1596659254298,37.1216554621379,
-227.537484019296));
#190184=CARTESIAN_POINT('Ctrl Pts',(-42.0508817378213,36.875278360935,-227.812856844476));
#190185=CARTESIAN_POINT('Ctrl Pts',(-42.0186496945452,36.7395078303233,
-227.945638225626));
#190186=CARTESIAN_POINT('Ctrl Pts',(-42.0144214928843,36.4424407209236,
-228.190025881898));
#190187=CARTESIAN_POINT('Ctrl Pts',(-42.0435120014734,36.2819711039298,
-228.300199623458));
#190188=CARTESIAN_POINT('Ctrl Pts',(-42.1845597227432,35.9630305475754,
-228.460113192376));
#190189=CARTESIAN_POINT('Ctrl Pts',(-42.2981827642303,35.8063936694652,
-228.507116757362));
#190190=CARTESIAN_POINT('Ctrl Pts',(-42.4431629103415,35.679860391633,-228.507034483728));
#190191=CARTESIAN_POINT('Ctrl Pts',(-42.6824807550637,35.9538445605081,
-228.35005));
#190192=CARTESIAN_POINT('Ctrl Pts',(-42.6612421131876,35.9708237622937,
-228.35005));
#190193=CARTESIAN_POINT('Ctrl Pts',(-42.6416747886319,35.9894679971484,
-228.348584527935));
#190194=CARTESIAN_POINT('Ctrl Pts',(-42.6238483368174,36.0095108015785,
-228.345682187426));
#190195=CARTESIAN_POINT('Ctrl Pts',(-42.6059666673684,36.0296156888201,
-228.342770856886));
#190196=CARTESIAN_POINT('Ctrl Pts',(-42.5898371951945,36.051127301889,-228.338413910558));
#190197=CARTESIAN_POINT('Ctrl Pts',(-42.5755217393577,36.0737850501726,
-228.33269132462));
#190198=CARTESIAN_POINT('Ctrl Pts',(-42.5611722482051,36.0964966677587,
-228.326955133107));
#190199=CARTESIAN_POINT('Ctrl Pts',(-42.548645882488,36.1203594054282,-228.31984714813));
#190200=CARTESIAN_POINT('Ctrl Pts',(-42.5379889612067,36.1451266982139,
-228.311495283899));
#190201=CARTESIAN_POINT('Ctrl Pts',(-42.5272658827256,36.1700477441047,
-228.303091572054));
#190202=CARTESIAN_POINT('Ctrl Pts',(-42.5184359407265,36.1958842028134,
-228.293428964205));
#190203=CARTESIAN_POINT('Ctrl Pts',(-42.5115234927364,36.2224076420049,
-228.282679485579));
#190204=CARTESIAN_POINT('Ctrl Pts',(-42.5096639751583,36.2295427121681,
-228.279787768421));
#190205=CARTESIAN_POINT('Ctrl Pts',(-42.5079430742378,36.2367276415673,
-228.276817606924));
#190206=CARTESIAN_POINT('Ctrl Pts',(-42.5063609306933,36.2439583155883,
-228.273772785812));
#190207=CARTESIAN_POINT('Ctrl Pts',(-42.499116500259,36.2770666357026,-228.259830944183));
#190208=CARTESIAN_POINT('Ctrl Pts',(-42.494659406233,36.3109617038901,-228.244340883019));
#190209=CARTESIAN_POINT('Ctrl Pts',(-42.4927644141358,36.3453020509556,
-228.227596971681));
#190210=CARTESIAN_POINT('Ctrl Pts',(-42.4908247467518,36.3804519870738,
-228.210458315139));
#190211=CARTESIAN_POINT('Ctrl Pts',(-42.4915690756913,36.4160687787602,
-228.192006435094));
#190212=CARTESIAN_POINT('Ctrl Pts',(-42.4947199712114,36.4518219988906,
-228.17253425434));
#190213=CARTESIAN_POINT('Ctrl Pts',(-42.4979832092334,36.4888499696984,
-228.152367809531));
#190214=CARTESIAN_POINT('Ctrl Pts',(-42.5038273540626,36.5260245969845,
-228.131107425433));
#190215=CARTESIAN_POINT('Ctrl Pts',(-42.5119112524688,36.5630117033036,
-228.10904757488));
#190216=CARTESIAN_POINT('Ctrl Pts',(-42.5146625727291,36.575600106803,-228.10153959906));
#190217=CARTESIAN_POINT('Ctrl Pts',(-42.5176730846629,36.5881670385908,
-228.093938733431));
#190218=CARTESIAN_POINT('Ctrl Pts',(-42.5209286169307,36.6007000433444,
-228.086255696196));
#190219=CARTESIAN_POINT('Ctrl Pts',(-42.529961845291,36.6354757680692,-228.064937329756));
#190220=CARTESIAN_POINT('Ctrl Pts',(-42.5408322428461,36.6698780646667,
-228.043043933556));
#190221=CARTESIAN_POINT('Ctrl Pts',(-42.5533688063073,36.703887121906,-228.020713953601));
#190222=CARTESIAN_POINT('Ctrl Pts',(-42.5662746745788,36.7388980253429,
-227.997726172244));
#190223=CARTESIAN_POINT('Ctrl Pts',(-42.580945768289,36.7734927289696,-227.974275110284));
#190224=CARTESIAN_POINT('Ctrl Pts',(-42.5972074794775,36.8076377013941,
-227.950458060818));
#190225=CARTESIAN_POINT('Ctrl Pts',(-42.6140741981072,36.8430530175208,
-227.925754911975));
#190226=CARTESIAN_POINT('Ctrl Pts',(-42.6326515546369,36.877985051418,-227.900657335133));
#190227=CARTESIAN_POINT('Ctrl Pts',(-42.6527659342923,36.9123752433028,
-227.875226912736));
#190228=CARTESIAN_POINT('Ctrl Pts',(-42.6592357673371,36.923436921748,-227.867047163224));
#190229=CARTESIAN_POINT('Ctrl Pts',(-42.6658648129815,36.9344423497653,
-227.858832670863));
#190230=CARTESIAN_POINT('Ctrl Pts',(-42.6726478674913,36.9453890066653,
-227.850584698399));
#190231=CARTESIAN_POINT('Ctrl Pts',(-42.6935377611533,36.9791016206895,
-227.825183270849));
#190232=CARTESIAN_POINT('Ctrl Pts',(-42.7157356438111,37.0120035407902,
-227.799674957455));
#190233=CARTESIAN_POINT('Ctrl Pts',(-42.7391629924829,37.044155356842,-227.774091800136));
#190234=CARTESIAN_POINT('Ctrl Pts',(-42.7629835616951,37.0768468308236,
-227.748079237719));
#190235=CARTESIAN_POINT('Ctrl Pts',(-42.7880749469651,37.1087630767367,
-227.721988306624));
#190236=CARTESIAN_POINT('Ctrl Pts',(-42.8143869883701,37.1399355114056,
-227.695823652788));
#190237=CARTESIAN_POINT('Ctrl Pts',(-42.840965774659,37.1714239644078,-227.669393748246));
#190238=CARTESIAN_POINT('Ctrl Pts',(-42.8687899359095,37.2021536040928,
-227.642887555501));
#190239=CARTESIAN_POINT('Ctrl Pts',(-42.8978437135211,37.2321209902752,
-227.616296132796));
#190240=CARTESIAN_POINT('Ctrl Pts',(-42.9037566503552,37.2382198619588,
-227.610884326976));
#190241=CARTESIAN_POINT('Ctrl Pts',(-42.9097206386978,37.2442870403172,
-227.605468976743));
#190242=CARTESIAN_POINT('Ctrl Pts',(-42.9157357330403,37.2503223096489,
-227.60005));
#190243=CARTESIAN_POINT('Origin',(-55.4874598092496,36.4953631270247,-218.849954951747));
#190244=CARTESIAN_POINT('',(-55.4814981831708,36.4969369346298,-218.349992971048));
#190245=CARTESIAN_POINT('Origin',(-55.4874598092437,36.4953631270311,-218.849954951747));
#190246=CARTESIAN_POINT('Origin',(-55.4874598092496,36.4953631270247,-218.849954951747));
#190247=CARTESIAN_POINT('Ctrl Pts',(-47.6725669502457,42.0231082257046,
-220.466889015618));
#190248=CARTESIAN_POINT('Ctrl Pts',(-47.4323473287633,41.7820828931217,
-220.144369179074));
#190249=CARTESIAN_POINT('Ctrl Pts',(-47.0855208017344,42.0968841351482,
-220.123650503535));
#190250=CARTESIAN_POINT('Ctrl Pts',(-46.0707360771706,40.4159047152535,
-222.861099896523));
#190251=CARTESIAN_POINT('Ctrl Pts',(-45.8332096734332,40.1775816336063,
-222.536757805232));
#190252=CARTESIAN_POINT('Ctrl Pts',(-45.484400697872,40.4881098339549,-222.518656969387));
#190253=CARTESIAN_POINT('Ctrl Pts',(-44.4733723917422,38.813183375666,-225.261296765486));
#190254=CARTESIAN_POINT('Ctrl Pts',(-44.2319528875239,38.5709541354632,
-224.942221240203));
#190255=CARTESIAN_POINT('Ctrl Pts',(-43.8866629950407,38.8855972869987,
-224.918940663302));
#190256=CARTESIAN_POINT('Ctrl Pts',(-42.8753796545602,37.2098308744472,
-227.66064404434));
#190257=CARTESIAN_POINT('Ctrl Pts',(-42.6348178655346,36.9684622266801,
-227.339136087256));
#190258=CARTESIAN_POINT('Ctrl Pts',(-42.288052160332,37.2828082188042,-227.318248057395));
#190259=CARTESIAN_POINT('',(-47.045128487469,42.0562187287015,-220.184138377616));
#190260=CARTESIAN_POINT('',(-47.632114758242,41.9825203546087,-220.52735443572));
#190261=CARTESIAN_POINT('Origin',(-47.2779699369656,42.3354813235036,-220.52735443572));
#190262=CARTESIAN_POINT('Ctrl Pts',(-47.0451284874689,42.0562187287015,
-220.184138377615));
#190263=CARTESIAN_POINT('Ctrl Pts',(-46.7366960558646,41.7463211125423,
-220.645534816153));
#190264=CARTESIAN_POINT('Ctrl Pts',(-46.4284290381068,41.4366970979731,
-221.107125178941));
#190265=CARTESIAN_POINT('Ctrl Pts',(-46.120270683096,41.1272424048856,-221.568864745196));
#190266=CARTESIAN_POINT('Ctrl Pts',(-45.9716601344877,40.9780066922679,
-221.79154042197));
#190267=CARTESIAN_POINT('Ctrl Pts',(-45.8230746082339,40.8288112637528,
-222.014250798809));
#190268=CARTESIAN_POINT('Ctrl Pts',(-45.6745073115757,40.6796484353907,
-222.236990859958));
#190269=CARTESIAN_POINT('Ctrl Pts',(-45.3447900435204,40.3486094963428,
-222.731320676143));
#190270=CARTESIAN_POINT('Ctrl Pts',(-45.0151589288621,40.0177304633959,
-223.225796697889));
#190271=CARTESIAN_POINT('Ctrl Pts',(-44.6855353620086,39.6869690109204,
-223.720364098522));
#190272=CARTESIAN_POINT('Ctrl Pts',(-44.3702745988347,39.3706199436151,
-224.193381539759));
#190273=CARTESIAN_POINT('Ctrl Pts',(-44.0550203277662,39.0543798419438,
-224.666482570011));
#190274=CARTESIAN_POINT('Ctrl Pts',(-43.7397498044305,38.7382135573481,
-225.139619221798));
#190275=CARTESIAN_POINT('Ctrl Pts',(-43.4407153855777,38.4383295080099,
-225.588389827462));
#190276=CARTESIAN_POINT('Ctrl Pts',(-43.1416663361619,38.1385125871435,
-226.03719248019));
#190277=CARTESIAN_POINT('Ctrl Pts',(-42.8426281635058,37.838720016404,-226.485986248233));
#190278=CARTESIAN_POINT('Ctrl Pts',(-42.6712323665805,37.6668918309996,
-226.743215500424));
#190279=CARTESIAN_POINT('Ctrl Pts',(-42.4998409833723,37.4950713442305,
-227.000441833917));
#190280=CARTESIAN_POINT('Ctrl Pts',(-42.3284659498332,37.3232472867749,
-227.25765754179));
#190281=CARTESIAN_POINT('Ctrl Pts',(-42.9157357330403,37.2503223096489,
-227.60005));
#190282=CARTESIAN_POINT('Ctrl Pts',(-44.486815106976,38.8266711785776,-225.241083793951));
#190283=CARTESIAN_POINT('Ctrl Pts',(-46.0573252848254,40.4024489423018,
-222.881355908373));
#190284=CARTESIAN_POINT('Ctrl Pts',(-47.632114758242,41.9825203546087,-220.52735443572));
#190285=CARTESIAN_POINT('Ctrl Pts',(-55.4804763444372,36.5293010961029,
-218.35005));
#190286=CARTESIAN_POINT('Ctrl Pts',(-54.9916284043978,36.4242882801267,
-218.35005));
#190287=CARTESIAN_POINT('Ctrl Pts',(-54.9916284043978,36.4242882801268,
-218.85005));
#190288=CARTESIAN_POINT('Ctrl Pts',(-55.4808808567138,36.5185275155889,
-218.35005));
#190289=CARTESIAN_POINT('Ctrl Pts',(-54.9932481939215,36.4167479617736,
-218.351913756624));
#190290=CARTESIAN_POINT('Ctrl Pts',(-54.9934502776071,36.4158072299129,
-218.850049997976));
#190291=CARTESIAN_POINT('Ctrl Pts',(-55.4812212937741,36.5077394466269,
-218.350030277458));
#190292=CARTESIAN_POINT('Ctrl Pts',(-54.9948238206649,36.4091341749127,
-218.353722457588));
#190293=CARTESIAN_POINT('Ctrl Pts',(-54.9951959309483,36.4073227473215,
-218.85001713104));
#190294=CARTESIAN_POINT('Ctrl Pts',(-55.4814981831709,36.4969369346252,
-218.349992971048));
#190295=CARTESIAN_POINT('Ctrl Pts',(-54.9963513974766,36.4014502251401,
-218.35547736011));
#190296=CARTESIAN_POINT('Ctrl Pts',(-54.9968660030035,36.3988348033192,
-218.849954951747));
#190297=CARTESIAN_POINT('',(-54.9916284043978,36.4242882801268,-218.85005));
#190298=CARTESIAN_POINT('',(-55.4804763444372,36.529301096103,-218.35005));
#190299=CARTESIAN_POINT('Origin',(-55.4804763444372,36.529301096103,-218.85005));
#190300=CARTESIAN_POINT('Ctrl Pts',(-54.9916284043978,36.4242882801268,
-218.85005));
#190301=CARTESIAN_POINT('Ctrl Pts',(-54.9934477121007,36.4158191726697,
-218.850049997978));
#190302=CARTESIAN_POINT('Ctrl Pts',(-54.9951937291456,36.4073339377235,
-218.850017211078));
#190303=CARTESIAN_POINT('Ctrl Pts',(-54.9968660030035,36.3988348033193,
-218.849954951747));
#190304=CARTESIAN_POINT('Ctrl Pts',(-55.4814981831708,36.4969369346298,
-218.349992971048));
#190305=CARTESIAN_POINT('Ctrl Pts',(-55.4812216183662,36.507726772777,-218.350030233692));
#190306=CARTESIAN_POINT('Ctrl Pts',(-55.4808813172563,36.5185152497272,
-218.35005));
#190307=CARTESIAN_POINT('Ctrl Pts',(-55.4804763444372,36.5293010961029,
-218.35005));
#190308=CARTESIAN_POINT('Ctrl Pts',(-47.0451284874689,42.0562187287016,
-220.184138377616));
#190309=CARTESIAN_POINT('Ctrl Pts',(-47.3919300806125,41.7415300830818,
-220.204915325333));
#190310=CARTESIAN_POINT('Ctrl Pts',(-47.6321147582419,41.9825203546088,
-220.52735443572));
#190311=CARTESIAN_POINT('Ctrl Pts',(-47.255889523814,42.2679809657455,-219.868852497358));
#190312=CARTESIAN_POINT('Ctrl Pts',(-47.5344785649843,41.9530961111727,
-219.935794482803));
#190313=CARTESIAN_POINT('Ctrl Pts',(-47.7902484566451,42.1411844429755,
-220.212182607147));
#190314=CARTESIAN_POINT('Ctrl Pts',(-47.5083824724237,42.4326649364373,
-219.563965012339));
#190315=CARTESIAN_POINT('Ctrl Pts',(-47.7321494909123,42.1394451765273,
-219.649704637013));
#190316=CARTESIAN_POINT('Ctrl Pts',(-47.979916006804,42.2643583982894,-219.907394043497));
#190317=CARTESIAN_POINT('Ctrl Pts',(-47.9638307571195,42.5902413709234,
-219.126165729975));
#190318=CARTESIAN_POINT('Ctrl Pts',(-48.1175959253334,42.3304889669946,
-219.231029546912));
#190319=CARTESIAN_POINT('Ctrl Pts',(-48.3223344522033,42.3817233472697,
-219.469720269686));
#190320=CARTESIAN_POINT('Ctrl Pts',(-48.1257697081407,42.6260372470742,
-218.986746587153));
#190321=CARTESIAN_POINT('Ctrl Pts',(-48.2547747023755,42.3779588184046,
-219.098571457423));
#190322=CARTESIAN_POINT('Ctrl Pts',(-48.4441285568114,42.4082510978143,
-219.330335434309));
#190323=CARTESIAN_POINT('Ctrl Pts',(-48.4690711499925,42.6549505391913,
-218.728256059429));
#190324=CARTESIAN_POINT('Ctrl Pts',(-48.5489925463843,42.4312682822097,
-218.853050886545));
#190325=CARTESIAN_POINT('Ctrl Pts',(-48.7024187673646,42.4292025475747,
-219.071888450682));
#190326=CARTESIAN_POINT('Ctrl Pts',(-48.653008232648,42.6479010052333,-218.607549287091));
#190327=CARTESIAN_POINT('Ctrl Pts',(-48.7086549671031,42.4384217702358,
-218.737132750756));
#190328=CARTESIAN_POINT('Ctrl Pts',(-48.8408569866015,42.4234942721777,
-218.951187879954));
#190329=CARTESIAN_POINT('Ctrl Pts',(-48.841793010828,42.6113834075459,-218.506376562157));
#190330=CARTESIAN_POINT('Ctrl Pts',(-48.874649979175,42.4168725889835,-218.639304842979));
#190331=CARTESIAN_POINT('Ctrl Pts',(-48.9829866058019,42.3956441991541,
-218.850009606915));
#190332=CARTESIAN_POINT('',(-48.8417930108281,42.6113834075459,-218.506376562157));
#190333=CARTESIAN_POINT('',(-48.9829866058019,42.3956441991541,-218.850009606915));
#190334=CARTESIAN_POINT('Origin',(-49.0791324003789,42.8863131162308,-218.850009606915));
#190335=CARTESIAN_POINT('Ctrl Pts',(-48.8417930108281,42.6113834075459,
-218.506376562157));
#190336=CARTESIAN_POINT('Ctrl Pts',(-48.653008232648,42.6479010052333,-218.607549287091));
#190337=CARTESIAN_POINT('Ctrl Pts',(-48.4690711499925,42.6549505391913,
-218.728256059429));
#190338=CARTESIAN_POINT('Ctrl Pts',(-48.1257697081407,42.6260372470742,
-218.986746587153));
#190339=CARTESIAN_POINT('Ctrl Pts',(-47.9638307571195,42.5902413709234,
-219.126165729975));
#190340=CARTESIAN_POINT('Ctrl Pts',(-47.5083824724237,42.4326649364373,
-219.563965012339));
#190341=CARTESIAN_POINT('Ctrl Pts',(-47.255889523814,42.2679809657455,-219.868852497358));
#190342=CARTESIAN_POINT('Ctrl Pts',(-47.045128487469,42.0562187287015,-220.184138377616));
#190343=CARTESIAN_POINT('Ctrl Pts',(-47.632114758242,41.9825203546087,-220.52735443572));
#190344=CARTESIAN_POINT('Ctrl Pts',(-47.7902484566451,42.1411844429755,
-220.212182607147));
#190345=CARTESIAN_POINT('Ctrl Pts',(-47.979916006804,42.2643583982894,-219.907394043497));
#190346=CARTESIAN_POINT('Ctrl Pts',(-48.3223344522033,42.3817233472697,
-219.469720269686));
#190347=CARTESIAN_POINT('Ctrl Pts',(-48.4441285568114,42.4082510978143,
-219.330335434309));
#190348=CARTESIAN_POINT('Ctrl Pts',(-48.7024187673646,42.4292025475747,
-219.071888450682));
#190349=CARTESIAN_POINT('Ctrl Pts',(-48.8408569866015,42.4234942721777,
-218.951187879954));
#190350=CARTESIAN_POINT('Ctrl Pts',(-48.9829866058019,42.3956441991541,
-218.850009606915));
#190351=CARTESIAN_POINT('Origin',(-53.5250845842796,36.1092498321983,-218.85005));
#190352=CARTESIAN_POINT('',(-54.6328983814091,37.1205601658197,-218.85005));
#190353=CARTESIAN_POINT('',(-55.0021696471189,37.4576636103602,-218.35005));
#190354=CARTESIAN_POINT('Origin',(-55.0021696471189,37.4576636103602,-218.85005));
#190355=CARTESIAN_POINT('Origin',(-53.5250845842796,36.1092498321983,-218.85005));
#190356=CARTESIAN_POINT('Origin',(-53.5250845842796,36.1092498321983,-218.35005));
#190357=CARTESIAN_POINT('Origin',(-49.0791324003789,42.8863131162308,-218.850009606915));
#190358=CARTESIAN_POINT('',(-49.0801870931398,42.8824343798319,-218.350025764149));
#190359=CARTESIAN_POINT('Origin',(-49.0791324003789,42.8863131162308,-218.850009606915));
#190360=CARTESIAN_POINT('Origin',(-49.0791324003789,42.8863131162308,-218.850009606915));
#190361=CARTESIAN_POINT('Origin',(-0.128459562639233,-12.6359082483571,
-218.85005));
#190362=CARTESIAN_POINT('',(-49.7021444432209,42.0348313420379,-218.85005));
#190363=CARTESIAN_POINT('',(-50.0380095169376,42.4052293067426,-218.35005));
#190364=CARTESIAN_POINT('Origin',(-50.0380095169376,42.4052293067426,-218.85005));
#190365=CARTESIAN_POINT('Origin',(-0.128459562639233,-12.6359082483571,
-218.85005));
#190366=CARTESIAN_POINT('Origin',(-0.128459562639233,-12.6359082483571,
-218.35005));
#190367=CARTESIAN_POINT('Ctrl Pts',(-48.999474814567,42.392317257495,-218.85005));
#190368=CARTESIAN_POINT('Ctrl Pts',(-48.9994748145671,42.3923172574951,
-218.35005));
#190369=CARTESIAN_POINT('Ctrl Pts',(-49.1011166787324,42.8818771940186,
-218.35005));
#190370=CARTESIAN_POINT('Ctrl Pts',(-48.9939799633645,42.3934580921056,
-218.85004999869));
#190371=CARTESIAN_POINT('Ctrl Pts',(-48.994587444257,42.3933319685669,-218.351257450515));
#190372=CARTESIAN_POINT('Ctrl Pts',(-49.09414603136,42.8820897398471,-218.35005));
#190373=CARTESIAN_POINT('Ctrl Pts',(-48.9884838968603,42.394567013707,-218.850036211906));
#190374=CARTESIAN_POINT('Ctrl Pts',(-48.9896694475663,42.3943279693454,
-218.352441808199));
#190375=CARTESIAN_POINT('Ctrl Pts',(-49.0871694989175,42.882275419924,-218.350041726378));
#190376=CARTESIAN_POINT('Ctrl Pts',(-48.9829866058019,42.3956441991541,
-218.850009606915));
#190377=CARTESIAN_POINT('Ctrl Pts',(-48.9847217242793,42.3953042054457,
-218.353603405568));
#190378=CARTESIAN_POINT('Ctrl Pts',(-49.0801870931398,42.8824343798319,
-218.350025764149));
#190379=CARTESIAN_POINT('',(-49.1011166787325,42.8818771940186,-218.35005));
#190380=CARTESIAN_POINT('',(-48.999474814567,42.392317257495,-218.85005));
#190381=CARTESIAN_POINT('Origin',(-49.1011166787325,42.8818771940186,-218.85005));
#190382=CARTESIAN_POINT('Ctrl Pts',(-49.1011166787325,42.8818771940186,
-218.35005));
#190383=CARTESIAN_POINT('Ctrl Pts',(-49.0941409157939,42.8820898960309,
-218.35005));
#190384=CARTESIAN_POINT('Ctrl Pts',(-49.0871642720694,42.8822755387356,
-218.35004171443));
#190385=CARTESIAN_POINT('Ctrl Pts',(-49.0801870931398,42.8824343798319,
-218.350025764149));
#190386=CARTESIAN_POINT('Ctrl Pts',(-48.9829866058019,42.3956441991541,
-218.850009606915));
#190387=CARTESIAN_POINT('Ctrl Pts',(-48.9884887606911,42.3945660606471,
-218.85003623417));
#190388=CARTESIAN_POINT('Ctrl Pts',(-48.993985033412,42.3934570394682,-218.850049998691));
#190389=CARTESIAN_POINT('Ctrl Pts',(-48.999474814567,42.392317257495,-218.85005));
#190390=CARTESIAN_POINT('Origin',(-48.6945492220708,40.9236374479242,-218.85005));
#190391=CARTESIAN_POINT('Origin',(-48.6945492220708,40.9236374479242,-218.35005));
#190392=CARTESIAN_POINT('Origin',(-48.6945492220708,40.9236374479242,-218.85005));
#190393=CARTESIAN_POINT('Origin',(-41.3132181298675,38.0528376956935,-205.84995));
#190394=CARTESIAN_POINT('',(-48.8684365469981,47.38326056293,-205.34995));
#190395=CARTESIAN_POINT('',(-48.5538345628697,46.9947384336248,-205.841223796781));
#190396=CARTESIAN_POINT('Origin',(-48.8684365469981,47.38326056293,-205.84995));
#190397=CARTESIAN_POINT('',(-43.5622571193626,49.8460535351382,-205.34995));
#190398=CARTESIAN_POINT('Origin',(-41.3132181298675,38.0528376956935,-205.34995));
#190399=CARTESIAN_POINT('',(-43.4686063353067,49.3549798298524,-205.841223796781));
#190400=CARTESIAN_POINT('Origin',(-43.5622571193626,49.8460535351382,-205.84995));
#190401=CARTESIAN_POINT('Origin',(-41.3132181298675,38.0528376956935,-205.841223796781));
#190402=CARTESIAN_POINT('Origin',(0.,-12.9675000200281,-205.84995));
#190403=CARTESIAN_POINT('',(-59.9876878113059,36.3459434263872,-205.34995));
#190404=CARTESIAN_POINT('',(-59.6015030478428,36.0284766063157,-205.841223796781));
#190405=CARTESIAN_POINT('Origin',(-59.9876878113059,36.3459434263873,-205.84995));
#190406=CARTESIAN_POINT('Origin',(0.,-12.9675000200281,-205.34995));
#190407=CARTESIAN_POINT('Origin',(0.,-12.9675000200281,-205.841223796781));
#190408=CARTESIAN_POINT('Origin',(-50.7133971693864,28.7219255026674,-205.84995));
#190409=CARTESIAN_POINT('',(-62.7097829146859,29.1961040154388,-205.34995));
#190410=CARTESIAN_POINT('',(-62.2102491422031,29.1763590533857,-205.841223796781));
#190411=CARTESIAN_POINT('Origin',(-62.709782914686,29.1961040154388,-205.84995));
#190412=CARTESIAN_POINT('Origin',(-50.7133971693864,28.7219255026674,-205.34995));
#190413=CARTESIAN_POINT('Origin',(-50.7133971693864,28.7219255026674,-205.841223796781));
#190414=CARTESIAN_POINT('Origin',(1004.,-12.967500020028,-205.84995));
#190415=CARTESIAN_POINT('',(-62.7097829146858,-55.1311040554952,-205.34995));
#190416=CARTESIAN_POINT('',(-62.210249142203,-55.1113590934421,-205.841223796781));
#190417=CARTESIAN_POINT('Origin',(-62.7097829146858,-55.1311040554952,-205.84995));
#190418=CARTESIAN_POINT('Origin',(1004.,-12.967500020028,-205.34995));
#190419=CARTESIAN_POINT('Origin',(1004.,-12.967500020028,-205.841223796781));
#190420=CARTESIAN_POINT('Origin',(-50.7133971693864,-54.6569255427236,-205.84995));
#190421=CARTESIAN_POINT('',(-59.9876878113058,-62.2809434664435,-205.34995));
#190422=CARTESIAN_POINT('',(-59.6015030478428,-61.963476646372,-205.841223796781));
#190423=CARTESIAN_POINT('Origin',(-59.9876878113059,-62.2809434664436,-205.84995));
#190424=CARTESIAN_POINT('Origin',(-50.7133971693864,-54.6569255427236,-205.34995));
#190425=CARTESIAN_POINT('Origin',(-50.7133971693864,-54.6569255427236,-205.841223796781));
#190426=CARTESIAN_POINT('Origin',(0.,-12.9675000200281,-205.84995));
#190427=CARTESIAN_POINT('',(-49.142885306769,-73.0949913797652,-205.34995));
#190428=CARTESIAN_POINT('',(-48.8265164945923,-72.7079065982776,-205.841223796781));
#190429=CARTESIAN_POINT('Origin',(-49.142885306769,-73.0949913797652,-205.84995));
#190430=CARTESIAN_POINT('Origin',(0.,-12.9675000200281,-205.34995));
#190431=CARTESIAN_POINT('Origin',(0.,-12.9675000200281,-205.841223796781));
#190432=CARTESIAN_POINT('Origin',(-41.5452362233251,-63.7990866568863,-205.84995));
#190433=CARTESIAN_POINT('',(-42.0177747166746,-75.7955371145968,-205.34995));
#190434=CARTESIAN_POINT('',(-41.998098045614,-75.2960006474661,-205.841223796781));
#190435=CARTESIAN_POINT('Origin',(-42.0177747166746,-75.7955371145968,-205.84995));
#190436=CARTESIAN_POINT('Origin',(-41.5452362233251,-63.7990866568863,-205.34995));
#190437=CARTESIAN_POINT('Origin',(-41.5452362233251,-63.7990866568863,-205.841223796781));
#190438=CARTESIAN_POINT('Ctrl Pts',(-54.8483808955534,-62.1772035872459,
-218.488025452358));
#190439=CARTESIAN_POINT('Ctrl Pts',(-54.9567009523893,-62.2733518205983,
-218.35005));
#190440=CARTESIAN_POINT('Ctrl Pts',(-55.1063041457931,-62.4061442430716,
-218.35005));
#190441=CARTESIAN_POINT('Ctrl Pts',(-54.9311672479915,-62.0839582776417,
-218.488011964977));
#190442=CARTESIAN_POINT('Ctrl Pts',(-55.0396688463703,-62.1798977449628,
-218.350049999993));
#190443=CARTESIAN_POINT('Ctrl Pts',(-55.1895187430304,-62.3123951477066,
-218.35005));
#190444=CARTESIAN_POINT('Ctrl Pts',(-55.0136740740184,-61.9904901268691,
-218.487996778696));
#190445=CARTESIAN_POINT('Ctrl Pts',(-55.1223583736924,-62.0862177900411,
-218.350049999995));
#190446=CARTESIAN_POINT('Ctrl Pts',(-55.2724546449993,-62.2184167144339,
-218.35005));
#190447=CARTESIAN_POINT('Ctrl Pts',(-55.0958998011493,-61.8967941020366,
-218.487980161586));
#190448=CARTESIAN_POINT('Ctrl Pts',(-55.2047676214781,-61.9923073188158,
-218.35005));
#190449=CARTESIAN_POINT('Ctrl Pts',(-55.3551085347194,-62.1242062049498,
-218.35005));
#190450=CARTESIAN_POINT('',(-55.3551085347089,-62.1242062049619,-218.35005));
#190451=CARTESIAN_POINT('Origin',(-6.53661556842313,-19.2936642511711,-218.35005));
#190452=CARTESIAN_POINT('',(-55.0958998011388,-61.8967941020485,-218.487980161586));
#190453=CARTESIAN_POINT('Origin',(-55.3551085347089,-62.1242062049619,-218.85005));
#190454=CARTESIAN_POINT('Origin',(-6.32111522020743,-19.0925325781086,-218.204999057165));
#190455=CARTESIAN_POINT('Ctrl Pts',(-55.4938952567199,-61.9654919306031,
-218.35005));
#190456=CARTESIAN_POINT('Ctrl Pts',(-55.3431423575669,-61.8341015991581,
-218.35005));
#190457=CARTESIAN_POINT('Ctrl Pts',(-55.2339673727997,-61.7389489519143,
-218.487950878256));
#190458=CARTESIAN_POINT('Ctrl Pts',(-55.4477195716702,-62.0184723768345,
-218.35005));
#190459=CARTESIAN_POINT('Ctrl Pts',(-55.2971033694472,-61.8869121544979,
-218.350049999996));
#190460=CARTESIAN_POINT('Ctrl Pts',(-55.1880309233148,-61.7916386130721,
-218.487961072495));
#190461=CARTESIAN_POINT('Ctrl Pts',(-55.4014572374666,-62.0713770530022,
-218.35005));
#190462=CARTESIAN_POINT('Ctrl Pts',(-55.2509784443238,-61.9396472076622,
-218.350050000013));
#190463=CARTESIAN_POINT('Ctrl Pts',(-55.14200840849,-61.8442534512036,-218.487970843436));
#190464=CARTESIAN_POINT('Ctrl Pts',(-55.3551085347089,-62.1242062049619,
-218.35005));
#190465=CARTESIAN_POINT('Ctrl Pts',(-55.2047676214677,-61.9923073188278,
-218.35005));
#190466=CARTESIAN_POINT('Ctrl Pts',(-55.0958998011388,-61.8967941020486,
-218.487980161586));
#190467=CARTESIAN_POINT('',(-55.2339673727996,-61.7389489519143,-218.487950878256));
#190468=CARTESIAN_POINT('',(-55.4938952567199,-61.9654919306031,-218.35005));
#190469=CARTESIAN_POINT('Origin',(-55.4938952567198,-61.9654919306031,-218.85005));
#190470=CARTESIAN_POINT('Origin',(-7.62393634648824,-43.3515330069781,-218.305892816451));
#190471=CARTESIAN_POINT('Ctrl Pts',(-55.3551085347089,-62.1242062049619,
-218.35005));
#190472=CARTESIAN_POINT('Ctrl Pts',(-55.4014571755248,-62.0713771235952,
-218.35005));
#190473=CARTESIAN_POINT('Ctrl Pts',(-55.4477196335097,-62.0184723058819,
-218.35005));
#190474=CARTESIAN_POINT('Ctrl Pts',(-55.4938952567199,-61.9654919306031,
-218.35005));
#190475=CARTESIAN_POINT('Ctrl Pts',(-48.9443109379934,-69.7210624363874,
-217.233400031701));
#190476=CARTESIAN_POINT('Ctrl Pts',(-49.0991171386077,-69.4468461963774,
-217.336253844649));
#190477=CARTESIAN_POINT('Ctrl Pts',(-49.2925903552098,-69.4989817480832,
-217.60005));
#190478=CARTESIAN_POINT('Ctrl Pts',(-48.8106894467424,-69.6845014967476,
-217.338910655172));
#190479=CARTESIAN_POINT('Ctrl Pts',(-48.9711549960785,-69.4349010506438,
-217.421407154983));
#190480=CARTESIAN_POINT('Ctrl Pts',(-49.1585563021333,-69.4628633673211,
-217.663314872408));
#190481=CARTESIAN_POINT('Ctrl Pts',(-48.6852690846176,-69.6367945835064,
-217.447311197387));
#190482=CARTESIAN_POINT('Ctrl Pts',(-48.8462037291419,-69.4114072943244,
-217.512721374121));
#190483=CARTESIAN_POINT('Ctrl Pts',(-49.0313897910431,-69.4205569633974,
-217.728324544416));
#190484=CARTESIAN_POINT('Ctrl Pts',(-48.4569758615832,-69.5115061162924,
-217.672103262066));
#190485=CARTESIAN_POINT('Ctrl Pts',(-48.617833871194,-69.3350054470626,
-217.703310121074));
#190486=CARTESIAN_POINT('Ctrl Pts',(-48.7961868532913,-69.3194593473905,
-217.86308947659));
#190487=CARTESIAN_POINT('Ctrl Pts',(-48.3517740014028,-69.4325906117154,
-217.790828095074));
#190488=CARTESIAN_POINT('Ctrl Pts',(-48.5104100125145,-69.2819129896144,
-217.805106001601));
#190489=CARTESIAN_POINT('Ctrl Pts',(-48.685721809208,-69.2595955427122,
-217.934254584857));
#190490=CARTESIAN_POINT('Ctrl Pts',(-48.1937459441518,-69.2310798747107,
-218.028989271677));
#190491=CARTESIAN_POINT('Ctrl Pts',(-48.3463679525101,-69.1352844945817,
-218.007643735867));
#190492=CARTESIAN_POINT('Ctrl Pts',(-48.5116380513506,-69.117661111215,
-218.07697894517));
#190493=CARTESIAN_POINT('Ctrl Pts',(-48.1412202429506,-69.1061885177359,
-218.149957970462));
#190494=CARTESIAN_POINT('Ctrl Pts',(-48.2880154025268,-69.0395906692494,
-218.111013157341));
#190495=CARTESIAN_POINT('Ctrl Pts',(-48.448087208547,-69.0341807326189,
-218.14945588291));
#190496=CARTESIAN_POINT('Ctrl Pts',(-48.1485991473491,-68.8903805804807,
-218.301008298776));
#190497=CARTESIAN_POINT('Ctrl Pts',(-48.2845085174756,-68.8714073071909,
-218.233969642811));
#190498=CARTESIAN_POINT('Ctrl Pts',(-48.434090564434,-68.8996196892853,
-218.239916153685));
#190499=CARTESIAN_POINT('Ctrl Pts',(-48.1657471491621,-68.8149276007785,
-218.34519506975));
#190500=CARTESIAN_POINT('Ctrl Pts',(-48.2974742535841,-68.8121010312849,
-218.268894159576));
#190501=CARTESIAN_POINT('Ctrl Pts',(-48.4434199676664,-68.8540114137795,
-218.266370341262));
#190502=CARTESIAN_POINT('Ctrl Pts',(-48.2274460866499,-68.6669868960869,
-218.415001874049));
#190503=CARTESIAN_POINT('Ctrl Pts',(-48.3498583953795,-68.6963155179756,
-218.320852508057));
#190504=CARTESIAN_POINT('Ctrl Pts',(-48.4891230485367,-68.7673591858045,
-218.308143757591));
#190505=CARTESIAN_POINT('Ctrl Pts',(-48.2716020915273,-68.5947725811949,
-218.440653607377));
#190506=CARTESIAN_POINT('Ctrl Pts',(-48.3890987036532,-68.639745098431,
-218.338051990079));
#190507=CARTESIAN_POINT('Ctrl Pts',(-48.525123832139,-68.7264593463756,
-218.323478979764));
#190508=CARTESIAN_POINT('Ctrl Pts',(-48.3245605310991,-68.5271120961851,
-218.457629631481));
#190509=CARTESIAN_POINT('Ctrl Pts',(-48.4365020850992,-68.587560591765,
-218.34711549972));
#190510=CARTESIAN_POINT('Ctrl Pts',(-48.5701931618904,-68.6892604152372,
-218.333619302448));
#190511=CARTESIAN_POINT('',(-48.9443109379934,-69.7210624363875,-217.233400031701));
#190512=CARTESIAN_POINT('Ctrl Pts',(-48.3245605310987,-68.5271120961857,
-218.45762963148));
#190513=CARTESIAN_POINT('Ctrl Pts',(-48.2716020915273,-68.5947725811949,
-218.440653607377));
#190514=CARTESIAN_POINT('Ctrl Pts',(-48.2274460866499,-68.6669868960869,
-218.415001874049));
#190515=CARTESIAN_POINT('Ctrl Pts',(-48.1657471491621,-68.8149276007785,
-218.34519506975));
#190516=CARTESIAN_POINT('Ctrl Pts',(-48.1485991473491,-68.8903805804807,
-218.301008298776));
#190517=CARTESIAN_POINT('Ctrl Pts',(-48.1412202429506,-69.1061885177359,
-218.149957970462));
#190518=CARTESIAN_POINT('Ctrl Pts',(-48.1937459441518,-69.2310798747107,
-218.028989271677));
#190519=CARTESIAN_POINT('Ctrl Pts',(-48.3517740014028,-69.4325906117154,
-217.790828095074));
#190520=CARTESIAN_POINT('Ctrl Pts',(-48.4569758615832,-69.5115061162924,
-217.672103262066));
#190521=CARTESIAN_POINT('Ctrl Pts',(-48.6852690846176,-69.6367945835064,
-217.447311197387));
#190522=CARTESIAN_POINT('Ctrl Pts',(-48.8106894467424,-69.6845014967476,
-217.338910655172));
#190523=CARTESIAN_POINT('Ctrl Pts',(-48.9443109379934,-69.7210624363875,
-217.233400031701));
#190524=CARTESIAN_POINT('',(-49.2925903552098,-69.4989817480832,-217.60005));
#190525=CARTESIAN_POINT('Origin',(-49.1624951782473,-69.9817604188332,-217.60005));
#190526=CARTESIAN_POINT('Ctrl Pts',(-49.2925903552098,-69.4989817480832,
-217.60005));
#190527=CARTESIAN_POINT('Ctrl Pts',(-49.1585563021333,-69.4628633673211,
-217.663314872408));
#190528=CARTESIAN_POINT('Ctrl Pts',(-49.0313897910431,-69.4205569633974,
-217.728324544416));
#190529=CARTESIAN_POINT('Ctrl Pts',(-48.7961868532913,-69.3194593473905,
-217.86308947659));
#190530=CARTESIAN_POINT('Ctrl Pts',(-48.685721809208,-69.2595955427122,
-217.934254584857));
#190531=CARTESIAN_POINT('Ctrl Pts',(-48.5116380513506,-69.117661111215,
-218.07697894517));
#190532=CARTESIAN_POINT('Ctrl Pts',(-48.448087208547,-69.0341807326189,
-218.14945588291));
#190533=CARTESIAN_POINT('Ctrl Pts',(-48.434090564434,-68.8996196892853,
-218.239916153685));
#190534=CARTESIAN_POINT('Ctrl Pts',(-48.4434199676664,-68.8540114137795,
-218.266370341262));
#190535=CARTESIAN_POINT('Ctrl Pts',(-48.4891230485367,-68.7673591858045,
-218.308143757591));
#190536=CARTESIAN_POINT('Ctrl Pts',(-48.525123832139,-68.7264593463756,
-218.323478979764));
#190537=CARTESIAN_POINT('Ctrl Pts',(-48.5701931618903,-68.6892604152372,
-218.333619302448));
#190538=CARTESIAN_POINT('Ctrl Pts',(-55.0927945669581,-61.9237522605322,
-218.473143922888));
#190539=CARTESIAN_POINT('Ctrl Pts',(-55.2402662392572,-62.0019900264124,
-218.318365680583));
#190540=CARTESIAN_POINT('Ctrl Pts',(-55.4233494278323,-62.1325346783774,
-218.34109494148));
#190541=CARTESIAN_POINT('Ctrl Pts',(-55.2398731800779,-61.7035250203945,
-218.506633117061));
#190542=CARTESIAN_POINT('Ctrl Pts',(-55.339847442567,-61.8077216182083,
-218.369411334443));
#190543=CARTESIAN_POINT('Ctrl Pts',(-55.4942885846974,-61.9313224231195,
-218.361210102213));
#190544=CARTESIAN_POINT('Ctrl Pts',(-55.4522263025615,-61.487229681304,
-218.488253912002));
#190545=CARTESIAN_POINT('Ctrl Pts',(-55.5089980550799,-61.6041191053711,
-218.374487087645));
#190546=CARTESIAN_POINT('Ctrl Pts',(-55.6061969562536,-61.7409934655382,
-218.350218604685));
#190547=CARTESIAN_POINT('Ctrl Pts',(-55.774137059737,-61.3702400653051,
-218.328065200791));
#190548=CARTESIAN_POINT('Ctrl Pts',(-55.7613227347501,-61.506523014171,
-218.253037832299));
#190549=CARTESIAN_POINT('Ctrl Pts',(-55.796657340851,-61.6580344229345,
-218.254184099553));
#190550=CARTESIAN_POINT('Ctrl Pts',(-55.8574514448172,-61.3576561642577,
-218.275537189096));
#190551=CARTESIAN_POINT('Ctrl Pts',(-55.8267293193376,-61.4983471195505,
-218.210866812023));
#190552=CARTESIAN_POINT('Ctrl Pts',(-55.8476827468257,-61.653839850603,
-218.222689657358));
#190553=CARTESIAN_POINT('Ctrl Pts',(-56.0156427621496,-61.3668889087165,
-218.155327703159));
#190554=CARTESIAN_POINT('Ctrl Pts',(-55.9490748084097,-61.515028576828,
-218.112202025634));
#190555=CARTESIAN_POINT('Ctrl Pts',(-55.9478088686909,-61.6782199479451,
-218.150610277818));
#190556=CARTESIAN_POINT('Ctrl Pts',(-56.0882800272526,-61.3885186677252,
-218.089385782703));
#190557=CARTESIAN_POINT('Ctrl Pts',(-56.0046279913313,-61.5397831272315,
-218.056774547579));
#190558=CARTESIAN_POINT('Ctrl Pts',(-55.995486790882,-61.7063946791486,
-218.11106824763));
#190559=CARTESIAN_POINT('Ctrl Pts',(-56.282274388892,-61.4870635747884,
-217.88822842421));
#190560=CARTESIAN_POINT('Ctrl Pts',(-56.1504429355983,-61.6458021440819,
-217.885983497565));
#190561=CARTESIAN_POINT('Ctrl Pts',(-56.1268157801208,-61.8214573400613,
-217.990439031765));
#190562=CARTESIAN_POINT('Ctrl Pts',(-56.3812088475294,-61.5957603700639,
-217.749760076526));
#190563=CARTESIAN_POINT('Ctrl Pts',(-56.2193581582234,-61.7580490411378,
-217.766950789269));
#190564=CARTESIAN_POINT('Ctrl Pts',(-56.1995158790201,-61.9371995248376,
-217.907396389637));
#190565=CARTESIAN_POINT('Ctrl Pts',(-56.5652163308461,-61.8918982137455,
-217.434373456315));
#190566=CARTESIAN_POINT('Ctrl Pts',(-56.3362907798363,-62.05739085945,-217.497500852187));
#190567=CARTESIAN_POINT('Ctrl Pts',(-56.3439416689173,-62.2442222025972,
-217.718239387215));
#190568=CARTESIAN_POINT('Ctrl Pts',(-56.6321920140805,-62.0996608522455,
-217.257993584228));
#190569=CARTESIAN_POINT('Ctrl Pts',(-56.3635142722379,-62.2656775410818,
-217.348845863301));
#190570=CARTESIAN_POINT('Ctrl Pts',(-56.4063229321979,-62.453644092428,
-217.612415918528));
#190571=CARTESIAN_POINT('Ctrl Pts',(-56.6726055091992,-62.3181114609455,
-217.093587076475));
#190572=CARTESIAN_POINT('Ctrl Pts',(-56.3642389105003,-62.4681884271343,
-217.222073078002));
#190573=CARTESIAN_POINT('Ctrl Pts',(-56.4530481014242,-62.6707334235198,
-217.513854009698));
#190574=CARTESIAN_POINT('',(-56.6309943627598,-62.1341374253209,-217.237388612086));
#190575=CARTESIAN_POINT('',(-56.4090189474477,-62.4870630585556,-217.60005));
#190576=CARTESIAN_POINT('Origin',(-56.8921651292037,-62.3583394513399,-217.60005));
#190577=CARTESIAN_POINT('Ctrl Pts',(-56.6309943627598,-62.1341374253209,
-217.237388612086));
#190578=CARTESIAN_POINT('Ctrl Pts',(-56.6071938355743,-62.0458440727314,
-217.309112681226));
#190579=CARTESIAN_POINT('Ctrl Pts',(-56.578015172952,-61.9606625433887,
-217.382726354161));
#190580=CARTESIAN_POINT('Ctrl Pts',(-56.5424466867555,-61.8803805048941,
-217.457905536343));
#190581=CARTESIAN_POINT('Ctrl Pts',(-56.5174877480173,-61.8240453977575,
-217.510659892886));
#190582=CARTESIAN_POINT('Ctrl Pts',(-56.4893817115847,-61.7701241681472,
-217.564185112257));
#190583=CARTESIAN_POINT('Ctrl Pts',(-56.4577719221838,-61.7192435082347,
-217.618369210985));
#190584=CARTESIAN_POINT('Ctrl Pts',(-56.4144730234454,-61.6495474873803,
-217.692590262391));
#190585=CARTESIAN_POINT('Ctrl Pts',(-56.364065657814,-61.5845363129302,
-217.76906264081));
#190586=CARTESIAN_POINT('Ctrl Pts',(-56.3050972761405,-61.5293160073526,
-217.845728184291));
#190587=CARTESIAN_POINT('Ctrl Pts',(-56.2596681710779,-61.4867744114587,
-217.904791141942));
#190588=CARTESIAN_POINT('Ctrl Pts',(-56.2091562799757,-61.4500471971335,
-217.963968745491));
#190589=CARTESIAN_POINT('Ctrl Pts',(-56.1528857709326,-61.42145819393,-218.022319919453));
#190590=CARTESIAN_POINT('Ctrl Pts',(-56.10949285456,-61.3994118281464,-218.067317337372));
#190591=CARTESIAN_POINT('Ctrl Pts',(-56.0625109582255,-61.3824132905256,
-218.111814382599));
#190592=CARTESIAN_POINT('Ctrl Pts',(-56.0123938152309,-61.3722265064741,
-218.154382249795));
#190593=CARTESIAN_POINT('Ctrl Pts',(-55.9878361395995,-61.3672349262779,
-218.175240738776));
#190594=CARTESIAN_POINT('Ctrl Pts',(-55.9625258661404,-61.3638782470511,
-218.195636021717));
#190595=CARTESIAN_POINT('Ctrl Pts',(-55.9365178644268,-61.3623594488966,
-218.215399995439));
#190596=CARTESIAN_POINT('Ctrl Pts',(-55.8847053173817,-61.3593337338995,
-218.254773332519));
#190597=CARTESIAN_POINT('Ctrl Pts',(-55.8310846986675,-61.3636853719657,
-218.290894690184));
#190598=CARTESIAN_POINT('Ctrl Pts',(-55.77644267487,-61.3757084773317,-218.322977700074));
#190599=CARTESIAN_POINT('Ctrl Pts',(-55.7476809181567,-61.38203704292,-218.339865136904));
#190600=CARTESIAN_POINT('Ctrl Pts',(-55.7186365522078,-61.3904902984303,
-218.35563370025));
#190601=CARTESIAN_POINT('Ctrl Pts',(-55.6894269915266,-61.4011060019289,
-218.370168708992));
#190602=CARTESIAN_POINT('Ctrl Pts',(-55.6216481299243,-61.4257390426686,
-218.403896239396));
#190603=CARTESIAN_POINT('Ctrl Pts',(-55.5558942263105,-61.4610272231835,
-218.429484990556));
#190604=CARTESIAN_POINT('Ctrl Pts',(-55.4931147424837,-61.5039756163701,
-218.44805034278));
#190605=CARTESIAN_POINT('Ctrl Pts',(-55.4378792223867,-61.5417630700155,
-218.464384769625));
#190606=CARTESIAN_POINT('Ctrl Pts',(-55.384946788007,-61.5854798144667,
-218.475282328939));
#190607=CARTESIAN_POINT('Ctrl Pts',(-55.3349600132919,-61.6331274503392,
-218.481502690929));
#190608=CARTESIAN_POINT('Ctrl Pts',(-55.2997615967411,-61.6666787515517,
-218.485882787337));
#190609=CARTESIAN_POINT('Ctrl Pts',(-55.2660236404548,-61.7021800146365,
-218.487943771794));
#190610=CARTESIAN_POINT('Ctrl Pts',(-55.2339673727996,-61.7389489519143,
-218.487950878256));
#190611=CARTESIAN_POINT('Ctrl Pts',(-55.4938952567199,-61.9654919306031,
-218.35005));
#190612=CARTESIAN_POINT('Ctrl Pts',(-55.5605571120519,-61.8331100589488,
-218.35005));
#190613=CARTESIAN_POINT('Ctrl Pts',(-55.6462938793267,-61.7235284039374,
-218.33000081413));
#190614=CARTESIAN_POINT('Ctrl Pts',(-55.796657340851,-61.6580344229345,
-218.254184099553));
#190615=CARTESIAN_POINT('Ctrl Pts',(-55.8476827468257,-61.653839850603,
-218.222689657358));
#190616=CARTESIAN_POINT('Ctrl Pts',(-55.9478088686909,-61.6782199479451,
-218.150610277818));
#190617=CARTESIAN_POINT('Ctrl Pts',(-55.995486790882,-61.7063946791486,
-218.11106824763));
#190618=CARTESIAN_POINT('Ctrl Pts',(-56.1268157801208,-61.8214573400613,
-217.990439031765));
#190619=CARTESIAN_POINT('Ctrl Pts',(-56.1995158790201,-61.9371995248376,
-217.907396389637));
#190620=CARTESIAN_POINT('Ctrl Pts',(-56.3198707039344,-62.1930517563039,
-217.749765554285));
#190621=CARTESIAN_POINT('Ctrl Pts',(-56.3688914254939,-62.3364499780597,
-217.673255297864));
#190622=CARTESIAN_POINT('Ctrl Pts',(-56.4090189474477,-62.4870630585556,
-217.60005));
#190623=CARTESIAN_POINT('Ctrl Pts',(-49.2925903552098,-69.4989817480832,
-217.60005));
#190624=CARTESIAN_POINT('Ctrl Pts',(-49.0991171386076,-69.4468461963775,
-217.336253844649));
#190625=CARTESIAN_POINT('Ctrl Pts',(-48.9443109379934,-69.7210624363875,
-217.233400031701));
#190626=CARTESIAN_POINT('Ctrl Pts',(-49.479508186842,-69.5493508092223,
-217.453006109745));
#190627=CARTESIAN_POINT('Ctrl Pts',(-49.2856293770243,-69.4971059616069,
-217.188797196021));
#190628=CARTESIAN_POINT('Ctrl Pts',(-49.130620489061,-69.7720396651474,
-217.086285690494));
#190629=CARTESIAN_POINT('Ctrl Pts',(-49.6662875276291,-69.5996825510014,
-217.305773775928));
#190630=CARTESIAN_POINT('Ctrl Pts',(-49.4718979894171,-69.5473000765824,
-217.041226996676));
#190631=CARTESIAN_POINT('Ctrl Pts',(-49.3167847015304,-69.8229858522605,
-216.938985563531));
#190632=CARTESIAN_POINT('Ctrl Pts',(-49.8529236261983,-69.6499756930601,
-217.158346534073));
#190633=CARTESIAN_POINT('Ctrl Pts',(-49.6579114178628,-69.5974254266744,
-216.893543128263));
#190634=CARTESIAN_POINT('Ctrl Pts',(-49.502798597092,-69.8738997057058,
-216.791493525167));
#190635=CARTESIAN_POINT('',(-49.8529236261983,-69.6499756930601,-217.158346534073));
#190636=CARTESIAN_POINT('',(-49.5029651331548,-69.874078287392,-216.790767750036));
#190637=CARTESIAN_POINT('Origin',(-49.7228284492359,-70.13275436381,-217.158346534073));
#190638=CARTESIAN_POINT('Origin',(165.63543440526,-11.5819668880935,75.4526175248521));
#190639=CARTESIAN_POINT('Origin',(167.970418940429,-23.6135530814242,73.4534718919959));
#190640=CARTESIAN_POINT('Ctrl Pts',(-56.5555093174817,-63.0368943169927,
-217.153871927429));
#190641=CARTESIAN_POINT('Ctrl Pts',(-56.5025836743465,-62.8382452661243,
-216.892152466627));
#190642=CARTESIAN_POINT('Ctrl Pts',(-56.7788252534563,-62.6825329319095,
-216.79113809033));
#190643=CARTESIAN_POINT('Ctrl Pts',(-56.5067115045409,-62.8537385034605,
-217.302758005793));
#190644=CARTESIAN_POINT('Ctrl Pts',(-56.4539126170321,-62.6555652121921,
-217.041204177849));
#190645=CARTESIAN_POINT('Ctrl Pts',(-56.7295803718938,-62.4998572980931,
-216.940045714159));
#190646=CARTESIAN_POINT('Ctrl Pts',(-56.4578811804683,-62.6704606639105,
-217.451483035533));
#190647=CARTESIAN_POINT('Ctrl Pts',(-56.4051889499832,-62.4726876949562,
-217.190156301151));
#190648=CARTESIAN_POINT('Ctrl Pts',(-56.680302877991,-62.3170582944071,
-217.088794981881));
#190649=CARTESIAN_POINT('Ctrl Pts',(-56.4090189474476,-62.4870630585555,
-217.60005));
#190650=CARTESIAN_POINT('Ctrl Pts',(-56.3564132949791,-62.2896150482124,
-217.339009989763));
#190651=CARTESIAN_POINT('Ctrl Pts',(-56.6309943627598,-62.1341374253209,
-217.237388612086));
#190652=CARTESIAN_POINT('',(-56.7789312838428,-62.6826300027679,-216.790395777257));
#190653=CARTESIAN_POINT('',(-56.5555093174817,-63.0368943169928,-217.153871927429));
#190654=CARTESIAN_POINT('Origin',(-57.0386554992377,-62.9081707097771,-217.153871927429));
#190655=CARTESIAN_POINT('Origin',(10.1481943050527,195.398995247496,121.950798030302));
#190656=CARTESIAN_POINT('Origin',(11.7909588194732,193.492081547376,120.824020637011));
#190657=CARTESIAN_POINT('Ctrl Pts',(-49.8082839038352,-69.6379465523126,
-217.193274451484));
#190658=CARTESIAN_POINT('Ctrl Pts',(-49.6148311193225,-69.5858165064744,
-216.925438823195));
#190659=CARTESIAN_POINT('Ctrl Pts',(-49.4605536752757,-69.8644275978415,
-216.823211012323));
#190660=CARTESIAN_POINT('Ctrl Pts',(-50.2515020504862,-69.7573812885902,
-216.849764285521));
#190661=CARTESIAN_POINT('Ctrl Pts',(-50.0368968810474,-69.6995512741769,
-216.615769374028));
#190662=CARTESIAN_POINT('Ctrl Pts',(-49.8798577876633,-69.9587340309451,
-216.511180111009));
#190663=CARTESIAN_POINT('Ctrl Pts',(-50.6419967392048,-69.8626085463579,
-216.450334359214));
#190664=CARTESIAN_POINT('Ctrl Pts',(-50.4172229593767,-69.8020383794606,
-216.246268361137));
#190665=CARTESIAN_POINT('Ctrl Pts',(-50.2489216341879,-70.0420065040121,
-216.148268825924));
#190666=CARTESIAN_POINT('Ctrl Pts',(-50.9693220996876,-69.9508134594501,
-215.987095704752));
#190667=CARTESIAN_POINT('Ctrl Pts',(-50.7368031033667,-69.8881561760894,
-215.810948949264));
#190668=CARTESIAN_POINT('Ctrl Pts',(-50.558073933031,-70.1119355639638,
-215.727306267195));
#190669=CARTESIAN_POINT('',(-50.9355365677156,-69.9417092155658,-216.034373717099));
#190670=CARTESIAN_POINT('',(-50.5260956696589,-70.1045979817023,-215.770197056231));
#190671=CARTESIAN_POINT('Origin',(-50.8054413907531,-70.4244878863158,-216.034373717099));
#190672=CARTESIAN_POINT('Ctrl Pts',(-50.9355365677156,-69.9417092155658,
-216.034373717099));
#190673=CARTESIAN_POINT('Ctrl Pts',(-50.8116343558523,-69.9083210790241,
-216.205819948822));
#190674=CARTESIAN_POINT('Ctrl Pts',(-50.6790456275845,-69.8725921723588,
-216.368291840782));
#190675=CARTESIAN_POINT('Ctrl Pts',(-50.5382668565241,-69.8346562811456,
-216.522302092547));
#190676=CARTESIAN_POINT('Ctrl Pts',(-50.3916404967027,-69.7951446303954,
-216.682709534816));
#190677=CARTESIAN_POINT('Ctrl Pts',(-50.2361294127355,-69.7532387981495,
-216.83393773326));
#190678=CARTESIAN_POINT('Ctrl Pts',(-50.0722553986644,-69.7090793931224,
-216.976525935756));
#190679=CARTESIAN_POINT('Ctrl Pts',(-50.0007248884689,-69.689803946741,
-217.038765253748));
#190680=CARTESIAN_POINT('Ctrl Pts',(-49.9276005183846,-69.6700990002661,
-217.099357901493));
#190681=CARTESIAN_POINT('Ctrl Pts',(-49.8529236261983,-69.6499756930601,
-217.158346534073));
#190682=CARTESIAN_POINT('Ctrl Pts',(-49.5030054850469,-69.8741215579534,
-216.790591893832));
#190683=CARTESIAN_POINT('Ctrl Pts',(-49.6024122858318,-69.8963860707776,
-216.715257484827));
#190684=CARTESIAN_POINT('Ctrl Pts',(-49.6989189612008,-69.9180032597767,
-216.636941400134));
#190685=CARTESIAN_POINT('Ctrl Pts',(-49.7924273507199,-69.9389873829446,
-216.555586604588));
#190686=CARTESIAN_POINT('Ctrl Pts',(-49.8839999749823,-69.9595371029881,
-216.4759159765));
#190687=CARTESIAN_POINT('Ctrl Pts',(-49.9726976882578,-69.9794801981767,
-216.39333040445));
#190688=CARTESIAN_POINT('Ctrl Pts',(-50.0584047953187,-69.9987982846587,
-216.307747992276));
#190689=CARTESIAN_POINT('Ctrl Pts',(-50.1422610001375,-70.0176991841558,
-216.224013789476));
#190690=CARTESIAN_POINT('Ctrl Pts',(-50.2232547532238,-70.0360021258001,
-216.137409962399));
#190691=CARTESIAN_POINT('Ctrl Pts',(-50.3012483834477,-70.053652984946,
-216.047843888945));
#190692=CARTESIAN_POINT('Ctrl Pts',(-50.3792420136716,-70.0713038440919,
-215.958277815491));
#190693=CARTESIAN_POINT('Ctrl Pts',(-50.4542359145046,-70.088302998853,
-215.865748569618));
#190694=CARTESIAN_POINT('Ctrl Pts',(-50.5260568508924,-70.1045534073545,
-215.770160360593));
#190695=CARTESIAN_POINT('Ctrl Pts',(-56.8374074136193,-64.0949596691002,
-216.027524728913));
#190696=CARTESIAN_POINT('Ctrl Pts',(-56.7751359198338,-63.8612322658189,
-215.850745835606));
#190697=CARTESIAN_POINT('Ctrl Pts',(-57.0010400290729,-63.6829857423181,
-215.767369567569));
#190698=CARTESIAN_POINT('Ctrl Pts',(-56.7544062418932,-63.7834262987405,
-216.468486417733));
#190699=CARTESIAN_POINT('Ctrl Pts',(-56.6940755894548,-63.5569835739616,
-216.264965542136));
#190700=CARTESIAN_POINT('Ctrl Pts',(-56.9355417877511,-63.3885831929649,
-216.168198383641));
#190701=CARTESIAN_POINT('Ctrl Pts',(-56.6561228522777,-63.4145332460213,
-216.852342060961));
#190702=CARTESIAN_POINT('Ctrl Pts',(-56.5983764095674,-63.1977899935455,
-216.620143992135));
#190703=CARTESIAN_POINT('Ctrl Pts',(-56.8580526697591,-63.039825113586,
-216.517093115455));
#190704=CARTESIAN_POINT('Ctrl Pts',(-56.5449338627868,-62.9972008165799,
-217.185865065935));
#190705=CARTESIAN_POINT('Ctrl Pts',(-56.4923730636171,-62.7999211568584,
-216.921403846993));
#190706=CARTESIAN_POINT('Ctrl Pts',(-56.7705238988762,-62.644964025511,
-216.820205369791));
#190707=CARTESIAN_POINT('',(-56.9945525157696,-63.6542608153715,-215.805929292345));
#190708=CARTESIAN_POINT('',(-56.8293274051384,-64.0646324794683,-216.070020447202));
#190709=CARTESIAN_POINT('Origin',(-57.3124735868944,-63.9359088722526,-216.070020447202));
#190710=CARTESIAN_POINT('Ctrl Pts',(-56.9944699555911,-63.6541878226909,
-215.805860863005));
#190711=CARTESIAN_POINT('Ctrl Pts',(-56.9787502340432,-63.5835644531967,
-215.900063590448));
#190712=CARTESIAN_POINT('Ctrl Pts',(-56.9623149510134,-63.5098655678024,
-215.991340416441));
#190713=CARTESIAN_POINT('Ctrl Pts',(-56.9452529548364,-63.4332525162424,
-216.079782169333));
#190714=CARTESIAN_POINT('Ctrl Pts',(-56.9277954510961,-63.3548635270355,
-216.170274056442));
#190715=CARTESIAN_POINT('Ctrl Pts',(-56.9096816135882,-63.2734234339984,
-216.257798849252));
#190716=CARTESIAN_POINT('Ctrl Pts',(-56.8909632509908,-63.1890692673191,
-216.34244940172));
#190717=CARTESIAN_POINT('Ctrl Pts',(-56.8716003694178,-63.1018105805022,
-216.430014679612));
#190718=CARTESIAN_POINT('Ctrl Pts',(-56.8515902874278,-63.0114333079711,
-216.514505339738));
#190719=CARTESIAN_POINT('Ctrl Pts',(-56.8309486552413,-62.918056159024,
-216.596004588349));
#190720=CARTESIAN_POINT('Ctrl Pts',(-56.8140435960204,-62.8415822533479,
-216.662750745425));
#190721=CARTESIAN_POINT('Ctrl Pts',(-56.7967139865683,-62.7630954660381,
-216.727490258555));
#190722=CARTESIAN_POINT('Ctrl Pts',(-56.7789516318256,-62.6826486313538,
-216.790253322115));
#190723=CARTESIAN_POINT('Ctrl Pts',(-56.5555093174817,-63.0368943169928,
-217.153871927429));
#190724=CARTESIAN_POINT('Ctrl Pts',(-56.6017653589548,-63.2105099443376,
-217.012740999607));
#190725=CARTESIAN_POINT('Ctrl Pts',(-56.6457145720419,-63.3754672117225,
-216.862817131854));
#190726=CARTESIAN_POINT('Ctrl Pts',(-56.6872100613017,-63.53121476751,-216.703540565444));
#190727=CARTESIAN_POINT('Ctrl Pts',(-56.7270307212962,-63.6806760842605,
-216.550692675005));
#190728=CARTESIAN_POINT('Ctrl Pts',(-56.7645917777113,-63.8216562928037,
-216.389231897203));
#190729=CARTESIAN_POINT('Ctrl Pts',(-56.7997545451796,-63.9536348568741,
-216.218629552571));
#190730=CARTESIAN_POINT('Ctrl Pts',(-56.809809462033,-63.9913745907946,
-216.169845212947));
#190731=CARTESIAN_POINT('Ctrl Pts',(-56.8196682125201,-64.0283780415039,
-216.120313149196));
#190732=CARTESIAN_POINT('Ctrl Pts',(-56.8293274051384,-64.0646324794683,
-216.070020447202));
#190733=CARTESIAN_POINT('Ctrl Pts',(-51.8506358032468,-69.9286975854491,
-213.227536545097));
#190734=CARTESIAN_POINT('Ctrl Pts',(-51.9051927775541,-69.878934733823,
-213.231804164287));
#190735=CARTESIAN_POINT('Ctrl Pts',(-51.9718267086835,-69.8471376007481,
-213.236262748316));
#190736=CARTESIAN_POINT('Ctrl Pts',(-51.8365119911318,-69.9357794545355,
-213.472190089507));
#190737=CARTESIAN_POINT('Ctrl Pts',(-51.8922394802453,-69.8844506593677,
-213.488613551225));
#190738=CARTESIAN_POINT('Ctrl Pts',(-51.9608269631738,-69.8523865837487,
-213.505363447503));
#190739=CARTESIAN_POINT('Ctrl Pts',(-51.764852960797,-69.9722040426621,
-213.699187231714));
#190740=CARTESIAN_POINT('Ctrl Pts',(-51.8262156776006,-69.9127229374064,
-213.727945792467));
#190741=CARTESIAN_POINT('Ctrl Pts',(-51.9055967467288,-69.8788950207841,
-213.755167329611));
#190742=CARTESIAN_POINT('Ctrl Pts',(-51.5795633434493,-70.0451552734412,
-214.141675371395));
#190743=CARTESIAN_POINT('Ctrl Pts',(-51.6562512817975,-69.9633349698509,
-214.190606504019));
#190744=CARTESIAN_POINT('Ctrl Pts',(-51.7621689112058,-69.9305269210584,
-214.242088767328));
#190745=CARTESIAN_POINT('Ctrl Pts',(-51.4650229856105,-70.0818854461224,
-214.356506299955));
#190746=CARTESIAN_POINT('Ctrl Pts',(-51.5502085021597,-69.9858444846014,
-214.415523245079));
#190747=CARTESIAN_POINT('Ctrl Pts',(-51.6732637051828,-69.9557792147167,
-214.478511967556));
#190748=CARTESIAN_POINT('Ctrl Pts',(-51.0983339320408,-70.159079780817,
-214.982290817329));
#190749=CARTESIAN_POINT('Ctrl Pts',(-51.2098831872327,-70.0159755958657,
-215.071812476474));
#190750=CARTESIAN_POINT('Ctrl Pts',(-51.3873507266844,-70.0045324525619,
-215.167197191036));
#190751=CARTESIAN_POINT('Ctrl Pts',(-50.818061750232,-70.1707056698672,
-215.381706149951));
#190752=CARTESIAN_POINT('Ctrl Pts',(-50.9474626754076,-69.9829235319172,
-215.48727868552));
#190753=CARTESIAN_POINT('Ctrl Pts',(-51.16741865858,-70.0041948709461,-215.606559872798));
#190754=CARTESIAN_POINT('Ctrl Pts',(-50.5261810352842,-70.1046957156775,
-215.770277860521));
#190755=CARTESIAN_POINT('Ctrl Pts',(-50.704122433655,-69.8793496612892,
-215.854989245265));
#190756=CARTESIAN_POINT('Ctrl Pts',(-50.9355365677157,-69.9417092155658,
-216.034373717099));
#190757=CARTESIAN_POINT('',(-51.9718267086745,-69.8471376007524,-213.236262748316));
#190758=CARTESIAN_POINT('',(-51.8506358032439,-69.9286975854465,-213.227536545096));
#190759=CARTESIAN_POINT('Origin',(-52.1871615786983,-70.2983923998978,-213.236262748316));
#190760=CARTESIAN_POINT('Ctrl Pts',(-51.9718267086745,-69.8471376007524,
-213.236262748316));
#190761=CARTESIAN_POINT('Ctrl Pts',(-51.9608269631738,-69.8523865837487,
-213.505363447503));
#190762=CARTESIAN_POINT('Ctrl Pts',(-51.9055967467288,-69.8788950207841,
-213.755167329611));
#190763=CARTESIAN_POINT('Ctrl Pts',(-51.7621689112058,-69.9305269210584,
-214.242088767328));
#190764=CARTESIAN_POINT('Ctrl Pts',(-51.6732637051828,-69.9557792147167,
-214.478511967556));
#190765=CARTESIAN_POINT('Ctrl Pts',(-51.3873507266844,-70.0045324525619,
-215.167197191036));
#190766=CARTESIAN_POINT('Ctrl Pts',(-51.16741865858,-70.0041948709461,-215.606559872798));
#190767=CARTESIAN_POINT('Ctrl Pts',(-50.9355365677156,-69.9417092155658,
-216.034373717099));
#190768=CARTESIAN_POINT('Ctrl Pts',(-50.5261810442127,-70.1046957176967,
-215.770277848635));
#190769=CARTESIAN_POINT('Ctrl Pts',(-50.8180617559476,-70.1707056696301,
-215.381706141806));
#190770=CARTESIAN_POINT('Ctrl Pts',(-51.0983339345335,-70.1590797802923,
-214.982290813075));
#190771=CARTESIAN_POINT('Ctrl Pts',(-51.4650229856105,-70.0818854461224,
-214.356506299955));
#190772=CARTESIAN_POINT('Ctrl Pts',(-51.5795633434493,-70.0451552734412,
-214.141675371395));
#190773=CARTESIAN_POINT('Ctrl Pts',(-51.764852960797,-69.9722040426621,
-213.699187231714));
#190774=CARTESIAN_POINT('Ctrl Pts',(-51.8365119911318,-69.9357794545355,
-213.472190089507));
#190775=CARTESIAN_POINT('Ctrl Pts',(-51.8506358032439,-69.9286975854465,
-213.227536545096));
#190776=CARTESIAN_POINT('Ctrl Pts',(-56.9946437140725,-63.654341638523,
-215.806005173342));
#190777=CARTESIAN_POINT('Ctrl Pts',(-56.7673159108321,-63.831880948128,
-215.890327243741));
#190778=CARTESIAN_POINT('Ctrl Pts',(-56.8293274051384,-64.0646324794683,
-216.070020447202));
#190779=CARTESIAN_POINT('Ctrl Pts',(-57.0593493067881,-63.9452064704916,
-215.417908776751));
#190780=CARTESIAN_POINT('Ctrl Pts',(-56.8699337341761,-64.0745035962365,
-215.52327792109));
#190781=CARTESIAN_POINT('Ctrl Pts',(-56.8908615653413,-64.2955924035464,
-215.642832329437));
#190782=CARTESIAN_POINT('Ctrl Pts',(-57.0473852485484,-64.223762372941,
-215.01984571743));
#190783=CARTESIAN_POINT('Ctrl Pts',(-56.9027383376601,-64.3353675625261,
-215.109528851524));
#190784=CARTESIAN_POINT('Ctrl Pts',(-56.8910066584284,-64.5140548708215,
-215.205129354443));
#190785=CARTESIAN_POINT('Ctrl Pts',(-56.9693188990643,-64.5910795515543,
-214.391115626198));
#190786=CARTESIAN_POINT('Ctrl Pts',(-56.8722601349262,-64.6764145103723,
-214.450264068639));
#190787=CARTESIAN_POINT('Ctrl Pts',(-56.8418253372028,-64.8002473979207,
-214.513441216471));
#190788=CARTESIAN_POINT('Ctrl Pts',(-56.9323676074197,-64.7055133030553,
-214.175785907962));
#190789=CARTESIAN_POINT('Ctrl Pts',(-56.8496536435939,-64.782388944382,
-214.224865863035));
#190790=CARTESIAN_POINT('Ctrl Pts',(-56.8164834138299,-64.8889909543264,
-214.276550655991));
#190791=CARTESIAN_POINT('Ctrl Pts',(-56.858924334145,-64.8909827727899,
-213.732482787358));
#190792=CARTESIAN_POINT('Ctrl Pts',(-56.7988096612268,-64.9525255862112,
-213.761447447143));
#190793=CARTESIAN_POINT('Ctrl Pts',(-56.7646526681549,-65.0323886578414,
-213.78887047881));
#190794=CARTESIAN_POINT('Ctrl Pts',(-56.8216885415319,-64.9639058228799,
-213.501324323514));
#190795=CARTESIAN_POINT('Ctrl Pts',(-56.7699730410421,-65.019697176522,
-213.517778991486));
#190796=CARTESIAN_POINT('Ctrl Pts',(-56.7376407413534,-65.088500914211,
-213.534553551187));
#190797=CARTESIAN_POINT('Ctrl Pts',(-56.8144552965912,-64.9781464054153,
-213.256094899171));
#190798=CARTESIAN_POINT('Ctrl Pts',(-56.7643939904929,-65.0327211703679,
-213.2603619646));
#190799=CARTESIAN_POINT('Ctrl Pts',(-56.7323722878852,-65.0994854859681,
-213.26482110239));
#190800=CARTESIAN_POINT('',(-56.8144552965909,-64.9781464054155,-213.256094899172));
#190801=CARTESIAN_POINT('',(-56.7323722878851,-65.0994854859682,-213.264821102391));
#190802=CARTESIAN_POINT('Origin',(-57.1832000972235,-65.315712880919,-213.264821102391));
#190803=CARTESIAN_POINT('Ctrl Pts',(-56.8144552965909,-64.9781464054155,
-213.256094899172));
#190804=CARTESIAN_POINT('Ctrl Pts',(-56.8216885415319,-64.9639058228799,
-213.501324323514));
#190805=CARTESIAN_POINT('Ctrl Pts',(-56.858924334145,-64.8909827727899,
-213.732482787358));
#190806=CARTESIAN_POINT('Ctrl Pts',(-56.9323676074197,-64.7055133030553,
-214.175785907962));
#190807=CARTESIAN_POINT('Ctrl Pts',(-56.9693188990643,-64.5910795515543,
-214.391115626198));
#190808=CARTESIAN_POINT('Ctrl Pts',(-57.0473852477809,-64.2237623765521,
-215.019845711248));
#190809=CARTESIAN_POINT('Ctrl Pts',(-57.0593493064353,-63.9452064787071,
-215.417908765011));
#190810=CARTESIAN_POINT('Ctrl Pts',(-56.9946437169351,-63.6543416513909,
-215.806005156172));
#190811=CARTESIAN_POINT('Ctrl Pts',(-56.8293274051384,-64.0646324794683,
-216.070020447202));
#190812=CARTESIAN_POINT('Ctrl Pts',(-56.8908615653413,-64.2955924035464,
-215.642832329437));
#190813=CARTESIAN_POINT('Ctrl Pts',(-56.8910066584284,-64.5140548708215,
-215.205129354443));
#190814=CARTESIAN_POINT('Ctrl Pts',(-56.8418253372028,-64.8002473979207,
-214.513441216471));
#190815=CARTESIAN_POINT('Ctrl Pts',(-56.8164834138299,-64.8889909543264,
-214.276550655991));
#190816=CARTESIAN_POINT('Ctrl Pts',(-56.7646526681549,-65.0323886578414,
-213.78887047881));
#190817=CARTESIAN_POINT('Ctrl Pts',(-56.7376407413534,-65.088500914211,
-213.534553551187));
#190818=CARTESIAN_POINT('Ctrl Pts',(-56.7323722878851,-65.0994854859682,
-213.264821102391));
#190819=CARTESIAN_POINT('Ctrl Pts',(-51.9513667677563,-69.856765622058,
-213.744232219612));
#190820=CARTESIAN_POINT('Ctrl Pts',(-51.8804433982802,-69.8893245968629,
-213.7397430898));
#190821=CARTESIAN_POINT('Ctrl Pts',(-51.8228503443836,-69.941996586685,
-213.735470748631));
#190822=CARTESIAN_POINT('Ctrl Pts',(-51.991780071228,-69.8379778346573,
-212.728235356937));
#190823=CARTESIAN_POINT('Ctrl Pts',(-51.92847890016,-69.8695011096845,-212.726011510236));
#190824=CARTESIAN_POINT('Ctrl Pts',(-51.8765276514693,-69.9171366797835,
-212.719415019637));
#190825=CARTESIAN_POINT('Ctrl Pts',(-52.0346456619607,-69.816925009228,
-211.71249177384));
#190826=CARTESIAN_POINT('Ctrl Pts',(-51.9794687356775,-69.8470038946562,
-211.710263762613));
#190827=CARTESIAN_POINT('Ctrl Pts',(-51.9334544096019,-69.8892734758674,
-211.703692143478));
#190828=CARTESIAN_POINT('Ctrl Pts',(-52.1138191538044,-69.7700067918124,
-210.276283653453));
#190829=CARTESIAN_POINT('Ctrl Pts',(-52.0734597321496,-69.7950116391772,
-210.272241986443));
#190830=CARTESIAN_POINT('Ctrl Pts',(-52.0385712075063,-69.827125844513,
-210.267504272468));
#190831=CARTESIAN_POINT('Ctrl Pts',(-52.1391384959575,-69.7543237267294,
-209.854167521602));
#190832=CARTESIAN_POINT('Ctrl Pts',(-52.1034382988765,-69.7775433560356,
-209.850130119974));
#190833=CARTESIAN_POINT('Ctrl Pts',(-52.0721853887123,-69.8063480382507,
-209.845388043713));
#190834=CARTESIAN_POINT('Ctrl Pts',(-52.1868109938527,-69.7218145199576,
-209.222414495584));
#190835=CARTESIAN_POINT('Ctrl Pts',(-52.1597481032178,-69.740831362429,
-209.21810272547));
#190836=CARTESIAN_POINT('Ctrl Pts',(-52.1354652353082,-69.7632628363318,
-209.213638050098));
#190837=CARTESIAN_POINT('Ctrl Pts',(-52.2041584674497,-69.7096301545639,
-209.011927312326));
#190838=CARTESIAN_POINT('Ctrl Pts',(-52.1802056110659,-69.7270298301123,
-209.007617928732));
#190839=CARTESIAN_POINT('Ctrl Pts',(-52.158491006019,-69.7471128108018,
-209.003150816985));
#190840=CARTESIAN_POINT('Ctrl Pts',(-52.2371408246248,-69.6848794419398,
-208.698381586053));
#190841=CARTESIAN_POINT('Ctrl Pts',(-52.2190101918289,-69.6987724358088,
-208.694007820048));
#190842=CARTESIAN_POINT('Ctrl Pts',(-52.2022638893194,-69.714299255283,
-208.689605786204));
#190843=CARTESIAN_POINT('Ctrl Pts',(-52.249174245292,-69.6756642254024,
-208.594104390417));
#190844=CARTESIAN_POINT('Ctrl Pts',(-52.2331514504352,-69.6882319207143,
-208.589731796556));
#190845=CARTESIAN_POINT('Ctrl Pts',(-52.2182336078508,-69.7020812266944,
-208.585328566142));
#190846=CARTESIAN_POINT('Ctrl Pts',(-52.2723150773139,-69.6570951860835,
-208.439912289689));
#190847=CARTESIAN_POINT('Ctrl Pts',(-52.2602903339987,-69.6668890135686,
-208.435525620945));
#190848=CARTESIAN_POINT('Ctrl Pts',(-52.2489412320906,-69.677457827406,
-208.431136608511));
#190849=CARTESIAN_POINT('Ctrl Pts',(-52.2807846875617,-69.6502015352889,
-208.388797146169));
#190850=CARTESIAN_POINT('Ctrl Pts',(-52.270214924355,-69.6589558945369,
-208.384411029018));
#190851=CARTESIAN_POINT('Ctrl Pts',(-52.26018000973,-69.6683161240624,-208.380021453291));
#190852=CARTESIAN_POINT('Ctrl Pts',(-52.2972292893049,-69.6363602565428,
-208.314505613017));
#190853=CARTESIAN_POINT('Ctrl Pts',(-52.2894520983595,-69.6429772988715,
-208.310116951883));
#190854=CARTESIAN_POINT('Ctrl Pts',(-52.281999678196,-69.6499593019997,
-208.305729941084));
#190855=CARTESIAN_POINT('Ctrl Pts',(-52.3032976103578,-69.6311990926332,
-208.290014406272));
#190856=CARTESIAN_POINT('Ctrl Pts',(-52.2965464863421,-69.6370140514492,
-208.285625985819));
#190857=CARTESIAN_POINT('Ctrl Pts',(-52.2900513245555,-69.6431141725604,
-208.281238728998));
#190858=CARTESIAN_POINT('Ctrl Pts',(-52.3149497431651,-69.6210491476294,
-208.256089330814));
#190859=CARTESIAN_POINT('Ctrl Pts',(-52.3101508205055,-69.6252622995574,
-208.251700725001));
#190860=CARTESIAN_POINT('Ctrl Pts',(-52.3055109262684,-69.6296515882696,
-208.24731365204));
#190861=CARTESIAN_POINT('Ctrl Pts',(-52.3192905030199,-69.6172377131638,
-208.245104578722));
#190862=CARTESIAN_POINT('Ctrl Pts',(-52.3152163853501,-69.6208465529984,
-208.24071608881));
#190863=CARTESIAN_POINT('Ctrl Pts',(-52.3112700002316,-69.624596121335,
-208.236328897454));
#190864=CARTESIAN_POINT('Ctrl Pts',(-52.3980737175552,-69.546924914442,
-208.107889777235));
#190865=CARTESIAN_POINT('Ctrl Pts',(-52.4070413724991,-69.5392973207823,
-208.103538654047));
#190866=CARTESIAN_POINT('Ctrl Pts',(-52.4157911999454,-69.5313285632377,
-208.099113657561));
#190867=CARTESIAN_POINT('Ctrl Pts',(-52.6906841717837,-69.273483049227,
-208.269888341076));
#190868=CARTESIAN_POINT('Ctrl Pts',(-52.7473775130203,-69.2207759621715,
-208.265385690945));
#190869=CARTESIAN_POINT('Ctrl Pts',(-52.8039539674267,-69.1685749088725,
-208.261113958564));
#190870=CARTESIAN_POINT('Ctrl Pts',(-53.1203834433686,-68.5685596498648,
-225.080427005024));
#190871=CARTESIAN_POINT('Ctrl Pts',(-53.2526829041072,-68.3309162879946,
-225.681318331167));
#190872=CARTESIAN_POINT('Ctrl Pts',(-53.3726051882034,-68.2329805102018,
-225.065027635246));
#190873=CARTESIAN_POINT('',(-52.3440043138885,-69.594874440935,-208.218811515427));
#190874=CARTESIAN_POINT('',(-52.3440560052495,-69.5949303622595,-208.210085312208));
#190875=CARTESIAN_POINT('Origin',(-52.6833983856504,-69.9620415201413,-208.218811515427));
#190876=CARTESIAN_POINT('Ctrl Pts',(-52.3440043138885,-69.594874440935,
-208.218811515427));
#190877=CARTESIAN_POINT('Ctrl Pts',(-52.3364108319347,-69.6018935417895,
-208.21881325288));
#190878=CARTESIAN_POINT('Ctrl Pts',(-52.3299368833625,-69.6077359836068,
-208.22656203798));
#190879=CARTESIAN_POINT('Ctrl Pts',(-52.3192905030199,-69.6172377131638,
-208.245104578722));
#190880=CARTESIAN_POINT('Ctrl Pts',(-52.3149497431651,-69.6210491476294,
-208.256089330814));
#190881=CARTESIAN_POINT('Ctrl Pts',(-52.3032976103578,-69.6311990926332,
-208.290014406272));
#190882=CARTESIAN_POINT('Ctrl Pts',(-52.2972292893049,-69.6363602565428,
-208.314505613017));
#190883=CARTESIAN_POINT('Ctrl Pts',(-52.2807846875617,-69.6502015352889,
-208.388797146169));
#190884=CARTESIAN_POINT('Ctrl Pts',(-52.2723150773139,-69.6570951860835,
-208.439912289689));
#190885=CARTESIAN_POINT('Ctrl Pts',(-52.249174245292,-69.6756642254024,
-208.594104390417));
#190886=CARTESIAN_POINT('Ctrl Pts',(-52.2371408246248,-69.6848794419398,
-208.698381586053));
#190887=CARTESIAN_POINT('Ctrl Pts',(-52.2041584674497,-69.7096301545639,
-209.011927312326));
#190888=CARTESIAN_POINT('Ctrl Pts',(-52.1868109938527,-69.7218145199576,
-209.222414495584));
#190889=CARTESIAN_POINT('Ctrl Pts',(-52.1391384959575,-69.7543237267294,
-209.854167521602));
#190890=CARTESIAN_POINT('Ctrl Pts',(-52.1138191538044,-69.7700067918124,
-210.276283653453));
#190891=CARTESIAN_POINT('Ctrl Pts',(-52.0439601904129,-69.8114052189438,
-211.543526112619));
#190892=CARTESIAN_POINT('Ctrl Pts',(-52.0064303120272,-69.8306250618399,
-212.389708318565));
#190893=CARTESIAN_POINT('Ctrl Pts',(-51.9718267086745,-69.8471376007524,
-213.236262748316));
#190894=CARTESIAN_POINT('Ctrl Pts',(-51.8506358032439,-69.9286975854465,
-213.227536545096));
#190895=CARTESIAN_POINT('Ctrl Pts',(-51.8965359306666,-69.9068955059224,
-212.381067577369));
#190896=CARTESIAN_POINT('Ctrl Pts',(-51.9463091177219,-69.8815088904097,
-211.535021517202));
#190897=CARTESIAN_POINT('Ctrl Pts',(-52.0389353307874,-69.8267824525318,
-210.267914982609));
#190898=CARTESIAN_POINT('Ctrl Pts',(-52.0725035102325,-69.806045505995,
-209.8458402758));
#190899=CARTESIAN_POINT('Ctrl Pts',(-52.1356910661391,-69.7630436587203,
-209.214130441658));
#190900=CARTESIAN_POINT('Ctrl Pts',(-52.1586824184498,-69.7469248062077,
-209.003656181328));
#190901=CARTESIAN_POINT('Ctrl Pts',(-52.2023855392512,-69.7141755312691,
-208.690099641439));
#190902=CARTESIAN_POINT('Ctrl Pts',(-52.2183291852341,-69.7019815954277,
-208.585816112664));
#190903=CARTESIAN_POINT('Ctrl Pts',(-52.2489833267826,-69.6774084341258,
-208.431581516949));
#190904=CARTESIAN_POINT('Ctrl Pts',(-52.2602021616247,-69.6682855321809,
-208.380448072074));
#190905=CARTESIAN_POINT('Ctrl Pts',(-52.2819812944307,-69.6499675527577,
-208.306095531171));
#190906=CARTESIAN_POINT('Ctrl Pts',(-52.2900177211888,-69.6431370963428,
-208.281577994998));
#190907=CARTESIAN_POINT('Ctrl Pts',(-52.3054538148208,-69.6296980513237,
-208.247576563664));
#190908=CARTESIAN_POINT('Ctrl Pts',(-52.3112042959167,-69.6246512725098,
-208.236560595082));
#190909=CARTESIAN_POINT('Ctrl Pts',(-52.3253253083163,-69.6120530454534,
-208.217923065672));
#190910=CARTESIAN_POINT('Ctrl Pts',(-52.3341567138414,-69.6040808580668,
-208.210085312176));
#190911=CARTESIAN_POINT('Ctrl Pts',(-52.3440560052495,-69.5949303622595,
-208.210085312208));
#190912=CARTESIAN_POINT('Ctrl Pts',(-56.478494115784,-65.4721095684411,
-208.218811515427));
#190913=CARTESIAN_POINT('Ctrl Pts',(-56.4784941157842,-65.4721095684412,
-208.214448081532));
#190914=CARTESIAN_POINT('Ctrl Pts',(-56.4785498900846,-65.4721614184049,
-208.210085312209));
#190915=CARTESIAN_POINT('Ctrl Pts',(-56.4856347339016,-65.464428502687,
-208.218813480809));
#190916=CARTESIAN_POINT('Ctrl Pts',(-56.4867940706151,-65.4631813685704,
-208.214450046893));
#190917=CARTESIAN_POINT('Ctrl Pts',(-56.4880093612199,-65.4619859436241,
-208.210087277606));
#190918=CARTESIAN_POINT('Ctrl Pts',(-56.4916787645948,-65.4577664915776,
-208.226946403507));
#190919=CARTESIAN_POINT('Ctrl Pts',(-56.4938064756652,-65.455425583918,
-208.222583010898));
#190920=CARTESIAN_POINT('Ctrl Pts',(-56.4960155064695,-65.4531598633657,
-208.218220200296));
#190921=CARTESIAN_POINT('Ctrl Pts',(-56.5012774655679,-65.4470659442998,
-208.245963459985));
#190922=CARTESIAN_POINT('Ctrl Pts',(-56.5049328760549,-65.4429598777431,
-208.241599714584));
#190923=CARTESIAN_POINT('Ctrl Pts',(-56.5087297972239,-65.4389829337676,
-208.237237256758));
#190924=CARTESIAN_POINT('Ctrl Pts',(-56.5051439252244,-65.4426842233343,
-208.257244986379));
#190925=CARTESIAN_POINT('Ctrl Pts',(-56.5094087292744,-65.4378503136699,
-208.25288112094));
#190926=CARTESIAN_POINT('Ctrl Pts',(-56.5138509238801,-65.4331773923495,
-208.248518783163));
#190927=CARTESIAN_POINT('Ctrl Pts',(-56.5153591918106,-65.4310145177164,
-208.291764410647));
#190928=CARTESIAN_POINT('Ctrl Pts',(-56.5212265334526,-65.4242355589788,
-208.287400749103));
#190929=CARTESIAN_POINT('Ctrl Pts',(-56.5273807159321,-65.4177153790657,
-208.283038207423));
#190930=CARTESIAN_POINT('Ctrl Pts',(-56.5204776688227,-65.4250252363654,
-208.316259455579));
#190931=CARTESIAN_POINT('Ctrl Pts',(-56.5271357114541,-65.4172387338904,
-208.311895535072));
#190932=CARTESIAN_POINT('Ctrl Pts',(-56.5341593626729,-65.4097792264604,
-208.307533252362));
#190933=CARTESIAN_POINT('Ctrl Pts',(-56.5343427956335,-65.4086346803882,
-208.391050209511));
#190934=CARTESIAN_POINT('Ctrl Pts',(-56.5431294167638,-65.3980791094533,
-208.386688866059));
#190935=CARTESIAN_POINT('Ctrl Pts',(-56.5525209588637,-65.3880602085305,
-208.38232400629));
#190936=CARTESIAN_POINT('Ctrl Pts',(-56.5412952751588,-65.4001361493426,
-208.442727536444));
#190937=CARTESIAN_POINT('Ctrl Pts',(-56.5511242891444,-65.3881281081246,
-208.438365624418));
#190938=CARTESIAN_POINT('Ctrl Pts',(-56.5617269524415,-65.3767978707557,
-208.434001333226));
#190939=CARTESIAN_POINT('Ctrl Pts',(-56.5599119337509,-65.3770518735271,
-208.597713229276));
#190940=CARTESIAN_POINT('Ctrl Pts',(-56.5725061054697,-65.3610757695375,
-208.59336548035));
#190941=CARTESIAN_POINT('Ctrl Pts',(-56.5863764886281,-65.3462052619613,
-208.588987026056));
#190942=CARTESIAN_POINT('Ctrl Pts',(-56.5691529780988,-65.365046299052,
-208.702360956951));
#190943=CARTESIAN_POINT('Ctrl Pts',(-56.5830688742296,-65.3469778303877,
-208.698012046015));
#190944=CARTESIAN_POINT('Ctrl Pts',(-56.5986098697023,-65.3302929526477,
-208.693634753733));
#190945=CARTESIAN_POINT('Ctrl Pts',(-56.594014810857,-65.3320840644752,
-209.017499153971));
#190946=CARTESIAN_POINT('Ctrl Pts',(-56.6114339742289,-65.3082260137793,
-209.013214961635));
#190947=CARTESIAN_POINT('Ctrl Pts',(-56.6315194173109,-65.2866023733443,
-209.008772950752));
#190948=CARTESIAN_POINT('Ctrl Pts',(-56.6062646503943,-65.3147324550994,
-209.229067091402));
#190949=CARTESIAN_POINT('Ctrl Pts',(-56.6253012100655,-65.2877789793426,
-209.224780476847));
#190950=CARTESIAN_POINT('Ctrl Pts',(-56.6477298291647,-65.2635998038976,
-209.220340888184));
#190951=CARTESIAN_POINT('Ctrl Pts',(-56.6389405444651,-65.2670590859439,
-209.863840624216));
#190952=CARTESIAN_POINT('Ctrl Pts',(-56.6621798760702,-65.2315103701136,
-209.859829541482));
#190953=CARTESIAN_POINT('Ctrl Pts',(-56.6909645146964,-65.2003964473429,
-209.855114420997));
#190954=CARTESIAN_POINT('Ctrl Pts',(-56.6547249564177,-65.2417076178786,
-210.288240216126));
#190955=CARTESIAN_POINT('Ctrl Pts',(-56.6797528213393,-65.2015162456806,
-210.284225552072));
#190956=CARTESIAN_POINT('Ctrl Pts',(-56.7118396592687,-65.1667799745591,
-210.279514012908));
#190957=CARTESIAN_POINT('Ctrl Pts',(-56.6963931899382,-65.1717493422662,
-211.562592707913));
#190958=CARTESIAN_POINT('Ctrl Pts',(-56.7258904584642,-65.1185576981398,
-211.559720606721));
#190959=CARTESIAN_POINT('Ctrl Pts',(-56.7669337250065,-65.0740063908786,
-211.553866504694));
#190960=CARTESIAN_POINT('Ctrl Pts',(-56.7157486990471,-65.1341451836486,
-212.413730817787));
#190961=CARTESIAN_POINT('Ctrl Pts',(-56.7467526277092,-65.0738827156515,
-212.410853939053));
#190962=CARTESIAN_POINT('Ctrl Pts',(-56.7925037337705,-65.0241267882654,
-212.404990365038));
#190963=CARTESIAN_POINT('Ctrl Pts',(-56.7323722878852,-65.0994854859681,
-213.264821102391));
#190964=CARTESIAN_POINT('Ctrl Pts',(-56.7643939904929,-65.0327211703679,
-213.2603619646));
#190965=CARTESIAN_POINT('Ctrl Pts',(-56.8144552965912,-64.9781464054152,
-213.256094899172));
#190966=CARTESIAN_POINT('',(-56.4785498900846,-65.4721614184049,-208.210085312208));
#190967=CARTESIAN_POINT('',(-56.478494115784,-65.4721095684411,-208.218811515426));
#190968=CARTESIAN_POINT('Origin',(-56.8446958677552,-65.8125449908831,-208.218811515427));
#190969=CARTESIAN_POINT('Ctrl Pts',(-56.4785498900846,-65.4721614184049,
-208.210085312209));
#190970=CARTESIAN_POINT('Ctrl Pts',(-56.4880134607985,-65.4619815336005,
-208.210087283952));
#190971=CARTESIAN_POINT('Ctrl Pts',(-56.4960210114868,-65.4531537245717,
-208.218228453105));
#190972=CARTESIAN_POINT('Ctrl Pts',(-56.5023726430475,-65.4460714077127,
-208.227728741309));
#190973=CARTESIAN_POINT('Ctrl Pts',(-56.5087366507261,-65.4389752909997,
-208.23724754077));
#190974=CARTESIAN_POINT('Ctrl Pts',(-56.513854727351,-65.433173044492,-208.248528534057));
#190975=CARTESIAN_POINT('Ctrl Pts',(-56.5183608448225,-65.4280233981992,
-208.260025266392));
#190976=CARTESIAN_POINT('Ctrl Pts',(-56.527384064744,-65.4177115518456,
-208.283046757708));
#190977=CARTESIAN_POINT('Ctrl Pts',(-56.5341620389057,-65.4097760673606,
-208.307543894395));
#190978=CARTESIAN_POINT('Ctrl Pts',(-56.5402792876314,-65.4025401997578,
-208.332463842479));
#190979=CARTESIAN_POINT('Ctrl Pts',(-56.5525225633485,-65.3880580810659,
-208.382339498829));
#190980=CARTESIAN_POINT('Ctrl Pts',(-56.5617281325892,-65.3767964110653,
-208.434008552021));
#190981=CARTESIAN_POINT('Ctrl Pts',(-56.5699429720804,-65.3666008613971,
-208.485663414341));
#190982=CARTESIAN_POINT('Ctrl Pts',(-56.5863768923929,-65.346204498088,
-208.588999808438));
#190983=CARTESIAN_POINT('Ctrl Pts',(-56.5986107835984,-65.3302917454577,
-208.693643261059));
#190984=CARTESIAN_POINT('Ctrl Pts',(-56.6095793668545,-65.3157298046138,
-208.79868090921));
#190985=CARTESIAN_POINT('Ctrl Pts',(-56.6315196526886,-65.2866017817001,
-209.008786076848));
#190986=CARTESIAN_POINT('Ctrl Pts',(-56.6477302855814,-65.2635991432574,
-209.220347327344));
#190987=CARTESIAN_POINT('Ctrl Pts',(-56.6621411615825,-65.2425322660162,
-209.431932106333));
#190988=CARTESIAN_POINT('Ctrl Pts',(-56.6909646006573,-65.200396045247,
-209.855126434415));
#190989=CARTESIAN_POINT('Ctrl Pts',(-56.7118400320305,-65.1667793523224,
-210.279522418803));
#190990=CARTESIAN_POINT('Ctrl Pts',(-56.7302042319515,-65.1358555723291,
-210.704298191087));
#190991=CARTESIAN_POINT('Ctrl Pts',(-56.7669339286709,-65.0740058285095,
-211.553879733264));
#190992=CARTESIAN_POINT('Ctrl Pts',(-56.7925011773325,-65.0241321427268,
-212.404891259688));
#190993=CARTESIAN_POINT('Ctrl Pts',(-56.8144552965909,-64.9781464054155,
-213.256094899172));
#190994=CARTESIAN_POINT('Ctrl Pts',(-56.7323722878851,-65.0994854859682,
-213.264821102391));
#190995=CARTESIAN_POINT('Ctrl Pts',(-56.7157486990471,-65.1341451836486,
-212.413730817787));
#190996=CARTESIAN_POINT('Ctrl Pts',(-56.6963931899382,-65.1717493422662,
-211.562592707913));
#190997=CARTESIAN_POINT('Ctrl Pts',(-56.6547249564177,-65.2417076178786,
-210.288240216126));
#190998=CARTESIAN_POINT('Ctrl Pts',(-56.6389405444651,-65.2670590859439,
-209.863840624216));
#190999=CARTESIAN_POINT('Ctrl Pts',(-56.6062646503943,-65.3147324550994,
-209.229067091402));
#191000=CARTESIAN_POINT('Ctrl Pts',(-56.594014810857,-65.3320840644752,
-209.017499153971));
#191001=CARTESIAN_POINT('Ctrl Pts',(-56.5691529780988,-65.365046299052,
-208.702360956951));
#191002=CARTESIAN_POINT('Ctrl Pts',(-56.5599119337509,-65.3770518735271,
-208.597713229276));
#191003=CARTESIAN_POINT('Ctrl Pts',(-56.5412952751588,-65.4001361493426,
-208.442727536444));
#191004=CARTESIAN_POINT('Ctrl Pts',(-56.5343427956335,-65.4086346803882,
-208.391050209511));
#191005=CARTESIAN_POINT('Ctrl Pts',(-56.5204776688227,-65.4250252363654,
-208.316259455579));
#191006=CARTESIAN_POINT('Ctrl Pts',(-56.5153591918106,-65.4310145177164,
-208.291764410647));
#191007=CARTESIAN_POINT('Ctrl Pts',(-56.5051439252244,-65.4426842233343,
-208.257244986379));
#191008=CARTESIAN_POINT('Ctrl Pts',(-56.5012774655679,-65.4470659442998,
-208.245963459985));
#191009=CARTESIAN_POINT('Ctrl Pts',(-56.4916787645948,-65.4577664915776,
-208.226946403507));
#191010=CARTESIAN_POINT('Ctrl Pts',(-56.4856347339016,-65.464428502687,
-208.218813480809));
#191011=CARTESIAN_POINT('Ctrl Pts',(-56.478494115784,-65.4721095684411,
-208.218811515426));
#191012=CARTESIAN_POINT('Origin',(0.,-12.9675000200281,-208.218811515427));
#191013=CARTESIAN_POINT('Origin',(0.,-12.9675000200281,-208.210085312208));
#191014=CARTESIAN_POINT('Origin',(0.,-12.9675000200281,-208.218811515427));
#191015=CARTESIAN_POINT('Ctrl Pts',(-56.6260312186758,39.26699791474,-213.932877779247));
#191016=CARTESIAN_POINT('Ctrl Pts',(-56.6591708158967,39.1947585157316,
-213.928380187744));
#191017=CARTESIAN_POINT('Ctrl Pts',(-56.7131249770401,39.136390603742,-213.924107582135));
#191018=CARTESIAN_POINT('Ctrl Pts',(-56.6069323298669,39.308101280162,-212.882516880404));
#191019=CARTESIAN_POINT('Ctrl Pts',(-56.6390541381501,39.2436411705138,
-212.880445101553));
#191020=CARTESIAN_POINT('Ctrl Pts',(-56.6878438485494,39.1909973438446,
-212.873680972192));
#191021=CARTESIAN_POINT('Ctrl Pts',(-56.5855128843193,39.3516918804354,
-211.83240628728));
#191022=CARTESIAN_POINT('Ctrl Pts',(-56.6161967667701,39.2955248737877,
-211.830328584023));
#191023=CARTESIAN_POINT('Ctrl Pts',(-56.6594850052376,39.248900569515,-211.823591080281));
#191024=CARTESIAN_POINT('Ctrl Pts',(-56.5376887518409,39.4321195627096,
-210.347455422068));
#191025=CARTESIAN_POINT('Ctrl Pts',(-56.5632284029527,39.3910644172893,
-210.343434951173));
#191026=CARTESIAN_POINT('Ctrl Pts',(-56.5961170971406,39.3557075607436,
-210.338665903179));
#191027=CARTESIAN_POINT('Ctrl Pts',(-56.5216963051399,39.4578331766847,
-209.910997266658));
#191028=CARTESIAN_POINT('Ctrl Pts',(-56.5454235880735,39.4215267027753,
-209.906981158345));
#191029=CARTESIAN_POINT('Ctrl Pts',(-56.5749226987295,39.3898533622913,
-209.90220762928));
#191030=CARTESIAN_POINT('Ctrl Pts',(-56.4885248990568,39.506210827646,-209.257701934938));
#191031=CARTESIAN_POINT('Ctrl Pts',(-56.5079716151444,39.4786993973283,
-209.253391637796));
#191032=CARTESIAN_POINT('Ctrl Pts',(-56.5309467959293,39.4540847109594,
-209.24891615073));
#191033=CARTESIAN_POINT('Ctrl Pts',(-56.4760962345234,39.5238015154724,
-209.040146260381));
#191034=CARTESIAN_POINT('Ctrl Pts',(-56.4938957981811,39.4994537797928,
-209.035838362477));
#191035=CARTESIAN_POINT('Ctrl Pts',(-56.5144681134185,39.4774389991119,
-209.031360415952));
#191036=CARTESIAN_POINT('Ctrl Pts',(-56.4508419233835,39.557225742165,-208.715924510879));
#191037=CARTESIAN_POINT('Ctrl Pts',(-56.4650653119284,39.5387956857416,
-208.711547487502));
#191038=CARTESIAN_POINT('Ctrl Pts',(-56.4809774462897,39.5218092152179,
-208.707139552256));
#191039=CARTESIAN_POINT('Ctrl Pts',(-56.4414369686318,39.5694195255203,
-208.60807433386));
#191040=CARTESIAN_POINT('Ctrl Pts',(-56.4543082678724,39.5531313413699,
-208.603698519052));
#191041=CARTESIAN_POINT('Ctrl Pts',(-56.4685043569935,39.5379957558533,
-208.599289345334));
#191042=CARTESIAN_POINT('Ctrl Pts',(-56.4224946430317,39.5928429539091,
-208.448559464111));
#191043=CARTESIAN_POINT('Ctrl Pts',(-56.4325361263003,39.5806119265652,
-208.444168467643));
#191044=CARTESIAN_POINT('Ctrl Pts',(-56.4433791076362,39.5690861270511,
-208.439774659198));
#191045=CARTESIAN_POINT('Ctrl Pts',(-56.4154558353936,39.6014220979252,
-208.395625171312));
#191046=CARTESIAN_POINT('Ctrl Pts',(-56.4244358024192,39.5906684103489,
-208.391234746251));
#191047=CARTESIAN_POINT('Ctrl Pts',(-56.4340423777229,39.5804730986549,
-208.386840352034));
#191048=CARTESIAN_POINT('Ctrl Pts',(-56.4013424744876,39.6180493256973,
-208.318678862813));
#191049=CARTESIAN_POINT('Ctrl Pts',(-56.4081423174308,39.6101253887744,
-208.314285655015));
#191050=CARTESIAN_POINT('Ctrl Pts',(-56.4153197235611,39.602540640524,-208.309894071191));
#191051=CARTESIAN_POINT('Ctrl Pts',(-56.3960980548982,39.6241637622927,
-208.293342260033));
#191052=CARTESIAN_POINT('Ctrl Pts',(-56.4020826208256,39.6172758938669,
-208.288949312307));
#191053=CARTESIAN_POINT('Ctrl Pts',(-56.4083623316493,39.6106555249509,
-208.284557461711));
#191054=CARTESIAN_POINT('Ctrl Pts',(-56.3856941549037,39.6360014284045,
-208.257923126188));
#191055=CARTESIAN_POINT('Ctrl Pts',(-56.3900359410543,39.6311005791763,
-208.253529947332));
#191056=CARTESIAN_POINT('Ctrl Pts',(-56.3945592936364,39.6263652686867,
-208.249138326507));
#191057=CARTESIAN_POINT('Ctrl Pts',(-56.3818606603298,39.6403285142035,
-208.246633418771));
#191058=CARTESIAN_POINT('Ctrl Pts',(-56.3855943263936,39.6361515194816,
-208.24224035659));
#191059=CARTESIAN_POINT('Ctrl Pts',(-56.3894732411015,39.6321076620074,
-208.237848616086));
#191060=CARTESIAN_POINT('Ctrl Pts',(-56.3097336024218,39.7204021456198,
-208.102340277927));
#191061=CARTESIAN_POINT('Ctrl Pts',(-56.3019347808255,39.7295012949886,
-208.097988441706));
#191062=CARTESIAN_POINT('Ctrl Pts',(-56.2937742808158,39.7383680155035,
-208.093554903205));
#191063=CARTESIAN_POINT('Ctrl Pts',(-56.0141418475234,40.0342093581467,
-208.239693755738));
#191064=CARTESIAN_POINT('Ctrl Pts',(-55.9576541168319,40.0945682331347,
-208.235168290733));
#191065=CARTESIAN_POINT('Ctrl Pts',(-55.901541357958,40.1547597432569,-208.230910731216));
#191066=CARTESIAN_POINT('Ctrl Pts',(-55.4188282852024,40.3069503931471,
-226.764375983926));
#191067=CARTESIAN_POINT('Ctrl Pts',(-55.1914520133701,40.4117219444719,
-227.50020914733));
#191068=CARTESIAN_POINT('Ctrl Pts',(-55.1111144719458,40.5151527971883,
-226.746035420514));
#191069=CARTESIAN_POINT('',(-56.6994898617306,39.1647669078403,-213.398999669105));
#191070=CARTESIAN_POINT('',(-56.6162420139465,39.2878063792742,-213.407725872324));
#191071=CARTESIAN_POINT('Origin',(-57.0675004159511,39.5031336989999,-213.407725872324));
#191072=CARTESIAN_POINT('',(-56.3587983457046,39.6656826243185,-208.210085312216));
#191073=CARTESIAN_POINT('Ctrl Pts',(-56.6994898617306,39.1647669078403,
-213.398999669105));
#191074=CARTESIAN_POINT('Ctrl Pts',(-56.6773193211235,39.2114480278548,
-212.523894235562));
#191075=CARTESIAN_POINT('Ctrl Pts',(-56.651479770637,39.2620537363991,-211.649203631226));
#191076=CARTESIAN_POINT('Ctrl Pts',(-56.5956975036787,39.3561498317412,
-210.339090933364));
#191077=CARTESIAN_POINT('Ctrl Pts',(-56.5745517354038,39.3902416134919,
-209.902674994602));
#191078=CARTESIAN_POINT('Ctrl Pts',(-56.5306742644768,39.4543652326716,
-209.24942443662));
#191079=CARTESIAN_POINT('Ctrl Pts',(-56.5142321837007,39.4776795989311,
-209.03188052566));
#191080=CARTESIAN_POINT('Ctrl Pts',(-56.480816494081,39.5219692158454,-208.70764780547));
#191081=CARTESIAN_POINT('Ctrl Pts',(-56.4683713984661,39.5381257486172,
-208.599790912822));
#191082=CARTESIAN_POINT('Ctrl Pts',(-56.4433041343981,39.569154837062,-208.440233728844));
#191083=CARTESIAN_POINT('Ctrl Pts',(-56.4339894177057,39.5805185781009,
-208.387282545977));
#191084=CARTESIAN_POINT('Ctrl Pts',(-56.4153107858428,39.6025404853857,
-208.310273287259));
#191085=CARTESIAN_POINT('Ctrl Pts',(-56.4083698728123,39.6106383616431,
-208.284910555051));
#191086=CARTESIAN_POINT('Ctrl Pts',(-56.394596442102,39.6263182576719,-208.249418094709));
#191087=CARTESIAN_POINT('Ctrl Pts',(-56.3895186643059,39.6320526747255,
-208.238093899573));
#191088=CARTESIAN_POINT('Ctrl Pts',(-56.3765990499463,39.6464010040802,
-208.218501926116));
#191089=CARTESIAN_POINT('Ctrl Pts',(-56.3682899804801,39.6555191285273,
-208.210085312216));
#191090=CARTESIAN_POINT('Ctrl Pts',(-56.3587983457046,39.6656826243185,
-208.210085312216));
#191091=CARTESIAN_POINT('',(-56.3587426896623,39.6656306474361,-208.218811515434));
#191092=CARTESIAN_POINT('Origin',(-56.7241679835722,40.0068993898824,-208.218811515434));
#191093=CARTESIAN_POINT('Ctrl Pts',(-56.3587426896623,39.6656306474361,
-208.218811515434));
#191094=CARTESIAN_POINT('Ctrl Pts',(-56.3660413076723,39.6578154000967,
-208.21881254009));
#191095=CARTESIAN_POINT('Ctrl Pts',(-56.3721137606125,39.6511492752057,
-208.227134345684));
#191096=CARTESIAN_POINT('Ctrl Pts',(-56.3818606603298,39.6403285142035,
-208.246633418771));
#191097=CARTESIAN_POINT('Ctrl Pts',(-56.3856941549037,39.6360014284045,
-208.257923126188));
#191098=CARTESIAN_POINT('Ctrl Pts',(-56.3960980548982,39.6241637622927,
-208.293342260033));
#191099=CARTESIAN_POINT('Ctrl Pts',(-56.4013424744876,39.6180493256973,
-208.318678862813));
#191100=CARTESIAN_POINT('Ctrl Pts',(-56.4154558353936,39.6014220979252,
-208.395625171312));
#191101=CARTESIAN_POINT('Ctrl Pts',(-56.4224946430317,39.5928429539091,
-208.448559464111));
#191102=CARTESIAN_POINT('Ctrl Pts',(-56.4414369686318,39.5694195255203,
-208.60807433386));
#191103=CARTESIAN_POINT('Ctrl Pts',(-56.4508419233835,39.557225742165,-208.715924510879));
#191104=CARTESIAN_POINT('Ctrl Pts',(-56.4760962345234,39.5238015154724,
-209.040146260381));
#191105=CARTESIAN_POINT('Ctrl Pts',(-56.4885248990568,39.506210827646,-209.257701934938));
#191106=CARTESIAN_POINT('Ctrl Pts',(-56.5216963051399,39.4578331766847,
-209.910997266658));
#191107=CARTESIAN_POINT('Ctrl Pts',(-56.5376887518409,39.4321195627096,
-210.347455422068));
#191108=CARTESIAN_POINT('Ctrl Pts',(-56.5798865157924,39.3611539607029,
-211.657706185491));
#191109=CARTESIAN_POINT('Ctrl Pts',(-56.5994497711951,39.3229976436235,
-212.532533071095));
#191110=CARTESIAN_POINT('Ctrl Pts',(-56.6162420139465,39.2878063792742,
-213.407725872324));
#191111=CARTESIAN_POINT('Origin',(0.,-12.9675000200281,-208.218811515434));
#191112=CARTESIAN_POINT('',(-52.2148720050704,43.7789665035542,-208.218811515434));
#191113=CARTESIAN_POINT('',(-52.2149235689092,43.779022542486,-208.210085312216));
#191114=CARTESIAN_POINT('Origin',(-52.5534287939255,44.1469057658247,-208.218811515435));
#191115=CARTESIAN_POINT('Origin',(0.,-12.9675000200281,-208.218811515434));
#191116=CARTESIAN_POINT('Origin',(0.,-12.9675000200281,-208.210085312216));
#191117=CARTESIAN_POINT('Ctrl Pts',(-56.6994898617306,39.1647669078403,
-213.398999669105));
#191118=CARTESIAN_POINT('Ctrl Pts',(-56.6485891211103,39.2200170067656,
-213.40326396142));
#191119=CARTESIAN_POINT('Ctrl Pts',(-56.6162420139465,39.2878063792742,
-213.407725872324));
#191120=CARTESIAN_POINT('Ctrl Pts',(-56.7065185819046,39.150823857201,-213.643232131226));
#191121=CARTESIAN_POINT('Ctrl Pts',(-56.65401999933,39.2072427576227,-213.659624098485));
#191122=CARTESIAN_POINT('Ctrl Pts',(-56.6213962984542,39.2770046185252,
-213.676360638228));
#191123=CARTESIAN_POINT('Ctrl Pts',(-56.7424050849715,39.0804003802149,
-213.870334716274));
#191124=CARTESIAN_POINT('Ctrl Pts',(-56.6817938786107,39.1423247455582,
-213.899040022644));
#191125=CARTESIAN_POINT('Ctrl Pts',(-56.6474543007565,39.2227628260081,
-213.926243763817));
#191126=CARTESIAN_POINT('Ctrl Pts',(-56.8149567807673,38.8971968180779,
-214.313055955637));
#191127=CARTESIAN_POINT('Ctrl Pts',(-56.7320119538466,38.9741928361746,
-214.361884513898));
#191128=CARTESIAN_POINT('Ctrl Pts',(-56.6987085996655,39.0810160666721,
-214.413338469428));
#191129=CARTESIAN_POINT('Ctrl Pts',(-56.8517306517416,38.7836290914654,
-214.528047686166));
#191130=CARTESIAN_POINT('Ctrl Pts',(-56.7545477049515,38.8689917647235,
-214.586934745154));
#191131=CARTESIAN_POINT('Ctrl Pts',(-56.7239630070022,38.9928957520747,
-214.64988909805));
#191132=CARTESIAN_POINT('Ctrl Pts',(-56.9296676067097,38.4194837815438,
-215.154132254812));
#191133=CARTESIAN_POINT('Ctrl Pts',(-56.7853204957809,38.530818668951,-215.243449487387));
#191134=CARTESIAN_POINT('Ctrl Pts',(-56.7732185725244,38.7090403847746,
-215.338759568586));
#191135=CARTESIAN_POINT('Ctrl Pts',(-56.9425587655176,38.1405794851196,
-215.553519015804));
#191136=CARTESIAN_POINT('Ctrl Pts',(-56.7534747673294,38.2694300870757,
-215.658829235944));
#191137=CARTESIAN_POINT('Ctrl Pts',(-56.7738348833635,38.4902290986137,
-215.777992061446));
#191138=CARTESIAN_POINT('Ctrl Pts',(-56.8784089512595,37.8494072532151,
-215.942196083675));
#191139=CARTESIAN_POINT('Ctrl Pts',(-56.6513917750256,38.0264112674188,
-216.026572725176));
#191140=CARTESIAN_POINT('Ctrl Pts',(-56.7127812850717,38.2589564044561,
-216.205851068199));
#191141=CARTESIAN_POINT('',(-56.8783191528564,37.8493275727119,-215.942121479197));
#191142=CARTESIAN_POINT('',(-56.7127812850717,38.2589564044561,-216.205851068199));
#191143=CARTESIAN_POINT('Origin',(-57.1962194441171,38.1313337325768,-216.205851068199));
#191144=CARTESIAN_POINT('Ctrl Pts',(-56.8784089539157,37.8494072652715,
-215.942196067581));
#191145=CARTESIAN_POINT('Ctrl Pts',(-56.9425587651617,38.1405794928185,
-215.553519004779));
#191146=CARTESIAN_POINT('Ctrl Pts',(-56.9296676059926,38.4194837848944,
-215.154132249051));
#191147=CARTESIAN_POINT('Ctrl Pts',(-56.8517306517416,38.7836290914654,
-214.528047686166));
#191148=CARTESIAN_POINT('Ctrl Pts',(-56.8149567807673,38.8971968180779,
-214.313055955637));
#191149=CARTESIAN_POINT('Ctrl Pts',(-56.7424050849715,39.0804003802149,
-213.870334716274));
#191150=CARTESIAN_POINT('Ctrl Pts',(-56.7065185819046,39.150823857201,-213.643232131226));
#191151=CARTESIAN_POINT('Ctrl Pts',(-56.6994898617306,39.1647669078403,
-213.398999669105));
#191152=CARTESIAN_POINT('Ctrl Pts',(-56.6162420139465,39.2878063792742,
-213.407725872324));
#191153=CARTESIAN_POINT('Ctrl Pts',(-56.6213962984542,39.2770046185252,
-213.676360638228));
#191154=CARTESIAN_POINT('Ctrl Pts',(-56.6474543007565,39.2227628260081,
-213.926243763817));
#191155=CARTESIAN_POINT('Ctrl Pts',(-56.6987085996655,39.0810160666721,
-214.413338469428));
#191156=CARTESIAN_POINT('Ctrl Pts',(-56.7239630070022,38.9928957520747,
-214.64988909805));
#191157=CARTESIAN_POINT('Ctrl Pts',(-56.7732185725244,38.7090403847746,
-215.338759568586));
#191158=CARTESIAN_POINT('Ctrl Pts',(-56.7738348833635,38.4902290986137,
-215.777992061446));
#191159=CARTESIAN_POINT('Ctrl Pts',(-56.7127812850717,38.2589564044561,
-216.205851068199));
#191160=CARTESIAN_POINT('Ctrl Pts',(-52.2148720050704,43.7789665035542,
-208.218811515435));
#191161=CARTESIAN_POINT('Ctrl Pts',(-52.2148720050705,43.7789665035542,
-208.214448081539));
#191162=CARTESIAN_POINT('Ctrl Pts',(-52.2149235689092,43.779022542486,-208.210085312216));
#191163=CARTESIAN_POINT('Ctrl Pts',(-52.2069166839655,43.7862865377113,
-208.21881354139));
#191164=CARTESIAN_POINT('Ctrl Pts',(-52.2056250202409,43.7874750042174,
-208.214450107462));
#191165=CARTESIAN_POINT('Ctrl Pts',(-52.2043847769924,43.7887196915372,
-208.210087338187));
#191166=CARTESIAN_POINT('Ctrl Pts',(-52.2000848734438,43.7924159898367,
-208.227398819688));
#191167=CARTESIAN_POINT('Ctrl Pts',(-52.1976712649932,43.7945859134348,
-208.223035434656));
#191168=CARTESIAN_POINT('Ctrl Pts',(-52.195333723769,43.7968389605576,-208.218672616477));
#191169=CARTESIAN_POINT('Ctrl Pts',(-52.1891506941446,43.8021155648562,
-208.247190155172));
#191170=CARTESIAN_POINT('Ctrl Pts',(-52.1849330344943,43.8058281558383,
-208.242826402981));
#191171=CARTESIAN_POINT('Ctrl Pts',(-52.1808472399183,43.8096868118422,
-208.238463951946));
#191172=CARTESIAN_POINT('Ctrl Pts',(-52.1846836299068,43.8060124062017,
-208.258883232989));
#191173=CARTESIAN_POINT('Ctrl Pts',(-52.1797237791601,43.8103385591305,
-208.254519356384));
#191174=CARTESIAN_POINT('Ctrl Pts',(-52.1749286143212,43.8148481482676,
-208.250157029773));
#191175=CARTESIAN_POINT('Ctrl Pts',(-52.1728001724479,43.8162953562062,
-208.294562380182));
#191176=CARTESIAN_POINT('Ctrl Pts',(-52.1658591933782,43.8222328676652,
-208.290198743649));
#191177=CARTESIAN_POINT('Ctrl Pts',(-52.1591833603872,43.828467493664,-208.285836176959));
#191178=CARTESIAN_POINT('Ctrl Pts',(-52.1666971009815,43.8214493653102,
-208.3198471127));
#191179=CARTESIAN_POINT('Ctrl Pts',(-52.1587292093287,43.8281818395797,
-208.315483211337));
#191180=CARTESIAN_POINT('Ctrl Pts',(-52.1510964156406,43.8352931366209,
-208.311120909483));
#191181=CARTESIAN_POINT('Ctrl Pts',(-52.1499948920096,43.8354085050508,
-208.397025142829));
#191182=CARTESIAN_POINT('Ctrl Pts',(-52.1392045981911,43.8442802812313,
-208.392664031458));
#191183=CARTESIAN_POINT('Ctrl Pts',(-52.1289643871997,43.8537790486242,
-208.388298939608));
#191184=CARTESIAN_POINT('Ctrl Pts',(-52.141343336723,43.8423973674724,-208.450246795732));
#191185=CARTESIAN_POINT('Ctrl Pts',(-52.1290740876191,43.852314411835,-208.445885091517));
#191186=CARTESIAN_POINT('Ctrl Pts',(-52.1174992362576,43.8630330920583,
-208.441520592514));
#191187=CARTESIAN_POINT('Ctrl Pts',(-52.1178275724807,43.8611200325978,
-208.609901492046));
#191188=CARTESIAN_POINT('Ctrl Pts',(-52.1015151102266,43.8738103589885,
-208.605554907233));
#191189=CARTESIAN_POINT('Ctrl Pts',(-52.0863347270061,43.8878226116337,
-208.601175288826));
#191190=CARTESIAN_POINT('Ctrl Pts',(-52.1055914799472,43.8704111305645,
-208.717677837571));
#191191=CARTESIAN_POINT('Ctrl Pts',(-52.0871460895594,43.884425032588,-208.713330067135));
#191192=CARTESIAN_POINT('Ctrl Pts',(-52.0701168476483,43.9001220002185,
-208.708951634353));
#191193=CARTESIAN_POINT('Ctrl Pts',(-52.071995743712,43.8953985191085,-209.042218804019));
#191194=CARTESIAN_POINT('Ctrl Pts',(-52.0476481597434,43.9129173610403,
-209.037939859074));
#191195=CARTESIAN_POINT('Ctrl Pts',(-52.0255864626054,43.9331969723227,
-209.0334926008));
#191196=CARTESIAN_POINT('Ctrl Pts',(-52.0543127614129,43.9076935513658,
-209.259992694935));
#191197=CARTESIAN_POINT('Ctrl Pts',(-52.0268103251713,43.9268242456044,
-209.255711234979));
#191198=CARTESIAN_POINT('Ctrl Pts',(-52.0021445297993,43.949466653783,-209.251266491716));
#191199=CARTESIAN_POINT('Ctrl Pts',(-52.0057184578615,43.940477854794,-209.913465487369));
#191200=CARTESIAN_POINT('Ctrl Pts',(-51.9694532568106,43.9637905045621,
-209.909476451697));
#191201=CARTESIAN_POINT('Ctrl Pts',(-51.937720029348,43.9928431481926,-209.90473928415));
#191202=CARTESIAN_POINT('Ctrl Pts',(-51.9798728970522,43.9562851731636,
-210.350348060599));
#191203=CARTESIAN_POINT('Ctrl Pts',(-51.9388750336111,43.9813630646936,
-210.346355470779));
#191204=CARTESIAN_POINT('Ctrl Pts',(-51.9034482509577,44.0137474304281,
-210.34162185738));
#191205=CARTESIAN_POINT('Ctrl Pts',(-51.9085528218201,43.9979691256788,
-211.662166712722));
#191206=CARTESIAN_POINT('Ctrl Pts',(-51.8543012271538,44.0274385666118,
-211.659386088869));
#191207=CARTESIAN_POINT('Ctrl Pts',(-51.8088683580654,44.0688586918087,
-211.653440509504));
#191208=CARTESIAN_POINT('Ctrl Pts',(-51.870219684202,44.0172576131423,-212.538231376868));
#191209=CARTESIAN_POINT('Ctrl Pts',(-51.8087639397327,44.0481656078252,
-212.535446734955));
#191210=CARTESIAN_POINT('Ctrl Pts',(-51.7580215322863,44.0943375071556,
-212.529490943221));
#191211=CARTESIAN_POINT('Ctrl Pts',(-51.8348891643276,44.0337882456516,
-213.414282330697));
#191212=CARTESIAN_POINT('Ctrl Pts',(-51.7668122505506,44.0656404359961,
-213.409820292477));
#191213=CARTESIAN_POINT('Ctrl Pts',(-51.7111509881033,44.1161634878026,
-213.405556127478));
#191214=CARTESIAN_POINT('',(-51.8348891643276,44.0337882456516,-213.414282330697));
#191215=CARTESIAN_POINT('',(-51.7111509881036,44.1161634878024,-213.405556127478));
#191216=CARTESIAN_POINT('Origin',(-52.0467850062684,44.4866680886213,-213.414282330697));
#191217=CARTESIAN_POINT('Ctrl Pts',(-51.8348891643276,44.0337882456516,
-213.414282330697));
#191218=CARTESIAN_POINT('Ctrl Pts',(-51.870219684202,44.0172576131423,-212.538231376868));
#191219=CARTESIAN_POINT('Ctrl Pts',(-51.9085528218201,43.9979691256788,
-211.662166712722));
#191220=CARTESIAN_POINT('Ctrl Pts',(-51.9798728970522,43.9562851731636,
-210.350348060599));
#191221=CARTESIAN_POINT('Ctrl Pts',(-52.0057184578615,43.940477854794,-209.913465487369));
#191222=CARTESIAN_POINT('Ctrl Pts',(-52.0543127614129,43.9076935513658,
-209.259992694935));
#191223=CARTESIAN_POINT('Ctrl Pts',(-52.071995743712,43.8953985191085,-209.042218804019));
#191224=CARTESIAN_POINT('Ctrl Pts',(-52.1055914799472,43.8704111305645,
-208.717677837571));
#191225=CARTESIAN_POINT('Ctrl Pts',(-52.1178275724807,43.8611200325978,
-208.609901492046));
#191226=CARTESIAN_POINT('Ctrl Pts',(-52.141343336723,43.8423973674724,-208.450246795732));
#191227=CARTESIAN_POINT('Ctrl Pts',(-52.1499948920096,43.8354085050508,
-208.397025142829));
#191228=CARTESIAN_POINT('Ctrl Pts',(-52.1666971009815,43.8214493653102,
-208.3198471127));
#191229=CARTESIAN_POINT('Ctrl Pts',(-52.1728001724479,43.8162953562062,
-208.294562380182));
#191230=CARTESIAN_POINT('Ctrl Pts',(-52.1846836299068,43.8060124062017,
-208.258883232989));
#191231=CARTESIAN_POINT('Ctrl Pts',(-52.1891506941446,43.8021155648562,
-208.247190155172));
#191232=CARTESIAN_POINT('Ctrl Pts',(-52.2000848734438,43.7924159898367,
-208.227398819688));
#191233=CARTESIAN_POINT('Ctrl Pts',(-52.2069166839655,43.7862865377113,
-208.21881354139));
#191234=CARTESIAN_POINT('Ctrl Pts',(-52.2148720050704,43.7789665035542,
-208.218811515434));
#191235=CARTESIAN_POINT('Ctrl Pts',(-52.2149235689092,43.779022542486,-208.210085312216));
#191236=CARTESIAN_POINT('Ctrl Pts',(-52.2043801934833,43.7887239088728,
-208.210087344463));
#191237=CARTESIAN_POINT('Ctrl Pts',(-52.1953274288659,43.796844542981,-208.218681234754));
#191238=CARTESIAN_POINT('Ctrl Pts',(-52.1880904910527,43.8032628774376,
-208.228568296719));
#191239=CARTESIAN_POINT('Ctrl Pts',(-52.1808394389761,43.8096937296283,
-208.238474641509));
#191240=CARTESIAN_POINT('Ctrl Pts',(-52.1749242234792,43.8148519452172,
-208.250167023561));
#191241=CARTESIAN_POINT('Ctrl Pts',(-52.1696802065441,43.8193879205004,
-208.262050087041));
#191242=CARTESIAN_POINT('Ctrl Pts',(-52.1591795680454,43.8284707738317,
-208.28584477638));
#191243=CARTESIAN_POINT('Ctrl Pts',(-52.1510932946611,43.8352957489707,
-208.311131552955));
#191244=CARTESIAN_POINT('Ctrl Pts',(-52.1437197227052,43.8414545028842,
-208.336847252802));
#191245=CARTESIAN_POINT('Ctrl Pts',(-52.1289623042575,43.8537805924866,
-208.38831448545));
#191246=CARTESIAN_POINT('Ctrl Pts',(-52.117497806034,43.8630342337481,-208.441527742187));
#191247=CARTESIAN_POINT('Ctrl Pts',(-52.1071115904079,43.871295780733,-208.494739003265));
#191248=CARTESIAN_POINT('Ctrl Pts',(-52.0863339472228,43.8878230204506,
-208.601188227497));
#191249=CARTESIAN_POINT('Ctrl Pts',(-52.0701156440688,43.9001228988017,
-208.708960203697));
#191250=CARTESIAN_POINT('Ctrl Pts',(-52.0552737632954,43.9111466435138,
-208.817132044246));
#191251=CARTESIAN_POINT('Ctrl Pts',(-52.0255859242023,43.9331971615186,
-209.033505443658));
#191252=CARTESIAN_POINT('Ctrl Pts',(-52.0021438786448,43.9494670967064,
-209.251272899507));
#191253=CARTESIAN_POINT('Ctrl Pts',(-51.980669942658,43.9639252593981,-209.469090795394));
#191254=CARTESIAN_POINT('Ctrl Pts',(-51.9377196179987,43.9928432361475,
-209.904751465645));
#191255=CARTESIAN_POINT('Ctrl Pts',(-51.9034476265843,44.0137477974947,
-210.34163037533));
#191256=CARTESIAN_POINT('Ctrl Pts',(-51.8719217450993,44.032117736709,-210.778894755328));
#191257=CARTESIAN_POINT('Ctrl Pts',(-51.8088678222893,44.0688588736632,
-211.653453472328));
#191258=CARTESIAN_POINT('Ctrl Pts',(-51.7580264403492,44.0943352215171,
-212.529399211082));
#191259=CARTESIAN_POINT('Ctrl Pts',(-51.7111509881036,44.1161634878024,
-213.405556127478));
#191260=CARTESIAN_POINT('Ctrl Pts',(-56.493933359474,37.4299544982648,-217.120571662276));
#191261=CARTESIAN_POINT('Ctrl Pts',(-56.4397634983909,37.224757588248,-216.873345412929));
#191262=CARTESIAN_POINT('Ctrl Pts',(-56.7060833516158,37.0658058009135,
-216.773500778908));
#191263=CARTESIAN_POINT('Ctrl Pts',(-56.5765881122648,37.7430529543375,
-216.842569308717));
#191264=CARTESIAN_POINT('Ctrl Pts',(-56.5188765640458,37.5244400369599,
-216.620195693846));
#191265=CARTESIAN_POINT('Ctrl Pts',(-56.7710955429381,37.361906243833,-216.520874647208));
#191266=CARTESIAN_POINT('Ctrl Pts',(-56.6508914688365,38.0245160939405,
-216.533616118302));
#191267=CARTESIAN_POINT('Ctrl Pts',(-56.5910528040772,37.7978456011263,
-216.333918533896));
#191268=CARTESIAN_POINT('Ctrl Pts',(-56.8296189005624,37.6279227921511,
-216.240093840689));
#191269=CARTESIAN_POINT('Ctrl Pts',(-56.7157183655621,38.2700821453947,
-216.190356702619));
#191270=CARTESIAN_POINT('Ctrl Pts',(-56.654233824142,38.0371770269228,-216.012141918556));
#191271=CARTESIAN_POINT('Ctrl Pts',(-56.8807321403751,37.8599121389907,
-215.928110733678));
#191272=CARTESIAN_POINT('',(-56.7089756139177,37.0787993772561,-216.761772606351));
#191273=CARTESIAN_POINT('',(-56.4975419847624,37.4436240691992,-217.108396707512));
#191274=CARTESIAN_POINT('Origin',(-56.9809801438088,37.3160013973188,-217.108396707512));
#191275=CARTESIAN_POINT('Ctrl Pts',(-56.7089871854676,37.0788107123884,
-216.761648750883));
#191276=CARTESIAN_POINT('Ctrl Pts',(-56.7294957256895,37.1726092366223,
-216.681203054031));
#191277=CARTESIAN_POINT('Ctrl Pts',(-56.7493601478726,37.2633733311913,
-216.597849124767));
#191278=CARTESIAN_POINT('Ctrl Pts',(-56.7685769354936,37.3509956263222,
-216.511522123815));
#191279=CARTESIAN_POINT('Ctrl Pts',(-56.7882832885266,37.4408501803435,
-216.422995862789));
#191280=CARTESIAN_POINT('Ctrl Pts',(-56.8073094114385,37.5274016027229,
-216.331342347585));
#191281=CARTESIAN_POINT('Ctrl Pts',(-56.8256102466557,37.6105017357572,
-216.236465902513));
#191282=CARTESIAN_POINT('Ctrl Pts',(-56.8424913406294,37.687155130989,-216.148949777368));
#191283=CARTESIAN_POINT('Ctrl Pts',(-56.8587552053145,37.7608719482353,
-216.058690386204));
#191284=CARTESIAN_POINT('Ctrl Pts',(-56.8743281021412,37.8315042449062,
-215.965604323594));
#191285=CARTESIAN_POINT('Ctrl Pts',(-56.8756378208087,37.8374445936102,
-215.95777555832));
#191286=CARTESIAN_POINT('Ctrl Pts',(-56.8769426285927,37.8433631050215,
-215.949926799156));
#191287=CARTESIAN_POINT('Ctrl Pts',(-56.8782424684775,37.8492596800232,
-215.942057996922));
#191288=CARTESIAN_POINT('Ctrl Pts',(-56.7127812850717,38.2589564044562,
-216.205851068199));
#191289=CARTESIAN_POINT('Ctrl Pts',(-56.675820350007,38.1189473751743,-216.400115647765));
#191290=CARTESIAN_POINT('Ctrl Pts',(-56.6358255784857,37.9674460907173,
-216.583274967065));
#191291=CARTESIAN_POINT('Ctrl Pts',(-56.5929883959844,37.8051776760066,
-216.756029715358));
#191292=CARTESIAN_POINT('Ctrl Pts',(-56.5625833082106,37.6900023749221,
-216.878648033801));
#191293=CARTESIAN_POINT('Ctrl Pts',(-56.5307460013724,37.5694017889912,
-216.996023775216));
#191294=CARTESIAN_POINT('Ctrl Pts',(-56.4975419847624,37.4436240691992,
-217.108396707512));
#191295=CARTESIAN_POINT('Ctrl Pts',(-50.3946838675078,44.2853208550272,
-215.949517829821));
#191296=CARTESIAN_POINT('Ctrl Pts',(-50.5733927277608,44.0594460487845,
-216.033846066216));
#191297=CARTESIAN_POINT('Ctrl Pts',(-50.8056178277775,44.122591905242,-216.213154850206));
#191298=CARTESIAN_POINT('Ctrl Pts',(-50.6840782755553,44.3512988155942,
-215.562426526428));
#191299=CARTESIAN_POINT('Ctrl Pts',(-50.8146150821098,44.1628990192414,
-215.667558528646));
#191300=CARTESIAN_POINT('Ctrl Pts',(-51.0353932564851,44.1850716554394,
-215.787037343168));
#191301=CARTESIAN_POINT('Ctrl Pts',(-50.9615743000221,44.3410430024776,
-215.16541559435));
#191302=CARTESIAN_POINT('Ctrl Pts',(-51.0742087234282,44.1970539660852,
-215.254908907856));
#191303=CARTESIAN_POINT('Ctrl Pts',(-51.2530132713136,44.1864939716348,
-215.350454259388));
#191304=CARTESIAN_POINT('Ctrl Pts',(-51.3272201973583,44.2660193725917,
-214.53815525918));
#191305=CARTESIAN_POINT('Ctrl Pts',(-51.4134751324715,44.1691804565493,
-214.597183792391));
#191306=CARTESIAN_POINT('Ctrl Pts',(-51.5379400316186,44.1395671487007,
-214.660316432704));
#191307=CARTESIAN_POINT('Ctrl Pts',(-51.4410933404088,44.2301818679357,
-214.323225058398));
#191308=CARTESIAN_POINT('Ctrl Pts',(-51.5188806364346,44.1475373241685,
-214.372200521963));
#191309=CARTESIAN_POINT('Ctrl Pts',(-51.6262699955377,44.115047729854,-214.423842816164));
#191310=CARTESIAN_POINT('Ctrl Pts',(-51.6251804607438,44.1590287655627,
-213.880764647617));
#191311=CARTESIAN_POINT('Ctrl Pts',(-51.6877019825951,44.0986734814325,
-213.909653665353));
#191312=CARTESIAN_POINT('Ctrl Pts',(-51.7686497926484,44.0649060154392,
-213.937052332728));
#191313=CARTESIAN_POINT('Ctrl Pts',(-51.6971249390044,44.1231091971094,
-213.650130074529));
#191314=CARTESIAN_POINT('Ctrl Pts',(-51.7539747290057,44.0709837332505,
-213.666541516794));
#191315=CARTESIAN_POINT('Ctrl Pts',(-51.8240398734104,44.0388644698843,
-213.683299458677));
#191316=CARTESIAN_POINT('Ctrl Pts',(-51.7111509881034,44.1161634878026,
-213.405556127478));
#191317=CARTESIAN_POINT('Ctrl Pts',(-51.7668122505508,44.0656404359961,
-213.409820292478));
#191318=CARTESIAN_POINT('Ctrl Pts',(-51.8348891643277,44.0337882456516,
-213.414282330697));
#191319=CARTESIAN_POINT('',(-50.8056178277775,44.122591905242,-216.213154850206));
#191320=CARTESIAN_POINT('',(-50.3946596588565,44.2852932582017,-215.949495022928));
#191321=CARTESIAN_POINT('Origin',(-50.6744232242015,44.605072968075,-216.213154850206));
#191322=CARTESIAN_POINT('',(-51.199201564042,44.1751972079741,-215.438515911214));
#191323=CARTESIAN_POINT('Ctrl Pts',(-50.8056178277775,44.122591905242,-216.213154850206));
#191324=CARTESIAN_POINT('Ctrl Pts',(-50.942180477307,44.1597255547226,-215.959527204626));
#191325=CARTESIAN_POINT('Ctrl Pts',(-51.0744557978905,44.1752936552023,
-215.702232151633));
#191326=CARTESIAN_POINT('Ctrl Pts',(-51.1992016385053,44.1751487167426,
-215.438515960385));
#191327=CARTESIAN_POINT('Ctrl Pts',(-51.1992014957792,44.1752416613772,
-215.438515866138));
#191328=CARTESIAN_POINT('Ctrl Pts',(-51.2842504005282,44.1752065198926,
-215.25904635145));
#191329=CARTESIAN_POINT('Ctrl Pts',(-51.3657803296688,44.1679108384777,
-215.076578914644));
#191330=CARTESIAN_POINT('Ctrl Pts',(-51.4427636582211,44.1552425471702,
-214.890248844184));
#191331=CARTESIAN_POINT('Ctrl Pts',(-51.4993014431223,44.1459387518877,
-214.753405067195));
#191332=CARTESIAN_POINT('Ctrl Pts',(-51.5534831111867,44.1334894340395,
-214.614283009387));
#191333=CARTESIAN_POINT('Ctrl Pts',(-51.6030992923736,44.1196492385698,
-214.47277824517));
#191334=CARTESIAN_POINT('Ctrl Pts',(-51.6368787254434,44.1102266279344,
-214.376439700011));
#191335=CARTESIAN_POINT('Ctrl Pts',(-51.6685414748578,44.1001594496879,
-214.278996905908));
#191336=CARTESIAN_POINT('Ctrl Pts',(-51.6973902398397,44.0900014094681,
-214.180417040629));
#191337=CARTESIAN_POINT('Ctrl Pts',(-51.7686127338013,44.0649230063313,
-213.937040803763));
#191338=CARTESIAN_POINT('Ctrl Pts',(-51.8240227963017,44.0388724600132,
-213.683298339373));
#191339=CARTESIAN_POINT('Ctrl Pts',(-51.8348891643276,44.0337882456516,
-213.414282330697));
#191340=CARTESIAN_POINT('Ctrl Pts',(-51.7111509881036,44.1161634878024,
-213.405556127478));
#191341=CARTESIAN_POINT('Ctrl Pts',(-51.6971249390044,44.1231091971094,
-213.650130074529));
#191342=CARTESIAN_POINT('Ctrl Pts',(-51.6251804607438,44.1590287655627,
-213.880764647617));
#191343=CARTESIAN_POINT('Ctrl Pts',(-51.4410933404088,44.2301818679357,
-214.323225058398));
#191344=CARTESIAN_POINT('Ctrl Pts',(-51.3272201973583,44.2660193725917,
-214.53815525918));
#191345=CARTESIAN_POINT('Ctrl Pts',(-50.9615743000221,44.3410430024776,
-215.16541559435));
#191346=CARTESIAN_POINT('Ctrl Pts',(-50.6840782755553,44.3512988155942,
-215.562426526428));
#191347=CARTESIAN_POINT('Ctrl Pts',(-50.3946838675078,44.2853208550272,
-215.949517829821));
#191348=CARTESIAN_POINT('Ctrl Pts',(-56.351930605989,36.892044198215,-217.60005));
#191349=CARTESIAN_POINT('Ctrl Pts',(-56.2980271921268,36.6878565975336,
-217.354444173088));
#191350=CARTESIAN_POINT('Ctrl Pts',(-56.5618180211198,36.5289367340068,
-217.254048694966));
#191351=CARTESIAN_POINT('Ctrl Pts',(-56.4005154364319,37.0760848599628,
-217.436382427969));
#191352=CARTESIAN_POINT('Ctrl Pts',(-56.3465050213663,36.8714919357672,
-217.190493004533));
#191353=CARTESIAN_POINT('Ctrl Pts',(-56.6108961448827,36.7123872459292,
-217.09039277187));
#191354=CARTESIAN_POINT('Ctrl Pts',(-56.4490528535666,37.2599459188071,
-217.272499319579));
#191355=CARTESIAN_POINT('Ctrl Pts',(-56.394913005841,37.054862700115,-217.026399523816));
#191356=CARTESIAN_POINT('Ctrl Pts',(-56.6599284966586,36.8956552674856,
-216.926524548004));
#191357=CARTESIAN_POINT('Ctrl Pts',(-56.4975419847625,37.4436240691992,
-217.108396707512));
#191358=CARTESIAN_POINT('Ctrl Pts',(-56.4432500919346,37.2379648996087,
-216.862162585543));
#191359=CARTESIAN_POINT('Ctrl Pts',(-56.7089132278424,37.0787382657863,
-216.762440352386));
#191360=CARTESIAN_POINT('',(-56.5618180211198,36.5289367340069,-217.254048694966));
#191361=CARTESIAN_POINT('',(-56.351930605989,36.892044198215,-217.60005));
#191362=CARTESIAN_POINT('Origin',(-56.8353687650353,36.7644215263347,-217.60005));
#191363=CARTESIAN_POINT('Origin',(-3.60305208601888,-172.041642880457,32.426831165629));
#191364=CARTESIAN_POINT('Origin',(-1.571323227265,-170.618389531262,32.0043824393251));
#191365=CARTESIAN_POINT('Ctrl Pts',(-50.8056178277775,44.122591905242,-216.213154850206));
#191366=CARTESIAN_POINT('Ctrl Pts',(-50.5733927277608,44.0594460487845,
-216.033846066216));
#191367=CARTESIAN_POINT('Ctrl Pts',(-50.3946838675078,44.2853208550272,
-215.949517829821));
#191368=CARTESIAN_POINT('Ctrl Pts',(-50.5708296219181,44.0587490977934,
-216.539715105359));
#191369=CARTESIAN_POINT('Ctrl Pts',(-50.3446120279677,43.9972367818614,
-216.339838795389));
#191370=CARTESIAN_POINT('Ctrl Pts',(-50.1727811095107,44.2347300586007,
-216.246332930804));
#191371=CARTESIAN_POINT('Ctrl Pts',(-50.3034496116678,43.9860440381524,
-216.835170188754));
#191372=CARTESIAN_POINT('Ctrl Pts',(-50.0849672365085,43.9266350565256,
-216.613616901689));
#191373=CARTESIAN_POINT('Ctrl Pts',(-49.9199744021421,44.177167823471,-216.514858553214));
#191374=CARTESIAN_POINT('Ctrl Pts',(-50.0071669705522,43.9054798737905,
-217.102435280211));
#191375=CARTESIAN_POINT('Ctrl Pts',(-49.8012110043667,43.8494770305304,
-216.857236779929));
#191376=CARTESIAN_POINT('Ctrl Pts',(-49.6396803417508,44.1134564636836,
-216.757742122242));
#191377=CARTESIAN_POINT('',(-50.0071669705522,43.9054798737905,-217.102435280211));
#191378=CARTESIAN_POINT('',(-49.6397984855042,44.1135871370244,-216.757171052671));
#191379=CARTESIAN_POINT('Origin',(-49.8759723669763,44.3879609366236,-217.102435280211));
#191380=CARTESIAN_POINT('Ctrl Pts',(-50.0071669705522,43.9054798737905,
-217.102435280211));
#191381=CARTESIAN_POINT('Ctrl Pts',(-50.1847337846688,43.9537632357311,
-216.94225913611));
#191382=CARTESIAN_POINT('Ctrl Pts',(-50.3518605126697,43.9992077650942,
-216.772016153319));
#191383=CARTESIAN_POINT('Ctrl Pts',(-50.5078320264292,44.0416190066809,
-216.591016782861));
#191384=CARTESIAN_POINT('Ctrl Pts',(-50.6121600770689,44.0699875340696,
-216.469947806663));
#191385=CARTESIAN_POINT('Ctrl Pts',(-50.7114964522535,44.0969987421085,
-216.344065601425));
#191386=CARTESIAN_POINT('Ctrl Pts',(-50.8056178277775,44.1225919052419,
-216.213154850206));
#191387=CARTESIAN_POINT('Ctrl Pts',(-50.3945871449412,44.2852102294111,
-215.949426636203));
#191388=CARTESIAN_POINT('Ctrl Pts',(-50.3238862622841,44.2690849821772,
-216.043975317111));
#191389=CARTESIAN_POINT('Ctrl Pts',(-50.2500250536189,44.2522227786124,
-216.135639498551));
#191390=CARTESIAN_POINT('Ctrl Pts',(-50.1731582085826,44.234703660966,-216.224503324805));
#191391=CARTESIAN_POINT('Ctrl Pts',(-50.0909523255552,44.2159676957354,
-216.319539478597));
#191392=CARTESIAN_POINT('Ctrl Pts',(-50.0053087127001,44.196480421214,-216.411373899394));
#191393=CARTESIAN_POINT('Ctrl Pts',(-49.9163764443311,44.1762907631104,
-216.500100361556));
#191394=CARTESIAN_POINT('Ctrl Pts',(-49.8274441759621,44.1561011050067,
-216.588826823719));
#191395=CARTESIAN_POINT('Ctrl Pts',(-49.7352226059874,44.135208399256,-216.674446234173));
#191396=CARTESIAN_POINT('Ctrl Pts',(-49.6398281339213,44.1136199297675,
-216.75702774159));
#191397=CARTESIAN_POINT('Ctrl Pts',(-56.5998602975341,36.7010789093092,
-217.106689509426));
#191398=CARTESIAN_POINT('Ctrl Pts',(-56.3034738562376,36.8544199785542,
-217.235822749176));
#191399=CARTESIAN_POINT('Ctrl Pts',(-56.3924021524771,37.0639192723716,
-217.511774135751));
#191400=CARTESIAN_POINT('Ctrl Pts',(-56.5630402918383,36.4948001608833,
-217.276505175982));
#191401=CARTESIAN_POINT('Ctrl Pts',(-56.3049395852604,36.6634137058091,
-217.365820774673));
#191402=CARTESIAN_POINT('Ctrl Pts',(-56.3493441379948,36.8590087399585,
-217.613536138229));
#191403=CARTESIAN_POINT('Ctrl Pts',(-56.5022140574202,36.3057210321513,
-217.452921387449));
#191404=CARTESIAN_POINT('Ctrl Pts',(-56.2819498379186,36.4743061370055,
-217.512980511932));
#191405=CARTESIAN_POINT('Ctrl Pts',(-56.2928273312848,36.6682242676255,
-217.719433251733));
#191406=CARTESIAN_POINT('Ctrl Pts',(-56.3592256802117,36.0944966789716,
-217.709486784208));
#191407=CARTESIAN_POINT('Ctrl Pts',(-56.1906627010658,36.2589234334196,
-217.731867301705));
#191408=CARTESIAN_POINT('Ctrl Pts',(-56.1827206487482,36.4479723499478,
-217.873318464));
#191409=CARTESIAN_POINT('Ctrl Pts',(-56.3158477513733,36.0436491754657,
-217.778350695569));
#191410=CARTESIAN_POINT('Ctrl Pts',(-56.1617340323702,36.2072924601779,
-217.789891061158));
#191411=CARTESIAN_POINT('Ctrl Pts',(-56.1506047053284,36.3940866925176,
-217.914618813864));
#191412=CARTESIAN_POINT('Ctrl Pts',(-56.2165191994686,35.9575384315461,
-217.915549753192));
#191413=CARTESIAN_POINT('Ctrl Pts',(-56.0920748178132,36.1188836138303,
-217.905196077141));
#191414=CARTESIAN_POINT('Ctrl Pts',(-56.080012372023,36.3003319845699,-217.996894716944));
#191415=CARTESIAN_POINT('Ctrl Pts',(-56.1595137194348,35.9216038074791,
-217.985179826652));
#191416=CARTESIAN_POINT('Ctrl Pts',(-56.0506116715503,36.0810322659478,
-217.963789723577));
#191417=CARTESIAN_POINT('Ctrl Pts',(-56.0408099000175,36.2597047407171,
-218.038646786212));
#191418=CARTESIAN_POINT('Ctrl Pts',(-56.0329463188087,35.8737089536201,
-218.118234524917));
#191419=CARTESIAN_POINT('Ctrl Pts',(-55.9560538608286,36.0284179459394,
-218.074544890872));
#191420=CARTESIAN_POINT('Ctrl Pts',(-55.9568695408965,36.2006683602997,
-218.118420398712));
#191421=CARTESIAN_POINT('Ctrl Pts',(-55.9615748547198,35.8614000834378,
-218.183336655256));
#191422=CARTESIAN_POINT('Ctrl Pts',(-55.9014450628778,36.0129000216887,
-218.128423068974));
#191423=CARTESIAN_POINT('Ctrl Pts',(-55.9109641207449,36.1817435745309,
-218.157447664942));
#191424=CARTESIAN_POINT('Ctrl Pts',(-55.8107887600364,35.8683604687332,
-218.29848588497));
#191425=CARTESIAN_POINT('Ctrl Pts',(-55.7849297648133,36.0123283043043,
-218.221238015638));
#191426=CARTESIAN_POINT('Ctrl Pts',(-55.8171829211833,36.1739792798186,
-218.226464537285));
#191427=CARTESIAN_POINT('Ctrl Pts',(-55.7298626364341,35.8880162468266,
-218.349466700677));
#191428=CARTESIAN_POINT('Ctrl Pts',(-55.7215158157664,36.0274854463032,
-218.261222954536));
#191429=CARTESIAN_POINT('Ctrl Pts',(-55.7683976723683,36.1853714927186,
-218.257013741027));
#191430=CARTESIAN_POINT('Ctrl Pts',(-55.4296619555845,36.0173958780985,
-218.499755650958));
#191431=CARTESIAN_POINT('Ctrl Pts',(-55.4862779948566,36.1379559621716,
-218.372291428693));
#191432=CARTESIAN_POINT('Ctrl Pts',(-55.5929099869609,36.2828149556278,
-218.347040602773));
#191433=CARTESIAN_POINT('Ctrl Pts',(-55.2185504504437,36.2273017846528,
-218.523434776138));
#191434=CARTESIAN_POINT('Ctrl Pts',(-55.3189357882185,36.3340027933732,
-218.370415986585));
#191435=CARTESIAN_POINT('Ctrl Pts',(-55.4813933689204,36.4668980232678,
-218.361137187739));
#191436=CARTESIAN_POINT('Ctrl Pts',(-55.07865466989,36.4312359741192,-218.492424312504));
#191437=CARTESIAN_POINT('Ctrl Pts',(-55.2233495790564,36.5130164548146,
-218.321717122596));
#191438=CARTESIAN_POINT('Ctrl Pts',(-55.4128172491991,36.6541279382314,
-218.342470788226));
#191439=CARTESIAN_POINT('Ctrl Pts',(-55.2146353748416,36.2578367651479,
-218.504776656653));
#191440=CARTESIAN_POINT('Ctrl Pts',(-55.260640995775,36.2060885425481,-218.50402374007));
#191441=CARTESIAN_POINT('Ctrl Pts',(-55.3103353936485,36.1563189022288,
-218.498881370272));
#191442=CARTESIAN_POINT('Ctrl Pts',(-55.3626215551361,36.1106564380767,
-218.488767188068));
#191443=CARTESIAN_POINT('Ctrl Pts',(-55.4208549058936,36.0598001844186,
-218.477502587586));
#191444=CARTESIAN_POINT('Ctrl Pts',(-55.4823027833847,36.0140385603264,
-218.460070833374));
#191445=CARTESIAN_POINT('Ctrl Pts',(-55.5454444482828,35.9763822852642,
-218.435667388483));
#191446=CARTESIAN_POINT('Ctrl Pts',(-55.5801575945066,35.9556801421612,
-218.422251202005));
#191447=CARTESIAN_POINT('Ctrl Pts',(-55.6153826094992,35.9374290183054,
-218.406727872537));
#191448=CARTESIAN_POINT('Ctrl Pts',(-55.6508670966856,35.9221355025851,
-218.388963715956));
#191449=CARTESIAN_POINT('Ctrl Pts',(-55.7069895268485,35.8979472069096,
-218.36086784319));
#191450=CARTESIAN_POINT('Ctrl Pts',(-55.7640866152408,35.8810200808859,
-218.327001834227));
#191451=CARTESIAN_POINT('Ctrl Pts',(-55.8194769037915,35.8720024376452,
-218.28910047931));
#191452=CARTESIAN_POINT('Ctrl Pts',(-55.8420472117827,35.8683279490187,
-218.273656521963));
#191453=CARTESIAN_POINT('Ctrl Pts',(-55.8643344920639,35.8659663152427,
-218.257542543503));
#191454=CARTESIAN_POINT('Ctrl Pts',(-55.8861588306467,35.8649593048988,
-218.240875914317));
#191455=CARTESIAN_POINT('Ctrl Pts',(-55.9373480158733,35.8625973529513,
-218.201784183528));
#191456=CARTESIAN_POINT('Ctrl Pts',(-55.9866847804406,35.8675108571836,
-218.159221503107));
#191457=CARTESIAN_POINT('Ctrl Pts',(-56.0328916678397,35.87841171425,-218.115098527541));
#191458=CARTESIAN_POINT('Ctrl Pts',(-56.0547315098726,35.8835640413111,
-218.094243653503));
#191459=CARTESIAN_POINT('Ctrl Pts',(-56.075872431505,35.890053191864,-218.073040207613));
#191460=CARTESIAN_POINT('Ctrl Pts',(-56.0961809284015,35.8977394644203,
-218.051689938455));
#191461=CARTESIAN_POINT('Ctrl Pts',(-56.1510011476436,35.9184875852112,
-217.994057586731));
#191462=CARTESIAN_POINT('Ctrl Pts',(-56.2011095262357,35.9482317464444,
-217.934096211335));
#191463=CARTESIAN_POINT('Ctrl Pts',(-56.2458141616989,35.9838108579469,
-217.874493673553));
#191464=CARTESIAN_POINT('Ctrl Pts',(-56.2527092449539,35.9892984529895,
-217.865300791071));
#191465=CARTESIAN_POINT('Ctrl Pts',(-56.2594757994001,35.9949247576492,
-217.856116444932));
#191466=CARTESIAN_POINT('Ctrl Pts',(-56.2661113023919,36.0006780842024,
-217.846950497198));
#191467=CARTESIAN_POINT('Ctrl Pts',(-56.3157684385378,36.0437334065035,
-217.778356644542));
#191468=CARTESIAN_POINT('Ctrl Pts',(-56.3591396849303,36.0945805785127,
-217.709498213182));
#191469=CARTESIAN_POINT('Ctrl Pts',(-56.3967623186957,36.1501656861841,
-217.641985775927));
#191470=CARTESIAN_POINT('Ctrl Pts',(-56.4488863231582,36.2271756695461,
-217.548451160497));
#191471=CARTESIAN_POINT('Ctrl Pts',(-56.4901050623955,36.3123762454183,
-217.458009117953));
#191472=CARTESIAN_POINT('Ctrl Pts',(-56.5229117001721,36.403789675791,-217.369929486757));
#191473=CARTESIAN_POINT('Ctrl Pts',(-56.5374641297148,36.4443390156475,
-217.330858959754));
#191474=CARTESIAN_POINT('Ctrl Pts',(-56.5503610043736,36.4861112162022,
-217.292253272313));
#191475=CARTESIAN_POINT('Ctrl Pts',(-56.5618180211198,36.5289367340068,
-217.254048694965));
#191476=CARTESIAN_POINT('Ctrl Pts',(-56.351930605989,36.892044198215,-217.60005));
#191477=CARTESIAN_POINT('Ctrl Pts',(-56.3410707608223,36.8509068087716,
-217.622000115692));
#191478=CARTESIAN_POINT('Ctrl Pts',(-56.3294340028219,36.810586059083,-217.644150772639));
#191479=CARTESIAN_POINT('Ctrl Pts',(-56.316972640641,36.7712007085407,-217.66656467806));
#191480=CARTESIAN_POINT('Ctrl Pts',(-56.3047871817314,36.7326873771965,
-217.688482323943));
#191481=CARTESIAN_POINT('Ctrl Pts',(-56.2918130999229,36.6950685168439,
-217.710652428266));
#191482=CARTESIAN_POINT('Ctrl Pts',(-56.2779625738601,36.6584665837728,
-217.73311366749));
#191483=CARTESIAN_POINT('Ctrl Pts',(-56.2646565449826,36.6233035599128,
-217.754691901876));
#191484=CARTESIAN_POINT('Ctrl Pts',(-56.2505413393021,36.5890791553865,
-217.776539440422));
#191485=CARTESIAN_POINT('Ctrl Pts',(-56.2355019342317,36.5559117536623,
-217.798662381777));
#191486=CARTESIAN_POINT('Ctrl Pts',(-56.2278151589798,36.5389595962098,
-217.80996961616));
#191487=CARTESIAN_POINT('Ctrl Pts',(-56.2198863685553,36.522283716404,-217.821348279737));
#191488=CARTESIAN_POINT('Ctrl Pts',(-56.211696626409,36.5059008653988,-217.832795341709));
#191489=CARTESIAN_POINT('Ctrl Pts',(-56.1942955844922,36.471091628189,-217.857117329096));
#191490=CARTESIAN_POINT('Ctrl Pts',(-56.1757634090178,36.4377519073116,
-217.881721925024));
#191491=CARTESIAN_POINT('Ctrl Pts',(-56.156087765869,36.4065179517719,-217.90641657657));
#191492=CARTESIAN_POINT('Ctrl Pts',(-56.1430013470316,36.3857440120816,
-217.922841175793));
#191493=CARTESIAN_POINT('Ctrl Pts',(-56.129409171891,36.36590157531,-217.939304646675));
#191494=CARTESIAN_POINT('Ctrl Pts',(-56.1153105737103,36.3471770581247,
-217.95573781425));
#191495=CARTESIAN_POINT('Ctrl Pts',(-56.097662539009,36.3237384917642,-217.976308165138));
#191496=CARTESIAN_POINT('Ctrl Pts',(-56.0790532646516,36.3018583859476,
-217.997031481476));
#191497=CARTESIAN_POINT('Ctrl Pts',(-56.0595942388362,36.2821522564186,
-218.017599237196));
#191498=CARTESIAN_POINT('Ctrl Pts',(-56.0413143454399,36.26364023272,-218.036920676282));
#191499=CARTESIAN_POINT('Ctrl Pts',(-56.0222848102711,36.2470466354578,
-218.056104053989));
#191500=CARTESIAN_POINT('Ctrl Pts',(-56.0026479840161,36.232868550874,-218.074892230468));
#191501=CARTESIAN_POINT('Ctrl Pts',(-56.0013813235415,36.2319540029163,
-218.076104149351));
#191502=CARTESIAN_POINT('Ctrl Pts',(-56.0001121536374,36.2310495008554,
-218.077314425724));
#191503=CARTESIAN_POINT('Ctrl Pts',(-55.9988405197347,36.2301551761968,
-218.078522991535));
#191504=CARTESIAN_POINT('Ctrl Pts',(-55.982614871827,36.2187438753542,-218.093943910471));
#191505=CARTESIAN_POINT('Ctrl Pts',(-55.9658224751974,36.2089101273231,
-218.109248815916));
#191506=CARTESIAN_POINT('Ctrl Pts',(-55.9485977186156,36.2009205165005,
-218.124206031859));
#191507=CARTESIAN_POINT('Ctrl Pts',(-55.9316558911205,36.193062140815,-218.138917564711));
#191508=CARTESIAN_POINT('Ctrl Pts',(-55.9142960214289,36.1869877564012,
-218.153292102777));
#191509=CARTESIAN_POINT('Ctrl Pts',(-55.8966891686622,36.1829396254735,
-218.167132444769));
#191510=CARTESIAN_POINT('Ctrl Pts',(-55.8858924165189,36.1804572587014,
-218.175619523298));
#191511=CARTESIAN_POINT('Ctrl Pts',(-55.875003635279,36.1787366017489,-218.183906226277));
#191512=CARTESIAN_POINT('Ctrl Pts',(-55.8640697402949,36.177831544681,-218.191953009136));
#191513=CARTESIAN_POINT('Ctrl Pts',(-55.8481788303697,36.1765161689285,
-218.203647899363));
#191514=CARTESIAN_POINT('Ctrl Pts',(-55.8320883840851,36.176950108085,-218.214915947184));
#191515=CARTESIAN_POINT('Ctrl Pts',(-55.815945290253,36.1791009722208,-218.225602523972));
#191516=CARTESIAN_POINT('Ctrl Pts',(-55.7998227364087,36.1812490996618,
-218.23627550348));
#191517=CARTESIAN_POINT('Ctrl Pts',(-55.7836481345545,36.1851096628078,
-218.246368068025));
#191518=CARTESIAN_POINT('Ctrl Pts',(-55.7675980596044,36.190642410556,-218.25576790198));
#191519=CARTESIAN_POINT('Ctrl Pts',(-55.752295973037,36.1959173133376,-218.264729671525));
#191520=CARTESIAN_POINT('Ctrl Pts',(-55.7371077176356,36.2027120043589,
-218.273061888544));
#191521=CARTESIAN_POINT('Ctrl Pts',(-55.722205392293,36.2109865653631,-218.280706779267));
#191522=CARTESIAN_POINT('Ctrl Pts',(-55.7011794829243,36.2226612648305,
-218.2914930677));
#191523=CARTESIAN_POINT('Ctrl Pts',(-55.6806056930362,36.2373092093391,
-218.300970061113));
#191524=CARTESIAN_POINT('Ctrl Pts',(-55.6606091228319,36.2544567781787,
-218.309139768336));
#191525=CARTESIAN_POINT('Ctrl Pts',(-55.6403487815878,36.2718305374108,
-218.317417240647));
#191526=CARTESIAN_POINT('Ctrl Pts',(-55.6206817127348,36.2917701088602,
-218.324352790158));
#191527=CARTESIAN_POINT('Ctrl Pts',(-55.6017333911266,36.313784106472,-218.330001945528));
#191528=CARTESIAN_POINT('Ctrl Pts',(-55.5825988134805,36.336014494752,-218.335706630316));
#191529=CARTESIAN_POINT('Ctrl Pts',(-55.5641978473481,36.3603601160687,
-218.340099821307));
#191530=CARTESIAN_POINT('Ctrl Pts',(-55.5466443792723,36.3863189965771,
-218.34328980866));
#191531=CARTESIAN_POINT('Ctrl Pts',(-55.5287333517844,36.4128066524827,
-218.346544775195));
#191532=CARTESIAN_POINT('Ctrl Pts',(-55.5117053063507,36.4409738003648,
-218.348547462775));
#191533=CARTESIAN_POINT('Ctrl Pts',(-55.4956555114404,36.4702939519707,
-218.349460215191));
#191534=CARTESIAN_POINT('Ctrl Pts',(-55.4908481711963,36.479076116825,-218.349733608804));
#191535=CARTESIAN_POINT('Ctrl Pts',(-55.4861283912204,36.4879617787818,
-218.349909507227));
#191536=CARTESIAN_POINT('Ctrl Pts',(-55.4814981831708,36.4969369346298,
-218.349992971048));
#191537=CARTESIAN_POINT('Ctrl Pts',(-50.0071669705522,43.9054798737905,
-217.102435280211));
#191538=CARTESIAN_POINT('Ctrl Pts',(-49.8012110043674,43.8494770305306,
-216.85723677993));
#191539=CARTESIAN_POINT('Ctrl Pts',(-49.6396803417518,44.1134564636829,
-216.757742122242));
#191540=CARTESIAN_POINT('Ctrl Pts',(-49.8231124216493,43.8554323891537,
-217.268463758512));
#191541=CARTESIAN_POINT('Ctrl Pts',(-49.6176813002303,43.7995722598871,
-217.023443915385));
#191542=CARTESIAN_POINT('Ctrl Pts',(-49.4561530329476,44.062897140813,-216.9238167844));
#191543=CARTESIAN_POINT('Ctrl Pts',(-49.6389254121935,43.8053488862956,
-217.43433427542));
#191544=CARTESIAN_POINT('Ctrl Pts',(-49.4339330913007,43.7496080741896,
-217.18956917487));
#191545=CARTESIAN_POINT('Ctrl Pts',(-49.2724911599438,44.0123032282188,
-217.089736149786));
#191546=CARTESIAN_POINT('Ctrl Pts',(-49.4546085996559,43.7552300878266,
-217.60005));
#191547=CARTESIAN_POINT('Ctrl Pts',(-49.249970603928,43.6995856225942,-217.355612986355));
#191548=CARTESIAN_POINT('Ctrl Pts',(-49.0886970638134,43.9616759445554,
-217.255503157469));
#191549=CARTESIAN_POINT('',(-49.4546085996559,43.7552300878266,-217.60005));
#191550=CARTESIAN_POINT('',(-49.0886970638134,43.9616759445554,-217.255503157469));
#191551=CARTESIAN_POINT('Origin',(-49.3234139960799,44.2377111506597,-217.60005));
#191552=CARTESIAN_POINT('Origin',(243.323155334121,-35.8559000200963,132.120548472853));
#191553=CARTESIAN_POINT('Origin',(245.875985088577,-31.0780147762713,132.706328537592));
#191554=CARTESIAN_POINT('Ctrl Pts',(-49.0178780104163,42.4745424717828,
-218.493732307887));
#191555=CARTESIAN_POINT('Ctrl Pts',(-49.0980960592463,42.6213810568613,
-218.320853182002));
#191556=CARTESIAN_POINT('Ctrl Pts',(-49.2388084250474,42.8138811978774,
-218.342362758509));
#191557=CARTESIAN_POINT('Ctrl Pts',(-48.8091338983078,42.6181464793408,
-218.524253922672));
#191558=CARTESIAN_POINT('Ctrl Pts',(-48.9155380997046,42.7194421825587,
-218.369459248669));
#191559=CARTESIAN_POINT('Ctrl Pts',(-49.0487592764839,42.8836112867869,
-218.360708612845));
#191560=CARTESIAN_POINT('Ctrl Pts',(-48.6016721112025,42.8218000792465,
-218.503396057022));
#191561=CARTESIAN_POINT('Ctrl Pts',(-48.7218532551691,42.8806175866196,
-218.373498979651));
#191562=CARTESIAN_POINT('Ctrl Pts',(-48.8668242681005,42.9907156714763,
-218.348253213533));
#191563=CARTESIAN_POINT('Ctrl Pts',(-48.4661332059182,43.1213427546988,
-218.355050582701));
#191564=CARTESIAN_POINT('Ctrl Pts',(-48.605885875072,43.1153009772418,-218.2644789636));
#191565=CARTESIAN_POINT('Ctrl Pts',(-48.7642205550627,43.1653602564368,
-218.259357276092));
#191566=CARTESIAN_POINT('Ctrl Pts',(-48.4447516601516,43.2015723683891,
-218.304994898973));
#191567=CARTESIAN_POINT('Ctrl Pts',(-48.5891386757002,43.1781849693815,
-218.225378312719));
#191568=CARTESIAN_POINT('Ctrl Pts',(-48.7512938451062,43.2136227234323,
-218.22935608099));
#191569=CARTESIAN_POINT('Ctrl Pts',(-48.4340253069588,43.353231429575,-218.190096441368));
#191570=CARTESIAN_POINT('Ctrl Pts',(-48.5863164838715,43.2954705062034,
-218.133030438493));
#191571=CARTESIAN_POINT('Ctrl Pts',(-48.7558233667416,43.3078094106078,
-218.160482894395));
#191572=CARTESIAN_POINT('Ctrl Pts',(-48.4443958234858,43.4248105481098,
-218.125333427438));
#191573=CARTESIAN_POINT('Ctrl Pts',(-48.6000491587584,43.350341157598,-218.079542364176));
#191574=CARTESIAN_POINT('Ctrl Pts',(-48.7730167596744,43.3537994708901,
-218.121658642789));
#191575=CARTESIAN_POINT('Ctrl Pts',(-48.5123865938013,43.6182701882203,
-217.923222587033));
#191576=CARTESIAN_POINT('Ctrl Pts',(-48.6760379810556,43.4959492709514,
-217.910707343414));
#191577=CARTESIAN_POINT('Ctrl Pts',(-48.8584723261946,43.4820777039722,
-218.00048845563));
#191578=CARTESIAN_POINT('Ctrl Pts',(-48.6035264565663,43.717348604409,-217.781587449044));
#191579=CARTESIAN_POINT('Ctrl Pts',(-48.7709936545123,43.5654352430393,
-217.790234240818));
#191580=CARTESIAN_POINT('Ctrl Pts',(-48.9571822978595,43.553382015829,-217.915564471715));
#191581=CARTESIAN_POINT('Ctrl Pts',(-48.8654374280519,43.8999422120516,
-217.456900727715));
#191582=CARTESIAN_POINT('Ctrl Pts',(-49.0360392072996,43.6817910219716,
-217.51611428222));
#191583=CARTESIAN_POINT('Ctrl Pts',(-49.2307518461237,43.6941518993825,
-217.720864823318));
#191584=CARTESIAN_POINT('Ctrl Pts',(-49.0543447941743,43.9629792153545,
-217.278009186719));
#191585=CARTESIAN_POINT('Ctrl Pts',(-49.2254032660268,43.7067173749548,
-217.366834723765));
#191586=CARTESIAN_POINT('Ctrl Pts',(-49.4213823984297,43.752590477188,-217.613522274393));
#191587=CARTESIAN_POINT('Ctrl Pts',(-49.2609648429284,44.000805570189,-217.106705723199));
#191588=CARTESIAN_POINT('Ctrl Pts',(-49.4167540467718,43.705944922211,-217.235986860284));
#191589=CARTESIAN_POINT('Ctrl Pts',(-49.626471378184,43.7968795640925,-217.51089121997));
#191590=CARTESIAN_POINT('Ctrl Pts',(-49.0801870931398,42.8824343798319,
-218.350025764149));
#191591=CARTESIAN_POINT('Ctrl Pts',(-48.9534766000575,42.9465755146882,
-218.349260885044));
#191592=CARTESIAN_POINT('Ctrl Pts',(-48.8452234864083,43.0274829525206,
-218.329538279335));
#191593=CARTESIAN_POINT('Ctrl Pts',(-48.7642205550627,43.1653602564368,
-218.259357276092));
#191594=CARTESIAN_POINT('Ctrl Pts',(-48.7512938451062,43.2136227234323,
-218.22935608099));
#191595=CARTESIAN_POINT('Ctrl Pts',(-48.7558233667416,43.3078094106078,
-218.160482894395));
#191596=CARTESIAN_POINT('Ctrl Pts',(-48.7730167596744,43.3537994708901,
-218.121658642789));
#191597=CARTESIAN_POINT('Ctrl Pts',(-48.8584723261946,43.4820777039722,
-218.00048845563));
#191598=CARTESIAN_POINT('Ctrl Pts',(-48.9571822978595,43.553382015829,-217.915564471715));
#191599=CARTESIAN_POINT('Ctrl Pts',(-49.185156921413,43.6706902521236,-217.753314764718));
#191600=CARTESIAN_POINT('Ctrl Pts',(-49.3149852106482,43.7172641725154,
-217.675369628552));
#191601=CARTESIAN_POINT('Ctrl Pts',(-49.4546085996559,43.7552300878266,
-217.60005));
#191602=CARTESIAN_POINT('Ctrl Pts',(-49.0886970638135,43.9616759445554,
-217.255503157469));
#191603=CARTESIAN_POINT('Ctrl Pts',(-48.9996384348295,43.9371441712379,
-217.335826637108));
#191604=CARTESIAN_POINT('Ctrl Pts',(-48.9153759396057,43.9062608655704,
-217.417907561279));
#191605=CARTESIAN_POINT('Ctrl Pts',(-48.8376533259605,43.867295402887,-217.502023817251));
#191606=CARTESIAN_POINT('Ctrl Pts',(-48.7938257341564,43.8453228737497,
-217.54945676833));
#191607=CARTESIAN_POINT('Ctrl Pts',(-48.7520786392416,43.8207798060945,
-217.597536915137));
#191608=CARTESIAN_POINT('Ctrl Pts',(-48.7127298749802,43.7933510418827,
-217.646314085193));
#191609=CARTESIAN_POINT('Ctrl Pts',(-48.650249816921,43.7497981930802,-217.7237650668));
#191610=CARTESIAN_POINT('Ctrl Pts',(-48.5936606238927,43.6987010978059,
-217.803297027915));
#191611=CARTESIAN_POINT('Ctrl Pts',(-48.5481954561807,43.6387791465335,
-217.882424454102));
#191612=CARTESIAN_POINT('Ctrl Pts',(-48.5142503744661,43.5940403798072,
-217.941502361058));
#191613=CARTESIAN_POINT('Ctrl Pts',(-48.4865083692682,43.5443812052436,
-218.000354765105));
#191614=CARTESIAN_POINT('Ctrl Pts',(-48.4671318833214,43.4892557804674,
-218.057947213938));
#191615=CARTESIAN_POINT('Ctrl Pts',(-48.451525691629,43.4448567109691,-218.104333271708));
#191616=CARTESIAN_POINT('Ctrl Pts',(-48.4417433467026,43.3970966887457,
-218.149483053803));
#191617=CARTESIAN_POINT('Ctrl Pts',(-48.4389192647052,43.3468995389881,
-218.191860029397));
#191618=CARTESIAN_POINT('Ctrl Pts',(-48.4376420131691,43.3241968034818,
-218.211025923738));
#191619=CARTESIAN_POINT('Ctrl Pts',(-48.4377874434161,43.3009957695441,
-218.229624642104));
#191620=CARTESIAN_POINT('Ctrl Pts',(-48.4394571325143,43.2773831398461,
-218.247514037176));
#191621=CARTESIAN_POINT('Ctrl Pts',(-48.4431471229734,43.2251995456732,
-218.287049359771));
#191622=CARTESIAN_POINT('Ctrl Pts',(-48.4544207656835,43.1709349171637,
-218.323082627899));
#191623=CARTESIAN_POINT('Ctrl Pts',(-48.4727225097299,43.1164732147517,
-218.354432513868));
#191624=CARTESIAN_POINT('Ctrl Pts',(-48.4810127962298,43.0918032644386,
-218.368633320947));
#191625=CARTESIAN_POINT('Ctrl Pts',(-48.4907445774782,43.0670933250239,
-218.381873149416));
#191626=CARTESIAN_POINT('Ctrl Pts',(-48.5018636359549,43.0425207969075,
-218.394042199469));
#191627=CARTESIAN_POINT('Ctrl Pts',(-48.5333210340713,42.9730016194245,
-218.428470173117));
#191628=CARTESIAN_POINT('Ctrl Pts',(-48.575477165605,42.9051779351441,-218.45412189569));
#191629=CARTESIAN_POINT('Ctrl Pts',(-48.6249680219686,42.8403879458241,
-218.472156073002));
#191630=CARTESIAN_POINT('Ctrl Pts',(-48.6690863768606,42.7826312620184,
-218.48823254234));
#191631=CARTESIAN_POINT('Ctrl Pts',(-48.7190328297175,42.7272860740426,
-218.498255550998));
#191632=CARTESIAN_POINT('Ctrl Pts',(-48.7724676216828,42.675306362178,-218.503045934624));
#191633=CARTESIAN_POINT('Ctrl Pts',(-48.7950121526649,42.6533757401717,
-218.505067032641));
#191634=CARTESIAN_POINT('Ctrl Pts',(-48.8181782375201,42.6320442164686,
-218.506156693031));
#191635=CARTESIAN_POINT('Ctrl Pts',(-48.8417930108281,42.6113834075459,
-218.506376562157));
#191636=CARTESIAN_POINT('Origin',(2.81802535037841,-9.69927298715315,-227.60005));
#191637=CARTESIAN_POINT('',(-48.1633319901564,41.4530789012665,-228.35005));
#191638=CARTESIAN_POINT('',(-48.1633319901564,41.4530789012665,-228.35005));
#191639=CARTESIAN_POINT('',(-47.632114758242,41.9825203546087,-227.60005));
#191640=CARTESIAN_POINT('Origin',(-48.1633319901564,41.4530789012665,-227.60005));
#191641=CARTESIAN_POINT('',(-41.9598150400404,36.2911954009805,-227.60005));
#191642=CARTESIAN_POINT('Ctrl Pts',(-49.7021444432209,42.0348313420379,
-227.60005));
#191643=CARTESIAN_POINT('Ctrl Pts',(-48.6421799545279,42.9959733704936,
-227.60005));
#191644=CARTESIAN_POINT('Ctrl Pts',(-47.6321147582419,41.9825203546088,
-227.60005));
#191645=CARTESIAN_POINT('Ctrl Pts',(-49.7021444432209,42.0348313420379,
-228.35005));
#191646=CARTESIAN_POINT('Ctrl Pts',(-48.6421799545279,42.9959733704936,
-228.35005));
#191647=CARTESIAN_POINT('Ctrl Pts',(-47.6321147582419,41.9825203546088,
-228.35005));
#191648=CARTESIAN_POINT('Ctrl Pts',(-49.1983468326458,41.479234394981,-228.35005));
#191649=CARTESIAN_POINT('Ctrl Pts',(-48.6683645882994,41.9598054092088,
-228.35005));
#191650=CARTESIAN_POINT('Ctrl Pts',(-48.1633319901564,41.4530789012665,
-228.35005));
#191651=CARTESIAN_POINT('',(-49.7021444432209,42.0348313420379,-227.60005));
#191652=CARTESIAN_POINT('Origin',(-48.6945492220708,40.9236374479242,-227.60005));
#191653=CARTESIAN_POINT('',(-49.1983468326459,41.4792343949811,-228.35005));
#191654=CARTESIAN_POINT('Origin',(-48.6945492220708,40.9236374479242,-228.35005));
#191655=CARTESIAN_POINT('Origin',(-49.1983468326459,41.4792343949811,-227.60005));
#191656=CARTESIAN_POINT('Origin',(-0.128459562639233,-12.6359082483571,
-227.60005));
#191657=CARTESIAN_POINT('',(-54.0789914828443,36.6149049990089,-228.35005));
#191658=CARTESIAN_POINT('Origin',(-0.128459562639233,-12.6359082483571,
-228.35005));
#191659=CARTESIAN_POINT('',(-54.6328983814091,37.1205601658197,-227.60005));
#191660=CARTESIAN_POINT('Origin',(-54.0789914828443,36.6149049990089,-227.60005));
#191661=CARTESIAN_POINT('Origin',(-0.128459562639233,-12.6359082483571,
-227.60005));
#191662=CARTESIAN_POINT('Origin',(-0.128459562639233,-12.6359082483571,
-228.35005));
#191663=CARTESIAN_POINT('Ctrl Pts',(-54.5875190481084,35.0503669255137,
-227.60005));
#191664=CARTESIAN_POINT('Ctrl Pts',(-55.5975842443944,36.0638199413983,
-227.60005));
#191665=CARTESIAN_POINT('Ctrl Pts',(-54.6328983814091,37.1205601658197,
-227.60005));
#191666=CARTESIAN_POINT('Ctrl Pts',(-54.5875190481084,35.0503669255137,
-228.35005));
#191667=CARTESIAN_POINT('Ctrl Pts',(-55.5975842443944,36.0638199413983,
-228.35005));
#191668=CARTESIAN_POINT('Ctrl Pts',(-54.6328983814091,37.1205601658197,
-228.35005));
#191669=CARTESIAN_POINT('Ctrl Pts',(-54.056301816194,35.579808378856,-228.35005));
#191670=CARTESIAN_POINT('Ctrl Pts',(-54.5613344143369,36.0865348867983,
-228.35005));
#191671=CARTESIAN_POINT('Ctrl Pts',(-54.0789914828443,36.614904999009,-228.35005));
#191672=CARTESIAN_POINT('',(-54.5875190481084,35.0503669255136,-227.60005));
#191673=CARTESIAN_POINT('',(-54.056301816194,35.579808378856,-228.35005));
#191674=CARTESIAN_POINT('Origin',(-54.056301816194,35.579808378856,-227.60005));
#191675=CARTESIAN_POINT('Origin',(-53.5250845842796,36.1092498321983,-227.60005));
#191676=CARTESIAN_POINT('Origin',(-53.5250845842796,36.1092498321983,-228.35005));
#191677=CARTESIAN_POINT('Origin',(-3.07494447565784,-15.5725435095623,-227.60005));
#191678=CARTESIAN_POINT('',(-54.5875190481084,35.0503669255136,-227.60005));
#191679=CARTESIAN_POINT('',(-48.3142830765682,29.8185305620001,-228.35005));
#191680=CARTESIAN_POINT('Origin',(10.7603008067452,26.6045648983079,-217.60005));
#191681=CARTESIAN_POINT('',(-51.0024097331414,43.3988703109923,-218.35005));
#191682=CARTESIAN_POINT('',(10.7603008067452,26.6045648983079,-218.35005));
#191683=CARTESIAN_POINT('',(-50.8056178277775,44.122591905242,-217.60005));
#191684=CARTESIAN_POINT('Origin',(-51.0024097331414,43.3988703109923,-217.60005));
#191685=CARTESIAN_POINT('',(-51.6000409161409,44.3386087195339,-217.60005));
#191686=CARTESIAN_POINT('Ctrl Pts',(-52.2148720050704,43.7789665035542,
-217.60005));
#191687=CARTESIAN_POINT('Ctrl Pts',(-51.6051500510689,44.3399979780626,
-217.60005));
#191688=CARTESIAN_POINT('Ctrl Pts',(-50.8056178277775,44.1225919052419,
-217.60005));
#191689=CARTESIAN_POINT('Ctrl Pts',(-52.2148720050704,43.7789665035542,
-218.35005));
#191690=CARTESIAN_POINT('Ctrl Pts',(-51.6051500510689,44.3399979780626,
-218.35005));
#191691=CARTESIAN_POINT('Ctrl Pts',(-50.8056178277775,44.1225919052419,
-218.35005));
#191692=CARTESIAN_POINT('Ctrl Pts',(-51.7070368217878,43.2270576101484,
-218.35005));
#191693=CARTESIAN_POINT('Ctrl Pts',(-51.4021758447871,43.5075733474026,
-218.35005));
#191694=CARTESIAN_POINT('Ctrl Pts',(-51.0024097331414,43.3988703109923,
-218.35005));
#191695=CARTESIAN_POINT('',(-52.2148720050704,43.7789665035542,-217.60005));
#191696=CARTESIAN_POINT('Origin',(-51.1992016385053,42.6751487167426,-217.60005));
#191697=CARTESIAN_POINT('',(-51.7070368217878,43.2270576101484,-218.35005));
#191698=CARTESIAN_POINT('Origin',(-51.1992016385053,42.6751487167426,-218.35005));
#191699=CARTESIAN_POINT('Origin',(-51.7070368217878,43.2270576101484,-217.60005));
#191700=CARTESIAN_POINT('Origin',(0.,-12.9675000200281,-217.60005));
#191701=CARTESIAN_POINT('',(-56.3587426896623,39.6656306474361,-217.60005));
#191702=CARTESIAN_POINT('',(-55.8106047487975,39.1537275337666,-218.35005));
#191703=CARTESIAN_POINT('Origin',(-55.8106047487975,39.1537275337666,-217.60005));
#191704=CARTESIAN_POINT('Origin',(0.,-12.9675000200281,-217.60005));
#191705=CARTESIAN_POINT('Origin',(0.,-12.9675000200281,-218.35005));
#191706=CARTESIAN_POINT('Ctrl Pts',(-56.7127812850717,38.2589564044561,
-217.60005));
#191707=CARTESIAN_POINT('Ctrl Pts',(-56.9242682147177,39.0600746573811,
-217.60005));
#191708=CARTESIAN_POINT('Ctrl Pts',(-56.3587426896623,39.6656306474361,
-217.60005));
#191709=CARTESIAN_POINT('Ctrl Pts',(-56.7127812850717,38.2589564044561,
-218.35005));
#191710=CARTESIAN_POINT('Ctrl Pts',(-56.9242682147177,39.0600746573811,
-218.35005));
#191711=CARTESIAN_POINT('Ctrl Pts',(-56.3587426896623,39.6656306474361,
-218.35005));
#191712=CARTESIAN_POINT('Ctrl Pts',(-55.9876240465022,38.4503904122767,
-218.35005));
#191713=CARTESIAN_POINT('Ctrl Pts',(-56.0933675113252,38.8509495387392,
-218.35005));
#191714=CARTESIAN_POINT('Ctrl Pts',(-55.8106047487975,39.1537275337666,
-218.35005));
#191715=CARTESIAN_POINT('',(-56.7127812850717,38.2589564044561,-217.60005));
#191716=CARTESIAN_POINT('',(-55.9876240465022,38.4503904122767,-218.35005));
#191717=CARTESIAN_POINT('Origin',(-55.9876240465022,38.4503904122767,-217.60005));
#191718=CARTESIAN_POINT('Origin',(-55.2624668079327,38.6418244200972,-217.60005));
#191719=CARTESIAN_POINT('Origin',(-55.2624668079327,38.6418244200972,-218.35005));
#191720=CARTESIAN_POINT('Origin',(-39.6505639028577,-23.4348386281926,-217.60005));
#191721=CARTESIAN_POINT('',(-51.3278340104563,17.8606293780317,-217.60005));
#191722=CARTESIAN_POINT('',(-39.6505639028577,-23.4348386281926,-218.35005));
#191723=CARTESIAN_POINT('Origin',(-39.6266165499379,-2.40986505017056,-217.60005));
#191724=CARTESIAN_POINT('',(-56.1046081325044,-64.2577178902918,-218.35005));
#191725=CARTESIAN_POINT('',(-56.1046081325044,-64.2577178902918,-218.35005));
#191726=CARTESIAN_POINT('',(-56.8293274051384,-64.0646324794683,-217.60005));
#191727=CARTESIAN_POINT('Origin',(-56.1046081325044,-64.2577178902918,-217.60005));
#191728=CARTESIAN_POINT('',(-56.0236521904458,-61.0406424582598,-217.60005));
#191729=CARTESIAN_POINT('Ctrl Pts',(-56.1046081325044,-64.2577178902918,
-218.35005));
#191730=CARTESIAN_POINT('Ctrl Pts',(-56.2112637919648,-64.658035095081,
-218.35005));
#191731=CARTESIAN_POINT('Ctrl Pts',(-55.9291914878272,-64.9614564347782,
-218.35005));
#191732=CARTESIAN_POINT('Ctrl Pts',(-56.8293274051384,-64.0646324794683,
-218.35005));
#191733=CARTESIAN_POINT('Ctrl Pts',(-57.0426387240591,-64.8652668890467,
-218.35005));
#191734=CARTESIAN_POINT('Ctrl Pts',(-56.478494115784,-65.4721095684411,
-218.35005));
#191735=CARTESIAN_POINT('Ctrl Pts',(-56.8293274051384,-64.0646324794683,
-217.60005));
#191736=CARTESIAN_POINT('Ctrl Pts',(-57.0426387240591,-64.8652668890467,
-217.60005));
#191737=CARTESIAN_POINT('Ctrl Pts',(-56.478494115784,-65.4721095684411,
-217.60005));
#191738=CARTESIAN_POINT('',(-56.478494115784,-65.4721095684411,-217.60005));
#191739=CARTESIAN_POINT('',(-55.9291914878272,-64.9614564347782,-218.35005));
#191740=CARTESIAN_POINT('Origin',(-55.9291914878272,-64.9614564347782,-217.60005));
#191741=CARTESIAN_POINT('Origin',(-55.3798888598704,-64.4508033011153,-217.60005));
#191742=CARTESIAN_POINT('Origin',(-55.3798888598704,-64.4508033011153,-218.35005));
#191743=CARTESIAN_POINT('Origin',(0.,-12.9675000200281,-217.60005));
#191744=CARTESIAN_POINT('',(-52.3440043138885,-69.594874440935,-217.60005));
#191745=CARTESIAN_POINT('',(-51.8349132062458,-69.0441238221254,-218.35005));
#191746=CARTESIAN_POINT('Origin',(-51.8349132062458,-69.0441238221255,-217.60005));
#191747=CARTESIAN_POINT('Origin',(0.,-12.9675000200281,-217.60005));
#191748=CARTESIAN_POINT('Origin',(0.,-12.9675000200281,-218.35005));
#191749=CARTESIAN_POINT('Ctrl Pts',(-51.8349132062458,-69.0441238221254,
-218.35005));
#191750=CARTESIAN_POINT('Ctrl Pts',(-51.5306920318089,-69.3253333012854,
-218.35005));
#191751=CARTESIAN_POINT('Ctrl Pts',(-51.1306793331593,-69.2175412094409,
-218.35005));
#191752=CARTESIAN_POINT('Ctrl Pts',(-52.3440043138886,-69.5948744409349,
-218.35005));
#191753=CARTESIAN_POINT('Ctrl Pts',(-51.7355619650149,-70.1572933992548,
-218.35005));
#191754=CARTESIAN_POINT('Ctrl Pts',(-50.9355365677156,-69.9417092155658,
-218.35005));
#191755=CARTESIAN_POINT('Ctrl Pts',(-52.3440043138886,-69.5948744409349,
-217.60005));
#191756=CARTESIAN_POINT('Ctrl Pts',(-51.7355619650149,-70.1572933992548,
-217.60005));
#191757=CARTESIAN_POINT('Ctrl Pts',(-50.9355365677156,-69.9417092155658,
-217.60005));
#191758=CARTESIAN_POINT('',(-51.1306793331593,-69.2175412094409,-218.35005));
#191759=CARTESIAN_POINT('Origin',(-51.325822098603,-68.4933732033159,-218.35005));
#191760=CARTESIAN_POINT('',(-50.9355365677156,-69.9417092155658,-217.60005));
#191761=CARTESIAN_POINT('Origin',(-51.1306793331593,-69.2175412094409,-217.60005));
#191762=CARTESIAN_POINT('Origin',(-51.325822098603,-68.4933732033159,-217.60005));
#191763=CARTESIAN_POINT('Origin',(10.6701281871898,-52.5639741032288,-217.60005));
#191764=CARTESIAN_POINT('',(-50.9355365677156,-69.9417092155658,-217.60005));
#191765=CARTESIAN_POINT('',(-48.0054978778587,-68.3753933286417,-218.35005));
#191766=CARTESIAN_POINT('Origin',(-3.09688044790867,-9.95712216328114,-227.60005));
#191767=CARTESIAN_POINT('',(-53.6770468827139,-61.5062120042031,-228.35005));
#191768=CARTESIAN_POINT('',(-3.09688044790867,-9.95712216328114,-228.35005));
#191769=CARTESIAN_POINT('',(-54.2123842387114,-60.9809369188682,-227.60005));
#191770=CARTESIAN_POINT('Origin',(-53.6770468827139,-61.5062120042031,-227.60005));
#191771=CARTESIAN_POINT('',(-55.2047656166361,-61.9923285455256,-227.60005));
#191772=CARTESIAN_POINT('Ctrl Pts',(-53.6770468827138,-61.5062120042031,
-228.35005));
#191773=CARTESIAN_POINT('Ctrl Pts',(-54.1781051950386,-62.0168686860244,
-228.35005));
#191774=CARTESIAN_POINT('Ctrl Pts',(-53.6916490178651,-62.5414543003222,
-228.35005));
#191775=CARTESIAN_POINT('Ctrl Pts',(-54.2123842387114,-60.9809369188682,
-228.35005));
#191776=CARTESIAN_POINT('Ctrl Pts',(-55.2145008633609,-62.0022502825108,
-228.35005));
#191777=CARTESIAN_POINT('Ctrl Pts',(-54.2415885090139,-63.0514215111064,
-228.35005));
#191778=CARTESIAN_POINT('Ctrl Pts',(-54.2123842387114,-60.9809369188682,
-227.60005));
#191779=CARTESIAN_POINT('Ctrl Pts',(-55.2145008633609,-62.0022502825108,
-227.60005));
#191780=CARTESIAN_POINT('Ctrl Pts',(-54.2415885090139,-63.0514215111064,
-227.60005));
#191781=CARTESIAN_POINT('',(-54.2415885090138,-63.0514215111064,-227.60005));
#191782=CARTESIAN_POINT('',(-53.6916490178651,-62.5414543003222,-228.35005));
#191783=CARTESIAN_POINT('Origin',(-53.6916490178651,-62.5414543003222,-227.60005));
#191784=CARTESIAN_POINT('Origin',(-53.1417095267163,-62.031487089538,-227.60005));
#191785=CARTESIAN_POINT('Origin',(-53.1417095267163,-62.031487089538,-228.35005));
#191786=CARTESIAN_POINT('Origin',(-0.127542579976414,-12.8706479699377,
-227.60005));
#191787=CARTESIAN_POINT('',(-49.2725916132775,-67.9270204940557,-227.60005));
#191788=CARTESIAN_POINT('',(-48.7731500580611,-67.3675045131195,-228.35005));
#191789=CARTESIAN_POINT('Origin',(-48.7731500580611,-67.3675045131195,-227.60005));
#191790=CARTESIAN_POINT('Origin',(-0.127542579976414,-12.8706479699377,
-227.60005));
#191791=CARTESIAN_POINT('Origin',(-0.127542579976414,-12.8706479699377,
-228.35005));
#191792=CARTESIAN_POINT('Ctrl Pts',(-48.7731500580611,-67.3675045131195,
-228.35005));
#191793=CARTESIAN_POINT('Ctrl Pts',(-48.2394294591717,-67.8439202993396,
-228.35005));
#191794=CARTESIAN_POINT('Ctrl Pts',(-47.738371146847,-67.3332636175182,
-228.35005));
#191795=CARTESIAN_POINT('Ctrl Pts',(-49.2725916132776,-67.9270204940556,
-228.35005));
#191796=CARTESIAN_POINT('Ctrl Pts',(-48.2051504154989,-68.8798520664959,
-228.35005));
#191797=CARTESIAN_POINT('Ctrl Pts',(-47.2030337908494,-67.858538702853,
-228.35005));
#191798=CARTESIAN_POINT('Ctrl Pts',(-49.2725916132776,-67.9270204940556,
-227.60005));
#191799=CARTESIAN_POINT('Ctrl Pts',(-48.2051504154989,-68.8798520664959,
-227.60005));
#191800=CARTESIAN_POINT('Ctrl Pts',(-47.2030337908494,-67.858538702853,
-227.60005));
#191801=CARTESIAN_POINT('',(-47.738371146847,-67.3332636175182,-228.35005));
#191802=CARTESIAN_POINT('Origin',(-48.2737085028446,-66.8079885321834,-228.35005));
#191803=CARTESIAN_POINT('',(-47.2030337908494,-67.858538702853,-227.60005));
#191804=CARTESIAN_POINT('Origin',(-47.738371146847,-67.3332636175182,-227.60005));
#191805=CARTESIAN_POINT('Origin',(-48.2737085028446,-66.8079885321834,-227.60005));
#191806=CARTESIAN_POINT('Origin',(2.84179528795572,-15.7841737765938,-227.60005));
#191807=CARTESIAN_POINT('',(-48.1954151687739,-68.8699303295103,-227.60005));
#191808=CARTESIAN_POINT('',(2.84179528795573,-15.7841737765938,-228.35005));
#191809=CARTESIAN_POINT('Origin',(-55.2624668079327,38.6418244200972,-167.906149834141));
#191810=CARTESIAN_POINT('',(-56.3587426896623,39.6656306474361,-167.906149834141));
#191811=CARTESIAN_POINT('',(-56.7127812850717,38.2589564044561,-167.906149834141));
#191812=CARTESIAN_POINT('Origin',(-51.1992016385053,42.6751487167426,-167.906149834141));
#191813=CARTESIAN_POINT('',(-50.8056178277775,44.1225919052419,-167.906149834141));
#191814=CARTESIAN_POINT('',(-52.2148720050704,43.7789665035542,-167.906149834141));
#191815=CARTESIAN_POINT('Origin',(-53.5250845842796,36.1092498321983,-228.35005));
#191816=CARTESIAN_POINT('',(-54.6328983814091,37.1205601658197,-228.35005));
#191817=CARTESIAN_POINT('',(-54.5875190481084,35.0503669255136,-228.35005));
#191818=CARTESIAN_POINT('Origin',(-48.6945492220708,40.9236374479242,-228.35005));
#191819=CARTESIAN_POINT('',(-47.632114758242,41.9825203546087,-228.35005));
#191820=CARTESIAN_POINT('',(-49.7021444432209,42.0348313420379,-228.35005));
#191821=CARTESIAN_POINT('Origin',(-53.1417095267163,-62.031487089538,-228.35005));
#191822=CARTESIAN_POINT('',(-54.2123842387114,-60.9809369188682,-228.35005));
#191823=CARTESIAN_POINT('',(-54.2415885090138,-63.0514215111064,-228.35005));
#191824=CARTESIAN_POINT('Origin',(-48.2737085028446,-66.8079885321834,-228.35005));
#191825=CARTESIAN_POINT('',(-47.2030337908494,-67.858538702853,-228.35005));
#191826=CARTESIAN_POINT('',(-49.2725916132775,-67.9270204940557,-228.35005));
#191827=CARTESIAN_POINT('Origin',(-51.325822098603,-68.4933732033159,-167.906149834141));
#191828=CARTESIAN_POINT('',(-52.3440043138885,-69.594874440935,-167.906149834141));
#191829=CARTESIAN_POINT('',(-50.9355365677156,-69.9417092155658,-167.906149834141));
#191830=CARTESIAN_POINT('Origin',(-55.3798888598704,-64.4508033011153,-167.906149834141));
#191831=CARTESIAN_POINT('',(-56.8293274051384,-64.0646324794683,-167.906149834141));
#191832=CARTESIAN_POINT('',(-56.478494115784,-65.4721095684411,-167.906149834141));
#191833=CARTESIAN_POINT('Origin',(-21.5,29.0311209585238,-234.90005));
#191834=CARTESIAN_POINT('',(-21.6266284449832,30.2244211038859,-235.35005));
#191835=CARTESIAN_POINT('',(-20.3,29.0311209585238,-235.35005));
#191836=CARTESIAN_POINT('Origin',(-21.5,29.0311209585238,-235.35005));
#191837=CARTESIAN_POINT('',(-20.75,29.0311209585238,-234.90005));
#191838=CARTESIAN_POINT('Origin',(-20.3,29.0311209585238,-234.90005));
#191839=CARTESIAN_POINT('',(-21.5791427781145,29.7769335493751,-234.90005));
#191840=CARTESIAN_POINT('Origin',(-21.5,29.0311209585238,-234.90005));
#191841=CARTESIAN_POINT('Origin',(-21.6266284449832,30.2244211038859,-234.90005));
#191842=CARTESIAN_POINT('Origin',(-20.3,-25.4138432731711,-234.90005));
#191843=CARTESIAN_POINT('',(-20.75,21.5631368321642,-234.90005));
#191844=CARTESIAN_POINT('',(-20.3,21.5631368321642,-235.35005));
#191845=CARTESIAN_POINT('Origin',(-20.3,21.5631368321642,-234.90005));
#191846=CARTESIAN_POINT('',(-20.75,29.0311209585238,-234.90005));
#191847=CARTESIAN_POINT('',(-20.3,21.5631368321642,-235.35005));
#191848=CARTESIAN_POINT('Origin',(2.61456814389029E-14,-173.57701443073,
-234.90005));
#191849=CARTESIAN_POINT('',(-25.0152849219089,29.8362882417925,-235.35005));
#191850=CARTESIAN_POINT('',(-24.960358769668,29.3896529120211,-234.90005));
#191851=CARTESIAN_POINT('Origin',(-25.0152849219089,29.8362882417925,-234.90005));
#191852=CARTESIAN_POINT('Origin',(2.61456814389029E-14,-173.57701443073,
-235.35005));
#191853=CARTESIAN_POINT('Origin',(2.61456814389029E-14,-173.57701443073,
-234.90005));
#191854=CARTESIAN_POINT('Origin',(-21.5,21.5631368321642,-234.90005));
#191855=CARTESIAN_POINT('',(-21.5,20.8131368321642,-234.90005));
#191856=CARTESIAN_POINT('',(-21.5,20.3631368321642,-235.35005));
#191857=CARTESIAN_POINT('Origin',(-21.5,20.3631368321642,-234.90005));
#191858=CARTESIAN_POINT('Origin',(-21.5,21.5631368321642,-234.90005));
#191859=CARTESIAN_POINT('Origin',(-21.5,21.5631368321642,-235.35005));
#191860=CARTESIAN_POINT('Origin',(-24.838300653577,28.3971299569735,-234.90005));
#191861=CARTESIAN_POINT('',(-25.604588652464,29.6281062779325,-235.35005));
#191862=CARTESIAN_POINT('',(-25.366775135568,29.2460791438418,-234.90005));
#191863=CARTESIAN_POINT('Origin',(-25.604588652464,29.6281062779325,-234.90005));
#191864=CARTESIAN_POINT('Origin',(-24.838300653577,28.3971299569735,-235.35005));
#191865=CARTESIAN_POINT('Origin',(-24.838300653577,28.3971299569735,-234.90005));
#191866=CARTESIAN_POINT('Origin',(296.501483394397,20.3631368321642,-234.90005));
#191867=CARTESIAN_POINT('',(-29.125,20.8131368321642,-234.90005));
#191868=CARTESIAN_POINT('',(-29.125,20.3631368321642,-235.35005));
#191869=CARTESIAN_POINT('Origin',(-29.125,20.3631368321642,-234.90005));
#191870=CARTESIAN_POINT('',(1.23757166668304E-15,20.8131368321642,-234.90005));
#191871=CARTESIAN_POINT('',(296.501483394397,20.3631368321642,-235.35005));
#191872=CARTESIAN_POINT('Origin',(6.29739814579425E-15,-11.5034818258363,
-234.90005));
#191873=CARTESIAN_POINT('',(-29.8646825396825,26.6475763089516,-235.35005));
#191874=CARTESIAN_POINT('',(-29.5873015873016,26.2932321157492,-234.90005));
#191875=CARTESIAN_POINT('Origin',(-29.8646825396825,26.6475763089516,-234.90005));
#191876=CARTESIAN_POINT('Origin',(6.29739814579425E-15,-11.5034818258363,
-235.35005));
#191877=CARTESIAN_POINT('Origin',(6.29739814579425E-15,-11.5034818258363,
-234.90005));
#191878=CARTESIAN_POINT('Origin',(-29.125,21.5631368321642,-234.90005));
#191879=CARTESIAN_POINT('',(-29.875,21.5631368321642,-234.90005));
#191880=CARTESIAN_POINT('',(-30.325,21.5631368321642,-235.35005));
#191881=CARTESIAN_POINT('Origin',(-30.325,21.5631368321642,-234.90005));
#191882=CARTESIAN_POINT('Origin',(-29.125,21.5631368321642,-234.90005));
#191883=CARTESIAN_POINT('Origin',(-29.125,21.5631368321642,-235.35005));
#191884=CARTESIAN_POINT('Origin',(-29.125,25.702658460412,-234.90005));
#191885=CARTESIAN_POINT('',(-30.325,25.702658460412,-235.35005));
#191886=CARTESIAN_POINT('',(-29.875,25.702658460412,-234.90005));
#191887=CARTESIAN_POINT('Origin',(-30.325,25.702658460412,-234.90005));
#191888=CARTESIAN_POINT('Origin',(-29.125,25.702658460412,-235.35005));
#191889=CARTESIAN_POINT('Origin',(-29.125,25.702658460412,-234.90005));
#191890=CARTESIAN_POINT('Origin',(-30.325,-25.4138432731711,-234.90005));
#191891=CARTESIAN_POINT('',(-30.325,25.702658460412,-235.35005));
#191892=CARTESIAN_POINT('',(-29.875,21.5631368321642,-234.90005));
#191893=CARTESIAN_POINT('Origin',(-11.3749999999999,29.8508988479304,-234.90005));
#191894=CARTESIAN_POINT('',(-11.4419952819386,31.0490272351235,-235.35005));
#191895=CARTESIAN_POINT('',(-10.1749999999999,29.8508988479304,-235.35005));
#191896=CARTESIAN_POINT('Origin',(-11.3749999999999,29.8508988479304,-235.35005));
#191897=CARTESIAN_POINT('',(-10.6249999999999,29.8508988479304,-234.90005));
#191898=CARTESIAN_POINT('Origin',(-10.1749999999999,29.8508988479304,-234.90005));
#191899=CARTESIAN_POINT('',(-11.4168720512116,30.5997290899261,-234.90005));
#191900=CARTESIAN_POINT('Origin',(-11.3749999999999,29.8508988479304,-234.90005));
#191901=CARTESIAN_POINT('Origin',(-11.4419952819386,31.0490272351235,-234.90005));
#191902=CARTESIAN_POINT('Origin',(-10.1749999999999,-25.4138432731711,-234.90005));
#191903=CARTESIAN_POINT('',(-10.6249999999999,21.5631368321642,-234.90005));
#191904=CARTESIAN_POINT('',(-10.1749999999999,21.5631368321642,-235.35005));
#191905=CARTESIAN_POINT('Origin',(-10.1749999999999,21.5631368321642,-234.90005));
#191906=CARTESIAN_POINT('',(-10.6249999999999,29.8508988479304,-234.90005));
#191907=CARTESIAN_POINT('',(-10.1749999999999,21.5631368321642,-235.35005));
#191908=CARTESIAN_POINT('Origin',(2.61456814389029E-14,-173.57701443073,
-234.90005));
#191909=CARTESIAN_POINT('',(-19.1119042071944,30.4756045219376,-235.35005));
#191910=CARTESIAN_POINT('',(-19.0699401294965,30.0275654430807,-234.90005));
#191911=CARTESIAN_POINT('Origin',(-19.1119042071944,30.4756045219376,-234.90005));
#191912=CARTESIAN_POINT('Origin',(2.61456814389029E-14,-173.57701443073,
-235.35005));
#191913=CARTESIAN_POINT('Origin',(2.61456814389029E-14,-173.57701443073,
-234.90005));
#191914=CARTESIAN_POINT('Origin',(-11.3749999999999,21.5631368321642,-234.90005));
#191915=CARTESIAN_POINT('',(-11.3749999999999,20.8131368321642,-234.90005));
#191916=CARTESIAN_POINT('',(-11.3749999999999,20.3631368321642,-235.35005));
#191917=CARTESIAN_POINT('Origin',(-11.3749999999999,20.3631368321642,-234.90005));
#191918=CARTESIAN_POINT('Origin',(-11.3749999999999,21.5631368321642,-234.90005));
#191919=CARTESIAN_POINT('Origin',(-11.3749999999999,21.5631368321642,-235.35005));
#191920=CARTESIAN_POINT('Origin',(-19.,29.2808336449858,-234.90005));
#191921=CARTESIAN_POINT('',(-20.2,29.2808336449858,-235.35005));
#191922=CARTESIAN_POINT('',(-19.75,29.2808336449858,-234.90005));
#191923=CARTESIAN_POINT('Origin',(-20.2,29.2808336449858,-234.90005));
#191924=CARTESIAN_POINT('Origin',(-19.,29.2808336449858,-235.35005));
#191925=CARTESIAN_POINT('Origin',(-19.,29.2808336449858,-234.90005));
#191926=CARTESIAN_POINT('Origin',(296.501483394397,20.3631368321642,-234.90005));
#191927=CARTESIAN_POINT('',(-19.,20.8131368321642,-234.90005));
#191928=CARTESIAN_POINT('',(-19.,20.3631368321642,-235.35005));
#191929=CARTESIAN_POINT('Origin',(-19.,20.3631368321642,-234.90005));
#191930=CARTESIAN_POINT('',(1.23757166668304E-15,20.8131368321642,-234.90005));
#191931=CARTESIAN_POINT('',(296.501483394397,20.3631368321642,-235.35005));
#191932=CARTESIAN_POINT('Origin',(-20.2,-25.4138432731711,-234.90005));
#191933=CARTESIAN_POINT('',(-20.2,21.5631368321642,-235.35005));
#191934=CARTESIAN_POINT('',(-19.75,21.5631368321642,-234.90005));
#191935=CARTESIAN_POINT('Origin',(-20.2,21.5631368321642,-234.90005));
#191936=CARTESIAN_POINT('',(-20.2,29.2808336449858,-235.35005));
#191937=CARTESIAN_POINT('',(-19.75,21.5631368321642,-234.90005));
#191938=CARTESIAN_POINT('Origin',(-19.,21.5631368321642,-234.90005));
#191939=CARTESIAN_POINT('Origin',(-19.,21.5631368321642,-235.35005));
#191940=CARTESIAN_POINT('Origin',(-19.,21.5631368321642,-234.90005));
#191941=CARTESIAN_POINT('Origin',(-1.25,30.1648419118246,-234.90005));
#191942=CARTESIAN_POINT('',(-1.25736211889437,31.3648193279477,-235.35005));
#191943=CARTESIAN_POINT('',(-0.0499999999999979,30.1648419118246,-235.35005));
#191944=CARTESIAN_POINT('Origin',(-1.25,30.1648419118246,-235.35005));
#191945=CARTESIAN_POINT('',(-0.5,30.1648419118246,-234.90005));
#191946=CARTESIAN_POINT('Origin',(-0.05,30.1648419118246,-234.90005));
#191947=CARTESIAN_POINT('',(-1.25460132430898,30.9148277969016,-234.90005));
#191948=CARTESIAN_POINT('Origin',(-1.25,30.1648419118246,-234.90005));
#191949=CARTESIAN_POINT('Origin',(-1.25736211889437,31.3648193279477,-234.90005));
#191950=CARTESIAN_POINT('Origin',(-0.0499999999999945,-25.4138432731711,
-234.90005));
#191951=CARTESIAN_POINT('',(-0.5,21.5631368321642,-234.90005));
#191952=CARTESIAN_POINT('',(-0.0499999999999974,21.5631368321642,-235.35005));
#191953=CARTESIAN_POINT('Origin',(-0.05,21.5631368321642,-234.90005));
#191954=CARTESIAN_POINT('',(-0.5,30.1648419118246,-234.90005));
#191955=CARTESIAN_POINT('',(-0.0499999999999974,21.5631368321642,-235.35005));
#191956=CARTESIAN_POINT('Origin',(2.61456814389029E-14,-173.57701443073,
-234.90005));
#191957=CARTESIAN_POINT('',(-8.9272710441499,31.1741516601419,-235.35005));
#191958=CARTESIAN_POINT('',(-8.90766940259363,30.7245787787886,-234.90005));
#191959=CARTESIAN_POINT('Origin',(-8.9272710441499,31.1741516601419,-234.90005));
#191960=CARTESIAN_POINT('Origin',(2.61456814389029E-14,-173.57701443073,
-235.35005));
#191961=CARTESIAN_POINT('Origin',(2.61456814389029E-14,-173.57701443073,
-234.90005));
#191962=CARTESIAN_POINT('Origin',(-1.25,21.5631368321642,-234.90005));
#191963=CARTESIAN_POINT('',(-1.25,20.8131368321642,-234.90005));
#191964=CARTESIAN_POINT('',(-1.25,20.3631368321642,-235.35005));
#191965=CARTESIAN_POINT('Origin',(-1.25,20.3631368321642,-234.90005));
#191966=CARTESIAN_POINT('Origin',(-1.25,21.5631368321642,-234.90005));
#191967=CARTESIAN_POINT('Origin',(-1.25,21.5631368321642,-235.35005));
#191968=CARTESIAN_POINT('Origin',(-8.87499999999986,29.9752906431998,-234.90005));
#191969=CARTESIAN_POINT('',(-10.075,29.9752906431998,-235.35005));
#191970=CARTESIAN_POINT('',(-9.62499999999986,29.9752906431998,-234.90005));
#191971=CARTESIAN_POINT('Origin',(-10.075,29.9752906431998,-234.90005));
#191972=CARTESIAN_POINT('Origin',(-8.87499999999986,29.9752906431998,-235.35005));
#191973=CARTESIAN_POINT('Origin',(-8.87499999999986,29.9752906431998,-234.90005));
#191974=CARTESIAN_POINT('Origin',(296.501483394397,20.3631368321642,-234.90005));
#191975=CARTESIAN_POINT('',(-8.87499999999986,20.8131368321642,-234.90005));
#191976=CARTESIAN_POINT('',(-8.87499999999986,20.3631368321642,-235.35005));
#191977=CARTESIAN_POINT('Origin',(-8.87499999999986,20.3631368321642,-234.90005));
#191978=CARTESIAN_POINT('',(1.23757166668304E-15,20.8131368321642,-234.90005));
#191979=CARTESIAN_POINT('',(296.501483394397,20.3631368321642,-235.35005));
#191980=CARTESIAN_POINT('Origin',(-10.075,-25.4138432731712,-234.90005));
#191981=CARTESIAN_POINT('',(-10.0749999999999,21.5631368321642,-235.35005));
#191982=CARTESIAN_POINT('',(-9.62499999999986,21.5631368321642,-234.90005));
#191983=CARTESIAN_POINT('Origin',(-10.0749999999999,21.5631368321642,-234.90005));
#191984=CARTESIAN_POINT('',(-10.075,29.9752906431998,-235.35005));
#191985=CARTESIAN_POINT('',(-9.62499999999986,21.5631368321642,-234.90005));
#191986=CARTESIAN_POINT('Origin',(-8.87499999999986,21.5631368321642,-234.90005));
#191987=CARTESIAN_POINT('Origin',(-8.87499999999986,21.5631368321642,-235.35005));
#191988=CARTESIAN_POINT('Origin',(-8.87499999999986,21.5631368321642,-234.90005));
#191989=CARTESIAN_POINT('Origin',(-1.25,19.0631368321642,-234.90005));
#191990=CARTESIAN_POINT('',(-1.25,20.2631368321642,-235.35005));
#191991=CARTESIAN_POINT('',(-1.25,19.8131368321642,-234.90005));
#191992=CARTESIAN_POINT('Origin',(-1.25,20.2631368321642,-234.90005));
#191993=CARTESIAN_POINT('',(-0.0499999999999972,19.0631368321642,-235.35005));
#191994=CARTESIAN_POINT('Origin',(-1.25,19.0631368321642,-235.35005));
#191995=CARTESIAN_POINT('',(-0.5,19.0631368321642,-234.90005));
#191996=CARTESIAN_POINT('Origin',(-0.0499999999999994,19.0631368321642,
-234.90005));
#191997=CARTESIAN_POINT('Origin',(-1.25,19.0631368321642,-234.90005));
#191998=CARTESIAN_POINT('Origin',(-0.0499999999999945,-25.4138432731711,
-234.90005));
#191999=CARTESIAN_POINT('',(-0.5,10.9575972794973,-234.90005));
#192000=CARTESIAN_POINT('',(-0.0499999999999967,10.9575972794973,-235.35005));
#192001=CARTESIAN_POINT('Origin',(-0.0499999999999989,10.9575972794973,
-234.90005));
#192002=CARTESIAN_POINT('',(-0.5,19.0631368321642,-234.90005));
#192003=CARTESIAN_POINT('',(-0.0499999999999967,10.9575972794973,-235.35005));
#192004=CARTESIAN_POINT('Origin',(296.501483394397,20.2631368321643,-234.90005));
#192005=CARTESIAN_POINT('',(-8.87499999999986,20.2631368321642,-235.35005));
#192006=CARTESIAN_POINT('',(-8.87499999999986,19.8131368321642,-234.90005));
#192007=CARTESIAN_POINT('Origin',(-8.87499999999986,20.2631368321642,-234.90005));
#192008=CARTESIAN_POINT('',(296.501483394397,20.2631368321643,-235.35005));
#192009=CARTESIAN_POINT('',(1.54373336646988E-15,19.8131368321642,-234.90005));
#192010=CARTESIAN_POINT('Origin',(-1.25,10.9575972794973,-234.90005));
#192011=CARTESIAN_POINT('',(-1.25,10.2075972794973,-234.90005));
#192012=CARTESIAN_POINT('',(-1.25,9.75759727949733,-235.35005));
#192013=CARTESIAN_POINT('Origin',(-1.25,9.75759727949733,-234.90005));
#192014=CARTESIAN_POINT('Origin',(-1.25,10.9575972794973,-234.90005));
#192015=CARTESIAN_POINT('Origin',(-1.25,10.9575972794973,-235.35005));
#192016=CARTESIAN_POINT('Origin',(-8.87499999999986,19.0631368321642,-234.90005));
#192017=CARTESIAN_POINT('',(-10.075,19.0631368321642,-235.35005));
#192018=CARTESIAN_POINT('',(-9.62499999999986,19.0631368321642,-234.90005));
#192019=CARTESIAN_POINT('Origin',(-10.075,19.0631368321642,-234.90005));
#192020=CARTESIAN_POINT('Origin',(-8.87499999999986,19.0631368321642,-235.35005));
#192021=CARTESIAN_POINT('Origin',(-8.87499999999986,19.0631368321642,-234.90005));
#192022=CARTESIAN_POINT('Origin',(296.501483394397,9.75759727949737,-234.90005));
#192023=CARTESIAN_POINT('',(-8.87499999999986,10.2075972794973,-234.90005));
#192024=CARTESIAN_POINT('',(-8.87499999999986,9.75759727949733,-235.35005));
#192025=CARTESIAN_POINT('Origin',(-8.87499999999986,9.75759727949733,-234.90005));
#192026=CARTESIAN_POINT('',(2.53637567332344E-15,10.2075972794973,-234.90005));
#192027=CARTESIAN_POINT('',(296.501483394397,9.75759727949736,-235.35005));
#192028=CARTESIAN_POINT('Origin',(-10.075,-25.4138432731712,-234.90005));
#192029=CARTESIAN_POINT('',(-10.0749999999998,10.9575972794973,-235.35005));
#192030=CARTESIAN_POINT('',(-9.62499999999986,10.9575972794973,-234.90005));
#192031=CARTESIAN_POINT('Origin',(-10.0749999999998,10.9575972794973,-234.90005));
#192032=CARTESIAN_POINT('',(-10.075,19.0631368321642,-235.35005));
#192033=CARTESIAN_POINT('',(-9.62499999999986,10.9575972794973,-234.90005));
#192034=CARTESIAN_POINT('Origin',(-8.87499999999986,10.9575972794973,-234.90005));
#192035=CARTESIAN_POINT('Origin',(-8.87499999999986,10.9575972794973,-235.35005));
#192036=CARTESIAN_POINT('Origin',(-8.87499999999986,10.9575972794973,-234.90005));
#192037=CARTESIAN_POINT('Origin',(-1.25,8.45759727949731,-234.90005));
#192038=CARTESIAN_POINT('',(-1.25,9.65759727949731,-235.35005));
#192039=CARTESIAN_POINT('',(-1.25,9.20759727949731,-234.90005));
#192040=CARTESIAN_POINT('Origin',(-1.25,9.65759727949731,-234.90005));
#192041=CARTESIAN_POINT('',(-0.0499999999999966,8.45759727949731,-235.35005));
#192042=CARTESIAN_POINT('Origin',(-1.25,8.45759727949731,-235.35005));
#192043=CARTESIAN_POINT('',(-0.5,8.45759727949731,-234.90005));
#192044=CARTESIAN_POINT('Origin',(-0.0499999999999987,8.45759727949731,
-234.90005));
#192045=CARTESIAN_POINT('Origin',(-1.25,8.45759727949731,-234.90005));
#192046=CARTESIAN_POINT('Origin',(-0.0499999999999945,-25.4138432731711,
-234.90005));
#192047=CARTESIAN_POINT('',(-0.5,2.29555713691451,-234.90005));
#192048=CARTESIAN_POINT('',(-0.0499999999999962,2.29555713691451,-235.35005));
#192049=CARTESIAN_POINT('Origin',(-0.0499999999999985,2.29555713691451,
-234.90005));
#192050=CARTESIAN_POINT('',(-0.5,8.45759727949731,-234.90005));
#192051=CARTESIAN_POINT('',(-0.0499999999999962,2.29555713691451,-235.35005));
#192052=CARTESIAN_POINT('Origin',(296.501483394397,9.65759727949727,-234.90005));
#192053=CARTESIAN_POINT('',(-8.87499999999986,9.65759727949731,-235.35005));
#192054=CARTESIAN_POINT('',(-8.87499999999986,9.20759727949731,-234.90005));
#192055=CARTESIAN_POINT('Origin',(-8.87499999999986,9.65759727949731,-234.90005));
#192056=CARTESIAN_POINT('',(296.501483394397,9.65759727949727,-235.35005));
#192057=CARTESIAN_POINT('',(2.8425373731103E-15,9.20759727949731,-234.90005));
#192058=CARTESIAN_POINT('Origin',(-1.25,2.29555713691451,-234.90005));
#192059=CARTESIAN_POINT('',(-1.18233753211584,1.54861551239502,-234.90005));
#192060=CARTESIAN_POINT('',(-1.14174005138535,1.10045053768332,-235.35005));
#192061=CARTESIAN_POINT('Origin',(-1.14174005138535,1.10045053768332,-234.90005));
#192062=CARTESIAN_POINT('Origin',(-1.25,2.29555713691451,-234.90005));
#192063=CARTESIAN_POINT('Origin',(-1.25,2.29555713691451,-235.35005));
#192064=CARTESIAN_POINT('Origin',(-8.87499999999986,8.45759727949731,-234.90005));
#192065=CARTESIAN_POINT('',(-10.075,8.45759727949731,-235.35005));
#192066=CARTESIAN_POINT('',(-9.62499999999986,8.45759727949731,-234.90005));
#192067=CARTESIAN_POINT('Origin',(-10.075,8.45759727949731,-234.90005));
#192068=CARTESIAN_POINT('Origin',(-8.87499999999986,8.45759727949731,-235.35005));
#192069=CARTESIAN_POINT('Origin',(-8.87499999999986,8.45759727949731,-234.90005));
#192070=CARTESIAN_POINT('Origin',(0.,-11.5034818258363,-234.90005));
#192071=CARTESIAN_POINT('',(-5.33358654455957,0.46765101689032,-234.90005));
#192072=CARTESIAN_POINT('',(-5.1504491822704,0.0566027149430096,-235.35005));
#192073=CARTESIAN_POINT('Origin',(-5.1504491822704,0.0566027149430111,-234.90005));
#192074=CARTESIAN_POINT('Origin',(0.,-11.5034818258363,-234.90005));
#192075=CARTESIAN_POINT('Origin',(0.,-11.5034818258363,-235.35005));
#192076=CARTESIAN_POINT('Origin',(-10.075,-25.4138432731712,-234.90005));
#192077=CARTESIAN_POINT('',(-10.0749999999998,0.367156910880383,-235.35005));
#192078=CARTESIAN_POINT('',(-9.62499999999985,0.367156910880383,-234.90005));
#192079=CARTESIAN_POINT('Origin',(-10.0749999999998,0.367156910880383,-234.90005));
#192080=CARTESIAN_POINT('',(-10.075,8.45759727949732,-235.35005));
#192081=CARTESIAN_POINT('',(-9.62499999999985,0.367156910880385,-234.90005));
#192082=CARTESIAN_POINT('Origin',(-9.40330570654115,9.60205772683049,-234.90005));
#192083=CARTESIAN_POINT('',(-8.83216440217218,-0.38161883095341,-234.90005));
#192084=CARTESIAN_POINT('',(-8.80646304347558,-0.830884276053686,-235.35005));
#192085=CARTESIAN_POINT('Origin',(-8.80646304347558,-0.830884276053684,
-234.90005));
#192086=CARTESIAN_POINT('Origin',(-9.40330570654115,9.60205772683049,-234.90005));
#192087=CARTESIAN_POINT('Origin',(-9.40330570654115,9.60205772683049,-235.35005));
#192088=CARTESIAN_POINT('Origin',(-8.87499999999985,0.367156910880384,-234.90005));
#192089=CARTESIAN_POINT('Origin',(-8.87499999999985,0.367156910880384,-234.90005));
#192090=CARTESIAN_POINT('Origin',(-8.87499999999985,0.367156910880384,-235.35005));
#192091=CARTESIAN_POINT('Origin',(-11.3749999999999,8.45759727949731,-234.90005));
#192092=CARTESIAN_POINT('',(-11.3749999999999,9.65759727949731,-235.35005));
#192093=CARTESIAN_POINT('',(-11.3749999999999,9.20759727949731,-234.90005));
#192094=CARTESIAN_POINT('Origin',(-11.3749999999999,9.65759727949731,-234.90005));
#192095=CARTESIAN_POINT('',(-10.1749999999999,8.45759727949731,-235.35005));
#192096=CARTESIAN_POINT('Origin',(-11.3749999999999,8.45759727949731,-235.35005));
#192097=CARTESIAN_POINT('',(-10.6249999999999,8.45759727949731,-234.90005));
#192098=CARTESIAN_POINT('Origin',(-10.1749999999999,8.45759727949731,-234.90005));
#192099=CARTESIAN_POINT('Origin',(-11.3749999999999,8.45759727949731,-234.90005));
#192100=CARTESIAN_POINT('Origin',(-10.1749999999999,-25.4138432731711,-234.90005));
#192101=CARTESIAN_POINT('',(-10.6249999999999,0.352057726830487,-234.90005));
#192102=CARTESIAN_POINT('',(-10.1749999999999,0.352057726830488,-235.35005));
#192103=CARTESIAN_POINT('Origin',(-10.1749999999999,0.352057726830487,-234.90005));
#192104=CARTESIAN_POINT('',(-10.6249999999999,8.45759727949731,-234.90005));
#192105=CARTESIAN_POINT('',(-10.1749999999999,0.352057726830487,-235.35005));
#192106=CARTESIAN_POINT('Origin',(296.501483394397,9.65759727949727,-234.90005));
#192107=CARTESIAN_POINT('',(-19.,9.65759727949731,-235.35005));
#192108=CARTESIAN_POINT('',(-19.,9.20759727949731,-234.90005));
#192109=CARTESIAN_POINT('Origin',(-19.,9.65759727949731,-234.90005));
#192110=CARTESIAN_POINT('',(296.501483394397,9.65759727949727,-235.35005));
#192111=CARTESIAN_POINT('',(2.8425373731103E-15,9.20759727949731,-234.90005));
#192112=CARTESIAN_POINT('Origin',(-11.3749999999999,0.352057726830487,-234.90005));
#192113=CARTESIAN_POINT('',(-11.3749999999999,-0.397942273169513,-234.90005));
#192114=CARTESIAN_POINT('',(-11.3749999999999,-0.847942273169513,-235.35005));
#192115=CARTESIAN_POINT('Origin',(-11.3749999999999,-0.847942273169513,
-234.90005));
#192116=CARTESIAN_POINT('Origin',(-11.3749999999999,0.352057726830487,-234.90005));
#192117=CARTESIAN_POINT('Origin',(-11.3749999999999,0.352057726830487,-235.35005));
#192118=CARTESIAN_POINT('Origin',(-19.,8.45759727949731,-234.90005));
#192119=CARTESIAN_POINT('',(-20.2,8.45759727949731,-235.35005));
#192120=CARTESIAN_POINT('',(-19.75,8.45759727949731,-234.90005));
#192121=CARTESIAN_POINT('Origin',(-20.2,8.45759727949731,-234.90005));
#192122=CARTESIAN_POINT('Origin',(-19.,8.45759727949731,-235.35005));
#192123=CARTESIAN_POINT('Origin',(-19.,8.45759727949731,-234.90005));
#192124=CARTESIAN_POINT('Origin',(296.501483394397,-0.84794227316963,-234.90005));
#192125=CARTESIAN_POINT('',(-19.,-0.39794227316951,-234.90005));
#192126=CARTESIAN_POINT('',(-19.,-0.847942273169513,-235.35005));
#192127=CARTESIAN_POINT('Origin',(-19.,-0.84794227316951,-234.90005));
#192128=CARTESIAN_POINT('',(1.11087130309497E-13,-0.397942273169517,-234.90005));
#192129=CARTESIAN_POINT('',(296.501483394397,-0.84794227316963,-235.35005));
#192130=CARTESIAN_POINT('Origin',(-20.2,-25.4138432731711,-234.90005));
#192131=CARTESIAN_POINT('',(-20.2,0.352057726830487,-235.35005));
#192132=CARTESIAN_POINT('',(-19.75,0.352057726830487,-234.90005));
#192133=CARTESIAN_POINT('Origin',(-20.2,0.352057726830487,-234.90005));
#192134=CARTESIAN_POINT('',(-20.2,8.45759727949731,-235.35005));
#192135=CARTESIAN_POINT('',(-19.75,0.352057726830487,-234.90005));
#192136=CARTESIAN_POINT('Origin',(-19.,0.35205772683049,-234.90005));
#192137=CARTESIAN_POINT('Origin',(-19.,0.35205772683049,-235.35005));
#192138=CARTESIAN_POINT('Origin',(-19.,0.35205772683049,-234.90005));
#192139=CARTESIAN_POINT('Origin',(-11.3749999999999,19.0631368321642,-234.90005));
#192140=CARTESIAN_POINT('',(-11.3749999999999,20.2631368321642,-235.35005));
#192141=CARTESIAN_POINT('',(-11.3749999999999,19.8131368321642,-234.90005));
#192142=CARTESIAN_POINT('Origin',(-11.3749999999999,20.2631368321642,-234.90005));
#192143=CARTESIAN_POINT('',(-10.1749999999999,19.0631368321642,-235.35005));
#192144=CARTESIAN_POINT('Origin',(-11.3749999999999,19.0631368321642,-235.35005));
#192145=CARTESIAN_POINT('',(-10.6249999999999,19.0631368321642,-234.90005));
#192146=CARTESIAN_POINT('Origin',(-10.1749999999999,19.0631368321642,-234.90005));
#192147=CARTESIAN_POINT('Origin',(-11.3749999999999,19.0631368321642,-234.90005));
#192148=CARTESIAN_POINT('Origin',(-10.1749999999999,-25.4138432731711,-234.90005));
#192149=CARTESIAN_POINT('',(-10.6249999999999,10.9575972794973,-234.90005));
#192150=CARTESIAN_POINT('',(-10.1749999999999,10.9575972794973,-235.35005));
#192151=CARTESIAN_POINT('Origin',(-10.1749999999999,10.9575972794973,-234.90005));
#192152=CARTESIAN_POINT('',(-10.6249999999999,19.0631368321642,-234.90005));
#192153=CARTESIAN_POINT('',(-10.1749999999999,10.9575972794973,-235.35005));
#192154=CARTESIAN_POINT('Origin',(296.501483394397,20.2631368321643,-234.90005));
#192155=CARTESIAN_POINT('',(-19.,20.2631368321642,-235.35005));
#192156=CARTESIAN_POINT('',(-19.,19.8131368321642,-234.90005));
#192157=CARTESIAN_POINT('Origin',(-19.,20.2631368321642,-234.90005));
#192158=CARTESIAN_POINT('',(296.501483394397,20.2631368321643,-235.35005));
#192159=CARTESIAN_POINT('',(1.54373336646988E-15,19.8131368321642,-234.90005));
#192160=CARTESIAN_POINT('Origin',(-11.3749999999999,10.9575972794973,-234.90005));
#192161=CARTESIAN_POINT('',(-11.3749999999999,10.2075972794973,-234.90005));
#192162=CARTESIAN_POINT('',(-11.3749999999999,9.75759727949733,-235.35005));
#192163=CARTESIAN_POINT('Origin',(-11.3749999999999,9.75759727949733,-234.90005));
#192164=CARTESIAN_POINT('Origin',(-11.3749999999999,10.9575972794973,-234.90005));
#192165=CARTESIAN_POINT('Origin',(-11.3749999999999,10.9575972794973,-235.35005));
#192166=CARTESIAN_POINT('Origin',(-19.,19.0631368321642,-234.90005));
#192167=CARTESIAN_POINT('',(-20.2,19.0631368321642,-235.35005));
#192168=CARTESIAN_POINT('',(-19.75,19.0631368321642,-234.90005));
#192169=CARTESIAN_POINT('Origin',(-20.2,19.0631368321642,-234.90005));
#192170=CARTESIAN_POINT('Origin',(-19.,19.0631368321642,-235.35005));
#192171=CARTESIAN_POINT('Origin',(-19.,19.0631368321642,-234.90005));
#192172=CARTESIAN_POINT('Origin',(296.501483394397,9.75759727949737,-234.90005));
#192173=CARTESIAN_POINT('',(-19.,10.2075972794973,-234.90005));
#192174=CARTESIAN_POINT('',(-19.,9.75759727949733,-235.35005));
#192175=CARTESIAN_POINT('Origin',(-19.,9.75759727949733,-234.90005));
#192176=CARTESIAN_POINT('',(2.53637567332344E-15,10.2075972794973,-234.90005));
#192177=CARTESIAN_POINT('',(296.501483394397,9.75759727949737,-235.35005));
#192178=CARTESIAN_POINT('Origin',(-20.2,-25.4138432731711,-234.90005));
#192179=CARTESIAN_POINT('',(-20.2,10.9575972794973,-235.35005));
#192180=CARTESIAN_POINT('',(-19.75,10.9575972794973,-234.90005));
#192181=CARTESIAN_POINT('Origin',(-20.2,10.9575972794973,-234.90005));
#192182=CARTESIAN_POINT('',(-20.2,19.0631368321642,-235.35005));
#192183=CARTESIAN_POINT('',(-19.75,10.9575972794973,-234.90005));
#192184=CARTESIAN_POINT('Origin',(-19.,10.9575972794973,-234.90005));
#192185=CARTESIAN_POINT('Origin',(-19.,10.9575972794973,-235.35005));
#192186=CARTESIAN_POINT('Origin',(-19.,10.9575972794973,-234.90005));
#192187=CARTESIAN_POINT('Origin',(-21.5,19.0631368321642,-234.90005));
#192188=CARTESIAN_POINT('',(-21.5,20.2631368321642,-235.35005));
#192189=CARTESIAN_POINT('',(-21.5,19.8131368321642,-234.90005));
#192190=CARTESIAN_POINT('Origin',(-21.5,20.2631368321642,-234.90005));
#192191=CARTESIAN_POINT('',(-20.3,19.0631368321642,-235.35005));
#192192=CARTESIAN_POINT('Origin',(-21.5,19.0631368321642,-235.35005));
#192193=CARTESIAN_POINT('',(-20.75,19.0631368321642,-234.90005));
#192194=CARTESIAN_POINT('Origin',(-20.3,19.0631368321642,-234.90005));
#192195=CARTESIAN_POINT('Origin',(-21.5,19.0631368321642,-234.90005));
#192196=CARTESIAN_POINT('Origin',(-20.3,-25.4138432731711,-234.90005));
#192197=CARTESIAN_POINT('',(-20.75,10.9575972794973,-234.90005));
#192198=CARTESIAN_POINT('',(-20.3,10.9575972794973,-235.35005));
#192199=CARTESIAN_POINT('Origin',(-20.3,10.9575972794973,-234.90005));
#192200=CARTESIAN_POINT('',(-20.75,19.0631368321642,-234.90005));
#192201=CARTESIAN_POINT('',(-20.3,10.9575972794973,-235.35005));
#192202=CARTESIAN_POINT('Origin',(296.501483394397,20.2631368321643,-234.90005));
#192203=CARTESIAN_POINT('',(-29.125,20.2631368321642,-235.35005));
#192204=CARTESIAN_POINT('',(-29.125,19.8131368321642,-234.90005));
#192205=CARTESIAN_POINT('Origin',(-29.125,20.2631368321642,-234.90005));
#192206=CARTESIAN_POINT('',(296.501483394397,20.2631368321643,-235.35005));
#192207=CARTESIAN_POINT('',(1.54373336646988E-15,19.8131368321642,-234.90005));
#192208=CARTESIAN_POINT('Origin',(-21.5,10.9575972794973,-234.90005));
#192209=CARTESIAN_POINT('',(-21.5,10.2075972794973,-234.90005));
#192210=CARTESIAN_POINT('',(-21.5,9.75759727949733,-235.35005));
#192211=CARTESIAN_POINT('Origin',(-21.5,9.75759727949733,-234.90005));
#192212=CARTESIAN_POINT('Origin',(-21.5,10.9575972794973,-234.90005));
#192213=CARTESIAN_POINT('Origin',(-21.5,10.9575972794973,-235.35005));
#192214=CARTESIAN_POINT('Origin',(-29.125,19.0631368321642,-234.90005));
#192215=CARTESIAN_POINT('',(-30.325,19.0631368321642,-235.35005));
#192216=CARTESIAN_POINT('',(-29.875,19.0631368321642,-234.90005));
#192217=CARTESIAN_POINT('Origin',(-30.325,19.0631368321642,-234.90005));
#192218=CARTESIAN_POINT('Origin',(-29.125,19.0631368321642,-235.35005));
#192219=CARTESIAN_POINT('Origin',(-29.125,19.0631368321642,-234.90005));
#192220=CARTESIAN_POINT('Origin',(296.501483394397,9.75759727949737,-234.90005));
#192221=CARTESIAN_POINT('',(-29.125,10.2075972794973,-234.90005));
#192222=CARTESIAN_POINT('',(-29.125,9.75759727949733,-235.35005));
#192223=CARTESIAN_POINT('Origin',(-29.125,9.75759727949733,-234.90005));
#192224=CARTESIAN_POINT('',(2.53637567332344E-15,10.2075972794973,-234.90005));
#192225=CARTESIAN_POINT('',(296.501483394397,9.75759727949737,-235.35005));
#192226=CARTESIAN_POINT('Origin',(-30.325,-25.4138432731711,-234.90005));
#192227=CARTESIAN_POINT('',(-30.325,10.9575972794973,-235.35005));
#192228=CARTESIAN_POINT('',(-29.875,10.9575972794973,-234.90005));
#192229=CARTESIAN_POINT('Origin',(-30.325,10.9575972794973,-234.90005));
#192230=CARTESIAN_POINT('',(-30.325,19.0631368321642,-235.35005));
#192231=CARTESIAN_POINT('',(-29.875,10.9575972794973,-234.90005));
#192232=CARTESIAN_POINT('Origin',(-29.125,10.9575972794973,-234.90005));
#192233=CARTESIAN_POINT('Origin',(-29.125,10.9575972794973,-235.35005));
#192234=CARTESIAN_POINT('Origin',(-29.125,10.9575972794973,-234.90005));
#192235=CARTESIAN_POINT('Origin',(-21.5,8.45759727949731,-234.90005));
#192236=CARTESIAN_POINT('',(-21.5,9.65759727949731,-235.35005));
#192237=CARTESIAN_POINT('',(-21.5,9.20759727949731,-234.90005));
#192238=CARTESIAN_POINT('Origin',(-21.5,9.65759727949731,-234.90005));
#192239=CARTESIAN_POINT('',(-20.3,8.45759727949731,-235.35005));
#192240=CARTESIAN_POINT('Origin',(-21.5,8.45759727949731,-235.35005));
#192241=CARTESIAN_POINT('',(-20.75,8.45759727949731,-234.90005));
#192242=CARTESIAN_POINT('Origin',(-20.3,8.45759727949731,-234.90005));
#192243=CARTESIAN_POINT('Origin',(-21.5,8.45759727949731,-234.90005));
#192244=CARTESIAN_POINT('Origin',(-20.3,-25.4138432731711,-234.90005));
#192245=CARTESIAN_POINT('',(-20.75,0.352057726830487,-234.90005));
#192246=CARTESIAN_POINT('',(-20.3,0.352057726830486,-235.35005));
#192247=CARTESIAN_POINT('Origin',(-20.3,0.352057726830486,-234.90005));
#192248=CARTESIAN_POINT('',(-20.75,8.45759727949731,-234.90005));
#192249=CARTESIAN_POINT('',(-20.3,0.352057726830487,-235.35005));
#192250=CARTESIAN_POINT('Origin',(296.501483394397,9.65759727949727,-234.90005));
#192251=CARTESIAN_POINT('',(-29.125,9.65759727949731,-235.35005));
#192252=CARTESIAN_POINT('',(-29.125,9.20759727949731,-234.90005));
#192253=CARTESIAN_POINT('Origin',(-29.125,9.65759727949731,-234.90005));
#192254=CARTESIAN_POINT('',(296.501483394397,9.65759727949727,-235.35005));
#192255=CARTESIAN_POINT('',(2.8425373731103E-15,9.20759727949731,-234.90005));
#192256=CARTESIAN_POINT('Origin',(-21.5,0.352057726830491,-234.90005));
#192257=CARTESIAN_POINT('',(-21.5,-0.397942273169509,-234.90005));
#192258=CARTESIAN_POINT('',(-21.5,-0.847942273169509,-235.35005));
#192259=CARTESIAN_POINT('Origin',(-21.5,-0.847942273169509,-234.90005));
#192260=CARTESIAN_POINT('Origin',(-21.5,0.352057726830491,-234.90005));
#192261=CARTESIAN_POINT('Origin',(-21.5,0.352057726830491,-235.35005));
#192262=CARTESIAN_POINT('Origin',(-29.125,8.45759727949731,-234.90005));
#192263=CARTESIAN_POINT('',(-30.325,8.45759727949731,-235.35005));
#192264=CARTESIAN_POINT('',(-29.875,8.45759727949731,-234.90005));
#192265=CARTESIAN_POINT('Origin',(-30.325,8.45759727949731,-234.90005));
#192266=CARTESIAN_POINT('Origin',(-29.125,8.45759727949731,-235.35005));
#192267=CARTESIAN_POINT('Origin',(-29.125,8.45759727949731,-234.90005));
#192268=CARTESIAN_POINT('Origin',(296.501483394397,-0.84794227316963,-234.90005));
#192269=CARTESIAN_POINT('',(-29.125,-0.397942273169507,-234.90005));
#192270=CARTESIAN_POINT('',(-29.125,-0.847942273169509,-235.35005));
#192271=CARTESIAN_POINT('Origin',(-29.125,-0.847942273169506,-234.90005));
#192272=CARTESIAN_POINT('',(1.11087130309497E-13,-0.397942273169517,-234.90005));
#192273=CARTESIAN_POINT('',(296.501483394397,-0.84794227316963,-235.35005));
#192274=CARTESIAN_POINT('Origin',(-30.325,-25.4138432731711,-234.90005));
#192275=CARTESIAN_POINT('',(-30.325,0.352057726830494,-235.35005));
#192276=CARTESIAN_POINT('',(-29.875,0.352057726830494,-234.90005));
#192277=CARTESIAN_POINT('Origin',(-30.325,0.352057726830494,-234.90005));
#192278=CARTESIAN_POINT('',(-30.325,8.45759727949732,-235.35005));
#192279=CARTESIAN_POINT('',(-29.875,0.352057726830494,-234.90005));
#192280=CARTESIAN_POINT('Origin',(-29.125,0.352057726830494,-234.90005));
#192281=CARTESIAN_POINT('Origin',(-29.125,0.352057726830494,-235.35005));
#192282=CARTESIAN_POINT('Origin',(-29.125,0.352057726830494,-234.90005));
#192283=CARTESIAN_POINT('Origin',(-31.625,8.45759727949731,-234.90005));
#192284=CARTESIAN_POINT('',(-31.625,9.65759727949731,-235.35005));
#192285=CARTESIAN_POINT('',(-31.625,9.20759727949731,-234.90005));
#192286=CARTESIAN_POINT('Origin',(-31.625,9.65759727949731,-234.90005));
#192287=CARTESIAN_POINT('',(-30.425,8.45759727949731,-235.35005));
#192288=CARTESIAN_POINT('Origin',(-31.625,8.45759727949731,-235.35005));
#192289=CARTESIAN_POINT('',(-30.875,8.45759727949731,-234.90005));
#192290=CARTESIAN_POINT('Origin',(-30.425,8.45759727949731,-234.90005));
#192291=CARTESIAN_POINT('Origin',(-31.625,8.45759727949731,-234.90005));
#192292=CARTESIAN_POINT('Origin',(-30.425,-25.4138432731711,-234.90005));
#192293=CARTESIAN_POINT('',(-30.875,0.352057726830494,-234.90005));
#192294=CARTESIAN_POINT('',(-30.425,0.352057726830494,-235.35005));
#192295=CARTESIAN_POINT('Origin',(-30.425,0.352057726830494,-234.90005));
#192296=CARTESIAN_POINT('',(-30.875,8.45759727949732,-234.90005));
#192297=CARTESIAN_POINT('',(-30.425,0.352057726830494,-235.35005));
#192298=CARTESIAN_POINT('Origin',(296.501483394397,9.65759727949727,-234.90005));
#192299=CARTESIAN_POINT('',(-39.4555265729267,9.65759727949731,-235.35005));
#192300=CARTESIAN_POINT('',(-39.4555265729267,9.20759727949731,-234.90005));
#192301=CARTESIAN_POINT('Origin',(-39.4555265729267,9.65759727949731,-234.90005));
#192302=CARTESIAN_POINT('',(296.501483394397,9.65759727949727,-235.35005));
#192303=CARTESIAN_POINT('',(2.8425373731103E-15,9.20759727949731,-234.90005));
#192304=CARTESIAN_POINT('Origin',(-31.625,0.352057726830494,-234.90005));
#192305=CARTESIAN_POINT('',(-31.625,-0.397942273169506,-234.90005));
#192306=CARTESIAN_POINT('',(-31.625,-0.847942273169506,-235.35005));
#192307=CARTESIAN_POINT('Origin',(-31.625,-0.847942273169505,-234.90005));
#192308=CARTESIAN_POINT('Origin',(-31.625,0.352057726830494,-234.90005));
#192309=CARTESIAN_POINT('Origin',(-31.625,0.352057726830495,-235.35005));
#192310=CARTESIAN_POINT('Origin',(-39.4555265729267,8.45759727949731,-234.90005));
#192311=CARTESIAN_POINT('',(-40.6550043680477,8.49299528808125,-235.35005));
#192312=CARTESIAN_POINT('',(-40.2052001948774,8.47972103486227,-234.90005));
#192313=CARTESIAN_POINT('Origin',(-40.6550043680477,8.49299528808125,-234.90005));
#192314=CARTESIAN_POINT('Origin',(-39.4555265729267,8.45759727949731,-235.35005));
#192315=CARTESIAN_POINT('Origin',(-39.4555265729267,8.45759727949731,-234.90005));
#192316=CARTESIAN_POINT('Origin',(296.501483394397,-0.84794227316963,-234.90005));
#192317=CARTESIAN_POINT('',(-39.6461373136998,-0.397942273169503,-234.90005));
#192318=CARTESIAN_POINT('',(-39.6461373136998,-0.847942273169505,-235.35005));
#192319=CARTESIAN_POINT('Origin',(-39.6461373136998,-0.847942273169502,
-234.90005));
#192320=CARTESIAN_POINT('',(1.11087130309497E-13,-0.397942273169517,-234.90005));
#192321=CARTESIAN_POINT('',(296.501483394397,-0.84794227316963,-235.35005));
#192322=CARTESIAN_POINT('Origin',(636.934816028482,-11.5034818258361,-234.90005));
#192323=CARTESIAN_POINT('',(-40.8459531286544,0.37308176509206,-235.35005));
#192324=CARTESIAN_POINT('',(-40.3960221980464,0.365197750743974,-234.90005));
#192325=CARTESIAN_POINT('Origin',(-40.8459531286544,0.37308176509206,-234.90005));
#192326=CARTESIAN_POINT('Origin',(636.934816028482,-11.5034818258361,-235.35005));
#192327=CARTESIAN_POINT('Origin',(636.934816028482,-11.5034818258361,-234.90005));
#192328=CARTESIAN_POINT('Origin',(-39.6461373136998,0.352057726830498,-234.90005));
#192329=CARTESIAN_POINT('Origin',(-39.6461373136998,0.352057726830498,-235.35005));
#192330=CARTESIAN_POINT('Origin',(-39.6461373136998,0.352057726830498,-234.90005));
#192331=CARTESIAN_POINT('Origin',(-31.625,19.0631368321642,-234.90005));
#192332=CARTESIAN_POINT('',(-31.625,20.2631368321642,-235.35005));
#192333=CARTESIAN_POINT('',(-31.625,19.8131368321642,-234.90005));
#192334=CARTESIAN_POINT('Origin',(-31.625,20.2631368321642,-234.90005));
#192335=CARTESIAN_POINT('',(-30.425,19.0631368321642,-235.35005));
#192336=CARTESIAN_POINT('Origin',(-31.625,19.0631368321642,-235.35005));
#192337=CARTESIAN_POINT('',(-30.875,19.0631368321642,-234.90005));
#192338=CARTESIAN_POINT('Origin',(-30.425,19.0631368321642,-234.90005));
#192339=CARTESIAN_POINT('Origin',(-31.625,19.0631368321642,-234.90005));
#192340=CARTESIAN_POINT('Origin',(-30.425,-25.4138432731711,-234.90005));
#192341=CARTESIAN_POINT('',(-30.875,10.9575972794973,-234.90005));
#192342=CARTESIAN_POINT('',(-30.425,10.9575972794973,-235.35005));
#192343=CARTESIAN_POINT('Origin',(-30.425,10.9575972794973,-234.90005));
#192344=CARTESIAN_POINT('',(-30.875,19.0631368321642,-234.90005));
#192345=CARTESIAN_POINT('',(-30.425,10.9575972794973,-235.35005));
#192346=CARTESIAN_POINT('Origin',(296.501483394397,20.2631368321643,-234.90005));
#192347=CARTESIAN_POINT('',(-36.0311576807679,20.2631368321642,-235.35005));
#192348=CARTESIAN_POINT('',(-36.0311576807679,19.8131368321642,-234.90005));
#192349=CARTESIAN_POINT('Origin',(-36.0311576807679,20.2631368321642,-234.90005));
#192350=CARTESIAN_POINT('',(296.501483394397,20.2631368321643,-235.35005));
#192351=CARTESIAN_POINT('',(1.54373336646988E-15,19.8131368321642,-234.90005));
#192352=CARTESIAN_POINT('Origin',(-31.625,10.9575972794973,-234.90005));
#192353=CARTESIAN_POINT('',(-31.625,10.2075972794973,-234.90005));
#192354=CARTESIAN_POINT('',(-31.625,9.75759727949733,-235.35005));
#192355=CARTESIAN_POINT('Origin',(-31.625,9.75759727949733,-234.90005));
#192356=CARTESIAN_POINT('Origin',(-31.625,10.9575972794973,-234.90005));
#192357=CARTESIAN_POINT('Origin',(-31.625,10.9575972794973,-235.35005));
#192358=CARTESIAN_POINT('Origin',(-36.0311576807679,19.0631368321642,-234.90005));
#192359=CARTESIAN_POINT('',(-36.9462347012319,19.8394319091927,-235.35005));
#192360=CARTESIAN_POINT('',(-36.6030808185579,19.548321255307,-234.90005));
#192361=CARTESIAN_POINT('Origin',(-36.9462347012319,19.8394319091927,-234.90005));
#192362=CARTESIAN_POINT('Origin',(-36.0311576807679,19.0631368321642,-235.35005));
#192363=CARTESIAN_POINT('Origin',(-36.0311576807679,19.0631368321642,-234.90005));
#192364=CARTESIAN_POINT('Origin',(296.501483394397,9.75759727949737,-234.90005));
#192365=CARTESIAN_POINT('',(-39.3771239584772,10.2075972794973,-234.90005));
#192366=CARTESIAN_POINT('',(-39.3771239584772,9.75759727949732,-235.35005));
#192367=CARTESIAN_POINT('Origin',(-39.3771239584772,9.75759727949733,-234.90005));
#192368=CARTESIAN_POINT('',(2.53637567332344E-15,10.2075972794973,-234.90005));
#192369=CARTESIAN_POINT('',(296.501483394397,9.75759727949737,-235.35005));
#192370=CARTESIAN_POINT('Origin',(6.29739814579425E-15,-11.5034818258363,
-234.90005));
#192371=CARTESIAN_POINT('',(-40.1936303108393,15.5496988085284,-235.35005));
#192372=CARTESIAN_POINT('',(-39.8203148590359,15.2984308769399,-234.90005));
#192373=CARTESIAN_POINT('Origin',(-40.1936303108393,15.5496988085284,-234.90005));
#192374=CARTESIAN_POINT('Origin',(6.29739814579425E-15,-11.5034818258363,
-235.35005));
#192375=CARTESIAN_POINT('Origin',(6.29739814579425E-15,-11.5034818258363,
-234.90005));
#192376=CARTESIAN_POINT('Origin',(-39.3771239584772,10.9575972794973,-234.90005));
#192377=CARTESIAN_POINT('',(-40.1267106833092,10.9824918965036,-234.90005));
#192378=CARTESIAN_POINT('',(-40.5764627182082,10.9974286667074,-235.35005));
#192379=CARTESIAN_POINT('Origin',(-40.5764627182083,10.9974286667074,-234.90005));
#192380=CARTESIAN_POINT('Origin',(-39.3771239584772,10.9575972794973,-234.90005));
#192381=CARTESIAN_POINT('Origin',(-39.3771239584772,10.9575972794973,-235.35005));
#192382=CARTESIAN_POINT('Origin',(-38.9907249661392,14.740057695632,-234.90005));
#192383=CARTESIAN_POINT('',(-40.4396332884467,14.7963131269086,-235.35005));
#192384=CARTESIAN_POINT('',(-39.989972084972,14.7788545447883,-234.90005));
#192385=CARTESIAN_POINT('Origin',(-40.4396332884467,14.7963131269086,-234.90005));
#192386=CARTESIAN_POINT('Origin',(-38.9907249661392,14.740057695632,-235.35005));
#192387=CARTESIAN_POINT('Origin',(-38.9907249661392,14.740057695632,-234.90005));
#192388=CARTESIAN_POINT('Origin',(636.934816028482,-11.5034818258361,-234.90005));
#192389=CARTESIAN_POINT('Origin',(636.934816028482,-11.5034818258361,-235.35005));
#192390=CARTESIAN_POINT('Origin',(636.934816028482,-11.5034818258361,-234.90005));
#192391=CARTESIAN_POINT('Origin',(-31.625,-2.14794227316952,-234.90005));
#192392=CARTESIAN_POINT('',(-31.625,-0.947942273169512,-235.35005));
#192393=CARTESIAN_POINT('',(-31.625,-1.39794227316951,-234.90005));
#192394=CARTESIAN_POINT('Origin',(-31.625,-0.947942273169512,-234.90005));
#192395=CARTESIAN_POINT('',(-30.425,-2.14794227316951,-235.35005));
#192396=CARTESIAN_POINT('Origin',(-31.625,-2.14794227316952,-235.35005));
#192397=CARTESIAN_POINT('',(-30.875,-2.14794227316951,-234.90005));
#192398=CARTESIAN_POINT('Origin',(-30.425,-2.14794227316951,-234.90005));
#192399=CARTESIAN_POINT('Origin',(-31.625,-2.14794227316952,-234.90005));
#192400=CARTESIAN_POINT('Origin',(-30.425,-25.4138432731711,-234.90005));
#192401=CARTESIAN_POINT('',(-30.875,-10.2534818258363,-234.90005));
#192402=CARTESIAN_POINT('',(-30.425,-10.2534818258363,-235.35005));
#192403=CARTESIAN_POINT('Origin',(-30.425,-10.2534818258363,-234.90005));
#192404=CARTESIAN_POINT('',(-30.875,-2.14794227316951,-234.90005));
#192405=CARTESIAN_POINT('',(-30.425,-10.2534818258363,-235.35005));
#192406=CARTESIAN_POINT('Origin',(296.501483394397,-0.94794227316939,-234.90005));
#192407=CARTESIAN_POINT('',(-39.6853241707135,-0.947942273169515,-235.35005));
#192408=CARTESIAN_POINT('',(-39.6853241707135,-1.39794227316951,-234.90005));
#192409=CARTESIAN_POINT('Origin',(-39.6853241707135,-0.947942273169515,
-234.90005));
#192410=CARTESIAN_POINT('',(296.501483394397,-0.94794227316939,-235.35005));
#192411=CARTESIAN_POINT('',(1.11087130309497E-13,-1.3979422731695,-234.90005));
#192412=CARTESIAN_POINT('Origin',(-31.625,-10.2534818258363,-234.90005));
#192413=CARTESIAN_POINT('',(-31.625,-11.0034818258363,-234.90005));
#192414=CARTESIAN_POINT('',(-31.625,-11.4534818258363,-235.35005));
#192415=CARTESIAN_POINT('Origin',(-31.625,-11.4534818258363,-234.90005));
#192416=CARTESIAN_POINT('Origin',(-31.625,-10.2534818258363,-234.90005));
#192417=CARTESIAN_POINT('Origin',(-31.625,-10.2534818258363,-235.35005));
#192418=CARTESIAN_POINT('Origin',(-39.6853241707135,-2.14794227316952,-234.90005));
#192419=CARTESIAN_POINT('',(-40.8852094777378,-2.13135161353407,-235.35005));
#192420=CARTESIAN_POINT('',(-40.4352524876037,-2.13757311089736,-234.90005));
#192421=CARTESIAN_POINT('Origin',(-40.8852094777378,-2.13135161353407,-234.90005));
#192422=CARTESIAN_POINT('Origin',(-39.6853241707135,-2.14794227316952,-235.35005));
#192423=CARTESIAN_POINT('Origin',(-39.6853241707135,-2.14794227316952,-234.90005));
#192424=CARTESIAN_POINT('Origin',(296.501483394397,-11.4534818258365,-234.90005));
#192425=CARTESIAN_POINT('',(-39.7488454733312,-11.0034818258363,-234.90005));
#192426=CARTESIAN_POINT('',(-39.7488454733312,-11.4534818258363,-235.35005));
#192427=CARTESIAN_POINT('Origin',(-39.7488454733312,-11.4534818258363,-234.90005));
#192428=CARTESIAN_POINT('',(2.22174260618994E-13,-11.0034818258363,-234.90005));
#192429=CARTESIAN_POINT('',(296.501483394397,-11.4534818258365,-235.35005));
#192430=CARTESIAN_POINT('Origin',(636.934816028482,-11.5034818258361,-234.90005));
#192431=CARTESIAN_POINT('',(-40.9488434259496,-10.2512651365233,-235.35005));
#192432=CARTESIAN_POINT('',(-40.4988441937178,-10.2520963950157,-234.90005));
#192433=CARTESIAN_POINT('Origin',(-40.9488434259496,-10.2512651365233,-234.90005));
#192434=CARTESIAN_POINT('Origin',(636.934816028482,-11.5034818258361,-235.35005));
#192435=CARTESIAN_POINT('Origin',(636.934816028482,-11.5034818258361,-234.90005));
#192436=CARTESIAN_POINT('Origin',(-39.7488454733312,-10.2534818258363,-234.90005));
#192437=CARTESIAN_POINT('Origin',(-39.7488454733312,-10.2534818258363,-235.35005));
#192438=CARTESIAN_POINT('Origin',(-39.7488454733312,-10.2534818258363,-234.90005));
#192439=CARTESIAN_POINT('Origin',(-21.5,-2.14794227316951,-234.90005));
#192440=CARTESIAN_POINT('',(-21.5,-0.947942273169508,-235.35005));
#192441=CARTESIAN_POINT('',(-21.5,-1.39794227316951,-234.90005));
#192442=CARTESIAN_POINT('Origin',(-21.5,-0.947942273169508,-234.90005));
#192443=CARTESIAN_POINT('',(-20.3,-2.14794227316951,-235.35005));
#192444=CARTESIAN_POINT('Origin',(-21.5,-2.14794227316951,-235.35005));
#192445=CARTESIAN_POINT('',(-20.75,-2.14794227316951,-234.90005));
#192446=CARTESIAN_POINT('Origin',(-20.3,-2.14794227316951,-234.90005));
#192447=CARTESIAN_POINT('Origin',(-21.5,-2.14794227316951,-234.90005));
#192448=CARTESIAN_POINT('Origin',(-20.3,-25.4138432731711,-234.90005));
#192449=CARTESIAN_POINT('',(-20.75,-10.2534818258363,-234.90005));
#192450=CARTESIAN_POINT('',(-20.3,-10.2534818258363,-235.35005));
#192451=CARTESIAN_POINT('Origin',(-20.3,-10.2534818258363,-234.90005));
#192452=CARTESIAN_POINT('',(-20.75,-2.14794227316951,-234.90005));
#192453=CARTESIAN_POINT('',(-20.3,-10.2534818258363,-235.35005));
#192454=CARTESIAN_POINT('Origin',(296.501483394397,-0.94794227316939,-234.90005));
#192455=CARTESIAN_POINT('',(-29.125,-0.947942273169511,-235.35005));
#192456=CARTESIAN_POINT('',(-29.125,-1.39794227316951,-234.90005));
#192457=CARTESIAN_POINT('Origin',(-29.125,-0.947942273169511,-234.90005));
#192458=CARTESIAN_POINT('',(296.501483394397,-0.94794227316939,-235.35005));
#192459=CARTESIAN_POINT('',(1.11087130309497E-13,-1.3979422731695,-234.90005));
#192460=CARTESIAN_POINT('Origin',(-21.5,-10.2534818258363,-234.90005));
#192461=CARTESIAN_POINT('',(-21.5,-11.0034818258363,-234.90005));
#192462=CARTESIAN_POINT('',(-21.5,-11.4534818258363,-235.35005));
#192463=CARTESIAN_POINT('Origin',(-21.5,-11.4534818258363,-234.90005));
#192464=CARTESIAN_POINT('Origin',(-21.5,-10.2534818258363,-234.90005));
#192465=CARTESIAN_POINT('Origin',(-21.5,-10.2534818258363,-235.35005));
#192466=CARTESIAN_POINT('Origin',(-29.125,-2.14794227316951,-234.90005));
#192467=CARTESIAN_POINT('',(-30.325,-2.14794227316951,-235.35005));
#192468=CARTESIAN_POINT('',(-29.875,-2.14794227316951,-234.90005));
#192469=CARTESIAN_POINT('Origin',(-30.325,-2.14794227316951,-234.90005));
#192470=CARTESIAN_POINT('Origin',(-29.125,-2.14794227316951,-235.35005));
#192471=CARTESIAN_POINT('Origin',(-29.125,-2.14794227316951,-234.90005));
#192472=CARTESIAN_POINT('Origin',(296.501483394397,-11.4534818258365,-234.90005));
#192473=CARTESIAN_POINT('',(-29.125,-11.0034818258363,-234.90005));
#192474=CARTESIAN_POINT('',(-29.125,-11.4534818258363,-235.35005));
#192475=CARTESIAN_POINT('Origin',(-29.125,-11.4534818258363,-234.90005));
#192476=CARTESIAN_POINT('',(2.22174260618994E-13,-11.0034818258363,-234.90005));
#192477=CARTESIAN_POINT('',(296.501483394397,-11.4534818258365,-235.35005));
#192478=CARTESIAN_POINT('Origin',(-30.325,-25.4138432731711,-234.90005));
#192479=CARTESIAN_POINT('',(-30.325,-10.2534818258363,-235.35005));
#192480=CARTESIAN_POINT('',(-29.875,-10.2534818258363,-234.90005));
#192481=CARTESIAN_POINT('Origin',(-30.325,-10.2534818258363,-234.90005));
#192482=CARTESIAN_POINT('',(-30.325,-2.14794227316951,-235.35005));
#192483=CARTESIAN_POINT('',(-29.875,-10.2534818258363,-234.90005));
#192484=CARTESIAN_POINT('Origin',(-29.125,-10.2534818258363,-234.90005));
#192485=CARTESIAN_POINT('Origin',(-29.125,-10.2534818258363,-235.35005));
#192486=CARTESIAN_POINT('Origin',(-29.125,-10.2534818258363,-234.90005));
#192487=CARTESIAN_POINT('Origin',(-12.7946237611812,-10.2534818258363,-234.90005));
#192488=CARTESIAN_POINT('',(-11.6003099441285,-10.370163042821,-235.35005));
#192489=CARTESIAN_POINT('',(-12.0481776255232,-10.3264075864518,-234.90005));
#192490=CARTESIAN_POINT('Origin',(-11.6003099441285,-10.370163042821,-234.90005));
#192491=CARTESIAN_POINT('',(-12.7946237611812,-11.4534818258363,-235.35005));
#192492=CARTESIAN_POINT('Origin',(-12.7946237611812,-10.2534818258363,-235.35005));
#192493=CARTESIAN_POINT('',(-12.7946237611812,-11.0034818258363,-234.90005));
#192494=CARTESIAN_POINT('Origin',(-12.7946237611812,-11.4534818258363,-234.90005));
#192495=CARTESIAN_POINT('Origin',(-12.7946237611812,-10.2534818258363,-234.90005));
#192496=CARTESIAN_POINT('Origin',(296.501483394397,-11.4534818258365,-234.90005));
#192497=CARTESIAN_POINT('',(-19.,-11.0034818258363,-234.90005));
#192498=CARTESIAN_POINT('',(-19.,-11.4534818258363,-235.35005));
#192499=CARTESIAN_POINT('Origin',(-19.,-11.4534818258363,-234.90005));
#192500=CARTESIAN_POINT('',(2.22174260618994E-13,-11.0034818258363,-234.90005));
#192501=CARTESIAN_POINT('',(296.501483394397,-11.4534818258365,-235.35005));
#192502=CARTESIAN_POINT('Origin',(0.,-11.5034818258363,-234.90005));
#192503=CARTESIAN_POINT('',(-10.8748986968178,-7.30965533947201,-235.35005));
#192504=CARTESIAN_POINT('',(-11.294759518486,-7.14773903260897,-234.90005));
#192505=CARTESIAN_POINT('Origin',(-10.8748986968178,-7.30965533947201,-234.90005));
#192506=CARTESIAN_POINT('Origin',(0.,-11.5034818258363,-235.35005));
#192507=CARTESIAN_POINT('Origin',(0.,-11.5034818258363,-234.90005));
#192508=CARTESIAN_POINT('Origin',(-19.,-10.2534818258363,-234.90005));
#192509=CARTESIAN_POINT('',(-19.75,-10.2534818258363,-234.90005));
#192510=CARTESIAN_POINT('',(-20.2,-10.2534818258363,-235.35005));
#192511=CARTESIAN_POINT('Origin',(-20.2,-10.2534818258363,-234.90005));
#192512=CARTESIAN_POINT('Origin',(-19.,-10.2534818258363,-234.90005));
#192513=CARTESIAN_POINT('Origin',(-19.,-10.2534818258363,-235.35005));
#192514=CARTESIAN_POINT('Origin',(-20.625,-3.54959888009691,-234.90005));
#192515=CARTESIAN_POINT('',(-10.1749999999999,-3.54959888009691,-235.35005));
#192516=CARTESIAN_POINT('',(-10.6249999999999,-3.54959888009691,-234.90005));
#192517=CARTESIAN_POINT('Origin',(-10.1749999999999,-3.54959888009691,-234.90005));
#192518=CARTESIAN_POINT('Origin',(-20.625,-3.54959888009691,-235.35005));
#192519=CARTESIAN_POINT('Origin',(-20.625,-3.54959888009691,-234.90005));
#192520=CARTESIAN_POINT('Origin',(-20.2,-25.4138432731711,-234.90005));
#192521=CARTESIAN_POINT('',(-19.75,-2.14794227316951,-234.90005));
#192522=CARTESIAN_POINT('',(-20.2,-2.14794227316951,-235.35005));
#192523=CARTESIAN_POINT('Origin',(-20.2,-2.14794227316951,-234.90005));
#192524=CARTESIAN_POINT('',(-19.75,-10.2534818258363,-234.90005));
#192525=CARTESIAN_POINT('',(-20.2,-2.14794227316951,-235.35005));
#192526=CARTESIAN_POINT('Origin',(-10.1749999999999,-25.4138432731711,-234.90005));
#192527=CARTESIAN_POINT('',(-10.1749999999999,-2.14794227316951,-235.35005));
#192528=CARTESIAN_POINT('',(-10.6249999999999,-2.14794227316951,-234.90005));
#192529=CARTESIAN_POINT('Origin',(-10.1749999999999,-2.14794227316951,-234.90005));
#192530=CARTESIAN_POINT('',(-10.1749999999999,-3.54959888009691,-235.35005));
#192531=CARTESIAN_POINT('',(-10.6249999999999,-2.14794227316951,-234.90005));
#192532=CARTESIAN_POINT('Origin',(-19.,-2.14794227316951,-234.90005));
#192533=CARTESIAN_POINT('',(-19.,-1.39794227316951,-234.90005));
#192534=CARTESIAN_POINT('',(-19.,-0.947942273169507,-235.35005));
#192535=CARTESIAN_POINT('Origin',(-19.,-0.947942273169508,-234.90005));
#192536=CARTESIAN_POINT('Origin',(-19.,-2.14794227316951,-234.90005));
#192537=CARTESIAN_POINT('Origin',(-19.,-2.14794227316951,-235.35005));
#192538=CARTESIAN_POINT('Origin',(-11.3749999999999,-2.14794227316951,-234.90005));
#192539=CARTESIAN_POINT('',(-11.3749999999999,-0.947942273169504,-235.35005));
#192540=CARTESIAN_POINT('',(-11.3749999999999,-1.3979422731695,-234.90005));
#192541=CARTESIAN_POINT('Origin',(-11.3749999999999,-0.947942273169504,
-234.90005));
#192542=CARTESIAN_POINT('Origin',(-11.3749999999999,-2.14794227316951,-235.35005));
#192543=CARTESIAN_POINT('Origin',(-11.3749999999999,-2.14794227316951,-234.90005));
#192544=CARTESIAN_POINT('Origin',(296.501483394397,-0.94794227316939,-234.90005));
#192545=CARTESIAN_POINT('',(296.501483394397,-0.94794227316939,-235.35005));
#192546=CARTESIAN_POINT('',(1.11087130309497E-13,-1.3979422731695,-234.90005));
#192547=CARTESIAN_POINT('Origin',(-11.3749999999999,-20.8590213785032,-234.90005));
#192548=CARTESIAN_POINT('',(-10.1749999999999,-20.8590213785032,-235.35005));
#192549=CARTESIAN_POINT('',(-10.6249999999999,-20.8590213785032,-234.90005));
#192550=CARTESIAN_POINT('Origin',(-10.1749999999999,-20.8590213785032,-234.90005));
#192551=CARTESIAN_POINT('',(-11.3749999999999,-22.0590213785032,-235.35005));
#192552=CARTESIAN_POINT('Origin',(-11.3749999999999,-20.8590213785032,-235.35005));
#192553=CARTESIAN_POINT('',(-11.3749999999999,-21.6090213785032,-234.90005));
#192554=CARTESIAN_POINT('Origin',(-11.3749999999999,-22.0590213785032,-234.90005));
#192555=CARTESIAN_POINT('Origin',(-11.3749999999999,-20.8590213785032,-234.90005));
#192556=CARTESIAN_POINT('Origin',(296.501483394397,-22.0590213785033,-234.90005));
#192557=CARTESIAN_POINT('',(-19.,-21.6090213785031,-234.90005));
#192558=CARTESIAN_POINT('',(-19.,-22.0590213785031,-235.35005));
#192559=CARTESIAN_POINT('Origin',(-19.,-22.0590213785031,-234.90005));
#192560=CARTESIAN_POINT('',(3.33261390928491E-13,-21.6090213785032,-234.90005));
#192561=CARTESIAN_POINT('',(296.501483394397,-22.0590213785033,-235.35005));
#192562=CARTESIAN_POINT('Origin',(-10.1749999999999,-25.4138432731711,-234.90005));
#192563=CARTESIAN_POINT('',(-10.1749999999999,-19.4573647715757,-235.35005));
#192564=CARTESIAN_POINT('',(-10.6249999999999,-19.4573647715757,-234.90005));
#192565=CARTESIAN_POINT('Origin',(-10.1749999999999,-19.4573647715757,-234.90005));
#192566=CARTESIAN_POINT('',(-10.1749999999999,-20.8590213785032,-235.35005));
#192567=CARTESIAN_POINT('',(-10.6249999999999,-19.4573647715757,-234.90005));
#192568=CARTESIAN_POINT('Origin',(-19.,-20.8590213785032,-234.90005));
#192569=CARTESIAN_POINT('',(-19.75,-20.8590213785032,-234.90005));
#192570=CARTESIAN_POINT('',(-20.2,-20.8590213785032,-235.35005));
#192571=CARTESIAN_POINT('Origin',(-20.2,-20.8590213785032,-234.90005));
#192572=CARTESIAN_POINT('Origin',(-19.,-20.8590213785032,-234.90005));
#192573=CARTESIAN_POINT('Origin',(-19.,-20.8590213785032,-235.35005));
#192574=CARTESIAN_POINT('Origin',(-20.625,-19.4573647715757,-234.90005));
#192575=CARTESIAN_POINT('',(-10.8748986968178,-15.6973083122006,-235.35005));
#192576=CARTESIAN_POINT('',(-11.294759518486,-15.8592246190636,-234.90005));
#192577=CARTESIAN_POINT('Origin',(-10.8748986968178,-15.6973083122006,-234.90005));
#192578=CARTESIAN_POINT('Origin',(-20.625,-19.4573647715757,-235.35005));
#192579=CARTESIAN_POINT('Origin',(-20.625,-19.4573647715757,-234.90005));
#192580=CARTESIAN_POINT('Origin',(-20.2,-25.4138432731711,-234.90005));
#192581=CARTESIAN_POINT('',(-19.75,-12.7534818258363,-234.90005));
#192582=CARTESIAN_POINT('',(-20.2,-12.7534818258363,-235.35005));
#192583=CARTESIAN_POINT('Origin',(-20.2,-12.7534818258363,-234.90005));
#192584=CARTESIAN_POINT('',(-19.75,-20.8590213785032,-234.90005));
#192585=CARTESIAN_POINT('',(-20.2,-12.7534818258363,-235.35005));
#192586=CARTESIAN_POINT('Origin',(0.,-11.5034818258363,-234.90005));
#192587=CARTESIAN_POINT('',(-11.6003099441285,-12.6368006088516,-235.35005));
#192588=CARTESIAN_POINT('',(-12.0481776255232,-12.6805560652209,-234.90005));
#192589=CARTESIAN_POINT('Origin',(-11.6003099441285,-12.6368006088516,-234.90005));
#192590=CARTESIAN_POINT('Origin',(0.,-11.5034818258363,-235.35005));
#192591=CARTESIAN_POINT('Origin',(0.,-11.5034818258363,-234.90005));
#192592=CARTESIAN_POINT('Origin',(-19.,-12.7534818258363,-234.90005));
#192593=CARTESIAN_POINT('',(-19.,-12.0034818258363,-234.90005));
#192594=CARTESIAN_POINT('',(-19.,-11.5534818258363,-235.35005));
#192595=CARTESIAN_POINT('Origin',(-19.,-11.5534818258363,-234.90005));
#192596=CARTESIAN_POINT('Origin',(-19.,-12.7534818258363,-234.90005));
#192597=CARTESIAN_POINT('Origin',(-19.,-12.7534818258363,-235.35005));
#192598=CARTESIAN_POINT('Origin',(-12.7946237611812,-12.7534818258363,-234.90005));
#192599=CARTESIAN_POINT('',(-12.7946237611812,-11.5534818258363,-235.35005));
#192600=CARTESIAN_POINT('',(-12.7946237611812,-12.0034818258363,-234.90005));
#192601=CARTESIAN_POINT('Origin',(-12.7946237611812,-11.5534818258363,-234.90005));
#192602=CARTESIAN_POINT('Origin',(-12.7946237611812,-12.7534818258363,-235.35005));
#192603=CARTESIAN_POINT('Origin',(-12.7946237611812,-12.7534818258363,-234.90005));
#192604=CARTESIAN_POINT('Origin',(296.501483394397,-11.5534818258362,-234.90005));
#192605=CARTESIAN_POINT('',(296.501483394397,-11.5534818258362,-235.35005));
#192606=CARTESIAN_POINT('',(2.22174260618994E-13,-12.0034818258363,-234.90005));
#192607=CARTESIAN_POINT('Origin',(-21.5,-20.8590213785032,-234.90005));
#192608=CARTESIAN_POINT('',(-20.3,-20.8590213785032,-235.35005));
#192609=CARTESIAN_POINT('',(-20.75,-20.8590213785032,-234.90005));
#192610=CARTESIAN_POINT('Origin',(-20.3,-20.8590213785032,-234.90005));
#192611=CARTESIAN_POINT('',(-21.5,-22.0590213785031,-235.35005));
#192612=CARTESIAN_POINT('Origin',(-21.5,-20.8590213785032,-235.35005));
#192613=CARTESIAN_POINT('',(-21.5,-21.6090213785031,-234.90005));
#192614=CARTESIAN_POINT('Origin',(-21.5,-22.0590213785031,-234.90005));
#192615=CARTESIAN_POINT('Origin',(-21.5,-20.8590213785032,-234.90005));
#192616=CARTESIAN_POINT('Origin',(296.501483394397,-22.0590213785033,-234.90005));
#192617=CARTESIAN_POINT('',(-29.125,-21.6090213785031,-234.90005));
#192618=CARTESIAN_POINT('',(-29.125,-22.0590213785031,-235.35005));
#192619=CARTESIAN_POINT('Origin',(-29.125,-22.0590213785031,-234.90005));
#192620=CARTESIAN_POINT('',(3.33261390928491E-13,-21.6090213785032,-234.90005));
#192621=CARTESIAN_POINT('',(296.501483394397,-22.0590213785033,-235.35005));
#192622=CARTESIAN_POINT('Origin',(-20.3,-25.4138432731711,-234.90005));
#192623=CARTESIAN_POINT('',(-20.3,-12.7534818258363,-235.35005));
#192624=CARTESIAN_POINT('',(-20.75,-12.7534818258363,-234.90005));
#192625=CARTESIAN_POINT('Origin',(-20.3,-12.7534818258363,-234.90005));
#192626=CARTESIAN_POINT('',(-20.3,-20.8590213785032,-235.35005));
#192627=CARTESIAN_POINT('',(-20.75,-12.7534818258363,-234.90005));
#192628=CARTESIAN_POINT('Origin',(-29.125,-20.8590213785032,-234.90005));
#192629=CARTESIAN_POINT('',(-29.875,-20.8590213785032,-234.90005));
#192630=CARTESIAN_POINT('',(-30.325,-20.8590213785032,-235.35005));
#192631=CARTESIAN_POINT('Origin',(-30.325,-20.8590213785032,-234.90005));
#192632=CARTESIAN_POINT('Origin',(-29.125,-20.8590213785032,-234.90005));
#192633=CARTESIAN_POINT('Origin',(-29.125,-20.8590213785032,-235.35005));
#192634=CARTESIAN_POINT('Origin',(-21.5,-12.7534818258363,-234.90005));
#192635=CARTESIAN_POINT('',(-21.5,-11.5534818258363,-235.35005));
#192636=CARTESIAN_POINT('',(-21.5,-12.0034818258363,-234.90005));
#192637=CARTESIAN_POINT('Origin',(-21.5,-11.5534818258363,-234.90005));
#192638=CARTESIAN_POINT('Origin',(-21.5,-12.7534818258363,-235.35005));
#192639=CARTESIAN_POINT('Origin',(-21.5,-12.7534818258363,-234.90005));
#192640=CARTESIAN_POINT('Origin',(-30.325,-25.4138432731711,-234.90005));
#192641=CARTESIAN_POINT('',(-29.875,-12.7534818258363,-234.90005));
#192642=CARTESIAN_POINT('',(-30.325,-12.7534818258363,-235.35005));
#192643=CARTESIAN_POINT('Origin',(-30.325,-12.7534818258363,-234.90005));
#192644=CARTESIAN_POINT('',(-29.875,-20.8590213785032,-234.90005));
#192645=CARTESIAN_POINT('',(-30.325,-12.7534818258363,-235.35005));
#192646=CARTESIAN_POINT('Origin',(296.501483394397,-11.5534818258362,-234.90005));
#192647=CARTESIAN_POINT('',(-29.125,-11.5534818258363,-235.35005));
#192648=CARTESIAN_POINT('',(-29.125,-12.0034818258363,-234.90005));
#192649=CARTESIAN_POINT('Origin',(-29.125,-11.5534818258363,-234.90005));
#192650=CARTESIAN_POINT('',(296.501483394397,-11.5534818258362,-235.35005));
#192651=CARTESIAN_POINT('',(2.22174260618994E-13,-12.0034818258363,-234.90005));
#192652=CARTESIAN_POINT('Origin',(-29.125,-12.7534818258363,-234.90005));
#192653=CARTESIAN_POINT('Origin',(-29.125,-12.7534818258363,-235.35005));
#192654=CARTESIAN_POINT('Origin',(-29.125,-12.7534818258363,-234.90005));
#192655=CARTESIAN_POINT('Origin',(-31.625,-20.8590213785032,-234.90005));
#192656=CARTESIAN_POINT('',(-30.425,-20.8590213785032,-235.35005));
#192657=CARTESIAN_POINT('',(-30.875,-20.8590213785032,-234.90005));
#192658=CARTESIAN_POINT('Origin',(-30.425,-20.8590213785032,-234.90005));
#192659=CARTESIAN_POINT('',(-31.625,-22.0590213785031,-235.35005));
#192660=CARTESIAN_POINT('Origin',(-31.625,-20.8590213785032,-235.35005));
#192661=CARTESIAN_POINT('',(-31.625,-21.6090213785031,-234.90005));
#192662=CARTESIAN_POINT('Origin',(-31.625,-22.0590213785031,-234.90005));
#192663=CARTESIAN_POINT('Origin',(-31.625,-20.8590213785032,-234.90005));
#192664=CARTESIAN_POINT('Origin',(296.501483394397,-22.0590213785033,-234.90005));
#192665=CARTESIAN_POINT('',(-39.6853241707135,-21.6090213785031,-234.90005));
#192666=CARTESIAN_POINT('',(-39.6853241707135,-22.0590213785031,-235.35005));
#192667=CARTESIAN_POINT('Origin',(-39.6853241707135,-22.0590213785031,-234.90005));
#192668=CARTESIAN_POINT('',(3.33261390928491E-13,-21.6090213785032,-234.90005));
#192669=CARTESIAN_POINT('',(296.501483394397,-22.0590213785033,-235.35005));
#192670=CARTESIAN_POINT('Origin',(-30.425,-25.4138432731711,-234.90005));
#192671=CARTESIAN_POINT('',(-30.425,-12.7534818258363,-235.35005));
#192672=CARTESIAN_POINT('',(-30.875,-12.7534818258363,-234.90005));
#192673=CARTESIAN_POINT('Origin',(-30.425,-12.7534818258363,-234.90005));
#192674=CARTESIAN_POINT('',(-30.425,-20.8590213785032,-235.35005));
#192675=CARTESIAN_POINT('',(-30.875,-12.7534818258363,-234.90005));
#192676=CARTESIAN_POINT('Origin',(-39.6853241707135,-20.8590213785032,-234.90005));
#192677=CARTESIAN_POINT('',(-40.4352524876037,-20.8693905407753,-234.90005));
#192678=CARTESIAN_POINT('',(-40.8852094777378,-20.8756120381386,-235.35005));
#192679=CARTESIAN_POINT('Origin',(-40.8852094777378,-20.8756120381386,-234.90005));
#192680=CARTESIAN_POINT('Origin',(-39.6853241707135,-20.8590213785032,-234.90005));
#192681=CARTESIAN_POINT('Origin',(-39.6853241707135,-20.8590213785032,-235.35005));
#192682=CARTESIAN_POINT('Origin',(-31.625,-12.7534818258363,-234.90005));
#192683=CARTESIAN_POINT('',(-31.625,-11.5534818258363,-235.35005));
#192684=CARTESIAN_POINT('',(-31.625,-12.0034818258363,-234.90005));
#192685=CARTESIAN_POINT('Origin',(-31.625,-11.5534818258363,-234.90005));
#192686=CARTESIAN_POINT('Origin',(-31.625,-12.7534818258363,-235.35005));
#192687=CARTESIAN_POINT('Origin',(-31.625,-12.7534818258363,-234.90005));
#192688=CARTESIAN_POINT('Origin',(636.934816028482,-11.5034818258361,-234.90005));
#192689=CARTESIAN_POINT('',(-40.4988441937178,-12.754867256657,-234.90005));
#192690=CARTESIAN_POINT('',(-40.9488434259496,-12.7556985151494,-235.35005));
#192691=CARTESIAN_POINT('Origin',(-40.9488434259496,-12.7556985151494,-234.90005));
#192692=CARTESIAN_POINT('Origin',(636.934816028482,-11.5034818258361,-234.90005));
#192693=CARTESIAN_POINT('Origin',(636.934816028482,-11.5034818258361,-235.35005));
#192694=CARTESIAN_POINT('Origin',(296.501483394397,-11.5534818258362,-234.90005));
#192695=CARTESIAN_POINT('',(-39.7488454733312,-11.5534818258363,-235.35005));
#192696=CARTESIAN_POINT('',(-39.7488454733312,-12.0034818258363,-234.90005));
#192697=CARTESIAN_POINT('Origin',(-39.7488454733312,-11.5534818258363,-234.90005));
#192698=CARTESIAN_POINT('',(296.501483394397,-11.5534818258362,-235.35005));
#192699=CARTESIAN_POINT('',(2.22174260618994E-13,-12.0034818258363,-234.90005));
#192700=CARTESIAN_POINT('Origin',(-39.7488454733312,-12.7534818258363,-234.90005));
#192701=CARTESIAN_POINT('Origin',(-39.7488454733312,-12.7534818258363,-235.35005));
#192702=CARTESIAN_POINT('Origin',(-39.7488454733312,-12.7534818258363,-234.90005));
#192703=CARTESIAN_POINT('Origin',(-29.125,-23.3590213785032,-234.90005));
#192704=CARTESIAN_POINT('',(-30.325,-23.3590213785032,-235.35005));
#192705=CARTESIAN_POINT('',(-29.875,-23.3590213785032,-234.90005));
#192706=CARTESIAN_POINT('Origin',(-30.325,-23.3590213785032,-234.90005));
#192707=CARTESIAN_POINT('',(-29.125,-22.1590213785032,-235.35005));
#192708=CARTESIAN_POINT('Origin',(-29.125,-23.3590213785032,-235.35005));
#192709=CARTESIAN_POINT('',(-29.125,-22.6090213785032,-234.90005));
#192710=CARTESIAN_POINT('Origin',(-29.125,-22.1590213785032,-234.90005));
#192711=CARTESIAN_POINT('Origin',(-29.125,-23.3590213785032,-234.90005));
#192712=CARTESIAN_POINT('Origin',(296.501483394397,-22.1590213785031,-234.90005));
#192713=CARTESIAN_POINT('',(-21.5,-22.6090213785032,-234.90005));
#192714=CARTESIAN_POINT('',(-21.5,-22.1590213785032,-235.35005));
#192715=CARTESIAN_POINT('Origin',(-21.5,-22.1590213785032,-234.90005));
#192716=CARTESIAN_POINT('',(3.33261390928491E-13,-22.6090213785032,-234.90005));
#192717=CARTESIAN_POINT('',(296.501483394397,-22.1590213785031,-235.35005));
#192718=CARTESIAN_POINT('Origin',(-30.325,-25.4138432731711,-234.90005));
#192719=CARTESIAN_POINT('',(-30.325,-31.46456093117,-235.35005));
#192720=CARTESIAN_POINT('',(-29.875,-31.46456093117,-234.90005));
#192721=CARTESIAN_POINT('Origin',(-30.325,-31.46456093117,-234.90005));
#192722=CARTESIAN_POINT('',(-30.325,-23.3590213785032,-235.35005));
#192723=CARTESIAN_POINT('',(-29.875,-31.46456093117,-234.90005));
#192724=CARTESIAN_POINT('Origin',(-21.5,-23.3590213785032,-234.90005));
#192725=CARTESIAN_POINT('',(-20.75,-23.3590213785032,-234.90005));
#192726=CARTESIAN_POINT('',(-20.3,-23.3590213785032,-235.35005));
#192727=CARTESIAN_POINT('Origin',(-20.3,-23.3590213785032,-234.90005));
#192728=CARTESIAN_POINT('Origin',(-21.5,-23.3590213785032,-234.90005));
#192729=CARTESIAN_POINT('Origin',(-21.5,-23.3590213785032,-235.35005));
#192730=CARTESIAN_POINT('Origin',(-29.125,-31.46456093117,-234.90005));
#192731=CARTESIAN_POINT('',(-29.125,-32.66456093117,-235.35005));
#192732=CARTESIAN_POINT('',(-29.125,-32.21456093117,-234.90005));
#192733=CARTESIAN_POINT('Origin',(-29.125,-32.66456093117,-234.90005));
#192734=CARTESIAN_POINT('Origin',(-29.125,-31.46456093117,-235.35005));
#192735=CARTESIAN_POINT('Origin',(-29.125,-31.46456093117,-234.90005));
#192736=CARTESIAN_POINT('Origin',(-20.3,-25.4138432731711,-234.90005));
#192737=CARTESIAN_POINT('',(-20.75,-31.46456093117,-234.90005));
#192738=CARTESIAN_POINT('',(-20.3,-31.46456093117,-235.35005));
#192739=CARTESIAN_POINT('Origin',(-20.3,-31.46456093117,-234.90005));
#192740=CARTESIAN_POINT('',(-20.75,-23.3590213785032,-234.90005));
#192741=CARTESIAN_POINT('',(-20.3,-31.46456093117,-235.35005));
#192742=CARTESIAN_POINT('Origin',(296.501483394397,-32.6645609311701,-234.90005));
#192743=CARTESIAN_POINT('',(-21.5,-32.66456093117,-235.35005));
#192744=CARTESIAN_POINT('',(-21.5,-32.21456093117,-234.90005));
#192745=CARTESIAN_POINT('Origin',(-21.5,-32.66456093117,-234.90005));
#192746=CARTESIAN_POINT('',(296.501483394397,-32.6645609311701,-235.35005));
#192747=CARTESIAN_POINT('',(0.,-32.21456093117,-234.90005));
#192748=CARTESIAN_POINT('Origin',(-21.5,-31.46456093117,-234.90005));
#192749=CARTESIAN_POINT('Origin',(-21.5,-31.46456093117,-235.35005));
#192750=CARTESIAN_POINT('Origin',(-21.5,-31.46456093117,-234.90005));
#192751=CARTESIAN_POINT('Origin',(-19.,-23.3590213785032,-234.90005));
#192752=CARTESIAN_POINT('',(-20.2,-23.3590213785032,-235.35005));
#192753=CARTESIAN_POINT('',(-19.75,-23.3590213785032,-234.90005));
#192754=CARTESIAN_POINT('Origin',(-20.2,-23.3590213785032,-234.90005));
#192755=CARTESIAN_POINT('',(-19.,-22.1590213785032,-235.35005));
#192756=CARTESIAN_POINT('Origin',(-19.,-23.3590213785032,-235.35005));
#192757=CARTESIAN_POINT('',(-19.,-22.6090213785032,-234.90005));
#192758=CARTESIAN_POINT('Origin',(-19.,-22.1590213785032,-234.90005));
#192759=CARTESIAN_POINT('Origin',(-19.,-23.3590213785032,-234.90005));
#192760=CARTESIAN_POINT('Origin',(296.501483394397,-22.1590213785031,-234.90005));
#192761=CARTESIAN_POINT('',(-11.3749999999999,-22.6090213785032,-234.90005));
#192762=CARTESIAN_POINT('',(-11.3749999999999,-22.1590213785032,-235.35005));
#192763=CARTESIAN_POINT('Origin',(-11.3749999999999,-22.1590213785032,-234.90005));
#192764=CARTESIAN_POINT('',(3.33261390928491E-13,-22.6090213785032,-234.90005));
#192765=CARTESIAN_POINT('',(296.501483394397,-22.1590213785031,-235.35005));
#192766=CARTESIAN_POINT('Origin',(-20.2,-25.4138432731711,-234.90005));
#192767=CARTESIAN_POINT('',(-20.2,-31.46456093117,-235.35005));
#192768=CARTESIAN_POINT('',(-19.75,-31.46456093117,-234.90005));
#192769=CARTESIAN_POINT('Origin',(-20.2,-31.46456093117,-234.90005));
#192770=CARTESIAN_POINT('',(-20.2,-23.3590213785032,-235.35005));
#192771=CARTESIAN_POINT('',(-19.75,-31.46456093117,-234.90005));
#192772=CARTESIAN_POINT('Origin',(-11.3749999999999,-23.3590213785032,-234.90005));
#192773=CARTESIAN_POINT('',(-10.6249999999999,-23.3590213785032,-234.90005));
#192774=CARTESIAN_POINT('',(-10.1749999999999,-23.3590213785032,-235.35005));
#192775=CARTESIAN_POINT('Origin',(-10.1749999999999,-23.3590213785032,-234.90005));
#192776=CARTESIAN_POINT('Origin',(-11.3749999999999,-23.3590213785032,-234.90005));
#192777=CARTESIAN_POINT('Origin',(-11.3749999999999,-23.3590213785032,-235.35005));
#192778=CARTESIAN_POINT('Origin',(-19.,-31.46456093117,-234.90005));
#192779=CARTESIAN_POINT('',(-19.,-32.66456093117,-235.35005));
#192780=CARTESIAN_POINT('',(-19.,-32.21456093117,-234.90005));
#192781=CARTESIAN_POINT('Origin',(-19.,-32.66456093117,-234.90005));
#192782=CARTESIAN_POINT('Origin',(-19.,-31.46456093117,-235.35005));
#192783=CARTESIAN_POINT('Origin',(-19.,-31.46456093117,-234.90005));
#192784=CARTESIAN_POINT('Origin',(-10.1749999999999,-25.4138432731711,-234.90005));
#192785=CARTESIAN_POINT('',(-10.6249999999999,-31.46456093117,-234.90005));
#192786=CARTESIAN_POINT('',(-10.1749999999999,-31.46456093117,-235.35005));
#192787=CARTESIAN_POINT('Origin',(-10.1749999999999,-31.46456093117,-234.90005));
#192788=CARTESIAN_POINT('',(-10.6249999999999,-23.3590213785032,-234.90005));
#192789=CARTESIAN_POINT('',(-10.1749999999999,-31.46456093117,-235.35005));
#192790=CARTESIAN_POINT('Origin',(296.501483394397,-32.6645609311701,-234.90005));
#192791=CARTESIAN_POINT('',(-11.3749999999999,-32.66456093117,-235.35005));
#192792=CARTESIAN_POINT('',(-11.3749999999999,-32.21456093117,-234.90005));
#192793=CARTESIAN_POINT('Origin',(-11.3749999999999,-32.66456093117,-234.90005));
#192794=CARTESIAN_POINT('',(296.501483394397,-32.6645609311701,-235.35005));
#192795=CARTESIAN_POINT('',(0.,-32.21456093117,-234.90005));
#192796=CARTESIAN_POINT('Origin',(-11.3749999999999,-31.46456093117,-234.90005));
#192797=CARTESIAN_POINT('Origin',(-11.3749999999999,-31.46456093117,-235.35005));
#192798=CARTESIAN_POINT('Origin',(-11.3749999999999,-31.46456093117,-234.90005));
#192799=CARTESIAN_POINT('Origin',(-1.25,-31.46456093117,-234.90005));
#192800=CARTESIAN_POINT('',(-0.0499999999999941,-31.46456093117,-235.35005));
#192801=CARTESIAN_POINT('',(-0.5,-31.46456093117,-234.90005));
#192802=CARTESIAN_POINT('Origin',(-0.0499999999999941,-31.46456093117,-234.90005));
#192803=CARTESIAN_POINT('',(-1.25,-32.66456093117,-235.35005));
#192804=CARTESIAN_POINT('Origin',(-1.25,-31.46456093117,-235.35005));
#192805=CARTESIAN_POINT('',(-1.25,-32.21456093117,-234.90005));
#192806=CARTESIAN_POINT('Origin',(-1.25,-32.66456093117,-234.90005));
#192807=CARTESIAN_POINT('Origin',(-1.25,-31.46456093117,-234.90005));
#192808=CARTESIAN_POINT('Origin',(296.501483394397,-32.6645609311701,-234.90005));
#192809=CARTESIAN_POINT('',(-8.87499999999984,-32.21456093117,-234.90005));
#192810=CARTESIAN_POINT('',(-8.87499999999984,-32.66456093117,-235.35005));
#192811=CARTESIAN_POINT('Origin',(-8.87499999999984,-32.66456093117,-234.90005));
#192812=CARTESIAN_POINT('',(0.,-32.21456093117,-234.90005));
#192813=CARTESIAN_POINT('',(296.501483394397,-32.6645609311701,-235.35005));
#192814=CARTESIAN_POINT('Origin',(-0.0499999999999945,-25.4138432731711,
-234.90005));
#192815=CARTESIAN_POINT('',(-0.0499999999999967,-25.3025207885872,-235.35005));
#192816=CARTESIAN_POINT('',(-0.5,-25.3025207885872,-234.90005));
#192817=CARTESIAN_POINT('Origin',(-0.0499999999999967,-25.3025207885872,
-234.90005));
#192818=CARTESIAN_POINT('',(-0.0499999999999941,-31.46456093117,-235.35005));
#192819=CARTESIAN_POINT('',(-0.5,-25.3025207885872,-234.90005));
#192820=CARTESIAN_POINT('Origin',(-8.87499999999984,-31.46456093117,-234.90005));
#192821=CARTESIAN_POINT('',(-9.62499999999984,-31.46456093117,-234.90005));
#192822=CARTESIAN_POINT('',(-10.0749999999998,-31.46456093117,-235.35005));
#192823=CARTESIAN_POINT('Origin',(-10.0749999999998,-31.46456093117,-234.90005));
#192824=CARTESIAN_POINT('Origin',(-8.87499999999984,-31.46456093117,-234.90005));
#192825=CARTESIAN_POINT('Origin',(-8.87499999999984,-31.46456093117,-235.35005));
#192826=CARTESIAN_POINT('Origin',(-1.25,-25.3025207885872,-234.90005));
#192827=CARTESIAN_POINT('',(-1.14174005138534,-24.107414189356,-235.35005));
#192828=CARTESIAN_POINT('',(-1.18233753211584,-24.5555791640676,-234.90005));
#192829=CARTESIAN_POINT('Origin',(-1.14174005138534,-24.107414189356,-234.90005));
#192830=CARTESIAN_POINT('Origin',(-1.25,-25.3025207885872,-235.35005));
#192831=CARTESIAN_POINT('Origin',(-1.25,-25.3025207885872,-234.90005));
#192832=CARTESIAN_POINT('Origin',(-10.075,-25.4138432731712,-234.90005));
#192833=CARTESIAN_POINT('',(-9.62499999999985,-23.3741205625531,-234.90005));
#192834=CARTESIAN_POINT('',(-10.075,-23.3741205625531,-235.35005));
#192835=CARTESIAN_POINT('Origin',(-10.0749999999998,-23.3741205625531,-234.90005));
#192836=CARTESIAN_POINT('',(-9.62499999999984,-31.46456093117,-234.90005));
#192837=CARTESIAN_POINT('',(-10.075,-23.3741205625531,-235.35005));
#192838=CARTESIAN_POINT('Origin',(0.,-11.5034818258363,-234.90005));
#192839=CARTESIAN_POINT('',(-5.15044918227034,-23.0635663666157,-235.35005));
#192840=CARTESIAN_POINT('',(-5.33358654455951,-23.474614668563,-234.90005));
#192841=CARTESIAN_POINT('Origin',(-5.15044918227034,-23.0635663666157,-234.90005));
#192842=CARTESIAN_POINT('Origin',(0.,-11.5034818258363,-235.35005));
#192843=CARTESIAN_POINT('Origin',(0.,-11.5034818258363,-234.90005));
#192844=CARTESIAN_POINT('Origin',(-8.87499999999985,-23.3741205625531,-234.90005));
#192845=CARTESIAN_POINT('',(-8.80646304347558,-22.176079375619,-235.35005));
#192846=CARTESIAN_POINT('Origin',(-8.87499999999985,-23.3741205625531,-235.35005));
#192847=CARTESIAN_POINT('',(-8.83216440217218,-22.6253448207192,-234.90005));
#192848=CARTESIAN_POINT('Origin',(-8.80646304347558,-22.176079375619,-234.90005));
#192849=CARTESIAN_POINT('Origin',(-8.87499999999985,-23.3741205625531,-234.90005));
#192850=CARTESIAN_POINT('Origin',(-9.40330570654103,-32.6090213785032,-234.90005));
#192851=CARTESIAN_POINT('Origin',(-9.40330570654103,-32.6090213785032,-234.90005));
#192852=CARTESIAN_POINT('Origin',(-9.40330570654103,-32.6090213785032,-235.35005));
#192853=CARTESIAN_POINT('Origin',(-31.625,-31.46456093117,-234.90005));
#192854=CARTESIAN_POINT('',(-30.425,-31.46456093117,-235.35005));
#192855=CARTESIAN_POINT('',(-30.875,-31.46456093117,-234.90005));
#192856=CARTESIAN_POINT('Origin',(-30.425,-31.46456093117,-234.90005));
#192857=CARTESIAN_POINT('',(-31.625,-32.66456093117,-235.35005));
#192858=CARTESIAN_POINT('Origin',(-31.625,-31.46456093117,-235.35005));
#192859=CARTESIAN_POINT('',(-31.625,-32.21456093117,-234.90005));
#192860=CARTESIAN_POINT('Origin',(-31.625,-32.66456093117,-234.90005));
#192861=CARTESIAN_POINT('Origin',(-31.625,-31.46456093117,-234.90005));
#192862=CARTESIAN_POINT('Origin',(296.501483394397,-32.6645609311701,-234.90005));
#192863=CARTESIAN_POINT('',(-39.4555265729267,-32.21456093117,-234.90005));
#192864=CARTESIAN_POINT('',(-39.4555265729267,-32.66456093117,-235.35005));
#192865=CARTESIAN_POINT('Origin',(-39.4555265729267,-32.66456093117,-234.90005));
#192866=CARTESIAN_POINT('',(0.,-32.21456093117,-234.90005));
#192867=CARTESIAN_POINT('',(296.501483394397,-32.6645609311701,-235.35005));
#192868=CARTESIAN_POINT('Origin',(-30.425,-25.4138432731711,-234.90005));
#192869=CARTESIAN_POINT('',(-30.425,-23.3590213785032,-235.35005));
#192870=CARTESIAN_POINT('',(-30.875,-23.3590213785032,-234.90005));
#192871=CARTESIAN_POINT('Origin',(-30.425,-23.3590213785032,-234.90005));
#192872=CARTESIAN_POINT('',(-30.425,-31.46456093117,-235.35005));
#192873=CARTESIAN_POINT('',(-30.875,-23.3590213785032,-234.90005));
#192874=CARTESIAN_POINT('Origin',(-39.4555265729267,-31.46456093117,-234.90005));
#192875=CARTESIAN_POINT('',(-40.2052001948774,-31.486684686535,-234.90005));
#192876=CARTESIAN_POINT('',(-40.6550043680477,-31.499958939754,-235.35005));
#192877=CARTESIAN_POINT('Origin',(-40.6550043680476,-31.499958939754,-234.90005));
#192878=CARTESIAN_POINT('Origin',(-39.4555265729267,-31.46456093117,-234.90005));
#192879=CARTESIAN_POINT('Origin',(-39.4555265729267,-31.46456093117,-235.35005));
#192880=CARTESIAN_POINT('Origin',(-31.625,-23.3590213785032,-234.90005));
#192881=CARTESIAN_POINT('',(-31.625,-22.1590213785032,-235.35005));
#192882=CARTESIAN_POINT('',(-31.625,-22.6090213785032,-234.90005));
#192883=CARTESIAN_POINT('Origin',(-31.625,-22.1590213785032,-234.90005));
#192884=CARTESIAN_POINT('Origin',(-31.625,-23.3590213785032,-235.35005));
#192885=CARTESIAN_POINT('Origin',(-31.625,-23.3590213785032,-234.90005));
#192886=CARTESIAN_POINT('Origin',(636.934816028482,-11.5034818258361,-234.90005));
#192887=CARTESIAN_POINT('',(-40.3960221980465,-23.3721614024167,-234.90005));
#192888=CARTESIAN_POINT('',(-40.8459531286544,-23.3800454167648,-235.35005));
#192889=CARTESIAN_POINT('Origin',(-40.8459531286544,-23.3800454167648,-234.90005));
#192890=CARTESIAN_POINT('Origin',(636.934816028482,-11.5034818258361,-234.90005));
#192891=CARTESIAN_POINT('Origin',(636.934816028482,-11.5034818258361,-235.35005));
#192892=CARTESIAN_POINT('Origin',(296.501483394397,-22.1590213785031,-234.90005));
#192893=CARTESIAN_POINT('',(-39.6461373136998,-22.1590213785032,-235.35005));
#192894=CARTESIAN_POINT('',(-39.6461373136998,-22.6090213785032,-234.90005));
#192895=CARTESIAN_POINT('Origin',(-39.6461373136998,-22.1590213785032,-234.90005));
#192896=CARTESIAN_POINT('',(296.501483394397,-22.1590213785031,-235.35005));
#192897=CARTESIAN_POINT('',(3.33261390928491E-13,-22.6090213785032,-234.90005));
#192898=CARTESIAN_POINT('Origin',(-39.6461373136998,-23.3590213785032,-234.90005));
#192899=CARTESIAN_POINT('Origin',(-39.6461373136998,-23.3590213785032,-235.35005));
#192900=CARTESIAN_POINT('Origin',(-39.6461373136998,-23.3590213785032,-234.90005));
#192901=CARTESIAN_POINT('Origin',(-31.625,-42.0701004838368,-234.90005));
#192902=CARTESIAN_POINT('',(-30.425,-42.0701004838368,-235.35005));
#192903=CARTESIAN_POINT('',(-30.875,-42.0701004838368,-234.90005));
#192904=CARTESIAN_POINT('Origin',(-30.425,-42.0701004838368,-234.90005));
#192905=CARTESIAN_POINT('',(-31.625,-43.2701004838368,-235.35005));
#192906=CARTESIAN_POINT('Origin',(-31.625,-42.0701004838368,-235.35005));
#192907=CARTESIAN_POINT('',(-31.625,-42.8201004838368,-234.90005));
#192908=CARTESIAN_POINT('Origin',(-31.625,-43.2701004838368,-234.90005));
#192909=CARTESIAN_POINT('Origin',(-31.625,-42.0701004838368,-234.90005));
#192910=CARTESIAN_POINT('Origin',(296.501483394397,-43.270100483837,-234.90005));
#192911=CARTESIAN_POINT('',(-36.0311576807678,-42.8201004838368,-234.90005));
#192912=CARTESIAN_POINT('',(-36.0311576807678,-43.2701004838368,-235.35005));
#192913=CARTESIAN_POINT('Origin',(-36.0311576807678,-43.2701004838368,-234.90005));
#192914=CARTESIAN_POINT('',(1.54373336646987E-15,-42.8201004838369,-234.90005));
#192915=CARTESIAN_POINT('',(296.501483394397,-43.270100483837,-235.35005));
#192916=CARTESIAN_POINT('Origin',(-30.425,-25.4138432731711,-234.90005));
#192917=CARTESIAN_POINT('',(-30.425,-33.96456093117,-235.35005));
#192918=CARTESIAN_POINT('',(-30.875,-33.96456093117,-234.90005));
#192919=CARTESIAN_POINT('Origin',(-30.425,-33.96456093117,-234.90005));
#192920=CARTESIAN_POINT('',(-30.425,-42.0701004838368,-235.35005));
#192921=CARTESIAN_POINT('',(-30.875,-33.96456093117,-234.90005));
#192922=CARTESIAN_POINT('Origin',(-36.0311576807678,-42.0701004838368,-234.90005));
#192923=CARTESIAN_POINT('',(-36.6030808185578,-42.5552849069797,-234.90005));
#192924=CARTESIAN_POINT('',(-36.9462347012318,-42.8463955608654,-235.35005));
#192925=CARTESIAN_POINT('Origin',(-36.9462347012318,-42.8463955608654,-234.90005));
#192926=CARTESIAN_POINT('Origin',(-36.0311576807678,-42.0701004838368,-234.90005));
#192927=CARTESIAN_POINT('Origin',(-36.0311576807678,-42.0701004838368,-235.35005));
#192928=CARTESIAN_POINT('Origin',(-31.625,-33.96456093117,-234.90005));
#192929=CARTESIAN_POINT('',(-31.625,-32.76456093117,-235.35005));
#192930=CARTESIAN_POINT('',(-31.625,-33.21456093117,-234.90005));
#192931=CARTESIAN_POINT('Origin',(-31.625,-32.76456093117,-234.90005));
#192932=CARTESIAN_POINT('Origin',(-31.625,-33.96456093117,-235.35005));
#192933=CARTESIAN_POINT('Origin',(-31.625,-33.96456093117,-234.90005));
#192934=CARTESIAN_POINT('Origin',(6.29739814579425E-15,-11.5034818258363,
-234.90005));
#192935=CARTESIAN_POINT('',(-39.8203148590358,-38.3053945286125,-234.90005));
#192936=CARTESIAN_POINT('',(-40.1936303108393,-38.5566624602009,-235.35005));
#192937=CARTESIAN_POINT('Origin',(-40.1936303108393,-38.5566624602009,-234.90005));
#192938=CARTESIAN_POINT('Origin',(6.29739814579425E-15,-11.5034818258363,
-234.90005));
#192939=CARTESIAN_POINT('Origin',(6.29739814579425E-15,-11.5034818258363,
-235.35005));
#192940=CARTESIAN_POINT('Origin',(296.501483394397,-32.7645609311699,-234.90005));
#192941=CARTESIAN_POINT('',(-39.3771239584772,-32.76456093117,-235.35005));
#192942=CARTESIAN_POINT('',(-39.3771239584772,-33.21456093117,-234.90005));
#192943=CARTESIAN_POINT('Origin',(-39.3771239584772,-32.76456093117,-234.90005));
#192944=CARTESIAN_POINT('',(296.501483394397,-32.7645609311699,-235.35005));
#192945=CARTESIAN_POINT('',(0.,-33.21456093117,-234.90005));
#192946=CARTESIAN_POINT('Origin',(-38.9907249661392,-37.7470213473046,-234.90005));
#192947=CARTESIAN_POINT('',(-39.989972084972,-37.7858181964606,-234.90005));
#192948=CARTESIAN_POINT('',(-40.4396332884467,-37.8032767785809,-235.35005));
#192949=CARTESIAN_POINT('Origin',(-40.4396332884467,-37.8032767785809,-234.90005));
#192950=CARTESIAN_POINT('Origin',(-38.9907249661392,-37.7470213473046,-234.90005));
#192951=CARTESIAN_POINT('Origin',(-38.9907249661392,-37.7470213473046,-235.35005));
#192952=CARTESIAN_POINT('Origin',(-39.3771239584772,-33.96456093117,-234.90005));
#192953=CARTESIAN_POINT('',(-40.5764627182082,-34.0043923183801,-235.35005));
#192954=CARTESIAN_POINT('',(-40.1267106833092,-33.9894555481763,-234.90005));
#192955=CARTESIAN_POINT('Origin',(-40.5764627182082,-34.0043923183801,-234.90005));
#192956=CARTESIAN_POINT('Origin',(-39.3771239584772,-33.96456093117,-235.35005));
#192957=CARTESIAN_POINT('Origin',(-39.3771239584772,-33.96456093117,-234.90005));
#192958=CARTESIAN_POINT('Origin',(636.934816028482,-11.5034818258361,-234.90005));
#192959=CARTESIAN_POINT('Origin',(636.934816028482,-11.5034818258361,-235.35005));
#192960=CARTESIAN_POINT('Origin',(636.934816028482,-11.5034818258361,-234.90005));
#192961=CARTESIAN_POINT('Origin',(-21.5,-42.0701004838368,-234.90005));
#192962=CARTESIAN_POINT('',(-20.3,-42.0701004838368,-235.35005));
#192963=CARTESIAN_POINT('',(-20.75,-42.0701004838368,-234.90005));
#192964=CARTESIAN_POINT('Origin',(-20.3,-42.0701004838368,-234.90005));
#192965=CARTESIAN_POINT('',(-21.5,-43.2701004838368,-235.35005));
#192966=CARTESIAN_POINT('Origin',(-21.5,-42.0701004838368,-235.35005));
#192967=CARTESIAN_POINT('',(-21.5,-42.8201004838368,-234.90005));
#192968=CARTESIAN_POINT('Origin',(-21.5,-43.2701004838368,-234.90005));
#192969=CARTESIAN_POINT('Origin',(-21.5,-42.0701004838368,-234.90005));
#192970=CARTESIAN_POINT('Origin',(296.501483394397,-43.270100483837,-234.90005));
#192971=CARTESIAN_POINT('',(-29.125,-42.8201004838368,-234.90005));
#192972=CARTESIAN_POINT('',(-29.125,-43.2701004838368,-235.35005));
#192973=CARTESIAN_POINT('Origin',(-29.125,-43.2701004838368,-234.90005));
#192974=CARTESIAN_POINT('',(1.54373336646987E-15,-42.8201004838369,-234.90005));
#192975=CARTESIAN_POINT('',(296.501483394397,-43.270100483837,-235.35005));
#192976=CARTESIAN_POINT('Origin',(-20.3,-25.4138432731711,-234.90005));
#192977=CARTESIAN_POINT('',(-20.3,-33.96456093117,-235.35005));
#192978=CARTESIAN_POINT('',(-20.75,-33.96456093117,-234.90005));
#192979=CARTESIAN_POINT('Origin',(-20.3,-33.96456093117,-234.90005));
#192980=CARTESIAN_POINT('',(-20.3,-42.0701004838368,-235.35005));
#192981=CARTESIAN_POINT('',(-20.75,-33.96456093117,-234.90005));
#192982=CARTESIAN_POINT('Origin',(-29.125,-42.0701004838368,-234.90005));
#192983=CARTESIAN_POINT('',(-29.875,-42.0701004838368,-234.90005));
#192984=CARTESIAN_POINT('',(-30.325,-42.0701004838368,-235.35005));
#192985=CARTESIAN_POINT('Origin',(-30.325,-42.0701004838368,-234.90005));
#192986=CARTESIAN_POINT('Origin',(-29.125,-42.0701004838368,-234.90005));
#192987=CARTESIAN_POINT('Origin',(-29.125,-42.0701004838368,-235.35005));
#192988=CARTESIAN_POINT('Origin',(-21.5,-33.96456093117,-234.90005));
#192989=CARTESIAN_POINT('',(-21.5,-32.76456093117,-235.35005));
#192990=CARTESIAN_POINT('',(-21.5,-33.21456093117,-234.90005));
#192991=CARTESIAN_POINT('Origin',(-21.5,-32.76456093117,-234.90005));
#192992=CARTESIAN_POINT('Origin',(-21.5,-33.96456093117,-235.35005));
#192993=CARTESIAN_POINT('Origin',(-21.5,-33.96456093117,-234.90005));
#192994=CARTESIAN_POINT('Origin',(-30.325,-25.4138432731711,-234.90005));
#192995=CARTESIAN_POINT('',(-29.875,-33.96456093117,-234.90005));
#192996=CARTESIAN_POINT('',(-30.325,-33.96456093117,-235.35005));
#192997=CARTESIAN_POINT('Origin',(-30.325,-33.96456093117,-234.90005));
#192998=CARTESIAN_POINT('',(-29.875,-42.0701004838368,-234.90005));
#192999=CARTESIAN_POINT('',(-30.325,-33.96456093117,-235.35005));
#193000=CARTESIAN_POINT('Origin',(296.501483394397,-32.7645609311699,-234.90005));
#193001=CARTESIAN_POINT('',(-29.125,-32.76456093117,-235.35005));
#193002=CARTESIAN_POINT('',(-29.125,-33.21456093117,-234.90005));
#193003=CARTESIAN_POINT('Origin',(-29.125,-32.76456093117,-234.90005));
#193004=CARTESIAN_POINT('',(296.501483394397,-32.7645609311699,-235.35005));
#193005=CARTESIAN_POINT('',(0.,-33.21456093117,-234.90005));
#193006=CARTESIAN_POINT('Origin',(-29.125,-33.96456093117,-234.90005));
#193007=CARTESIAN_POINT('Origin',(-29.125,-33.96456093117,-235.35005));
#193008=CARTESIAN_POINT('Origin',(-29.125,-33.96456093117,-234.90005));
#193009=CARTESIAN_POINT('Origin',(-29.125,-44.5701004838368,-234.90005));
#193010=CARTESIAN_POINT('',(-30.325,-44.5701004838368,-235.35005));
#193011=CARTESIAN_POINT('',(-29.875,-44.5701004838368,-234.90005));
#193012=CARTESIAN_POINT('Origin',(-30.325,-44.5701004838368,-234.90005));
#193013=CARTESIAN_POINT('',(-29.125,-43.3701004838369,-235.35005));
#193014=CARTESIAN_POINT('Origin',(-29.125,-44.5701004838368,-235.35005));
#193015=CARTESIAN_POINT('',(-29.125,-43.8201004838368,-234.90005));
#193016=CARTESIAN_POINT('Origin',(-29.125,-43.3701004838369,-234.90005));
#193017=CARTESIAN_POINT('Origin',(-29.125,-44.5701004838368,-234.90005));
#193018=CARTESIAN_POINT('Origin',(296.501483394397,-43.3701004838369,-234.90005));
#193019=CARTESIAN_POINT('',(-21.5,-43.8201004838368,-234.90005));
#193020=CARTESIAN_POINT('',(-21.5,-43.3701004838369,-235.35005));
#193021=CARTESIAN_POINT('Origin',(-21.5,-43.3701004838369,-234.90005));
#193022=CARTESIAN_POINT('',(1.23757166668304E-15,-43.8201004838368,-234.90005));
#193023=CARTESIAN_POINT('',(296.501483394397,-43.3701004838369,-235.35005));
#193024=CARTESIAN_POINT('Origin',(-30.325,-25.4138432731711,-234.90005));
#193025=CARTESIAN_POINT('',(-30.325,-48.7096221120845,-235.35005));
#193026=CARTESIAN_POINT('',(-29.875,-48.7096221120845,-234.90005));
#193027=CARTESIAN_POINT('Origin',(-30.325,-48.7096221120845,-234.90005));
#193028=CARTESIAN_POINT('',(-30.325,-44.5701004838368,-235.35005));
#193029=CARTESIAN_POINT('',(-29.875,-48.7096221120845,-234.90005));
#193030=CARTESIAN_POINT('Origin',(-21.5,-44.5701004838368,-234.90005));
#193031=CARTESIAN_POINT('',(-20.75,-44.5701004838368,-234.90005));
#193032=CARTESIAN_POINT('',(-20.3,-44.5701004838368,-235.35005));
#193033=CARTESIAN_POINT('Origin',(-20.3,-44.5701004838368,-234.90005));
#193034=CARTESIAN_POINT('Origin',(-21.5,-44.5701004838368,-234.90005));
#193035=CARTESIAN_POINT('Origin',(-21.5,-44.5701004838368,-235.35005));
#193036=CARTESIAN_POINT('Origin',(-29.125,-48.7096221120845,-234.90005));
#193037=CARTESIAN_POINT('',(-29.8646825396825,-49.6545399606241,-235.35005));
#193038=CARTESIAN_POINT('',(-29.5873015873016,-49.3001957674217,-234.90005));
#193039=CARTESIAN_POINT('Origin',(-29.8646825396825,-49.6545399606241,-234.90005));
#193040=CARTESIAN_POINT('Origin',(-29.125,-48.7096221120845,-235.35005));
#193041=CARTESIAN_POINT('Origin',(-29.125,-48.7096221120845,-234.90005));
#193042=CARTESIAN_POINT('Origin',(-20.3,-25.4138432731711,-234.90005));
#193043=CARTESIAN_POINT('',(-20.75,-52.8339989151841,-234.90005));
#193044=CARTESIAN_POINT('',(-20.3,-52.8339989151841,-235.35005));
#193045=CARTESIAN_POINT('Origin',(-20.3,-52.8339989151841,-234.90005));
#193046=CARTESIAN_POINT('',(-20.75,-44.5701004838368,-234.90005));
#193047=CARTESIAN_POINT('',(-20.3,-52.8339989151841,-235.35005));
#193048=CARTESIAN_POINT('Origin',(6.29739814579425E-15,-11.5034818258363,
-234.90005));
#193049=CARTESIAN_POINT('',(-23.6248477671233,-53.8032344017111,-235.35005));
#193050=CARTESIAN_POINT('',(-23.4054219364689,-53.410357442802,-234.90005));
#193051=CARTESIAN_POINT('Origin',(-23.6248477671233,-53.8032344017111,-234.90005));
#193052=CARTESIAN_POINT('Origin',(6.29739814579425E-15,-11.5034818258363,
-235.35005));
#193053=CARTESIAN_POINT('Origin',(6.29739814579425E-15,-11.5034818258363,
-234.90005));
#193054=CARTESIAN_POINT('Origin',(-21.5,-52.8339989151841,-234.90005));
#193055=CARTESIAN_POINT('',(-21.5238294101154,-53.5836202590729,-234.90005));
#193056=CARTESIAN_POINT('',(-21.5381270561845,-54.0333930654061,-235.35005));
#193057=CARTESIAN_POINT('Origin',(-21.5381270561845,-54.0333930654061,-234.90005));
#193058=CARTESIAN_POINT('Origin',(-21.5,-52.8339989151841,-234.90005));
#193059=CARTESIAN_POINT('Origin',(-21.5,-52.8339989151841,-235.35005));
#193060=CARTESIAN_POINT('Origin',(-22.9178089794592,-52.5372975341153,-234.90005));
#193061=CARTESIAN_POINT('',(-22.9669354026308,-53.9864650863833,-235.35005));
#193062=CARTESIAN_POINT('',(-22.9516892713016,-53.5367234322311,-234.90005));
#193063=CARTESIAN_POINT('Origin',(-22.9669354026308,-53.9864650863833,-234.90005));
#193064=CARTESIAN_POINT('Origin',(-22.9178089794592,-52.5372975341153,-235.35005));
#193065=CARTESIAN_POINT('Origin',(-22.9178089794592,-52.5372975341153,-234.90005));
#193066=CARTESIAN_POINT('Origin',(-7.14692237356698E-14,623.509175991979,
-234.90005));
#193067=CARTESIAN_POINT('Origin',(-7.14692237356698E-14,623.509175991979,
-235.35005));
#193068=CARTESIAN_POINT('Origin',(-7.14692237356698E-14,623.509175991979,
-234.90005));
#193069=CARTESIAN_POINT('Origin',(-19.,-44.5701004838368,-234.90005));
#193070=CARTESIAN_POINT('',(-20.2,-44.5701004838368,-235.35005));
#193071=CARTESIAN_POINT('',(-19.75,-44.5701004838368,-234.90005));
#193072=CARTESIAN_POINT('Origin',(-20.2,-44.5701004838368,-234.90005));
#193073=CARTESIAN_POINT('',(-19.,-43.3701004838369,-235.35005));
#193074=CARTESIAN_POINT('Origin',(-19.,-44.5701004838368,-235.35005));
#193075=CARTESIAN_POINT('',(-19.,-43.8201004838368,-234.90005));
#193076=CARTESIAN_POINT('Origin',(-19.,-43.3701004838369,-234.90005));
#193077=CARTESIAN_POINT('Origin',(-19.,-44.5701004838368,-234.90005));
#193078=CARTESIAN_POINT('Origin',(296.501483394397,-43.3701004838369,-234.90005));
#193079=CARTESIAN_POINT('',(-11.3749999999999,-43.8201004838368,-234.90005));
#193080=CARTESIAN_POINT('',(-11.3749999999999,-43.3701004838369,-235.35005));
#193081=CARTESIAN_POINT('Origin',(-11.3749999999999,-43.3701004838369,-234.90005));
#193082=CARTESIAN_POINT('',(1.23757166668304E-15,-43.8201004838368,-234.90005));
#193083=CARTESIAN_POINT('',(296.501483394397,-43.3701004838369,-235.35005));
#193084=CARTESIAN_POINT('Origin',(-20.2,-25.4138432731711,-234.90005));
#193085=CARTESIAN_POINT('',(-20.2,-52.9088458284789,-235.35005));
#193086=CARTESIAN_POINT('',(-19.75,-52.9088458284789,-234.90005));
#193087=CARTESIAN_POINT('Origin',(-20.2,-52.9088458284789,-234.90005));
#193088=CARTESIAN_POINT('',(-20.2,-44.5701004838368,-235.35005));
#193089=CARTESIAN_POINT('',(-19.75,-52.9088458284789,-234.90005));
#193090=CARTESIAN_POINT('Origin',(-11.3749999999999,-44.5701004838369,-234.90005));
#193091=CARTESIAN_POINT('',(-10.6249999999999,-44.5701004838369,-234.90005));
#193092=CARTESIAN_POINT('',(-10.1749999999999,-44.5701004838369,-235.35005));
#193093=CARTESIAN_POINT('Origin',(-10.1749999999999,-44.5701004838369,-234.90005));
#193094=CARTESIAN_POINT('Origin',(-11.3749999999999,-44.5701004838369,-234.90005));
#193095=CARTESIAN_POINT('Origin',(-11.3749999999999,-44.5701004838369,-235.35005));
#193096=CARTESIAN_POINT('Origin',(-19.,-52.9088458284789,-234.90005));
#193097=CARTESIAN_POINT('',(-19.0336936775584,-54.1083727085831,-235.35005));
#193098=CARTESIAN_POINT('',(-19.021058548474,-53.6585501285442,-234.90005));
#193099=CARTESIAN_POINT('Origin',(-19.0336936775584,-54.1083727085831,-234.90005));
#193100=CARTESIAN_POINT('Origin',(-19.,-52.9088458284789,-235.35005));
#193101=CARTESIAN_POINT('Origin',(-19.,-52.9088458284789,-234.90005));
#193102=CARTESIAN_POINT('Origin',(-10.1749999999999,-25.4138432731711,-234.90005));
#193103=CARTESIAN_POINT('',(-10.6249999999999,-53.08002700974,-234.90005));
#193104=CARTESIAN_POINT('',(-10.1749999999999,-53.08002700974,-235.35005));
#193105=CARTESIAN_POINT('Origin',(-10.1749999999999,-53.08002700974,-234.90005));
#193106=CARTESIAN_POINT('',(-10.6249999999999,-44.5701004838369,-234.90005));
#193107=CARTESIAN_POINT('',(-10.1749999999999,-53.08002700974,-235.35005));
#193108=CARTESIAN_POINT('Origin',(-7.14692237356698E-14,623.509175991979,
-234.90005));
#193109=CARTESIAN_POINT('',(-11.3951718727487,-54.2798574542403,-235.35005));
#193110=CARTESIAN_POINT('',(-11.3876074204679,-53.8299210375529,-234.90005));
#193111=CARTESIAN_POINT('Origin',(-11.3951718727487,-54.2798574542403,-234.90005));
#193112=CARTESIAN_POINT('Origin',(-7.14692237356698E-14,623.509175991979,
-235.35005));
#193113=CARTESIAN_POINT('Origin',(-7.14692237356698E-14,623.509175991979,
-234.90005));
#193114=CARTESIAN_POINT('Origin',(-11.3749999999999,-53.08002700974,-234.90005));
#193115=CARTESIAN_POINT('Origin',(-11.3749999999999,-53.08002700974,-235.35005));
#193116=CARTESIAN_POINT('Origin',(-11.3749999999999,-53.08002700974,-234.90005));
#193117=CARTESIAN_POINT('Origin',(-11.3749999999999,-42.0701004838369,-234.90005));
#193118=CARTESIAN_POINT('',(-10.1749999999999,-42.0701004838368,-235.35005));
#193119=CARTESIAN_POINT('',(-10.6249999999999,-42.0701004838368,-234.90005));
#193120=CARTESIAN_POINT('Origin',(-10.1749999999999,-42.0701004838368,-234.90005));
#193121=CARTESIAN_POINT('',(-11.3749999999999,-43.2701004838368,-235.35005));
#193122=CARTESIAN_POINT('Origin',(-11.3749999999999,-42.0701004838369,-235.35005));
#193123=CARTESIAN_POINT('',(-11.3749999999999,-42.8201004838369,-234.90005));
#193124=CARTESIAN_POINT('Origin',(-11.3749999999999,-43.2701004838368,-234.90005));
#193125=CARTESIAN_POINT('Origin',(-11.3749999999999,-42.0701004838369,-234.90005));
#193126=CARTESIAN_POINT('Origin',(296.501483394397,-43.270100483837,-234.90005));
#193127=CARTESIAN_POINT('',(-19.,-42.8201004838368,-234.90005));
#193128=CARTESIAN_POINT('',(-19.,-43.2701004838368,-235.35005));
#193129=CARTESIAN_POINT('Origin',(-19.,-43.2701004838368,-234.90005));
#193130=CARTESIAN_POINT('',(1.54373336646987E-15,-42.8201004838369,-234.90005));
#193131=CARTESIAN_POINT('',(296.501483394397,-43.270100483837,-235.35005));
#193132=CARTESIAN_POINT('Origin',(-10.1749999999999,-25.4138432731711,-234.90005));
#193133=CARTESIAN_POINT('',(-10.1749999999999,-33.96456093117,-235.35005));
#193134=CARTESIAN_POINT('',(-10.6249999999999,-33.96456093117,-234.90005));
#193135=CARTESIAN_POINT('Origin',(-10.1749999999999,-33.96456093117,-234.90005));
#193136=CARTESIAN_POINT('',(-10.1749999999999,-42.0701004838368,-235.35005));
#193137=CARTESIAN_POINT('',(-10.6249999999999,-33.96456093117,-234.90005));
#193138=CARTESIAN_POINT('Origin',(-19.,-42.0701004838368,-234.90005));
#193139=CARTESIAN_POINT('',(-19.75,-42.0701004838368,-234.90005));
#193140=CARTESIAN_POINT('',(-20.2,-42.0701004838368,-235.35005));
#193141=CARTESIAN_POINT('Origin',(-20.2,-42.0701004838368,-234.90005));
#193142=CARTESIAN_POINT('Origin',(-19.,-42.0701004838368,-234.90005));
#193143=CARTESIAN_POINT('Origin',(-19.,-42.0701004838368,-235.35005));
#193144=CARTESIAN_POINT('Origin',(-11.3749999999999,-33.96456093117,-234.90005));
#193145=CARTESIAN_POINT('',(-11.3749999999999,-32.76456093117,-235.35005));
#193146=CARTESIAN_POINT('',(-11.3749999999999,-33.21456093117,-234.90005));
#193147=CARTESIAN_POINT('Origin',(-11.3749999999999,-32.76456093117,-234.90005));
#193148=CARTESIAN_POINT('Origin',(-11.3749999999999,-33.96456093117,-235.35005));
#193149=CARTESIAN_POINT('Origin',(-11.3749999999999,-33.96456093117,-234.90005));
#193150=CARTESIAN_POINT('Origin',(-20.2,-25.4138432731711,-234.90005));
#193151=CARTESIAN_POINT('',(-19.75,-33.96456093117,-234.90005));
#193152=CARTESIAN_POINT('',(-20.2,-33.96456093117,-235.35005));
#193153=CARTESIAN_POINT('Origin',(-20.2,-33.96456093117,-234.90005));
#193154=CARTESIAN_POINT('',(-19.75,-42.0701004838368,-234.90005));
#193155=CARTESIAN_POINT('',(-20.2,-33.96456093117,-235.35005));
#193156=CARTESIAN_POINT('Origin',(296.501483394397,-32.7645609311699,-234.90005));
#193157=CARTESIAN_POINT('',(-19.,-32.76456093117,-235.35005));
#193158=CARTESIAN_POINT('',(-19.,-33.21456093117,-234.90005));
#193159=CARTESIAN_POINT('Origin',(-19.,-32.76456093117,-234.90005));
#193160=CARTESIAN_POINT('',(296.501483394397,-32.7645609311699,-235.35005));
#193161=CARTESIAN_POINT('',(0.,-33.21456093117,-234.90005));
#193162=CARTESIAN_POINT('Origin',(-19.,-33.96456093117,-234.90005));
#193163=CARTESIAN_POINT('Origin',(-19.,-33.96456093117,-235.35005));
#193164=CARTESIAN_POINT('Origin',(-19.,-33.96456093117,-234.90005));
#193165=CARTESIAN_POINT('Origin',(-8.87499999999984,-44.5701004838369,-234.90005));
#193166=CARTESIAN_POINT('',(-10.075,-44.5701004838369,-235.35005));
#193167=CARTESIAN_POINT('',(-9.62499999999984,-44.5701004838369,-234.90005));
#193168=CARTESIAN_POINT('Origin',(-10.075,-44.5701004838369,-234.90005));
#193169=CARTESIAN_POINT('',(-8.87499999999984,-43.3701004838369,-235.35005));
#193170=CARTESIAN_POINT('Origin',(-8.87499999999984,-44.5701004838369,-235.35005));
#193171=CARTESIAN_POINT('',(-8.87499999999984,-43.8201004838368,-234.90005));
#193172=CARTESIAN_POINT('Origin',(-8.87499999999984,-43.3701004838369,-234.90005));
#193173=CARTESIAN_POINT('Origin',(-8.87499999999984,-44.5701004838369,-234.90005));
#193174=CARTESIAN_POINT('Origin',(296.501483394397,-43.3701004838369,-234.90005));
#193175=CARTESIAN_POINT('',(-1.25,-43.8201004838368,-234.90005));
#193176=CARTESIAN_POINT('',(-1.25,-43.3701004838369,-235.35005));
#193177=CARTESIAN_POINT('Origin',(-1.25,-43.3701004838369,-234.90005));
#193178=CARTESIAN_POINT('',(1.23757166668304E-15,-43.8201004838368,-234.90005));
#193179=CARTESIAN_POINT('',(296.501483394397,-43.3701004838369,-235.35005));
#193180=CARTESIAN_POINT('Origin',(-10.075,-25.4138432731712,-234.90005));
#193181=CARTESIAN_POINT('',(-10.0749999999998,-53.1174378937751,-235.35005));
#193182=CARTESIAN_POINT('',(-9.62499999999984,-53.1174378937751,-234.90005));
#193183=CARTESIAN_POINT('Origin',(-10.0749999999998,-53.1174378937751,-234.90005));
#193184=CARTESIAN_POINT('',(-10.075,-44.5701004838369,-235.35005));
#193185=CARTESIAN_POINT('',(-9.62499999999984,-53.1174378937751,-234.90005));
#193186=CARTESIAN_POINT('Origin',(-1.25,-44.5701004838369,-234.90005));
#193187=CARTESIAN_POINT('',(-0.5,-44.5701004838369,-234.90005));
#193188=CARTESIAN_POINT('',(-0.0499999999999953,-44.5701004838369,-235.35005));
#193189=CARTESIAN_POINT('Origin',(-0.0499999999999955,-44.5701004838369,
-234.90005));
#193190=CARTESIAN_POINT('Origin',(-1.25,-44.5701004838369,-234.90005));
#193191=CARTESIAN_POINT('Origin',(-1.25,-44.5701004838369,-235.35005));
#193192=CARTESIAN_POINT('Origin',(-8.87499999999984,-53.1174378937751,-234.90005));
#193193=CARTESIAN_POINT('',(-8.89073849412256,-54.3173346809209,-235.35005));
#193194=CARTESIAN_POINT('',(-8.88483655882654,-53.8673733857413,-234.90005));
#193195=CARTESIAN_POINT('Origin',(-8.89073849412256,-54.3173346809209,-234.90005));
#193196=CARTESIAN_POINT('Origin',(-8.87499999999984,-53.1174378937751,-235.35005));
#193197=CARTESIAN_POINT('Origin',(-8.87499999999984,-53.1174378937751,-234.90005));
#193198=CARTESIAN_POINT('Origin',(-0.0499999999999945,-25.4138432731711,
-234.90005));
#193199=CARTESIAN_POINT('',(-0.5,-53.1744855098348,-234.90005));
#193200=CARTESIAN_POINT('',(-0.0499999999999928,-53.1744855098348,-235.35005));
#193201=CARTESIAN_POINT('Origin',(-0.049999999999995,-53.1744855098348,
-234.90005));
#193202=CARTESIAN_POINT('',(-0.5,-44.5701004838369,-234.90005));
#193203=CARTESIAN_POINT('',(-0.0499999999999928,-53.1744855098348,-235.35005));
#193204=CARTESIAN_POINT('Origin',(-7.14692237356698E-14,623.509175991979,
-234.90005));
#193205=CARTESIAN_POINT('',(-1.25221668931305,-54.3744834624533,-235.35005));
#193206=CARTESIAN_POINT('',(-1.25138543082066,-53.9244842302215,-234.90005));
#193207=CARTESIAN_POINT('Origin',(-1.25221668931305,-54.3744834624533,-234.90005));
#193208=CARTESIAN_POINT('Origin',(-7.14692237356698E-14,623.509175991979,
-235.35005));
#193209=CARTESIAN_POINT('Origin',(-7.14692237356698E-14,623.509175991979,
-234.90005));
#193210=CARTESIAN_POINT('Origin',(-1.25,-53.1744855098348,-234.90005));
#193211=CARTESIAN_POINT('Origin',(-1.25,-53.1744855098348,-235.35005));
#193212=CARTESIAN_POINT('Origin',(-1.25,-53.1744855098348,-234.90005));
#193213=CARTESIAN_POINT('Origin',(-1.25,-42.0701004838369,-234.90005));
#193214=CARTESIAN_POINT('',(-0.0499999999999935,-42.0701004838369,-235.35005));
#193215=CARTESIAN_POINT('',(-0.5,-42.0701004838369,-234.90005));
#193216=CARTESIAN_POINT('Origin',(-0.0499999999999935,-42.0701004838369,
-234.90005));
#193217=CARTESIAN_POINT('',(-1.25,-43.2701004838368,-235.35005));
#193218=CARTESIAN_POINT('Origin',(-1.25,-42.0701004838369,-235.35005));
#193219=CARTESIAN_POINT('',(-1.25,-42.8201004838369,-234.90005));
#193220=CARTESIAN_POINT('Origin',(-1.25,-43.2701004838368,-234.90005));
#193221=CARTESIAN_POINT('Origin',(-1.25,-42.0701004838369,-234.90005));
#193222=CARTESIAN_POINT('Origin',(296.501483394397,-43.270100483837,-234.90005));
#193223=CARTESIAN_POINT('',(-8.87499999999984,-42.8201004838369,-234.90005));
#193224=CARTESIAN_POINT('',(-8.87499999999984,-43.2701004838368,-235.35005));
#193225=CARTESIAN_POINT('Origin',(-8.87499999999984,-43.2701004838368,-234.90005));
#193226=CARTESIAN_POINT('',(1.54373336646987E-15,-42.8201004838369,-234.90005));
#193227=CARTESIAN_POINT('',(296.501483394397,-43.270100483837,-235.35005));
#193228=CARTESIAN_POINT('Origin',(-0.0499999999999945,-25.4138432731711,
-234.90005));
#193229=CARTESIAN_POINT('',(-0.0499999999999959,-33.96456093117,-235.35005));
#193230=CARTESIAN_POINT('',(-0.5,-33.96456093117,-234.90005));
#193231=CARTESIAN_POINT('Origin',(-0.0499999999999959,-33.96456093117,-234.90005));
#193232=CARTESIAN_POINT('',(-0.0499999999999935,-42.0701004838369,-235.35005));
#193233=CARTESIAN_POINT('',(-0.5,-33.96456093117,-234.90005));
#193234=CARTESIAN_POINT('Origin',(-8.87499999999984,-42.0701004838369,-234.90005));
#193235=CARTESIAN_POINT('',(-9.62499999999984,-42.0701004838368,-234.90005));
#193236=CARTESIAN_POINT('',(-10.0749999999998,-42.0701004838368,-235.35005));
#193237=CARTESIAN_POINT('Origin',(-10.0749999999998,-42.0701004838368,-234.90005));
#193238=CARTESIAN_POINT('Origin',(-8.87499999999984,-42.0701004838369,-234.90005));
#193239=CARTESIAN_POINT('Origin',(-8.87499999999984,-42.0701004838369,-235.35005));
#193240=CARTESIAN_POINT('Origin',(-1.25,-33.96456093117,-234.90005));
#193241=CARTESIAN_POINT('',(-1.25,-32.76456093117,-235.35005));
#193242=CARTESIAN_POINT('',(-1.25,-33.21456093117,-234.90005));
#193243=CARTESIAN_POINT('Origin',(-1.25,-32.76456093117,-234.90005));
#193244=CARTESIAN_POINT('Origin',(-1.25,-33.96456093117,-235.35005));
#193245=CARTESIAN_POINT('Origin',(-1.25,-33.96456093117,-234.90005));
#193246=CARTESIAN_POINT('Origin',(-10.075,-25.4138432731712,-234.90005));
#193247=CARTESIAN_POINT('',(-9.62499999999984,-33.96456093117,-234.90005));
#193248=CARTESIAN_POINT('',(-10.075,-33.96456093117,-235.35005));
#193249=CARTESIAN_POINT('Origin',(-10.0749999999998,-33.96456093117,-234.90005));
#193250=CARTESIAN_POINT('',(-9.62499999999984,-42.0701004838368,-234.90005));
#193251=CARTESIAN_POINT('',(-10.075,-33.96456093117,-235.35005));
#193252=CARTESIAN_POINT('Origin',(296.501483394397,-32.7645609311699,-234.90005));
#193253=CARTESIAN_POINT('',(-8.87499999999984,-32.76456093117,-235.35005));
#193254=CARTESIAN_POINT('',(-8.87499999999984,-33.21456093117,-234.90005));
#193255=CARTESIAN_POINT('Origin',(-8.87499999999984,-32.76456093117,-234.90005));
#193256=CARTESIAN_POINT('',(296.501483394397,-32.7645609311699,-235.35005));
#193257=CARTESIAN_POINT('',(0.,-33.21456093117,-234.90005));
#193258=CARTESIAN_POINT('Origin',(-8.87499999999984,-33.96456093117,-234.90005));
#193259=CARTESIAN_POINT('Origin',(-8.87499999999984,-33.96456093117,-235.35005));
#193260=CARTESIAN_POINT('Origin',(-8.87499999999984,-33.96456093117,-234.90005));
#193261=CARTESIAN_POINT('Origin',(-33.7514626427707,-44.5701004838368,-234.90005));
#193262=CARTESIAN_POINT('',(-34.6086426463967,-45.4098876243575,-235.35005));
#193263=CARTESIAN_POINT('',(-34.2872001450369,-45.0949674466622,-234.90005));
#193264=CARTESIAN_POINT('Origin',(-34.6086426463967,-45.4098876243575,-234.90005));
#193265=CARTESIAN_POINT('',(-33.7514626427707,-43.3701004838369,-235.35005));
#193266=CARTESIAN_POINT('Origin',(-33.7514626427707,-44.5701004838368,-235.35005));
#193267=CARTESIAN_POINT('',(-33.7514626427707,-43.8201004838368,-234.90005));
#193268=CARTESIAN_POINT('Origin',(-33.7514626427707,-43.3701004838369,-234.90005));
#193269=CARTESIAN_POINT('Origin',(-33.7514626427707,-44.5701004838368,-234.90005));
#193270=CARTESIAN_POINT('Origin',(296.501483394397,-43.3701004838369,-234.90005));
#193271=CARTESIAN_POINT('',(-31.625,-43.8201004838368,-234.90005));
#193272=CARTESIAN_POINT('',(-31.625,-43.3701004838369,-235.35005));
#193273=CARTESIAN_POINT('Origin',(-31.625,-43.3701004838369,-234.90005));
#193274=CARTESIAN_POINT('',(1.23757166668304E-15,-43.8201004838368,-234.90005));
#193275=CARTESIAN_POINT('',(296.501483394397,-43.3701004838369,-235.35005));
#193276=CARTESIAN_POINT('Origin',(6.29739814579425E-15,-11.5034818258363,
-234.90005));
#193277=CARTESIAN_POINT('',(-32.4281746031746,-47.5009260671432,-235.35005));
#193278=CARTESIAN_POINT('',(-32.1269841269841,-47.1665844797626,-234.90005));
#193279=CARTESIAN_POINT('Origin',(-32.4281746031746,-47.5009260671432,-234.90005));
#193280=CARTESIAN_POINT('Origin',(6.29739814579425E-15,-11.5034818258363,
-235.35005));
#193281=CARTESIAN_POINT('Origin',(6.29739814579425E-15,-11.5034818258363,
-234.90005));
#193282=CARTESIAN_POINT('Origin',(-31.625,-44.5701004838368,-234.90005));
#193283=CARTESIAN_POINT('',(-30.875,-44.5701004838368,-234.90005));
#193284=CARTESIAN_POINT('',(-30.425,-44.5701004838368,-235.35005));
#193285=CARTESIAN_POINT('Origin',(-30.425,-44.5701004838368,-234.90005));
#193286=CARTESIAN_POINT('Origin',(-31.625,-44.5701004838368,-234.90005));
#193287=CARTESIAN_POINT('Origin',(-31.625,-44.5701004838368,-235.35005));
#193288=CARTESIAN_POINT('Origin',(-31.625,-46.609348500795,-234.90005));
#193289=CARTESIAN_POINT('',(-30.425,-46.609348500795,-235.35005));
#193290=CARTESIAN_POINT('',(-30.875,-46.609348500795,-234.90005));
#193291=CARTESIAN_POINT('Origin',(-30.425,-46.609348500795,-234.90005));
#193292=CARTESIAN_POINT('Origin',(-31.625,-46.609348500795,-235.35005));
#193293=CARTESIAN_POINT('Origin',(-31.625,-46.609348500795,-234.90005));
#193294=CARTESIAN_POINT('Origin',(-30.425,-25.4138432731711,-234.90005));
#193295=CARTESIAN_POINT('',(-30.425,-46.609348500795,-235.35005));
#193296=CARTESIAN_POINT('',(-30.875,-44.5701004838368,-234.90005));
#193297=CARTESIAN_POINT('Origin',(-31.625,23.6023848491226,-234.90005));
#193298=CARTESIAN_POINT('',(-32.4281746031746,24.4939624154707,-235.35005));
#193299=CARTESIAN_POINT('',(-30.425,23.6023848491226,-235.35005));
#193300=CARTESIAN_POINT('Origin',(-31.625,23.6023848491226,-235.35005));
#193301=CARTESIAN_POINT('',(-30.875,23.6023848491226,-234.90005));
#193302=CARTESIAN_POINT('Origin',(-30.425,23.6023848491226,-234.90005));
#193303=CARTESIAN_POINT('',(-32.1269841269841,24.1596208280901,-234.90005));
#193304=CARTESIAN_POINT('Origin',(-31.625,23.6023848491226,-234.90005));
#193305=CARTESIAN_POINT('Origin',(-32.4281746031746,24.4939624154707,-234.90005));
#193306=CARTESIAN_POINT('Origin',(-30.425,-25.4138432731711,-234.90005));
#193307=CARTESIAN_POINT('',(-30.875,21.5631368321642,-234.90005));
#193308=CARTESIAN_POINT('',(-30.425,21.5631368321642,-235.35005));
#193309=CARTESIAN_POINT('Origin',(-30.425,21.5631368321642,-234.90005));
#193310=CARTESIAN_POINT('',(-30.875,23.6023848491225,-234.90005));
#193311=CARTESIAN_POINT('',(-30.425,21.5631368321642,-235.35005));
#193312=CARTESIAN_POINT('Origin',(6.29739814579425E-15,-11.5034818258363,
-234.90005));
#193313=CARTESIAN_POINT('',(-34.6086426463969,22.4029239726848,-235.35005));
#193314=CARTESIAN_POINT('',(-34.2872001450371,22.0880037949896,-234.90005));
#193315=CARTESIAN_POINT('Origin',(-34.6086426463969,22.4029239726848,-234.90005));
#193316=CARTESIAN_POINT('Origin',(6.29739814579425E-15,-11.5034818258363,
-235.35005));
#193317=CARTESIAN_POINT('Origin',(6.29739814579425E-15,-11.5034818258363,
-234.90005));
#193318=CARTESIAN_POINT('Origin',(-31.625,21.5631368321642,-234.90005));
#193319=CARTESIAN_POINT('',(-31.625,20.8131368321642,-234.90005));
#193320=CARTESIAN_POINT('',(-31.625,20.3631368321642,-235.35005));
#193321=CARTESIAN_POINT('Origin',(-31.625,20.3631368321642,-234.90005));
#193322=CARTESIAN_POINT('Origin',(-31.625,21.5631368321642,-234.90005));
#193323=CARTESIAN_POINT('Origin',(-31.625,21.5631368321642,-235.35005));
#193324=CARTESIAN_POINT('Origin',(-33.751462642771,21.5631368321642,-234.90005));
#193325=CARTESIAN_POINT('',(-33.751462642771,20.3631368321642,-235.35005));
#193326=CARTESIAN_POINT('',(-33.751462642771,20.8131368321642,-234.90005));
#193327=CARTESIAN_POINT('Origin',(-33.751462642771,20.3631368321642,-234.90005));
#193328=CARTESIAN_POINT('Origin',(-33.751462642771,21.5631368321642,-235.35005));
#193329=CARTESIAN_POINT('Origin',(-33.751462642771,21.5631368321642,-234.90005));
#193330=CARTESIAN_POINT('Origin',(296.501483394397,20.3631368321642,-234.90005));
#193331=CARTESIAN_POINT('',(296.501483394397,20.3631368321642,-235.35005));
#193332=CARTESIAN_POINT('',(1.23757166668304E-15,20.8131368321642,-234.90005));
#193333=CARTESIAN_POINT('Origin',(-22.9178089794592,-52.5372975341153,-234.90005));
#193334=CARTESIAN_POINT('',(-25.8434867215177,-57.775656986236,-234.90005));
#193335=CARTESIAN_POINT('',(-26.0629125521721,-58.168533945145,-235.35005));
#193336=CARTESIAN_POINT('Origin',(-26.0629125521721,-58.168533945145,-234.90005));
#193337=CARTESIAN_POINT('',(-23.121090730514,-58.5338529228103,-234.90005));
#193338=CARTESIAN_POINT('Origin',(-22.9178089794592,-52.5372975341153,-234.90005));
#193339=CARTESIAN_POINT('',(-23.1363368618431,-58.9835945769624,-235.35005));
#193340=CARTESIAN_POINT('Origin',(-23.1363368618431,-58.9835945769624,-234.90005));
#193341=CARTESIAN_POINT('Origin',(-22.9178089794592,-52.5372975341153,-235.35005));
#193342=CARTESIAN_POINT('Origin',(6.29739814579425E-15,-11.5034818258363,
-234.90005));
#193343=CARTESIAN_POINT('',(-43.9682643235187,-41.0972604351516,-234.90005));
#193344=CARTESIAN_POINT('',(-44.3415797753222,-41.3485283667401,-235.35005));
#193345=CARTESIAN_POINT('Origin',(-44.3415797753222,-41.3485283667401,-234.90005));
#193346=CARTESIAN_POINT('Origin',(6.29739814579425E-15,-11.5034818258363,
-234.90005));
#193347=CARTESIAN_POINT('Origin',(6.29739814579425E-15,-11.5034818258363,
-235.35005));
#193348=CARTESIAN_POINT('Origin',(-38.9907249661392,-37.7470213473046,-234.90005));
#193349=CARTESIAN_POINT('',(-44.9862076791357,-37.9798024422418,-234.90005));
#193350=CARTESIAN_POINT('',(-45.4358688826104,-37.9972610243621,-235.35005));
#193351=CARTESIAN_POINT('Origin',(-45.4358688826105,-37.9972610243621,-234.90005));
#193352=CARTESIAN_POINT('Origin',(-38.9907249661392,-37.7470213473046,-234.90005));
#193353=CARTESIAN_POINT('Origin',(-38.9907249661392,-37.7470213473046,-235.35005));
#193354=CARTESIAN_POINT('Origin',(636.934816028482,-11.5034818258361,-234.90005));
#193355=CARTESIAN_POINT('',(-44.9862076791357,14.9728387905693,-234.90005));
#193356=CARTESIAN_POINT('',(-45.4358688826104,14.9902973726896,-235.35005));
#193357=CARTESIAN_POINT('Origin',(-45.4358688826104,14.9902973726896,-234.90005));
#193358=CARTESIAN_POINT('Origin',(636.934816028482,-11.5034818258361,-234.90005));
#193359=CARTESIAN_POINT('Origin',(636.934816028482,-11.5034818258361,-235.35005));
#193360=CARTESIAN_POINT('Origin',(-38.9907249661392,14.740057695632,-234.90005));
#193361=CARTESIAN_POINT('',(-43.9682643235187,18.0902967834791,-234.90005));
#193362=CARTESIAN_POINT('',(-44.3415797753222,18.3415647150676,-235.35005));
#193363=CARTESIAN_POINT('Origin',(-44.3415797753222,18.3415647150676,-234.90005));
#193364=CARTESIAN_POINT('Origin',(-38.9907249661392,14.740057695632,-234.90005));
#193365=CARTESIAN_POINT('Origin',(-38.9907249661392,14.740057695632,-235.35005));
#193366=CARTESIAN_POINT('Origin',(6.29739814579425E-15,-11.5034818258363,
-234.90005));
#193367=CARTESIAN_POINT('',(-28.0091475455229,33.4908250781833,-234.90005));
#193368=CARTESIAN_POINT('',(-28.2469610624189,33.872852212274,-235.35005));
#193369=CARTESIAN_POINT('Origin',(-28.2469610624189,33.872852212274,-234.90005));
#193370=CARTESIAN_POINT('Origin',(6.29739814579425E-15,-11.5034818258363,
-234.90005));
#193371=CARTESIAN_POINT('Origin',(6.29739814579425E-15,-11.5034818258363,
-235.35005));
#193372=CARTESIAN_POINT('Origin',(-24.838300653577,28.3971299569735,-234.90005));
#193373=CARTESIAN_POINT('',(-25.5706493501227,34.3522676872588,-234.90005));
#193374=CARTESIAN_POINT('',(-25.6255755023637,34.7989030170302,-235.35005));
#193375=CARTESIAN_POINT('Origin',(-25.6255755023637,34.7989030170302,-234.90005));
#193376=CARTESIAN_POINT('Origin',(-24.838300653577,28.3971299569735,-234.90005));
#193377=CARTESIAN_POINT('Origin',(-24.838300653577,28.3971299569735,-235.35005));
#193378=CARTESIAN_POINT('Origin',(-22.9178089794592,-52.5372975341153,-234.90005));
#193379=CARTESIAN_POINT('',(-25.0389253424516,-56.3351081369028,-235.35005));
#193380=CARTESIAN_POINT('',(-25.258351173106,-56.7279850958119,-234.90005));
#193381=CARTESIAN_POINT('Origin',(-25.0389253424516,-56.3351081369028,-234.90005));
#193382=CARTESIAN_POINT('',(-23.0651882489741,-56.8848001909192,-235.35005));
#193383=CARTESIAN_POINT('Origin',(-22.9178089794592,-52.5372975341153,-235.35005));
#193384=CARTESIAN_POINT('',(-23.0804343803032,-57.3345418450714,-234.90005));
#193385=CARTESIAN_POINT('Origin',(-23.0651882489741,-56.8848001909192,-234.90005));
#193386=CARTESIAN_POINT('Origin',(-22.9178089794592,-52.5372975341153,-234.90005));
#193387=CARTESIAN_POINT('Origin',(6.29739814579425E-15,-11.5034818258363,
-234.90005));
#193388=CARTESIAN_POINT('',(-42.5994410002394,-40.1759446859937,-235.35005));
#193389=CARTESIAN_POINT('',(-42.9727564520428,-40.4272126175822,-234.90005));
#193390=CARTESIAN_POINT('Origin',(-42.5994410002394,-40.1759446859937,-234.90005));
#193391=CARTESIAN_POINT('Origin',(6.29739814579425E-15,-11.5034818258363,
-235.35005));
#193392=CARTESIAN_POINT('Origin',(6.29739814579425E-15,-11.5034818258363,
-234.90005));
#193393=CARTESIAN_POINT('Origin',(-38.9907249661392,-37.7470213473046,-234.90005));
#193394=CARTESIAN_POINT('',(-43.3374499330618,-37.915787641134,-235.35005));
#193395=CARTESIAN_POINT('',(-43.7871111365364,-37.9332462232544,-234.90005));
#193396=CARTESIAN_POINT('Origin',(-43.3374499330618,-37.915787641134,-234.90005));
#193397=CARTESIAN_POINT('Origin',(-38.9907249661392,-37.7470213473046,-235.35005));
#193398=CARTESIAN_POINT('Origin',(-38.9907249661392,-37.7470213473046,-234.90005));
#193399=CARTESIAN_POINT('Origin',(636.934816028482,-11.5034818258361,-234.90005));
#193400=CARTESIAN_POINT('',(-43.3374499330618,14.9088239894616,-235.35005));
#193401=CARTESIAN_POINT('',(-43.7871111365364,14.9262825715819,-234.90005));
#193402=CARTESIAN_POINT('Origin',(-43.3374499330618,14.9088239894616,-234.90005));
#193403=CARTESIAN_POINT('Origin',(636.934816028482,-11.5034818258361,-235.35005));
#193404=CARTESIAN_POINT('Origin',(636.934816028482,-11.5034818258361,-234.90005));
#193405=CARTESIAN_POINT('Origin',(-38.9907249661392,14.740057695632,-234.90005));
#193406=CARTESIAN_POINT('',(-42.5994410002394,17.1689810343211,-235.35005));
#193407=CARTESIAN_POINT('',(-42.9727564520429,17.4202489659097,-234.90005));
#193408=CARTESIAN_POINT('Origin',(-42.5994410002394,17.1689810343211,-234.90005));
#193409=CARTESIAN_POINT('Origin',(-38.9907249661392,14.740057695632,-235.35005));
#193410=CARTESIAN_POINT('Origin',(-38.9907249661392,14.740057695632,-234.90005));
#193411=CARTESIAN_POINT('Origin',(6.29739814579425E-15,-11.5034818258363,
-234.90005));
#193412=CARTESIAN_POINT('',(-27.1371646502378,32.0900589198506,-235.35005));
#193413=CARTESIAN_POINT('',(-27.3749781671338,32.4720860539414,-234.90005));
#193414=CARTESIAN_POINT('Origin',(-27.1371646502378,32.0900589198506,-234.90005));
#193415=CARTESIAN_POINT('Origin',(6.29739814579425E-15,-11.5034818258363,
-235.35005));
#193416=CARTESIAN_POINT('Origin',(6.29739814579425E-15,-11.5034818258363,
-234.90005));
#193417=CARTESIAN_POINT('Origin',(-24.838300653577,28.3971299569735,-234.90005));
#193418=CARTESIAN_POINT('',(-25.3692534585727,32.7146048114303,-235.35005));
#193419=CARTESIAN_POINT('',(-25.4241796108136,33.1612401412018,-234.90005));
#193420=CARTESIAN_POINT('Origin',(-25.3692534585727,32.7146048114303,-234.90005));
#193421=CARTESIAN_POINT('Origin',(-24.838300653577,28.3971299569735,-235.35005));
#193422=CARTESIAN_POINT('Origin',(-24.838300653577,28.3971299569735,-234.90005));
#193423=CARTESIAN_POINT('Origin',(-6.95148506756697,-6.01736880073005,-234.90005));
#193424=CARTESIAN_POINT('',(-6.08254860609655,-5.18975208634635,-235.35005));
#193425=CARTESIAN_POINT('',(-6.40839977914796,-5.50010835424024,-234.90005));
#193426=CARTESIAN_POINT('Origin',(-6.08254860609655,-5.18975208634635,-234.90005));
#193427=CARTESIAN_POINT('',(-5.76949205973895,-5.81026368383122,-235.35005));
#193428=CARTESIAN_POINT('Origin',(-6.95148506756697,-6.01736880073005,-235.35005));
#193429=CARTESIAN_POINT('',(-6.36274467860838,-6.48200280121742,-234.90005));
#193430=CARTESIAN_POINT('Ctrl Pts',(-5.76949205973896,-5.81026368383122,
-235.35005));
#193431=CARTESIAN_POINT('Ctrl Pts',(-5.82092507341363,-5.86238576252255,
-235.35005));
#193432=CARTESIAN_POINT('Ctrl Pts',(-5.87146206806168,-5.91503600112616,
-235.33821291833));
#193433=CARTESIAN_POINT('Ctrl Pts',(-6.00423457196878,-6.05699737629989,
-235.282379503985));
#193434=CARTESIAN_POINT('Ctrl Pts',(-6.07889780142458,-6.14101690884917,
-235.222495970419));
#193435=CARTESIAN_POINT('Ctrl Pts',(-6.22023885093967,-6.30512731290958,
-235.083822800187));
#193436=CARTESIAN_POINT('Ctrl Pts',(-6.29326617328538,-6.39403176703484,
-234.990808270705));
#193437=CARTESIAN_POINT('Ctrl Pts',(-6.36151501319033,-6.48044497931282,
-234.901656863128));
#193438=CARTESIAN_POINT('Ctrl Pts',(-6.36212991841606,-6.48122383507554,
-234.900853430267));
#193439=CARTESIAN_POINT('Ctrl Pts',(-6.36274467860838,-6.48200280121742,
-234.90005));
#193440=CARTESIAN_POINT('Origin',(-6.95148506756697,-6.01736880073005,-234.90005));
#193441=CARTESIAN_POINT('Origin',(147.944423723881,-166.906703884593,-234.90005));
#193442=CARTESIAN_POINT('',(-7.1259980697973,-4.09420716929315,-235.35005));
#193443=CARTESIAN_POINT('',(-7.45184924284871,-4.40456343718705,-234.90005));
#193444=CARTESIAN_POINT('Origin',(-7.1259980697973,-4.09420716929315,-234.90005));
#193445=CARTESIAN_POINT('',(147.944423723881,-166.906703884593,-235.35005));
#193446=CARTESIAN_POINT('',(-6.10697827817035,-5.81657868152891,-234.90005));
#193447=CARTESIAN_POINT('Origin',(-7.99493453126772,-4.92182388367686,-234.90005));
#193448=CARTESIAN_POINT('',(-8.92138760391815,-4.15914131263135,-235.35005));
#193449=CARTESIAN_POINT('Origin',(-7.99493453126772,-4.92182388367686,-235.35005));
#193450=CARTESIAN_POINT('',(-8.57396770167424,-4.44514727677342,-234.90005));
#193451=CARTESIAN_POINT('Origin',(-7.99493453126772,-4.92182388367686,-234.90005));
#193452=CARTESIAN_POINT('Origin',(-8.92138760391815,-4.15914131263135,-234.90005));
#193453=CARTESIAN_POINT('Origin',(0.,-11.5034818258363,-234.90005));
#193454=CARTESIAN_POINT('',(-11.4710456282303,-10.1086318165856,-235.35005));
#193455=CARTESIAN_POINT('',(-11.0243360211906,-10.1629505700546,-234.90005));
#193456=CARTESIAN_POINT('Origin',(-11.4710456282303,-10.1086318165856,-234.90005));
#193457=CARTESIAN_POINT('Origin',(0.,-11.5034818258363,-235.35005));
#193458=CARTESIAN_POINT('Origin',(0.,-11.5034818258363,-234.90005));
#193459=CARTESIAN_POINT('Origin',(-10.2798200094577,-10.2534818258363,-234.90005));
#193460=CARTESIAN_POINT('',(-10.2798200094577,-11.4534818258363,-235.35005));
#193461=CARTESIAN_POINT('',(-10.2798200094577,-11.0034818258363,-234.90005));
#193462=CARTESIAN_POINT('Origin',(-10.2798200094577,-11.4534818258363,-234.90005));
#193463=CARTESIAN_POINT('Origin',(-10.2798200094577,-10.2534818258363,-235.35005));
#193464=CARTESIAN_POINT('Origin',(-10.2798200094577,-10.2534818258363,-234.90005));
#193465=CARTESIAN_POINT('Origin',(296.501483394397,-11.4534818258365,-234.90005));
#193466=CARTESIAN_POINT('',(-8.76687405914145,-11.4534818258363,-235.35005));
#193467=CARTESIAN_POINT('',(-8.76687405914145,-11.0034818258363,-234.90005));
#193468=CARTESIAN_POINT('Origin',(-8.76687405914145,-11.4534818258363,-234.90005));
#193469=CARTESIAN_POINT('',(296.501483394397,-11.4534818258365,-235.35005));
#193470=CARTESIAN_POINT('',(2.22174260618994E-13,-11.0034818258363,-234.90005));
#193471=CARTESIAN_POINT('Origin',(-8.76687405914145,-10.2534818258363,-234.90005));
#193472=CARTESIAN_POINT('',(-8.02438338364376,-10.3593477636964,-234.90005));
#193473=CARTESIAN_POINT('',(-8.1016440740309,-11.2522155575736,-235.35005));
#193474=CARTESIAN_POINT('Ctrl Pts',(-8.02438338364377,-10.3593477636964,
-234.90005));
#193475=CARTESIAN_POINT('Ctrl Pts',(-8.02452345554005,-10.3603301578355,
-234.900853430281));
#193476=CARTESIAN_POINT('Ctrl Pts',(-8.02466334747473,-10.3613125808142,
-234.901656863113));
#193477=CARTESIAN_POINT('Ctrl Pts',(-8.04016643948374,-10.4703300185996,
-234.990808271414));
#193478=CARTESIAN_POINT('Ctrl Pts',(-8.05417784702261,-10.5845257804583,
-235.083822800183));
#193479=CARTESIAN_POINT('Ctrl Pts',(-8.07553226267947,-10.8000565344901,
-235.222495970419));
#193480=CARTESIAN_POINT('Ctrl Pts',(-8.08487817822972,-10.9120678443883,
-235.282379503985));
#193481=CARTESIAN_POINT('Ctrl Pts',(-8.09610373786709,-11.1061182415686,
-235.33821291833));
#193482=CARTESIAN_POINT('Ctrl Pts',(-8.09937411333572,-11.1790246205581,
-235.35005));
#193483=CARTESIAN_POINT('Ctrl Pts',(-8.10164407403091,-11.2522155575736,
-235.35005));
#193484=CARTESIAN_POINT('Origin',(-8.76687405914145,-10.2534818258363,-235.35005));
#193485=CARTESIAN_POINT('Origin',(-8.76687405914145,-10.2534818258363,-234.90005));
#193486=CARTESIAN_POINT('Origin',(-8.76687405914144,-12.7534818258363,-234.90005));
#193487=CARTESIAN_POINT('',(-8.76687405914144,-11.5534818258363,-235.35005));
#193488=CARTESIAN_POINT('',(-8.76687405914144,-12.0034818258363,-234.90005));
#193489=CARTESIAN_POINT('Origin',(-8.76687405914144,-11.5534818258363,-234.90005));
#193490=CARTESIAN_POINT('',(-8.1016440740309,-11.7547480940991,-235.35005));
#193491=CARTESIAN_POINT('Origin',(-8.76687405914144,-12.7534818258363,-235.35005));
#193492=CARTESIAN_POINT('',(-8.02438338364376,-12.6476158879763,-234.90005));
#193493=CARTESIAN_POINT('Ctrl Pts',(-8.10164407403091,-11.7547480940991,
-235.35005));
#193494=CARTESIAN_POINT('Ctrl Pts',(-8.09937411333571,-11.8279390311146,
-235.35005));
#193495=CARTESIAN_POINT('Ctrl Pts',(-8.09610373786709,-11.9008454101041,
-235.33821291833));
#193496=CARTESIAN_POINT('Ctrl Pts',(-8.08487817822972,-12.0948958072843,
-235.282379503985));
#193497=CARTESIAN_POINT('Ctrl Pts',(-8.07553226267949,-12.2069071171824,
-235.222495970419));
#193498=CARTESIAN_POINT('Ctrl Pts',(-8.05417784702484,-12.4224378711919,
-235.083822800197));
#193499=CARTESIAN_POINT('Ctrl Pts',(-8.04016643880974,-12.5366336378126,
-234.990808267567));
#193500=CARTESIAN_POINT('Ctrl Pts',(-8.02466334748842,-12.6456510707622,
-234.90165686319));
#193501=CARTESIAN_POINT('Ctrl Pts',(-8.0245234555264,-12.6466334939328,
-234.900853430203));
#193502=CARTESIAN_POINT('Ctrl Pts',(-8.02438338364376,-12.6476158879763,
-234.90005));
#193503=CARTESIAN_POINT('Origin',(-8.76687405914144,-12.7534818258363,-234.90005));
#193504=CARTESIAN_POINT('Origin',(296.501483394397,-11.5534818258362,-234.90005));
#193505=CARTESIAN_POINT('',(-10.2798200094577,-11.5534818258363,-235.35005));
#193506=CARTESIAN_POINT('',(-10.2798200094577,-12.0034818258363,-234.90005));
#193507=CARTESIAN_POINT('Origin',(-10.2798200094577,-11.5534818258363,-234.90005));
#193508=CARTESIAN_POINT('',(296.501483394397,-11.5534818258362,-235.35005));
#193509=CARTESIAN_POINT('',(2.22174260618994E-13,-12.0034818258363,-234.90005));
#193510=CARTESIAN_POINT('Origin',(-10.2798200094577,-12.7534818258363,-234.90005));
#193511=CARTESIAN_POINT('',(-11.4710456282303,-12.8983318350871,-235.35005));
#193512=CARTESIAN_POINT('',(-11.0243360211906,-12.844013081618,-234.90005));
#193513=CARTESIAN_POINT('Origin',(-11.4710456282303,-12.8983318350871,-234.90005));
#193514=CARTESIAN_POINT('Origin',(-10.2798200094577,-12.7534818258363,-235.35005));
#193515=CARTESIAN_POINT('Origin',(-10.2798200094577,-12.7534818258363,-234.90005));
#193516=CARTESIAN_POINT('Origin',(0.,-11.5034818258363,-234.90005));
#193517=CARTESIAN_POINT('',(-8.92138760391814,-18.8478223390413,-235.35005));
#193518=CARTESIAN_POINT('',(-8.57396770167423,-18.5618163748993,-234.90005));
#193519=CARTESIAN_POINT('Origin',(-8.92138760391814,-18.8478223390413,-234.90005));
#193520=CARTESIAN_POINT('Origin',(0.,-11.5034818258363,-235.35005));
#193521=CARTESIAN_POINT('Origin',(0.,-11.5034818258363,-234.90005));
#193522=CARTESIAN_POINT('Origin',(-7.99493453126771,-18.0851397679958,-234.90005));
#193523=CARTESIAN_POINT('',(-7.1259980697973,-18.9127564823795,-235.35005));
#193524=CARTESIAN_POINT('',(-7.4518492428487,-18.6024002144856,-234.90005));
#193525=CARTESIAN_POINT('Origin',(-7.12599806979729,-18.9127564823795,-234.90005));
#193526=CARTESIAN_POINT('Origin',(-7.99493453126771,-18.0851397679958,-235.35005));
#193527=CARTESIAN_POINT('Origin',(-7.99493453126771,-18.0851397679958,-234.90005));
#193528=CARTESIAN_POINT('Origin',(5.70871573332976,-5.43725435410305,-234.90005));
#193529=CARTESIAN_POINT('',(-6.08254860609655,-17.8172115653263,-235.35005));
#193530=CARTESIAN_POINT('',(-6.40839977914795,-17.5068552974324,-234.90005));
#193531=CARTESIAN_POINT('Origin',(-6.08254860609655,-17.8172115653263,-234.90005));
#193532=CARTESIAN_POINT('',(-7.1259980697973,-18.9127564823795,-235.35005));
#193533=CARTESIAN_POINT('',(-6.40839977914795,-17.5068552974324,-234.90005));
#193534=CARTESIAN_POINT('Origin',(-6.95148506756696,-16.9895948509426,-234.90005));
#193535=CARTESIAN_POINT('',(-6.36274467860837,-16.5249608504553,-234.90005));
#193536=CARTESIAN_POINT('',(-5.76949205973894,-17.1966999678414,-235.35005));
#193537=CARTESIAN_POINT('Ctrl Pts',(-6.36274467860837,-16.5249608504552,
-234.90005));
#193538=CARTESIAN_POINT('Ctrl Pts',(-6.36212991839128,-16.5257398166285,
-234.900853430299));
#193539=CARTESIAN_POINT('Ctrl Pts',(-6.36151501321541,-16.5265186723281,
-234.901656863095));
#193540=CARTESIAN_POINT('Ctrl Pts',(-6.2932661720145,-16.6129318862469,
-234.990808272351));
#193541=CARTESIAN_POINT('Ctrl Pts',(-6.22023885094759,-16.7018363387539,
-235.083822800179));
#193542=CARTESIAN_POINT('Ctrl Pts',(-6.07889780142461,-16.8659467428234,
-235.222495970419));
#193543=CARTESIAN_POINT('Ctrl Pts',(-6.0042345719688,-16.9499662753727,
-235.282379503985));
#193544=CARTESIAN_POINT('Ctrl Pts',(-5.87146206806167,-17.0919276505465,
-235.33821291833));
#193545=CARTESIAN_POINT('Ctrl Pts',(-5.82092507341363,-17.1445778891501,
-235.35005));
#193546=CARTESIAN_POINT('Ctrl Pts',(-5.76949205973896,-17.1966999678414,
-235.35005));
#193547=CARTESIAN_POINT('Origin',(-6.95148506756696,-16.9895948509426,-235.35005));
#193548=CARTESIAN_POINT('Origin',(-6.95148506756696,-16.9895948509426,-234.90005));
#193549=CARTESIAN_POINT('Origin',(-1.25,-2.73660776669487,-234.90005));
#193550=CARTESIAN_POINT('',(-0.0499999999999959,-2.73660776669487,-235.35005));
#193551=CARTESIAN_POINT('',(-0.5,-2.73660776669487,-234.90005));
#193552=CARTESIAN_POINT('Origin',(-0.0499999999999959,-2.73660776669487,
-234.90005));
#193553=CARTESIAN_POINT('',(-0.251266268262739,-3.40183775180542,-235.35005));
#193554=CARTESIAN_POINT('Origin',(-1.25,-2.73660776669487,-235.35005));
#193555=CARTESIAN_POINT('',(-1.14413406213993,-3.47909844219256,-234.90005));
#193556=CARTESIAN_POINT('Ctrl Pts',(-0.251266268262739,-3.40183775180541,
-235.35005));
#193557=CARTESIAN_POINT('Ctrl Pts',(-0.32445720527824,-3.4041077125006,
-235.35005));
#193558=CARTESIAN_POINT('Ctrl Pts',(-0.397363584267787,-3.40737808796923,
-235.33821291833));
#193559=CARTESIAN_POINT('Ctrl Pts',(-0.59141398144801,-3.4186036476066,
-235.282379503985));
#193560=CARTESIAN_POINT('Ctrl Pts',(-0.703425291346146,-3.42794956315684,
-235.222495970419));
#193561=CARTESIAN_POINT('Ctrl Pts',(-0.918956045360097,-3.44930397881193,
-235.083822800194));
#193562=CARTESIAN_POINT('Ctrl Pts',(-1.03315181083036,-3.46331538686362,
-234.990808268497));
#193563=CARTESIAN_POINT('Ctrl Pts',(-1.14216924494834,-3.4788184783511,
-234.901656863172));
#193564=CARTESIAN_POINT('Ctrl Pts',(-1.14315166807396,-3.47895837030671,
-234.900853430222));
#193565=CARTESIAN_POINT('Ctrl Pts',(-1.14413406213993,-3.47909844219256,
-234.90005));
#193566=CARTESIAN_POINT('Origin',(-1.25,-2.73660776669487,-234.90005));
#193567=CARTESIAN_POINT('Origin',(-0.0499999999999945,-25.4138432731711,
-234.90005));
#193568=CARTESIAN_POINT('',(-0.0499999999999981,-1.22366181637858,-235.35005));
#193569=CARTESIAN_POINT('',(-0.5,-1.22366181637858,-234.90005));
#193570=CARTESIAN_POINT('Origin',(-0.0499999999999981,-1.22366181637858,
-234.90005));
#193571=CARTESIAN_POINT('',(-0.0499999999999959,-2.73660776669487,-235.35005));
#193572=CARTESIAN_POINT('',(-0.5,-1.22366181637858,-234.90005));
#193573=CARTESIAN_POINT('Origin',(-1.25,-1.22366181637858,-234.90005));
#193574=CARTESIAN_POINT('',(-1.39485000925072,-0.0324361976060192,-235.35005));
#193575=CARTESIAN_POINT('Origin',(-1.25,-1.22366181637858,-235.35005));
#193576=CARTESIAN_POINT('',(-1.3405312557817,-0.479145804645727,-234.90005));
#193577=CARTESIAN_POINT('Origin',(-1.25,-1.22366181637858,-234.90005));
#193578=CARTESIAN_POINT('Origin',(-1.39485000925072,-0.0324361976060193,
-234.90005));
#193579=CARTESIAN_POINT('Origin',(0.,-11.5034818258363,-234.90005));
#193580=CARTESIAN_POINT('',(-6.90132755171766,-2.23513934310776,-235.35005));
#193581=CARTESIAN_POINT('',(-6.63257355852517,-2.59607048770891,-234.90005));
#193582=CARTESIAN_POINT('Origin',(-6.90132755171766,-2.23513934310776,-234.90005));
#193583=CARTESIAN_POINT('Origin',(0.,-11.5034818258363,-235.35005));
#193584=CARTESIAN_POINT('Origin',(0.,-11.5034818258363,-234.90005));
#193585=CARTESIAN_POINT('Origin',(-6.18465023653769,-3.19762239537748,-234.90005));
#193586=CARTESIAN_POINT('',(-7.05358669800811,-4.02523910976119,-235.35005));
#193587=CARTESIAN_POINT('',(-6.7277355249567,-3.7148828418673,-234.90005));
#193588=CARTESIAN_POINT('Origin',(-7.05358669800812,-4.0252391097612,-234.90005));
#193589=CARTESIAN_POINT('Origin',(-6.18465023653769,-3.19762239537748,-235.35005));
#193590=CARTESIAN_POINT('Origin',(-6.18465023653769,-3.19762239537748,-234.90005));
#193591=CARTESIAN_POINT('Origin',(148.016835095671,-166.837735825062,-234.90005));
#193592=CARTESIAN_POINT('',(-6.01013723430737,-5.12078402681439,-235.35005));
#193593=CARTESIAN_POINT('',(-5.68428606125595,-4.81042775892049,-234.90005));
#193594=CARTESIAN_POINT('Origin',(-6.01013723430736,-5.12078402681438,-234.90005));
#193595=CARTESIAN_POINT('',(148.016835095671,-166.837735825062,-235.35005));
#193596=CARTESIAN_POINT('',(-5.38286456027834,-5.12689808620916,-234.90005));
#193597=CARTESIAN_POINT('Origin',(-5.14120077283694,-4.29316731243068,-234.90005));
#193598=CARTESIAN_POINT('',(-4.70577833960231,-4.90382867901287,-234.90005));
#193599=CARTESIAN_POINT('',(-5.40560135635379,-5.46367674487279,-235.35005));
#193600=CARTESIAN_POINT('Ctrl Pts',(-4.70577833960231,-4.90382867901288,
-234.90005));
#193601=CARTESIAN_POINT('Ctrl Pts',(-4.70658630946365,-4.90440478914896,
-234.900853430202));
#193602=CARTESIAN_POINT('Ctrl Pts',(-4.7073941763327,-4.9049810496594,-234.901656863192));
#193603=CARTESIAN_POINT('Ctrl Pts',(-4.7970273762009,-4.96894225656959,
-234.990808267499));
#193604=CARTESIAN_POINT('Ctrl Pts',(-4.88938149376754,-5.03755500803177,
-235.083822800199));
#193605=CARTESIAN_POINT('Ctrl Pts',(-5.06017799547275,-5.17073936145204,
-235.222495970419));
#193606=CARTESIAN_POINT('Ctrl Pts',(-5.14773261812954,-5.24122388268893,
-235.282379503985));
#193607=CARTESIAN_POINT('Ctrl Pts',(-5.29598922334359,-5.36692809441377,
-235.33821291833));
#193608=CARTESIAN_POINT('Ctrl Pts',(-5.35103724699188,-5.41484208553839,
-235.35005));
#193609=CARTESIAN_POINT('Ctrl Pts',(-5.40560135635379,-5.46367674487279,
-235.35005));
#193610=CARTESIAN_POINT('Origin',(-5.14120077283694,-4.29316731243068,-235.35005));
#193611=CARTESIAN_POINT('Origin',(-5.14120077283694,-4.29316731243068,-234.90005));
#193612=CARTESIAN_POINT('Origin',(-5.14120077283693,-18.713796339242,-234.90005));
#193613=CARTESIAN_POINT('',(-5.40560135635378,-17.5432869067998,-235.35005));
#193614=CARTESIAN_POINT('',(-4.7057783396023,-18.1031349726598,-234.90005));
#193615=CARTESIAN_POINT('Ctrl Pts',(-4.7057783396023,-18.1031349726598,
-234.90005));
#193616=CARTESIAN_POINT('Ctrl Pts',(-4.70658630927984,-18.1025588626547,
-234.900853430019));
#193617=CARTESIAN_POINT('Ctrl Pts',(-4.70739417651803,-18.101982601881,
-234.901656863374));
#193618=CARTESIAN_POINT('Ctrl Pts',(-4.79702736710127,-18.0380214015964,
-234.990808258517));
#193619=CARTESIAN_POINT('Ctrl Pts',(-4.88938149380989,-17.9694086436079,
-235.083822800233));
#193620=CARTESIAN_POINT('Ctrl Pts',(-5.06017799547342,-17.8362242902201,
-235.222495970419));
#193621=CARTESIAN_POINT('Ctrl Pts',(-5.14773261813007,-17.7657397689833,
-235.282379503985));
#193622=CARTESIAN_POINT('Ctrl Pts',(-5.29598922334368,-17.6400355572588,
-235.33821291833));
#193623=CARTESIAN_POINT('Ctrl Pts',(-5.35103724699192,-17.5921215661342,
-235.35005));
#193624=CARTESIAN_POINT('Ctrl Pts',(-5.40560135635379,-17.5432869067999,
-235.35005));
#193625=CARTESIAN_POINT('',(-5.68428606125594,-18.1965358927522,-234.90005));
#193626=CARTESIAN_POINT('Origin',(-5.14120077283693,-18.713796339242,-234.90005));
#193627=CARTESIAN_POINT('',(-6.01013723430735,-17.8861796248583,-235.35005));
#193628=CARTESIAN_POINT('Origin',(-6.01013723430735,-17.8861796248583,-234.90005));
#193629=CARTESIAN_POINT('Origin',(-5.14120077283693,-18.713796339242,-235.35005));
#193630=CARTESIAN_POINT('Origin',(5.78112710511895,-5.50622241363502,-234.90005));
#193631=CARTESIAN_POINT('',(-7.0535866980081,-18.9817245419115,-235.35005));
#193632=CARTESIAN_POINT('',(-6.72773552495669,-19.2920808098054,-234.90005));
#193633=CARTESIAN_POINT('Origin',(-7.0535866980081,-18.9817245419115,-234.90005));
#193634=CARTESIAN_POINT('',(-6.01013723430735,-17.8861796248583,-235.35005));
#193635=CARTESIAN_POINT('',(-6.7277355249567,-19.2920808098054,-234.90005));
#193636=CARTESIAN_POINT('Origin',(-6.18465023653768,-19.8093412562951,-234.90005));
#193637=CARTESIAN_POINT('',(-6.90132755171765,-20.7718243085649,-235.35005));
#193638=CARTESIAN_POINT('',(-6.63257355852516,-20.4108931639637,-234.90005));
#193639=CARTESIAN_POINT('Origin',(-6.90132755171765,-20.7718243085649,-234.90005));
#193640=CARTESIAN_POINT('Origin',(-6.18465023653768,-19.8093412562951,-235.35005));
#193641=CARTESIAN_POINT('Origin',(-6.18465023653768,-19.8093412562951,-234.90005));
#193642=CARTESIAN_POINT('Origin',(0.,-11.5034818258363,-234.90005));
#193643=CARTESIAN_POINT('',(-1.39485000925072,-22.9745274540666,-235.35005));
#193644=CARTESIAN_POINT('',(-1.3405312557817,-22.5278178470269,-234.90005));
#193645=CARTESIAN_POINT('Origin',(-1.39485000925072,-22.9745274540666,-234.90005));
#193646=CARTESIAN_POINT('Origin',(0.,-11.5034818258363,-235.35005));
#193647=CARTESIAN_POINT('Origin',(0.,-11.5034818258363,-234.90005));
#193648=CARTESIAN_POINT('Origin',(-1.25,-21.7833018352941,-234.90005));
#193649=CARTESIAN_POINT('',(-0.0499999999999969,-21.7833018352941,-235.35005));
#193650=CARTESIAN_POINT('',(-0.5,-21.7833018352941,-234.90005));
#193651=CARTESIAN_POINT('Origin',(-0.0499999999999947,-21.7833018352941,
-234.90005));
#193652=CARTESIAN_POINT('Origin',(-1.25,-21.7833018352941,-235.35005));
#193653=CARTESIAN_POINT('Origin',(-1.25,-21.7833018352941,-234.90005));
#193654=CARTESIAN_POINT('Origin',(-0.0499999999999945,-25.4138432731711,
-234.90005));
#193655=CARTESIAN_POINT('',(-0.0499999999999948,-20.2703558849778,-235.35005));
#193656=CARTESIAN_POINT('',(-0.5,-20.2703558849778,-234.90005));
#193657=CARTESIAN_POINT('Origin',(-0.049999999999997,-20.2703558849778,
-234.90005));
#193658=CARTESIAN_POINT('',(-0.0499999999999947,-21.7833018352941,-235.35005));
#193659=CARTESIAN_POINT('',(-0.5,-20.2703558849778,-234.90005));
#193660=CARTESIAN_POINT('Origin',(-1.25,-20.2703558849778,-234.90005));
#193661=CARTESIAN_POINT('',(-1.14413406213993,-19.5278652094801,-234.90005));
#193662=CARTESIAN_POINT('',(-0.251266268262739,-19.6051258998672,-235.35005));
#193663=CARTESIAN_POINT('Ctrl Pts',(-1.14413406213993,-19.5278652094801,
-234.90005));
#193664=CARTESIAN_POINT('Ctrl Pts',(-1.1431516683171,-19.5280052813313,
-234.900853430023));
#193665=CARTESIAN_POINT('Ctrl Pts',(-1.14216924470318,-19.5281451733564,
-234.90165686337));
#193666=CARTESIAN_POINT('Ctrl Pts',(-1.03315182292617,-19.5436482630889,
-234.990808258681));
#193667=CARTESIAN_POINT('Ctrl Pts',(-0.918956045301575,-19.5576596728665,
-235.083822800232));
#193668=CARTESIAN_POINT('Ctrl Pts',(-0.703425291345268,-19.5790140885159,
-235.222495970419));
#193669=CARTESIAN_POINT('Ctrl Pts',(-0.591413981447289,-19.5883600040661,
-235.282379503985));
#193670=CARTESIAN_POINT('Ctrl Pts',(-0.397363584267675,-19.5995855637034,
-235.33821291833));
#193671=CARTESIAN_POINT('Ctrl Pts',(-0.324457205278181,-19.602855939172,
-235.35005));
#193672=CARTESIAN_POINT('Ctrl Pts',(-0.25126626826274,-19.6051258998672,
-235.35005));
#193673=CARTESIAN_POINT('Origin',(-1.25,-20.2703558849778,-235.35005));
#193674=CARTESIAN_POINT('Origin',(-1.25,-20.2703558849778,-234.90005));
#193675=CARTESIAN_POINT('Origin',(-41.3132181298675,38.0528376956935,-203.84995));
#193676=CARTESIAN_POINT('',(-50.148669624411,48.964302343774,-203.876128609656));
#193677=CARTESIAN_POINT('',(-49.2048636720257,47.7987359558583,-205.34995));
#193678=CARTESIAN_POINT('Origin',(-49.2048636720257,47.7987359558583,-203.84995));
#193679=CARTESIAN_POINT('',(-43.9433571680673,51.844416014308,-203.876128609656));
#193680=CARTESIAN_POINT('Origin',(-41.3132181298675,38.0528376956935,-203.876128609656));
#193681=CARTESIAN_POINT('',(-43.6624048158998,50.3711948984507,-205.34995));
#193682=CARTESIAN_POINT('Origin',(-43.6624048158998,50.3711948984507,-203.84995));
#193683=CARTESIAN_POINT('Origin',(-41.3132181298675,38.0528376956935,-205.34995));
#193684=CARTESIAN_POINT('Origin',(0.,-12.9675000200281,-203.84995));
#193685=CARTESIAN_POINT('',(-61.5592179767879,37.6378345921813,-203.876128609656));
#193686=CARTESIAN_POINT('',(-60.4006636863987,36.6854341319664,-205.34995));
#193687=CARTESIAN_POINT('Origin',(-60.4006636863987,36.6854341319665,-203.84995));
#193688=CARTESIAN_POINT('Origin',(0.,-12.9675000200281,-203.876128609656));
#193689=CARTESIAN_POINT('Origin',(0.,-12.9675000200281,-205.34995));
#193690=CARTESIAN_POINT('Origin',(-50.7133971693864,28.7219255026674,-203.84995));
#193691=CARTESIAN_POINT('',(-64.7425725698088,29.2764536470619,-203.876128609656));
#193692=CARTESIAN_POINT('',(-63.2439712523603,29.2172187609027,-205.34995));
#193693=CARTESIAN_POINT('Origin',(-63.2439712523603,29.2172187609027,-203.84995));
#193694=CARTESIAN_POINT('Origin',(-50.7133971693864,28.7219255026673,-203.876128609656));
#193695=CARTESIAN_POINT('Origin',(-50.7133971693864,28.7219255026674,-205.34995));
#193696=CARTESIAN_POINT('Origin',(1004.,-12.967500020028,-203.84995));
#193697=CARTESIAN_POINT('',(-64.7425725698087,-55.2114536871185,-203.876128609656));
#193698=CARTESIAN_POINT('',(-63.2439712523603,-55.1522188009592,-205.34995));
#193699=CARTESIAN_POINT('Origin',(-63.2439712523603,-55.1522188009592,-203.84995));
#193700=CARTESIAN_POINT('Origin',(1004.,-12.967500020028,-203.87612860965));
#193701=CARTESIAN_POINT('Origin',(1004.,-12.967500020028,-205.34995));
#193702=CARTESIAN_POINT('Origin',(-50.7133971693864,-54.6569255427236,-203.84995));
#193703=CARTESIAN_POINT('',(-61.5592179767879,-63.5728346322375,-203.876128609656));
#193704=CARTESIAN_POINT('',(-60.4006636863987,-62.6204341720228,-205.34995));
#193705=CARTESIAN_POINT('Origin',(-60.4006636863987,-62.6204341720228,-203.84995));
#193706=CARTESIAN_POINT('Origin',(-50.7133971693864,-54.6569255427236,-203.876128609656));
#193707=CARTESIAN_POINT('Origin',(-50.7133971693864,-54.6569255427236,-205.34995));
#193708=CARTESIAN_POINT('Origin',(0.,-12.9675000200281,-203.84995));
#193709=CARTESIAN_POINT('',(-50.4303082679829,-74.6701840550325,-203.876128609656));
#193710=CARTESIAN_POINT('',(-49.481201831453,-73.5089297105696,-205.34995));
#193711=CARTESIAN_POINT('Origin',(-49.481201831453,-73.5089297105696,-203.84995));
#193712=CARTESIAN_POINT('Origin',(0.,-12.9675000200281,-203.876128609656));
#193713=CARTESIAN_POINT('Origin',(0.,-12.9675000200281,-205.34995));
#193714=CARTESIAN_POINT('Origin',(-41.5452362233251,-63.7990866568863,-203.84995));
#193715=CARTESIAN_POINT('',(-42.0978464467214,-77.8283377352489,-203.876128609656));
#193716=CARTESIAN_POINT('',(-42.0388164335396,-76.329728333857,-205.34995));
#193717=CARTESIAN_POINT('Origin',(-42.0388164335396,-76.329728333857,-203.84995));
#193718=CARTESIAN_POINT('Origin',(-41.5452362233251,-63.7990866568863,-203.876128609656));
#193719=CARTESIAN_POINT('Origin',(-41.5452362233251,-63.7990866568863,-205.34995));
#193720=CARTESIAN_POINT('Ctrl Pts',(-23.3965212694791,39.0700122934506,
-234.574197273323));
#193721=CARTESIAN_POINT('Ctrl Pts',(-23.441207715325,38.6446575693707,-235.35005));
#193722=CARTESIAN_POINT('Ctrl Pts',(-23.5337713018193,37.7635770079652,
-235.35005));
#193723=CARTESIAN_POINT('Ctrl Pts',(-21.5285729617573,38.8429287236754,
-234.629840683519));
#193724=CARTESIAN_POINT('Ctrl Pts',(-21.5595177806197,38.4044126698907,
-235.350049999891));
#193725=CARTESIAN_POINT('Ctrl Pts',(-21.5449677583916,37.5546394871488,
-235.35005));
#193726=CARTESIAN_POINT('Ctrl Pts',(-19.6686582940338,38.873624481404,-234.667826224195));
#193727=CARTESIAN_POINT('Ctrl Pts',(-19.6461032038161,38.4273266114594,
-235.350050000221));
#193728=CARTESIAN_POINT('Ctrl Pts',(-19.5728087819113,37.6143598891179,
-235.35005));
#193729=CARTESIAN_POINT('Ctrl Pts',(-17.3605227404968,39.2364170937257,
-234.700260615516));
#193730=CARTESIAN_POINT('Ctrl Pts',(-17.2775810752257,38.7970065033925,
-235.350049999945));
#193731=CARTESIAN_POINT('Ctrl Pts',(-17.1293181159922,38.0221098574478,
-235.35005));
#193732=CARTESIAN_POINT('Ctrl Pts',(-16.8996944960412,39.3254277923721,
-234.705962605482));
#193733=CARTESIAN_POINT('Ctrl Pts',(-16.8064955068198,38.8875662731569,
-235.350049999917));
#193734=CARTESIAN_POINT('Ctrl Pts',(-16.6417036623955,38.1205664042693,
-235.35005));
#193735=CARTESIAN_POINT('Ctrl Pts',(-16.4255331955625,39.4347061351644,
-234.711087809772));
#193736=CARTESIAN_POINT('Ctrl Pts',(-16.3214053907335,38.9990490260666,
-235.350050000003));
#193737=CARTESIAN_POINT('Ctrl Pts',(-16.1400046132382,38.2400981928593,
-235.35005));
#193738=CARTESIAN_POINT('Ctrl Pts',(-16.4084238303339,39.4389694488068,
-234.710829083432));
#193739=CARTESIAN_POINT('Ctrl Pts',(-16.3050101388373,39.0031621878097,
-235.35005));
#193740=CARTESIAN_POINT('Ctrl Pts',(-16.1248016481815,38.2437210060648,
-235.35005));
#193741=CARTESIAN_POINT('Ctrl Pts',(-16.3761129052093,39.4467740117303,
-234.710599688867));
#193742=CARTESIAN_POINT('Ctrl Pts',(-16.2734102840084,39.0108163690221,
-235.35005));
#193743=CARTESIAN_POINT('Ctrl Pts',(-16.0943932022442,38.2509106188218,
-235.35005));
#193744=CARTESIAN_POINT('Ctrl Pts',(-16.3599561657618,39.450655986529,-234.710484721543));
#193745=CARTESIAN_POINT('Ctrl Pts',(-16.2576091615606,39.0146236300189,
-235.35005));
#193746=CARTESIAN_POINT('Ctrl Pts',(-16.0791881138821,38.2544860972426,
-235.35005));
#193747=CARTESIAN_POINT('Ctrl Pts',(-16.3114821481724,39.4622410332486,
-234.710139015331));
#193748=CARTESIAN_POINT('Ctrl Pts',(-16.2102010812718,39.0259862502062,
-235.35005));
#193749=CARTESIAN_POINT('Ctrl Pts',(-16.033570255147,38.2651546046657,-235.35005));
#193750=CARTESIAN_POINT('Ctrl Pts',(-16.2791610701706,39.469883227432,-234.709907472259));
#193751=CARTESIAN_POINT('Ctrl Pts',(-16.1785917022065,39.0334818852873,
-235.350050000003));
#193752=CARTESIAN_POINT('Ctrl Pts',(-16.0031548911028,38.2721897057073,
-235.35005));
#193753=CARTESIAN_POINT('Ctrl Pts',(-16.1821828897582,39.4925666443581,
-234.709209671843));
#193754=CARTESIAN_POINT('Ctrl Pts',(-16.0837448349166,39.0557325021636,
-235.350049999995));
#193755=CARTESIAN_POINT('Ctrl Pts',(-15.9118984444987,38.293063747877,-235.35005));
#193756=CARTESIAN_POINT('Ctrl Pts',(-16.1175108380135,39.5073646989989,
-234.708740244041));
#193757=CARTESIAN_POINT('Ctrl Pts',(-16.0204977871684,39.0702489458226,
-235.350049999996));
#193758=CARTESIAN_POINT('Ctrl Pts',(-15.8510470074106,38.3066714267388,
-235.35005));
#193759=CARTESIAN_POINT('Ctrl Pts',(-15.923436929361,39.5507890631334,-234.707319617973));
#193760=CARTESIAN_POINT('Ctrl Pts',(-15.8306827227777,39.1128561089809,
-235.350050000009));
#193761=CARTESIAN_POINT('Ctrl Pts',(-15.6684514414679,38.3465730642683,
-235.35005));
#193762=CARTESIAN_POINT('Ctrl Pts',(-15.7939773013225,39.5784455268499,
-234.706356088967));
#193763=CARTESIAN_POINT('Ctrl Pts',(-15.7040775100839,39.1399955931374,
-235.350050000029));
#193764=CARTESIAN_POINT('Ctrl Pts',(-15.5466660570668,38.3719456051061,
-235.35005));
#193765=CARTESIAN_POINT('Ctrl Pts',(-15.4053840336983,39.6575602691303,
-234.703418469392));
#193766=CARTESIAN_POINT('Ctrl Pts',(-15.3239745423948,39.2176705993572,
-235.350049999942));
#193767=CARTESIAN_POINT('Ctrl Pts',(-15.1811462198576,38.4444074430163,
-235.35005));
#193768=CARTESIAN_POINT('Ctrl Pts',(-15.1460359232891,39.7051631376525,
-234.701397554764));
#193769=CARTESIAN_POINT('Ctrl Pts',(-15.0703368511065,39.2644253992522,
-235.350050000007));
#193770=CARTESIAN_POINT('Ctrl Pts',(-14.9372480705784,38.4878406764273,
-235.35005));
#193771=CARTESIAN_POINT('Ctrl Pts',(-13.8480945051425,39.9178513634478,
-234.690999263195));
#193772=CARTESIAN_POINT('Ctrl Pts',(-13.7992252388259,39.4738011152816,
-235.350049999972));
#193773=CARTESIAN_POINT('Ctrl Pts',(-13.7166846430007,38.681049143284,-235.35005));
#193774=CARTESIAN_POINT('Ctrl Pts',(-12.8051801439163,40.0076434448158,
-234.681621861006));
#193775=CARTESIAN_POINT('Ctrl Pts',(-12.7786604443217,39.5624349839993,
-235.350049999918));
#193776=CARTESIAN_POINT('Ctrl Pts',(-12.7368211885109,38.7593950182271,
-235.35005));
#193777=CARTESIAN_POINT('Ctrl Pts',(-11.2337410805306,40.0229720626152,
-234.665772580439));
#193778=CARTESIAN_POINT('Ctrl Pts',(-11.2431493991504,39.5795098549774,
-235.350050000041));
#193779=CARTESIAN_POINT('Ctrl Pts',(-11.2619727865364,38.7640531506757,
-235.35005));
#193780=CARTESIAN_POINT('Ctrl Pts',(-10.7088507580156,40.0081380134295,
-234.660205544568));
#193781=CARTESIAN_POINT('Ctrl Pts',(-10.7295202598973,39.5657289156652,
-235.350049999972));
#193782=CARTESIAN_POINT('Ctrl Pts',(-10.769512598989,38.7467544284794,-235.35005));
#193783=CARTESIAN_POINT('Ctrl Pts',(-9.91948648717853,39.955281844485,-234.651341964047));
#193784=CARTESIAN_POINT('Ctrl Pts',(-9.95765099397115,39.5153737946489,
-235.350050000014));
#193785=CARTESIAN_POINT('Ctrl Pts',(-10.0295286270685,38.6919125336202,
-235.35005));
#193786=CARTESIAN_POINT('Ctrl Pts',(-9.65606191081629,39.9325482704366,
-234.648309008783));
#193787=CARTESIAN_POINT('Ctrl Pts',(-9.69987071016349,39.4935906245988,
-235.350050000035));
#193788=CARTESIAN_POINT('Ctrl Pts',(-9.78265126312491,38.6688067780134,
-235.35005));
#193789=CARTESIAN_POINT('Ctrl Pts',(-9.37589591312305,39.9028851219532,
-234.645007706899));
#193790=CARTESIAN_POINT('Ctrl Pts',(-9.42585059617205,39.4651058329293,
-235.350049999998));
#193791=CARTESIAN_POINT('Ctrl Pts',(-9.52011153215911,38.6390634524768,
-235.35005));
#193792=CARTESIAN_POINT('Ctrl Pts',(-9.36305882799351,39.9011137141232,
-234.645527469892));
#193793=CARTESIAN_POINT('Ctrl Pts',(-9.41213306277311,39.4631587775859,
-235.350050000001));
#193794=CARTESIAN_POINT('Ctrl Pts',(-9.5046684958238,38.6373245043133,-235.35005));
#193795=CARTESIAN_POINT('Ctrl Pts',(-9.33400183059134,39.8976433794956,
-234.645901386584));
#193796=CARTESIAN_POINT('Ctrl Pts',(-9.38245770550587,39.4595650288394,
-235.350049999999));
#193797=CARTESIAN_POINT('Ctrl Pts',(-9.47378419368037,38.6338861514567,
-235.35005));
#193798=CARTESIAN_POINT('Ctrl Pts',(-9.31947356561741,39.8959244662302,
-234.646087475637));
#193799=CARTESIAN_POINT('Ctrl Pts',(-9.36762025207224,39.4577849263438,
-235.350049999996));
#193800=CARTESIAN_POINT('Ctrl Pts',(-9.4583427946727,38.6321837720633,-235.35005));
#193801=CARTESIAN_POINT('Ctrl Pts',(-9.27588952240145,39.8908164251014,
-234.64664315687));
#193802=CARTESIAN_POINT('Ctrl Pts',(-9.32311043679367,39.4524950861104,
-235.350050000007));
#193803=CARTESIAN_POINT('Ctrl Pts',(-9.41202085079896,38.6271269561732,
-235.35005));
#193804=CARTESIAN_POINT('Ctrl Pts',(-9.24683449671838,39.8874759952947,
-234.647010163276));
#193805=CARTESIAN_POINT('Ctrl Pts',(-9.29343696234345,39.4490353641227,
-235.350050000002));
#193806=CARTESIAN_POINT('Ctrl Pts',(-9.38114255901401,38.6238228412382,
-235.35005));
#193807=CARTESIAN_POINT('Ctrl Pts',(-9.15967282997768,39.8776490180443,
-234.64810100638));
#193808=CARTESIAN_POINT('Ctrl Pts',(-9.20442696746952,39.438857479744,-235.350049999996));
#193809=CARTESIAN_POINT('Ctrl Pts',(-9.28851667274619,38.6141112622619,
-235.35005));
#193810=CARTESIAN_POINT('Ctrl Pts',(-9.10156960385291,39.8713567716217,
-234.648814670252));
#193811=CARTESIAN_POINT('Ctrl Pts',(-9.14508625993128,39.4323387903818,
-235.35005));
#193812=CARTESIAN_POINT('Ctrl Pts',(-9.22677806679909,38.6079045517242,
-235.35005));
#193813=CARTESIAN_POINT('Ctrl Pts',(-8.92727674161121,39.853253826224,-234.650916177606));
#193814=CARTESIAN_POINT('Ctrl Pts',(-8.9671077921105,39.4135836156387,-235.350049999998));
#193815=CARTESIAN_POINT('Ctrl Pts',(-9.04159803735041,38.5900837326631,
-235.35005));
#193816=CARTESIAN_POINT('Ctrl Pts',(-8.81110395292333,39.8422167453627,
-234.652264586384));
#193817=CARTESIAN_POINT('Ctrl Pts',(-8.84845540125615,39.4021407470111,
-235.350049999988));
#193818=CARTESIAN_POINT('Ctrl Pts',(-8.91819239372934,38.5792687468256,
-235.35005));
#193819=CARTESIAN_POINT('Ctrl Pts',(-7.76582421746211,39.7521044618495,
-234.66395028747));
#193820=CARTESIAN_POINT('Ctrl Pts',(-7.78295296745438,39.3088433368614,
-235.350050000096));
#193821=CARTESIAN_POINT('Ctrl Pts',(-7.80796793853896,38.4914558623083,
-235.35005));
#193822=CARTESIAN_POINT('Ctrl Pts',(-6.84026829339966,39.7375184536817,
-234.671163119943));
#193823=CARTESIAN_POINT('Ctrl Pts',(-6.83602394718808,39.2929688862628,
-235.350050000027));
#193824=CARTESIAN_POINT('Ctrl Pts',(-6.82559161828985,38.4810313542666,
-235.35005));
#193825=CARTESIAN_POINT('Ctrl Pts',(-5.45752242742407,39.8114784377381,
-234.677676143363));
#193826=CARTESIAN_POINT('Ctrl Pts',(-5.4226222629611,39.3679214220723,-235.350049999987));
#193827=CARTESIAN_POINT('Ctrl Pts',(-5.35870347059637,38.5640529809275,
-235.35005));
#193828=CARTESIAN_POINT('Ctrl Pts',(-4.99769610645251,39.8521042185811,
-234.679138440416));
#193829=CARTESIAN_POINT('Ctrl Pts',(-4.95262310277034,39.4092970533836,
-235.350050000034));
#193830=CARTESIAN_POINT('Ctrl Pts',(-4.87084783106756,38.6081920654726,
-235.35005));
#193831=CARTESIAN_POINT('Ctrl Pts',(-4.30945715270495,39.9372528391947,
-234.680264606398));
#193832=CARTESIAN_POINT('Ctrl Pts',(-4.24936647991965,39.4961966039752,
-235.350049999983));
#193833=CARTESIAN_POINT('Ctrl Pts',(-4.14073989606153,38.699320253323,-235.35005));
#193834=CARTESIAN_POINT('Ctrl Pts',(-4.08028903034606,39.9696611739215,
-234.680464330858));
#193835=CARTESIAN_POINT('Ctrl Pts',(-4.01520883927272,39.5292913024185,
-235.350050000003));
#193836=CARTESIAN_POINT('Ctrl Pts',(-3.89764918017226,38.7338397861251,
-235.35005));
#193837=CARTESIAN_POINT('Ctrl Pts',(-3.79422129172372,40.0152320597201,
-234.680493511581));
#193838=CARTESIAN_POINT('Ctrl Pts',(-3.72292214062828,39.5758501073975,
-235.350049999999));
#193839=CARTESIAN_POINT('Ctrl Pts',(-3.59413684837652,38.7822104558047,
-235.35005));
#193840=CARTESIAN_POINT('Ctrl Pts',(-3.73702740263105,40.0245994768347,
-234.680488271922));
#193841=CARTESIAN_POINT('Ctrl Pts',(-3.66448423965549,39.585421766879,-235.350050000009));
#193842=CARTESIAN_POINT('Ctrl Pts',(-3.5334519508703,38.7921458859281,-235.35005));
#193843=CARTESIAN_POINT('Ctrl Pts',(-3.62268126481012,40.0438423896311,
-234.680455404551));
#193844=CARTESIAN_POINT('Ctrl Pts',(-3.54764974254042,39.6050865585617,
-235.350049999992));
#193845=CARTESIAN_POINT('Ctrl Pts',(-3.41211742808775,38.8125413393334,
-235.35005));
#193846=CARTESIAN_POINT('Ctrl Pts',(-3.5692122635324,40.0532709032775,-234.680346020914));
#193847=CARTESIAN_POINT('Ctrl Pts',(-3.49163377701029,39.6149697737271,
-235.350049999997));
#193848=CARTESIAN_POINT('Ctrl Pts',(-3.3514772908386,38.8231424750591,-235.35005));
#193849=CARTESIAN_POINT('Ctrl Pts',(-3.37543931947594,40.086677128215,-234.680722248495));
#193850=CARTESIAN_POINT('Ctrl Pts',(-3.30206245560333,39.6476048575096,
-235.350050000005));
#193851=CARTESIAN_POINT('Ctrl Pts',(-3.16954343953211,38.8547460000193,
-235.35005));
#193852=CARTESIAN_POINT('Ctrl Pts',(-3.24615627214412,40.107698597565,-234.680959769804));
#193853=CARTESIAN_POINT('Ctrl Pts',(-3.17558645022547,39.6681405857535,
-235.350050000007));
#193854=CARTESIAN_POINT('Ctrl Pts',(-3.04817458518233,38.8746308506878,
-235.35005));
#193855=CARTESIAN_POINT('Ctrl Pts',(-2.08187343433102,40.2856482090734,
-234.68297582909));
#193856=CARTESIAN_POINT('Ctrl Pts',(-2.03698344603342,39.8419168609564,
-235.350049999946));
#193857=CARTESIAN_POINT('Ctrl Pts',(-1.95514022672127,39.0429654436086,
-235.35005));
#193858=CARTESIAN_POINT('Ctrl Pts',(-1.03992589660121,40.3642807862687,
-234.683880644658));
#193859=CARTESIAN_POINT('Ctrl Pts',(-1.01727787524803,39.9187933007582,
-235.35004999981));
#193860=CARTESIAN_POINT('Ctrl Pts',(-0.976538624615736,39.1173940812476,
-235.35005));
#193861=CARTESIAN_POINT('Ctrl Pts',(1.55890162323515E-9,40.3642807857292,
-234.68388064352));
#193862=CARTESIAN_POINT('Ctrl Pts',(1.00185676570813E-9,39.9187933003983,
-235.35005));
#193863=CARTESIAN_POINT('Ctrl Pts',(-2.25962702508982E-13,39.1173940795976,
-235.35005));
#193864=CARTESIAN_POINT('',(-16.4332022013982,39.4328349445453,-234.711150502351));
#193865=CARTESIAN_POINT('',(-9.39019377446308,39.9042990656516,-234.645334714758));
#193866=CARTESIAN_POINT('Ctrl Pts',(-16.4332022013982,39.4328349445453,
-234.711150502351));
#193867=CARTESIAN_POINT('Ctrl Pts',(-16.3992276324636,39.4408576593895,
-234.711246833797));
#193868=CARTESIAN_POINT('Ctrl Pts',(-16.3607560482782,39.4503671063563,
-234.710664303478));
#193869=CARTESIAN_POINT('Ctrl Pts',(-16.2880944548047,39.4676591916655,
-234.7101449985));
#193870=CARTESIAN_POINT('Ctrl Pts',(-16.1790829189936,39.4932896670378,
-234.709361988129));
#193871=CARTESIAN_POINT('Ctrl Pts',(-15.9245911466271,39.5509439815655,
-234.707507047121));
#193872=CARTESIAN_POINT('Ctrl Pts',(-15.7062385667385,39.5966884073824,
-234.705870653621));
#193873=CARTESIAN_POINT('Ctrl Pts',(-15.2692680789422,39.683314194241,-234.702539239027));
#193874=CARTESIAN_POINT('Ctrl Pts',(-14.9776205594326,39.7345686697748,
-234.70024310695));
#193875=CARTESIAN_POINT('Ctrl Pts',(-14.1016635745331,39.86930023212,-234.693111997869));
#193876=CARTESIAN_POINT('Ctrl Pts',(-13.516248031243,39.9337488812737,-234.688020797378));
#193877=CARTESIAN_POINT('Ctrl Pts',(-12.3424751228906,40.0121804061296,
-234.677117952301));
#193878=CARTESIAN_POINT('Ctrl Pts',(-11.7541027116113,40.0262438052819,
-234.671305171419));
#193879=CARTESIAN_POINT('Ctrl Pts',(-10.8693864701415,40.0093800798719,
-234.662019550443));
#193880=CARTESIAN_POINT('Ctrl Pts',(-10.574107832413,39.997403078896,-234.658827716551));
#193881=CARTESIAN_POINT('Ctrl Pts',(-10.1305567950971,39.9697814600154,
-234.65387955676));
#193882=CARTESIAN_POINT('Ctrl Pts',(-9.98260217772238,39.9589639695816,
-234.65220378061));
#193883=CARTESIAN_POINT('Ctrl Pts',(-9.76053944083152,39.9402973568872,
-234.649654708411));
#193884=CARTESIAN_POINT('Ctrl Pts',(-9.68649604578775,39.9336687262222,
-234.648798971929));
#193885=CARTESIAN_POINT('Ctrl Pts',(-9.53836616196596,39.9195955120497,
-234.647075597267));
#193886=CARTESIAN_POINT('Ctrl Pts',(-9.46288115140502,39.9121528807897,
-234.645933903814));
#193887=CARTESIAN_POINT('Ctrl Pts',(-9.39019377446308,39.9042990656516,
-234.645334714758));
#193888=CARTESIAN_POINT('',(-4.87988937169148E-10,40.3641796532955,-234.68403185425));
#193889=CARTESIAN_POINT('Ctrl Pts',(-9.39019377446308,39.9042990656516,
-234.645334714758));
#193890=CARTESIAN_POINT('Ctrl Pts',(-9.3747535947859,39.9026279267357,-234.64521229516));
#193891=CARTESIAN_POINT('Ctrl Pts',(-9.36241902555493,39.9009373782415,
-234.645694440806));
#193892=CARTESIAN_POINT('Ctrl Pts',(-9.33401274103675,39.8975447406835,
-234.646059912463));
#193893=CARTESIAN_POINT('Ctrl Pts',(-9.31948440688403,39.8958258096469,
-234.646245966043));
#193894=CARTESIAN_POINT('Ctrl Pts',(-9.27590015649556,39.8907177156527,
-234.646801541329));
#193895=CARTESIAN_POINT('Ctrl Pts',(-9.24684499237614,39.8873772511015,
-234.647168477744));
#193896=CARTESIAN_POINT('Ctrl Pts',(-9.15968291175106,39.8775501713831,
-234.648259112729));
#193897=CARTESIAN_POINT('Ctrl Pts',(-9.10157940837895,39.8712578586117,
-234.648972640374));
#193898=CARTESIAN_POINT('Ctrl Pts',(-8.92728571984679,39.8531547210409,
-234.651073746281));
#193899=CARTESIAN_POINT('Ctrl Pts',(-8.81111237470077,39.8421175196824,
-234.652421897223));
#193900=CARTESIAN_POINT('Ctrl Pts',(-7.76582808922892,39.7520042646991,
-234.664105356224));
#193901=CARTESIAN_POINT('Ctrl Pts',(-6.84026733244978,39.737417809177,-234.671316797084));
#193902=CARTESIAN_POINT('Ctrl Pts',(-5.45751451507149,39.8113778773355,
-234.677828559475));
#193903=CARTESIAN_POINT('Ctrl Pts',(-4.9976858845813,39.8520037966934,-234.679290572791));
#193904=CARTESIAN_POINT('Ctrl Pts',(-4.30944352176845,39.9371527902381,
-234.680416520115));
#193905=CARTESIAN_POINT('Ctrl Pts',(-4.0802742669589,39.9695612763832,-234.680616205782));
#193906=CARTESIAN_POINT('Ctrl Pts',(-3.79420511746956,40.015132385667,-234.680645380837));
#193907=CARTESIAN_POINT('Ctrl Pts',(-3.73701094619056,40.024499849226,-234.680640142195));
#193908=CARTESIAN_POINT('Ctrl Pts',(-3.6226642440044,40.0437428584269,-234.680607281209));
#193909=CARTESIAN_POINT('Ctrl Pts',(-3.56919466536356,40.0531714775527,
-234.680497918817));
#193910=CARTESIAN_POINT('Ctrl Pts',(-3.37542267307509,40.0865775195304,
-234.680874073317));
#193911=CARTESIAN_POINT('Ctrl Pts',(-3.24614026173874,40.1075988736087,
-234.681111548481));
#193912=CARTESIAN_POINT('Ctrl Pts',(-2.08186324557725,40.285547494813,-234.683127215862));
#193913=CARTESIAN_POINT('Ctrl Pts',(-1.03992075515157,40.3641796537477,
-234.684031855518));
#193914=CARTESIAN_POINT('Ctrl Pts',(3.8825005278725E-15,40.3641796532956,
-234.68403185425));
#193915=CARTESIAN_POINT('',(-4.88066281613177E-10,39.1173940795976,-235.35005));
#193916=CARTESIAN_POINT('Origin',(-1.46397402467705E-9,39.1173940795976,
-233.85005));
#193917=CARTESIAN_POINT('',(-23.5337713018193,37.7635770079652,-235.35005));
#193918=CARTESIAN_POINT('Ctrl Pts',(-4.88056262071268E-10,39.1173940795976,
-235.35005));
#193919=CARTESIAN_POINT('Ctrl Pts',(-0.356337354408647,39.1173940801907,
-235.35005));
#193920=CARTESIAN_POINT('Ctrl Pts',(-0.712421386489358,39.1074881627783,
-235.35005));
#193921=CARTESIAN_POINT('Ctrl Pts',(-1.06804669090614,39.0877008682734,
-235.35005));
#193922=CARTESIAN_POINT('Ctrl Pts',(-1.42342102172174,39.0679275381532,
-235.35005));
#193923=CARTESIAN_POINT('Ctrl Pts',(-1.77833765771469,39.0382867855085,
-235.35005));
#193924=CARTESIAN_POINT('Ctrl Pts',(-2.13259508534334,38.9987512850576,
-235.35005));
#193925=CARTESIAN_POINT('Ctrl Pts',(-2.3977029451949,38.9691649698663,-235.35005));
#193926=CARTESIAN_POINT('Ctrl Pts',(-2.66244173694949,38.9340362908303,
-235.35005));
#193927=CARTESIAN_POINT('Ctrl Pts',(-2.92672632410968,38.8933347006997,
-235.35005));
#193928=CARTESIAN_POINT('Ctrl Pts',(-2.92737060582729,38.8932354770155,
-235.35005));
#193929=CARTESIAN_POINT('Ctrl Pts',(-2.92801488569497,38.8931362200352,
-235.35005));
#193930=CARTESIAN_POINT('Ctrl Pts',(-2.9286591637141,38.8930369297577,-235.35005));
#193931=CARTESIAN_POINT('Ctrl Pts',(-3.04946230530941,38.8744198466251,
-235.35005));
#193932=CARTESIAN_POINT('Ctrl Pts',(-3.17018687876639,38.8546342346527,
-235.35005));
#193933=CARTESIAN_POINT('Ctrl Pts',(-3.2908326746107,38.8336769884121,-235.35005));
#193934=CARTESIAN_POINT('Ctrl Pts',(-3.35147729175591,38.8231424798055,
-235.35005));
#193935=CARTESIAN_POINT('Ctrl Pts',(-3.41211742901483,38.8125413440661,
-235.35005));
#193936=CARTESIAN_POINT('Ctrl Pts',(-3.47278469039213,38.8023436180629,
-235.35005));
#193937=CARTESIAN_POINT('Ctrl Pts',(-3.53345195207147,38.792145892009,-235.35005));
#193938=CARTESIAN_POINT('Ctrl Pts',(-3.59413684982628,38.7822104632522,
-235.35005));
#193939=CARTESIAN_POINT('Ctrl Pts',(-3.65483931632616,38.7725363318486,
-235.35005));
#193940=CARTESIAN_POINT('Ctrl Pts',(-3.65546036670289,38.7724373552617,
-235.35005));
#193941=CARTESIAN_POINT('Ctrl Pts',(-3.65608141891697,38.7723384060014,
-235.35005));
#193942=CARTESIAN_POINT('Ctrl Pts',(-3.65670247296838,38.7722394840674,
-235.35005));
#193943=CARTESIAN_POINT('Ctrl Pts',(-3.89889272070765,38.7336632479809,
-235.35005));
#193944=CARTESIAN_POINT('Ctrl Pts',(-4.14136237950718,38.6992425871297,
-235.35005));
#193945=CARTESIAN_POINT('Ctrl Pts',(-4.38410921010885,38.6689442097637,
-235.35005));
#193946=CARTESIAN_POINT('Ctrl Pts',(-4.38470863655102,38.668869392521,-235.35005));
#193947=CARTESIAN_POINT('Ctrl Pts',(-4.3853080646873,38.668794600474,-235.35005));
#193948=CARTESIAN_POINT('Ctrl Pts',(-4.38590749451765,38.6687198336225,
-235.35005));
#193949=CARTESIAN_POINT('Ctrl Pts',(-4.87204943971823,38.6080833741381,
-235.35005));
#193950=CARTESIAN_POINT('Ctrl Pts',(-5.3593056525522,38.5640188990606,-235.35005));
#193951=CARTESIAN_POINT('Ctrl Pts',(-5.8476661903511,38.5363791735204,-235.35005));
#193952=CARTESIAN_POINT('Ctrl Pts',(-5.84822203537533,38.5363477143775,
-235.35005));
#193953=CARTESIAN_POINT('Ctrl Pts',(-5.84877788183748,38.5363162764838,
-235.35005));
#193954=CARTESIAN_POINT('Ctrl Pts',(-5.84933372973754,38.5362848598395,
-235.35005));
#193955=CARTESIAN_POINT('Ctrl Pts',(-6.82670834791507,38.4810434337014,
-235.35005));
#193956=CARTESIAN_POINT('Ctrl Pts',(-7.80852886358045,38.4915002286893,
-235.35005));
#193957=CARTESIAN_POINT('Ctrl Pts',(-8.79483412069355,38.5695117626516,
-235.35005));
#193958=CARTESIAN_POINT('Ctrl Pts',(-8.79530155976179,38.5695487346118,
-235.35005));
#193959=CARTESIAN_POINT('Ctrl Pts',(-8.79576899951021,38.5695857217635,
-235.35005));
#193960=CARTESIAN_POINT('Ctrl Pts',(-8.79623643993881,38.5696227241071,
-235.35005));
#193961=CARTESIAN_POINT('Ctrl Pts',(-8.91912763148384,38.5793507275409,
-235.35005));
#193962=CARTESIAN_POINT('Ctrl Pts',(-9.0420658365827,38.5901287540257,-235.35005));
#193963=CARTESIAN_POINT('Ctrl Pts',(-9.16505139013463,38.6019642805906,
-235.35005));
#193964=CARTESIAN_POINT('Ctrl Pts',(-9.22677806664333,38.6079045532363,
-235.35005));
#193965=CARTESIAN_POINT('Ctrl Pts',(-9.28851667261295,38.6141112633977,
-235.35005));
#193966=CARTESIAN_POINT('Ctrl Pts',(-9.35026726349676,38.6205856491488,
-235.35005));
#193967=CARTESIAN_POINT('Ctrl Pts',(-9.38114255892181,38.6238228420226,
-235.35005));
#193968=CARTESIAN_POINT('Ctrl Pts',(-9.41202085071314,38.6271269568751,
-235.35005));
#193969=CARTESIAN_POINT('Ctrl Pts',(-9.44290214664127,38.6304981674401,
-235.35005));
#193970=CARTESIAN_POINT('Ctrl Pts',(-9.45834279459725,38.6321837727217,
-235.35005));
#193971=CARTESIAN_POINT('Ctrl Pts',(-9.47378419360446,38.6338861521134,
-235.35005));
#193972=CARTESIAN_POINT('Ctrl Pts',(-9.48922634467739,38.6356053285559,
-235.35005));
#193973=CARTESIAN_POINT('Ctrl Pts',(-9.50466849574347,38.6373245049977,
-235.35005));
#193974=CARTESIAN_POINT('Ctrl Pts',(-9.5201115320738,38.6390634531904,-235.35005));
#193975=CARTESIAN_POINT('Ctrl Pts',(-9.53555504565915,38.6408130606221,
-235.35005));
#193976=CARTESIAN_POINT('Ctrl Pts',(-9.53599979614812,38.6408634467442,
-235.35005));
#193977=CARTESIAN_POINT('Ctrl Pts',(-9.53644454592807,38.6409138170309,
-235.35005));
#193978=CARTESIAN_POINT('Ctrl Pts',(-9.53688929499903,38.6409641714826,
-235.35005));
#193979=CARTESIAN_POINT('Ctrl Pts',(-9.78353997567394,38.6688899404139,
-235.35005));
#193980=CARTESIAN_POINT('Ctrl Pts',(-10.0299725958919,38.6919454677587,
-235.35005));
#193981=CARTESIAN_POINT('Ctrl Pts',(-10.2761899495318,38.7101931856168,
-235.35005));
#193982=CARTESIAN_POINT('Ctrl Pts',(-10.276610550529,38.7102243572958,-235.35005));
#193983=CARTESIAN_POINT('Ctrl Pts',(-10.2770311508993,38.7102555149728,
-235.35005));
#193984=CARTESIAN_POINT('Ctrl Pts',(-10.2774517506426,38.7102866586477,
-235.35005));
#193985=CARTESIAN_POINT('Ctrl Pts',(-10.7703523229537,38.7467839115718,
-235.35005));
#193986=CARTESIAN_POINT('Ctrl Pts',(-11.2623919369706,38.7640519886334,
-235.35005));
#193987=CARTESIAN_POINT('Ctrl Pts',(-11.7535889208686,38.7625005477271,
-235.35005));
#193988=CARTESIAN_POINT('Ctrl Pts',(-11.7539614951304,38.7624993709549,
-235.35005));
#193989=CARTESIAN_POINT('Ctrl Pts',(-11.7543340689085,38.7624981833791,
-235.35005));
#193990=CARTESIAN_POINT('Ctrl Pts',(-11.7547066422029,38.7624969849996,
-235.35005));
#193991=CARTESIAN_POINT('Ctrl Pts',(-12.7375637756362,38.7593356316055,
-235.35005));
#193992=CARTESIAN_POINT('Ctrl Pts',(-13.717054647793,38.6809905735713,-235.35005));
#193993=CARTESIAN_POINT('Ctrl Pts',(-14.6931353852465,38.5264823709591,
-235.35005));
#193994=CARTESIAN_POINT('Ctrl Pts',(-14.6934128886607,38.5264384436977,
-235.35005));
#193995=CARTESIAN_POINT('Ctrl Pts',(-14.6936903917976,38.5263945102443,
-235.35005));
#193996=CARTESIAN_POINT('Ctrl Pts',(-14.6939678946573,38.5263505705987,
-235.35005));
#193997=CARTESIAN_POINT('Ctrl Pts',(-14.9378025765395,38.4877419252278,
-235.35005));
#193998=CARTESIAN_POINT('Ctrl Pts',(-15.1814232314178,38.4443525285445,
-235.35005));
#193999=CARTESIAN_POINT('Ctrl Pts',(-15.4248261118799,38.3960995538484,
-235.35005));
#194000=CARTESIAN_POINT('Ctrl Pts',(-15.5466660626659,38.3719456077197,
-235.35005));
#194001=CARTESIAN_POINT('Ctrl Pts',(-15.6684514489775,38.3465730677093,
-235.35005));
#194002=CARTESIAN_POINT('Ctrl Pts',(-15.7901818202738,38.3199719794952,
-235.35005));
#194003=CARTESIAN_POINT('Ctrl Pts',(-15.8510470114032,38.3066714341903,
-235.35005));
#194004=CARTESIAN_POINT('Ctrl Pts',(-15.9118984489941,38.2930637564789,
-235.35005));
#194005=CARTESIAN_POINT('Ctrl Pts',(-15.9727360779946,38.2791477303716,
-235.35005));
#194006=CARTESIAN_POINT('Ctrl Pts',(-16.0031548943984,38.2721897168825,
-235.35005));
#194007=CARTESIAN_POINT('Ctrl Pts',(-16.0335702586684,38.2651546166131,
-235.35005));
#194008=CARTESIAN_POINT('Ctrl Pts',(-16.0639821640006,38.2580422793406,
-235.35005));
#194009=CARTESIAN_POINT('Ctrl Pts',(-16.0791881172091,38.2544861105775,
-235.35005));
#194010=CARTESIAN_POINT('Ctrl Pts',(-16.0943932056889,38.2509106325926,
-235.35005));
#194011=CARTESIAN_POINT('Ctrl Pts',(-16.1095974285865,38.2473158267122,
-235.35005));
#194012=CARTESIAN_POINT('Ctrl Pts',(-16.1248016518712,38.2437210207403,
-235.35005));
#194013=CARTESIAN_POINT('Ctrl Pts',(-16.1400046170681,38.2400982079978,
-235.35005));
#194014=CARTESIAN_POINT('Ctrl Pts',(-16.1552076184638,38.2364760331285,
-235.35005));
#194015=CARTESIAN_POINT('Ctrl Pts',(-16.1554380521512,38.2364211313963,
-235.35005));
#194016=CARTESIAN_POINT('Ctrl Pts',(-16.1556684860895,38.2363662335797,
-235.35005));
#194017=CARTESIAN_POINT('Ctrl Pts',(-16.1558989202786,38.2363113396788,
-235.35005));
#194018=CARTESIAN_POINT('Ctrl Pts',(-16.6421654926102,38.1204731945478,
-235.35005));
#194019=CARTESIAN_POINT('Ctrl Pts',(-17.12954963108,38.0220712232547,-235.35005));
#194020=CARTESIAN_POINT('Ctrl Pts',(-17.618016277175,37.9405600315694,-235.35005));
#194021=CARTESIAN_POINT('Ctrl Pts',(-17.6182014585966,37.9405291300565,
-235.35005));
#194022=CARTESIAN_POINT('Ctrl Pts',(-17.6183866401739,37.9404982309351,
-235.35005));
#194023=CARTESIAN_POINT('Ctrl Pts',(-17.6185718219071,37.9404673342052,
-235.35005));
#194024=CARTESIAN_POINT('Ctrl Pts',(-18.5958771217091,37.7774083899232,
-235.35005));
#194025=CARTESIAN_POINT('Ctrl Pts',(-19.5774518164939,37.6809633951768,
-235.35005));
#194026=CARTESIAN_POINT('Ctrl Pts',(-20.5633123297537,37.6513870472257,
-235.35005));
#194027=CARTESIAN_POINT('Ctrl Pts',(-21.5491728430134,37.6218106992746,
-235.35005));
#194028=CARTESIAN_POINT('Ctrl Pts',(-22.5393191900798,37.6591029589903,
-235.35005));
#194029=CARTESIAN_POINT('Ctrl Pts',(-23.5337713018193,37.7635770079652,
-235.35005));
#194030=CARTESIAN_POINT('',(-23.3965311730466,39.0699180248394,-234.574369193924));
#194031=CARTESIAN_POINT('Origin',(-23.5337713018193,37.7635770079652,-233.85005));
#194032=CARTESIAN_POINT('Ctrl Pts',(-23.3965311730097,39.0699180251917,
-234.574369193282));
#194033=CARTESIAN_POINT('Ctrl Pts',(-22.2279621072998,38.927851533746,-234.609178040102));
#194034=CARTESIAN_POINT('Ctrl Pts',(-20.4798185422076,38.8660796071235,
-234.651026311726));
#194035=CARTESIAN_POINT('Ctrl Pts',(-18.7417049717577,39.032269945489,-234.680423055754));
#194036=CARTESIAN_POINT('Ctrl Pts',(-17.8745669582133,39.1534396965386,
-234.693304161216));
#194037=CARTESIAN_POINT('Ctrl Pts',(-17.5858370342812,39.2001485327806,
-234.697297627868));
#194038=CARTESIAN_POINT('Ctrl Pts',(-17.0451048369348,39.2999745776045,
-234.704218024849));
#194039=CARTESIAN_POINT('Ctrl Pts',(-16.7930294294645,39.351547020454,-234.70721839636));
#194040=CARTESIAN_POINT('Ctrl Pts',(-16.5052918362263,39.4162808271944,
-234.710395408776));
#194041=CARTESIAN_POINT('Ctrl Pts',(-16.4710147540983,39.4239043905358,
-234.71104178217));
#194042=CARTESIAN_POINT('Ctrl Pts',(-16.4332022013982,39.4328349445453,
-234.711150502351));
#194043=CARTESIAN_POINT('Ctrl Pts',(-23.5337713018193,37.7635770079652,
-235.35005));
#194044=CARTESIAN_POINT('Ctrl Pts',(-23.4412215482421,38.6445258986454,
-235.35005));
#194045=CARTESIAN_POINT('Ctrl Pts',(-23.3965311730093,39.0699180251918,
-234.574369193281));
#194046=CARTESIAN_POINT('Ctrl Pts',(-23.6412313452744,37.7748664312125,
-235.35005));
#194047=CARTESIAN_POINT('Ctrl Pts',(-23.6100297261144,38.6346548826691,
-235.35005));
#194048=CARTESIAN_POINT('Ctrl Pts',(-23.5947564504146,39.0708169807221,
-234.610306553998));
#194049=CARTESIAN_POINT('Ctrl Pts',(-23.7487418755492,37.7752275005428,
-235.35005));
#194050=CARTESIAN_POINT('Ctrl Pts',(-23.778719103045,38.6109201787134,-235.35005));
#194051=CARTESIAN_POINT('Ctrl Pts',(-23.7949692188817,39.052344777689,-234.642115924617));
#194052=CARTESIAN_POINT('Ctrl Pts',(-23.8561664752437,37.7630917536255,
-235.35005));
#194053=CARTESIAN_POINT('Ctrl Pts',(-23.9474058055444,38.5707334611873,
-235.35005));
#194054=CARTESIAN_POINT('Ctrl Pts',(-23.9972286658429,39.0117605909835,
-234.669151698811));
#194055=CARTESIAN_POINT('',(-23.997228665843,39.0117605909833,-234.669151698811));
#194056=CARTESIAN_POINT('',(-23.8561664752437,37.7630917536256,-235.35005));
#194057=CARTESIAN_POINT('Origin',(-23.8561664752439,37.7630917536255,-233.85005));
#194058=CARTESIAN_POINT('Ctrl Pts',(-23.9972286658434,39.0117605909834,
-234.669151698811));
#194059=CARTESIAN_POINT('Ctrl Pts',(-23.7949692188817,39.052344777689,-234.642115924617));
#194060=CARTESIAN_POINT('Ctrl Pts',(-23.5947564504146,39.0708169807221,
-234.610306553998));
#194061=CARTESIAN_POINT('Ctrl Pts',(-23.3965311730097,39.0699180251917,
-234.574369193282));
#194062=CARTESIAN_POINT('Ctrl Pts',(-23.5337713018193,37.7635770079652,
-235.35005));
#194063=CARTESIAN_POINT('Ctrl Pts',(-23.6412535989187,37.7748687641791,
-235.35005));
#194064=CARTESIAN_POINT('Ctrl Pts',(-23.7487194439798,37.7752300509467,
-235.35005));
#194065=CARTESIAN_POINT('Ctrl Pts',(-23.8561664752437,37.7630917536256,
-235.35005));
#194066=CARTESIAN_POINT('Ctrl Pts',(-23.8561664752439,37.7630917536255,
-235.35005));
#194067=CARTESIAN_POINT('Ctrl Pts',(-23.9474058055448,38.5707334611872,
-235.35005));
#194068=CARTESIAN_POINT('Ctrl Pts',(-23.9972286658434,39.0117605909834,
-234.669151698811));
#194069=CARTESIAN_POINT('Ctrl Pts',(-25.0882853750842,37.6238992104159,
-235.35005));
#194070=CARTESIAN_POINT('Ctrl Pts',(-25.1842887597299,38.431109053993,-235.350049999742));
#194071=CARTESIAN_POINT('Ctrl Pts',(-25.2366484173464,38.8718330388058,
-234.669014852156));
#194072=CARTESIAN_POINT('Ctrl Pts',(-26.319091123968,37.47392953931,-235.35005));
#194073=CARTESIAN_POINT('Ctrl Pts',(-26.4198403391809,38.280686857661,-235.35005000043));
#194074=CARTESIAN_POINT('Ctrl Pts',(-26.4747606339603,38.7210799284767,
-234.668852342857));
#194075=CARTESIAN_POINT('Ctrl Pts',(-27.5485779004777,37.3131372941855,
-235.35005));
#194076=CARTESIAN_POINT('Ctrl Pts',(-27.654024085186,38.1194242486926,-235.35005));
#194077=CARTESIAN_POINT('Ctrl Pts',(-27.711570814231,38.5594513301076,-234.668667513818));
#194078=CARTESIAN_POINT('',(-27.7115708142298,38.5594513301044,-234.66866751382));
#194079=CARTESIAN_POINT('',(-27.5485779004777,37.3131372941855,-235.35005));
#194080=CARTESIAN_POINT('Origin',(-27.5485779004728,37.3131372941843,-233.850050000003));
#194081=CARTESIAN_POINT('Origin',(-0.0438186590672052,-173.169156331663,
-234.199437903576));
#194082=CARTESIAN_POINT('Origin',(-0.0633608499784,-172.860463397816,-235.350049999539));
#194083=CARTESIAN_POINT('Ctrl Pts',(-27.5485779004728,37.3131372941862,
-235.35005));
#194084=CARTESIAN_POINT('Ctrl Pts',(-27.654024085184,38.1194242486908,-235.35005));
#194085=CARTESIAN_POINT('Ctrl Pts',(-27.7115708142308,38.559451330106,-234.66866751382));
#194086=CARTESIAN_POINT('Ctrl Pts',(-27.6119495440962,37.3048495676945,
-235.35005));
#194087=CARTESIAN_POINT('Ctrl Pts',(-27.7265642955278,38.1035833263501,
-235.350049999996));
#194088=CARTESIAN_POINT('Ctrl Pts',(-27.7898688006155,38.543857161573,-234.676819323508));
#194089=CARTESIAN_POINT('Ctrl Pts',(-27.6750964089389,37.2953595442226,
-235.35005));
#194090=CARTESIAN_POINT('Ctrl Pts',(-27.803498135569,38.0832505563202,-235.350049999997));
#194091=CARTESIAN_POINT('Ctrl Pts',(-27.8754619604023,38.52353948073,-234.688258517325));
#194092=CARTESIAN_POINT('Ctrl Pts',(-27.7691733848276,37.2776980879525,
-235.35005));
#194093=CARTESIAN_POINT('Ctrl Pts',(-27.9226851009708,38.0444330714304,
-235.350050000001));
#194094=CARTESIAN_POINT('Ctrl Pts',(-28.0106528477426,38.4835354389051,
-234.709081676005));
#194095=CARTESIAN_POINT('Ctrl Pts',(-27.8004215724929,37.2712202551586,
-235.35005));
#194096=CARTESIAN_POINT('Ctrl Pts',(-27.962669518358,38.0303893933949,-235.350049999995));
#194097=CARTESIAN_POINT('Ctrl Pts',(-28.0564170190361,38.4688219126267,
-234.716327424367));
#194098=CARTESIAN_POINT('Ctrl Pts',(-27.8627200032187,37.2572093770216,
-235.35005));
#194099=CARTESIAN_POINT('Ctrl Pts',(-28.0390618914339,38.0040014727884,
-235.350050000004));
#194100=CARTESIAN_POINT('Ctrl Pts',(-28.1423078435221,38.4410402419925,
-234.727885440078));
#194101=CARTESIAN_POINT('Ctrl Pts',(-27.8937776977631,37.249697476023,-235.35005));
#194102=CARTESIAN_POINT('Ctrl Pts',(-28.07508312287,37.9920997651976,-235.350050000001));
#194103=CARTESIAN_POINT('Ctrl Pts',(-28.1816910211067,38.4285212429546,
-234.731834361418));
#194104=CARTESIAN_POINT('Ctrl Pts',(-27.9867858054616,37.226404790223,-235.35005));
#194105=CARTESIAN_POINT('Ctrl Pts',(-28.1793531401323,37.9589854504683,
-235.350049999998));
#194106=CARTESIAN_POINT('Ctrl Pts',(-28.2937808316253,38.3938810745564,
-234.740558887245));
#194107=CARTESIAN_POINT('Ctrl Pts',(-28.0485551598146,37.2098945175254,
-235.35005));
#194108=CARTESIAN_POINT('Ctrl Pts',(-28.251028133496,37.9337425924481,-235.35004999998));
#194109=CARTESIAN_POINT('Ctrl Pts',(-28.3724365366315,38.3671595974566,
-234.748243384598));
#194110=CARTESIAN_POINT('Ctrl Pts',(-28.1402497418155,37.1819908028498,
-235.35005));
#194111=CARTESIAN_POINT('Ctrl Pts',(-28.3633757810457,37.8864187374528,
-235.35005000001));
#194112=CARTESIAN_POINT('Ctrl Pts',(-28.499410390972,38.315752826462,-234.764279480932));
#194113=CARTESIAN_POINT('Ctrl Pts',(-28.1706617267493,37.1721527193585,
-235.35005));
#194114=CARTESIAN_POINT('Ctrl Pts',(-28.4004253047465,37.8701990320713,
-235.350049999998));
#194115=CARTESIAN_POINT('Ctrl Pts',(-28.541281614628,38.2980250294177,-234.769400544257));
#194116=CARTESIAN_POINT('Ctrl Pts',(-28.2311847426228,37.1515938768492,
-235.35005));
#194117=CARTESIAN_POINT('Ctrl Pts',(-28.4719778581327,37.8390215876304,
-235.350050000002));
#194118=CARTESIAN_POINT('Ctrl Pts',(-28.6209241135967,38.2641359479009,
-234.77768479838));
#194119=CARTESIAN_POINT('Ctrl Pts',(-28.2612972505945,37.1409013962204,
-235.35005));
#194120=CARTESIAN_POINT('Ctrl Pts',(-28.5064923453729,37.824118998956,-235.350049999988));
#194121=CARTESIAN_POINT('Ctrl Pts',(-28.6586684014758,38.248067198284,-234.780840885022));
#194122=CARTESIAN_POINT('Ctrl Pts',(-28.3512820909987,37.1078462406674,
-235.35005));
#194123=CARTESIAN_POINT('Ctrl Pts',(-28.6091714812706,37.7788267124199,
-235.350050000025));
#194124=CARTESIAN_POINT('Ctrl Pts',(-28.7708554177228,38.1992011674236,
-234.789873968856));
#194125=CARTESIAN_POINT('Ctrl Pts',(-28.4108519482495,37.0845842971443,
-235.35005));
#194126=CARTESIAN_POINT('Ctrl Pts',(-28.6757355642658,37.7490178712301,
-235.350049999991));
#194127=CARTESIAN_POINT('Ctrl Pts',(-28.8426158139035,38.1672985579224,
-234.794421341942));
#194128=CARTESIAN_POINT('Ctrl Pts',(-28.5284852992461,37.0351888006413,
-235.35005));
#194129=CARTESIAN_POINT('Ctrl Pts',(-28.8128694279278,37.6793814787632,
-235.350050000009));
#194130=CARTESIAN_POINT('Ctrl Pts',(-28.9946891933229,38.0909484466884,
-234.808461686233));
#194131=CARTESIAN_POINT('Ctrl Pts',(-28.5864462918562,37.0087322113245,
-235.35005));
#194132=CARTESIAN_POINT('Ctrl Pts',(-28.8808495685014,37.641668601605,-235.350050000012));
#194133=CARTESIAN_POINT('Ctrl Pts',(-29.0705233204497,38.0492577914762,
-234.816069500032));
#194134=CARTESIAN_POINT('Ctrl Pts',(-28.6725892746692,36.9674060120273,
-235.35005));
#194135=CARTESIAN_POINT('Ctrl Pts',(-28.9759803010192,37.5902912511275,
-235.350049999993));
#194136=CARTESIAN_POINT('Ctrl Pts',(-29.1727005271663,37.9941274022379,
-234.822565471198));
#194137=CARTESIAN_POINT('Ctrl Pts',(-28.7011808463655,36.9533782896452,
-235.35005));
#194138=CARTESIAN_POINT('Ctrl Pts',(-29.0070493823103,37.5734789125125,
-235.350049999995));
#194139=CARTESIAN_POINT('Ctrl Pts',(-29.2057300258169,37.9762393089045,
-234.824326831928));
#194140=CARTESIAN_POINT('Ctrl Pts',(-28.7439306930081,36.9320540547938,
-235.35005));
#194141=CARTESIAN_POINT('Ctrl Pts',(-29.0531052906671,37.5484365661045,
-235.350050000003));
#194142=CARTESIAN_POINT('Ctrl Pts',(-29.2544014035152,37.9497400570338,
-234.826647318416));
#194143=CARTESIAN_POINT('Ctrl Pts',(-28.7581616928441,36.9249070270844,
-235.35005));
#194144=CARTESIAN_POINT('Ctrl Pts',(-29.0681955001819,37.5403535418641,
-235.350050000002));
#194145=CARTESIAN_POINT('Ctrl Pts',(-29.2701706937271,37.9412800343878,
-234.827215664254));
#194146=CARTESIAN_POINT('Ctrl Pts',(-28.7865561585441,36.9104741568002,
-235.35005));
#194147=CARTESIAN_POINT('Ctrl Pts',(-29.100049296179,37.5217456532107,-235.350049999998));
#194148=CARTESIAN_POINT('Ctrl Pts',(-29.3048419252274,37.921051821916,-234.829913631261));
#194149=CARTESIAN_POINT('Ctrl Pts',(-28.8007140683774,36.9031768938705,
-235.35005));
#194150=CARTESIAN_POINT('Ctrl Pts',(-29.1166642642298,37.5113826540724,
-235.350049999998));
#194151=CARTESIAN_POINT('Ctrl Pts',(-29.3234878417255,37.9094999507468,
-234.831922289268));
#194152=CARTESIAN_POINT('Ctrl Pts',(-28.8711899004085,36.866045739172,-235.35005));
#194153=CARTESIAN_POINT('Ctrl Pts',(-29.2004368662993,37.4572474244772,
-235.350050000008));
#194154=CARTESIAN_POINT('Ctrl Pts',(-29.4185209864353,37.8485528906136,
-234.842993006465));
#194155=CARTESIAN_POINT('Ctrl Pts',(-28.9265109080764,36.8341627598888,
-235.35005));
#194156=CARTESIAN_POINT('Ctrl Pts',(-29.2654910265155,37.4132275967966,
-235.350050000058));
#194157=CARTESIAN_POINT('Ctrl Pts',(-29.4914664732662,37.799141309411,-234.849921198629));
#194158=CARTESIAN_POINT('Ctrl Pts',(-28.9814172171127,36.8014272692485,
-235.35005));
#194159=CARTESIAN_POINT('Ctrl Pts',(-29.3235739752808,37.3753174315542,
-235.35005));
#194160=CARTESIAN_POINT('Ctrl Pts',(-29.5524353619884,37.759180369309,-234.853368133768));
#194161=CARTESIAN_POINT('',(-29.5524353619882,37.7591803693089,-234.853368133768));
#194162=CARTESIAN_POINT('',(-28.9814172171126,36.8014272692484,-235.35005));
#194163=CARTESIAN_POINT('Origin',(-28.9814172171126,36.8014272692485,-233.85005));
#194164=CARTESIAN_POINT('Ctrl Pts',(-29.5524353619882,37.7591803693089,
-234.853368133768));
#194165=CARTESIAN_POINT('Ctrl Pts',(-29.4914664732662,37.799141309411,-234.849921198629));
#194166=CARTESIAN_POINT('Ctrl Pts',(-29.4185209864353,37.8485528906136,
-234.842993006465));
#194167=CARTESIAN_POINT('Ctrl Pts',(-29.3234878417255,37.9094999507468,
-234.831922289268));
#194168=CARTESIAN_POINT('Ctrl Pts',(-29.3048419252274,37.921051821916,-234.829913631261));
#194169=CARTESIAN_POINT('Ctrl Pts',(-29.2701706937271,37.9412800343878,
-234.827215664254));
#194170=CARTESIAN_POINT('Ctrl Pts',(-29.2544014035152,37.9497400570338,
-234.826647318416));
#194171=CARTESIAN_POINT('Ctrl Pts',(-29.2057300258169,37.9762393089045,
-234.824326831928));
#194172=CARTESIAN_POINT('Ctrl Pts',(-29.1727005271663,37.9941274022379,
-234.822565471198));
#194173=CARTESIAN_POINT('Ctrl Pts',(-29.0705233204497,38.0492577914762,
-234.816069500032));
#194174=CARTESIAN_POINT('Ctrl Pts',(-28.9946891933229,38.0909484466884,
-234.808461686233));
#194175=CARTESIAN_POINT('Ctrl Pts',(-28.8426158139035,38.1672985579224,
-234.794421341942));
#194176=CARTESIAN_POINT('Ctrl Pts',(-28.7708554177228,38.1992011674236,
-234.789873968856));
#194177=CARTESIAN_POINT('Ctrl Pts',(-28.6586684014758,38.248067198284,-234.780840885022));
#194178=CARTESIAN_POINT('Ctrl Pts',(-28.6209241135967,38.2641359479009,
-234.77768479838));
#194179=CARTESIAN_POINT('Ctrl Pts',(-28.541281614628,38.2980250294177,-234.769400544257));
#194180=CARTESIAN_POINT('Ctrl Pts',(-28.499410390972,38.315752826462,-234.764279480932));
#194181=CARTESIAN_POINT('Ctrl Pts',(-28.3724365366315,38.3671595974566,
-234.748243384598));
#194182=CARTESIAN_POINT('Ctrl Pts',(-28.2937808316253,38.3938810745564,
-234.740558887245));
#194183=CARTESIAN_POINT('Ctrl Pts',(-28.1816910211067,38.4285212429546,
-234.731834361418));
#194184=CARTESIAN_POINT('Ctrl Pts',(-28.1423078435221,38.4410402419925,
-234.727885440078));
#194185=CARTESIAN_POINT('Ctrl Pts',(-28.0564170190361,38.4688219126267,
-234.716327424367));
#194186=CARTESIAN_POINT('Ctrl Pts',(-28.0106528477426,38.4835354389051,
-234.709081676005));
#194187=CARTESIAN_POINT('Ctrl Pts',(-27.8754619604023,38.52353948073,-234.688258517325));
#194188=CARTESIAN_POINT('Ctrl Pts',(-27.7898688006155,38.543857161573,-234.676819323508));
#194189=CARTESIAN_POINT('Ctrl Pts',(-27.7115708142298,38.5594513301044,
-234.66866751382));
#194190=CARTESIAN_POINT('Ctrl Pts',(-27.5485779004777,37.3131372941856,
-235.35005));
#194191=CARTESIAN_POINT('Ctrl Pts',(-27.6119497053713,37.3048495466029,
-235.35005));
#194192=CARTESIAN_POINT('Ctrl Pts',(-27.6750965458531,37.2953595193401,
-235.35005));
#194193=CARTESIAN_POINT('Ctrl Pts',(-27.7378143932095,37.2835852418792,
-235.35005));
#194194=CARTESIAN_POINT('Ctrl Pts',(-27.7691734109443,37.2776980854911,
-235.35005));
#194195=CARTESIAN_POINT('Ctrl Pts',(-27.8004215957617,37.2712202529943,
-235.35005));
#194196=CARTESIAN_POINT('Ctrl Pts',(-27.8315707886446,37.2642148195972,
-235.35005));
#194197=CARTESIAN_POINT('Ctrl Pts',(-27.8627200211639,37.257209377286,-235.35005));
#194198=CARTESIAN_POINT('Ctrl Pts',(-27.8937777129896,37.2496974771633,
-235.35005));
#194199=CARTESIAN_POINT('Ctrl Pts',(-27.9247804016332,37.2419332526298,
-235.35005));
#194200=CARTESIAN_POINT('Ctrl Pts',(-27.9867858296455,37.2264047908593,
-235.35005));
#194201=CARTESIAN_POINT('Ctrl Pts',(-28.0485551618066,37.2098945246507,
-235.35005));
#194202=CARTESIAN_POINT('Ctrl Pts',(-28.1096848833639,37.191292048355,-235.35005));
#194203=CARTESIAN_POINT('Ctrl Pts',(-28.1402497358115,37.1819908127424,
-235.35005));
#194204=CARTESIAN_POINT('Ctrl Pts',(-28.1706617181454,37.1721527303683,
-235.35005));
#194205=CARTESIAN_POINT('Ctrl Pts',(-28.2009232370621,37.1618733050988,
-235.35005));
#194206=CARTESIAN_POINT('Ctrl Pts',(-28.2311847284776,37.151593889171,-235.35005));
#194207=CARTESIAN_POINT('Ctrl Pts',(-28.2612972337605,37.1409014094734,
-235.35005));
#194208=CARTESIAN_POINT('Ctrl Pts',(-28.2912921994267,37.129883016559,-235.35005));
#194209=CARTESIAN_POINT('Ctrl Pts',(-28.3512820882545,37.1078462463438,
-235.35005));
#194210=CARTESIAN_POINT('Ctrl Pts',(-28.4108519466395,37.0845843013711,
-235.35005));
#194211=CARTESIAN_POINT('Ctrl Pts',(-28.4696686246939,37.0598865511459,
-235.35005));
#194212=CARTESIAN_POINT('Ctrl Pts',(-28.5284852999082,37.0351888021132,
-235.35005));
#194213=CARTESIAN_POINT('Ctrl Pts',(-28.5864462936913,37.0087322116309,
-235.35005));
#194214=CARTESIAN_POINT('Ctrl Pts',(-28.6438749473726,36.9811814124344,
-235.35005));
#194215=CARTESIAN_POINT('Ctrl Pts',(-28.6725892757669,36.9674060120908,
-235.35005));
#194216=CARTESIAN_POINT('Ctrl Pts',(-28.7011808475711,36.9533782894892,
-235.35005));
#194217=CARTESIAN_POINT('Ctrl Pts',(-28.7296807442605,36.9391621333448,
-235.35005));
#194218=CARTESIAN_POINT('Ctrl Pts',(-28.7439306934412,36.9320540548556,
-235.35005));
#194219=CARTESIAN_POINT('Ctrl Pts',(-28.7581616932791,36.9249070270955,
-235.35005));
#194220=CARTESIAN_POINT('Ctrl Pts',(-28.7723589257722,36.9176905920959,
-235.35005));
#194221=CARTESIAN_POINT('Ctrl Pts',(-28.7865561589916,36.9104741567272,
-235.35005));
#194222=CARTESIAN_POINT('Ctrl Pts',(-28.8007140688312,36.9031768937556,
-235.350049999999));
#194223=CARTESIAN_POINT('Ctrl Pts',(-28.8148092348245,36.8957506630084,
-235.350049999999));
#194224=CARTESIAN_POINT('Ctrl Pts',(-28.8711899085552,36.8660457348789,
-235.35005));
#194225=CARTESIAN_POINT('Ctrl Pts',(-28.9265109173313,36.834162754371,-235.35005));
#194226=CARTESIAN_POINT('Ctrl Pts',(-28.9814172171126,36.8014272692486,
-235.35005));
#194227=CARTESIAN_POINT('Ctrl Pts',(-28.6235999918556,37.0129901885974,
-235.35005));
#194228=CARTESIAN_POINT('Ctrl Pts',(-28.9622480552984,37.5906356762342,
-235.350050000051));
#194229=CARTESIAN_POINT('Ctrl Pts',(-29.1883500929521,37.9763249213013,
-234.851571244636));
#194230=CARTESIAN_POINT('Ctrl Pts',(-30.6324251188938,35.835135935805,-235.35005));
#194231=CARTESIAN_POINT('Ctrl Pts',(-30.988382838386,36.3951824447949,-235.350049999742));
#194232=CARTESIAN_POINT('Ctrl Pts',(-31.2333771101203,36.7689146204159,
-234.859578762431));
#194233=CARTESIAN_POINT('Ctrl Pts',(-32.5473006228093,34.546799247056,-235.35005));
#194234=CARTESIAN_POINT('Ctrl Pts',(-32.9234562736393,35.0863223646416,
-235.350049999872));
#194235=CARTESIAN_POINT('Ctrl Pts',(-33.1818988153925,35.4495637346705,
-234.86713813913));
#194236=CARTESIAN_POINT('Ctrl Pts',(-36.0822840599884,31.8353365675869,
-235.35005));
#194237=CARTESIAN_POINT('Ctrl Pts',(-36.4952941667597,32.3353752136231,
-235.35005000012));
#194238=CARTESIAN_POINT('Ctrl Pts',(-36.7813559352307,32.6757871555092,
-234.878086065553));
#194239=CARTESIAN_POINT('Ctrl Pts',(-37.7150530376205,30.426874953249,-235.35005));
#194240=CARTESIAN_POINT('Ctrl Pts',(-38.145619897874,30.908582788892,-235.35004999988));
#194241=CARTESIAN_POINT('Ctrl Pts',(-38.4423674553364,31.2390085277979,
-234.881236143903));
#194242=CARTESIAN_POINT('Ctrl Pts',(-40.0413171754775,28.170164696784,-235.35005));
#194243=CARTESIAN_POINT('Ctrl Pts',(-40.498678297905,28.6233702148686,-235.35005000006));
#194244=CARTESIAN_POINT('Ctrl Pts',(-40.8139548555995,28.9354139317848,
-234.883441337666));
#194245=CARTESIAN_POINT('Ctrl Pts',(-40.7957050001434,27.3932780662659,
-235.35005));
#194246=CARTESIAN_POINT('Ctrl Pts',(-41.2617903522464,27.8372407096767,
-235.35005));
#194247=CARTESIAN_POINT('Ctrl Pts',(-41.5829037502019,28.1432199774246,
-234.883656797018));
#194248=CARTESIAN_POINT('Ctrl Pts',(-42.2637158381442,25.7917312522435,
-235.35005));
#194249=CARTESIAN_POINT('Ctrl Pts',(-42.7468027345624,26.2176715878726,
-235.35005));
#194250=CARTESIAN_POINT('Ctrl Pts',(-43.079491346636,26.5111087013005,-234.883221890728));
#194251=CARTESIAN_POINT('Ctrl Pts',(-42.9787004139624,24.9654368934267,
-235.35005));
#194252=CARTESIAN_POINT('Ctrl Pts',(-43.4703807122323,25.3822490016404,
-235.35005));
#194253=CARTESIAN_POINT('Ctrl Pts',(-43.8085884283688,25.6694567559007,
-234.88257445635));
#194254=CARTESIAN_POINT('Ctrl Pts',(-45.1373606477486,22.3164313732977,
-235.35005));
#194255=CARTESIAN_POINT('Ctrl Pts',(-45.6568207031231,22.7034238305282,
-235.35005));
#194256=CARTESIAN_POINT('Ctrl Pts',(-46.0121606676539,22.9702919294327,
-234.879269810321));
#194257=CARTESIAN_POINT('Ctrl Pts',(-46.4872712478119,20.4281942415639,
-235.350050000001));
#194258=CARTESIAN_POINT('Ctrl Pts',(-47.0253273852194,20.7945808946792,
-235.350049999074));
#194259=CARTESIAN_POINT('Ctrl Pts',(-47.391560949626,21.047345630817,-234.875206256712));
#194260=CARTESIAN_POINT('Ctrl Pts',(-47.7222658457636,18.4560958919691,
-235.350050000001));
#194261=CARTESIAN_POINT('Ctrl Pts',(-48.2758175822674,18.8027406871144,
-235.350050000176));
#194262=CARTESIAN_POINT('Ctrl Pts',(-48.6529331431024,19.0388789631468,
-234.871921744022));
#194263=CARTESIAN_POINT('',(-48.4260896922586,19.3965417854656,-234.872874618363));
#194264=CARTESIAN_POINT('',(-47.5004483343782,18.8074595529612,-235.35005));
#194265=CARTESIAN_POINT('Origin',(-47.5004483343794,18.8074595529594,-233.85005));
#194266=CARTESIAN_POINT('Ctrl Pts',(-48.4260896922585,19.3965417854656,
-234.872874618363));
#194267=CARTESIAN_POINT('Ctrl Pts',(-48.2336681176016,19.6980174947172,
-234.873382411966));
#194268=CARTESIAN_POINT('Ctrl Pts',(-48.0384640363657,19.9976369248559,
-234.873904410919));
#194269=CARTESIAN_POINT('Ctrl Pts',(-47.8405525939515,20.295311591735,-234.874431710577));
#194270=CARTESIAN_POINT('Ctrl Pts',(-47.6376543543754,20.6004868011085,
-234.874972296665));
#194271=CARTESIAN_POINT('Ctrl Pts',(-47.4319106874047,20.9036183295806,
-234.875518453947));
#194272=CARTESIAN_POINT('Ctrl Pts',(-47.2233678006824,21.2046536835508,
-234.876060587562));
#194273=CARTESIAN_POINT('Ctrl Pts',(-47.0069805666097,21.5170124919834,
-234.87662311355));
#194274=CARTESIAN_POINT('Ctrl Pts',(-46.7875797475729,21.82711474811,-234.877181307477));
#194275=CARTESIAN_POINT('Ctrl Pts',(-46.5651778092407,22.1349427753502,
-234.87772445051));
#194276=CARTESIAN_POINT('Ctrl Pts',(-46.338367265686,22.4488727829,-234.878278360099));
#194277=CARTESIAN_POINT('Ctrl Pts',(-46.1084355256474,22.760437932076,-234.878816616181));
#194278=CARTESIAN_POINT('Ctrl Pts',(-45.8753539608744,23.0696556340549,
-234.879327849776));
#194279=CARTESIAN_POINT('Ctrl Pts',(-45.6359567474781,23.387251992474,-234.87985293591));
#194280=CARTESIAN_POINT('Ctrl Pts',(-45.3932368521758,23.7023723875432,
-234.880349515298));
#194281=CARTESIAN_POINT('Ctrl Pts',(-45.1471176554437,24.0150669690212,
-234.880805269517));
#194282=CARTESIAN_POINT('Ctrl Pts',(-45.0039085531397,24.1970142161412,
-234.881070458716));
#194283=CARTESIAN_POINT('Ctrl Pts',(-44.8595476865727,24.3781406979818,
-234.881321825681));
#194284=CARTESIAN_POINT('Ctrl Pts',(-44.714012850909,24.5584600979606,-234.881556943632));
#194285=CARTESIAN_POINT('Ctrl Pts',(-44.6472900780137,24.641130410663,-234.881664737217));
#194286=CARTESIAN_POINT('Ctrl Pts',(-44.580320486115,24.7236311095871,-234.881769115404));
#194287=CARTESIAN_POINT('Ctrl Pts',(-44.5131079214061,24.8059600647562,
-234.881869844336));
#194288=CARTESIAN_POINT('Ctrl Pts',(-44.2745002008715,25.0982316721848,
-234.882227436712));
#194289=CARTESIAN_POINT('Ctrl Pts',(-44.0330777967232,25.3880385557821,
-234.882538122664));
#194290=CARTESIAN_POINT('Ctrl Pts',(-43.7890811769961,25.6752036410983,
-234.88280110814));
#194291=CARTESIAN_POINT('Ctrl Pts',(-43.5336383710576,25.975839999269,-234.883076430592));
#194292=CARTESIAN_POINT('Ctrl Pts',(-43.2753741805736,26.2735811812503,
-234.883299472219));
#194293=CARTESIAN_POINT('Ctrl Pts',(-43.0145135093598,26.5682532856333,
-234.883469321896));
#194294=CARTESIAN_POINT('Ctrl Pts',(-42.7885691451028,26.8234834089756,
-234.883616437124));
#194295=CARTESIAN_POINT('Ctrl Pts',(-42.5606759082898,27.0764117290122,
-234.883723646947));
#194296=CARTESIAN_POINT('Ctrl Pts',(-42.3309515524768,27.3269388059103,
-234.883790359317));
#194297=CARTESIAN_POINT('Ctrl Pts',(-42.0612872616582,27.6210225841997,
-234.883868670318));
#194298=CARTESIAN_POINT('Ctrl Pts',(-41.7889144466608,27.9120032296393,
-234.883890797532));
#194299=CARTESIAN_POINT('Ctrl Pts',(-41.5138321388492,28.1998649984553,
-234.883852686351));
#194300=CARTESIAN_POINT('Ctrl Pts',(-41.2299540147919,28.4969312095447,
-234.883813356558));
#194301=CARTESIAN_POINT('Ctrl Pts',(-40.9431900644798,28.7906768036788,
-234.88370987451));
#194302=CARTESIAN_POINT('Ctrl Pts',(-40.6534840262211,29.0810776426265,
-234.883537784092));
#194303=CARTESIAN_POINT('Ctrl Pts',(-40.4729316819002,29.262063004823,-234.883430532864));
#194304=CARTESIAN_POINT('Ctrl Pts',(-40.2912355238482,29.4417490417126,
-234.883296633411));
#194305=CARTESIAN_POINT('Ctrl Pts',(-40.1083724339856,29.6201262193833,
-234.883135007052));
#194306=CARTESIAN_POINT('Ctrl Pts',(-40.0800074003628,29.6477954152061,
-234.88310993618));
#194307=CARTESIAN_POINT('Ctrl Pts',(-40.051614276085,29.6754331110842,-234.88308419817));
#194308=CARTESIAN_POINT('Ctrl Pts',(-40.0231931536369,29.7030394061776,
-234.883057788995));
#194309=CARTESIAN_POINT('Ctrl Pts',(-39.7383427980406,29.9797231644769,
-234.882793103363));
#194310=CARTESIAN_POINT('Ctrl Pts',(-39.4508577652458,30.2530692798036,
-234.882473924431));
#194311=CARTESIAN_POINT('Ctrl Pts',(-39.1607632606661,30.5232243371498,
-234.882097470483));
#194312=CARTESIAN_POINT('Ctrl Pts',(-38.8687717624806,30.7951459995445,
-234.881718554817));
#194313=CARTESIAN_POINT('Ctrl Pts',(-38.5741356572691,31.0638353734139,
-234.881281612617));
#194314=CARTESIAN_POINT('Ctrl Pts',(-38.2768465821868,31.3294021629668,
-234.88078380724));
#194315=CARTESIAN_POINT('Ctrl Pts',(-37.9875650741985,31.5878158343478,
-234.880299410394));
#194316=CARTESIAN_POINT('Ctrl Pts',(-37.6957706557468,31.8432732365712,
-234.879757384948));
#194317=CARTESIAN_POINT('Ctrl Pts',(-37.401437189756,32.0958308802778,-234.879155117356));
#194318=CARTESIAN_POINT('Ctrl Pts',(-37.115266360764,32.3413844398245,-234.87856955222));
#194319=CARTESIAN_POINT('Ctrl Pts',(-36.8266945892579,32.5841971463957,
-234.877927039951));
#194320=CARTESIAN_POINT('Ctrl Pts',(-36.5356924808088,32.824273442989,-234.877225178471));
#194321=CARTESIAN_POINT('Ctrl Pts',(-36.2588701791423,33.0526514205671,
-234.876557516949));
#194322=CARTESIAN_POINT('Ctrl Pts',(-35.9798480396065,33.2785532299222,
-234.875836149178));
#194323=CARTESIAN_POINT('Ctrl Pts',(-35.6986053783016,33.5019368424606,
-234.875059007386));
#194324=CARTESIAN_POINT('Ctrl Pts',(-35.4793033421191,33.6761226535753,
-234.874453022588));
#194325=CARTESIAN_POINT('Ctrl Pts',(-35.2586511672865,33.8487765152758,
-234.873813125676));
#194326=CARTESIAN_POINT('Ctrl Pts',(-35.0366444584247,34.0198570237832,
-234.873138336286));
#194327=CARTESIAN_POINT('Ctrl Pts',(-34.9904940629195,34.0554209631404,
-234.87299806216));
#194328=CARTESIAN_POINT('Ctrl Pts',(-34.9442874985273,34.0909146676626,
-234.872856601922));
#194329=CARTESIAN_POINT('Ctrl Pts',(-34.8980249060694,34.1263375479426,
-234.872713978188));
#194330=CARTESIAN_POINT('Ctrl Pts',(-34.5916777753735,34.3609049847902,
-234.871769535396));
#194331=CARTESIAN_POINT('Ctrl Pts',(-34.2828722423169,34.5923705644,-234.870774073449));
#194332=CARTESIAN_POINT('Ctrl Pts',(-33.971520157457,34.8208350455687,-234.869734158406));
#194333=CARTESIAN_POINT('Ctrl Pts',(-33.6669144793353,35.0443491365196,
-234.868716776342));
#194334=CARTESIAN_POINT('Ctrl Pts',(-33.359870956103,35.2649906993816,-234.867656846737));
#194335=CARTESIAN_POINT('Ctrl Pts',(-33.0503299156795,35.4828099737801,
-234.866560518012));
#194336=CARTESIAN_POINT('Ctrl Pts',(-32.752262989056,35.6925550905844,-234.865504828164));
#194337=CARTESIAN_POINT('Ctrl Pts',(-32.4518799457129,35.8996831079268,
-234.864415387677));
#194338=CARTESIAN_POINT('Ctrl Pts',(-32.1491544499317,36.1041994670095,
-234.863297686268));
#194339=CARTESIAN_POINT('Ctrl Pts',(-31.8529815111427,36.3042890265084,
-234.862204177742));
#194340=CARTESIAN_POINT('Ctrl Pts',(-31.5545660682366,36.5018787132748,
-234.861083618481));
#194341=CARTESIAN_POINT('Ctrl Pts',(-31.2539148013445,36.696936587115,-234.859941149384));
#194342=CARTESIAN_POINT('Ctrl Pts',(-30.9639839854485,36.8850391988021,
-234.858839417798));
#194343=CARTESIAN_POINT('Ctrl Pts',(-30.6719737130795,37.0707872104706,
-234.857717311017));
#194344=CARTESIAN_POINT('Ctrl Pts',(-30.3779236186945,37.2541185543487,
-234.856579439382));
#194345=CARTESIAN_POINT('Ctrl Pts',(-30.1045036246594,37.4245876543653,
-234.855521399064));
#194346=CARTESIAN_POINT('Ctrl Pts',(-29.8293200171223,37.5929670251938,
-234.854449728371));
#194347=CARTESIAN_POINT('Ctrl Pts',(-29.5524353619882,37.7591803693088,
-234.853368133768));
#194348=CARTESIAN_POINT('Ctrl Pts',(-28.9814172171126,36.8014272692485,
-235.35005));
#194349=CARTESIAN_POINT('Ctrl Pts',(-30.4445221387403,35.9291153361899,
-235.35005));
#194350=CARTESIAN_POINT('Ctrl Pts',(-31.8571523563207,34.9976505207191,
-235.35005));
#194351=CARTESIAN_POINT('Ctrl Pts',(-33.2197493322593,34.0075501952557,
-235.35005));
#194352=CARTESIAN_POINT('Ctrl Pts',(-33.6068768507121,33.7262527252154,
-235.35005));
#194353=CARTESIAN_POINT('Ctrl Pts',(-33.9899655501571,33.4402220370472,
-235.35005));
#194354=CARTESIAN_POINT('Ctrl Pts',(-34.3690250580976,33.1494694133448,
-235.35005));
#194355=CARTESIAN_POINT('Ctrl Pts',(-36.0822840600053,31.8353365675737,
-235.35005));
#194356=CARTESIAN_POINT('Ctrl Pts',(-37.7150530376344,30.4268749532356,
-235.35005));
#194357=CARTESIAN_POINT('Ctrl Pts',(-39.2658957962434,28.9224014489936,
-235.35005));
#194358=CARTESIAN_POINT('Ctrl Pts',(-40.0413171755479,28.1701646968727,
-235.35005));
#194359=CARTESIAN_POINT('Ctrl Pts',(-40.7957050001266,27.3932780662842,
-235.35005));
#194360=CARTESIAN_POINT('Ctrl Pts',(-41.52971041916,26.5925046592713,-235.35005));
#194361=CARTESIAN_POINT('Ctrl Pts',(-42.2637158381934,25.7917312522584,
-235.35005));
#194362=CARTESIAN_POINT('Ctrl Pts',(-42.9787004139405,24.9654368934535,
-235.35005));
#194363=CARTESIAN_POINT('Ctrl Pts',(-43.669114034758,24.1181940231093,-235.35005));
#194364=CARTESIAN_POINT('Ctrl Pts',(-45.0499412763931,22.423708282421,-235.35005));
#194365=CARTESIAN_POINT('Ctrl Pts',(-46.3260905825898,20.6527606745438,
-235.350050000001));
#194366=CARTESIAN_POINT('Ctrl Pts',(-47.5004483343782,18.8074595529613,
-235.350050000001));
#194367=CARTESIAN_POINT('Ctrl Pts',(-47.5004483343777,18.8074595529617,
-235.35005));
#194368=CARTESIAN_POINT('Ctrl Pts',(-48.0508084453082,19.1577111488619,
-235.35005));
#194369=CARTESIAN_POINT('Ctrl Pts',(-48.4260896922579,19.3965417854669,
-234.872874618363));
#194370=CARTESIAN_POINT('Ctrl Pts',(-47.5233281555475,18.7715078669293,
-235.35005));
#194371=CARTESIAN_POINT('Ctrl Pts',(-48.0771976901895,19.1185775087876,
-235.350049999978));
#194372=CARTESIAN_POINT('Ctrl Pts',(-48.4542924222552,19.3549004456767,
-234.871334334863));
#194373=CARTESIAN_POINT('Ctrl Pts',(-47.5458232280531,18.7353573183218,
-235.35005));
#194374=CARTESIAN_POINT('Ctrl Pts',(-48.1039998334649,19.0785250138959,
-235.350050000005));
#194375=CARTESIAN_POINT('Ctrl Pts',(-48.4833024022839,19.3117585055263,
-234.869397699979));
#194376=CARTESIAN_POINT('Ctrl Pts',(-47.5895300323829,18.6623978031499,
-235.35005));
#194377=CARTESIAN_POINT('Ctrl Pts',(-48.1593257378831,18.9948843873186,
-235.350049999995));
#194378=CARTESIAN_POINT('Ctrl Pts',(-48.5444255909505,19.2196347103286,
-234.863872863852));
#194379=CARTESIAN_POINT('Ctrl Pts',(-47.6106972731343,18.625565406903,-235.35005));
#194380=CARTESIAN_POINT('Ctrl Pts',(-48.1884776688448,18.9506324984654,
-235.350050000003));
#194381=CARTESIAN_POINT('Ctrl Pts',(-48.5774448328292,19.1695186218693,
-234.85990679963));
#194382=CARTESIAN_POINT('Ctrl Pts',(-47.6410934853577,18.569620618322,-235.35005));
#194383=CARTESIAN_POINT('Ctrl Pts',(-48.229986112641,18.8839741987186,-235.350049999998));
#194384=CARTESIAN_POINT('Ctrl Pts',(-48.6241839653041,19.0944106548932,
-234.85414296838));
#194385=CARTESIAN_POINT('Ctrl Pts',(-47.6510095952452,18.550861366784,-235.35005));
#194386=CARTESIAN_POINT('Ctrl Pts',(-48.2431911415777,18.8619616358506,
-235.350049999998));
#194387=CARTESIAN_POINT('Ctrl Pts',(-48.638908043659,19.069857746375,-234.852410933521));
#194388=CARTESIAN_POINT('Ctrl Pts',(-47.6705745922183,18.513205530003,-235.35005));
#194389=CARTESIAN_POINT('Ctrl Pts',(-48.2671819452163,18.8197560443254,
-235.350050000002));
#194390=CARTESIAN_POINT('Ctrl Pts',(-48.6649527674787,19.024147533775,-234.850139144187));
#194391=CARTESIAN_POINT('Ctrl Pts',(-47.6802441619202,18.4943195741576,
-235.35005));
#194392=CARTESIAN_POINT('Ctrl Pts',(-48.2778090546859,18.799757048935,-235.350050000001));
#194393=CARTESIAN_POINT('Ctrl Pts',(-48.6760466930021,19.003315780373,-234.84970575966));
#194394=CARTESIAN_POINT('Ctrl Pts',(-47.7090490788398,18.4375569718045,
-235.35005));
#194395=CARTESIAN_POINT('Ctrl Pts',(-48.310705894182,18.7384640963053,-235.350049999999));
#194396=CARTESIAN_POINT('Ctrl Pts',(-48.7108682070929,18.9386166159486,
-234.847719038782));
#194397=CARTESIAN_POINT('Ctrl Pts',(-47.7279282401082,18.3995486637502,
-235.35005));
#194398=CARTESIAN_POINT('Ctrl Pts',(-48.3327596867691,18.6969547523118,
-235.350050000006));
#194399=CARTESIAN_POINT('Ctrl Pts',(-48.7343909692929,18.8944723982682,
-234.846132537133));
#194400=CARTESIAN_POINT('Ctrl Pts',(-47.7647487546851,18.3230500802882,
-235.35005));
#194401=CARTESIAN_POINT('Ctrl Pts',(-48.3775414056939,18.6116695818104,
-235.350049999994));
#194402=CARTESIAN_POINT('Ctrl Pts',(-48.7827487476233,18.8025467359427,
-234.841945226815));
#194403=CARTESIAN_POINT('Ctrl Pts',(-47.7827001660699,18.2845649741211,
-235.35005));
#194404=CARTESIAN_POINT('Ctrl Pts',(-48.4004562638174,18.5677247892466,
-235.350050000015));
#194405=CARTESIAN_POINT('Ctrl Pts',(-48.8078323528047,18.7544974911258,
-234.839249257519));
#194406=CARTESIAN_POINT('Ctrl Pts',(-47.81709615277,18.2068203539689,-235.35005));
#194407=CARTESIAN_POINT('Ctrl Pts',(-48.4474727822696,18.4757807159189,
-235.350049999985));
#194408=CARTESIAN_POINT('Ctrl Pts',(-48.8601288350238,18.6518909794679,
-234.832008606249));
#194409=CARTESIAN_POINT('Ctrl Pts',(-47.8335233281929,18.1675458631259,
-235.35005));
#194410=CARTESIAN_POINT('Ctrl Pts',(-48.4700885563297,18.4292216092512,
-235.350049999999));
#194411=CARTESIAN_POINT('Ctrl Pts',(-48.8852514246585,18.5999224430555,
-234.828363590487));
#194412=CARTESIAN_POINT('Ctrl Pts',(-47.8650504941538,18.0883394728593,
-235.35005));
#194413=CARTESIAN_POINT('Ctrl Pts',(-48.5118155154303,18.3374118427688,
-235.350050000001));
#194414=CARTESIAN_POINT('Ctrl Pts',(-48.931027462954,18.4988900212735,-234.822325836545));
#194415=CARTESIAN_POINT('Ctrl Pts',(-47.8801543850424,18.0485058523287,
-235.35005));
#194416=CARTESIAN_POINT('Ctrl Pts',(-48.530298509796,18.2930230307278,-235.350050000003));
#194417=CARTESIAN_POINT('Ctrl Pts',(-48.9508554755667,18.4512226738463,
-234.820369930511));
#194418=CARTESIAN_POINT('Ctrl Pts',(-47.9094666156693,17.9685258021276,
-235.35005));
#194419=CARTESIAN_POINT('Ctrl Pts',(-48.5670290414783,18.203228539971,-235.350049999996));
#194420=CARTESIAN_POINT('Ctrl Pts',(-48.990407903663,18.3543737889356,-234.815860390008));
#194421=CARTESIAN_POINT('Ctrl Pts',(-47.9236194657386,17.9283599903447,
-235.35005));
#194422=CARTESIAN_POINT('Ctrl Pts',(-48.5855270232061,18.1574071922804,
-235.350050000007));
#194423=CARTESIAN_POINT('Ctrl Pts',(-49.0104806988515,18.3045019253958,
-234.813092565269));
#194424=CARTESIAN_POINT('Ctrl Pts',(-47.9505381729848,17.8475439007782,
-235.35005));
#194425=CARTESIAN_POINT('Ctrl Pts',(-48.6229814684107,18.062872852205,-235.350049999994));
#194426=CARTESIAN_POINT('Ctrl Pts',(-49.0515011390314,18.2001358516365,
-234.805958241058));
#194427=CARTESIAN_POINT('Ctrl Pts',(-47.9632560597789,17.8068666429648,
-235.35005));
#194428=CARTESIAN_POINT('Ctrl Pts',(-48.6424408675579,18.0133995657985,
-235.350050000009));
#194429=CARTESIAN_POINT('Ctrl Pts',(-49.0730847555093,18.14440457461,-234.80115919183));
#194430=CARTESIAN_POINT('Ctrl Pts',(-47.9870034052699,17.7249653914156,
-235.35005));
#194431=CARTESIAN_POINT('Ctrl Pts',(-48.6779790062891,17.915615235708,-235.350049999991));
#194432=CARTESIAN_POINT('Ctrl Pts',(-49.112076978178,18.0354393113711,-234.792427668388));
#194433=CARTESIAN_POINT('Ctrl Pts',(-47.9980630400304,17.6838206475214,
-235.35005));
#194434=CARTESIAN_POINT('Ctrl Pts',(-48.6943197391833,17.8671438309789,
-235.35005000001));
#194435=CARTESIAN_POINT('Ctrl Pts',(-49.1298441237351,17.981860251528,-234.788349296066));
#194436=CARTESIAN_POINT('Ctrl Pts',(-48.0189197776842,17.6012300921137,
-235.35005));
#194437=CARTESIAN_POINT('Ctrl Pts',(-48.7242285116606,17.771770777776,-235.35004999999));
#194438=CARTESIAN_POINT('Ctrl Pts',(-49.162044625621,17.8776762330174,-234.781180866063));
#194439=CARTESIAN_POINT('Ctrl Pts',(-48.0287613458656,17.5597948840364,
-235.35005));
#194440=CARTESIAN_POINT('Ctrl Pts',(-48.7384179936011,17.7241346288096,
-235.350049999995));
#194441=CARTESIAN_POINT('Ctrl Pts',(-49.1772563366924,17.8258110055907,
-234.777634115965));
#194442=CARTESIAN_POINT('Ctrl Pts',(-48.0470227250193,17.4765854309817,
-235.35005));
#194443=CARTESIAN_POINT('Ctrl Pts',(-48.7670952112289,17.6259226184369,
-235.350050000005));
#194444=CARTESIAN_POINT('Ctrl Pts',(-49.2081218683014,17.7174394526145,
-234.76877506552));
#194445=CARTESIAN_POINT('Ctrl Pts',(-48.0554329780656,17.4347916601489,
-235.35005));
#194446=CARTESIAN_POINT('Ctrl Pts',(-48.7812919042116,17.5756645037128,
-235.350050000005));
#194447=CARTESIAN_POINT('Ctrl Pts',(-49.2234010254764,17.6615278352864,
-234.763682646456));
#194448=CARTESIAN_POINT('Ctrl Pts',(-48.0705953135359,17.3508835165529,
-235.35005));
#194449=CARTESIAN_POINT('Ctrl Pts',(-48.808104677187,17.4743257669527,-235.350049999995));
#194450=CARTESIAN_POINT('Ctrl Pts',(-49.2520548027181,17.5486925247621,
-234.75299425464));
#194451=CARTESIAN_POINT('Ctrl Pts',(-48.0773499548877,17.3088369763077,
-235.350050000001));
#194452=CARTESIAN_POINT('Ctrl Pts',(-48.8202836830788,17.4239614927865,
-235.35005));
#194453=CARTESIAN_POINT('Ctrl Pts',(-49.2649325810603,17.4929198622924,
-234.747809920555));
#194454=CARTESIAN_POINT('Ctrl Pts',(-48.0894592880343,17.2245872750773,
-235.350050000001));
#194455=CARTESIAN_POINT('Ctrl Pts',(-48.8422242267331,17.3243377880475,
-235.35005));
#194456=CARTESIAN_POINT('Ctrl Pts',(-49.2879043244386,17.3834514853175,
-234.738139816296));
#194457=CARTESIAN_POINT('Ctrl Pts',(-48.094834615712,17.1823864227582,-235.35005));
#194458=CARTESIAN_POINT('Ctrl Pts',(-48.8514819375229,17.2759479237276,
-235.350050000014));
#194459=CARTESIAN_POINT('Ctrl Pts',(-49.2974763354349,17.3311532118177,
-234.734202664179));
#194460=CARTESIAN_POINT('Ctrl Pts',(-48.1091464500575,17.0555809060241,
-235.35005));
#194461=CARTESIAN_POINT('Ctrl Pts',(-48.8799935741974,17.1259395893774,
-235.350049999972));
#194462=CARTESIAN_POINT('Ctrl Pts',(-49.3267656585904,17.1669449229297,
-234.719429103118));
#194463=CARTESIAN_POINT('Ctrl Pts',(-48.1154436500424,16.9706923807857,
-235.350050000001));
#194464=CARTESIAN_POINT('Ctrl Pts',(-48.8997687328372,17.016853275791,-235.35004999989));
#194465=CARTESIAN_POINT('Ctrl Pts',(-49.3465478480362,17.0432452943168,
-234.704309415519));
#194466=CARTESIAN_POINT('Ctrl Pts',(-48.1189208895433,16.8854655414009,
-235.350050000001));
#194467=CARTESIAN_POINT('Ctrl Pts',(-48.9115061644414,16.9178030353161,
-235.350050000001));
#194468=CARTESIAN_POINT('Ctrl Pts',(-49.3576635057813,16.9360062631172,
-234.694420988468));
#194469=CARTESIAN_POINT('',(-49.3576635057812,16.9360062631145,-234.694420988467));
#194470=CARTESIAN_POINT('',(-48.1189208895436,16.8854655414,-235.35005));
#194471=CARTESIAN_POINT('Origin',(-48.1189208895436,16.8854655414,-233.85005));
#194472=CARTESIAN_POINT('Ctrl Pts',(-49.3576635057812,16.9360062631145,
-234.694420988467));
#194473=CARTESIAN_POINT('Ctrl Pts',(-49.3465478480362,17.0432452943168,
-234.704309415519));
#194474=CARTESIAN_POINT('Ctrl Pts',(-49.3267656585904,17.1669449229297,
-234.719429103118));
#194475=CARTESIAN_POINT('Ctrl Pts',(-49.2974763354349,17.3311532118177,
-234.734202664179));
#194476=CARTESIAN_POINT('Ctrl Pts',(-49.2879043244386,17.3834514853175,
-234.738139816296));
#194477=CARTESIAN_POINT('Ctrl Pts',(-49.2649325810603,17.4929198622924,
-234.747809920555));
#194478=CARTESIAN_POINT('Ctrl Pts',(-49.2520548027181,17.5486925247621,
-234.75299425464));
#194479=CARTESIAN_POINT('Ctrl Pts',(-49.2234010254764,17.6615278352864,
-234.763682646456));
#194480=CARTESIAN_POINT('Ctrl Pts',(-49.2081218683014,17.7174394526145,
-234.76877506552));
#194481=CARTESIAN_POINT('Ctrl Pts',(-49.1772563366924,17.8258110055907,
-234.777634115965));
#194482=CARTESIAN_POINT('Ctrl Pts',(-49.162044625621,17.8776762330174,-234.781180866063));
#194483=CARTESIAN_POINT('Ctrl Pts',(-49.1298441237351,17.981860251528,-234.788349296066));
#194484=CARTESIAN_POINT('Ctrl Pts',(-49.112076978178,18.0354393113711,-234.792427668388));
#194485=CARTESIAN_POINT('Ctrl Pts',(-49.0730847555093,18.14440457461,-234.80115919183));
#194486=CARTESIAN_POINT('Ctrl Pts',(-49.0515011390314,18.2001358516365,
-234.805958241058));
#194487=CARTESIAN_POINT('Ctrl Pts',(-49.0104806988515,18.3045019253958,
-234.813092565269));
#194488=CARTESIAN_POINT('Ctrl Pts',(-48.990407903663,18.3543737889356,-234.815860390008));
#194489=CARTESIAN_POINT('Ctrl Pts',(-48.9508554755667,18.4512226738463,
-234.820369930511));
#194490=CARTESIAN_POINT('Ctrl Pts',(-48.931027462954,18.4988900212735,-234.822325836545));
#194491=CARTESIAN_POINT('Ctrl Pts',(-48.8852514246585,18.5999224430555,
-234.828363590487));
#194492=CARTESIAN_POINT('Ctrl Pts',(-48.8601288350238,18.6518909794679,
-234.832008606249));
#194493=CARTESIAN_POINT('Ctrl Pts',(-48.8078323528047,18.7544974911258,
-234.839249257519));
#194494=CARTESIAN_POINT('Ctrl Pts',(-48.7827487476233,18.8025467359427,
-234.841945226815));
#194495=CARTESIAN_POINT('Ctrl Pts',(-48.7343909692929,18.8944723982682,
-234.846132537133));
#194496=CARTESIAN_POINT('Ctrl Pts',(-48.7108682070929,18.9386166159486,
-234.847719038782));
#194497=CARTESIAN_POINT('Ctrl Pts',(-48.6760466930021,19.003315780373,-234.84970575966));
#194498=CARTESIAN_POINT('Ctrl Pts',(-48.6649527674787,19.024147533775,-234.850139144187));
#194499=CARTESIAN_POINT('Ctrl Pts',(-48.638908043659,19.069857746375,-234.852410933521));
#194500=CARTESIAN_POINT('Ctrl Pts',(-48.6241839653041,19.0944106548932,
-234.85414296838));
#194501=CARTESIAN_POINT('Ctrl Pts',(-48.5774448328292,19.1695186218693,
-234.85990679963));
#194502=CARTESIAN_POINT('Ctrl Pts',(-48.5444255909505,19.2196347103286,
-234.863872863852));
#194503=CARTESIAN_POINT('Ctrl Pts',(-48.4833024022839,19.3117585055263,
-234.869397699979));
#194504=CARTESIAN_POINT('Ctrl Pts',(-48.4542924222552,19.3549004456767,
-234.871334334863));
#194505=CARTESIAN_POINT('Ctrl Pts',(-48.4260896922586,19.3965417854656,
-234.872874618363));
#194506=CARTESIAN_POINT('Ctrl Pts',(-47.5004483343782,18.8074595529612,
-235.35005));
#194507=CARTESIAN_POINT('Ctrl Pts',(-47.523328218883,18.7715077674088,-235.35005));
#194508=CARTESIAN_POINT('Ctrl Pts',(-47.5458232845143,18.7353572240715,
-235.35005));
#194509=CARTESIAN_POINT('Ctrl Pts',(-47.5676766302509,18.6988775607556,
-235.35005));
#194510=CARTESIAN_POINT('Ctrl Pts',(-47.5895300808456,18.6623977224007,
-235.35005));
#194511=CARTESIAN_POINT('Ctrl Pts',(-47.6106973144047,18.6255653312655,
-235.35005));
#194512=CARTESIAN_POINT('Ctrl Pts',(-47.6309614148883,18.58826888133,-235.35005));
#194513=CARTESIAN_POINT('Ctrl Pts',(-47.6410934945813,18.5696206021569,
-235.35005));
#194514=CARTESIAN_POINT('Ctrl Pts',(-47.6510096037987,18.5508613513732,
-235.35005));
#194515=CARTESIAN_POINT('Ctrl Pts',(-47.6607920942703,18.5320334486734,
-235.35005));
#194516=CARTESIAN_POINT('Ctrl Pts',(-47.6705746000884,18.513205516437,-235.35005));
#194517=CARTESIAN_POINT('Ctrl Pts',(-47.6802441693448,18.4943195614609,
-235.35005));
#194518=CARTESIAN_POINT('Ctrl Pts',(-47.6898458018307,18.4753987071822,
-235.35005));
#194519=CARTESIAN_POINT('Ctrl Pts',(-47.70904910136,18.4375569305264,-235.35005));
#194520=CARTESIAN_POINT('Ctrl Pts',(-47.7279282587774,18.3995486292809,
-235.35005));
#194521=CARTESIAN_POINT('Ctrl Pts',(-47.7463384996528,18.3612993731052,
-235.35005));
#194522=CARTESIAN_POINT('Ctrl Pts',(-47.7647487677154,18.323050060445,-235.35005));
#194523=CARTESIAN_POINT('Ctrl Pts',(-47.7827001759863,18.2845649614141,
-235.35005));
#194524=CARTESIAN_POINT('Ctrl Pts',(-47.7998981639292,18.24569266604,-235.35005));
#194525=CARTESIAN_POINT('Ctrl Pts',(-47.8170961582275,18.2068203563009,
-235.35005));
#194526=CARTESIAN_POINT('Ctrl Pts',(-47.8335233318918,18.1675458731571,
-235.35005));
#194527=CARTESIAN_POINT('Ctrl Pts',(-47.8492869191686,18.127942671175,-235.35005));
#194528=CARTESIAN_POINT('Ctrl Pts',(-47.8650504948173,18.0883394984066,
-235.35005));
#194529=CARTESIAN_POINT('Ctrl Pts',(-47.8801543852333,18.0485058859946,
-235.35005));
#194530=CARTESIAN_POINT('Ctrl Pts',(-47.8948105132744,18.0085158319627,
-235.35005));
#194531=CARTESIAN_POINT('Ctrl Pts',(-47.909466614277,17.9685258517065,-235.35005));
#194532=CARTESIAN_POINT('Ctrl Pts',(-47.9236194654021,17.9283600484622,
-235.35005));
#194533=CARTESIAN_POINT('Ctrl Pts',(-47.9370788390041,17.887951952103,-235.35005));
#194534=CARTESIAN_POINT('Ctrl Pts',(-47.9505379989423,17.847544497211,-235.35005));
#194535=CARTESIAN_POINT('Ctrl Pts',(-47.9632559353684,17.8068671621608,
-235.35005));
#194536=CARTESIAN_POINT('Ctrl Pts',(-47.9751297575526,17.7659160244471,
-235.35005));
#194537=CARTESIAN_POINT('Ctrl Pts',(-47.9870033323709,17.7249657398638,
-235.35005));
#194538=CARTESIAN_POINT('Ctrl Pts',(-47.9980630011651,17.6838209125432,
-235.35005));
#194539=CARTESIAN_POINT('Ctrl Pts',(-48.0084914348375,17.6425253763784,
-235.35005));
#194540=CARTESIAN_POINT('Ctrl Pts',(-48.0189197816014,17.6012301843623,
-235.35005));
#194541=CARTESIAN_POINT('Ctrl Pts',(-48.0287613705984,17.5597948897797,
-235.35005));
#194542=CARTESIAN_POINT('Ctrl Pts',(-48.0378920589035,17.5181901626578,
-235.35005));
#194543=CARTESIAN_POINT('Ctrl Pts',(-48.0470227852353,17.4765852622638,
-235.35005));
#194544=CARTESIAN_POINT('Ctrl Pts',(-48.0554330459596,17.4347914019545,
-235.35005));
#194545=CARTESIAN_POINT('Ctrl Pts',(-48.063014164453,17.3928375917214,-235.35005));
#194546=CARTESIAN_POINT('Ctrl Pts',(-48.0705954092764,17.3508830823798,
-235.35005));
#194547=CARTESIAN_POINT('Ctrl Pts',(-48.0773500452528,17.3088364520712,
-235.350050000001));
#194548=CARTESIAN_POINT('Ctrl Pts',(-48.0834046340598,17.2667121275033,
-235.350050000001));
#194549=CARTESIAN_POINT('Ctrl Pts',(-48.0894593994455,17.2245865744039,
-235.350050000001));
#194550=CARTESIAN_POINT('Ctrl Pts',(-48.0948347135637,17.1823856312802,
-235.35005));
#194551=CARTESIAN_POINT('Ctrl Pts',(-48.0996052337066,17.140117917919,-235.35005));
#194552=CARTESIAN_POINT('Ctrl Pts',(-48.1091469299998,17.0555766788456,
-235.35005));
#194553=CARTESIAN_POINT('Ctrl Pts',(-48.115443852909,16.9706874085479,-235.350050000001));
#194554=CARTESIAN_POINT('Ctrl Pts',(-48.1189208895436,16.885465541401,-235.350050000001));
#194555=CARTESIAN_POINT('Ctrl Pts',(-48.1189208895436,16.8854655414,-235.35005));
#194556=CARTESIAN_POINT('Ctrl Pts',(-48.9115061644421,16.9178030353144,
-235.35005));
#194557=CARTESIAN_POINT('Ctrl Pts',(-49.357663505782,16.9360062631151,-234.694420988466));
#194558=CARTESIAN_POINT('Ctrl Pts',(-48.2232158057592,14.3292187542857,
-235.35005));
#194559=CARTESIAN_POINT('Ctrl Pts',(-49.0175817386228,14.3575637238871,
-235.350050000391));
#194560=CARTESIAN_POINT('Ctrl Pts',(-49.4635649335608,14.3752531202943,
-234.692333873014));
#194561=CARTESIAN_POINT('Ctrl Pts',(-48.3134219778347,11.7724738102799,
-235.35005));
#194562=CARTESIAN_POINT('Ctrl Pts',(-49.1092649251398,11.7982892962054,
-235.350049999822));
#194563=CARTESIAN_POINT('Ctrl Pts',(-49.5551530156078,11.8140213189959,
-234.690527234957));
#194564=CARTESIAN_POINT('Ctrl Pts',(-48.3895556141632,9.21523338364434,
-235.35005));
#194565=CARTESIAN_POINT('Ctrl Pts',(-49.1866080561977,9.23896306516062,
-235.35005));
#194566=CARTESIAN_POINT('Ctrl Pts',(-49.6324230235364,9.25223577675678,
-234.689044294154));
#194567=CARTESIAN_POINT('',(-49.6324230236214,9.25223577621558,-234.689044294051));
#194568=CARTESIAN_POINT('',(-48.3895556141631,9.21523338364434,-235.35005));
#194569=CARTESIAN_POINT('Origin',(-48.3895556141631,9.21523338364435,-233.85005));
#194570=CARTESIAN_POINT('Origin',(637.557461367465,-11.4839373498759,-249.18849675272));
#194571=CARTESIAN_POINT('Origin',(648.115804222845,-11.5202125233637,-235.35005));
#194572=CARTESIAN_POINT('Ctrl Pts',(-48.3895556141631,9.21523338364434,
-235.35005));
#194573=CARTESIAN_POINT('Ctrl Pts',(-49.1866080561976,9.2389630651606,-235.35005));
#194574=CARTESIAN_POINT('Ctrl Pts',(-49.6324230235363,9.25223577675675,
-234.689044294154));
#194575=CARTESIAN_POINT('Ctrl Pts',(-48.3941977967819,9.05930695550865,
-235.35005));
#194576=CARTESIAN_POINT('Ctrl Pts',(-49.2342501491402,9.001739953271,-235.35005));
#194577=CARTESIAN_POINT('Ctrl Pts',(-49.6757365198119,8.97285489239317,
-234.637202259114));
#194578=CARTESIAN_POINT('Ctrl Pts',(-48.3758516795198,8.90558680151918,
-235.35005));
#194579=CARTESIAN_POINT('Ctrl Pts',(-49.2516340201201,8.76786001619219,
-235.35005));
#194580=CARTESIAN_POINT('Ctrl Pts',(-49.6780275597748,8.70253397403411,
-234.577829926993));
#194581=CARTESIAN_POINT('Ctrl Pts',(-48.3395182384273,8.75410525715266,
-235.35005));
#194582=CARTESIAN_POINT('Ctrl Pts',(-49.2471092638204,8.53641604164419,
-235.35005));
#194583=CARTESIAN_POINT('Ctrl Pts',(-49.6480781836462,8.44024209637809,
-234.512742074857));
#194584=CARTESIAN_POINT('',(-49.6480781836462,8.4402420963781,-234.512742074857));
#194585=CARTESIAN_POINT('',(-48.3395182384274,8.75410525715259,-235.35005));
#194586=CARTESIAN_POINT('Origin',(-48.3395182384273,8.75410525715261,-233.85005));
#194587=CARTESIAN_POINT('Ctrl Pts',(-49.6480781836462,8.44024209637808,
-234.512742074857));
#194588=CARTESIAN_POINT('Ctrl Pts',(-49.6780275597748,8.70253397403411,
-234.577829926993));
#194589=CARTESIAN_POINT('Ctrl Pts',(-49.6757365198119,8.97285489239317,
-234.637202259114));
#194590=CARTESIAN_POINT('Ctrl Pts',(-49.6324230235363,9.25223577675679,
-234.689044294154));
#194591=CARTESIAN_POINT('Ctrl Pts',(-48.3895556141631,9.21523338364434,
-235.35005));
#194592=CARTESIAN_POINT('Ctrl Pts',(-48.3942007072891,9.05921010043768,
-235.35005));
#194593=CARTESIAN_POINT('Ctrl Pts',(-48.3758739100739,8.90567951512196,
-235.35005));
#194594=CARTESIAN_POINT('Ctrl Pts',(-48.3395182384274,8.75410525715259,
-235.35005));
#194595=CARTESIAN_POINT('Ctrl Pts',(-48.3395182384273,8.75410525715258,
-235.35005));
#194596=CARTESIAN_POINT('Ctrl Pts',(-49.2472715290903,8.53637712169199,
-235.35005));
#194597=CARTESIAN_POINT('Ctrl Pts',(-49.6481815209496,8.44021731052644,
-234.512526241039));
#194598=CARTESIAN_POINT('Ctrl Pts',(-48.1420785222883,7.9309385499425,-235.35005));
#194599=CARTESIAN_POINT('Ctrl Pts',(-49.0294131223446,7.77639740475676,
-235.350049999895));
#194600=CARTESIAN_POINT('Ctrl Pts',(-49.4453995747691,7.69019452166921,
-234.55773567316));
#194601=CARTESIAN_POINT('Ctrl Pts',(-48.0110562568883,7.10334135417386,
-235.35005));
#194602=CARTESIAN_POINT('Ctrl Pts',(-48.8755547320805,6.99587710352252,
-235.350049999977));
#194603=CARTESIAN_POINT('Ctrl Pts',(-49.3042975972362,6.93367143720089,
-234.594758063933));
#194604=CARTESIAN_POINT('Ctrl Pts',(-47.8801847113252,5.43950276679566,
-235.35005));
#194605=CARTESIAN_POINT('Ctrl Pts',(-48.7049699708569,5.42468658168255,
-235.350050000023));
#194606=CARTESIAN_POINT('Ctrl Pts',(-49.1474389986164,5.40777060896425,
-234.655599767885));
#194607=CARTESIAN_POINT('Ctrl Pts',(-47.8802911702592,4.60324650202951,
-235.35005));
#194608=CARTESIAN_POINT('Ctrl Pts',(-48.6857137786293,4.62945747049866,
-235.350049999965));
#194609=CARTESIAN_POINT('Ctrl Pts',(-49.1316168687632,4.63854634449982,
-234.679496688758));
#194610=CARTESIAN_POINT('Ctrl Pts',(-47.9840461137012,3.34200714134957,
-235.35005));
#194611=CARTESIAN_POINT('Ctrl Pts',(-48.7629781465623,3.42847856723455,
-235.350050000018));
#194612=CARTESIAN_POINT('Ctrl Pts',(-49.2081948431086,3.47653001453442,
-234.707152337111));
#194613=CARTESIAN_POINT('Ctrl Pts',(-48.0360840389224,2.92068200690756,
-235.35005));
#194614=CARTESIAN_POINT('Ctrl Pts',(-48.8063313608279,3.02739794392703,
-235.350050000023));
#194615=CARTESIAN_POINT('Ctrl Pts',(-49.2506302602395,3.08799066764764,
-234.714964437313));
#194616=CARTESIAN_POINT('Ctrl Pts',(-48.1401430583213,2.2930545562818,-235.35005));
#194617=CARTESIAN_POINT('Ctrl Pts',(-48.8978289995632,2.42958777593589,
-235.350049999988));
#194618=CARTESIAN_POINT('Ctrl Pts',(-49.3396413190743,2.5089581698339,-234.724628454032));
#194619=CARTESIAN_POINT('Ctrl Pts',(-48.1791846215008,2.08432209117866,
-235.35005));
#194620=CARTESIAN_POINT('Ctrl Pts',(-48.932713688424,2.23083484320497,-235.350050000003));
#194621=CARTESIAN_POINT('Ctrl Pts',(-49.3735508031399,2.31635516053753,
-234.727514226363));
#194622=CARTESIAN_POINT('Ctrl Pts',(-48.228072252525,1.85004158947422,-235.35005));
#194623=CARTESIAN_POINT('Ctrl Pts',(-48.9769897078866,2.0076757336604,-235.35005));
#194624=CARTESIAN_POINT('Ctrl Pts',(-49.4165272131256,2.10018771678728,
-234.730394424523));
#194625=CARTESIAN_POINT('Ctrl Pts',(-48.2336222089945,1.8240233376047,-235.35005));
#194626=CARTESIAN_POINT('Ctrl Pts',(-48.9818156073548,1.98338263954127,
-235.35005));
#194627=CARTESIAN_POINT('Ctrl Pts',(-49.421152047383,2.07696182865743,-234.730846041466));
#194628=CARTESIAN_POINT('Ctrl Pts',(-48.2445959867496,1.77197302819215,
-235.35005));
#194629=CARTESIAN_POINT('Ctrl Pts',(-48.9941558750127,1.92837971028397,
-235.35005));
#194630=CARTESIAN_POINT('Ctrl Pts',(-49.4338273118493,2.0201275975502,-234.729910687298));
#194631=CARTESIAN_POINT('Ctrl Pts',(-48.2500003143967,1.7459388370457,-235.35005));
#194632=CARTESIAN_POINT('Ctrl Pts',(-49.0002396819616,1.90086620641864,
-235.350049999998));
#194633=CARTESIAN_POINT('Ctrl Pts',(-49.4400753518836,1.99169798970336,
-234.729442130167));
#194634=CARTESIAN_POINT('Ctrl Pts',(-48.2659659469638,1.66780919078281,
-235.35005));
#194635=CARTESIAN_POINT('Ctrl Pts',(-49.0182341893565,1.81828164539219,
-235.350050000004));
#194636=CARTESIAN_POINT('Ctrl Pts',(-49.4585508766027,1.90637194168949,
-234.728033882328));
#194637=CARTESIAN_POINT('Ctrl Pts',(-48.2762799057323,1.61568666327167,
-235.35005));
#194638=CARTESIAN_POINT('Ctrl Pts',(-49.0298842521479,1.76318267619767,
-235.350049999997));
#194639=CARTESIAN_POINT('Ctrl Pts',(-49.4705097695714,1.84943827229719,
-234.727091615801));
#194640=CARTESIAN_POINT('Ctrl Pts',(-48.3062349042401,1.45921106566498,
-235.35005));
#194641=CARTESIAN_POINT('Ctrl Pts',(-49.0638081444409,1.59771048446028,
-235.350050000006));
#194642=CARTESIAN_POINT('Ctrl Pts',(-49.5053134343056,1.67849037267874,
-234.724254996978));
#194643=CARTESIAN_POINT('Ctrl Pts',(-48.3248891349689,1.35474998793845,
-235.35005));
#194644=CARTESIAN_POINT('Ctrl Pts',(-49.0850407737684,1.48722661629604,
-235.35005));
#194645=CARTESIAN_POINT('Ctrl Pts',(-49.5270852372327,1.56432923319846,
-234.722350837375));
#194646=CARTESIAN_POINT('Ctrl Pts',(-48.4809881192922,0.413309956198443,
-235.35005));
#194647=CARTESIAN_POINT('Ctrl Pts',(-49.2642810383497,0.488366675923553,
-235.35005));
#194648=CARTESIAN_POINT('Ctrl Pts',(-49.710183690821,0.535165240177996,
-234.705106054305));
#194649=CARTESIAN_POINT('Ctrl Pts',(-48.536801379512,-0.432603676106494,
-235.35005));
#194650=CARTESIAN_POINT('Ctrl Pts',(-49.3355324653308,-0.409176197440279,
-235.350050000012));
#194651=CARTESIAN_POINT('Ctrl Pts',(-49.7825193026416,-0.391551959040333,
-234.689053205068));
#194652=CARTESIAN_POINT('Ctrl Pts',(-48.4927543039942,-1.71545839400357,
-235.35005));
#194653=CARTESIAN_POINT('Ctrl Pts',(-49.3082764037978,-1.77136040509552,
-235.350049999994));
#194654=CARTESIAN_POINT('Ctrl Pts',(-49.7507288283362,-1.80056236505131,
-234.663753597616));
#194655=CARTESIAN_POINT('Ctrl Pts',(-48.4566916340738,-2.14207645769056,
-235.35005));
#194656=CARTESIAN_POINT('Ctrl Pts',(-49.2764210778577,-2.22581389857566,
-235.350050000023));
#194657=CARTESIAN_POINT('Ctrl Pts',(-49.7166012702585,-2.26961303439206,
-234.655203456267));
#194658=CARTESIAN_POINT('Ctrl Pts',(-48.3849699272127,-2.67235166449409,
-235.35005));
#194659=CARTESIAN_POINT('Ctrl Pts',(-49.2084397535132,-2.79078396174404,
-235.350049999994));
#194660=CARTESIAN_POINT('Ctrl Pts',(-49.6445034279608,-2.85342594052608,
-234.644346442065));
#194661=CARTESIAN_POINT('Ctrl Pts',(-48.3692885871419,-2.77828474965782,
-235.35005));
#194662=CARTESIAN_POINT('Ctrl Pts',(-49.193398982803,-2.90385097056055,
-235.350050000001));
#194663=CARTESIAN_POINT('Ctrl Pts',(-49.6286066062384,-2.97008785028305,
-234.642167439818));
#194664=CARTESIAN_POINT('Ctrl Pts',(-48.3437536505604,-2.93700076554913,
-235.35005));
#194665=CARTESIAN_POINT('Ctrl Pts',(-49.1686998051045,-3.07327329064321,
-235.350049999999));
#194666=CARTESIAN_POINT('Ctrl Pts',(-49.6025360173428,-3.14492002789723,
-234.638888778593));
#194667=CARTESIAN_POINT('Ctrl Pts',(-48.3349064994216,-2.98987550056776,
-235.35005));
#194668=CARTESIAN_POINT('Ctrl Pts',(-49.1601069182845,-3.12973803229213,
-235.350049999997));
#194669=CARTESIAN_POINT('Ctrl Pts',(-49.5934749193683,-3.20317062991129,
-234.637794194996));
#194670=CARTESIAN_POINT('Ctrl Pts',(-48.3234272698566,-3.05593058196302,
-235.35005));
#194671=CARTESIAN_POINT('Ctrl Pts',(-49.1489197764021,-3.20027698459844,
-235.350050000001));
#194672=CARTESIAN_POINT('Ctrl Pts',(-49.5816838579669,-3.27594936010119,
-234.636423946058));
#194673=CARTESIAN_POINT('Ctrl Pts',(-48.3211104090697,-3.06913968133917,
-235.35005));
#194674=CARTESIAN_POINT('Ctrl Pts',(-49.1466595294267,-3.21438584913259,
-235.350049999999));
#194675=CARTESIAN_POINT('Ctrl Pts',(-49.5793024111936,-3.29050337910297,
-234.636149795232));
#194676=CARTESIAN_POINT('Ctrl Pts',(-48.3164346335911,-3.09555404408755,
-235.35005));
#194677=CARTESIAN_POINT('Ctrl Pts',(-49.1420941838039,-3.24260063609391,
-235.350050000001));
#194678=CARTESIAN_POINT('Ctrl Pts',(-49.574493021136,-3.31960793810423,
-234.635601293727));
#194679=CARTESIAN_POINT('Ctrl Pts',(-48.3140690695237,-3.10875870092911,
-235.35005));
#194680=CARTESIAN_POINT('Ctrl Pts',(-49.1398758067619,-3.25784913209198,
-235.350049999999));
#194681=CARTESIAN_POINT('Ctrl Pts',(-49.5719898593111,-3.33586395411082,
-234.63494477827));
#194682=CARTESIAN_POINT('Ctrl Pts',(-48.3069527703726,-3.14837088297125,
-235.35005));
#194683=CARTESIAN_POINT('Ctrl Pts',(-49.1325141063836,-3.29520795233012,
-235.350050000002));
#194684=CARTESIAN_POINT('Ctrl Pts',(-49.5649563519778,-3.37212886380977,
-234.635775552688));
#194685=CARTESIAN_POINT('Ctrl Pts',(-48.3022780138372,-3.17478533866626,
-235.35005));
#194686=CARTESIAN_POINT('Ctrl Pts',(-49.1276759101128,-3.32012439113747,
-235.350050000001));
#194687=CARTESIAN_POINT('Ctrl Pts',(-49.5603339841976,-3.39631357393668,
-234.636323283642));
#194688=CARTESIAN_POINT('Ctrl Pts',(-48.260829396598,-3.41257237641022,
-235.35005));
#194689=CARTESIAN_POINT('Ctrl Pts',(-49.0847964911652,-3.54426580816513,
-235.350049999991));
#194690=CARTESIAN_POINT('Ctrl Pts',(-49.5193318923867,-3.61404804116118,
-234.641198325652));
#194691=CARTESIAN_POINT('Ctrl Pts',(-48.2284220495721,-3.6243432560285,
-235.35005));
#194692=CARTESIAN_POINT('Ctrl Pts',(-49.0511033314479,-3.74426713955755,
-235.350049999982));
#194693=CARTESIAN_POINT('Ctrl Pts',(-49.487144398575,-3.80810162390295,
-234.645144669832));
#194694=CARTESIAN_POINT('Ctrl Pts',(-48.144430583747,-4.26086274000263,
-235.35005));
#194695=CARTESIAN_POINT('Ctrl Pts',(-48.9634476725892,-4.34524549861128,
-235.350050000035));
#194696=CARTESIAN_POINT('Ctrl Pts',(-49.4033209083405,-4.39164979328187,
-234.655896371867));
#194697=CARTESIAN_POINT('Ctrl Pts',(-48.1060703916391,-4.68681758304716,
-235.35005));
#194698=CARTESIAN_POINT('Ctrl Pts',(-48.9226394477868,-4.74845242256804,
-235.350050000024));
#194699=CARTESIAN_POINT('Ctrl Pts',(-49.3644187765574,-4.7824530264519,
-234.661627301873));
#194700=CARTESIAN_POINT('Ctrl Pts',(-48.0648194622892,-5.541962664716,-235.35005));
#194701=CARTESIAN_POINT('Ctrl Pts',(-48.8768530903346,-5.55812616662415,
-235.350049999976));
#194702=CARTESIAN_POINT('Ctrl Pts',(-49.3208923248062,-5.56761936750886,
-234.670334826408));
#194703=CARTESIAN_POINT('Ctrl Pts',(-48.0619566741598,-5.9722387873912,
-235.35005));
#194704=CARTESIAN_POINT('Ctrl Pts',(-48.8717934133749,-5.96601881198723,
-235.350049999988));
#194705=CARTESIAN_POINT('Ctrl Pts',(-49.316286029903,-5.96285167976809,
-234.673332973669));
#194706=CARTESIAN_POINT('Ctrl Pts',(-48.10749380005,-7.25998633045287,-235.35005));
#194707=CARTESIAN_POINT('Ctrl Pts',(-48.9111302298558,-7.1858727298053,
-235.350050000024));
#194708=CARTESIAN_POINT('Ctrl Pts',(-49.3548824427616,-7.14594001291835,
-234.678250097988));
#194709=CARTESIAN_POINT('Ctrl Pts',(-48.2090347928457,-8.11012177193449,
-235.35005));
#194710=CARTESIAN_POINT('Ctrl Pts',(-49.0092881727724,-7.99360123144335,
-235.350050000012));
#194711=CARTESIAN_POINT('Ctrl Pts',(-49.4496009034112,-7.92719424599897,
-234.676205023672));
#194712=CARTESIAN_POINT('Ctrl Pts',(-48.3844338019353,-8.96504977313631,
-235.35005));
#194713=CARTESIAN_POINT('Ctrl Pts',(-49.1809368960491,-8.80091402256234,
-235.35005));
#194714=CARTESIAN_POINT('Ctrl Pts',(-49.6155653128172,-8.71134938327683,
-234.668556283135));
#194715=CARTESIAN_POINT('Ctrl Pts',(-48.3871335037843,-8.97820236411209,
-235.35005));
#194716=CARTESIAN_POINT('Ctrl Pts',(-49.1838435713664,-8.81569314774841,
-235.350050000001));
#194717=CARTESIAN_POINT('Ctrl Pts',(-49.6186704393278,-8.7269994720143,
-234.668716968957));
#194718=CARTESIAN_POINT('Ctrl Pts',(-48.392472005857,-9.00451470107218,
-235.35005));
#194719=CARTESIAN_POINT('Ctrl Pts',(-49.1894173582549,-8.84368723057296,
-235.35005));
#194720=CARTESIAN_POINT('Ctrl Pts',(-49.6244440767192,-8.75589699832511,
-234.668851427174));
#194721=CARTESIAN_POINT('Ctrl Pts',(-48.3951203393894,-9.01767332704875,
-235.35005));
#194722=CARTESIAN_POINT('Ctrl Pts',(-49.192181971171,-8.8576866421715,-235.35005));
#194723=CARTESIAN_POINT('Ctrl Pts',(-49.6273078813533,-8.77034819797795,
-234.668918648051));
#194724=CARTESIAN_POINT('Ctrl Pts',(-48.4030026471238,-9.05715657045287,
-235.35005));
#194725=CARTESIAN_POINT('Ctrl Pts',(-49.2004089183163,-8.89969141086334,
-235.35005));
#194726=CARTESIAN_POINT('Ctrl Pts',(-49.6358303332325,-8.81370915928673,
-234.669120288507));
#194727=CARTESIAN_POINT('Ctrl Pts',(-48.4081739296747,-9.08348855318983,
-235.35005));
#194728=CARTESIAN_POINT('Ctrl Pts',(-49.2058046086555,-8.92770451878634,
-235.350049999999));
#194729=CARTESIAN_POINT('Ctrl Pts',(-49.6414200199811,-8.84262628275649,
-234.669254685915));
#194730=CARTESIAN_POINT('Ctrl Pts',(-48.4234374397461,-9.16251391233196,
-235.35005));
#194731=CARTESIAN_POINT('Ctrl Pts',(-49.2217246547772,-9.01177023695605,
-235.350050000003));
#194732=CARTESIAN_POINT('Ctrl Pts',(-49.657913818345,-8.92940752669542,
-234.669657810828));
#194733=CARTESIAN_POINT('Ctrl Pts',(-48.4332793497998,-9.21523669725127,
-235.35005));
#194734=CARTESIAN_POINT('Ctrl Pts',(-49.2319829940889,-9.06785410630298,
-235.350050000001));
#194735=CARTESIAN_POINT('Ctrl Pts',(-49.668542693497,-8.98730151744689,
-234.669926470633));
#194736=CARTESIAN_POINT('Ctrl Pts',(-48.4618064955616,-9.37352237066705,
-235.35005));
#194737=CARTESIAN_POINT('Ctrl Pts',(-49.2616934080035,-9.23621342522619,
-235.350049999999));
#194738=CARTESIAN_POINT('Ctrl Pts',(-49.6993320627288,-9.16110643572959,
-234.67073236696));
#194739=CARTESIAN_POINT('Ctrl Pts',(-48.4794934628256,-9.47920254067735,
-235.35005));
#194740=CARTESIAN_POINT('Ctrl Pts',(-49.2800851841445,-9.34861599525297,
-235.350049999994));
#194741=CARTESIAN_POINT('Ctrl Pts',(-49.7183957005529,-9.277140274608,-234.671269513827));
#194742=CARTESIAN_POINT('Ctrl Pts',(-48.5285710814135,-9.79671102654565,
-235.35005));
#194743=CARTESIAN_POINT('Ctrl Pts',(-49.3310169468997,-9.68627262463685,
-235.350050000012));
#194744=CARTESIAN_POINT('Ctrl Pts',(-49.7712138422074,-9.6257621620448,
-234.672882347017));
#194745=CARTESIAN_POINT('Ctrl Pts',(-48.5559827004535,-10.0090068188063,
-235.35005));
#194746=CARTESIAN_POINT('Ctrl Pts',(-49.3593305570913,-9.91200108309528,
-235.350049999985));
#194747=CARTESIAN_POINT('Ctrl Pts',(-49.8005924106469,-9.8587900325559,
-234.673953662556));
#194748=CARTESIAN_POINT('Ctrl Pts',(-48.6223270802844,-10.6477610876399,
-235.35005));
#194749=CARTESIAN_POINT('Ctrl Pts',(-49.427355877287,-10.5909621394109,
-235.35005000003));
#194750=CARTESIAN_POINT('Ctrl Pts',(-49.8712887313567,-10.5599275885378,
-234.677167109714));
#194751=CARTESIAN_POINT('Ctrl Pts',(-48.6453046118701,-11.0773736644593,
-235.35005));
#194752=CARTESIAN_POINT('Ctrl Pts',(-49.4501374566631,-11.0475237351948,
-235.350050000012));
#194753=CARTESIAN_POINT('Ctrl Pts',(-49.8950789101635,-11.0313011583583,
-234.679301565053));
#194754=CARTESIAN_POINT('Ctrl Pts',(-48.6501328458788,-12.3566962654659,
-235.35005));
#194755=CARTESIAN_POINT('Ctrl Pts',(-49.4504015731985,-12.4060784579424,
-235.350049999976));
#194756=CARTESIAN_POINT('Ctrl Pts',(-49.8961844037889,-12.4347055151062,
-234.685595719225));
#194757=CARTESIAN_POINT('Ctrl Pts',(-48.5694097707421,-13.2010981453996,
-235.35005));
#194758=CARTESIAN_POINT('Ctrl Pts',(-49.3616578254152,-13.3025722383012,
-235.350050000024));
#194759=CARTESIAN_POINT('Ctrl Pts',(-49.8049050012374,-13.3604031808191,
-234.689647068821));
#194760=CARTESIAN_POINT('Ctrl Pts',(-48.3999288819756,-14.0631760578291,
-235.35005));
#194761=CARTESIAN_POINT('Ctrl Pts',(-49.1784903666304,-14.2179091212367,
-235.35005));
#194762=CARTESIAN_POINT('Ctrl Pts',(-49.6163897775734,-14.3049392848125,
-234.693720565574));
#194763=CARTESIAN_POINT('Ctrl Pts',(-48.3947106332052,-14.089291300339,
-235.35005));
#194764=CARTESIAN_POINT('Ctrl Pts',(-49.172856954301,-14.2456147707397,
-235.350050000001));
#194765=CARTESIAN_POINT('Ctrl Pts',(-49.6105868475141,-14.3335523084377,
-234.693843927845));
#194766=CARTESIAN_POINT('Ctrl Pts',(-48.3867592982998,-14.1284516414382,
-235.35005));
#194767=CARTESIAN_POINT('Ctrl Pts',(-49.1642752691847,-14.2871601252974,
-235.35005));
#194768=CARTESIAN_POINT('Ctrl Pts',(-49.6017465855193,-14.3764581150203,
-234.694028868984));
#194769=CARTESIAN_POINT('Ctrl Pts',(-48.3840780941576,-14.1415019811602,
-235.35005));
#194770=CARTESIAN_POINT('Ctrl Pts',(-49.1612266343483,-14.3016684110766,
-235.35005));
#194771=CARTESIAN_POINT('Ctrl Pts',(-49.5985360159632,-14.3917957223577,
-234.694115256963));
#194772=CARTESIAN_POINT('Ctrl Pts',(-48.3787223515611,-14.1676033339819,
-235.35005));
#194773=CARTESIAN_POINT('Ctrl Pts',(-49.1561371684305,-14.326418078323,
-235.35005));
#194774=CARTESIAN_POINT('Ctrl Pts',(-49.5936036508982,-14.415786266369,
-234.694129273138));
#194775=CARTESIAN_POINT('Ctrl Pts',(-48.3760618298762,-14.1806557630565,
-235.35005));
#194776=CARTESIAN_POINT('Ctrl Pts',(-49.1536098434105,-14.3387948688079,
-235.350050000001));
#194777=CARTESIAN_POINT('Ctrl Pts',(-49.5911542470628,-14.4277834533854,
-234.694134995679));
#194778=CARTESIAN_POINT('Ctrl Pts',(-48.3628458825965,-14.2459266629983,
-235.35005));
#194779=CARTESIAN_POINT('Ctrl Pts',(-49.1410602317348,-14.4006882956361,
-235.350049999995));
#194780=CARTESIAN_POINT('Ctrl Pts',(-49.5789910512861,-14.4877788919854,
-234.694157190572));
#194781=CARTESIAN_POINT('Ctrl Pts',(-48.3525504293568,-14.2981713963959,
-235.35005));
#194782=CARTESIAN_POINT('Ctrl Pts',(-49.1312987239013,-14.4502345980385,
-235.35005));
#194783=CARTESIAN_POINT('Ctrl Pts',(-49.5695287198168,-14.5358056523908,
-234.694154412176));
#194784=CARTESIAN_POINT('Ctrl Pts',(-48.3224929218234,-14.4549893276864,
-235.35005));
#194785=CARTESIAN_POINT('Ctrl Pts',(-49.1028465494228,-14.5989634011547,
-235.35005));
#194786=CARTESIAN_POINT('Ctrl Pts',(-49.5419439476953,-14.6799744510311,
-234.694084786526));
#194787=CARTESIAN_POINT('Ctrl Pts',(-48.3035595793916,-14.5596462424765,
-235.35005));
#194788=CARTESIAN_POINT('Ctrl Pts',(-49.0849874724743,-14.6982394950892,
-235.350049999998));
#194789=CARTESIAN_POINT('Ctrl Pts',(-49.5246236070435,-14.7762049884194,
-234.693956683334));
#194790=CARTESIAN_POINT('Ctrl Pts',(-48.2500551817889,-14.8739499130376,
-235.35005));
#194791=CARTESIAN_POINT('Ctrl Pts',(-49.0347221330771,-14.9964132146763,
-235.350050000003));
#194792=CARTESIAN_POINT('Ctrl Pts',(-49.4758559537979,-15.0652295831884,
-234.69332855221));
#194793=CARTESIAN_POINT('Ctrl Pts',(-48.2187775910813,-15.0839293763448,
-235.35005));
#194794=CARTESIAN_POINT('Ctrl Pts',(-49.0056251748038,-15.1956711360348,
-235.350049999997));
#194795=CARTESIAN_POINT('Ctrl Pts',(-49.447600122929,-15.2583563846847,
-234.692585242987));
#194796=CARTESIAN_POINT('Ctrl Pts',(-48.1380456036249,-15.7151912142403,
-235.35005));
#194797=CARTESIAN_POINT('Ctrl Pts',(-48.9315200735598,-15.7947230301441,
-235.350050000006));
#194798=CARTESIAN_POINT('Ctrl Pts',(-49.3755486131225,-15.8389090912121,
-234.689371821595));
#194799=CARTESIAN_POINT('Ctrl Pts',(-48.1017687499515,-16.1377801895033,
-235.35005));
#194800=CARTESIAN_POINT('Ctrl Pts',(-48.8997990349571,-16.1958775231026,
-235.350049999994));
#194801=CARTESIAN_POINT('Ctrl Pts',(-49.3445349115517,-16.2275468702548,
-234.68591772599));
#194802=CARTESIAN_POINT('Ctrl Pts',(-48.0452056587669,-17.4030250963116,
-235.35005));
#194803=CARTESIAN_POINT('Ctrl Pts',(-48.8571760735594,-17.3969404754266,
-235.350050000012));
#194804=CARTESIAN_POINT('Ctrl Pts',(-49.3020545258986,-17.3907951876548,
-234.671624111816));
#194805=CARTESIAN_POINT('Ctrl Pts',(-48.0765553834797,-18.2457723122435,
-235.35005));
#194806=CARTESIAN_POINT('Ctrl Pts',(-48.8989420124693,-18.1971730763996,
-235.350049999929));
#194807=CARTESIAN_POINT('Ctrl Pts',(-49.3406485147144,-18.164819270942,
-234.656852423361));
#194808=CARTESIAN_POINT('Ctrl Pts',(-48.202136382695,-19.2982688285888,
-235.35005));
#194809=CARTESIAN_POINT('Ctrl Pts',(-49.0372739509851,-19.1873904238028,
-235.350050000017));
#194810=CARTESIAN_POINT('Ctrl Pts',(-49.4718969222247,-19.1292954138514,
-234.630751354067));
#194811=CARTESIAN_POINT('Ctrl Pts',(-48.2315724527526,-19.5085474359625,
-235.35005));
#194812=CARTESIAN_POINT('Ctrl Pts',(-49.0694140435013,-19.3857696629781,
-235.350049999994));
#194813=CARTESIAN_POINT('Ctrl Pts',(-49.5022925238141,-19.3218807036188,
-234.625150148995));
#194814=CARTESIAN_POINT('Ctrl Pts',(-48.2737849902378,-19.7710257016811,
-235.35005));
#194815=CARTESIAN_POINT('Ctrl Pts',(-49.11500096125,-19.6328314628528,-235.350050000002));
#194816=CARTESIAN_POINT('Ctrl Pts',(-49.5454678269032,-19.5620862891172,
-234.617636622494));
#194817=CARTESIAN_POINT('Ctrl Pts',(-48.2824987027496,-19.82350433647,-235.35005));
#194818=CARTESIAN_POINT('Ctrl Pts',(-49.1244019347077,-19.682263630747,
-235.350049999999));
#194819=CARTESIAN_POINT('Ctrl Pts',(-49.5543622366061,-19.6101024448334,
-234.616108235133));
#194820=CARTESIAN_POINT('Ctrl Pts',(-48.2959770869867,-19.9021966978926,
-235.35005));
#194821=CARTESIAN_POINT('Ctrl Pts',(-49.1389129882989,-19.7563522352633,
-235.35005));
#194822=CARTESIAN_POINT('Ctrl Pts',(-49.5680934468262,-19.6820882105088,
-234.613776279329));
#194823=CARTESIAN_POINT('Ctrl Pts',(-48.3005378529525,-19.9284232197851,
-235.35005));
#194824=CARTESIAN_POINT('Ctrl Pts',(-49.1438196314223,-19.7810450643495,
-235.350050000005));
#194825=CARTESIAN_POINT('Ctrl Pts',(-49.5727354507713,-19.7060770526268,
-234.612992397751));
#194826=CARTESIAN_POINT('Ctrl Pts',(-48.3074811028276,-19.9677565956903,
-235.35005));
#194827=CARTESIAN_POINT('Ctrl Pts',(-49.1512821856062,-19.8180692694358,
-235.350049999998));
#194828=CARTESIAN_POINT('Ctrl Pts',(-49.5797959434908,-19.7420505664417,
-234.61180661903));
#194829=CARTESIAN_POINT('Ctrl Pts',(-48.3098125363869,-19.9808666531709,
-235.35005));
#194830=CARTESIAN_POINT('Ctrl Pts',(-49.1537871425354,-19.8304098086682,
-235.350050000001));
#194831=CARTESIAN_POINT('Ctrl Pts',(-49.5821656888743,-19.7540401124037,
-234.611409700054));
#194832=CARTESIAN_POINT('Ctrl Pts',(-48.3145094629338,-20.0070846308637,
-235.35005));
#194833=CARTESIAN_POINT('Ctrl Pts',(-49.1588315088273,-19.855086940684,
-235.350049999999));
#194834=CARTESIAN_POINT('Ctrl Pts',(-49.5869376908479,-19.7780159321077,
-234.610612524155));
#194835=CARTESIAN_POINT('Ctrl Pts',(-48.3168699427918,-20.0201928656617,
-235.35005));
#194836=CARTESIAN_POINT('Ctrl Pts',(-49.1609637431947,-19.869444669877,
-235.35005));
#194837=CARTESIAN_POINT('Ctrl Pts',(-49.5892803760666,-19.7929526511806,
-234.611191018229));
#194838=CARTESIAN_POINT('Ctrl Pts',(-48.3378149961279,-20.1381857579918,
-235.35005));
#194839=CARTESIAN_POINT('Ctrl Pts',(-49.1803832875034,-19.9958192386853,
-235.350050000002));
#194840=CARTESIAN_POINT('Ctrl Pts',(-49.6101145207749,-19.9233239035134,
-234.615047470178));
#194841=CARTESIAN_POINT('Ctrl Pts',(-48.3550896009133,-20.2431526171789,
-235.35005));
#194842=CARTESIAN_POINT('Ctrl Pts',(-49.1962287252122,-20.1082560487782,
-235.350049999994));
#194843=CARTESIAN_POINT('Ctrl Pts',(-49.6271396690249,-20.0392626516645,
-234.618456601287));
#194844=CARTESIAN_POINT('Ctrl Pts',(-48.4347895563001,-20.7684056538746,
-235.35005));
#194845=CARTESIAN_POINT('Ctrl Pts',(-49.2681921281626,-20.6693028847357,
-235.350050000023));
#194846=CARTESIAN_POINT('Ctrl Pts',(-49.7048510075002,-20.6191868386639,
-234.635401433285));
#194847=CARTESIAN_POINT('Ctrl Pts',(-48.4772403630273,-21.1899452510999,
-235.35005));
#194848=CARTESIAN_POINT('Ctrl Pts',(-49.3034028549804,-21.1195336358382,
-235.35005));
#194849=CARTESIAN_POINT('Ctrl Pts',(-49.7433516745446,-21.0837395665231,
-234.64859809159));
#194850=CARTESIAN_POINT('Ctrl Pts',(-48.5415386498259,-22.458520743411,
-235.35005));
#194851=CARTESIAN_POINT('Ctrl Pts',(-49.3419650219896,-22.4675064520562,
-235.35005));
#194852=CARTESIAN_POINT('Ctrl Pts',(-49.7892124454036,-22.4793485342635,
-234.687225534828));
#194853=CARTESIAN_POINT('Ctrl Pts',(-48.5005032094983,-23.311667738302,
-235.35005));
#194854=CARTESIAN_POINT('Ctrl Pts',(-49.2800794163868,-23.3730401250582,
-235.35005));
#194855=CARTESIAN_POINT('Ctrl Pts',(-49.7271015354622,-23.4144460560838,
-234.711697624812));
#194856=CARTESIAN_POINT('Ctrl Pts',(-48.3390590324706,-24.3778343529881,
-235.35005));
#194857=CARTESIAN_POINT('Ctrl Pts',(-49.086074667266,-24.5037177534246,
-235.35005));
#194858=CARTESIAN_POINT('Ctrl Pts',(-49.5294900946094,-24.5788354560032,
-234.740523989368));
#194859=CARTESIAN_POINT('Ctrl Pts',(-48.3012455308433,-24.5909867391319,
-235.35005));
#194860=CARTESIAN_POINT('Ctrl Pts',(-49.0416655455856,-24.7287449779651,
-235.350050000018));
#194861=CARTESIAN_POINT('Ctrl Pts',(-49.4839495431616,-24.8114203403136,
-234.746200830511));
#194862=CARTESIAN_POINT('Ctrl Pts',(-48.2523434883265,-24.8306899717521,
-235.35005));
#194863=CARTESIAN_POINT('Ctrl Pts',(-48.9850331973951,-24.9817901079185,
-235.350049999998));
#194864=CARTESIAN_POINT('Ctrl Pts',(-49.4258297714769,-25.0727001745,-234.752473563172));
#194865=CARTESIAN_POINT('Ctrl Pts',(-48.2468215385715,-24.857322369352,
-235.35005));
#194866=CARTESIAN_POINT('Ctrl Pts',(-48.9786554175451,-25.0098727669535,
-235.350049999997));
#194867=CARTESIAN_POINT('Ctrl Pts',(-49.4192763488556,-25.1017260271132,
-234.753168950875));
#194868=CARTESIAN_POINT('Ctrl Pts',(-48.2356002982336,-24.910584566504,
-235.35005));
#194869=CARTESIAN_POINT('Ctrl Pts',(-48.9657159328337,-25.0660281153669,
-235.350050000003));
#194870=CARTESIAN_POINT('Ctrl Pts',(-49.4059777280254,-25.1597670748574,
-234.754556505762));
#194871=CARTESIAN_POINT('Ctrl Pts',(-48.2299135975692,-24.9372145504824,
-235.35005));
#194872=CARTESIAN_POINT('Ctrl Pts',(-48.9608504508884,-25.0911588778292,
-235.350049999999));
#194873=CARTESIAN_POINT('Ctrl Pts',(-49.4013021218481,-25.1839185178113,
-234.753925525474));
#194874=CARTESIAN_POINT('Ctrl Pts',(-48.2132345171348,-25.0171100844526,
-235.35005));
#194875=CARTESIAN_POINT('Ctrl Pts',(-48.946142631535,-25.1674232304628,
-235.350050000002));
#194876=CARTESIAN_POINT('Ctrl Pts',(-49.3870431573761,-25.2578284787265,
-234.752406627079));
#194877=CARTESIAN_POINT('Ctrl Pts',(-48.2024091551349,-25.0703780812323,
-235.35005));
#194878=CARTESIAN_POINT('Ctrl Pts',(-48.9366357051972,-25.2182625009279,
-235.350049999999));
#194879=CARTESIAN_POINT('Ctrl Pts',(-49.3778231822086,-25.3071039363646,
-234.751372563654));
#194880=CARTESIAN_POINT('Ctrl Pts',(-48.1708085736138,-25.2301948978772,
-235.35005));
#194881=CARTESIAN_POINT('Ctrl Pts',(-48.9089945694079,-25.3708143302532,
-235.350050000001));
#194882=CARTESIAN_POINT('Ctrl Pts',(-49.3510150827827,-25.454934683882,
-234.748205410904));
#194883=CARTESIAN_POINT('Ctrl Pts',(-48.1509087141736,-25.3367565417747,
-235.35005));
#194884=CARTESIAN_POINT('Ctrl Pts',(-48.8917526157755,-25.4724994483113,
-235.350050000001));
#194885=CARTESIAN_POINT('Ctrl Pts',(-49.3342786576262,-25.5534943522782,
-234.746007383865));
#194886=CARTESIAN_POINT('Ctrl Pts',(-48.0571667807649,-25.8696491072789,
-235.35005));
#194887=CARTESIAN_POINT('Ctrl Pts',(-48.811261859734,-25.9816228925711,
-235.350049999994));
#194888=CARTESIAN_POINT('Ctrl Pts',(-49.2562000930912,-26.0462949080656,
-234.734575161191));
#194889=CARTESIAN_POINT('Ctrl Pts',(-48.000556289185,-26.2962324730956,
-235.35005));
#194890=CARTESIAN_POINT('Ctrl Pts',(-48.7656505977619,-26.3885598012182,
-235.350049999982));
#194891=CARTESIAN_POINT('Ctrl Pts',(-49.211634953002,-26.4405395961576,
-234.724022357095));
#194892=CARTESIAN_POINT('Ctrl Pts',(-47.8838810362842,-27.5767613139966,
-235.35005));
#194893=CARTESIAN_POINT('Ctrl Pts',(-48.6827507003063,-27.6106377649942,
-235.350050000036));
#194894=CARTESIAN_POINT('Ctrl Pts',(-49.1296257840991,-27.6223459390551,
-234.687604363246));
#194895=CARTESIAN_POINT('Ctrl Pts',(-47.876633025442,-28.431480559278,-235.35005));
#194896=CARTESIAN_POINT('Ctrl Pts',(-48.7005291317402,-28.4246911972351,
-235.350049999953));
#194897=CARTESIAN_POINT('Ctrl Pts',(-49.1434150770831,-28.4094549490855,
-234.657217580316));
#194898=CARTESIAN_POINT('Ctrl Pts',(-48.0026713456265,-30.1816730688289,
-235.35005));
#194899=CARTESIAN_POINT('Ctrl Pts',(-48.8799154192025,-30.0782314618698,
-235.35005000005));
#194900=CARTESIAN_POINT('Ctrl Pts',(-49.3058185785018,-30.0154916213199,
-234.579129604302));
#194901=CARTESIAN_POINT('Ctrl Pts',(-48.1423359832808,-31.0772709955632,
-235.35005));
#194902=CARTESIAN_POINT('Ctrl Pts',(-49.0516357944767,-30.9231333337257,
-235.350050000035));
#194903=CARTESIAN_POINT('Ctrl Pts',(-49.4605472095348,-30.8341434889496,
-234.530604785809));
#194904=CARTESIAN_POINT('Ctrl Pts',(-48.3606172463808,-31.9739539840651,
-235.35005));
#194905=CARTESIAN_POINT('Ctrl Pts',(-49.2988059683443,-31.7455385989255,
-235.350049999995));
#194906=CARTESIAN_POINT('Ctrl Pts',(-49.6872475187014,-31.6509467871898,
-234.471114721056));
#194907=CARTESIAN_POINT('',(-49.6580996754574,-31.5448418565169,-234.479004868619));
#194908=CARTESIAN_POINT('',(-48.3327003568643,-31.8574637039841,-235.35005));
#194909=CARTESIAN_POINT('Origin',(-48.3327003568642,-31.8574637039841,-233.85005));
#194910=CARTESIAN_POINT('',(-49.4065653148269,-25.1565430143321,-234.754641484296));
#194911=CARTESIAN_POINT('Ctrl Pts',(-49.6580996754575,-31.5448418565169,
-234.479004868619));
#194912=CARTESIAN_POINT('Ctrl Pts',(-49.590346126536,-31.2938113421995,
-234.497007566398));
#194913=CARTESIAN_POINT('Ctrl Pts',(-49.5294056430117,-31.0426055563327,
-234.513982723729));
#194914=CARTESIAN_POINT('Ctrl Pts',(-49.4752396727556,-30.7912125751541,
-234.529999882613));
#194915=CARTESIAN_POINT('Ctrl Pts',(-49.4410958566977,-30.6327456324031,
-234.540096386453));
#194916=CARTESIAN_POINT('Ctrl Pts',(-49.4096449111297,-30.4742042661059,
-234.549812231499));
#194917=CARTESIAN_POINT('Ctrl Pts',(-49.3808878256904,-30.3155859402117,
-234.559164835971));
#194918=CARTESIAN_POINT('Ctrl Pts',(-49.3353805488539,-30.0645769120863,
-234.57396506883));
#194919=CARTESIAN_POINT('Ctrl Pts',(-49.2966167553167,-29.8133745672487,
-234.587855668465));
#194920=CARTESIAN_POINT('Ctrl Pts',(-49.2645915793269,-29.5619803241126,
-234.600905660719));
#194921=CARTESIAN_POINT('Ctrl Pts',(-49.232878789184,-29.3130382768225,
-234.613828358344));
#194922=CARTESIAN_POINT('Ctrl Pts',(-49.2077738585867,-29.0639076727252,
-234.625926767819));
#194923=CARTESIAN_POINT('Ctrl Pts',(-49.1893215480184,-28.8146023258056,
-234.637267914711));
#194924=CARTESIAN_POINT('Ctrl Pts',(-49.1831955148801,-28.7318347606741,
-234.641033093139));
#194925=CARTESIAN_POINT('Ctrl Pts',(-49.177803131853,-28.6490480630386,
-234.644714806706));
#194926=CARTESIAN_POINT('Ctrl Pts',(-49.1731472439229,-28.5662431585057,
-234.64831550801));
#194927=CARTESIAN_POINT('Ctrl Pts',(-49.1692623684599,-28.497150700383,
-234.651319935169));
#194928=CARTESIAN_POINT('Ctrl Pts',(-49.1658902704926,-28.4280455697387,
-234.654267959623));
#194929=CARTESIAN_POINT('Ctrl Pts',(-49.163031882372,-28.3589283663495,
-234.65716100616));
#194930=CARTESIAN_POINT('Ctrl Pts',(-49.1525743380049,-28.1060598997706,
-234.667745349937));
#194931=CARTESIAN_POINT('Ctrl Pts',(-49.1489996771991,-27.8530509491739,
-234.677576545427));
#194932=CARTESIAN_POINT('Ctrl Pts',(-49.1523917163603,-27.5999159742951,
-234.68671666602));
#194933=CARTESIAN_POINT('Ctrl Pts',(-49.1555766840377,-27.362233956278,
-234.695298815952));
#194934=CARTESIAN_POINT('Ctrl Pts',(-49.1649042233204,-27.1244406564733,
-234.703271690739));
#194935=CARTESIAN_POINT('Ctrl Pts',(-49.1804897356957,-26.886572392946,
-234.71068667557));
#194936=CARTESIAN_POINT('Ctrl Pts',(-49.1815030317473,-26.8711073272851,
-234.711168762695));
#194937=CARTESIAN_POINT('Ctrl Pts',(-49.1825427958084,-26.8556419543378,
-234.711648491628));
#194938=CARTESIAN_POINT('Ctrl Pts',(-49.1836090661316,-26.8401762881947,
-234.712125876492));
#194939=CARTESIAN_POINT('Ctrl Pts',(-49.1854658975133,-26.8132439675545,
-234.712957207137));
#194940=CARTESIAN_POINT('Ctrl Pts',(-49.1874031105211,-26.7863107575068,
-234.713781429235));
#194941=CARTESIAN_POINT('Ctrl Pts',(-49.1894208472892,-26.7593767202999,
-234.714598617361));
#194942=CARTESIAN_POINT('Ctrl Pts',(-49.2071135019829,-26.5232038818332,
-234.721764184036));
#194943=CARTESIAN_POINT('Ctrl Pts',(-49.2310148167691,-26.2869277163969,
-234.728364686713));
#194944=CARTESIAN_POINT('Ctrl Pts',(-49.2612614314676,-26.0506127383107,
-234.734435211101));
#194945=CARTESIAN_POINT('Ctrl Pts',(-49.2651872190284,-26.019940796652,
-234.735223120405));
#194946=CARTESIAN_POINT('Ctrl Pts',(-49.2692199568921,-25.9892682458034,
-234.736002101628));
#194947=CARTESIAN_POINT('Ctrl Pts',(-49.2733599943998,-25.9585952679501,
-234.736772231484));
#194948=CARTESIAN_POINT('Ctrl Pts',(-49.2913786753514,-25.8250972982491,
-234.740124066862));
#194949=CARTESIAN_POINT('Ctrl Pts',(-49.3114284827361,-25.6915901763045,
-234.743309777531));
#194950=CARTESIAN_POINT('Ctrl Pts',(-49.3335417708821,-25.5580868232228,
-234.746335595632));
#194951=CARTESIAN_POINT('Ctrl Pts',(-49.344598414955,-25.4913351466819,
-234.747848504682));
#194952=CARTESIAN_POINT('Ctrl Pts',(-49.3561712624554,-25.4245844267277,
-234.749321105246));
#194953=CARTESIAN_POINT('Ctrl Pts',(-49.3682650086808,-25.3578363353345,
-234.750754002269));
#194954=CARTESIAN_POINT('Ctrl Pts',(-49.3743118817935,-25.3244622896378,
-234.751470450781));
#194955=CARTESIAN_POINT('Ctrl Pts',(-49.3804889830364,-25.2910889018601,
-234.752176976097));
#194956=CARTESIAN_POINT('Ctrl Pts',(-49.3867969582897,-25.2577163848095,
-234.752873621892));
#194957=CARTESIAN_POINT('Ctrl Pts',(-49.3913647572992,-25.233550318171,
-234.753378084551));
#194958=CARTESIAN_POINT('Ctrl Pts',(-49.3956861054634,-25.2101556288682,
-234.754075989134));
#194959=CARTESIAN_POINT('Ctrl Pts',(-49.4006156889099,-25.1854554901182,
-234.754424809087));
#194960=CARTESIAN_POINT('Ctrl Pts',(-49.4024936927336,-25.1760455763752,
-234.754557697639));
#194961=CARTESIAN_POINT('Ctrl Pts',(-49.4044604812417,-25.1664462685349,
-234.754639921753));
#194962=CARTESIAN_POINT('Ctrl Pts',(-49.4065653148269,-25.1565430143321,
-234.754641484296));
#194963=CARTESIAN_POINT('',(-49.5863631216035,-19.7758588045606,-234.610932138786));
#194964=CARTESIAN_POINT('Ctrl Pts',(-49.4065714250583,-25.1565443079239,
-234.754646206088));
#194965=CARTESIAN_POINT('Ctrl Pts',(-49.4083225452229,-25.1482850280493,
-234.754642899617));
#194966=CARTESIAN_POINT('Ctrl Pts',(-49.41020323589,-25.1397150740938,-234.754554876728));
#194967=CARTESIAN_POINT('Ctrl Pts',(-49.4122755477287,-25.1306724979893,
-234.754338313619));
#194968=CARTESIAN_POINT('Ctrl Pts',(-49.4166128694744,-25.111746503724,
-234.753885049844));
#194969=CARTESIAN_POINT('Ctrl Pts',(-49.4209094077061,-25.0928182406844,
-234.753431099368));
#194970=CARTESIAN_POINT('Ctrl Pts',(-49.4251652238492,-25.0738877287661,
-234.752976469689));
#194971=CARTESIAN_POINT('Ctrl Pts',(-49.427434911034,-25.0637918179333,
-234.752734009225));
#194972=CARTESIAN_POINT('Ctrl Pts',(-49.4296930160082,-25.0536952676186,
-234.752491355368));
#194973=CARTESIAN_POINT('Ctrl Pts',(-49.4319395478169,-25.0435980813769,
-234.752248509462));
#194974=CARTESIAN_POINT('Ctrl Pts',(-49.4359180394011,-25.0257164870321,
-234.751818441929));
#194975=CARTESIAN_POINT('Ctrl Pts',(-49.4398602422247,-25.0078328970427,
-234.751387773391));
#194976=CARTESIAN_POINT('Ctrl Pts',(-49.4437662024039,-24.9899473318732,
-234.750956510672));
#194977=CARTESIAN_POINT('Ctrl Pts',(-49.4559892738732,-24.9339773446458,
-234.749606943654));
#194978=CARTESIAN_POINT('Ctrl Pts',(-49.4678574396967,-24.8779880059922,
-234.748251547475));
#194979=CARTESIAN_POINT('Ctrl Pts',(-49.4793721424816,-24.8219799161756,
-234.746890499776));
#194980=CARTESIAN_POINT('Ctrl Pts',(-49.5024015480513,-24.7099637365424,
-234.744168404378));
#194981=CARTESIAN_POINT('Ctrl Pts',(-49.524017101493,-24.5978725522242,
-234.741423702898));
#194982=CARTESIAN_POINT('Ctrl Pts',(-49.5442303524539,-24.4857111577519,
-234.738657807323));
#194983=CARTESIAN_POINT('Ctrl Pts',(-49.552626376232,-24.4391224255984,
-234.73750893102));
#194984=CARTESIAN_POINT('Ctrl Pts',(-49.5607804549896,-24.3925215798048,
-234.736356398016));
#194985=CARTESIAN_POINT('Ctrl Pts',(-49.5686934164371,-24.3459089640037,
-234.735200309511));
#194986=CARTESIAN_POINT('Ctrl Pts',(-49.7268222749508,-23.4144246167288,
-234.71209758661));
#194987=CARTESIAN_POINT('Ctrl Pts',(-49.7889759213309,-22.4793462204463,
-234.687578993421));
#194988=CARTESIAN_POINT('Ctrl Pts',(-49.7584449475999,-21.548951679417,
-234.661775242303));
#194989=CARTESIAN_POINT('Ctrl Pts',(-49.7431794607344,-21.0837544089024,
-234.648873366744));
#194990=CARTESIAN_POINT('Ctrl Pts',(-49.704700149341,-20.6192049141822,
-234.63564923189));
#194991=CARTESIAN_POINT('Ctrl Pts',(-49.6425520532046,-20.155267103844,
-234.622064432487));
#194992=CARTESIAN_POINT('Ctrl Pts',(-49.6405496054477,-20.1403187581116,
-234.621626722359));
#194993=CARTESIAN_POINT('Ctrl Pts',(-49.6385225254361,-20.1253711747348,
-234.621188675716));
#194994=CARTESIAN_POINT('Ctrl Pts',(-49.636470789184,-20.1104243691117,
-234.620750295427));
#194995=CARTESIAN_POINT('Ctrl Pts',(-49.6249635842442,-20.0265949025698,
-234.618291630563));
#194996=CARTESIAN_POINT('Ctrl Pts',(-49.6126808048582,-19.9427899006565,
-234.615822470671));
#194997=CARTESIAN_POINT('Ctrl Pts',(-49.5996182194956,-19.8590120799471,
-234.613343321822));
#194998=CARTESIAN_POINT('Ctrl Pts',(-49.5969386465566,-19.8418264482341,
-234.612834765515));
#194999=CARTESIAN_POINT('Ctrl Pts',(-49.5942262585936,-19.824641947958,
-234.612325786926));
#195000=CARTESIAN_POINT('Ctrl Pts',(-49.5914810209125,-19.8074586253538,
-234.611816394022));
#195001=CARTESIAN_POINT('Ctrl Pts',(-49.5897653609845,-19.7967197599277,
-234.61149804454));
#195002=CARTESIAN_POINT('Ctrl Pts',(-49.5880344428409,-19.7857330389408,
-234.611097274937));
#195003=CARTESIAN_POINT('Ctrl Pts',(-49.5862818832396,-19.7758835630004,
-234.611073196375));
#195004=CARTESIAN_POINT('',(-49.6141588435918,-8.70526933620937,-234.668797542549));
#195005=CARTESIAN_POINT('Ctrl Pts',(-49.586393185248,-19.775849642277,-234.610879938015));
#195006=CARTESIAN_POINT('Ctrl Pts',(-49.5856686445096,-19.7724384225141,
-234.611065158657));
#195007=CARTESIAN_POINT('Ctrl Pts',(-49.585055184216,-19.7691449560952,
-234.61110291388));
#195008=CARTESIAN_POINT('Ctrl Pts',(-49.5820527790106,-19.7540602415442,
-234.61160435363));
#195009=CARTESIAN_POINT('Ctrl Pts',(-49.5796829880909,-19.7420706048251,
-234.612001185075));
#195010=CARTESIAN_POINT('Ctrl Pts',(-49.5726223597956,-19.7060968192221,
-234.613186702187));
#195011=CARTESIAN_POINT('Ctrl Pts',(-49.5679802665039,-19.6821077948723,
-234.613970410723));
#195012=CARTESIAN_POINT('Ctrl Pts',(-49.5542487923194,-19.6101214844369,
-234.616301851302));
#195013=CARTESIAN_POINT('Ctrl Pts',(-49.5453542107186,-19.5621049613933,
-234.617829900602));
#195014=CARTESIAN_POINT('Ctrl Pts',(-49.5021780821526,-19.3218975941556,
-234.625341761091));
#195015=CARTESIAN_POINT('Ctrl Pts',(-49.47178187823,-19.1293107914889,-234.630941719413));
#195016=CARTESIAN_POINT('Ctrl Pts',(-49.3405309283227,-18.1648278835588,
-234.657036929293));
#195017=CARTESIAN_POINT('Ctrl Pts',(-49.3019357180199,-17.3907968286783,
-234.671805261636));
#195018=CARTESIAN_POINT('Ctrl Pts',(-49.3444157773257,-16.2275383867562,
-234.686095603872));
#195019=CARTESIAN_POINT('Ctrl Pts',(-49.375429580623,-15.8388972460656,
-234.689548905031));
#195020=CARTESIAN_POINT('Ctrl Pts',(-49.447481559703,-15.2583395688747,
-234.692761586072));
#195021=CARTESIAN_POINT('Ctrl Pts',(-49.4757375974629,-15.065211119735,
-234.693504723861));
#195022=CARTESIAN_POINT('Ctrl Pts',(-49.5245056367494,-14.7761840674541,
-234.694132710065));
#195023=CARTESIAN_POINT('Ctrl Pts',(-49.541826118748,-14.6799527122396,
-234.694260783696));
#195024=CARTESIAN_POINT('Ctrl Pts',(-49.5694111218869,-14.5357826896111,
-234.694330393278));
#195025=CARTESIAN_POINT('Ctrl Pts',(-49.5788735335699,-14.4877555214266,
-234.694333171033));
#195026=CARTESIAN_POINT('Ctrl Pts',(-49.5910368335956,-14.4277595736188,
-234.694310981262));
#195027=CARTESIAN_POINT('Ctrl Pts',(-49.5934862584839,-14.4157622847663,
-234.694305260041));
#195028=CARTESIAN_POINT('Ctrl Pts',(-49.5984186660568,-14.3917715371195,
-234.694291247101));
#195029=CARTESIAN_POINT('Ctrl Pts',(-49.601629194319,-14.3764341527676,
-234.694204879058));
#195030=CARTESIAN_POINT('Ctrl Pts',(-49.6104693915555,-14.3335287121791,
-234.694019980594));
#195031=CARTESIAN_POINT('Ctrl Pts',(-49.6162722792166,-14.3049159326432,
-234.693896646787));
#195032=CARTESIAN_POINT('Ctrl Pts',(-49.8047861711799,-13.3603876769755,
-234.689824088937));
#195033=CARTESIAN_POINT('Ctrl Pts',(-49.8960649973424,-12.4346978471695,
-234.685773671066));
#195034=CARTESIAN_POINT('Ctrl Pts',(-49.8949598896238,-11.0313054978619,
-234.679480960353));
#195035=CARTESIAN_POINT('Ctrl Pts',(-49.8711700349691,-10.5599358864017,
-234.677346993428));
#195036=CARTESIAN_POINT('Ctrl Pts',(-49.8004745098102,-9.85880425002941,
-234.674134280509));
#195037=CARTESIAN_POINT('Ctrl Pts',(-49.7710962529965,-9.6257783261272,
-234.673063209476));
#195038=CARTESIAN_POINT('Ctrl Pts',(-49.7182786558539,-9.27715936120124,
-234.671450744111));
#195039=CARTESIAN_POINT('Ctrl Pts',(-49.6992152109465,-9.16112648968467,
-234.670913719678));
#195040=CARTESIAN_POINT('Ctrl Pts',(-49.6684261500172,-8.98732302167439,
-234.670108006972));
#195041=CARTESIAN_POINT('Ctrl Pts',(-49.6577973805173,-8.92942951287929,
-234.669839408363));
#195042=CARTESIAN_POINT('Ctrl Pts',(-49.641303745405,-8.84264899186087,
-234.669436375258));
#195043=CARTESIAN_POINT('Ctrl Pts',(-49.6357141138013,-8.81373210902702,
-234.669302008454));
#195044=CARTESIAN_POINT('Ctrl Pts',(-49.6271917458389,-8.77037150869081,
-234.669100413908));
#195045=CARTESIAN_POINT('Ctrl Pts',(-49.6243279693599,-8.75592042928144,
-234.669033208336));
#195046=CARTESIAN_POINT('Ctrl Pts',(-49.619010147934,-8.72930425914983,
-234.668909392277));
#195047=CARTESIAN_POINT('Ctrl Pts',(-49.6164243197397,-8.71628486654336,
-234.668786528383));
#195048=CARTESIAN_POINT('Ctrl Pts',(-49.6141588435918,-8.70526933620937,
-234.668797542549));
#195049=CARTESIAN_POINT('',(-49.5702506762146,-3.34422295956514,-234.635326079404));
#195050=CARTESIAN_POINT('Ctrl Pts',(-49.6141588435918,-8.70526933620937,
-234.668797542549));
#195051=CARTESIAN_POINT('Ctrl Pts',(-49.6137159717685,-8.7032079193402,
-234.668825566832));
#195052=CARTESIAN_POINT('Ctrl Pts',(-49.6132991067888,-8.70121390385896,
-234.668837203907));
#195053=CARTESIAN_POINT('Ctrl Pts',(-49.4494831990987,-7.92721199780516,
-234.676385127567));
#195054=CARTESIAN_POINT('Ctrl Pts',(-49.354763767086,-7.14595069243807,
-234.678429733985));
#195055=CARTESIAN_POINT('Ctrl Pts',(-49.3161672816753,-5.96285252589225,
-234.673513733305));
#195056=CARTESIAN_POINT('Ctrl Pts',(-49.3207737741258,-5.56761683301845,
-234.670516269794));
#195057=CARTESIAN_POINT('Ctrl Pts',(-49.3643010504721,-4.7824439659427,
-234.66181072458));
#195058=CARTESIAN_POINT('Ctrl Pts',(-49.4032038353068,-4.39163744274392,
-234.656081092301));
#195059=CARTESIAN_POINT('Ctrl Pts',(-49.4870286161152,-3.80808467387458,
-234.645331813477));
#195060=CARTESIAN_POINT('Ctrl Pts',(-49.5192166088196,-3.61402952773642,
-234.641386355201));
#195061=CARTESIAN_POINT('Ctrl Pts',(-49.5602193207635,-3.39629338221077,
-234.636512404777));
#195062=CARTESIAN_POINT('Ctrl Pts',(-49.5648417594533,-3.37210848059925,
-234.635964796292));
#195063=CARTESIAN_POINT('Ctrl Pts',(-49.569763243633,-3.34673339462103,
-234.63538362583));
#195064=CARTESIAN_POINT('Ctrl Pts',(-49.5699972088521,-3.34549415662508,
-234.63536535131));
#195065=CARTESIAN_POINT('Ctrl Pts',(-49.5702506762146,-3.34422295956515,
-234.635326079404));
#195066=CARTESIAN_POINT('',(-49.4221349129046,2.07190323615638,-234.730930503295));
#195067=CARTESIAN_POINT('Ctrl Pts',(-49.5702506762145,-3.34422295956514,
-234.635326079404));
#195068=CARTESIAN_POINT('Ctrl Pts',(-49.5725443585339,-3.33171731241385,
-234.635256188693));
#195069=CARTESIAN_POINT('Ctrl Pts',(-49.5749633883434,-3.31606110740682,
-234.635858145233));
#195070=CARTESIAN_POINT('Ctrl Pts',(-49.5772982878406,-3.30190915561709,
-234.63612532881));
#195071=CARTESIAN_POINT('Ctrl Pts',(-49.5796331873378,-3.28775720382736,
-234.636392512386));
#195072=CARTESIAN_POINT('Ctrl Pts',(-49.5819461014599,-3.27360360893774,
-234.636659600886));
#195073=CARTESIAN_POINT('Ctrl Pts',(-49.5842370427662,-3.2594483830597,
-234.636926593251));
#195074=CARTESIAN_POINT('Ctrl Pts',(-49.5888189253789,-3.23113793130363,
-234.637460577982));
#195075=CARTESIAN_POINT('Ctrl Pts',(-49.5933129168553,-3.20282095561616,
-234.637994178256));
#195076=CARTESIAN_POINT('Ctrl Pts',(-49.5977191159129,-3.1744975522657,
-234.63852738515));
#195077=CARTESIAN_POINT('Ctrl Pts',(-49.6065315140282,-3.1178507455648,
-234.639593798937));
#195078=CARTESIAN_POINT('Ctrl Pts',(-49.6149927444874,-3.0611782285275,
-234.64065864047));
#195079=CARTESIAN_POINT('Ctrl Pts',(-49.623103570814,-3.00448076372669,
-234.641721827183));
#195080=CARTESIAN_POINT('Ctrl Pts',(-49.6393252234671,-2.89108583412506,
-234.643848200611));
#195081=CARTESIAN_POINT('Ctrl Pts',(-49.6541442741062,-2.77759734013229,
-234.645968344266));
#195082=CARTESIAN_POINT('Ctrl Pts',(-49.6675699640164,-2.66399952726585,
-234.648080155094));
#195083=CARTESIAN_POINT('Ctrl Pts',(-49.6942342683747,-2.43838678952438,
-234.652274350481));
#195084=CARTESIAN_POINT('Ctrl Pts',(-49.7154039683314,-2.21232427078163,
-234.656434408125));
#195085=CARTESIAN_POINT('Ctrl Pts',(-49.7310906888788,-1.98596836913008,
-234.660568429307));
#195086=CARTESIAN_POINT('Ctrl Pts',(-49.731200746147,-1.98438026713683,
-234.660597433398));
#195087=CARTESIAN_POINT('Ctrl Pts',(-49.7313105335634,-1.98279215070767,
-234.660626436208));
#195088=CARTESIAN_POINT('Ctrl Pts',(-49.7314200511205,-1.98120401989647,
-234.660655437739));
#195089=CARTESIAN_POINT('Ctrl Pts',(-49.7440903886979,-1.79746952081599,
-234.664010691441));
#195090=CARTESIAN_POINT('Ctrl Pts',(-49.753152861207,-1.61344027535473,
-234.667348492208));
#195091=CARTESIAN_POINT('Ctrl Pts',(-49.7585935976184,-1.42950334434026,
-234.670659997496));
#195092=CARTESIAN_POINT('Ctrl Pts',(-49.7640516342342,-1.24498153909823,
-234.673982032556));
#195093=CARTESIAN_POINT('Ctrl Pts',(-49.7658648777063,-1.06055277865886,
-234.677277604645));
#195094=CARTESIAN_POINT('Ctrl Pts',(-49.7640718178133,-0.876606063108709,
-234.680537786596));
#195095=CARTESIAN_POINT('Ctrl Pts',(-49.7632599069805,-0.793313624531679,
-234.68201402119));
#195096=CARTESIAN_POINT('Ctrl Pts',(-49.761709289772,-0.710119984785798,
-234.683482999582));
#195097=CARTESIAN_POINT('Ctrl Pts',(-49.7594270415185,-0.627061021642988,
-234.684943892965));
#195098=CARTESIAN_POINT('Ctrl Pts',(-49.7593072107643,-0.62269996312015,
-234.68502059801));
#195099=CARTESIAN_POINT('Ctrl Pts',(-49.7591853635195,-0.61833927583606,
-234.685097280766));
#195100=CARTESIAN_POINT('Ctrl Pts',(-49.7590615007317,-0.613978964973898,
-234.685173941114));
#195101=CARTESIAN_POINT('Ctrl Pts',(-49.7511603447154,-0.33583653809922,
-234.690064072969));
#195102=CARTESIAN_POINT('Ctrl Pts',(-49.7350315142723,-0.0588012353609941,
-234.694898048003));
#195103=CARTESIAN_POINT('Ctrl Pts',(-49.7107736848362,0.21714818401575,
-234.699679453349));
#195104=CARTESIAN_POINT('Ctrl Pts',(-49.6957904178448,0.387593105213088,
-234.702632770878));
#195105=CARTESIAN_POINT('Ctrl Pts',(-49.677704809517,0.557623896906549,
-234.705566032397));
#195106=CARTESIAN_POINT('Ctrl Pts',(-49.6565302394471,0.727246567549798,
-234.708480083205));
#195107=CARTESIAN_POINT('Ctrl Pts',(-49.6560765351483,0.730881046766953,
-234.708542522129));
#195108=CARTESIAN_POINT('Ctrl Pts',(-49.6556214123894,0.734515338631977,
-234.708604952234));
#195109=CARTESIAN_POINT('Ctrl Pts',(-49.6551648711012,0.738149443195642,
-234.708667373527));
#195110=CARTESIAN_POINT('Ctrl Pts',(-49.6270351753479,0.962064033984754,
-234.712513448409));
#195111=CARTESIAN_POINT('Ctrl Pts',(-49.5935238039947,1.185267081603,-234.716323147795));
#195112=CARTESIAN_POINT('Ctrl Pts',(-49.5546302331264,1.40776084764246,
-234.720064924914));
#195113=CARTESIAN_POINT('Ctrl Pts',(-49.5351834476923,1.51900773066219,
-234.721935813473));
#195114=CARTESIAN_POINT('Ctrl Pts',(-49.5143888724467,1.63007607867294,
-234.723792668997));
#195115=CARTESIAN_POINT('Ctrl Pts',(-49.4922409964726,1.74095941338489,
-234.725638579284));
#195116=CARTESIAN_POINT('Ctrl Pts',(-49.4811670584855,1.79640108074087,
-234.726561534428));
#195117=CARTESIAN_POINT('Ctrl Pts',(-49.4697549987091,1.85179661207854,
-234.727481429318));
#195118=CARTESIAN_POINT('Ctrl Pts',(-49.4580044102124,1.90714539349383,
-234.728398121989));
#195119=CARTESIAN_POINT('Ctrl Pts',(-49.452129115964,1.93481978420148,-234.728856468325));
#195120=CARTESIAN_POINT('Ctrl Pts',(-49.4461691890908,1.96248248734993,
-234.729314013782));
#195121=CARTESIAN_POINT('Ctrl Pts',(-49.4401245757343,1.99013342604581,
-234.729770739067));
#195122=CARTESIAN_POINT('Ctrl Pts',(-49.4352881443074,2.0122575655073,-234.730136175264));
#195123=CARTESIAN_POINT('Ctrl Pts',(-49.4301142570603,2.03519025837516,
-234.730650175937));
#195124=CARTESIAN_POINT('Ctrl Pts',(-49.4254861417503,2.05638458372418,
-234.73084835146));
#195125=CARTESIAN_POINT('Ctrl Pts',(-49.4243299992465,2.06167910616649,
-234.730897857389));
#195126=CARTESIAN_POINT('Ctrl Pts',(-49.4232081718496,2.06686519529321,
-234.730927654475));
#195127=CARTESIAN_POINT('Ctrl Pts',(-49.4221349129046,2.07190323615638,
-234.730930503295));
#195128=CARTESIAN_POINT('Ctrl Pts',(-49.4221408870578,2.07190450442766,
-234.730934934417));
#195129=CARTESIAN_POINT('Ctrl Pts',(-49.4182221517136,2.09035813821035,
-234.730952342309));
#195130=CARTESIAN_POINT('Ctrl Pts',(-49.4148993121985,2.10705514859158,
-234.730657481109));
#195131=CARTESIAN_POINT('Ctrl Pts',(-49.411500307874,2.12415379256605,-234.730429273799));
#195132=CARTESIAN_POINT('Ctrl Pts',(-49.3733025605228,2.31630702928812,
-234.72786469773));
#195133=CARTESIAN_POINT('Ctrl Pts',(-49.3393967227227,2.50891424783426,
-234.724974624097));
#195134=CARTESIAN_POINT('Ctrl Pts',(-49.3097301337179,2.70192914560597,
-234.721749061531));
#195135=CARTESIAN_POINT('Ctrl Pts',(-49.2503969557082,3.08795894114938,
-234.7152979364));
#195136=CARTESIAN_POINT('Ctrl Pts',(-49.207969579461,3.47650574288954,-234.70747771265));
#195137=CARTESIAN_POINT('Ctrl Pts',(-49.1824520139602,3.86385136380115,
-234.698251165921));
#195138=CARTESIAN_POINT('Ctrl Pts',(-49.1314168829586,4.63854260562436,
-234.679798072463));
#195139=CARTESIAN_POINT('Ctrl Pts',(-49.1472577098392,5.40777762062993,
-234.655885603971));
#195140=CARTESIAN_POINT('Ctrl Pts',(-49.2257062624418,6.17073512744913,
-234.625448311592));
#195141=CARTESIAN_POINT('Ctrl Pts',(-49.3041548150444,6.93369263426832,
-234.595011019214));
#195142=CARTESIAN_POINT('Ctrl Pts',(-49.4452772362161,7.69022032934419,
-234.557971217237));
#195143=CARTESIAN_POINT('Ctrl Pts',(-49.6480781836462,8.44024209637807,
-234.512742074857));
#195144=CARTESIAN_POINT('Ctrl Pts',(-48.3395182384274,8.75410525715256,
-235.35005));
#195145=CARTESIAN_POINT('Ctrl Pts',(-48.1420743191374,7.93092102614352,
-235.35005));
#195146=CARTESIAN_POINT('Ctrl Pts',(-48.0110562569534,7.1033413541692,-235.35005));
#195147=CARTESIAN_POINT('Ctrl Pts',(-47.9456204841389,6.27142206048251,
-235.35005));
#195148=CARTESIAN_POINT('Ctrl Pts',(-47.8801847113245,5.43950276679582,
-235.35005));
#195149=CARTESIAN_POINT('Ctrl Pts',(-47.8802911706055,4.60324650205529,
-235.35005));
#195150=CARTESIAN_POINT('Ctrl Pts',(-47.9494611326687,3.76242026158568,
-235.35005));
#195151=CARTESIAN_POINT('Ctrl Pts',(-47.9840461137003,3.34200714135087,
-235.35005));
#195152=CARTESIAN_POINT('Ctrl Pts',(-48.0360840389923,2.92068200696516,
-235.35005));
#195153=CARTESIAN_POINT('Ctrl Pts',(-48.1054567185474,2.50226370649453,
-235.35005));
#195154=CARTESIAN_POINT('Ctrl Pts',(-48.140143058325,2.29305455625922,-235.35005));
#195155=CARTESIAN_POINT('Ctrl Pts',(-48.179184621567,2.08432209117834,-235.35005));
#195156=CARTESIAN_POINT('Ctrl Pts',(-48.222640293554,1.87607275633673,-235.35005));
#195157=CARTESIAN_POINT('Ctrl Pts',(-48.2280722525526,1.85004158948043,
-235.35005));
#195158=CARTESIAN_POINT('Ctrl Pts',(-48.2336222090191,1.82402333761035,
-235.35005));
#195159=CARTESIAN_POINT('Ctrl Pts',(-48.2391090978947,1.79799818290319,
-235.35005));
#195160=CARTESIAN_POINT('Ctrl Pts',(-48.2445959867701,1.77197302819679,
-235.35005));
#195161=CARTESIAN_POINT('Ctrl Pts',(-48.2500003144159,1.74593883705,-235.35005));
#195162=CARTESIAN_POINT('Ctrl Pts',(-48.2553221919377,1.71989562162854,
-235.35005));
#195163=CARTESIAN_POINT('Ctrl Pts',(-48.265965946981,1.66780919078707,-235.35005));
#195164=CARTESIAN_POINT('Ctrl Pts',(-48.2762799057507,1.61568666327577,
-235.35005));
#195165=CARTESIAN_POINT('Ctrl Pts',(-48.2862649052553,1.56352813074,-235.35005));
#195166=CARTESIAN_POINT('Ctrl Pts',(-48.3062349042647,1.45921106566753,
-235.35005));
#195167=CARTESIAN_POINT('Ctrl Pts',(-48.3248891350009,1.35474998793937,
-235.35005));
#195168=CARTESIAN_POINT('Ctrl Pts',(-48.3422334665882,1.25014553997188,
-235.35005));
#195169=CARTESIAN_POINT('Ctrl Pts',(-48.4809881192878,0.41330995622679,
-235.35005));
#195170=CARTESIAN_POINT('Ctrl Pts',(-48.5368013795039,-0.432603676297867,
-235.35005));
#195171=CARTESIAN_POINT('Ctrl Pts',(-48.5074366626247,-1.28784015470909,
-235.35005));
#195172=CARTESIAN_POINT('Ctrl Pts',(-48.492754304185,-1.7154583939147,-235.35005));
#195173=CARTESIAN_POINT('Ctrl Pts',(-48.4566916340691,-2.14207645772467,
-235.35005));
#195174=CARTESIAN_POINT('Ctrl Pts',(-48.3993142685993,-2.56629662313498,
-235.35005));
#195175=CARTESIAN_POINT('Ctrl Pts',(-48.3849699272317,-2.67235166448867,
-235.35005));
#195176=CARTESIAN_POINT('Ctrl Pts',(-48.369288587157,-2.77828474965553,
-235.35005));
#195177=CARTESIAN_POINT('Ctrl Pts',(-48.3522652960998,-2.88409542692066,
-235.35005));
#195178=CARTESIAN_POINT('Ctrl Pts',(-48.3437536505715,-2.93700076555113,
-235.35005));
#195179=CARTESIAN_POINT('Ctrl Pts',(-48.3349064994319,-2.98987550057009,
-235.35005));
#195180=CARTESIAN_POINT('Ctrl Pts',(-48.3257231157807,-3.0427195656859,
-235.35005));
#195181=CARTESIAN_POINT('Ctrl Pts',(-48.3234272698678,-3.05593058196506,
-235.35005));
#195182=CARTESIAN_POINT('Ctrl Pts',(-48.3211104090812,-3.06913968134127,
-235.35005));
#195183=CARTESIAN_POINT('Ctrl Pts',(-48.3187725213423,-3.08234686271546,
-235.35005));
#195184=CARTESIAN_POINT('Ctrl Pts',(-48.3164346336033,-3.09555404408982,
-235.35005));
#195185=CARTESIAN_POINT('Ctrl Pts',(-48.3140690695364,-3.1087587009315,
-235.35005));
#195186=CARTESIAN_POINT('Ctrl Pts',(-48.31169696982,-3.12196276161221,-235.35005));
#195187=CARTESIAN_POINT('Ctrl Pts',(-48.306952770387,-3.14837088297426,
-235.35005));
#195188=CARTESIAN_POINT('Ctrl Pts',(-48.3022780138533,-3.17478533866958,
-235.35005));
#195189=CARTESIAN_POINT('Ctrl Pts',(-48.2976726119403,-3.20120612064097,
-235.35005));
#195190=CARTESIAN_POINT('Ctrl Pts',(-48.2608293966366,-3.41257237640728,
-235.35005));
#195191=CARTESIAN_POINT('Ctrl Pts',(-48.2284220495736,-3.62434325601736,
-235.35005));
#195192=CARTESIAN_POINT('Ctrl Pts',(-48.2004248943047,-3.83651641735441,
-235.35005));
#195193=CARTESIAN_POINT('Ctrl Pts',(-48.144430583767,-4.2608627400285,-235.35005));
#195194=CARTESIAN_POINT('Ctrl Pts',(-48.1060703916864,-4.6868175831452,
-235.35005));
#195195=CARTESIAN_POINT('Ctrl Pts',(-48.0854449269901,-5.11439012388267,
-235.35005));
#195196=CARTESIAN_POINT('Ctrl Pts',(-48.0648194622937,-5.54196266462014,
-235.35005));
#195197=CARTESIAN_POINT('Ctrl Pts',(-48.0619566741596,-5.97223878738515,
-235.35005));
#195198=CARTESIAN_POINT('Ctrl Pts',(-48.0771357161752,-6.40148796840999,
-235.35005));
#195199=CARTESIAN_POINT('Ctrl Pts',(-48.1074938002064,-7.25998633045966,
-235.35005));
#195200=CARTESIAN_POINT('Ctrl Pts',(-48.2090347930406,-8.11012177188801,
-235.35005));
#195201=CARTESIAN_POINT('Ctrl Pts',(-48.3817353557071,-8.95189703464271,
-235.35005));
#195202=CARTESIAN_POINT('Ctrl Pts',(-48.3844338019987,-8.96504977312313,
-235.35005));
#195203=CARTESIAN_POINT('Ctrl Pts',(-48.3871335038458,-8.97820236409949,
-235.35005));
#195204=CARTESIAN_POINT('Ctrl Pts',(-48.3898027548802,-8.99135853258005,
-235.35005));
#195205=CARTESIAN_POINT('Ctrl Pts',(-48.3924720059147,-9.00451470106053,
-235.35005));
#195206=CARTESIAN_POINT('Ctrl Pts',(-48.3951203394452,-9.01767332703754,
-235.35005));
#195207=CARTESIAN_POINT('Ctrl Pts',(-48.3977477753549,-9.03083440817268,
-235.35005));
#195208=CARTESIAN_POINT('Ctrl Pts',(-48.4030026471742,-9.05715657044287,
-235.35005));
#195209=CARTESIAN_POINT('Ctrl Pts',(-48.4081739297218,-9.08348855318059,
-235.35005));
#195210=CARTESIAN_POINT('Ctrl Pts',(-48.4132617664092,-9.10983033956203,
-235.35005));
#195211=CARTESIAN_POINT('Ctrl Pts',(-48.4234374397839,-9.16251391232474,
-235.35005));
#195212=CARTESIAN_POINT('Ctrl Pts',(-48.4332793498323,-9.21523669724522,
-235.35005));
#195213=CARTESIAN_POINT('Ctrl Pts',(-48.4427883984152,-9.26799858838481,
-235.35005));
#195214=CARTESIAN_POINT('Ctrl Pts',(-48.4618064955809,-9.37352237066414,
-235.35005));
#195215=CARTESIAN_POINT('Ctrl Pts',(-48.4794934628395,-9.47920254067582,
-235.35005));
#195216=CARTESIAN_POINT('Ctrl Pts',(-48.4958526690327,-9.58503870263172,
-235.35005));
#195217=CARTESIAN_POINT('Ctrl Pts',(-48.5285710814205,-9.79671102655205,
-235.35005));
#195218=CARTESIAN_POINT('Ctrl Pts',(-48.5559827004663,-10.0090068188147,
-235.35005));
#195219=CARTESIAN_POINT('Ctrl Pts',(-48.5780974937539,-10.2219249084145,
-235.35005));
#195220=CARTESIAN_POINT('Ctrl Pts',(-48.6223270803283,-10.6477610876057,
-235.35005));
#195221=CARTESIAN_POINT('Ctrl Pts',(-48.6453046119738,-11.0773736644268,
-235.35005));
#195222=CARTESIAN_POINT('Ctrl Pts',(-48.6469140232755,-11.5038145314612,
-235.35005));
#195223=CARTESIAN_POINT('Ctrl Pts',(-48.6501328458788,-12.3566962655301,
-235.35005));
#195224=CARTESIAN_POINT('Ctrl Pts',(-48.5694097707119,-13.201098145554,
-235.35005));
#195225=CARTESIAN_POINT('Ctrl Pts',(-48.4050646665376,-14.0370524847357,
-235.35005));
#195226=CARTESIAN_POINT('Ctrl Pts',(-48.3999288820313,-14.0631760578391,
-235.35005));
#195227=CARTESIAN_POINT('Ctrl Pts',(-48.3947106332613,-14.0892913003493,
-235.35005));
#195228=CARTESIAN_POINT('Ctrl Pts',(-48.3894097433237,-14.1153981944164,
-235.35005));
#195229=CARTESIAN_POINT('Ctrl Pts',(-48.386759298355,-14.1284516414493,
-235.35005));
#195230=CARTESIAN_POINT('Ctrl Pts',(-48.3840780942122,-14.1415019811713,
-235.35005));
#195231=CARTESIAN_POINT('Ctrl Pts',(-48.3814002229133,-14.1545526575822,
-235.35005));
#195232=CARTESIAN_POINT('Ctrl Pts',(-48.3787223516144,-14.1676033339926,
-235.35005));
#195233=CARTESIAN_POINT('Ctrl Pts',(-48.3760618299286,-14.1806557630669,
-235.35005));
#195234=CARTESIAN_POINT('Ctrl Pts',(-48.3734186404716,-14.1937099430552,
-235.35005));
#195235=CARTESIAN_POINT('Ctrl Pts',(-48.3628458826442,-14.2459266630052,
-235.35005));
#195236=CARTESIAN_POINT('Ctrl Pts',(-48.3525504293979,-14.2981713964018,
-235.35005));
#195237=CARTESIAN_POINT('Ctrl Pts',(-48.3425312602132,-14.350444040166,
-235.35005));
#195238=CARTESIAN_POINT('Ctrl Pts',(-48.3224929218452,-14.4549893276876,
-235.35005));
#195239=CARTESIAN_POINT('Ctrl Pts',(-48.3035595794002,-14.5596462424789,
-235.35005));
#195240=CARTESIAN_POINT('Ctrl Pts',(-48.2857247802083,-14.6644141326663,
-235.35005));
#195241=CARTESIAN_POINT('Ctrl Pts',(-48.2500551818223,-14.8739499130538,
-235.35005));
#195242=CARTESIAN_POINT('Ctrl Pts',(-48.2187775910825,-15.0839293763357,
-235.35005));
#195243=CARTESIAN_POINT('Ctrl Pts',(-48.1918669286016,-15.2943499889772,
-235.35005));
#195244=CARTESIAN_POINT('Ctrl Pts',(-48.13804560364,-15.71519121426,-235.35005));
#195245=CARTESIAN_POINT('Ctrl Pts',(-48.1017687499494,-16.1377801895464,
-235.35005));
#195246=CARTESIAN_POINT('Ctrl Pts',(-48.0829143862637,-16.5595284917746,
-235.35005));
#195247=CARTESIAN_POINT('Ctrl Pts',(-48.0452056588921,-17.4030250962311,
-235.35005));
#195248=CARTESIAN_POINT('Ctrl Pts',(-48.0765553835769,-18.2457723122303,
-235.35005));
#195249=CARTESIAN_POINT('Ctrl Pts',(-48.1770201828715,-19.0877695253175,
-235.35005));
#195250=CARTESIAN_POINT('Ctrl Pts',(-48.2021363826951,-19.2982688285893,
-235.35005));
#195251=CARTESIAN_POINT('Ctrl Pts',(-48.2315724527786,-19.5085474359751,
-235.35005));
#195252=CARTESIAN_POINT('Ctrl Pts',(-48.2653424827524,-19.7185300485352,
-235.35005));
#195253=CARTESIAN_POINT('Ctrl Pts',(-48.2737849902462,-19.7710257016774,
-235.35005));
#195254=CARTESIAN_POINT('Ctrl Pts',(-48.282498702759,-19.8235043364666,
-235.35005));
#195255=CARTESIAN_POINT('Ctrl Pts',(-48.2914842922534,-19.8759659107496,
-235.35005));
#195256=CARTESIAN_POINT('Ctrl Pts',(-48.2959770870004,-19.9021966978899,
-235.35005));
#195257=CARTESIAN_POINT('Ctrl Pts',(-48.300537852968,-19.9284232197822,
-235.35005));
#195258=CARTESIAN_POINT('Ctrl Pts',(-48.3051666862202,-19.9546454703855,
-235.35005));
#195259=CARTESIAN_POINT('Ctrl Pts',(-48.3074811028462,-19.967756595687,
-235.35005));
#195260=CARTESIAN_POINT('Ctrl Pts',(-48.3098125364066,-19.9808666531674,
-235.35005));
#195261=CARTESIAN_POINT('Ctrl Pts',(-48.3121609996811,-19.9939756420136,
-235.35005));
#195262=CARTESIAN_POINT('Ctrl Pts',(-48.3145094629556,-20.0070846308597,
-235.35005));
#195263=CARTESIAN_POINT('Ctrl Pts',(-48.3168699428148,-20.0201928656576,
-235.35005));
#195264=CARTESIAN_POINT('Ctrl Pts',(-48.3191971709643,-20.0333031870275,
-235.35005));
#195265=CARTESIAN_POINT('Ctrl Pts',(-48.337814996161,-20.1381857579874,
-235.35005));
#195266=CARTESIAN_POINT('Ctrl Pts',(-48.3550896009549,-20.2431526171762,
-235.35005));
#195267=CARTESIAN_POINT('Ctrl Pts',(-48.3710295920234,-20.3482032245128,
-235.35005));
#195268=CARTESIAN_POINT('Ctrl Pts',(-48.4347895562984,-20.7684056538652,
-235.35005));
#195269=CARTESIAN_POINT('Ctrl Pts',(-48.4772403630263,-21.1899452510779,
-235.35005));
#195270=CARTESIAN_POINT('Ctrl Pts',(-48.4986731253089,-21.612803748536,
-235.35005));
#195271=CARTESIAN_POINT('Ctrl Pts',(-48.541538649874,-22.458520743452,-235.35005));
#195272=CARTESIAN_POINT('Ctrl Pts',(-48.5005032095075,-23.3116677382499,
-235.35005));
#195273=CARTESIAN_POINT('Ctrl Pts',(-48.3713478679476,-24.1646010300614,
-235.35005));
#195274=CARTESIAN_POINT('Ctrl Pts',(-48.3390590325577,-24.3778343530143,
-235.35005));
#195275=CARTESIAN_POINT('Ctrl Pts',(-48.3012455308435,-24.5909867391319,
-235.35005));
#195276=CARTESIAN_POINT('Ctrl Pts',(-48.2577770486563,-24.8040562792487,
-235.35005));
#195277=CARTESIAN_POINT('Ctrl Pts',(-48.2523434883829,-24.8306899717632,
-235.35005));
#195278=CARTESIAN_POINT('Ctrl Pts',(-48.2468215386317,-24.8573223693642,
-235.35005));
#195279=CARTESIAN_POINT('Ctrl Pts',(-48.2412109184648,-24.8839534679411,
-235.35005));
#195280=CARTESIAN_POINT('Ctrl Pts',(-48.235600298298,-24.9105845665175,
-235.35005));
#195281=CARTESIAN_POINT('Ctrl Pts',(-48.2299135976341,-24.9372145504959,
-235.35005));
#195282=CARTESIAN_POINT('Ctrl Pts',(-48.2243539041553,-24.9638463951525,
-235.35005));
#195283=CARTESIAN_POINT('Ctrl Pts',(-48.2132345171977,-25.0171100844654,
-235.35005));
#195284=CARTESIAN_POINT('Ctrl Pts',(-48.2024091551918,-25.0703780812439,
-235.35005));
#195285=CARTESIAN_POINT('Ctrl Pts',(-48.1918756280125,-25.1236503534574,
-235.35005));
#195286=CARTESIAN_POINT('Ctrl Pts',(-48.1708085736529,-25.2301948978888,
-235.35005));
#195287=CARTESIAN_POINT('Ctrl Pts',(-48.1509087142019,-25.3367565417865,
-235.35005));
#195288=CARTESIAN_POINT('Ctrl Pts',(-48.1321603275509,-25.4433350548857,
-235.35005));
#195289=CARTESIAN_POINT('Ctrl Pts',(-48.0571667809486,-25.8696491072753,
-235.35005));
#195290=CARTESIAN_POINT('Ctrl Pts',(-48.000556289184,-26.2962324731006,
-235.35005));
#195291=CARTESIAN_POINT('Ctrl Pts',(-47.9616645382749,-26.7230754200676,
-235.35005));
#195292=CARTESIAN_POINT('Ctrl Pts',(-47.8838810364566,-27.5767613140017,
-235.35005));
#195293=CARTESIAN_POINT('Ctrl Pts',(-47.87663302545,-28.4314805592623,-235.35005));
#195294=CARTESIAN_POINT('Ctrl Pts',(-47.9382574172368,-29.287208791445,
-235.35005));
#195295=CARTESIAN_POINT('Ctrl Pts',(-47.9998818090236,-30.1429370236277,
-235.35005));
#195296=CARTESIAN_POINT('Ctrl Pts',(-48.1303735979639,-30.9996741692801,
-235.35005));
#195297=CARTESIAN_POINT('Ctrl Pts',(-48.3327003568643,-31.8574637039839,
-235.35005));
#195298=CARTESIAN_POINT('Ctrl Pts',(-48.3307545488269,-31.8493376071772,
-235.35004999994));
#195299=CARTESIAN_POINT('Ctrl Pts',(-49.2665966890958,-31.6249695531388,
-235.350058621518));
#195300=CARTESIAN_POINT('Ctrl Pts',(-49.6566766583008,-31.531451804001,
-234.47528355851));
#195301=CARTESIAN_POINT('Ctrl Pts',(-48.372551678047,-32.0237574776621,
-235.350049999945));
#195302=CARTESIAN_POINT('Ctrl Pts',(-49.2656683159424,-31.8826538814243,
-235.350057688891));
#195303=CARTESIAN_POINT('Ctrl Pts',(-49.6877952499862,-31.818666798948,
-234.555234217691));
#195304=CARTESIAN_POINT('Ctrl Pts',(-48.393897970712,-32.2007826737009,
-235.35004999995));
#195305=CARTESIAN_POINT('Ctrl Pts',(-49.2406129702643,-32.143223893466,
-235.350056855992));
#195306=CARTESIAN_POINT('Ctrl Pts',(-49.6816879330612,-32.1154681493768,
-234.629557346798));
#195307=CARTESIAN_POINT('Ctrl Pts',(-48.3876860767769,-32.3803569706164,
-235.350049999955));
#195308=CARTESIAN_POINT('Ctrl Pts',(-49.1793203036772,-32.4078529308044,
-235.350056136573));
#195309=CARTESIAN_POINT('Ctrl Pts',(-49.6257204831723,-32.4233553155217,
-234.695894022066));
#195310=CARTESIAN_POINT('',(-49.628292312036,-32.4090169804993,-234.692797218033));
#195311=CARTESIAN_POINT('',(-48.3879672519817,-32.371991693197,-235.35005));
#195312=CARTESIAN_POINT('Origin',(-48.3879672519817,-32.371991693197,-233.85005));
#195313=CARTESIAN_POINT('Ctrl Pts',(-49.628292311974,-32.4090169808449,
-234.692797218109));
#195314=CARTESIAN_POINT('Ctrl Pts',(-49.6810233914157,-32.1110273722408,
-234.628281397553));
#195315=CARTESIAN_POINT('Ctrl Pts',(-49.687128176312,-31.8234236701372,
-234.556301998219));
#195316=CARTESIAN_POINT('Ctrl Pts',(-49.6580996754574,-31.544841856517,
-234.479004868619));
#195317=CARTESIAN_POINT('Ctrl Pts',(-48.3327003568643,-31.8574637039841,
-235.35005));
#195318=CARTESIAN_POINT('Ctrl Pts',(-48.3726098627487,-32.0266650324685,
-235.35005));
#195319=CARTESIAN_POINT('Ctrl Pts',(-48.3931627529261,-32.1979455093617,
-235.35005));
#195320=CARTESIAN_POINT('Ctrl Pts',(-48.3879672519817,-32.371991693197,
-235.35005));
#195321=CARTESIAN_POINT('Ctrl Pts',(-48.3879672519816,-32.371991693197,
-235.35005));
#195322=CARTESIAN_POINT('Ctrl Pts',(-49.1821150693849,-32.3956980201291,
-235.35005));
#195323=CARTESIAN_POINT('Ctrl Pts',(-49.6282923119739,-32.4090169808449,
-234.692797218109));
#195324=CARTESIAN_POINT('Ctrl Pts',(-48.3122036088614,-34.9100285686315,
-235.35005));
#195325=CARTESIAN_POINT('Ctrl Pts',(-49.1048103477618,-34.9355482471023,
-235.350050000493));
#195326=CARTESIAN_POINT('Ctrl Pts',(-49.5510892026461,-34.9515478422503,
-234.694718333571));
#195327=CARTESIAN_POINT('Ctrl Pts',(-48.2225732111533,-37.4475766604583,
-235.35005));
#195328=CARTESIAN_POINT('Ctrl Pts',(-49.0133760622712,-37.4755964900674,
-235.350049998731));
#195329=CARTESIAN_POINT('Ctrl Pts',(-49.4597789489883,-37.4935285423766,
-234.696950276065));
#195330=CARTESIAN_POINT('Ctrl Pts',(-48.1190600870606,-39.984633316822,
-235.35005));
#195331=CARTESIAN_POINT('Ctrl Pts',(-48.9077504789076,-40.0168122617172,
-235.35005));
#195332=CARTESIAN_POINT('Ctrl Pts',(-49.3543621196711,-40.035034230092,
-234.699454871761));
#195333=CARTESIAN_POINT('',(-49.354362119671,-40.035034230092,-234.699454871761));
#195334=CARTESIAN_POINT('',(-48.1190600870606,-39.9846333168228,-235.35005));
#195335=CARTESIAN_POINT('Origin',(-48.1190600870606,-39.9846333168229,-233.85005));
#195336=CARTESIAN_POINT('Origin',(637.300587775051,-11.5397323655281,-248.898224599212));
#195337=CARTESIAN_POINT('Origin',(647.878174797988,-11.588320224684,-235.350049996435));
#195338=CARTESIAN_POINT('Ctrl Pts',(-48.1190600870606,-39.9846333168228,
-235.35005));
#195339=CARTESIAN_POINT('Ctrl Pts',(-48.9077504789077,-40.0168122617177,
-235.35005));
#195340=CARTESIAN_POINT('Ctrl Pts',(-49.3543621196712,-40.0350342300922,
-234.69945487176));
#195341=CARTESIAN_POINT('Ctrl Pts',(-48.1156571344711,-40.0680385041539,
-235.35005));
#195342=CARTESIAN_POINT('Ctrl Pts',(-48.8941878304705,-40.1139469219292,
-235.350049999983));
#195343=CARTESIAN_POINT('Ctrl Pts',(-49.3415926503895,-40.1404174549493,
-234.711772602598));
#195344=CARTESIAN_POINT('Ctrl Pts',(-48.1094046180063,-40.1511102451508,
-235.35005));
#195345=CARTESIAN_POINT('Ctrl Pts',(-48.8709781715377,-40.2220121424719,
-235.35004999999));
#195346=CARTESIAN_POINT('Ctrl Pts',(-49.3183790954466,-40.2639303612825,
-234.731242016098));
#195347=CARTESIAN_POINT('Ctrl Pts',(-48.0952241561347,-40.2752167333539,
-235.35005));
#195348=CARTESIAN_POINT('Ctrl Pts',(-48.8404013751985,-40.3682352258384,
-235.350050000006));
#195349=CARTESIAN_POINT('Ctrl Pts',(-49.2869295306867,-40.4240408437502,
-234.748883360049));
#195350=CARTESIAN_POINT('Ctrl Pts',(-48.0899153448806,-40.3165225558374,
-235.35005));
#195351=CARTESIAN_POINT('Ctrl Pts',(-48.830421545654,-40.4157032323804,
-235.35005));
#195352=CARTESIAN_POINT('Ctrl Pts',(-49.2765808080252,-40.4755275655264,
-234.753809123677));
#195353=CARTESIAN_POINT('Ctrl Pts',(-48.0779218876032,-40.3989852515461,
-235.35005));
#195354=CARTESIAN_POINT('Ctrl Pts',(-48.8066893271687,-40.513370761674,
-235.350049999999));
#195355=CARTESIAN_POINT('Ctrl Pts',(-49.251626649492,-40.5832746725427,
-234.765851629537));
#195356=CARTESIAN_POINT('Ctrl Pts',(-48.0712183175412,-40.4401628322643,
-235.350050000001));
#195357=CARTESIAN_POINT('Ctrl Pts',(-48.7934838819703,-40.5628189902028,
-235.350050000007));
#195358=CARTESIAN_POINT('Ctrl Pts',(-49.2375840222482,-40.6383093361276,
-234.772359011183));
#195359=CARTESIAN_POINT('Ctrl Pts',(-48.0561422093234,-40.5222290742639,
-235.350050000001));
#195360=CARTESIAN_POINT('Ctrl Pts',(-48.764457764962,-40.6622349257811,
-235.350049999994));
#195361=CARTESIAN_POINT('Ctrl Pts',(-49.2063354527156,-40.7496495874624,
-234.785817239668));
#195362=CARTESIAN_POINT('Ctrl Pts',(-48.047773596518,-40.5630852304628,
-235.35005));
#195363=CARTESIAN_POINT('Ctrl Pts',(-48.7495575164579,-40.7110546556452,
-235.350050000008));
#195364=CARTESIAN_POINT('Ctrl Pts',(-49.1901931274652,-40.8040214971111,
-234.791881131089));
#195365=CARTESIAN_POINT('Ctrl Pts',(-48.0296425423562,-40.6445005636306,
-235.35005));
#195366=CARTESIAN_POINT('Ctrl Pts',(-48.7198529923868,-40.8064170701649,
-235.35004999999));
#195367=CARTESIAN_POINT('Ctrl Pts',(-49.1580329424021,-40.9092699497394,
-234.80233714665));
#195368=CARTESIAN_POINT('Ctrl Pts',(-48.0199029877981,-40.6850741153181,
-235.35005));
#195369=CARTESIAN_POINT('Ctrl Pts',(-48.7056393397796,-40.8523724308093,
-235.350049999989));
#195370=CARTESIAN_POINT('Ctrl Pts',(-49.1427597364121,-40.9590683152935,
-234.806236550506));
#195371=CARTESIAN_POINT('Ctrl Pts',(-47.9992940161415,-40.7659290146224,
-235.35005));
#195372=CARTESIAN_POINT('Ctrl Pts',(-48.6746942895135,-40.9454780254451,
-235.35005000001));
#195373=CARTESIAN_POINT('Ctrl Pts',(-49.1091912161129,-41.0610374960301,
-234.815043280514));
#195374=CARTESIAN_POINT('Ctrl Pts',(-47.9883597239418,-40.8062069855079,
-235.35005));
#195375=CARTESIAN_POINT('Ctrl Pts',(-48.6576049577959,-40.9929195436597,
-235.350049999994));
#195376=CARTESIAN_POINT('Ctrl Pts',(-49.0904332941573,-41.1137361405253,
-234.82018153471));
#195377=CARTESIAN_POINT('Ctrl Pts',(-47.9648484820867,-40.886240947879,
-235.35005));
#195378=CARTESIAN_POINT('Ctrl Pts',(-48.6202908038635,-41.0885568169624,
-235.350050000006));
#195379=CARTESIAN_POINT('Ctrl Pts',(-49.0490372574119,-41.2209607216622,
-234.831270117331));
#195380=CARTESIAN_POINT('Ctrl Pts',(-47.9522083925962,-40.9259746645696,
-235.35005));
#195381=CARTESIAN_POINT('Ctrl Pts',(-48.6000967774269,-41.136585315531,
-235.350050000005));
#195382=CARTESIAN_POINT('Ctrl Pts',(-49.0264208357049,-41.2752201799367,
-234.837105794306));
#195383=CARTESIAN_POINT('Ctrl Pts',(-47.9122208177014,-41.0445137282603,
-235.35005));
#195384=CARTESIAN_POINT('Ctrl Pts',(-48.5437175410231,-41.2731792254645,
-235.350049999989));
#195385=CARTESIAN_POINT('Ctrl Pts',(-48.964349840243,-41.4256874560579,
-234.84928310824));
#195386=CARTESIAN_POINT('Ctrl Pts',(-47.8834173029482,-41.1228515949417,
-235.35005));
#195387=CARTESIAN_POINT('Ctrl Pts',(-48.5108776537541,-41.3567902125311,
-235.350049999988));
#195388=CARTESIAN_POINT('Ctrl Pts',(-48.9298467764963,-41.513182231287,
-234.851751686106));
#195389=CARTESIAN_POINT('Ctrl Pts',(-47.8371337927352,-41.2386632571498,
-235.35005));
#195390=CARTESIAN_POINT('Ctrl Pts',(-48.4472327735751,-41.4907743916649,
-235.350050000005));
#195391=CARTESIAN_POINT('Ctrl Pts',(-48.8593613765109,-41.6611254214954,
-234.863347210043));
#195392=CARTESIAN_POINT('Ctrl Pts',(-47.8210253111431,-41.2769359664061,
-235.35005));
#195393=CARTESIAN_POINT('Ctrl Pts',(-48.4238255405523,-41.5362680262328,
-235.35005));
#195394=CARTESIAN_POINT('Ctrl Pts',(-48.832972869674,-41.7123406931751,
-234.868203498974));
#195395=CARTESIAN_POINT('Ctrl Pts',(-47.787220073548,-41.3527085858238,
-235.35005));
#195396=CARTESIAN_POINT('Ctrl Pts',(-48.3763605083435,-41.6250538530374,
-235.35005));
#195397=CARTESIAN_POINT('Ctrl Pts',(-48.7797020312914,-41.8115618811122,
-234.877028502702));
#195398=CARTESIAN_POINT('Ctrl Pts',(-47.7696001307559,-41.3902458706063,
-235.35005));
#195399=CARTESIAN_POINT('Ctrl Pts',(-48.3541637623008,-41.6669126397123,
-235.350050000011));
#195400=CARTESIAN_POINT('Ctrl Pts',(-48.7554615646751,-41.8568726544237,
-234.879814510279));
#195401=CARTESIAN_POINT('Ctrl Pts',(-47.7335555457799,-41.4649289014138,
-235.35005));
#195402=CARTESIAN_POINT('Ctrl Pts',(-48.3105107159968,-41.7488046878741,
-235.350049999989));
#195403=CARTESIAN_POINT('Ctrl Pts',(-48.7083373512675,-41.9445758791192,
-234.884369803896));
#195404=CARTESIAN_POINT('Ctrl Pts',(-47.7151163766151,-41.5020675791261,
-235.35005));
#195405=CARTESIAN_POINT('Ctrl Pts',(-48.2891485822549,-41.7887312087111,
-235.35005));
#195406=CARTESIAN_POINT('Ctrl Pts',(-48.6856039311336,-41.9867349750483,
-234.886044416602));
#195407=CARTESIAN_POINT('Ctrl Pts',(-47.6870475431915,-41.5575760651628,
-235.35005));
#195408=CARTESIAN_POINT('Ctrl Pts',(-48.2574046215262,-41.847779872134,
-235.35005));
#195409=CARTESIAN_POINT('Ctrl Pts',(-48.6521086576215,-42.0486144262277,
-234.888099431162));
#195410=CARTESIAN_POINT('Ctrl Pts',(-47.677640411345,-41.5760541500354,
-235.35005));
#195411=CARTESIAN_POINT('Ctrl Pts',(-48.2470403251889,-41.8672107704492,
-235.35005));
#195412=CARTESIAN_POINT('Ctrl Pts',(-48.6412778638178,-42.0688098769786,
-234.888619834342));
#195413=CARTESIAN_POINT('Ctrl Pts',(-47.6585760783126,-41.6128886447362,
-235.35005));
#195414=CARTESIAN_POINT('Ctrl Pts',(-48.2228963762585,-41.9084918903695,
-235.35005));
#195415=CARTESIAN_POINT('Ctrl Pts',(-48.6147495311229,-42.113763065292,
-234.891630453002));
#195416=CARTESIAN_POINT('Ctrl Pts',(-47.6488991764614,-41.6312354689061,
-235.35005));
#195417=CARTESIAN_POINT('Ctrl Pts',(-48.2093956206664,-41.9300731458053,
-235.350050000003));
#195418=CARTESIAN_POINT('Ctrl Pts',(-48.5994498402746,-42.1380513796496,
-234.893925232714));
#195419=CARTESIAN_POINT('Ctrl Pts',(-47.6191741486339,-41.6859381083017,
-235.35005));
#195420=CARTESIAN_POINT('Ctrl Pts',(-48.1671827615658,-41.9951014194116,
-235.350049999995));
#195421=CARTESIAN_POINT('Ctrl Pts',(-48.5512188371181,-42.211817336402,
-234.901278569161));
#195422=CARTESIAN_POINT('Ctrl Pts',(-47.5984065010933,-41.7219438293822,
-235.35005));
#195423=CARTESIAN_POINT('Ctrl Pts',(-48.1381497307774,-42.0377252505059,
-235.350050000006));
#195424=CARTESIAN_POINT('Ctrl Pts',(-48.5180631792116,-42.2600391416596,
-234.905912731492));
#195425=CARTESIAN_POINT('Ctrl Pts',(-47.5555678143129,-41.7933210863947,
-235.35005));
#195426=CARTESIAN_POINT('Ctrl Pts',(-48.0836613352502,-42.1183565908771,
-235.350049999994));
#195427=CARTESIAN_POINT('Ctrl Pts',(-48.457597592579,-42.3485528957682,
-234.91222746163));
#195428=CARTESIAN_POINT('Ctrl Pts',(-47.5335333913842,-41.8287112184799,
-235.35005));
#195429=CARTESIAN_POINT('Ctrl Pts',(-48.0574563285157,-42.1570164665365,
-235.350049999952));
#195430=CARTESIAN_POINT('Ctrl Pts',(-48.4291976744607,-42.3899883957637,
-234.914384660568));
#195431=CARTESIAN_POINT('Ctrl Pts',(-47.511140470057,-41.8639253579254,
-235.35005));
#195432=CARTESIAN_POINT('Ctrl Pts',(-48.0316514259825,-42.1949218242413,
-235.35005));
#195433=CARTESIAN_POINT('Ctrl Pts',(-48.4015825627194,-42.4301635567087,
-234.916111528175));
#195434=CARTESIAN_POINT('',(-48.4015825627194,-42.4301635567086,-234.916111528175));
#195435=CARTESIAN_POINT('',(-47.511140470057,-41.8639253579254,-235.35005));
#195436=CARTESIAN_POINT('Origin',(-47.5111404700569,-41.8639253579254,-233.85005));
#195437=CARTESIAN_POINT('Ctrl Pts',(-48.4015825627194,-42.4301635567086,
-234.916111528175));
#195438=CARTESIAN_POINT('Ctrl Pts',(-48.4291976744607,-42.3899883957637,
-234.914384660568));
#195439=CARTESIAN_POINT('Ctrl Pts',(-48.457597592579,-42.3485528957682,
-234.91222746163));
#195440=CARTESIAN_POINT('Ctrl Pts',(-48.5180631792116,-42.2600391416596,
-234.905912731492));
#195441=CARTESIAN_POINT('Ctrl Pts',(-48.5512188371181,-42.211817336402,
-234.901278569161));
#195442=CARTESIAN_POINT('Ctrl Pts',(-48.5994498402746,-42.1380513796496,
-234.893925232714));
#195443=CARTESIAN_POINT('Ctrl Pts',(-48.6147495311229,-42.113763065292,
-234.891630453002));
#195444=CARTESIAN_POINT('Ctrl Pts',(-48.6412778638178,-42.0688098769786,
-234.888619834342));
#195445=CARTESIAN_POINT('Ctrl Pts',(-48.6521086576215,-42.0486144262277,
-234.888099431162));
#195446=CARTESIAN_POINT('Ctrl Pts',(-48.6856039311336,-41.9867349750483,
-234.886044416602));
#195447=CARTESIAN_POINT('Ctrl Pts',(-48.7083373512675,-41.9445758791192,
-234.884369803896));
#195448=CARTESIAN_POINT('Ctrl Pts',(-48.7554615646751,-41.8568726544237,
-234.879814510279));
#195449=CARTESIAN_POINT('Ctrl Pts',(-48.7797020312914,-41.8115618811122,
-234.877028502702));
#195450=CARTESIAN_POINT('Ctrl Pts',(-48.832972869674,-41.7123406931751,
-234.868203498974));
#195451=CARTESIAN_POINT('Ctrl Pts',(-48.8593613765109,-41.6611254214954,
-234.863347210043));
#195452=CARTESIAN_POINT('Ctrl Pts',(-48.9298467764963,-41.513182231287,
-234.851751686106));
#195453=CARTESIAN_POINT('Ctrl Pts',(-48.964349840243,-41.4256874560579,
-234.84928310824));
#195454=CARTESIAN_POINT('Ctrl Pts',(-49.0264208357049,-41.2752201799367,
-234.837105794306));
#195455=CARTESIAN_POINT('Ctrl Pts',(-49.0490372574119,-41.2209607216622,
-234.831270117331));
#195456=CARTESIAN_POINT('Ctrl Pts',(-49.0904332941573,-41.1137361405253,
-234.82018153471));
#195457=CARTESIAN_POINT('Ctrl Pts',(-49.1091912161129,-41.0610374960301,
-234.815043280514));
#195458=CARTESIAN_POINT('Ctrl Pts',(-49.1427597364121,-40.9590683152935,
-234.806236550506));
#195459=CARTESIAN_POINT('Ctrl Pts',(-49.1580329424021,-40.9092699497394,
-234.80233714665));
#195460=CARTESIAN_POINT('Ctrl Pts',(-49.1901931274652,-40.8040214971111,
-234.791881131089));
#195461=CARTESIAN_POINT('Ctrl Pts',(-49.2063354527156,-40.7496495874624,
-234.785817239668));
#195462=CARTESIAN_POINT('Ctrl Pts',(-49.2375840222482,-40.6383093361276,
-234.772359011183));
#195463=CARTESIAN_POINT('Ctrl Pts',(-49.251626649492,-40.5832746725427,
-234.765851629537));
#195464=CARTESIAN_POINT('Ctrl Pts',(-49.2765808080252,-40.4755275655264,
-234.753809123677));
#195465=CARTESIAN_POINT('Ctrl Pts',(-49.2869295306867,-40.4240408437502,
-234.748883360049));
#195466=CARTESIAN_POINT('Ctrl Pts',(-49.3183790954466,-40.2639303612825,
-234.731242016098));
#195467=CARTESIAN_POINT('Ctrl Pts',(-49.3415926503895,-40.1404174549493,
-234.711772602598));
#195468=CARTESIAN_POINT('Ctrl Pts',(-49.354362119671,-40.035034230092,-234.699454871761));
#195469=CARTESIAN_POINT('Ctrl Pts',(-48.1190600870606,-39.9846333168228,
-235.35005));
#195470=CARTESIAN_POINT('Ctrl Pts',(-48.1156573562241,-40.0680330690653,
-235.35005));
#195471=CARTESIAN_POINT('Ctrl Pts',(-48.1094051493674,-40.1511056240727,
-235.35005));
#195472=CARTESIAN_POINT('Ctrl Pts',(-48.0999509844461,-40.2338479048312,
-235.35005));
#195473=CARTESIAN_POINT('Ctrl Pts',(-48.0952242649892,-40.2752158682241,
-235.35005));
#195474=CARTESIAN_POINT('Ctrl Pts',(-48.089915468827,-40.3165217899444,
-235.35005));
#195475=CARTESIAN_POINT('Ctrl Pts',(-48.0839186309937,-40.3577539058372,
-235.35005));
#195476=CARTESIAN_POINT('Ctrl Pts',(-48.0779219885029,-40.398984678624,
-235.35005));
#195477=CARTESIAN_POINT('Ctrl Pts',(-48.0712184248364,-40.4401623582127,
-235.350050000001));
#195478=CARTESIAN_POINT('Ctrl Pts',(-48.0636802851834,-40.4811959572599,
-235.350050000001));
#195479=CARTESIAN_POINT('Ctrl Pts',(-48.0561422858351,-40.5222287925639,
-235.350050000001));
#195480=CARTESIAN_POINT('Ctrl Pts',(-48.0477736645017,-40.563085046475,
-235.35005));
#195481=CARTESIAN_POINT('Ctrl Pts',(-48.0387080967012,-40.6037929031184,
-235.35005));
#195482=CARTESIAN_POINT('Ctrl Pts',(-48.0296425710794,-40.6445005703635,
-235.35005));
#195483=CARTESIAN_POINT('Ctrl Pts',(-48.0199029935916,-40.6850742166469,
-235.35005));
#195484=CARTESIAN_POINT('Ctrl Pts',(-48.0095985320967,-40.7255015726492,
-235.35005));
#195485=CARTESIAN_POINT('Ctrl Pts',(-47.9992939746968,-40.7659293049141,
-235.35005));
#195486=CARTESIAN_POINT('Ctrl Pts',(-47.9883596446658,-40.8062073663638,
-235.35005));
#195487=CARTESIAN_POINT('Ctrl Pts',(-47.9766041319244,-40.8462239751862,
-235.35005));
#195488=CARTESIAN_POINT('Ctrl Pts',(-47.9648483456559,-40.8862415151148,
-235.35005));
#195489=CARTESIAN_POINT('Ctrl Pts',(-47.9522082011025,-40.9259753165071,
-235.35005));
#195490=CARTESIAN_POINT('Ctrl Pts',(-47.9388792235724,-40.965487693427,
-235.35005));
#195491=CARTESIAN_POINT('Ctrl Pts',(-47.9122207498503,-41.0445139847866,
-235.35005));
#195492=CARTESIAN_POINT('Ctrl Pts',(-47.8834172501653,-41.1228517627344,
-235.35005));
#195493=CARTESIAN_POINT('Ctrl Pts',(-47.8525616386501,-41.2000593734148,
-235.35005));
#195494=CARTESIAN_POINT('Ctrl Pts',(-47.8371337962268,-41.2386632705008,
-235.35005));
#195495=CARTESIAN_POINT('Ctrl Pts',(-47.8210253173756,-41.2769359691183,
-235.35005));
#195496=CARTESIAN_POINT('Ctrl Pts',(-47.8041226974982,-41.3148222784138,
-235.35005));
#195497=CARTESIAN_POINT('Ctrl Pts',(-47.7872200865336,-41.3527085677318,
-235.35005));
#195498=CARTESIAN_POINT('Ctrl Pts',(-47.7696001482572,-41.3902458425851,
-235.35005));
#195499=CARTESIAN_POINT('Ctrl Pts',(-47.7515778408436,-41.4275873872532,
-235.35005));
#195500=CARTESIAN_POINT('Ctrl Pts',(-47.7335555714763,-41.4649288530907,
-235.35005));
#195501=CARTESIAN_POINT('Ctrl Pts',(-47.7151164076773,-41.5020675212465,
-235.35005));
#195502=CARTESIAN_POINT('Ctrl Pts',(-47.69640382207,-41.5390732370252,-235.35005));
#195503=CARTESIAN_POINT('Ctrl Pts',(-47.6870475533414,-41.5575760473041,
-235.35005));
#195504=CARTESIAN_POINT('Ctrl Pts',(-47.6776404221482,-41.5760541309719,
-235.35005));
#195505=CARTESIAN_POINT('Ctrl Pts',(-47.6681082454436,-41.594471397704,
-235.35005));
#195506=CARTESIAN_POINT('Ctrl Pts',(-47.6585760901228,-41.6128886231199,
-235.35005));
#195507=CARTESIAN_POINT('Ctrl Pts',(-47.6488991892717,-41.6312354462549,
-235.35005));
#195508=CARTESIAN_POINT('Ctrl Pts',(-47.6389908341615,-41.649469682206,
-235.35005));
#195509=CARTESIAN_POINT('Ctrl Pts',(-47.6191742063161,-41.6859380025145,
-235.35005));
#195510=CARTESIAN_POINT('Ctrl Pts',(-47.5984065690065,-41.7219437163951,
-235.35005));
#195511=CARTESIAN_POINT('Ctrl Pts',(-47.5769871577403,-41.7576324579108,
-235.35005));
#195512=CARTESIAN_POINT('Ctrl Pts',(-47.5555678934573,-41.7933209545252,
-235.35005));
#195513=CARTESIAN_POINT('Ctrl Pts',(-47.5335334800369,-41.8287110790685,
-235.35005));
#195514=CARTESIAN_POINT('Ctrl Pts',(-47.511140470057,-41.8639253579254,
-235.35005));
#195515=CARTESIAN_POINT('Ctrl Pts',(-47.8490613455157,-41.3259332563119,
-235.35005));
#195516=CARTESIAN_POINT('Ctrl Pts',(-48.3747699923712,-41.6520493882069,
-235.350050000092));
#195517=CARTESIAN_POINT('Ctrl Pts',(-48.7476545690025,-41.8833242138032,
-234.913932346582));
#195518=CARTESIAN_POINT('Ctrl Pts',(-46.4600121576292,-43.5649251296408,
-235.35005));
#195519=CARTESIAN_POINT('Ctrl Pts',(-46.9677567717061,-43.9091204986021,
-235.350049999619));
#195520=CARTESIAN_POINT('Ctrl Pts',(-47.3267956366018,-44.1603069972551,
-234.920895256829));
#195521=CARTESIAN_POINT('Ctrl Pts',(-44.9336721901564,-45.6801579018413,
-235.35005));
#195522=CARTESIAN_POINT('Ctrl Pts',(-45.4194497174212,-46.0456552594643,
-235.35005000036));
#195523=CARTESIAN_POINT('Ctrl Pts',(-45.766217636631,-46.3109458093001,
-234.927737734568));
#195524=CARTESIAN_POINT('Ctrl Pts',(-41.7430470430268,-49.5044128120585,
-235.35005));
#195525=CARTESIAN_POINT('Ctrl Pts',(-42.1885337805295,-49.9078910798639,
-235.350049999669));
#195526=CARTESIAN_POINT('Ctrl Pts',(-42.5090368690587,-50.2021749925663,
-234.935613379076));
#195527=CARTESIAN_POINT('Ctrl Pts',(-40.1030327246601,-51.2355371590317,
-235.35005));
#195528=CARTESIAN_POINT('Ctrl Pts',(-40.5296034202201,-51.6572713554155,
-235.350049999933));
#195529=CARTESIAN_POINT('Ctrl Pts',(-40.8393366907154,-51.9623573328398,
-234.937115568349));
#195530=CARTESIAN_POINT('Ctrl Pts',(-37.4698285345256,-53.6756545350797,
-235.35005));
#195531=CARTESIAN_POINT('Ctrl Pts',(-37.8681542571236,-54.12532384821,-235.350050000033));
#195532=CARTESIAN_POINT('Ctrl Pts',(-38.156565261625,-54.4506060236705,
-234.935579133827));
#195533=CARTESIAN_POINT('Ctrl Pts',(-36.5624534933628,-54.4622301034484,
-235.35005));
#195534=CARTESIAN_POINT('Ctrl Pts',(-36.9514272410634,-54.9212055845083,
-235.350050000067));
#195535=CARTESIAN_POINT('Ctrl Pts',(-37.2331480650446,-55.2526051792597,
-234.934472078277));
#195536=CARTESIAN_POINT('Ctrl Pts',(-34.6902365366833,-55.9834272130437,
-235.35005));
#195537=CARTESIAN_POINT('Ctrl Pts',(-35.0610225513123,-56.460769206042,
-235.350049999933));
#195538=CARTESIAN_POINT('Ctrl Pts',(-35.3287738309422,-56.8043909143739,
-234.931153092782));
#195539=CARTESIAN_POINT('Ctrl Pts',(-33.7267628103062,-56.7166866533048,
-235.35005));
#195540=CARTESIAN_POINT('Ctrl Pts',(-34.0882410053241,-57.2034119551093,
-235.35005000005));
#195541=CARTESIAN_POINT('Ctrl Pts',(-34.3491709331613,-57.5528337949308,
-234.928940594182));
#195542=CARTESIAN_POINT('Ctrl Pts',(-30.6073913272127,-58.9341159455743,
-235.35005));
#195543=CARTESIAN_POINT('Ctrl Pts',(-30.9368021706629,-59.4530013653618,
-235.350049999891));
#195544=CARTESIAN_POINT('Ctrl Pts',(-31.1761355813162,-59.8199396241448,
-234.919813894401));
#195545=CARTESIAN_POINT('Ctrl Pts',(-28.3683440394259,-60.2964424520783,
-235.35005));
#195546=CARTESIAN_POINT('Ctrl Pts',(-28.6756334162834,-60.836946555824,
-235.350050001328));
#195547=CARTESIAN_POINT('Ctrl Pts',(-28.8994459060213,-61.2157980870126,
-234.910838324051));
#195548=CARTESIAN_POINT('Ctrl Pts',(-26.0302603908518,-61.5065343641464,
-235.35005));
#195549=CARTESIAN_POINT('Ctrl Pts',(-26.3187522905012,-62.0639404421789,
-235.350049999653));
#195550=CARTESIAN_POINT('Ctrl Pts',(-26.5212311387933,-62.4552736145252,
-234.903064166399));
#195551=CARTESIAN_POINT('',(-27.0930165135311,-62.1526330725429,-234.905475377596));
#195552=CARTESIAN_POINT('',(-26.5926469327273,-61.2115127003622,-235.35005));
#195553=CARTESIAN_POINT('Origin',(-26.5926469327274,-61.2115127003622,-233.85005));
#195554=CARTESIAN_POINT('Ctrl Pts',(-27.0930165135311,-62.1526330725429,
-234.905475377596));
#195555=CARTESIAN_POINT('Ctrl Pts',(-27.413195626475,-61.9811958993946,
-234.906550894347));
#195556=CARTESIAN_POINT('Ctrl Pts',(-27.7316250998112,-61.806783331475,
-234.907642668818));
#195557=CARTESIAN_POINT('Ctrl Pts',(-28.0482019218833,-61.6294717423287,
-234.908740933506));
#195558=CARTESIAN_POINT('Ctrl Pts',(-28.3727830990628,-61.4476769919867,
-234.909866966812));
#195559=CARTESIAN_POINT('Ctrl Pts',(-28.6954170670635,-61.2628348870667,
-234.910999822682));
#195560=CARTESIAN_POINT('Ctrl Pts',(-29.0160394951108,-61.0749975381793,
-234.912128973837));
#195561=CARTESIAN_POINT('Ctrl Pts',(-29.3446312847752,-60.8824913214041,
-234.913286191069));
#195562=CARTESIAN_POINT('Ctrl Pts',(-29.6711106331574,-60.6868392410698,
-234.914439517128));
#195563=CARTESIAN_POINT('Ctrl Pts',(-29.9954516963743,-60.4880641482463,
-234.915577620065));
#195564=CARTESIAN_POINT('Ctrl Pts',(-30.3309190242629,-60.2824702324498,
-234.916754764727));
#195565=CARTESIAN_POINT('Ctrl Pts',(-30.6640991632103,-60.0735355716976,
-234.917915623919));
#195566=CARTESIAN_POINT('Ctrl Pts',(-30.995004380144,-59.8612476284684,
-234.919047659027));
#195567=CARTESIAN_POINT('Ctrl Pts',(-31.3472214532825,-59.6352873407472,
-234.920252602533));
#195568=CARTESIAN_POINT('Ctrl Pts',(-31.6968613621572,-59.405528414312,
-234.921424889581));
#195569=CARTESIAN_POINT('Ctrl Pts',(-32.0439803902238,-59.1719078383533,
-234.92254939954));
#195570=CARTESIAN_POINT('Ctrl Pts',(-32.3910994182905,-58.9382872623945,
-234.9236739095));
#195571=CARTESIAN_POINT('Ctrl Pts',(-32.7356982077542,-58.7008050508717,
-234.924750642371));
#195572=CARTESIAN_POINT('Ctrl Pts',(-33.0778659127508,-58.4593486694961,
-234.925764477524));
#195573=CARTESIAN_POINT('Ctrl Pts',(-33.1685786188303,-58.3953357266178,
-234.926033257216));
#195574=CARTESIAN_POINT('Ctrl Pts',(-33.2591205999179,-58.3310432043412,
-234.926297616187));
#195575=CARTESIAN_POINT('Ctrl Pts',(-33.349489416723,-58.2664755177344,
-234.926557272691));
#195576=CARTESIAN_POINT('Ctrl Pts',(-33.6805726000371,-58.0299196351103,
-234.927508573207));
#195577=CARTESIAN_POINT('Ctrl Pts',(-34.0095024056148,-57.7895622326326,
-234.92838728666));
#195578=CARTESIAN_POINT('Ctrl Pts',(-34.3359738414799,-57.5456966712594,
-234.929197374532));
#195579=CARTESIAN_POINT('Ctrl Pts',(-34.6775776197641,-57.290527648776,
-234.930045010948));
#195580=CARTESIAN_POINT('Ctrl Pts',(-35.0164901255299,-57.0315177572273,
-234.930817512589));
#195581=CARTESIAN_POINT('Ctrl Pts',(-35.3523953581095,-56.7689545310704,
-234.931519417723));
#195582=CARTESIAN_POINT('Ctrl Pts',(-35.6644839022428,-56.5250078251351,
-234.932171555677));
#195583=CARTESIAN_POINT('Ctrl Pts',(-35.9739771741295,-56.2779931164497,
-234.932762753228));
#195584=CARTESIAN_POINT('Ctrl Pts',(-36.2806420570433,-56.0281062971809,
-234.933296650138));
#195585=CARTESIAN_POINT('Ctrl Pts',(-36.5944525970113,-55.7723968173717,
-234.933842987482));
#195586=CARTESIAN_POINT('Ctrl Pts',(-36.9051332693568,-55.513819084103,
-234.934329384607));
#195587=CARTESIAN_POINT('Ctrl Pts',(-37.212676387903,-55.2523756338014,
-234.934754322762));
#195588=CARTESIAN_POINT('Ctrl Pts',(-37.5296715840886,-54.9828969401745,
-234.935192321032));
#195589=CARTESIAN_POINT('Ctrl Pts',(-37.843334309156,-54.7103734208553,
-234.9355650245));
#195590=CARTESIAN_POINT('Ctrl Pts',(-38.1536516617129,-54.4347520208089,
-234.935870770035));
#195591=CARTESIAN_POINT('Ctrl Pts',(-38.4373467668722,-54.1827762887848,
-234.93615028554));
#195592=CARTESIAN_POINT('Ctrl Pts',(-38.7182463400772,-53.9282104733727,
-234.936373838997));
#195593=CARTESIAN_POINT('Ctrl Pts',(-38.9963275074405,-53.6709782511683,
-234.936540159646));
#195594=CARTESIAN_POINT('Ctrl Pts',(-39.0143899505921,-53.6542700273271,
-234.936550962813));
#195595=CARTESIAN_POINT('Ctrl Pts',(-39.0324404966293,-53.6375505430169,
-234.936561524514));
#195596=CARTESIAN_POINT('Ctrl Pts',(-39.0504791753982,-53.6208198170148,
-234.936571844402));
#195597=CARTESIAN_POINT('Ctrl Pts',(-39.3472231023317,-53.345592268593,
-234.936741610941));
#195598=CARTESIAN_POINT('Ctrl Pts',(-39.6405448825184,-53.0675295916505,
-234.936841900903));
#195599=CARTESIAN_POINT('Ctrl Pts',(-39.9306089570722,-52.7866701993791,
-234.936873881775));
#195600=CARTESIAN_POINT('Ctrl Pts',(-40.2222927218382,-52.5042425149663,
-234.936906041225));
#195601=CARTESIAN_POINT('Ctrl Pts',(-40.5106828951419,-52.2189859602739,
-234.936869126592));
#195602=CARTESIAN_POINT('Ctrl Pts',(-40.795907303629,-51.9309049610937,
-234.936764325029));
#195603=CARTESIAN_POINT('Ctrl Pts',(-41.0810717798481,-51.6428844944174,
-234.936659545487));
#195604=CARTESIAN_POINT('Ctrl Pts',(-41.3630724097311,-51.3520399040605,
-234.936486907542));
#195605=CARTESIAN_POINT('Ctrl Pts',(-41.6419888382853,-51.0583539066569,
-234.936247597597));
#195606=CARTESIAN_POINT('Ctrl Pts',(-41.9064967149108,-50.7798394427705,
-234.936020650171));
#195607=CARTESIAN_POINT('Ctrl Pts',(-42.1682309029012,-50.4987687635823,
-234.935733741244));
#195608=CARTESIAN_POINT('Ctrl Pts',(-42.4272119239977,-50.2151197543423,
-234.935387882688));
#195609=CARTESIAN_POINT('Ctrl Pts',(-42.6786802319399,-49.9396990455156,
-234.935052057053));
#195610=CARTESIAN_POINT('Ctrl Pts',(-42.9275530115785,-49.661846815414,
-234.934660652292));
#195611=CARTESIAN_POINT('Ctrl Pts',(-43.1738006413473,-49.3815456163509,
-234.934214594749));
#195612=CARTESIAN_POINT('Ctrl Pts',(-43.4097500016249,-49.1129668338219,
-234.933787191683));
#195613=CARTESIAN_POINT('Ctrl Pts',(-43.6432892642155,-48.8421391713728,
-234.933309611494));
#195614=CARTESIAN_POINT('Ctrl Pts',(-43.8743453439068,-48.569057500808,
-234.932782669097));
#195615=CARTESIAN_POINT('Ctrl Pts',(-43.9394227130495,-48.4921435468224,
-234.932634254803));
#195616=CARTESIAN_POINT('Ctrl Pts',(-44.0043027963191,-48.4150508747269,
-234.932481924716));
#195617=CARTESIAN_POINT('Ctrl Pts',(-44.0689832334686,-48.3377796011446,
-234.932325697043));
#195618=CARTESIAN_POINT('Ctrl Pts',(-44.1257979573804,-48.2699051978728,
-234.932188468037));
#195619=CARTESIAN_POINT('Ctrl Pts',(-44.1824559314928,-48.2018963303122,
-234.932048170913));
#195620=CARTESIAN_POINT('Ctrl Pts',(-44.2389548542018,-48.1337537075507,
-234.931904903882));
#195621=CARTESIAN_POINT('Ctrl Pts',(-44.4921805476008,-47.8283414612372,
-234.931262787335));
#195622=CARTESIAN_POINT('Ctrl Pts',(-44.7422147854006,-47.5202407572862,
-234.930561011512));
#195623=CARTESIAN_POINT('Ctrl Pts',(-44.989159053384,-47.2093593138889,
-234.929808418714));
#195624=CARTESIAN_POINT('Ctrl Pts',(-45.2313979342307,-46.9044015453222,
-234.929070166157));
#195625=CARTESIAN_POINT('Ctrl Pts',(-45.4706633831556,-46.5967675687619,
-234.928283014753));
#195626=CARTESIAN_POINT('Ctrl Pts',(-45.7070074376436,-46.2863940216118,
-234.927455310917));
#195627=CARTESIAN_POINT('Ctrl Pts',(-45.9433319726432,-45.9760461079935,
-234.92662767544));
#195628=CARTESIAN_POINT('Ctrl Pts',(-46.1767356503047,-45.6629585377323,
-234.92575949423));
#195629=CARTESIAN_POINT('Ctrl Pts',(-46.4072264172074,-45.3470992417083,
-234.924859111632));
#195630=CARTESIAN_POINT('Ctrl Pts',(-46.6250331931149,-45.0486217979831,
-234.924008277417));
#195631=CARTESIAN_POINT('Ctrl Pts',(-46.8402385289181,-44.7476691212717,
-234.923128688407));
#195632=CARTESIAN_POINT('Ctrl Pts',(-47.0528122363433,-44.4442466607797,
-234.922227385789));
#195633=CARTESIAN_POINT('Ctrl Pts',(-47.2609703925988,-44.1471268489858,
-234.921344804901));
#195634=CARTESIAN_POINT('Ctrl Pts',(-47.4666050432284,-43.8476384603018,
-234.920441403102));
#195635=CARTESIAN_POINT('Ctrl Pts',(-47.6696538011198,-43.545822585116,
-234.919523791852));
#195636=CARTESIAN_POINT('Ctrl Pts',(-47.8666767356436,-43.2529636184694,
-234.918633412305));
#195637=CARTESIAN_POINT('Ctrl Pts',(-48.0612648724898,-42.9579130133239,
-234.917729654174));
#195638=CARTESIAN_POINT('Ctrl Pts',(-48.2533302009523,-42.6607466370678,
-234.916818557597));
#195639=CARTESIAN_POINT('Ctrl Pts',(-48.3029165880433,-42.5840258302391,
-234.916583335613));
#195640=CARTESIAN_POINT('Ctrl Pts',(-48.3523346590842,-42.5071642134369,
-234.916347624492));
#195641=CARTESIAN_POINT('Ctrl Pts',(-48.4015825627194,-42.4301635567086,
-234.916111528174));
#195642=CARTESIAN_POINT('Ctrl Pts',(-47.511140470057,-41.8639253579254,
-235.35005));
#195643=CARTESIAN_POINT('Ctrl Pts',(-46.5263591620702,-43.4125505315913,
-235.35005));
#195644=CARTESIAN_POINT('Ctrl Pts',(-45.4748377912678,-44.9008380775538,
-235.35005));
#195645=CARTESIAN_POINT('Ctrl Pts',(-44.3570056200861,-46.3291760712173,
-235.35005));
#195646=CARTESIAN_POINT('Ctrl Pts',(-44.0018587501911,-46.7829738600798,
-235.35005));
#195647=CARTESIAN_POINT('Ctrl Pts',(-43.6400181829371,-47.2307200839753,
-235.35005));
#195648=CARTESIAN_POINT('Ctrl Pts',(-43.2714968690733,-47.6724264514822,
-235.35005));
#195649=CARTESIAN_POINT('Ctrl Pts',(-41.7430470430284,-49.5044128120552,
-235.35005));
#195650=CARTESIAN_POINT('Ctrl Pts',(-40.1030327246406,-51.2355371590496,
-235.35005));
#195651=CARTESIAN_POINT('Ctrl Pts',(-38.3475632646338,-52.8622820764655,
-235.35005));
#195652=CARTESIAN_POINT('Ctrl Pts',(-37.4698285346305,-53.6756545351735,
-235.35005));
#195653=CARTESIAN_POINT('Ctrl Pts',(-36.5624534933633,-54.462230103448,
-235.35005));
#195654=CARTESIAN_POINT('Ctrl Pts',(-35.626345015024,-55.2228286582473,
-235.35005));
#195655=CARTESIAN_POINT('Ctrl Pts',(-34.6902365366847,-55.9834272130465,
-235.35005));
#195656=CARTESIAN_POINT('Ctrl Pts',(-33.7267628103146,-56.7166866532988,
-235.35005));
#195657=CARTESIAN_POINT('Ctrl Pts',(-32.7442779891666,-57.4150935706736,
-235.35005));
#195658=CARTESIAN_POINT('Ctrl Pts',(-30.9377005462682,-58.6993130881001,
-235.35005));
#195659=CARTESIAN_POINT('Ctrl Pts',(-29.058139432765,-59.8715157745017,
-235.35005));
#195660=CARTESIAN_POINT('Ctrl Pts',(-27.1073861239119,-60.9344512250895,
-235.35005));
#195661=CARTESIAN_POINT('Ctrl Pts',(-26.9363532638007,-61.0276443979026,
-235.35005));
#195662=CARTESIAN_POINT('Ctrl Pts',(-26.7647731343801,-61.119997610569,
-235.35005));
#195663=CARTESIAN_POINT('Ctrl Pts',(-26.5926469327273,-61.2115127003622,
-235.35005));
#195664=CARTESIAN_POINT('Ctrl Pts',(-26.5926469327274,-61.2115127003621,
-235.35005));
#195665=CARTESIAN_POINT('Ctrl Pts',(-26.8863570828205,-61.7639375806376,
-235.35005));
#195666=CARTESIAN_POINT('Ctrl Pts',(-27.0930165135311,-62.1526330725429,
-234.905475377596));
#195667=CARTESIAN_POINT('Ctrl Pts',(-26.5307880850042,-61.2444014821219,
-235.35005));
#195668=CARTESIAN_POINT('Ctrl Pts',(-26.821340159478,-61.8016677190097,
-235.350049999993));
#195669=CARTESIAN_POINT('Ctrl Pts',(-27.0252222584354,-62.1924330785486,
-234.902126572898));
#195670=CARTESIAN_POINT('Ctrl Pts',(-26.4686210255564,-61.2766595567632,
-235.35005));
#195671=CARTESIAN_POINT('Ctrl Pts',(-26.7519016982533,-61.843293170753,
-235.350049999997));
#195672=CARTESIAN_POINT('Ctrl Pts',(-26.9497402120697,-62.2385292812946,
-234.896449373983));
#195673=CARTESIAN_POINT('Ctrl Pts',(-26.3891388204284,-61.3131722991992,
-235.35005));
#195674=CARTESIAN_POINT('Ctrl Pts',(-26.6543883005772,-61.9032639296083,
-235.350050000001));
#195675=CARTESIAN_POINT('Ctrl Pts',(-26.8364482204274,-62.3082529158846,
-234.8795305279));
#195676=CARTESIAN_POINT('Ctrl Pts',(-26.3731447836042,-61.3202661527697,
-235.35005));
#195677=CARTESIAN_POINT('Ctrl Pts',(-26.634890969524,-61.9147711240481,
-235.350050000004));
#195678=CARTESIAN_POINT('Ctrl Pts',(-26.8139780721898,-62.3215114290266,
-234.876306139112));
#195679=CARTESIAN_POINT('Ctrl Pts',(-26.341052548261,-61.3342311248494,
-235.35005));
#195680=CARTESIAN_POINT('Ctrl Pts',(-26.5987725347511,-61.9335243765778,
-235.350049999996));
#195681=CARTESIAN_POINT('Ctrl Pts',(-26.7745169875525,-62.3421733148585,
-234.872883709682));
#195682=CARTESIAN_POINT('Ctrl Pts',(-26.324963993434,-61.3411228649431,
-235.35005));
#195683=CARTESIAN_POINT('Ctrl Pts',(-26.5822418971017,-61.9407189173202,
-235.350050000003));
#195684=CARTESIAN_POINT('Ctrl Pts',(-26.7576550280567,-62.3495221049909,
-234.872747949079));
#195685=CARTESIAN_POINT('Ctrl Pts',(-26.2766869482483,-61.3617737493097,
-235.35005));
#195686=CARTESIAN_POINT('Ctrl Pts',(-26.5322022210074,-61.9628463306943,
-235.350049999995));
#195687=CARTESIAN_POINT('Ctrl Pts',(-26.7062785831568,-62.3723269401802,
-234.871930575498));
#195688=CARTESIAN_POINT('Ctrl Pts',(-26.2444517981386,-61.3754399401447,
-235.35005));
#195689=CARTESIAN_POINT('Ctrl Pts',(-26.4983809904187,-61.9780069834906,
-235.350049999998));
#195690=CARTESIAN_POINT('Ctrl Pts',(-26.6712306199245,-62.3881303051001,
-234.871005091044));
#195691=CARTESIAN_POINT('Ctrl Pts',(-26.1797908377429,-61.4023344685258,
-235.35005));
#195692=CARTESIAN_POINT('Ctrl Pts',(-26.4290695787371,-62.0096639879438,
-235.350050000002));
#195693=CARTESIAN_POINT('Ctrl Pts',(-26.598219218148,-62.4217260874495,
-234.867787528297));
#195694=CARTESIAN_POINT('Ctrl Pts',(-26.1473795281051,-61.4155758832315,
-235.35005));
#195695=CARTESIAN_POINT('Ctrl Pts',(-26.3937643073098,-62.0259679052544,
-235.350050000003));
#195696=CARTESIAN_POINT('Ctrl Pts',(-26.5606263859936,-62.4392448432971,
-234.865676603548));
#195697=CARTESIAN_POINT('Ctrl Pts',(-26.0821804763413,-61.4411000467081,
-235.35005));
#195698=CARTESIAN_POINT('Ctrl Pts',(-26.3181216753443,-62.0629567534453,
-235.350049999997));
#195699=CARTESIAN_POINT('Ctrl Pts',(-26.4765766579827,-62.4804755152087,
-234.857183986946));
#195700=CARTESIAN_POINT('Ctrl Pts',(-26.0493312864126,-61.4532499966124,
-235.350050000001));
#195701=CARTESIAN_POINT('Ctrl Pts',(-26.2774828535028,-62.0835800223265,
-235.350050000008));
#195702=CARTESIAN_POINT('Ctrl Pts',(-26.4297212650746,-62.5040608637178,
-234.850690950979));
#195703=CARTESIAN_POINT('Ctrl Pts',(-25.9501566901715,-61.4879342004266,
-235.350050000001));
#195704=CARTESIAN_POINT('Ctrl Pts',(-26.1609807722306,-62.1355066696273,
-235.350049999986));
#195705=CARTESIAN_POINT('Ctrl Pts',(-26.299935026532,-62.5618001346298,
-234.837570256781));
#195706=CARTESIAN_POINT('Ctrl Pts',(-25.8834819572284,-61.509419252042,
-235.35005));
#195707=CARTESIAN_POINT('Ctrl Pts',(-26.0918719141122,-62.1577719822702,
-235.350049999986));
#195708=CARTESIAN_POINT('Ctrl Pts',(-26.2291985619127,-62.5845560253671,
-234.837502470078));
#195709=CARTESIAN_POINT('Ctrl Pts',(-25.7996807895498,-61.534730893345,
-235.35005));
#195710=CARTESIAN_POINT('Ctrl Pts',(-25.9958115105161,-62.1946041207473,
-235.350050000004));
#195711=CARTESIAN_POINT('Ctrl Pts',(-26.1237073939439,-62.6248724643351,
-234.828124366513));
#195712=CARTESIAN_POINT('Ctrl Pts',(-25.7828903569215,-61.5396828918313,
-235.35005));
#195713=CARTESIAN_POINT('Ctrl Pts',(-25.976181775626,-62.2022533875226,
-235.35005000001));
#195714=CARTESIAN_POINT('Ctrl Pts',(-26.1019429230186,-62.6332968405534,
-234.825896748429));
#195715=CARTESIAN_POINT('Ctrl Pts',(-25.7492255098059,-61.5492800686396,
-235.35005));
#195716=CARTESIAN_POINT('Ctrl Pts',(-25.9355808625229,-62.2185181387375,
-235.35004999999));
#195717=CARTESIAN_POINT('Ctrl Pts',(-26.056126511479,-62.651374227355,-234.820237176746));
#195718=CARTESIAN_POINT('Ctrl Pts',(-25.7323477164287,-61.5539129022783,
-235.35005));
#195719=CARTESIAN_POINT('Ctrl Pts',(-25.9142407405854,-62.2274858229347,
-235.350050000002));
#195720=CARTESIAN_POINT('Ctrl Pts',(-26.0314456183935,-62.6614557970582,
-234.816472473606));
#195721=CARTESIAN_POINT('Ctrl Pts',(-25.6815605387409,-61.5672495175189,
-235.35005));
#195722=CARTESIAN_POINT('Ctrl Pts',(-25.8513370817052,-62.2523278228314,
-235.350049999996));
#195723=CARTESIAN_POINT('Ctrl Pts',(-25.9596326032101,-62.6890827742206,
-234.806344353949));
#195724=CARTESIAN_POINT('Ctrl Pts',(-25.6474983161402,-61.5754339876196,
-235.35005));
#195725=CARTESIAN_POINT('Ctrl Pts',(-25.8103146214907,-62.2668945351399,
-235.350050000001));
#195726=CARTESIAN_POINT('Ctrl Pts',(-25.9135255401439,-62.7050301838465,
-234.800516173084));
#195727=CARTESIAN_POINT('Ctrl Pts',(-25.5791807904238,-61.5908730316921,
-235.35005));
#195728=CARTESIAN_POINT('Ctrl Pts',(-25.731028783567,-62.2921464778074,
-235.350049999999));
#195729=CARTESIAN_POINT('Ctrl Pts',(-25.8263731088601,-62.7322675488681,
-234.791463019912));
#195730=CARTESIAN_POINT('Ctrl Pts',(-25.5449390466137,-61.5981933980485,
-235.35005));
#195731=CARTESIAN_POINT('Ctrl Pts',(-25.6927227699064,-62.3029939210129,
-235.350050000007));
#195732=CARTESIAN_POINT('Ctrl Pts',(-25.7851988792686,-62.7437844019476,
-234.788172738052));
#195733=CARTESIAN_POINT('Ctrl Pts',(-25.4762602753847,-61.6118947761917,
-235.35005));
#195734=CARTESIAN_POINT('Ctrl Pts',(-25.6117842070045,-62.3276542792517,
-235.350049999993));
#195735=CARTESIAN_POINT('Ctrl Pts',(-25.6956346706304,-62.770238922023,
-234.777569028842));
#195736=CARTESIAN_POINT('Ctrl Pts',(-25.441793602875,-61.6182439225594,
-235.35005));
#195737=CARTESIAN_POINT('Ctrl Pts',(-25.5698816498182,-62.3406532746031,
-235.350049999995));
#195738=CARTESIAN_POINT('Ctrl Pts',(-25.6485908901075,-62.7841922736754,
-234.770997188221));
#195739=CARTESIAN_POINT('Ctrl Pts',(-25.3727171465013,-61.6295518156141,
-235.35005));
#195740=CARTESIAN_POINT('Ctrl Pts',(-25.4834982706708,-62.367218439294,
-235.350050000006));
#195741=CARTESIAN_POINT('Ctrl Pts',(-25.5504255841634,-62.8124292406126,
-234.755348365089));
#195742=CARTESIAN_POINT('Ctrl Pts',(-25.3381059806223,-61.6345074287981,
-235.35005));
#195743=CARTESIAN_POINT('Ctrl Pts',(-25.4409641703014,-62.3790113723438,
-235.350050000011));
#195744=CARTESIAN_POINT('Ctrl Pts',(-25.502603574716,-62.8247454634089,
-234.748093190059));
#195745=CARTESIAN_POINT('Ctrl Pts',(-25.2687752030225,-61.6433803535082,
-235.35005));
#195746=CARTESIAN_POINT('Ctrl Pts',(-25.3578642498523,-62.399590514639,
-235.350049999988));
#195747=CARTESIAN_POINT('Ctrl Pts',(-25.4105087856878,-62.8459575195944,
-234.735446711282));
#195748=CARTESIAN_POINT('Ctrl Pts',(-25.2340567625657,-61.647308878831,
-235.35005));
#195749=CARTESIAN_POINT('Ctrl Pts',(-25.3180366392519,-62.4077933846439,
-235.350049999987));
#195750=CARTESIAN_POINT('Ctrl Pts',(-25.3673989913123,-62.8542900606576,
-234.730725127778));
#195751=CARTESIAN_POINT('Ctrl Pts',(-25.1645355171699,-61.6543581913618,
-235.35005));
#195752=CARTESIAN_POINT('Ctrl Pts',(-25.2357480959957,-62.4254349365975,
-235.350050000013));
#195753=CARTESIAN_POINT('Ctrl Pts',(-25.277049571495,-62.8720350725204,
-234.718828491406));
#195754=CARTESIAN_POINT('Ctrl Pts',(-25.1297211288812,-61.6573680755603,
-235.350050000001));
#195755=CARTESIAN_POINT('Ctrl Pts',(-25.1911613073834,-62.4364284584908,
-235.350049999998));
#195756=CARTESIAN_POINT('Ctrl Pts',(-25.2264460848463,-62.8829206549938,
-234.709697846434));
#195757=CARTESIAN_POINT('Ctrl Pts',(-25.0599498736116,-61.6620236980061,
-235.350050000001));
#195758=CARTESIAN_POINT('Ctrl Pts',(-25.1032793349872,-62.4555089444949,
-235.350050000003));
#195759=CARTESIAN_POINT('Ctrl Pts',(-25.1276927878133,-62.9012647282465,
-234.692677918945));
#195760=CARTESIAN_POINT('Ctrl Pts',(-25.0249977138784,-61.6637138702923,
-235.35005));
#195761=CARTESIAN_POINT('Ctrl Pts',(-25.0601909996374,-62.4634558478501,
-235.350050000029));
#195762=CARTESIAN_POINT('Ctrl Pts',(-25.0798352875815,-62.9086680015632,
-234.685060290672));
#195763=CARTESIAN_POINT('Ctrl Pts',(-24.989999724813,-61.6649665253884,
-235.35005));
#195764=CARTESIAN_POINT('Ctrl Pts',(-25.0188032481003,-62.4697021984285,
-235.35005));
#195765=CARTESIAN_POINT('Ctrl Pts',(-25.0347190704466,-62.9143710634145,
-234.67889768232));
#195766=CARTESIAN_POINT('',(-25.0347190704488,-62.9143710634153,-234.678897682319));
#195767=CARTESIAN_POINT('',(-24.9899997248189,-61.6649665253882,-235.35005));
#195768=CARTESIAN_POINT('Origin',(-24.9899997248189,-61.6649665253882,-233.85005));
#195769=CARTESIAN_POINT('Ctrl Pts',(-25.0347190704488,-62.9143710634153,
-234.678897682319));
#195770=CARTESIAN_POINT('Ctrl Pts',(-25.0798352875815,-62.9086680015632,
-234.685060290672));
#195771=CARTESIAN_POINT('Ctrl Pts',(-25.1276927878133,-62.9012647282465,
-234.692677918945));
#195772=CARTESIAN_POINT('Ctrl Pts',(-25.2264460848463,-62.8829206549938,
-234.709697846434));
#195773=CARTESIAN_POINT('Ctrl Pts',(-25.277049571495,-62.8720350725204,
-234.718828491406));
#195774=CARTESIAN_POINT('Ctrl Pts',(-25.3673989913123,-62.8542900606576,
-234.730725127778));
#195775=CARTESIAN_POINT('Ctrl Pts',(-25.4105087856878,-62.8459575195944,
-234.735446711282));
#195776=CARTESIAN_POINT('Ctrl Pts',(-25.502603574716,-62.8247454634089,
-234.748093190059));
#195777=CARTESIAN_POINT('Ctrl Pts',(-25.5504255841634,-62.8124292406126,
-234.755348365089));
#195778=CARTESIAN_POINT('Ctrl Pts',(-25.6485908901075,-62.7841922736754,
-234.770997188221));
#195779=CARTESIAN_POINT('Ctrl Pts',(-25.6956346706304,-62.770238922023,
-234.777569028842));
#195780=CARTESIAN_POINT('Ctrl Pts',(-25.7851988792686,-62.7437844019476,
-234.788172738052));
#195781=CARTESIAN_POINT('Ctrl Pts',(-25.8263731088601,-62.7322675488681,
-234.791463019912));
#195782=CARTESIAN_POINT('Ctrl Pts',(-25.9135255401439,-62.7050301838465,
-234.800516173084));
#195783=CARTESIAN_POINT('Ctrl Pts',(-25.9596326032101,-62.6890827742206,
-234.806344353949));
#195784=CARTESIAN_POINT('Ctrl Pts',(-26.0314456183935,-62.6614557970582,
-234.816472473606));
#195785=CARTESIAN_POINT('Ctrl Pts',(-26.056126511479,-62.651374227355,-234.820237176746));
#195786=CARTESIAN_POINT('Ctrl Pts',(-26.1019429230186,-62.6332968405534,
-234.825896748429));
#195787=CARTESIAN_POINT('Ctrl Pts',(-26.1237073939439,-62.6248724643351,
-234.828124366513));
#195788=CARTESIAN_POINT('Ctrl Pts',(-26.2291985619127,-62.5845560253671,
-234.837502470078));
#195789=CARTESIAN_POINT('Ctrl Pts',(-26.299935026532,-62.5618001346298,
-234.837570256781));
#195790=CARTESIAN_POINT('Ctrl Pts',(-26.4297212650746,-62.5040608637178,
-234.850690950979));
#195791=CARTESIAN_POINT('Ctrl Pts',(-26.4765766579827,-62.4804755152087,
-234.857183986946));
#195792=CARTESIAN_POINT('Ctrl Pts',(-26.5606263859936,-62.4392448432971,
-234.865676603548));
#195793=CARTESIAN_POINT('Ctrl Pts',(-26.598219218148,-62.4217260874495,
-234.867787528297));
#195794=CARTESIAN_POINT('Ctrl Pts',(-26.6712306199245,-62.3881303051001,
-234.871005091044));
#195795=CARTESIAN_POINT('Ctrl Pts',(-26.7062785831568,-62.3723269401802,
-234.871930575498));
#195796=CARTESIAN_POINT('Ctrl Pts',(-26.7576550280567,-62.3495221049909,
-234.872747949079));
#195797=CARTESIAN_POINT('Ctrl Pts',(-26.7745169875525,-62.3421733148585,
-234.872883709682));
#195798=CARTESIAN_POINT('Ctrl Pts',(-26.8139780721898,-62.3215114290266,
-234.876306139112));
#195799=CARTESIAN_POINT('Ctrl Pts',(-26.8364482204274,-62.3082529158846,
-234.8795305279));
#195800=CARTESIAN_POINT('Ctrl Pts',(-26.9497402120697,-62.2385292812946,
-234.896449373983));
#195801=CARTESIAN_POINT('Ctrl Pts',(-27.0252222584354,-62.1924330785486,
-234.902126572898));
#195802=CARTESIAN_POINT('Ctrl Pts',(-27.0930165135311,-62.1526330725429,
-234.905475377596));
#195803=CARTESIAN_POINT('Ctrl Pts',(-26.5926469327273,-61.2115127003622,
-235.35005));
#195804=CARTESIAN_POINT('Ctrl Pts',(-26.5307857619515,-61.2444027172302,
-235.35005));
#195805=CARTESIAN_POINT('Ctrl Pts',(-26.4686189787879,-61.276660497005,
-235.35005));
#195806=CARTESIAN_POINT('Ctrl Pts',(-26.4050352616636,-61.3058697511684,
-235.35005));
#195807=CARTESIAN_POINT('Ctrl Pts',(-26.3891387194065,-61.3131723462998,
-235.35005));
#195808=CARTESIAN_POINT('Ctrl Pts',(-26.3731446870696,-61.3202661956383,
-235.35005));
#195809=CARTESIAN_POINT('Ctrl Pts',(-26.3570986663275,-61.327248639717,
-235.35005));
#195810=CARTESIAN_POINT('Ctrl Pts',(-26.3410524626378,-61.3342311634055,
-235.35005));
#195811=CARTESIAN_POINT('Ctrl Pts',(-26.3249639130519,-61.3411229008801,
-235.35005));
#195812=CARTESIAN_POINT('Ctrl Pts',(-26.3088716457128,-61.3480064946411,
-235.35005));
#195813=CARTESIAN_POINT('Ctrl Pts',(-26.2766866901153,-61.3617738622147,
-235.35005));
#195814=CARTESIAN_POINT('Ctrl Pts',(-26.2444515824955,-61.3754400331407,
-235.35005));
#195815=CARTESIAN_POINT('Ctrl Pts',(-26.212121319506,-61.3888872080985,
-235.35005));
#195816=CARTESIAN_POINT('Ctrl Pts',(-26.1797907095899,-61.4023345273539,
-235.35005));
#195817=CARTESIAN_POINT('Ctrl Pts',(-26.1473794430666,-61.4155759233805,
-235.350049999999));
#195818=CARTESIAN_POINT('Ctrl Pts',(-26.1147800051491,-61.4283379724439,
-235.350049999999));
#195819=CARTESIAN_POINT('Ctrl Pts',(-26.0821804798061,-61.4411000557326,
-235.35005));
#195820=CARTESIAN_POINT('Ctrl Pts',(-26.0493313347784,-61.4532499920652,
-235.350050000001));
#195821=CARTESIAN_POINT('Ctrl Pts',(-26.0162730923146,-61.464811411177,
-235.350050000001));
#195822=CARTESIAN_POINT('Ctrl Pts',(-25.9501574057461,-61.4879339701914,
-235.350050000001));
#195823=CARTESIAN_POINT('Ctrl Pts',(-25.8834830443658,-61.5094189499966,
-235.35005));
#195824=CARTESIAN_POINT('Ctrl Pts',(-25.816441032895,-61.5296685975531,
-235.35005));
#195825=CARTESIAN_POINT('Ctrl Pts',(-25.799680801709,-61.5347309273823,
-235.35005));
#195826=CARTESIAN_POINT('Ctrl Pts',(-25.7828903692931,-61.5396829277202,
-235.35005));
#195827=CARTESIAN_POINT('Ctrl Pts',(-25.7660579441618,-61.5444815181131,
-235.35005));
#195828=CARTESIAN_POINT('Ctrl Pts',(-25.7492255222735,-61.5492801075815,
-235.35005));
#195829=CARTESIAN_POINT('Ctrl Pts',(-25.7323477287723,-61.5539129424998,
-235.35005));
#195830=CARTESIAN_POINT('Ctrl Pts',(-25.7154186680902,-61.558358482165,
-235.35005));
#195831=CARTESIAN_POINT('Ctrl Pts',(-25.6815605534858,-61.5672495597203,
-235.35005));
#195832=CARTESIAN_POINT('Ctrl Pts',(-25.6474983294595,-61.5754340306918,
-235.35005));
#195833=CARTESIAN_POINT('Ctrl Pts',(-25.6133395630491,-61.5831535528751,
-235.35005));
#195834=CARTESIAN_POINT('Ctrl Pts',(-25.5791808006497,-61.590873074152,
-235.35005));
#195835=CARTESIAN_POINT('Ctrl Pts',(-25.5449390551878,-61.5981934391817,
-235.35005));
#195836=CARTESIAN_POINT('Ctrl Pts',(-25.510599668782,-61.6050441261316,
-235.35005));
#195837=CARTESIAN_POINT('Ctrl Pts',(-25.4762602802774,-61.6118948135003,
-235.35005));
#195838=CARTESIAN_POINT('Ctrl Pts',(-25.4417936057802,-61.6182439572411,
-235.35005));
#195839=CARTESIAN_POINT('Ctrl Pts',(-25.4072553797815,-61.6238979002003,
-235.35005));
#195840=CARTESIAN_POINT('Ctrl Pts',(-25.3727171455055,-61.6295518445145,
-235.35005));
#195841=CARTESIAN_POINT('Ctrl Pts',(-25.3381059777677,-61.6345074541881,
-235.35005));
#195842=CARTESIAN_POINT('Ctrl Pts',(-25.3034405945236,-61.6389439122599,
-235.35005));
#195843=CARTESIAN_POINT('Ctrl Pts',(-25.2687751967828,-61.643380372187,
-235.35005));
#195844=CARTESIAN_POINT('Ctrl Pts',(-25.234056754758,-61.6473088938803,
-235.35005));
#195845=CARTESIAN_POINT('Ctrl Pts',(-25.1992961409817,-61.6508335460814,
-235.35005));
#195846=CARTESIAN_POINT('Ctrl Pts',(-25.1645355064627,-61.6543582003856,
-235.35005));
#195847=CARTESIAN_POINT('Ctrl Pts',(-25.1297211167782,-61.6573680815383,
-235.350050000001));
#195848=CARTESIAN_POINT('Ctrl Pts',(-25.0948355014582,-61.6596958899581,
-235.350050000001));
#195849=CARTESIAN_POINT('Ctrl Pts',(-25.0599498590945,-61.6620237001823,
-235.350050000001));
#195850=CARTESIAN_POINT('Ctrl Pts',(-25.0249976982331,-61.6637138708523,
-235.35005));
#195851=CARTESIAN_POINT('Ctrl Pts',(-24.9899997248189,-61.6649665253882,
-235.35005));
#195852=CARTESIAN_POINT('Ctrl Pts',(-24.9899997248189,-61.6649665253882,
-235.35005));
#195853=CARTESIAN_POINT('Ctrl Pts',(-25.0188032481045,-62.4697021984296,
-235.35005));
#195854=CARTESIAN_POINT('Ctrl Pts',(-25.0347190704499,-62.9143710634155,
-234.678897682318));
#195855=CARTESIAN_POINT('Ctrl Pts',(-23.5944744924679,-61.7149158997446,
-235.35005));
#195856=CARTESIAN_POINT('Ctrl Pts',(-23.6213321581707,-62.5206566084218,
-235.350050000019));
#195857=CARTESIAN_POINT('Ctrl Pts',(-23.6367128243542,-62.9652114948589,
-234.677688363322));
#195858=CARTESIAN_POINT('Ctrl Pts',(-22.1988114399884,-61.7606622187164,
-235.35005));
#195859=CARTESIAN_POINT('Ctrl Pts',(-22.2241440176947,-62.5673064456533,
-235.350049999981));
#195860=CARTESIAN_POINT('Ctrl Pts',(-22.2385723540716,-63.0117706699204,
-234.676581567471));
#195861=CARTESIAN_POINT('Ctrl Pts',(-20.8030114294341,-61.8022299494809,
-235.35005));
#195862=CARTESIAN_POINT('Ctrl Pts',(-20.8270581434285,-62.6096929286678,
-235.35005));
#195863=CARTESIAN_POINT('Ctrl Pts',(-20.8402921969906,-63.0540783161444,
-234.675571538939));
#195864=CARTESIAN_POINT('',(-20.8402919613448,-63.0540783782995,-234.675571450239));
#195865=CARTESIAN_POINT('',(-20.803011429434,-61.8022299494809,-235.35005));
#195866=CARTESIAN_POINT('Origin',(-20.803011429434,-61.802229949481,-233.85005));
#195867=CARTESIAN_POINT('Origin',(-0.0417395060045145,624.033047422002,
-250.70813398415));
#195868=CARTESIAN_POINT('Origin',(-0.0402464098217781,635.457880431084,
-235.35004999212));
#195869=CARTESIAN_POINT('Ctrl Pts',(-20.8103261415008,-61.8019857359798,
-235.350049999965));
#195870=CARTESIAN_POINT('Ctrl Pts',(-20.8379442866863,-62.6073572538772,
-235.350055531337));
#195871=CARTESIAN_POINT('Ctrl Pts',(-20.8531893512146,-63.0519698953505,
-234.678137626134));
#195872=CARTESIAN_POINT('Ctrl Pts',(-20.6414007909339,-61.8077587731983,
-235.350049999962));
#195873=CARTESIAN_POINT('Ctrl Pts',(-20.5833425691332,-62.6623713318805,
-235.350056095672));
#195874=CARTESIAN_POINT('Ctrl Pts',(-20.5552714958317,-63.1013208767041,
-234.619006716613));
#195875=CARTESIAN_POINT('Ctrl Pts',(-20.4749301547618,-61.7876897269827,
-235.350049999958));
#195876=CARTESIAN_POINT('Ctrl Pts',(-20.332371777071,-62.6832275069745,
-235.350056755447));
#195877=CARTESIAN_POINT('Ctrl Pts',(-20.2675410707633,-63.1041069278272,
-234.551887687313));
#195878=CARTESIAN_POINT('Ctrl Pts',(-20.3109688043558,-61.7477838180328,
-235.350049999954));
#195879=CARTESIAN_POINT('Ctrl Pts',(-20.0839608523746,-62.6801181224961,
-235.350057499857));
#195880=CARTESIAN_POINT('Ctrl Pts',(-19.9887981368535,-63.070968475606,
-234.478875287122));
#195881=CARTESIAN_POINT('',(-20.0008767707152,-63.0723812833681,-234.482033933863));
#195882=CARTESIAN_POINT('',(-20.3180691938068,-61.7495111937247,-235.35005));
#195883=CARTESIAN_POINT('Origin',(-20.3180691938068,-61.7495111937247,-233.85005));
#195884=CARTESIAN_POINT('Ctrl Pts',(-20.0008767707152,-63.0723812833681,
-234.482033933863));
#195885=CARTESIAN_POINT('Ctrl Pts',(-20.271823216313,-63.1035533395417,
-234.552772407528));
#195886=CARTESIAN_POINT('Ctrl Pts',(-20.5512619539194,-63.1007007148801,
-234.617924419256));
#195887=CARTESIAN_POINT('Ctrl Pts',(-20.8402919498871,-63.0540783560036,
-234.675571489654));
#195888=CARTESIAN_POINT('Ctrl Pts',(-20.803011429434,-61.8022299494809,
-235.35005));
#195889=CARTESIAN_POINT('Ctrl Pts',(-20.6389224043824,-61.8071166154417,
-235.35005));
#195890=CARTESIAN_POINT('Ctrl Pts',(-20.4774719299468,-61.7877321350851,
-235.35005));
#195891=CARTESIAN_POINT('Ctrl Pts',(-20.3180691938068,-61.7495111937247,
-235.35005));
#195892=CARTESIAN_POINT('Ctrl Pts',(-56.7978769236249,-64.9962486583172,
-213.25615446688));
#195893=CARTESIAN_POINT('Ctrl Pts',(-56.7746082597229,-64.9675904302956,
-215.348143273993));
#195894=CARTESIAN_POINT('Ctrl Pts',(-55.6596124147223,-63.9410622767582,
-216.790642532039));
#195895=CARTESIAN_POINT('Ctrl Pts',(-57.7238224635574,-63.9855135774691,
-213.252837709814));
#195896=CARTESIAN_POINT('Ctrl Pts',(-57.7003423852215,-63.9568776618465,
-215.347378844935));
#195897=CARTESIAN_POINT('Ctrl Pts',(-56.564654667179,-62.9482476744094,
-216.790318465523));
#195898=CARTESIAN_POINT('Ctrl Pts',(-58.6299194066539,-62.941827293528,
-213.246154460261));
#195899=CARTESIAN_POINT('Ctrl Pts',(-58.6117008786858,-62.9065844937392,
-215.346095403409));
#195900=CARTESIAN_POINT('Ctrl Pts',(-57.4569850683431,-61.9095456343501,
-216.789947871074));
#195901=CARTESIAN_POINT('Ctrl Pts',(-59.5017489787801,-61.8814728748856,
-213.239284157696));
#195902=CARTESIAN_POINT('Ctrl Pts',(-59.4805126951739,-61.8494200250926,
-215.345222444811));
#195903=CARTESIAN_POINT('Ctrl Pts',(-58.3016167962822,-60.8701016111416,
-216.790073419041));
#195904=CARTESIAN_POINT('',(-59.5017489787801,-61.8814728748856,-213.239284157696));
#195905=CARTESIAN_POINT('Ctrl Pts',(-56.8144552965909,-64.9781464054155,
-213.256094899172));
#195906=CARTESIAN_POINT('Ctrl Pts',(-57.7346379419056,-63.9730537814781,
-213.25275810317));
#195907=CARTESIAN_POINT('Ctrl Pts',(-58.6351232191172,-62.9354982011503,
-213.246113635462));
#195908=CARTESIAN_POINT('Ctrl Pts',(-59.5017489787801,-61.8814728748856,
-213.239284157696));
#195909=CARTESIAN_POINT('',(-58.3016167962821,-60.8701016111416,-216.790073419041));
#195910=CARTESIAN_POINT('Origin',(-55.6399013441494,-58.7068046741696,-213.15202212551));
#195911=CARTESIAN_POINT('Origin',(-1.94290616455451,-15.0706582410416,-217.44150863223));
#195912=CARTESIAN_POINT('Ctrl Pts',(-58.6463245735781,-60.4071924582901,
-216.811211134516));
#195913=CARTESIAN_POINT('Ctrl Pts',(-59.9794428890559,-61.1951119486122,
-215.368374394716));
#195914=CARTESIAN_POINT('Ctrl Pts',(-60.0946517248888,-61.0923008758321,
-213.257460793579));
#195915=CARTESIAN_POINT('Ctrl Pts',(-58.5374530973566,-60.5671124334838,
-216.797054630904));
#195916=CARTESIAN_POINT('Ctrl Pts',(-59.8200433378109,-61.420251027068,
-215.35259069506));
#195917=CARTESIAN_POINT('Ctrl Pts',(-59.9074639858675,-61.3655831923351,
-213.24427462457));
#195918=CARTESIAN_POINT('Ctrl Pts',(-58.4224878547923,-60.721351931509,
-216.7900913853));
#195919=CARTESIAN_POINT('Ctrl Pts',(-59.6536675829205,-61.6382804704421,
-215.344967772293));
#195920=CARTESIAN_POINT('Ctrl Pts',(-59.7097127443643,-61.6285208837113,
-213.238301674026));
#195921=CARTESIAN_POINT('Ctrl Pts',(-58.3016167962821,-60.8701016111416,
-216.790073419041));
#195922=CARTESIAN_POINT('Ctrl Pts',(-59.4805126951738,-61.8494200250926,
-215.345222444811));
#195923=CARTESIAN_POINT('Ctrl Pts',(-59.5017489787801,-61.8814728748855,
-213.239284157696));
#195924=CARTESIAN_POINT('',(-58.6463245735781,-60.4071924582901,-216.811211134516));
#195925=CARTESIAN_POINT('',(-60.094651724889,-61.0923008758319,-213.257460793579));
#195926=CARTESIAN_POINT('Origin',(-55.9721510687884,-58.2643380616866,-213.170198761392));
#195927=CARTESIAN_POINT('Origin',(-55.2663427916624,-58.4039463264878,-220.170489403551));
#195928=CARTESIAN_POINT('Origin',(-52.480669683245,-56.0916407951787,-217.694018753789));
#195929=CARTESIAN_POINT('Ctrl Pts',(-60.0946517248887,-61.0923008758322,
-213.257460793579));
#195930=CARTESIAN_POINT('Ctrl Pts',(-59.9794428890558,-61.1951119486123,
-215.368374394716));
#195931=CARTESIAN_POINT('Ctrl Pts',(-58.6463245735781,-60.4071924582901,
-216.811211134516));
#195932=CARTESIAN_POINT('Ctrl Pts',(-60.1704014750534,-60.9817110085918,
-213.262796876316));
#195933=CARTESIAN_POINT('Ctrl Pts',(-60.0526858896249,-61.0914110515479,
-215.370164057538));
#195934=CARTESIAN_POINT('Ctrl Pts',(-58.7107161648513,-60.3252040601318,
-216.812171008252));
#195935=CARTESIAN_POINT('Ctrl Pts',(-60.2441117511573,-60.869896564576,
-213.268474581372));
#195936=CARTESIAN_POINT('Ctrl Pts',(-60.124312865506,-60.986260523149,-215.371696130155));
#195937=CARTESIAN_POINT('Ctrl Pts',(-58.774689151411,-60.2421218021171,
-216.812772355214));
#195938=CARTESIAN_POINT('Ctrl Pts',(-60.3516186472783,-60.7003634878465,
-213.277642216535));
#195939=CARTESIAN_POINT('Ctrl Pts',(-60.2274858612712,-60.8293599818386,
-215.375374274252));
#195940=CARTESIAN_POINT('Ctrl Pts',(-58.8650026632788,-60.119575817198,
-216.814991469675));
#195941=CARTESIAN_POINT('Ctrl Pts',(-60.3869441313356,-60.6435508076619,
-213.280811345681));
#195942=CARTESIAN_POINT('Ctrl Pts',(-60.2611846671316,-60.7771794814514,
-215.376816670917));
#195943=CARTESIAN_POINT('Ctrl Pts',(-58.8942226240245,-60.0790466940644,
-216.81593623579));
#195944=CARTESIAN_POINT('Ctrl Pts',(-60.4565718022257,-60.5293282074256,
-213.287428511106));
#195945=CARTESIAN_POINT('Ctrl Pts',(-60.3271928115902,-60.6731602773773,
-215.380263890201));
#195946=CARTESIAN_POINT('Ctrl Pts',(-58.9507651838229,-59.99875439683,-216.818366528164));
#195947=CARTESIAN_POINT('Ctrl Pts',(-60.4908728037509,-60.4719198229617,
-213.290891213231));
#195948=CARTESIAN_POINT('Ctrl Pts',(-60.3592441835178,-60.6217751917873,
-215.382474260201));
#195949=CARTESIAN_POINT('Ctrl Pts',(-58.9774007039939,-59.9596050477392,
-216.820063085709));
#195950=CARTESIAN_POINT('Ctrl Pts',(-60.5922460955565,-60.2987937844743,
-213.301646644734));
#195951=CARTESIAN_POINT('Ctrl Pts',(-60.4575958918302,-60.4609801138041,
-215.386947861197));
#195952=CARTESIAN_POINT('Ctrl Pts',(-59.065516004555,-59.8335652392552,
-216.822864771484));
#195953=CARTESIAN_POINT('Ctrl Pts',(-60.6577989462613,-60.1821636194365,
-213.309190814844));
#195954=CARTESIAN_POINT('Ctrl Pts',(-60.524785077188,-60.3468286312902,
-215.387646798153));
#195955=CARTESIAN_POINT('Ctrl Pts',(-59.1321238001163,-59.7406787706502,
-216.822297086344));
#195956=CARTESIAN_POINT('Ctrl Pts',(-60.7848819389683,-59.9464002293958,
-213.324386876108));
#195957=CARTESIAN_POINT('Ctrl Pts',(-60.6548197305022,-60.1165130022809,
-215.388612783322));
#195958=CARTESIAN_POINT('Ctrl Pts',(-59.2620524978691,-59.5533695928239,
-216.820501321751));
#195959=CARTESIAN_POINT('Ctrl Pts',(-60.846408364668,-59.8272707790866,
-213.332077521835));
#195960=CARTESIAN_POINT('Ctrl Pts',(-60.717483170112,-60.0008089880217,
-215.389142461384));
#195961=CARTESIAN_POINT('Ctrl Pts',(-59.3247742637059,-59.4595472933127,
-216.819551739489));
#195962=CARTESIAN_POINT('Ctrl Pts',(-61.0248485991141,-59.4661777525867,
-213.356063148721));
#195963=CARTESIAN_POINT('Ctrl Pts',(-60.8960486551615,-59.6575831535381,
-215.394209213837));
#195964=CARTESIAN_POINT('Ctrl Pts',(-59.4988121913041,-59.1848780549995,
-216.820109150524));
#195965=CARTESIAN_POINT('Ctrl Pts',(-61.1355702178952,-59.2205125002381,
-213.373562975861));
#195966=CARTESIAN_POINT('Ctrl Pts',(-61.0052724474296,-59.4293377571138,
-215.400754444119));
#195967=CARTESIAN_POINT('Ctrl Pts',(-59.6026295906798,-59.0049501184268,
-216.82348683657));
#195968=CARTESIAN_POINT('Ctrl Pts',(-61.2879458897718,-58.8475849978711,
-213.4017996738));
#195969=CARTESIAN_POINT('Ctrl Pts',(-61.1609971430838,-59.0727673884097,
-215.407072797124));
#195970=CARTESIAN_POINT('Ctrl Pts',(-59.7633470952239,-58.7169241462467,
-216.824211264365));
#195971=CARTESIAN_POINT('Ctrl Pts',(-61.3365745411413,-58.7222537892455,
-213.411505588854));
#195972=CARTESIAN_POINT('Ctrl Pts',(-61.2121129425345,-58.9499342096063,
-215.407804375258));
#195973=CARTESIAN_POINT('Ctrl Pts',(-59.8197452350376,-58.6155814760437,
-216.822862462453));
#195974=CARTESIAN_POINT('Ctrl Pts',(-61.4291203581917,-58.4706258868742,
-213.431043252622));
#195975=CARTESIAN_POINT('Ctrl Pts',(-61.3093836883139,-58.7040108957773,
-215.409273509837));
#195976=CARTESIAN_POINT('Ctrl Pts',(-59.9282088629343,-58.4125887823326,
-216.819930966461));
#195977=CARTESIAN_POINT('Ctrl Pts',(-61.4730253185692,-58.3443774822963,
-213.440939227881));
#195978=CARTESIAN_POINT('Ctrl Pts',(-61.3551954026654,-58.5820063400323,
-215.410605991783));
#195979=CARTESIAN_POINT('Ctrl Pts',(-59.9789475628393,-58.3124784035116,
-216.819006081135));
#195980=CARTESIAN_POINT('Ctrl Pts',(-61.597714293997,-57.9644548462852,
-213.471381381521));
#195981=CARTESIAN_POINT('Ctrl Pts',(-61.4853747357745,-58.2167534861039,
-215.415702792428));
#195982=CARTESIAN_POINT('Ctrl Pts',(-60.1242796010941,-58.0129426112489,
-216.817104343704));
#195983=CARTESIAN_POINT('Ctrl Pts',(-61.6714754954506,-57.7096224302906,
-213.492744357615));
#195984=CARTESIAN_POINT('Ctrl Pts',(-61.5626827464202,-57.9741101500247,
-215.420785448757));
#195985=CARTESIAN_POINT('Ctrl Pts',(-60.2117828099091,-57.8147192880101,
-216.81725313496));
#195986=CARTESIAN_POINT('Ctrl Pts',(-61.800714404647,-57.1969944640406,
-213.537796166935));
#195987=CARTESIAN_POINT('Ctrl Pts',(-61.7018747842135,-57.4797917294326,
-215.428818601372));
#195988=CARTESIAN_POINT('Ctrl Pts',(-60.3818196482663,-57.4046185752289,
-216.814021419008));
#195989=CARTESIAN_POINT('Ctrl Pts',(-61.8562081200387,-56.939151684957,
-213.561315895465));
#195990=CARTESIAN_POINT('Ctrl Pts',(-61.7636709827336,-57.2277557399495,
-215.431290276296));
#195991=CARTESIAN_POINT('Ctrl Pts',(-60.4646332997325,-57.1919561113795,
-216.810066154251));
#195992=CARTESIAN_POINT('Ctrl Pts',(-61.9491342563485,-56.4203496751014,
-213.610036002534));
#195993=CARTESIAN_POINT('Ctrl Pts',(-61.869519178268,-56.7212110326965,
-215.436505159072));
#195994=CARTESIAN_POINT('Ctrl Pts',(-60.6164006800181,-56.7621465040705,
-216.801040019797));
#195995=CARTESIAN_POINT('Ctrl Pts',(-61.9865582056648,-56.1594017177566,
-213.635279158387));
#195996=CARTESIAN_POINT('Ctrl Pts',(-61.9133916888105,-56.468424334395,
-215.440252708081));
#195997=CARTESIAN_POINT('Ctrl Pts',(-60.6835863552341,-56.54770132465,-216.797176937873));
#195998=CARTESIAN_POINT('Ctrl Pts',(-62.0431863828312,-55.6347775839173,
-213.688884450398));
#195999=CARTESIAN_POINT('Ctrl Pts',(-61.9838074416176,-55.9626753631027,
-215.450801296784));
#196000=CARTESIAN_POINT('Ctrl Pts',(-60.8026418999236,-56.1177717712389,
-216.79143672755));
#196001=CARTESIAN_POINT('Ctrl Pts',(-62.0623954799918,-55.3711251235972,
-213.717367123901));
#196002=CARTESIAN_POINT('Ctrl Pts',(-62.0107144541483,-55.7085961605345,
-215.45590742182));
#196003=CARTESIAN_POINT('Ctrl Pts',(-60.8571508863725,-55.9007000271699,
-216.787671355125));
#196004=CARTESIAN_POINT('Ctrl Pts',(-62.0723653519315,-55.1059089910526,
-213.746749287635));
#196005=CARTESIAN_POINT('Ctrl Pts',(-62.0291783705537,-55.4425764560866,
-215.457214771211));
#196006=CARTESIAN_POINT('Ctrl Pts',(-60.911917075676,-55.663399014185,-216.777770284882));
#196007=CARTESIAN_POINT('',(-60.9119170756758,-55.6633990141858,-216.777770284882));
#196008=CARTESIAN_POINT('',(-62.0723653519316,-55.1059089910534,-213.746749287634));
#196009=CARTESIAN_POINT('Origin',(-57.0770276271036,-54.9084593705222,-213.659487255448));
#196010=CARTESIAN_POINT('Ctrl Pts',(-60.9119170756758,-55.6633990141858,
-216.777770284882));
#196011=CARTESIAN_POINT('Ctrl Pts',(-60.8571508863725,-55.9007000271699,
-216.787671355125));
#196012=CARTESIAN_POINT('Ctrl Pts',(-60.8026418999236,-56.1177717712389,
-216.79143672755));
#196013=CARTESIAN_POINT('Ctrl Pts',(-60.6835863552341,-56.54770132465,-216.797176937873));
#196014=CARTESIAN_POINT('Ctrl Pts',(-60.6164006800181,-56.7621465040705,
-216.801040019797));
#196015=CARTESIAN_POINT('Ctrl Pts',(-60.4646332997325,-57.1919561113795,
-216.810066154251));
#196016=CARTESIAN_POINT('Ctrl Pts',(-60.3818196482663,-57.4046185752289,
-216.814021419008));
#196017=CARTESIAN_POINT('Ctrl Pts',(-60.2117828099091,-57.8147192880101,
-216.81725313496));
#196018=CARTESIAN_POINT('Ctrl Pts',(-60.1242796010941,-58.0129426112489,
-216.817104343704));
#196019=CARTESIAN_POINT('Ctrl Pts',(-59.9789475628393,-58.3124784035116,
-216.819006081135));
#196020=CARTESIAN_POINT('Ctrl Pts',(-59.9282088629343,-58.4125887823326,
-216.819930966461));
#196021=CARTESIAN_POINT('Ctrl Pts',(-59.8197452350376,-58.6155814760437,
-216.822862462453));
#196022=CARTESIAN_POINT('Ctrl Pts',(-59.7633470952239,-58.7169241462467,
-216.824211264365));
#196023=CARTESIAN_POINT('Ctrl Pts',(-59.6026295906798,-59.0049501184268,
-216.82348683657));
#196024=CARTESIAN_POINT('Ctrl Pts',(-59.4988121913041,-59.1848780549995,
-216.820109150524));
#196025=CARTESIAN_POINT('Ctrl Pts',(-59.3247742637059,-59.4595472933127,
-216.819551739489));
#196026=CARTESIAN_POINT('Ctrl Pts',(-59.2620524978691,-59.5533695928239,
-216.820501321751));
#196027=CARTESIAN_POINT('Ctrl Pts',(-59.1321238001163,-59.7406787706502,
-216.822297086344));
#196028=CARTESIAN_POINT('Ctrl Pts',(-59.065516004555,-59.8335652392552,
-216.822864771484));
#196029=CARTESIAN_POINT('Ctrl Pts',(-58.9774007039939,-59.9596050477392,
-216.820063085709));
#196030=CARTESIAN_POINT('Ctrl Pts',(-58.9507651838229,-59.99875439683,-216.818366528164));
#196031=CARTESIAN_POINT('Ctrl Pts',(-58.8942226240245,-60.0790466940644,
-216.81593623579));
#196032=CARTESIAN_POINT('Ctrl Pts',(-58.8650026632788,-60.119575817198,
-216.814991469675));
#196033=CARTESIAN_POINT('Ctrl Pts',(-58.774689151411,-60.2421218021171,
-216.812772355214));
#196034=CARTESIAN_POINT('Ctrl Pts',(-58.7107161648513,-60.3252040601318,
-216.812171008252));
#196035=CARTESIAN_POINT('Ctrl Pts',(-58.6463245735781,-60.4071924582901,
-216.811211134516));
#196036=CARTESIAN_POINT('Ctrl Pts',(-60.094651724889,-61.0923008758319,
-213.257460793579));
#196037=CARTESIAN_POINT('Ctrl Pts',(-60.1704014750534,-60.9817110085918,
-213.262796876316));
#196038=CARTESIAN_POINT('Ctrl Pts',(-60.2441117511573,-60.869896564576,
-213.268474581372));
#196039=CARTESIAN_POINT('Ctrl Pts',(-60.3516186472783,-60.7003634878465,
-213.277642216535));
#196040=CARTESIAN_POINT('Ctrl Pts',(-60.3869441313356,-60.6435508076619,
-213.280811345681));
#196041=CARTESIAN_POINT('Ctrl Pts',(-60.4565718022257,-60.5293282074256,
-213.287428511106));
#196042=CARTESIAN_POINT('Ctrl Pts',(-60.4908728037509,-60.4719198229617,
-213.290891213231));
#196043=CARTESIAN_POINT('Ctrl Pts',(-60.5922460955565,-60.2987937844743,
-213.301646644734));
#196044=CARTESIAN_POINT('Ctrl Pts',(-60.6577989462613,-60.1821636194365,
-213.309190814844));
#196045=CARTESIAN_POINT('Ctrl Pts',(-60.7848819389683,-59.9464002293958,
-213.324386876108));
#196046=CARTESIAN_POINT('Ctrl Pts',(-60.846408364668,-59.8272707790866,
-213.332077521835));
#196047=CARTESIAN_POINT('Ctrl Pts',(-61.0248485991141,-59.4661777525867,
-213.356063148721));
#196048=CARTESIAN_POINT('Ctrl Pts',(-61.1355702178952,-59.2205125002381,
-213.373562975861));
#196049=CARTESIAN_POINT('Ctrl Pts',(-61.2879458897718,-58.8475849978711,
-213.4017996738));
#196050=CARTESIAN_POINT('Ctrl Pts',(-61.3365745411413,-58.7222537892455,
-213.411505588854));
#196051=CARTESIAN_POINT('Ctrl Pts',(-61.4291203581917,-58.4706258868742,
-213.431043252622));
#196052=CARTESIAN_POINT('Ctrl Pts',(-61.4730253185692,-58.3443774822963,
-213.440939227881));
#196053=CARTESIAN_POINT('Ctrl Pts',(-61.597714293997,-57.9644548462852,
-213.471381381521));
#196054=CARTESIAN_POINT('Ctrl Pts',(-61.6714754954506,-57.7096224302906,
-213.492744357615));
#196055=CARTESIAN_POINT('Ctrl Pts',(-61.800714404647,-57.1969944640406,
-213.537796166935));
#196056=CARTESIAN_POINT('Ctrl Pts',(-61.8562081200387,-56.939151684957,
-213.561315895465));
#196057=CARTESIAN_POINT('Ctrl Pts',(-61.9491342563485,-56.4203496751014,
-213.610036002534));
#196058=CARTESIAN_POINT('Ctrl Pts',(-61.9865582056648,-56.1594017177566,
-213.635279158387));
#196059=CARTESIAN_POINT('Ctrl Pts',(-62.0431863828312,-55.6347775839173,
-213.688884450398));
#196060=CARTESIAN_POINT('Ctrl Pts',(-62.0623954799918,-55.3711251235972,
-213.717367123901));
#196061=CARTESIAN_POINT('Ctrl Pts',(-62.0723653519316,-55.1059089910534,
-213.746749287634));
#196062=CARTESIAN_POINT('Ctrl Pts',(-61.2313176176751,-54.1392424392483,
-216.589725631894));
#196063=CARTESIAN_POINT('Ctrl Pts',(-62.0809182617279,-54.1703109655338,
-215.350650293751));
#196064=CARTESIAN_POINT('Ctrl Pts',(-62.1072060041624,-54.1692103455255,
-213.848185004792));
#196065=CARTESIAN_POINT('Ctrl Pts',(-61.2063940314189,-54.2739747051073,
-216.618254256554));
#196066=CARTESIAN_POINT('Ctrl Pts',(-62.0763273182448,-54.2805873286282,
-215.369481660389));
#196067=CARTESIAN_POINT('Ctrl Pts',(-62.1041253019867,-54.2489750153891,
-213.848073204958));
#196068=CARTESIAN_POINT('Ctrl Pts',(-61.1772202905008,-54.4149797409396,
-216.647503745936));
#196069=CARTESIAN_POINT('Ctrl Pts',(-62.0715862894379,-54.394279767702,
-215.38841245438));
#196070=CARTESIAN_POINT('Ctrl Pts',(-62.1010994294235,-54.3282171953391,
-213.845465532169));
#196071=CARTESIAN_POINT('Ctrl Pts',(-61.1205413775905,-54.685792621321,
-216.694769237218));
#196072=CARTESIAN_POINT('Ctrl Pts',(-62.062453045182,-54.6155354879892,
-215.418086549984));
#196073=CARTESIAN_POINT('Ctrl Pts',(-62.0951493333573,-54.4857552569525,
-213.83553633607));
#196074=CARTESIAN_POINT('Ctrl Pts',(-61.0934782087293,-54.8149371689336,
-216.712721476424));
#196075=CARTESIAN_POINT('Ctrl Pts',(-62.058078131037,-54.7227047882016,
-215.428743044064));
#196076=CARTESIAN_POINT('Ctrl Pts',(-62.0922232746451,-54.5640610712258,
-213.828298048155));
#196077=CARTESIAN_POINT('Ctrl Pts',(-61.0165420227469,-55.1872292058749,
-216.753620691064));
#196078=CARTESIAN_POINT('Ctrl Pts',(-62.0453942577027,-55.0361844349794,
-215.450995476348));
#196079=CARTESIAN_POINT('Ctrl Pts',(-62.0835491986123,-54.7979388895741,
-213.801481239476));
#196080=CARTESIAN_POINT('Ctrl Pts',(-60.9675295053391,-55.4224312521647,
-216.767716225312));
#196081=CARTESIAN_POINT('Ctrl Pts',(-62.0373485839771,-55.237798506958,
-215.455648829851));
#196082=CARTESIAN_POINT('Ctrl Pts',(-62.0779017065461,-54.9524994590213,
-213.77694217629));
#196083=CARTESIAN_POINT('Ctrl Pts',(-60.9119170756759,-55.6633990141857,
-216.777770284882));
#196084=CARTESIAN_POINT('Ctrl Pts',(-62.0291783705539,-55.4425764560874,
-215.457214771212));
#196085=CARTESIAN_POINT('Ctrl Pts',(-62.0723653519316,-55.1059089910533,
-213.746749287634));
#196086=CARTESIAN_POINT('',(-61.2313176176752,-54.1392424392486,-216.589725631893));
#196087=CARTESIAN_POINT('',(-62.1072060041622,-54.1692103455281,-213.848185004792));
#196088=CARTESIAN_POINT('Origin',(-57.1116967348753,-53.976149530741,-213.760922972606));
#196089=CARTESIAN_POINT('Ctrl Pts',(-61.2313176176752,-54.1392424392486,
-216.589725631893));
#196090=CARTESIAN_POINT('Ctrl Pts',(-61.2241039156532,-54.1782415195011,
-216.597982568441));
#196091=CARTESIAN_POINT('Ctrl Pts',(-61.2128225788744,-54.2380631026322,
-216.610636660612));
#196092=CARTESIAN_POINT('Ctrl Pts',(-61.1926443983631,-54.3394047229831,
-216.63095046008));
#196093=CARTESIAN_POINT('Ctrl Pts',(-61.1881937267781,-54.361555288859,
-216.635330103797));
#196094=CARTESIAN_POINT('Ctrl Pts',(-61.1800246564408,-54.4018751062487,
-216.643185612872));
#196095=CARTESIAN_POINT('Ctrl Pts',(-61.1761441785378,-54.4208709408331,
-216.646828561234));
#196096=CARTESIAN_POINT('Ctrl Pts',(-61.1651728277633,-54.4743055729631,
-216.65692461498));
#196097=CARTESIAN_POINT('Ctrl Pts',(-61.1587578593242,-54.5051808903392,
-216.66254143341));
#196098=CARTESIAN_POINT('Ctrl Pts',(-61.1478391319696,-54.5574987649835,
-216.671816784675));
#196099=CARTESIAN_POINT('Ctrl Pts',(-61.1438644307081,-54.576427809643,
-216.675098825188));
#196100=CARTESIAN_POINT('Ctrl Pts',(-61.1344526503841,-54.621125696205,
-216.682563391224));
#196101=CARTESIAN_POINT('Ctrl Pts',(-61.1309617856826,-54.6376829199064,
-216.685279573515));
#196102=CARTESIAN_POINT('Ctrl Pts',(-61.1252140310211,-54.6649222567372,
-216.68962143623));
#196103=CARTESIAN_POINT('Ctrl Pts',(-61.1235283000098,-54.6729072328791,
-216.690884505207));
#196104=CARTESIAN_POINT('Ctrl Pts',(-61.118185976056,-54.6982145931637,
-216.694798416799));
#196105=CARTESIAN_POINT('Ctrl Pts',(-61.1157556494703,-54.7097314783994,
-216.69653968148));
#196106=CARTESIAN_POINT('Ctrl Pts',(-61.1091703270707,-54.7409497931566,
-216.701186611476));
#196107=CARTESIAN_POINT('Ctrl Pts',(-61.1057199535694,-54.75732388421,-216.703519943178));
#196108=CARTESIAN_POINT('Ctrl Pts',(-61.1006329227755,-54.7814840900207,
-216.706914183641));
#196109=CARTESIAN_POINT('Ctrl Pts',(-61.0994351791443,-54.7871763864764,
-216.707691861462));
#196110=CARTESIAN_POINT('Ctrl Pts',(-61.0950260074423,-54.8082043156478,
-216.710539837749));
#196111=CARTESIAN_POINT('Ctrl Pts',(-61.0901727033295,-54.8314262316928,
-216.713633471544));
#196112=CARTESIAN_POINT('Ctrl Pts',(-61.0768562795503,-54.8954423983165,
-216.721485807188));
#196113=CARTESIAN_POINT('Ctrl Pts',(-61.0684423125124,-54.9361308500724,
-216.726184275623));
#196114=CARTESIAN_POINT('Ctrl Pts',(-61.0570157190733,-54.9913415509466,
-216.73193045932));
#196115=CARTESIAN_POINT('Ctrl Pts',(-61.0557184685048,-54.9976077539097,
-216.732575505159));
#196116=CARTESIAN_POINT('Ctrl Pts',(-61.0530686957251,-55.010402144142,
-216.733876911098));
#196117=CARTESIAN_POINT('Ctrl Pts',(-61.0524981665959,-55.0131555164942,
-216.734152799324));
#196118=CARTESIAN_POINT('Ctrl Pts',(-61.0465955441629,-55.0416386881539,
-216.737003562727));
#196119=CARTESIAN_POINT('Ctrl Pts',(-61.0011802341201,-55.2603871152587,
-216.757910091499));
#196120=CARTESIAN_POINT('Ctrl Pts',(-60.9561319024597,-55.4718168818616,
-216.769776775062));
#196121=CARTESIAN_POINT('Ctrl Pts',(-60.9119170756758,-55.6633990141858,
-216.777770284882));
#196122=CARTESIAN_POINT('Ctrl Pts',(-62.0723653519316,-55.1059089910533,
-213.746749287634));
#196123=CARTESIAN_POINT('Ctrl Pts',(-62.0768793934835,-54.9808272269194,
-213.771366922062));
#196124=CARTESIAN_POINT('Ctrl Pts',(-62.0814562559514,-54.8552883758853,
-213.792161075494));
#196125=CARTESIAN_POINT('Ctrl Pts',(-62.0861030190532,-54.7293175792547,
-213.808641588779));
#196126=CARTESIAN_POINT('Ctrl Pts',(-62.0871755723782,-54.7002413397708,
-213.812445576401));
#196127=CARTESIAN_POINT('Ctrl Pts',(-62.0882518451934,-54.6711421311991,
-213.816019960739));
#196128=CARTESIAN_POINT('Ctrl Pts',(-62.0893319159675,-54.6420203440086,
-213.819359111929));
#196129=CARTESIAN_POINT('Ctrl Pts',(-62.0922302587963,-54.5638727585977,
-213.828319640385));
#196130=CARTESIAN_POINT('Ctrl Pts',(-62.0951568916024,-54.485555140642,
-213.835548948857));
#196131=CARTESIAN_POINT('Ctrl Pts',(-62.0981243813904,-54.4069862261458,
-213.840500934119));
#196132=CARTESIAN_POINT('Ctrl Pts',(-62.1011078230663,-54.327994960571,
-213.845479539022));
#196133=CARTESIAN_POINT('Ctrl Pts',(-62.10413438511,-54.2487398377294,-213.848073534587));
#196134=CARTESIAN_POINT('Ctrl Pts',(-62.1072060041623,-54.1692103455281,
-213.848185004792));
#196135=CARTESIAN_POINT('Ctrl Pts',(-62.1072060041624,-54.1692103455281,
-213.848185004792));
#196136=CARTESIAN_POINT('Ctrl Pts',(-62.080918261728,-54.1703109655354,
-215.35065029375));
#196137=CARTESIAN_POINT('Ctrl Pts',(-61.2313176176758,-54.1392424392492,
-216.589725631893));
#196138=CARTESIAN_POINT('Ctrl Pts',(-62.2073146990343,-51.5772242306456,
-213.851818178108));
#196139=CARTESIAN_POINT('Ctrl Pts',(-62.1810780798828,-51.5788094394115,
-215.350579261556));
#196140=CARTESIAN_POINT('Ctrl Pts',(-61.3352033241752,-51.5493321211721,
-216.587755286117));
#196141=CARTESIAN_POINT('Ctrl Pts',(-62.2979780119689,-48.9848138223874,
-213.855140923934));
#196142=CARTESIAN_POINT('Ctrl Pts',(-62.2718155003498,-48.9862078816536,
-215.350513478475));
#196143=CARTESIAN_POINT('Ctrl Pts',(-61.4293178843156,-48.9588621990226,
-216.585940879345));
#196144=CARTESIAN_POINT('Ctrl Pts',(-62.3791894693652,-46.3921971636372,
-213.85810601718));
#196145=CARTESIAN_POINT('Ctrl Pts',(-62.3531001006731,-46.3930946875274,
-215.350420378609));
#196146=CARTESIAN_POINT('Ctrl Pts',(-61.5136373793521,-46.3682170785133,
-216.584262774589));
#196147=CARTESIAN_POINT('',(-61.744621222757,-46.4961938535833,-216.203488008845));
#196148=CARTESIAN_POINT('',(-62.3685684251148,-46.7295482205574,-213.857736690702));
#196149=CARTESIAN_POINT('Ctrl Pts',(-61.744621222757,-46.4961938535833,
-216.203488008845));
#196150=CARTESIAN_POINT('Ctrl Pts',(-61.9444015485133,-46.53632319838,-215.842641422324));
#196151=CARTESIAN_POINT('Ctrl Pts',(-62.0956418404579,-46.575986655544,
-215.465343832456));
#196152=CARTESIAN_POINT('Ctrl Pts',(-62.3051774478038,-46.6542220635401,
-214.679483825453));
#196153=CARTESIAN_POINT('Ctrl Pts',(-62.3625672140424,-46.6930523819976,
-214.267454208411));
#196154=CARTESIAN_POINT('Ctrl Pts',(-62.3685683162547,-46.7295549501427,
-213.857737288663));
#196155=CARTESIAN_POINT('',(-61.5121276274155,-46.4145707938183,-216.584292819094));
#196156=CARTESIAN_POINT('Ctrl Pts',(-61.5121276273779,-46.414570793914,
-216.584292819144));
#196157=CARTESIAN_POINT('Ctrl Pts',(-61.5887158305549,-46.4514128718707,
-216.470096233485));
#196158=CARTESIAN_POINT('Ctrl Pts',(-61.6670075359489,-46.4806037630794,
-216.343675158136));
#196159=CARTESIAN_POINT('Ctrl Pts',(-61.744621222757,-46.4961938535833,
-216.203488008845));
#196160=CARTESIAN_POINT('Origin',(967.127514096642,-12.8777453687604,-231.930774818293));
#196161=CARTESIAN_POINT('Origin',(1003.27568749664,-12.9672887026865,-175.207747633911));
#196162=CARTESIAN_POINT('Ctrl Pts',(-61.5121276273784,-46.4145707939176,
-216.584292819143));
#196163=CARTESIAN_POINT('Ctrl Pts',(-61.6347030716742,-46.0974912749705,
-216.419279621934));
#196164=CARTESIAN_POINT('Ctrl Pts',(-61.6760242364037,-45.7878268313144,
-216.206690793879));
#196165=CARTESIAN_POINT('Ctrl Pts',(-61.5887158305549,-46.4514128718707,
-216.470096233485));
#196166=CARTESIAN_POINT('Ctrl Pts',(-61.683502987622,-46.1340834295878,
-216.336103167041));
#196167=CARTESIAN_POINT('Ctrl Pts',(-61.705984565682,-45.8233265979214,
-216.161095232372));
#196168=CARTESIAN_POINT('Ctrl Pts',(-61.6670075359489,-46.4806037630794,
-216.343675158136));
#196169=CARTESIAN_POINT('Ctrl Pts',(-61.734382175831,-46.1635375612304,
-216.245336224123));
#196170=CARTESIAN_POINT('Ctrl Pts',(-61.7366373868477,-45.8522624046448,
-216.111341099556));
#196171=CARTESIAN_POINT('Ctrl Pts',(-61.7446212227572,-46.4961938535835,
-216.203488008845));
#196172=CARTESIAN_POINT('Ctrl Pts',(-61.7864942538559,-46.180062496681,
-216.146540979352));
#196173=CARTESIAN_POINT('Ctrl Pts',(-61.7670197730424,-45.8692809645531,
-216.057260894206));
#196174=CARTESIAN_POINT('',(-61.7670229802613,-45.8692803056811,-216.057262488689));
#196175=CARTESIAN_POINT('',(-61.6760242364037,-45.7878268313144,-216.206690793879));
#196176=CARTESIAN_POINT('Ctrl Pts',(-61.7670197730424,-45.8692809645531,
-216.057260894206));
#196177=CARTESIAN_POINT('Ctrl Pts',(-61.7550845759282,-45.8625955281523,
-216.078505376257));
#196178=CARTESIAN_POINT('Ctrl Pts',(-61.7431797205979,-45.8541157626504,
-216.09895572827));
#196179=CARTESIAN_POINT('Ctrl Pts',(-61.7313327668648,-45.8441875369102,
-216.118692873593));
#196180=CARTESIAN_POINT('Ctrl Pts',(-61.7181196244691,-45.8331143898888,
-216.140706103113));
#196181=CARTESIAN_POINT('Ctrl Pts',(-61.7049782693999,-45.8202388887419,
-216.161832421571));
#196182=CARTESIAN_POINT('Ctrl Pts',(-61.691944049084,-45.8059771350208,
-216.18216400124));
#196183=CARTESIAN_POINT('Ctrl Pts',(-61.6866187518076,-45.8001503132848,
-216.190470727935));
#196184=CARTESIAN_POINT('Ctrl Pts',(-61.6813113292403,-45.7940914674599,
-216.198644554988));
#196185=CARTESIAN_POINT('Ctrl Pts',(-61.6760242364037,-45.7878268313144,
-216.206690793879));
#196186=CARTESIAN_POINT('Origin',(-59.0334256450291,-46.3348777618666,-214.896191665971));
#196187=CARTESIAN_POINT('Origin',(-59.1250215884199,-46.412156871143,-214.743818340268));
#196188=CARTESIAN_POINT('Ctrl Pts',(-61.744621222757,-46.4961938535834,
-216.203488008845));
#196189=CARTESIAN_POINT('Ctrl Pts',(-61.7864942538559,-46.1800624966811,
-216.146540979352));
#196190=CARTESIAN_POINT('Ctrl Pts',(-61.7670197730426,-45.8692809645531,
-216.057260894206));
#196191=CARTESIAN_POINT('Ctrl Pts',(-61.9444015484922,-46.5363231985591,
-215.842641422359));
#196192=CARTESIAN_POINT('Ctrl Pts',(-61.9754348687076,-46.2721634433876,
-215.791058678043));
#196193=CARTESIAN_POINT('Ctrl Pts',(-61.9631621369174,-46.0106807568515,
-215.721163036308));
#196194=CARTESIAN_POINT('Ctrl Pts',(-62.0956418404433,-46.5759866556878,
-215.465343832486));
#196195=CARTESIAN_POINT('Ctrl Pts',(-62.1171497321372,-46.3642951884269,
-215.421651993854));
#196196=CARTESIAN_POINT('Ctrl Pts',(-62.1106980495454,-46.1537572969976,
-215.368567684276));
#196197=CARTESIAN_POINT('Ctrl Pts',(-62.3051790602976,-46.6542226656792,
-214.679477777819));
#196198=CARTESIAN_POINT('Ctrl Pts',(-62.3119048875977,-46.5481874588022,
-214.656051542736));
#196199=CARTESIAN_POINT('Ctrl Pts',(-62.3127271221,-46.4421422876624,-214.631724106531));
#196200=CARTESIAN_POINT('Ctrl Pts',(-62.3625689806341,-46.6930535773299,
-214.267441525086));
#196201=CARTESIAN_POINT('Ctrl Pts',(-62.3644265280729,-46.6408054190759,
-214.25579858017));
#196202=CARTESIAN_POINT('Ctrl Pts',(-62.3662837353377,-46.5885519083916,
-214.24418481767));
#196203=CARTESIAN_POINT('Ctrl Pts',(-62.3685685933127,-46.7295566356152,
-213.857718370431));
#196204=CARTESIAN_POINT('Ctrl Pts',(-62.3685685933127,-46.7295566356152,
-213.857718370431));
#196205=CARTESIAN_POINT('Ctrl Pts',(-62.3685685933127,-46.7295566356152,
-213.857718370431));
#196206=CARTESIAN_POINT('Ctrl Pts',(-61.7670197730478,-45.8692809645569,
-216.057260894197));
#196207=CARTESIAN_POINT('Ctrl Pts',(-61.7860307089207,-45.8829860222033,
-216.024684888233));
#196208=CARTESIAN_POINT('Ctrl Pts',(-61.8063428741164,-45.8979710373087,
-215.988950140515));
#196209=CARTESIAN_POINT('Ctrl Pts',(-61.8277026039749,-45.914260388285,
-215.949926047446));
#196210=CARTESIAN_POINT('Ctrl Pts',(-61.8490085554087,-45.9305087267746,
-215.911000207224));
#196211=CARTESIAN_POINT('Ctrl Pts',(-61.8713568284104,-45.9480548595732,
-215.86880157429));
#196212=CARTESIAN_POINT('Ctrl Pts',(-61.8944466268228,-45.9669239189239,
-215.823183826969));
#196213=CARTESIAN_POINT('Ctrl Pts',(-61.9174819143512,-45.9857484318006,
-215.777673774989));
#196214=CARTESIAN_POINT('Ctrl Pts',(-61.9412552413371,-46.0058896543611,
-215.728760738867));
#196215=CARTESIAN_POINT('Ctrl Pts',(-61.9654187894528,-46.0273731743951,
-215.676282670045));
#196216=CARTESIAN_POINT('Ctrl Pts',(-61.9707824231834,-46.0321419166408,
-215.664634002444));
#196217=CARTESIAN_POINT('Ctrl Pts',(-61.9761650911893,-46.0369767977574,
-215.652809614194));
#196218=CARTESIAN_POINT('Ctrl Pts',(-61.9815626594367,-46.0418781000279,
-215.640807620315));
#196219=CARTESIAN_POINT('Ctrl Pts',(-62.0078995976887,-46.0657935540502,
-215.582244994109));
#196220=CARTESIAN_POINT('Ctrl Pts',(-62.0345910813097,-46.0912866876058,
-215.519464379018));
#196221=CARTESIAN_POINT('Ctrl Pts',(-62.0610868871434,-46.1183546518921,
-215.452322901564));
#196222=CARTESIAN_POINT('Ctrl Pts',(-62.0786458767962,-46.1362928156833,
-215.407827689179));
#196223=CARTESIAN_POINT('Ctrl Pts',(-62.0961186585576,-46.1549235122947,
-215.361414642324));
#196224=CARTESIAN_POINT('Ctrl Pts',(-62.1133307833226,-46.1742425534407,
-215.31304610448));
#196225=CARTESIAN_POINT('Ctrl Pts',(-62.128223696963,-46.1909584914978,
-215.271194882341));
#196226=CARTESIAN_POINT('Ctrl Pts',(-62.1429202037568,-46.208188641063,
-215.227882394232));
#196227=CARTESIAN_POINT('Ctrl Pts',(-62.1573003639315,-46.2259262935355,
-215.183092496691));
#196228=CARTESIAN_POINT('Ctrl Pts',(-62.1661086492019,-46.2367911449076,
-215.155657322814));
#196229=CARTESIAN_POINT('Ctrl Pts',(-62.1749359514523,-46.2480214779255,
-215.127224607864));
#196230=CARTESIAN_POINT('Ctrl Pts',(-62.1835512608191,-46.2593673508619,
-215.09841714778));
#196231=CARTESIAN_POINT('Ctrl Pts',(-62.192090487231,-46.2706130268697,
-215.069864090247));
#196232=CARTESIAN_POINT('Ctrl Pts',(-62.2004213907544,-46.2819722055932,
-215.04094285704));
#196233=CARTESIAN_POINT('Ctrl Pts',(-62.2083681674017,-46.2932002549787,
-215.012276600892));
#196234=CARTESIAN_POINT('Ctrl Pts',(-62.2094184292088,-46.2946841763169,
-215.008488011465));
#196235=CARTESIAN_POINT('Ctrl Pts',(-62.2104620521714,-46.2961658055334,
-215.004703899692));
#196236=CARTESIAN_POINT('Ctrl Pts',(-62.2114986946153,-46.2976445763721,
-215.000925725915));
#196237=CARTESIAN_POINT('Ctrl Pts',(-62.2115700245438,-46.2977463285421,
-215.000665755019));
#196238=CARTESIAN_POINT('Ctrl Pts',(-62.2116413216157,-46.297848067624,
-215.000405811611));
#196239=CARTESIAN_POINT('Ctrl Pts',(-62.2117125858462,-46.2979497936101,
-215.000145895713));
#196240=CARTESIAN_POINT('Ctrl Pts',(-62.2298446813421,-46.3238324177585,
-214.934014263643));
#196241=CARTESIAN_POINT('Ctrl Pts',(-62.2458179332301,-46.3489008751118,
-214.869560714848));
#196242=CARTESIAN_POINT('Ctrl Pts',(-62.2598734755854,-46.3729950016063,
-214.807262372277));
#196243=CARTESIAN_POINT('Ctrl Pts',(-62.2741714237111,-46.3975046620692,
-214.743889615262));
#196244=CARTESIAN_POINT('Ctrl Pts',(-62.2864855615421,-46.4210061172213,
-214.682747266005));
#196245=CARTESIAN_POINT('Ctrl Pts',(-62.297096987798,-46.4433539938431,
-214.624295756784));
#196246=CARTESIAN_POINT('Ctrl Pts',(-62.3081336004919,-46.4665973216352,
-214.563502169468));
#196247=CARTESIAN_POINT('Ctrl Pts',(-62.3173291366072,-46.4885928399262,
-214.505619582526));
#196248=CARTESIAN_POINT('Ctrl Pts',(-62.3250181713757,-46.5092013876676,
-214.451117556556));
#196249=CARTESIAN_POINT('Ctrl Pts',(-62.3295400872478,-46.5213212599191,
-214.419064953893));
#196250=CARTESIAN_POINT('Ctrl Pts',(-62.3335412504316,-46.53296189092,-214.388180620701));
#196251=CARTESIAN_POINT('Ctrl Pts',(-62.3370905398435,-46.5440983979919,
-214.3585525217));
#196252=CARTESIAN_POINT('Ctrl Pts',(-62.3431483131307,-46.563105705434,
-214.307984566864));
#196253=CARTESIAN_POINT('Ctrl Pts',(-62.3481974598883,-46.5816012447937,
-214.258543468685));
#196254=CARTESIAN_POINT('Ctrl Pts',(-62.3523753769479,-46.5997120229032,
-214.209924790467));
#196255=CARTESIAN_POINT('Ctrl Pts',(-62.3566237941043,-46.6181284106238,
-214.16048569828));
#196256=CARTESIAN_POINT('Ctrl Pts',(-62.3599712539605,-46.6361470995734,
-214.111896534487));
#196257=CARTESIAN_POINT('Ctrl Pts',(-62.3625099115766,-46.6539010598174,
-214.063821875696));
#196258=CARTESIAN_POINT('Ctrl Pts',(-62.3650776056205,-46.6718580846975,
-214.015197352934));
#196259=CARTESIAN_POINT('Ctrl Pts',(-62.3668178742564,-46.6895444447507,
-213.967098722728));
#196260=CARTESIAN_POINT('Ctrl Pts',(-62.3677738035265,-46.7070947829981,
-213.919170467337));
#196261=CARTESIAN_POINT('Ctrl Pts',(-62.3681826664685,-46.7146012828563,
-213.89867095119));
#196262=CARTESIAN_POINT('Ctrl Pts',(-62.3684473988348,-46.7220828491721,
-213.878202538093));
#196263=CARTESIAN_POINT('Ctrl Pts',(-62.3685684816626,-46.7295497479019,
-213.857737248298));
#196264=CARTESIAN_POINT('Ctrl Pts',(-61.7048393179462,20.3302886060538,
-216.296804750573));
#196265=CARTESIAN_POINT('Ctrl Pts',(-62.3412105997785,20.8703282681299,
-215.296246486213));
#196266=CARTESIAN_POINT('Ctrl Pts',(-62.3422326083537,21.4655488148376,
-214.137178092368));
#196267=CARTESIAN_POINT('Ctrl Pts',(-61.7197275390738,19.826031280405,-216.049349212268));
#196268=CARTESIAN_POINT('Ctrl Pts',(-62.3639049458357,20.3085254361885,
-215.01549277859));
#196269=CARTESIAN_POINT('Ctrl Pts',(-62.3680533687934,20.8390832880415,
-213.816997588));
#196270=CARTESIAN_POINT('Ctrl Pts',(-61.7308466500715,19.2797411012228,
-215.844507094054));
#196271=CARTESIAN_POINT('Ctrl Pts',(-62.3866177449706,19.7060437424658,
-214.781622878777));
#196272=CARTESIAN_POINT('Ctrl Pts',(-62.3936763768326,20.173797793921,-213.547199312721));
#196273=CARTESIAN_POINT('Ctrl Pts',(-61.7466079433738,18.1603035078498,
-215.528079628832));
#196274=CARTESIAN_POINT('Ctrl Pts',(-62.4297966614041,18.4809322317388,
-214.415601481719));
#196275=CARTESIAN_POINT('Ctrl Pts',(-62.4421294023084,18.8292102512286,
-213.116884807332));
#196276=CARTESIAN_POINT('Ctrl Pts',(-61.7513829905102,17.5842705648492,
-215.414156702354));
#196277=CARTESIAN_POINT('Ctrl Pts',(-62.4504311411109,17.8546566875628,
-214.280854067528));
#196278=CARTESIAN_POINT('Ctrl Pts',(-62.465140608479,18.1462075363528,-212.953486548188));
#196279=CARTESIAN_POINT('Ctrl Pts',(-61.75613865849,16.4063111425851,-215.262563594693));
#196280=CARTESIAN_POINT('Ctrl Pts',(-62.4897414461557,16.5806351950176,
-214.093342676416));
#196281=CARTESIAN_POINT('Ctrl Pts',(-62.5088056235126,16.7621631730818,
-212.713827714098));
#196282=CARTESIAN_POINT('Ctrl Pts',(-61.7560859039706,15.8044369348897,
-215.225019582751));
#196283=CARTESIAN_POINT('Ctrl Pts',(-62.5084194911065,15.9326272322602,
-214.040799041022));
#196284=CARTESIAN_POINT('Ctrl Pts',(-62.5294585302,16.0610980086206,-212.637681074466));
#196285=CARTESIAN_POINT('Ctrl Pts',(-61.75170975595,14.5794316584473,-215.219446270607));
#196286=CARTESIAN_POINT('Ctrl Pts',(-62.5437558590124,14.61854768797,-214.009629694108));
#196287=CARTESIAN_POINT('Ctrl Pts',(-62.568416048291,14.6428357290722,-212.563275779234));
#196288=CARTESIAN_POINT('Ctrl Pts',(-61.7474254168418,13.9650471940131,
-215.251428369238));
#196289=CARTESIAN_POINT('Ctrl Pts',(-62.5601618106751,13.9616961240068,
-214.031343271628));
#196290=CARTESIAN_POINT('Ctrl Pts',(-62.5864410346862,13.9358240577698,
-212.565541839207));
#196291=CARTESIAN_POINT('Ctrl Pts',(-61.7289261711493,12.1227396799969,
-215.437974674513));
#196292=CARTESIAN_POINT('Ctrl Pts',(-62.6058121860344,11.9946652158632,
-214.19272370704));
#196293=CARTESIAN_POINT('Ctrl Pts',(-62.6364325628104,11.8237195743705,
-212.673714044577));
#196294=CARTESIAN_POINT('Ctrl Pts',(-61.7091779624899,10.8934347501059,
-215.682357515454));
#196295=CARTESIAN_POINT('Ctrl Pts',(-62.6314451217397,10.6892364940185,
-214.428306849402));
#196296=CARTESIAN_POINT('Ctrl Pts',(-62.6643973443486,10.4250272317226,
-212.879944055009));
#196297=CARTESIAN_POINT('Ctrl Pts',(-61.6812232412141,9.63282158578171,
-216.039230989765));
#196298=CARTESIAN_POINT('Ctrl Pts',(-62.6532663489862,9.3570927525791,-214.780166408587));
#196299=CARTESIAN_POINT('Ctrl Pts',(-62.6882099634729,8.99324453840434,
-213.207737243319));
#196300=CARTESIAN_POINT('Ctrl Pts',(-61.6803687865461,9.59462850398232,
-216.050145822074));
#196301=CARTESIAN_POINT('Ctrl Pts',(-62.6539249040132,9.31663341093719,
-214.790961694005));
#196302=CARTESIAN_POINT('Ctrl Pts',(-62.6889267575668,8.94986797086315,
-213.217780919797));
#196303=CARTESIAN_POINT('Ctrl Pts',(-61.6790760497614,9.53735006211111,
-216.06666835234));
#196304=CARTESIAN_POINT('Ctrl Pts',(-62.6549061690901,9.25596256650207,
-214.807312410465));
#196305=CARTESIAN_POINT('Ctrl Pts',(-62.6899947648924,8.88481924518834,
-213.233011700938));
#196306=CARTESIAN_POINT('Ctrl Pts',(-61.6813278541514,9.51005174913774,
-216.070633460958));
#196307=CARTESIAN_POINT('Ctrl Pts',(-62.6553509085009,9.23107896539847,
-214.811457518833));
#196308=CARTESIAN_POINT('Ctrl Pts',(-62.6903499578521,8.86313707307296,
-213.238096257499));
#196309=CARTESIAN_POINT('Ctrl Pts',(-61.6842939631037,9.46010771421665,
-216.079339374395));
#196310=CARTESIAN_POINT('Ctrl Pts',(-62.6561734349085,9.18394861329238,
-214.820392132479));
#196311=CARTESIAN_POINT('Ctrl Pts',(-62.6910610727134,8.81976237959425,
-213.24815996515));
#196312=CARTESIAN_POINT('Ctrl Pts',(-61.6857737786881,9.43512707163234,
-216.083656167532));
#196313=CARTESIAN_POINT('Ctrl Pts',(-62.6565846451019,9.16037796026954,
-214.824824505124));
#196314=CARTESIAN_POINT('Ctrl Pts',(-62.6914166532021,8.79807157636304,
-213.253156652719));
#196315=CARTESIAN_POINT('Ctrl Pts',(-61.6931565890002,9.31018038032887,
-216.105058365171));
#196316=CARTESIAN_POINT('Ctrl Pts',(-62.6586400955044,9.04251720585592,
-214.846806972038));
#196317=CARTESIAN_POINT('Ctrl Pts',(-62.693194685499,8.68960018849763,-213.277963347887));
#196318=CARTESIAN_POINT('Ctrl Pts',(-61.6990107871747,9.21008393110796,
-216.12159850752));
#196319=CARTESIAN_POINT('Ctrl Pts',(-62.6602839455125,8.94812374264299,
-214.863834333959));
#196320=CARTESIAN_POINT('Ctrl Pts',(-62.6946175261465,8.60276749258736,
-213.297243169367));
#196321=CARTESIAN_POINT('Ctrl Pts',(-61.7164142065137,8.90936371264559,
-216.169436492099));
#196322=CARTESIAN_POINT('Ctrl Pts',(-62.665212603975,8.66473293878732,-214.913181982244));
#196323=CARTESIAN_POINT('Ctrl Pts',(-62.6988878681185,8.34209912341666,
-213.353350073391));
#196324=CARTESIAN_POINT('Ctrl Pts',(-61.7278043599611,8.70830926312332,
-216.198952520733));
#196325=CARTESIAN_POINT('Ctrl Pts',(-62.6684968108444,8.47539373639615,
-214.943794401356));
#196326=CARTESIAN_POINT('Ctrl Pts',(-62.7017371797689,8.16809322419483,
-213.388445162646));
#196327=CARTESIAN_POINT('Ctrl Pts',(-61.7613103499456,8.10330948564394,
-216.280050016991));
#196328=CARTESIAN_POINT('Ctrl Pts',(-62.6783432928825,7.90644691041792,
-215.028387072985));
#196329=CARTESIAN_POINT('Ctrl Pts',(-62.7102973061948,7.64536444873709,
-213.486494648338));
#196330=CARTESIAN_POINT('Ctrl Pts',(-61.7827637049333,7.69753105649767,
-216.324192904775));
#196331=CARTESIAN_POINT('Ctrl Pts',(-62.6849084717677,7.52538355400632,
-215.075235965833));
#196332=CARTESIAN_POINT('Ctrl Pts',(-62.7160201318226,7.29593153216955,
-213.542223849032));
#196333=CARTESIAN_POINT('Ctrl Pts',(-61.8441798777663,6.47185390193823,
-216.423878386747));
#196334=CARTESIAN_POINT('Ctrl Pts',(-62.7046282021264,6.37770422140462,
-215.184004366012));
#196335=CARTESIAN_POINT('Ctrl Pts',(-62.7332823333847,6.24451635056923,
-213.677692349319));
#196336=CARTESIAN_POINT('Ctrl Pts',(-61.8807935575335,5.64537503727213,
-216.447122146682));
#196337=CARTESIAN_POINT('Ctrl Pts',(-62.7178214583037,5.60536816135207,
-215.214862678102));
#196338=CARTESIAN_POINT('Ctrl Pts',(-62.7449139403618,5.53942734608012,
-213.725811404425));
#196339=CARTESIAN_POINT('Ctrl Pts',(-61.9276637801842,4.38900749273041,
-216.405043063736));
#196340=CARTESIAN_POINT('Ctrl Pts',(-62.737836834247,4.4352006251806,-215.186375172552));
#196341=CARTESIAN_POINT('Ctrl Pts',(-62.7627331655823,4.47441539748971,
-213.722866226851));
#196342=CARTESIAN_POINT('Ctrl Pts',(-61.9418614366659,3.96797397400649,
-216.378259335607));
#196343=CARTESIAN_POINT('Ctrl Pts',(-62.7445389526157,4.0435897159706,-215.164491462244));
#196344=CARTESIAN_POINT('Ctrl Pts',(-62.768735486043,4.11817803005001,-213.709326696003));
#196345=CARTESIAN_POINT('Ctrl Pts',(-61.9671948784838,3.12080313566866,
-216.297090847051));
#196346=CARTESIAN_POINT('Ctrl Pts',(-62.7580382224546,3.2566272438502,-215.093872524279));
#196347=CARTESIAN_POINT('Ctrl Pts',(-62.7808960763507,3.40303826439861,
-213.655109821494));
#196348=CARTESIAN_POINT('Ctrl Pts',(-61.9783399396214,2.69421717174147,
-216.242544071251));
#196349=CARTESIAN_POINT('Ctrl Pts',(-62.7648437006275,2.86082211157324,
-215.045005100094));
#196350=CARTESIAN_POINT('Ctrl Pts',(-62.7870578417518,3.04396622992889,
-213.614329768932));
#196351=CARTESIAN_POINT('Ctrl Pts',(-61.9971071789784,1.84291295407256,
-216.104949160831));
#196352=CARTESIAN_POINT('Ctrl Pts',(-62.7784709761191,2.07150539346803,
-214.919405013978));
#196353=CARTESIAN_POINT('Ctrl Pts',(-62.7994785535875,2.32831168170424,
-213.504372226852));
#196354=CARTESIAN_POINT('Ctrl Pts',(-62.0047577753412,1.41755300336648,
-216.021919722206));
#196355=CARTESIAN_POINT('Ctrl Pts',(-62.7853055583149,1.6772084331531,-214.842667949039));
#196356=CARTESIAN_POINT('Ctrl Pts',(-62.8057475169848,1.97109323824117,
-213.43520790963));
#196357=CARTESIAN_POINT('Ctrl Pts',(-62.01209734533,0.886092884169537,-215.899694254584));
#196358=CARTESIAN_POINT('Ctrl Pts',(-62.7938861397906,1.18486559069481,
-214.728722297667));
#196359=CARTESIAN_POINT('Ctrl Pts',(-62.8136699413683,1.52535840970665,
-213.330389729488));
#196360=CARTESIAN_POINT('Ctrl Pts',(-62.0134539642545,0.779812584027515,
-215.874326692892));
#196361=CARTESIAN_POINT('Ctrl Pts',(-62.7956043592763,1.08641018260874,
-214.705028633956));
#196362=CARTESIAN_POINT('Ctrl Pts',(-62.815258743729,1.43625087082071,-213.308507593622));
#196363=CARTESIAN_POINT('Ctrl Pts',(-62.0153204933596,0.620406471798272,
-215.834877732922));
#196364=CARTESIAN_POINT('Ctrl Pts',(-62.7981848937995,0.938758219164633,
-214.668121421941));
#196365=CARTESIAN_POINT('Ctrl Pts',(-62.8176486878298,1.30264926379029,
-213.27429362079));
#196366=CARTESIAN_POINT('Ctrl Pts',(-62.01591460122,0.567273487007788,-215.8214951353));
#196367=CARTESIAN_POINT('Ctrl Pts',(-62.7990456346484,0.889544467315833,
-214.655590802865));
#196368=CARTESIAN_POINT('Ctrl Pts',(-62.8184464593903,1.25812534522924,
-213.262657162745));
#196369=CARTESIAN_POINT('Ctrl Pts',(-62.0166219833978,0.500859866452599,
-215.804474193104));
#196370=CARTESIAN_POINT('Ctrl Pts',(-62.8001222578722,0.828033612066846,
-214.639641386032));
#196371=CARTESIAN_POINT('Ctrl Pts',(-62.8194451065877,1.20248294550228,
-213.247820438255));
#196372=CARTESIAN_POINT('Ctrl Pts',(-62.0167616971461,0.487577272851923,
-215.801055369767));
#196373=CARTESIAN_POINT('Ctrl Pts',(-62.8003376213968,0.815731527809191,
-214.636437135192));
#196374=CARTESIAN_POINT('Ctrl Pts',(-62.8196449076661,1.19135509048132,
-213.24483853566));
#196375=CARTESIAN_POINT('Ctrl Pts',(-62.0170375949548,0.461012336886231,
-215.79418841463));
#196376=CARTESIAN_POINT('Ctrl Pts',(-62.8007684207769,0.791127882266898,
-214.629999954911));
#196377=CARTESIAN_POINT('Ctrl Pts',(-62.8200446538203,1.16910063183232,
-213.238845579474));
#196378=CARTESIAN_POINT('Ctrl Pts',(-62.0171192435935,0.445144526651812,
-215.79019033046));
#196379=CARTESIAN_POINT('Ctrl Pts',(-62.8010073784724,0.777422914824527,
-214.626482823901));
#196380=CARTESIAN_POINT('Ctrl Pts',(-62.8202446769488,1.15797422718805,
-213.235829903834));
#196381=CARTESIAN_POINT('Ctrl Pts',(-62.0177632729019,0.416720308882189,
-215.782227774949));
#196382=CARTESIAN_POINT('Ctrl Pts',(-62.8015499256584,0.746719684915778,
-214.617992853663));
#196383=CARTESIAN_POINT('Ctrl Pts',(-62.820844450332,1.12459558461347,-213.226769479741));
#196384=CARTESIAN_POINT('Ctrl Pts',(-62.0181895523145,0.397765742510003,
-215.776959654906));
#196385=CARTESIAN_POINT('Ctrl Pts',(-62.8019103468331,0.726247045178752,
-214.612375378367));
#196386=CARTESIAN_POINT('Ctrl Pts',(-62.8212428505405,1.1023412309075,-213.220773750029));
#196387=CARTESIAN_POINT('Ctrl Pts',(-62.021998557213,0.227129297670825,
-215.729907595764));
#196388=CARTESIAN_POINT('Ctrl Pts',(-62.8051425298092,0.541966547718803,
-214.562201271057));
#196389=CARTESIAN_POINT('Ctrl Pts',(-62.8248154365297,0.902034785262884,
-213.16721163518));
#196390=CARTESIAN_POINT('Ctrl Pts',(-62.0251888105107,0.0751301734146063,
-215.69065008324));
#196391=CARTESIAN_POINT('Ctrl Pts',(-62.8079340444995,0.377915226937975,
-214.520310461555));
#196392=CARTESIAN_POINT('Ctrl Pts',(-62.8278985261067,0.72386189685476,
-213.122440498364));
#196393=CARTESIAN_POINT('Ctrl Pts',(-62.0522125573282,-1.29554564506861,
-215.359846846471));
#196394=CARTESIAN_POINT('Ctrl Pts',(-62.8323237597321,-1.10022488337052,
-214.167113276732));
#196395=CARTESIAN_POINT('Ctrl Pts',(-62.8548240427874,-0.880767445010574,
-212.744334484548));
#196396=CARTESIAN_POINT('Ctrl Pts',(-62.0645369285303,-2.53275074795512,
-215.223595176109));
#196397=CARTESIAN_POINT('Ctrl Pts',(-62.8488703095335,-2.42925885397665,
-214.019298532614));
#196398=CARTESIAN_POINT('Ctrl Pts',(-62.8729565843244,-2.31461725004268,
-212.582049783317));
#196399=CARTESIAN_POINT('Ctrl Pts',(-62.0693960981775,-5.02446259512134,
-215.234052482319));
#196400=CARTESIAN_POINT('Ctrl Pts',(-62.8719056110164,-5.1003827717422,
-214.019608088502));
#196401=CARTESIAN_POINT('Ctrl Pts',(-62.8981414605001,-5.19559191584348,
-212.564399664962));
#196402=CARTESIAN_POINT('Ctrl Pts',(-62.0618907988487,-6.27912184780759,
-215.381002476288));
#196403=CARTESIAN_POINT('Ctrl Pts',(-62.8783989700247,-6.4443743523136,
-214.168268362741));
#196404=CARTESIAN_POINT('Ctrl Pts',(-62.9051900334741,-6.64273030664321,
-212.709348944425));
#196405=CARTESIAN_POINT('Ctrl Pts',(-62.0408583819432,-7.6912959294504,
-215.713424151605));
#196406=CARTESIAN_POINT('Ctrl Pts',(-62.8798161172096,-7.9569135349361,
-214.509722650088));
#196407=CARTESIAN_POINT('Ctrl Pts',(-62.9066422728629,-8.27861416050181,
-213.053996708501));
#196408=CARTESIAN_POINT('Ctrl Pts',(-62.0383424658172,-7.84822778562573,
-215.752714376751));
#196409=CARTESIAN_POINT('Ctrl Pts',(-62.8798914154057,-8.12519201954069,
-214.550165533701));
#196410=CARTESIAN_POINT('Ctrl Pts',(-62.9067130375752,-8.46050513615589,
-213.09485254092));
#196411=CARTESIAN_POINT('Ctrl Pts',(-62.0342925038254,-8.08357756168836,
-215.815225127789));
#196412=CARTESIAN_POINT('Ctrl Pts',(-62.8798796987704,-8.37759392911409,
-214.614571441277));
#196413=CARTESIAN_POINT('Ctrl Pts',(-62.9066818269245,-8.7334636680148,
-213.160032454394));
#196414=CARTESIAN_POINT('Ctrl Pts',(-62.0328986542006,-8.16189402537491,
-215.836624633389));
#196415=CARTESIAN_POINT('Ctrl Pts',(-62.8798550144986,-8.46160075459694,
-214.636632184066));
#196416=CARTESIAN_POINT('Ctrl Pts',(-62.9066485485958,-8.82432470155739,
-213.182373733743));
#196417=CARTESIAN_POINT('Ctrl Pts',(-62.0311011014652,-8.25962032848021,
-215.864076645694));
#196418=CARTESIAN_POINT('Ctrl Pts',(-62.879798315969,-8.5664344313122,-214.664943966702));
#196419=CARTESIAN_POINT('Ctrl Pts',(-62.9065784769814,-8.9377445621295,
-213.211068643959));
#196420=CARTESIAN_POINT('Ctrl Pts',(-62.0307388286769,-8.27915712437951,
-215.869602181102));
#196421=CARTESIAN_POINT('Ctrl Pts',(-62.8797856829879,-8.58739394937797,
-214.670643537108));
#196422=CARTESIAN_POINT('Ctrl Pts',(-62.9065630389366,-8.96042071227823,
-213.21684604351));
#196423=CARTESIAN_POINT('Ctrl Pts',(-62.0301912677851,-8.30844957422519,
-215.877943176995));
#196424=CARTESIAN_POINT('Ctrl Pts',(-62.8797647971169,-8.6188202438996,
-214.679248133562));
#196425=CARTESIAN_POINT('Ctrl Pts',(-62.9065377484219,-8.99442320332278,
-213.225569775073));
#196426=CARTESIAN_POINT('Ctrl Pts',(-62.0296632681837,-8.31557091097187,
-215.880572879503));
#196427=CARTESIAN_POINT('Ctrl Pts',(-62.8797526332712,-8.62783903034508,
-214.682096820377));
#196428=CARTESIAN_POINT('Ctrl Pts',(-62.9065289038154,-9.00575475319362,
-213.228490523493));
#196429=CARTESIAN_POINT('Ctrl Pts',(-62.0302223796579,-8.34218925560487,
-215.886598433304));
#196430=CARTESIAN_POINT('Ctrl Pts',(-62.8797505157256,-8.65269102163767,
-214.687948520214));
#196431=CARTESIAN_POINT('Ctrl Pts',(-62.9065107565237,-9.02841676695755,
-213.234337353351));
#196432=CARTESIAN_POINT('Ctrl Pts',(-62.0305005605521,-8.35550200411735,
-215.889599207275));
#196433=CARTESIAN_POINT('Ctrl Pts',(-62.8797494596239,-8.66511992948451,
-214.690862545141));
#196434=CARTESIAN_POINT('Ctrl Pts',(-62.9065017229464,-9.03975023999172,
-213.237248654769));
#196435=CARTESIAN_POINT('Ctrl Pts',(-62.0318845638498,-8.4220835950757,
-215.904542950278));
#196436=CARTESIAN_POINT('Ctrl Pts',(-62.8797441930548,-8.72727623804196,
-214.705372782964));
#196437=CARTESIAN_POINT('Ctrl Pts',(-62.9064567562113,-9.0964299581106,
-213.251744484892));
#196438=CARTESIAN_POINT('Ctrl Pts',(-62.0329696818077,-8.47540598081262,
-215.916305535754));
#196439=CARTESIAN_POINT('Ctrl Pts',(-62.8797400235165,-8.77705017731475,
-214.716791984103));
#196440=CARTESIAN_POINT('Ctrl Pts',(-62.906421426558,-9.14181326257087,
-213.263146980914));
#196441=CARTESIAN_POINT('Ctrl Pts',(-62.0425339213031,-8.95581758539506,
-216.020424374309));
#196442=CARTESIAN_POINT('Ctrl Pts',(-62.8797029458838,-9.22525437208547,
-214.817805862891));
#196443=CARTESIAN_POINT('Ctrl Pts',(-62.9061093426684,-9.55062130297945,
-213.364009501424));
#196444=CARTESIAN_POINT('Ctrl Pts',(-62.0495923408927,-9.38642678550509,
-216.100559216461));
#196445=CARTESIAN_POINT('Ctrl Pts',(-62.8796731221476,-9.62683004577358,
-214.895428417083));
#196446=CARTESIAN_POINT('Ctrl Pts',(-62.9058739446102,-9.91655549914845,
-213.44114324688));
#196447=CARTESIAN_POINT('Ctrl Pts',(-62.0605543158907,-10.2546820187393,
-216.234694113546));
#196448=CARTESIAN_POINT('Ctrl Pts',(-62.8796223280864,-10.4359064752367,
-215.024917585528));
#196449=CARTESIAN_POINT('Ctrl Pts',(-62.9054945382152,-10.6537874440521,
-213.569065352509));
#196450=CARTESIAN_POINT('Ctrl Pts',(-62.0644591054324,-10.6938948125732,
-216.288789203932));
#196451=CARTESIAN_POINT('Ctrl Pts',(-62.8796013738763,-10.8450105623093,
-215.076911105874));
#196452=CARTESIAN_POINT('Ctrl Pts',(-62.905350423994,-11.0264379343114,
-213.619939162974));
#196453=CARTESIAN_POINT('Ctrl Pts',(-62.0688689645132,-11.5686947372008,
-216.368854953593));
#196454=CARTESIAN_POINT('Ctrl Pts',(-62.8795684212377,-11.6595117932001,
-215.153252185298));
#196455=CARTESIAN_POINT('Ctrl Pts',(-62.9051593336146,-11.7684901551169,
-213.693446645343));
#196456=CARTESIAN_POINT('Ctrl Pts',(-62.069391577455,-12.004576298268,-216.394995859349));
#196457=CARTESIAN_POINT('Ctrl Pts',(-62.8795563368116,-12.0653505367772,
-215.177787425828));
#196458=CARTESIAN_POINT('Ctrl Pts',(-62.9051117861205,-12.1381923296176,
-213.716251957739));
#196459=CARTESIAN_POINT('Ctrl Pts',(-62.0660431402244,-13.3071722247956,
-216.432951006704));
#196460=CARTESIAN_POINT('Ctrl Pts',(-62.8795272203036,-13.2782401253067,
-215.211670172273));
#196461=CARTESIAN_POINT('Ctrl Pts',(-62.9051036527997,-13.243445563085,
-213.744071341037));
#196462=CARTESIAN_POINT('Ctrl Pts',(-62.0572284163516,-14.1686539550577,
-216.404224735683));
#196463=CARTESIAN_POINT('Ctrl Pts',(-62.8795183650933,-14.0812399938794,
-215.181181755551));
#196464=CARTESIAN_POINT('Ctrl Pts',(-62.9052789204624,-13.9751373806058,
-213.708426173576));
#196465=CARTESIAN_POINT('Ctrl Pts',(-62.0352390706104,-15.4484326336701,
-216.286430648765));
#196466=CARTESIAN_POINT('Ctrl Pts',(-62.8794726572187,-15.2751677276984,
-215.062361671888));
#196467=CARTESIAN_POINT('Ctrl Pts',(-62.9057445940404,-15.0655774299771,
-213.580180828239));
#196468=CARTESIAN_POINT('Ctrl Pts',(-62.0264514220739,-15.8729863495462,
-216.234737322802));
#196469=CARTESIAN_POINT('Ctrl Pts',(-62.8794515889032,-15.6718235071092,
-215.010536635359));
#196470=CARTESIAN_POINT('Ctrl Pts',(-62.9059331942183,-15.4278764578916,
-213.524990067771));
#196471=CARTESIAN_POINT('Ctrl Pts',(-62.0112934704005,-16.5064765229115,
-216.139470449859));
#196472=CARTESIAN_POINT('Ctrl Pts',(-62.8794032606368,-16.2642082032074,
-214.915478455953));
#196473=CARTESIAN_POINT('Ctrl Pts',(-62.9062547760745,-15.9696430762714,
-213.424484058152));
#196474=CARTESIAN_POINT('Ctrl Pts',(-62.0059085609425,-16.7171041054341,
-216.104763566933));
#196475=CARTESIAN_POINT('Ctrl Pts',(-62.879384268395,-16.4613492368974,
-214.880888370633));
#196476=CARTESIAN_POINT('Ctrl Pts',(-62.9063683773708,-16.1499518187337,
-213.38803074649));
#196477=CARTESIAN_POINT('Ctrl Pts',(-61.9973599442118,-17.0322203070265,
-216.048392932234));
#196478=CARTESIAN_POINT('Ctrl Pts',(-62.8793503960171,-16.7564347142257,
-214.824791986014));
#196479=CARTESIAN_POINT('Ctrl Pts',(-62.9065468872613,-16.4200061599841,
-213.329044171076));
#196480=CARTESIAN_POINT('Ctrl Pts',(-61.9944321038605,-17.1371201989063,
-216.028884375262));
#196481=CARTESIAN_POINT('Ctrl Pts',(-62.8793382060926,-16.8547164489359,
-214.805385954228));
#196482=CARTESIAN_POINT('Ctrl Pts',(-62.9066077402092,-16.5099561526457,
-213.308664291015));
#196483=CARTESIAN_POINT('Ctrl Pts',(-61.9899270123872,-17.2942564226434,
-215.998559354035));
#196484=CARTESIAN_POINT('Ctrl Pts',(-62.8793184382364,-17.0019805803341,
-214.775238880667));
#196485=CARTESIAN_POINT('Ctrl Pts',(-62.9067008407091,-16.644780457911,
-213.277033722408));
#196486=CARTESIAN_POINT('Ctrl Pts',(-61.9884064283002,-17.3465995634399,
-215.98827398914));
#196487=CARTESIAN_POINT('Ctrl Pts',(-62.8793116007265,-17.0510484368828,
-214.765015498814));
#196488=CARTESIAN_POINT('Ctrl Pts',(-62.9067321776173,-16.6897051128861,
-213.266313413053));
#196489=CARTESIAN_POINT('Ctrl Pts',(-61.9860977496528,-17.4250602397112,
-215.972582374709));
#196490=CARTESIAN_POINT('Ctrl Pts',(-62.8793009553668,-17.1246105011707,
-214.749422813232));
#196491=CARTESIAN_POINT('Ctrl Pts',(-62.9067796117351,-16.7570671165656,
-213.249969786042));
#196492=CARTESIAN_POINT('Ctrl Pts',(-61.9853235564599,-17.4512047924259,
-215.967307909158));
#196493=CARTESIAN_POINT('Ctrl Pts',(-62.8792973418093,-17.1491261237452,
-214.744181975806));
#196494=CARTESIAN_POINT('Ctrl Pts',(-62.9067954945617,-16.7795169546794,
-213.244478050128));
#196495=CARTESIAN_POINT('Ctrl Pts',(-61.9841553829125,-17.4904080355635,
-215.959330569069));
#196496=CARTESIAN_POINT('Ctrl Pts',(-62.8792918218644,-17.1858896145504,
-214.736256555115));
#196497=CARTESIAN_POINT('Ctrl Pts',(-62.9068194226298,-16.8131854913724,
-213.236174910655));
#196498=CARTESIAN_POINT('Ctrl Pts',(-61.9837648444543,-17.5034735188566,
-215.956660515446));
#196499=CARTESIAN_POINT('Ctrl Pts',(-62.8792899652221,-17.1981428428804,
-214.733603968975));
#196500=CARTESIAN_POINT('Ctrl Pts',(-62.9068274159574,-16.8244073001866,
-213.233396274889));
#196501=CARTESIAN_POINT('Ctrl Pts',(-61.9829814841363,-17.5295999440097,
-215.951298569524));
#196502=CARTESIAN_POINT('Ctrl Pts',(-62.8792862182922,-17.2226462406558,
-214.728277392464));
#196503=CARTESIAN_POINT('Ctrl Pts',(-62.9068434366578,-16.8468488483916,
-213.227817200875));
#196504=CARTESIAN_POINT('Ctrl Pts',(-61.9837428929013,-17.5368644595024,
-215.948389601018));
#196505=CARTESIAN_POINT('Ctrl Pts',(-62.8793014620505,-17.231672318972,
-214.725294222846));
#196506=CARTESIAN_POINT('Ctrl Pts',(-62.9068512246001,-16.8580698646293,
-213.225030214802));
#196507=CARTESIAN_POINT('Ctrl Pts',(-62.0181703622904,-18.7944029448088,
-215.587225509336));
#196508=CARTESIAN_POINT('Ctrl Pts',(-62.880264860769,-18.5719548213566,
-214.360359994756));
#196509=CARTESIAN_POINT('Ctrl Pts',(-62.9078064251384,-18.3057228153494,
-212.867003491606));
#196510=CARTESIAN_POINT('Ctrl Pts',(-62.0423858502321,-20.0566437152891,
-215.359087336711));
#196511=CARTESIAN_POINT('Ctrl Pts',(-62.8762911738208,-19.9202073218907,
-214.133506617223));
#196512=CARTESIAN_POINT('Ctrl Pts',(-62.9033129898347,-19.7553919607571,
-212.653495577744));
#196513=CARTESIAN_POINT('Ctrl Pts',(-62.0716387653447,-22.571278684854,
-215.180930588057));
#196514=CARTESIAN_POINT('Ctrl Pts',(-62.8581514858358,-22.6113837391411,
-213.972570780553));
#196515=CARTESIAN_POINT('Ctrl Pts',(-62.8830851680151,-22.6547081034196,
-212.52986856343));
#196516=CARTESIAN_POINT('Ctrl Pts',(-62.0768709559833,-23.8284596089826,
-215.229198343105));
#196517=CARTESIAN_POINT('Ctrl Pts',(-62.8440002381499,-23.960868557364,
-214.035847577147));
#196518=CARTESIAN_POINT('Ctrl Pts',(-62.8673563795348,-24.1094370634132,
-212.617838162856));
#196519=CARTESIAN_POINT('Ctrl Pts',(-62.0687933625429,-25.3808544123227,
-215.497967942811));
#196520=CARTESIAN_POINT('Ctrl Pts',(-62.8194037351821,-25.6376387826187,
-214.336265031285));
#196521=CARTESIAN_POINT('Ctrl Pts',(-62.8399085993614,-25.9282456355465,
-212.959941102891));
#196522=CARTESIAN_POINT('Ctrl Pts',(-62.0664266960169,-25.6901805447464,
-215.562269443776));
#196523=CARTESIAN_POINT('Ctrl Pts',(-62.8141424132872,-25.9721673633214,
-214.407507976939));
#196524=CARTESIAN_POINT('Ctrl Pts',(-62.8340297350373,-26.2918276350188,
-213.04012465042));
#196525=CARTESIAN_POINT('Ctrl Pts',(-62.0624202311128,-26.0751062786157,
-215.656867415151));
#196526=CARTESIAN_POINT('Ctrl Pts',(-62.8071202348902,-26.3892914434607,
-214.511710407704));
#196527=CARTESIAN_POINT('Ctrl Pts',(-62.8261731592035,-26.7460613321195,
-213.156334850816));
#196528=CARTESIAN_POINT('Ctrl Pts',(-62.0615663934927,-26.1520046023118,
-215.676499151611));
#196529=CARTESIAN_POINT('Ctrl Pts',(-62.8056936212433,-26.4726579103633,
-214.533307712649));
#196530=CARTESIAN_POINT('Ctrl Pts',(-62.8245764208426,-26.8368958608041,
-213.180377302496));
#196531=CARTESIAN_POINT('Ctrl Pts',(-62.0604313366008,-26.2480138120354,
-215.701948095613));
#196532=CARTESIAN_POINT('Ctrl Pts',(-62.8038822013363,-26.5767984556868,
-214.561274047172));
#196533=CARTESIAN_POINT('Ctrl Pts',(-62.822548322552,-26.9504234038111,
-213.211454506226));
#196534=CARTESIAN_POINT('Ctrl Pts',(-62.0602009365971,-26.2672099682503,
-215.707083353122));
#196535=CARTESIAN_POINT('Ctrl Pts',(-62.8035185165143,-26.5976227967682,
-214.566915697153));
#196536=CARTESIAN_POINT('Ctrl Pts',(-62.8221410940186,-26.9731281314353,
-213.217721160276));
#196537=CARTESIAN_POINT('Ctrl Pts',(-62.0598502125763,-26.2959955735649,
-215.714854815994));
#196538=CARTESIAN_POINT('Ctrl Pts',(-62.8029708726847,-26.6288541544021,
-214.575451318361));
#196539=CARTESIAN_POINT('Ctrl Pts',(-62.8215278301374,-27.0071840444203,
-213.227198424034));
#196540=CARTESIAN_POINT('Ctrl Pts',(-62.0597324505761,-26.3055893371753,
-215.717456733094));
#196541=CARTESIAN_POINT('Ctrl Pts',(-62.8027879726431,-26.6392637102074,
-214.578308705998));
#196542=CARTESIAN_POINT('Ctrl Pts',(-62.8213230053295,-27.0185358190149,
-213.230370392442));
#196543=CARTESIAN_POINT('Ctrl Pts',(-62.0595545213414,-26.3199778126609,
-215.721376800301));
#196544=CARTESIAN_POINT('Ctrl Pts',(-62.8025130927215,-26.6548767478047,
-214.582613127237));
#196545=CARTESIAN_POINT('Ctrl Pts',(-62.8210151618606,-27.0355631854271,
-213.235147724465));
#196546=CARTESIAN_POINT('Ctrl Pts',(-62.0594949972346,-26.3247736095024,
-215.722686354616));
#196547=CARTESIAN_POINT('Ctrl Pts',(-62.8024213779408,-26.6600808682157,
-214.584050988303));
#196548=CARTESIAN_POINT('Ctrl Pts',(-62.8209124463284,-27.0412389249773,
-213.236743398352));
#196549=CARTESIAN_POINT('Ctrl Pts',(-62.0593755193932,-26.3343644777571,
-215.725311201717));
#196550=CARTESIAN_POINT('Ctrl Pts',(-62.8022377717518,-26.6704886693638,
-214.586932830867));
#196551=CARTESIAN_POINT('Ctrl Pts',(-62.8207068130132,-27.052590305443,
-213.239941215787));
#196552=CARTESIAN_POINT('Ctrl Pts',(-62.0591904267342,-26.3423678600797,
-215.727641643505));
#196553=CARTESIAN_POINT('Ctrl Pts',(-62.8021133629123,-26.6774201434905,
-214.588932611784));
#196554=CARTESIAN_POINT('Ctrl Pts',(-62.8206039569716,-27.0582660000666,
-213.241539781896));
#196555=CARTESIAN_POINT('Ctrl Pts',(-62.0579195947297,-26.4041206938665,
-215.745297553372));
#196556=CARTESIAN_POINT('Ctrl Pts',(-62.8010984184952,-26.7342691805765,
-214.605084908191));
#196557=CARTESIAN_POINT('Ctrl Pts',(-62.8196787974583,-27.1093480735134,
-213.255871682944));
#196558=CARTESIAN_POINT('Ctrl Pts',(-62.0567567001996,-26.4589929636436,
-215.760704173281));
#196559=CARTESIAN_POINT('Ctrl Pts',(-62.8001976805287,-26.7847921675662,
-214.619163948744));
#196560=CARTESIAN_POINT('Ctrl Pts',(-62.8188583609005,-27.154758511644,
-213.268331481196));
#196561=CARTESIAN_POINT('Ctrl Pts',(-62.0507778370158,-26.7332616168239,
-215.836316781018));
#196562=CARTESIAN_POINT('Ctrl Pts',(-62.7957006936856,-27.0373714949889,
-214.688185492659));
#196563=CARTESIAN_POINT('Ctrl Pts',(-62.8147655328416,-27.3818312159389,
-213.329248041551));
#196564=CARTESIAN_POINT('Ctrl Pts',(-62.0454689865543,-26.952380588705,
-215.892263197796));
#196565=CARTESIAN_POINT('Ctrl Pts',(-62.7921249336556,-27.2392985917041,
-214.739001463284));
#196566=CARTESIAN_POINT('Ctrl Pts',(-62.811521179222,-27.5635550010564,
-213.373559009004));
#196567=CARTESIAN_POINT('Ctrl Pts',(-62.0164077141018,-28.0466591076513,
-216.150292769558));
#196568=CARTESIAN_POINT('Ctrl Pts',(-62.7743327848849,-28.2486351141899,
-214.972122127568));
#196569=CARTESIAN_POINT('Ctrl Pts',(-62.7954319749737,-28.4724876729194,
-213.573958234288));
#196570=CARTESIAN_POINT('Ctrl Pts',(-61.9849863797742,-28.9185203866592,
-216.287393756369));
#196571=CARTESIAN_POINT('Ctrl Pts',(-62.7603778330476,-29.0550555751074,
-215.09135055822));
#196572=CARTESIAN_POINT('Ctrl Pts',(-62.7829855880221,-29.2006385623869,
-213.666528824391));
#196573=CARTESIAN_POINT('Ctrl Pts',(-61.8719372658986,-31.5146432828636,
-216.52155335041));
#196574=CARTESIAN_POINT('Ctrl Pts',(-62.7188819350269,-31.4677732499339,
-215.279252210143));
#196575=CARTESIAN_POINT('Ctrl Pts',(-62.7463293349613,-31.3876040978064,
-213.774365476491));
#196576=CARTESIAN_POINT('Ctrl Pts',(-61.7714592397433,-33.2214602041654,
-216.443548517691));
#196577=CARTESIAN_POINT('Ctrl Pts',(-62.6916591462751,-33.0686179338109,
-215.178100628118));
#196578=CARTESIAN_POINT('Ctrl Pts',(-62.7227759583433,-32.8489094530129,
-213.621230861645));
#196579=CARTESIAN_POINT('Ctrl Pts',(-61.6527757155717,-35.0048119699771,
-216.189409048519));
#196580=CARTESIAN_POINT('Ctrl Pts',(-62.6622409902955,-34.7480221415653,
-214.910242320336));
#196581=CARTESIAN_POINT('Ctrl Pts',(-62.6973153894391,-34.4039131251359,
-213.29729287427));
#196582=CARTESIAN_POINT('Ctrl Pts',(-61.6457452969654,-35.1096181707137,
-216.173825932635));
#196583=CARTESIAN_POINT('Ctrl Pts',(-62.660500652564,-34.8471952613371,
-214.89381401442));
#196584=CARTESIAN_POINT('Ctrl Pts',(-62.6958162562244,-34.4953927542598,
-213.277636702578));
#196585=CARTESIAN_POINT('Ctrl Pts',(-61.6368972733854,-35.2405100086795,
-216.153573540134));
#196586=CARTESIAN_POINT('Ctrl Pts',(-62.6583222139731,-34.9710950849282,
-214.872545527579));
#196587=CARTESIAN_POINT('Ctrl Pts',(-62.6939402205331,-34.6097530635753,
-213.252332432694));
#196588=CARTESIAN_POINT('Ctrl Pts',(-61.6351246682154,-35.2666825779689,
-216.149484383413));
#196589=CARTESIAN_POINT('Ctrl Pts',(-62.6578862571906,-34.9958784408532,
-214.868253991386));
#196590=CARTESIAN_POINT('Ctrl Pts',(-62.693564907493,-34.632625664116,-213.247234872735));
#196591=CARTESIAN_POINT('Ctrl Pts',(-61.6324612821853,-35.3059328288065,
-216.143292970413));
#196592=CARTESIAN_POINT('Ctrl Pts',(-62.6572320773096,-35.0330492303192,
-214.86176188503));
#196593=CARTESIAN_POINT('Ctrl Pts',(-62.6930017735533,-34.6669353682907,
-213.23953378686));
#196594=CARTESIAN_POINT('Ctrl Pts',(-61.6315727404868,-35.3190148116817,
-216.141219553062));
#196595=CARTESIAN_POINT('Ctrl Pts',(-62.6570139646951,-35.0454394602782,
-214.859588596064));
#196596=CARTESIAN_POINT('Ctrl Pts',(-62.6928140348453,-34.6783720702307,
-213.236957633838));
#196597=CARTESIAN_POINT('Ctrl Pts',(-61.6297941680007,-35.3451759247511,
-216.13705354844));
#196598=CARTESIAN_POINT('Ctrl Pts',(-62.6565776489529,-35.0702189633633,
-214.855223724628));
#196599=CARTESIAN_POINT('Ctrl Pts',(-62.6924385017243,-34.701245741126,
-213.231787130788));
#196600=CARTESIAN_POINT('Ctrl Pts',(-61.6310293684106,-35.3530107643184,
-216.133482239242));
#196601=CARTESIAN_POINT('Ctrl Pts',(-62.6564417977456,-35.0795905313491,
-214.851837785791));
#196602=CARTESIAN_POINT('Ctrl Pts',(-62.6922505031027,-34.712682531357,
-213.229204685838));
#196603=CARTESIAN_POINT('Ctrl Pts',(-61.6325094322944,-35.4037694797289,
-216.118959911289));
#196604=CARTESIAN_POINT('Ctrl Pts',(-62.6555787703405,-35.1331120907873,
-214.837616627857));
#196605=CARTESIAN_POINT('Ctrl Pts',(-62.6913088110132,-34.7698657850322,
-213.216337901175));
#196606=CARTESIAN_POINT('Ctrl Pts',(-61.6336864900504,-35.4443701357922,
-216.107444248921));
#196607=CARTESIAN_POINT('Ctrl Pts',(-62.6548838887415,-35.1759301641451,
-214.826347135623));
#196608=CARTESIAN_POINT('Ctrl Pts',(-62.6905505732429,-34.8156106395167,
-213.206157663245));
#196609=CARTESIAN_POINT('Ctrl Pts',(-61.639536989153,-35.647340776021,-216.050378480442));
#196610=CARTESIAN_POINT('Ctrl Pts',(-62.6513884920124,-35.3899422289628,
-214.770560243673));
#196611=CARTESIAN_POINT('Ctrl Pts',(-62.6867349314889,-35.0443261389348,
-213.155824498556));
#196612=CARTESIAN_POINT('Ctrl Pts',(-61.6441060885591,-35.8096128160609,
-216.006365733016));
#196613=CARTESIAN_POINT('Ctrl Pts',(-62.6485208043159,-35.5611635627003,
-214.727654113872));
#196614=CARTESIAN_POINT('Ctrl Pts',(-62.6836041752041,-35.227270469846,
-213.117375270572));
#196615=CARTESIAN_POINT('Ctrl Pts',(-61.6574855827294,-36.2960730265464,
-215.879313463721));
#196616=CARTESIAN_POINT('Ctrl Pts',(-62.6397088692154,-36.0744688616432,
-214.604282321189));
#196617=CARTESIAN_POINT('Ctrl Pts',(-62.6739757829555,-35.7760179301451,
-213.007568080921));
#196618=CARTESIAN_POINT('Ctrl Pts',(-61.6659645557888,-36.619740284584,
-215.801290160767));
#196619=CARTESIAN_POINT('Ctrl Pts',(-62.6335526368642,-36.4164413462367,
-214.529072745108));
#196620=CARTESIAN_POINT('Ctrl Pts',(-62.6672458339371,-36.1415480006374,
-212.941772621246));
#196621=CARTESIAN_POINT('Ctrl Pts',(-61.6901615834725,-37.590390336358,
-215.587521646834));
#196622=CARTESIAN_POINT('Ctrl Pts',(-62.6142130892345,-37.4422426685059,
-214.325282532427));
#196623=CARTESIAN_POINT('Ctrl Pts',(-62.6460655421939,-37.2394079985843,
-212.767180740501));
#196624=CARTESIAN_POINT('Ctrl Pts',(-61.7046609397659,-38.2370900188355,
-215.471974562704));
#196625=CARTESIAN_POINT('Ctrl Pts',(-62.6001319557833,-38.1277065556804,
-214.21795893023));
#196626=CARTESIAN_POINT('Ctrl Pts',(-62.6306238454685,-37.9731020338337,
-212.681065126222));
#196627=CARTESIAN_POINT('Ctrl Pts',(-61.7302717981392,-39.5279866016878,
-215.301479571241));
#196628=CARTESIAN_POINT('Ctrl Pts',(-62.5694775958684,-39.4998723159367,
-214.068577411316));
#196629=CARTESIAN_POINT('Ctrl Pts',(-62.5969132094274,-39.4445711917008,
-212.57789537765));
#196630=CARTESIAN_POINT('Ctrl Pts',(-61.7413754773038,-40.1722445347539,
-215.246464457873));
#196631=CARTESIAN_POINT('Ctrl Pts',(-62.5529100079014,-40.1867078641608,
-214.026226040623));
#196632=CARTESIAN_POINT('Ctrl Pts',(-62.5786465561158,-40.1823394734508,
-212.560726431139));
#196633=CARTESIAN_POINT('Ctrl Pts',(-61.7551693704691,-41.1348830401125,
-215.217380280251));
#196634=CARTESIAN_POINT('Ctrl Pts',(-62.5260264335553,-41.2178782666483,
-214.020805002663));
#196635=CARTESIAN_POINT('Ctrl Pts',(-62.5489095967685,-41.2926666211446,
-212.597076537354));
#196636=CARTESIAN_POINT('Ctrl Pts',(-61.7592997587092,-41.4560741015586,
-215.216683316051));
#196637=CARTESIAN_POINT('Ctrl Pts',(-62.5167061217927,-41.5624453099376,
-214.028776153341));
#196638=CARTESIAN_POINT('Ctrl Pts',(-62.538573302366,-41.664507942645,-212.619734584269));
#196639=CARTESIAN_POINT('Ctrl Pts',(-61.7663955397543,-42.090104539572,
-215.23491686589));
#196640=CARTESIAN_POINT('Ctrl Pts',(-62.4975638186773,-42.2442869424654,
-214.06597330712));
#196641=CARTESIAN_POINT('Ctrl Pts',(-62.5172963966413,-42.4017436060914,
-212.687617475151));
#196642=CARTESIAN_POINT('Ctrl Pts',(-61.7693696651392,-42.4032937510997,
-215.253774289279));
#196643=CARTESIAN_POINT('Ctrl Pts',(-62.4877344671727,-42.5819624883669,
-214.095102448274));
#196644=CARTESIAN_POINT('Ctrl Pts',(-62.5063477838443,-42.7675314704734,
-212.732780967688));
#196645=CARTESIAN_POINT('Ctrl Pts',(-61.776403466414,-43.3300284309475,
-215.341514528131));
#196646=CARTESIAN_POINT('Ctrl Pts',(-62.4575092043709,-43.5834625000428,
-214.216422194191));
#196647=CARTESIAN_POINT('Ctrl Pts',(-62.4725701813145,-43.8557232524164,
-212.904651540624));
#196648=CARTESIAN_POINT('Ctrl Pts',(-61.7786393212107,-43.9308451169452,
-215.441224005761));
#196649=CARTESIAN_POINT('Ctrl Pts',(-62.4363373124719,-44.2373732157453,
-214.342183062308));
#196650=CARTESIAN_POINT('Ctrl Pts',(-62.4488123543693,-44.5690597591983,
-213.067323574879));
#196651=CARTESIAN_POINT('Ctrl Pts',(-61.7768758323447,-44.799108393107,
-215.66489855191));
#196652=CARTESIAN_POINT('Ctrl Pts',(-62.4031169014029,-45.1908126884628,
-214.61302309293));
#196653=CARTESIAN_POINT('Ctrl Pts',(-62.4112691380312,-45.6166733720198,
-213.400195879714));
#196654=CARTESIAN_POINT('Ctrl Pts',(-61.7754229930674,-45.0830122299898,
-215.75187598791));
#196655=CARTESIAN_POINT('Ctrl Pts',(-62.391806053278,-45.5038767861212,
-214.716988414011));
#196656=CARTESIAN_POINT('Ctrl Pts',(-62.3984364151395,-45.9621252239228,
-213.526046844411));
#196657=CARTESIAN_POINT('Ctrl Pts',(-61.7703563686195,-45.6378757088274,
-215.953838120193));
#196658=CARTESIAN_POINT('Ctrl Pts',(-62.368710967822,-46.1191184830862,
-214.956162974242));
#196659=CARTESIAN_POINT('Ctrl Pts',(-62.3721154800584,-46.6444314431026,
-213.811880088338));
#196660=CARTESIAN_POINT('Ctrl Pts',(-61.766714425071,-45.9100219139299,
-216.069514739708));
#196661=CARTESIAN_POINT('Ctrl Pts',(-62.3568675933792,-46.4227073678569,
-215.092174735303));
#196662=CARTESIAN_POINT('Ctrl Pts',(-62.3585615338666,-46.9827912699289,
-213.972791370408));
#196663=CARTESIAN_POINT('Ctrl Pts',(-61.7617700838064,-46.1695632659449,
-216.198756570055));
#196664=CARTESIAN_POINT('Ctrl Pts',(-62.3450157861073,-46.7143916405499,
-215.243383403778));
#196665=CARTESIAN_POINT('Ctrl Pts',(-62.3449264240553,-47.3099624311764,
-214.150201433913));
#196666=CARTESIAN_POINT('',(-61.7131389055822,20.0389433648605,-216.160156268336));
#196667=CARTESIAN_POINT('',(-62.3650443003751,20.9007294710183,-213.866597158632));
#196668=CARTESIAN_POINT('Ctrl Pts',(-61.7131389055822,20.0389433648605,
-216.160156268336));
#196669=CARTESIAN_POINT('Ctrl Pts',(-61.7678693862137,20.0751773182081,
-216.070351472292));
#196670=CARTESIAN_POINT('Ctrl Pts',(-61.8190760855121,20.1115905721978,
-215.979264091882));
#196671=CARTESIAN_POINT('Ctrl Pts',(-61.8668444683366,20.1481502791898,
-215.886955305269));
#196672=CARTESIAN_POINT('Ctrl Pts',(-61.9150658374495,20.1850566808991,
-215.793771156917));
#196673=CARTESIAN_POINT('Ctrl Pts',(-61.9597841805652,20.2221126942381,
-215.699341685683));
#196674=CARTESIAN_POINT('Ctrl Pts',(-62.0010568508086,20.2593031022775,
-215.603689573791));
#196675=CARTESIAN_POINT('Ctrl Pts',(-62.0425779998727,20.2967174122036,
-215.507461595986));
#196676=CARTESIAN_POINT('Ctrl Pts',(-62.0806125017358,20.3342681742483,
-215.409995389685));
#196677=CARTESIAN_POINT('Ctrl Pts',(-62.1151769896773,20.3719525091287,
-215.311284621693));
#196678=CARTESIAN_POINT('Ctrl Pts',(-62.1441447947059,20.4035349953873,
-215.228557104182));
#196679=CARTESIAN_POINT('Ctrl Pts',(-62.1706747072058,20.4352116636552,
-215.144954624778));
#196680=CARTESIAN_POINT('Ctrl Pts',(-62.1947499260075,20.4669841010193,
-215.060464474434));
#196681=CARTESIAN_POINT('Ctrl Pts',(-62.222160692488,20.5031585120715,-214.964268473059));
#196682=CARTESIAN_POINT('Ctrl Pts',(-62.2464217468638,20.5395075487633,
-214.866780056301));
#196683=CARTESIAN_POINT('Ctrl Pts',(-62.2673852527365,20.5758942372261,
-214.768340219344));
#196684=CARTESIAN_POINT('Ctrl Pts',(-62.2876551758303,20.611077063098,-214.673157288751));
#196685=CARTESIAN_POINT('Ctrl Pts',(-62.3048421853943,20.646294816521,-214.57708549284));
#196686=CARTESIAN_POINT('Ctrl Pts',(-62.3188618795333,20.6814237204261,
-214.480452073967));
#196687=CARTESIAN_POINT('Ctrl Pts',(-62.3336011485597,20.7183556506185,
-214.378858847781));
#196688=CARTESIAN_POINT('Ctrl Pts',(-62.3448390172506,20.7551890290087,
-214.276645420069));
#196689=CARTESIAN_POINT('Ctrl Pts',(-62.3525380749027,20.7917848562111,
-214.174204593435));
#196690=CARTESIAN_POINT('Ctrl Pts',(-62.3602371325547,20.8283806834136,
-214.071763766801));
#196691=CARTESIAN_POINT('Ctrl Pts',(-62.3643974261569,20.8647386489197,
-213.969096262343));
#196692=CARTESIAN_POINT('Ctrl Pts',(-62.3650443003751,20.9007294710183,
-213.866597158632));
#196693=CARTESIAN_POINT('',(-61.6795259610279,9.54487883260503,-216.064115826141));
#196694=CARTESIAN_POINT('Ctrl Pts',(-61.7131389055531,20.0389433648412,
-216.160156268384));
#196695=CARTESIAN_POINT('Ctrl Pts',(-61.7230421999514,19.657421912819,-215.99031134923));
#196696=CARTESIAN_POINT('Ctrl Pts',(-61.7309654538443,19.2561357591709,
-215.843887564221));
#196697=CARTESIAN_POINT('Ctrl Pts',(-61.7371187378078,18.8464365470887,
-215.722479103759));
#196698=CARTESIAN_POINT('Ctrl Pts',(-61.7377497043543,18.8044254033654,
-215.710029706418));
#196699=CARTESIAN_POINT('Ctrl Pts',(-61.7383620608911,18.7623257911141,
-215.697843334498));
#196700=CARTESIAN_POINT('Ctrl Pts',(-61.7389560341596,18.7201499473734,
-215.685921705516));
#196701=CARTESIAN_POINT('Ctrl Pts',(-61.7468389712057,18.1604117593227,
-215.527703388753));
#196702=CARTESIAN_POINT('Ctrl Pts',(-61.7516168666685,17.5843608729145,
-215.413777537614));
#196703=CARTESIAN_POINT('Ctrl Pts',(-61.7539978140095,16.9953644593714,
-215.337979225164));
#196704=CARTESIAN_POINT('Ctrl Pts',(-61.7563787613503,16.4063680458282,
-215.262180912713));
#196705=CARTESIAN_POINT('Ctrl Pts',(-61.7563293945832,15.8044782872716,
-215.224636336423));
#196706=CARTESIAN_POINT('Ctrl Pts',(-61.7541448402693,15.1919610915637,
-215.221849976965));
#196707=CARTESIAN_POINT('Ctrl Pts',(-61.7519602859553,14.5794438958557,
-215.219063617507));
#196708=CARTESIAN_POINT('Ctrl Pts',(-61.7476795068394,13.965046025957,-215.251046967269));
#196709=CARTESIAN_POINT('Ctrl Pts',(-61.741516620175,13.350930867722,-215.313231000222));
#196710=CARTESIAN_POINT('Ctrl Pts',(-61.7332980686954,12.5319742135963,
-215.396156860111));
#196711=CARTESIAN_POINT('Ctrl Pts',(-61.7217826330292,11.7125302862904,
-215.532443369588));
#196712=CARTESIAN_POINT('Ctrl Pts',(-61.7069868899011,10.8949681526562,
-215.716652557842));
#196713=CARTESIAN_POINT('Ctrl Pts',(-61.700872312975,10.557097556047,-215.792779944099));
#196714=CARTESIAN_POINT('Ctrl Pts',(-61.6941974964507,10.2195483491066,
-215.877091985145));
#196715=CARTESIAN_POINT('Ctrl Pts',(-61.6869636101976,9.88248774578141,
-215.969204864317));
#196716=CARTESIAN_POINT('Ctrl Pts',(-61.6857579624888,9.82631097856056,
-215.984557010846));
#196717=CARTESIAN_POINT('Ctrl Pts',(-61.6845367850159,9.77014778356728,
-216.000125847253));
#196718=CARTESIAN_POINT('Ctrl Pts',(-61.6833001414503,9.71399890071897,
-216.015909525897));
#196719=CARTESIAN_POINT('Ctrl Pts',(-61.6829840313086,9.69964615445876,
-216.019944141069));
#196720=CARTESIAN_POINT('Ctrl Pts',(-61.6826668840306,9.68529435909321,
-216.023992826748));
#196721=CARTESIAN_POINT('Ctrl Pts',(-61.6823487176854,9.67094351669723,
-216.028055531282));
#196722=CARTESIAN_POINT('Ctrl Pts',(-61.6820445402464,9.65722364168979,
-216.031939609782));
#196723=CARTESIAN_POINT('Ctrl Pts',(-61.6817394113119,9.64350470966858,
-216.035836656236));
#196724=CARTESIAN_POINT('Ctrl Pts',(-61.6814333454261,9.62978671861984,
-216.039746637367));
#196725=CARTESIAN_POINT('Ctrl Pts',(-61.6811202416631,9.61575328719779,
-216.043746527138));
#196726=CARTESIAN_POINT('Ctrl Pts',(-61.6808061369332,9.60172085660555,
-216.047759977122));
#196727=CARTESIAN_POINT('Ctrl Pts',(-61.6804910519492,9.58768941584011,
-216.05178694695));
#196728=CARTESIAN_POINT('Ctrl Pts',(-61.6804122807032,9.58418155564876,
-216.052793689406));
#196729=CARTESIAN_POINT('Ctrl Pts',(-61.6803089880787,9.58074834654284,
-216.053815574226));
#196730=CARTESIAN_POINT('Ctrl Pts',(-61.6801992274307,9.57732260329995,
-216.054845098855));
#196731=CARTESIAN_POINT('Ctrl Pts',(-61.6800345864587,9.57218398843562,
-216.056389385797));
#196732=CARTESIAN_POINT('Ctrl Pts',(-61.6798553763802,9.56706216868915,
-216.057950850523));
#196733=CARTESIAN_POINT('Ctrl Pts',(-61.6797228065068,9.56173044678179,
-216.059504376507));
#196734=CARTESIAN_POINT('Ctrl Pts',(-61.6795902366675,9.55639872624344,
-216.061057902091));
#196735=CARTESIAN_POINT('Ctrl Pts',(-61.6795044690351,9.55085713443771,
-216.062603607648));
#196736=CARTESIAN_POINT('Ctrl Pts',(-61.6795253586028,9.54487871892934,
-216.064115384928));
#196737=CARTESIAN_POINT('',(-62.0174913981677,0.438806380665441,-215.788052143479));
#196738=CARTESIAN_POINT('Ctrl Pts',(-61.6795265634691,9.54487894167559,
-216.064116268519));
#196739=CARTESIAN_POINT('Ctrl Pts',(-61.6801741939043,9.52709136950118,
-216.067812212364));
#196740=CARTESIAN_POINT('Ctrl Pts',(-61.6818851148242,9.50527890530528,
-216.07109134272));
#196741=CARTESIAN_POINT('Ctrl Pts',(-61.684571979164,9.46002870807816,-216.078979205164));
#196742=CARTESIAN_POINT('Ctrl Pts',(-61.6860515048732,9.43504846440253,
-216.083296010875));
#196743=CARTESIAN_POINT('Ctrl Pts',(-61.6934328695196,9.31010377869919,
-216.104698272446));
#196744=CARTESIAN_POINT('Ctrl Pts',(-61.6992859244921,9.21000894480459,
-216.121238473637));
#196745=CARTESIAN_POINT('Ctrl Pts',(-61.7166859533339,8.90929364047332,
-216.169076652063));
#196746=CARTESIAN_POINT('Ctrl Pts',(-61.7280739009634,8.7082425179926,-216.198592840276));
#196747=CARTESIAN_POINT('Ctrl Pts',(-61.7615734406237,8.10325300133128,
-216.279690889332));
#196748=CARTESIAN_POINT('Ctrl Pts',(-61.7830227272411,7.69748162474272,
-216.32383427267));
#196749=CARTESIAN_POINT('Ctrl Pts',(-61.8444274680599,6.47182680783556,
-216.423521585247));
#196750=CARTESIAN_POINT('Ctrl Pts',(-61.8810347009149,5.64536351003889,
-216.446767106403));
#196751=CARTESIAN_POINT('Ctrl Pts',(-61.9278975062939,4.38902081980034,
-216.404691459093));
#196752=CARTESIAN_POINT('Ctrl Pts',(-61.9420930876676,3.96799579818035,
-216.377909012764));
#196753=CARTESIAN_POINT('Ctrl Pts',(-61.9674232473587,3.12084236030756,
-216.296743366476));
#196754=CARTESIAN_POINT('Ctrl Pts',(-61.9785671023287,2.6942652956053,-216.242198159345));
#196755=CARTESIAN_POINT('Ctrl Pts',(-61.9973329077485,1.84297899797596,
-216.104606636849));
#196756=CARTESIAN_POINT('Ctrl Pts',(-62.0049832725563,1.41762802329507,
-216.02157900986));
#196757=CARTESIAN_POINT('Ctrl Pts',(-62.0123231790164,0.88617919753532,
-215.899355967453));
#196758=CARTESIAN_POINT('Ctrl Pts',(-62.0136798966164,0.779901155695931,
-215.873988897971));
#196759=CARTESIAN_POINT('Ctrl Pts',(-62.0155466212184,0.620498434716868,
-215.834540688288));
#196760=CARTESIAN_POINT('Ctrl Pts',(-62.0161408021641,0.567366580471024,
-215.821158342626));
#196761=CARTESIAN_POINT('Ctrl Pts',(-62.0168482856434,0.500954373935468,
-215.804137717908));
#196762=CARTESIAN_POINT('Ctrl Pts',(-62.01698802015,0.48767206310896,-215.800718958175));
#196763=CARTESIAN_POINT('Ctrl Pts',(-62.017250081267,0.462443823410336,
-215.794197517145));
#196764=CARTESIAN_POINT('Ctrl Pts',(-62.0173286470213,0.448406688707245,
-215.790652827454));
#196765=CARTESIAN_POINT('Ctrl Pts',(-62.0174913981677,0.438806380665441,
-215.788052143479));
#196766=CARTESIAN_POINT('',(-62.030115892062,-8.32556237289759,-215.882468962491));
#196767=CARTESIAN_POINT('Ctrl Pts',(-62.0174913981677,0.438806380665441,
-215.788052143479));
#196768=CARTESIAN_POINT('Ctrl Pts',(-62.0175184759225,0.437736514029309,
-215.787747559075));
#196769=CARTESIAN_POINT('Ctrl Pts',(-62.0175387248819,0.436718687877101,
-215.787466956657));
#196770=CARTESIAN_POINT('Ctrl Pts',(-62.017989654052,0.416815630977219,
-215.781891478117));
#196771=CARTESIAN_POINT('Ctrl Pts',(-62.0184159156524,0.397860626607022,
-215.776623255365));
#196772=CARTESIAN_POINT('Ctrl Pts',(-62.0222247646125,0.227220244864405,
-215.72957027851));
#196773=CARTESIAN_POINT('Ctrl Pts',(-62.0254149107006,0.075217642154615,
-215.69031199341));
#196774=CARTESIAN_POINT('Ctrl Pts',(-62.052437955369,-1.2954892060821,-215.359502197812));
#196775=CARTESIAN_POINT('Ctrl Pts',(-62.0647635114806,-2.53272084807531,
-215.223247240007));
#196776=CARTESIAN_POINT('Ctrl Pts',(-62.0696277257875,-5.02448450998964,
-215.233701926329));
#196777=CARTESIAN_POINT('Ctrl Pts',(-62.0621262930632,-6.27916951367206,
-215.380652672016));
#196778=CARTESIAN_POINT('Ctrl Pts',(-62.041100054462,-7.69137245107917,
-215.713077377955));
#196779=CARTESIAN_POINT('Ctrl Pts',(-62.0385848503381,-7.84830756476466,
-215.752367984344));
#196780=CARTESIAN_POINT('Ctrl Pts',(-62.0345359973834,-8.08366223386927,
-215.814879358009));
#196781=CARTESIAN_POINT('Ctrl Pts',(-62.0331425236356,-8.16198032978614,
-215.83627908007));
#196782=CARTESIAN_POINT('Ctrl Pts',(-62.031345448701,-8.25970867107241,
-215.863731373079));
#196783=CARTESIAN_POINT('Ctrl Pts',(-62.0309832718629,-8.27924587491217,
-215.869256965251));
#196784=CARTESIAN_POINT('Ctrl Pts',(-62.0304520415348,-8.30767279756168,
-215.87735141746));
#196785=CARTESIAN_POINT('Ctrl Pts',(-62.0299989262911,-8.31437654383897,
-215.879760093338));
#196786=CARTESIAN_POINT('Ctrl Pts',(-62.030115892062,-8.32556237289759,
-215.882468962491));
#196787=CARTESIAN_POINT('',(-61.9835319875972,-17.519732572983,-215.952954107728));
#196788=CARTESIAN_POINT('Ctrl Pts',(-62.030115892062,-8.32556237289759,
-215.882468962491));
#196789=CARTESIAN_POINT('Ctrl Pts',(-62.0301442467716,-8.32665730522469,
-215.882709095953));
#196790=CARTESIAN_POINT('Ctrl Pts',(-62.0301626852208,-8.32778917970396,
-215.882973325792));
#196791=CARTESIAN_POINT('Ctrl Pts',(-62.0304669547665,-8.34227865585374,
-215.886253315709));
#196792=CARTESIAN_POINT('Ctrl Pts',(-62.0307450589222,-8.35559115122019,
-215.88925405955));
#196793=CARTESIAN_POINT('Ctrl Pts',(-62.0321286803914,-8.42217147455135,
-215.904197652088));
#196794=CARTESIAN_POINT('Ctrl Pts',(-62.0332134989248,-8.47549284357947,
-215.915960118575));
#196795=CARTESIAN_POINT('Ctrl Pts',(-62.042775097603,-8.95589521339918,
-216.020077885304));
#196796=CARTESIAN_POINT('Ctrl Pts',(-62.0498315656512,-9.38649607478912,
-216.100211872333));
#196797=CARTESIAN_POINT('Ctrl Pts',(-62.060790505385,-10.2547342820899,
-216.234345225865));
#196798=CARTESIAN_POINT('Ctrl Pts',(-62.0646942119403,-10.6939384019574,
-216.288439637279));
#196799=CARTESIAN_POINT('Ctrl Pts',(-62.0691028446192,-11.5687209395696,
-216.368504230108));
#196800=CARTESIAN_POINT('Ctrl Pts',(-62.0696253097439,-12.0045938332199,
-216.39464466293));
#196801=CARTESIAN_POINT('Ctrl Pts',(-62.0662777878625,-13.3071638786316,
-216.432598698728));
#196802=CARTESIAN_POINT('Ctrl Pts',(-62.0574654920844,-14.1686287502632,
-216.403872085794));
#196803=CARTESIAN_POINT('Ctrl Pts',(-62.0354821865879,-15.4483827335448,
-216.28607811805));
#196804=CARTESIAN_POINT('Ctrl Pts',(-62.0266969469883,-15.8729284420891,
-216.234384919981));
#196805=CARTESIAN_POINT('Ctrl Pts',(-62.0115431415321,-16.5064068392879,
-216.139118393046));
#196806=CARTESIAN_POINT('Ctrl Pts',(-62.0061597028118,-16.7170305638983,
-216.104411645275));
#196807=CARTESIAN_POINT('Ctrl Pts',(-61.9976134180043,-17.0321410420476,
-216.048041250619));
#196808=CARTESIAN_POINT('Ctrl Pts',(-61.994686375636,-17.1370390445088,
-216.028532778314));
#196809=CARTESIAN_POINT('Ctrl Pts',(-61.9901825112225,-17.2941724515911,
-215.998207893143));
#196810=CARTESIAN_POINT('Ctrl Pts',(-61.9886623411118,-17.3465146583208,
-215.987922574716));
#196811=CARTESIAN_POINT('Ctrl Pts',(-61.9863542907869,-17.4249739380202,
-215.972231032217));
#196812=CARTESIAN_POINT('Ctrl Pts',(-61.9851933169768,-17.4641900706523,
-215.964319370264));
#196813=CARTESIAN_POINT('Ctrl Pts',(-61.9840220202716,-17.5033858261321,
-215.956309246507));
#196814=CARTESIAN_POINT('Ctrl Pts',(-61.9835964522753,-17.5175828670638,
-215.953395539067));
#196815=CARTESIAN_POINT('Ctrl Pts',(-61.9835711461698,-17.518673228533,
-215.953161073408));
#196816=CARTESIAN_POINT('Ctrl Pts',(-61.9835319875972,-17.519732572983,
-215.952954107728));
#196817=CARTESIAN_POINT('',(-62.0596235416337,-26.3318125162586,-215.724256795808));
#196818=CARTESIAN_POINT('Ctrl Pts',(-61.9835319875972,-17.519732572983,
-215.952954107728));
#196819=CARTESIAN_POINT('Ctrl Pts',(-61.9833142085583,-17.5339497172701,
-215.949734813099));
#196820=CARTESIAN_POINT('Ctrl Pts',(-61.9841625478236,-17.5427031512807,
-215.946332937118));
#196821=CARTESIAN_POINT('Ctrl Pts',(-61.9866649807491,-17.6342468174392,
-215.92008209154));
#196822=CARTESIAN_POINT('Ctrl Pts',(-61.9912692518142,-17.8060184448602,
-215.872011733283));
#196823=CARTESIAN_POINT('Ctrl Pts',(-62.0003968515277,-18.1615280644974,
-215.777781255583));
#196824=CARTESIAN_POINT('Ctrl Pts',(-62.0157672317227,-18.8050666555655,
-215.622415496145));
#196825=CARTESIAN_POINT('Ctrl Pts',(-62.0270350697659,-19.3583964345396,
-215.514965174136));
#196826=CARTESIAN_POINT('Ctrl Pts',(-62.0470553637187,-20.4658877553282,
-215.335027953477));
#196827=CARTESIAN_POINT('Ctrl Pts',(-62.0570575007116,-21.2047372367089,
-215.261640165529));
#196828=CARTESIAN_POINT('Ctrl Pts',(-62.0704693967988,-22.6800067729646,
-215.21176681083));
#196829=CARTESIAN_POINT('Ctrl Pts',(-62.0738081330386,-23.4167268528398,
-215.235823868393));
#196830=CARTESIAN_POINT('Ctrl Pts',(-62.0730682231818,-24.5158481803566,
-215.354315196491));
#196831=CARTESIAN_POINT('Ctrl Pts',(-62.071872155047,-24.8812952930637,
-215.407491584122));
#196832=CARTESIAN_POINT('Ctrl Pts',(-62.0685244646623,-25.4271720126043,
-215.509160665575));
#196833=CARTESIAN_POINT('Ctrl Pts',(-62.0671442433642,-25.6087188491995,
-215.546736924888));
#196834=CARTESIAN_POINT('Ctrl Pts',(-62.0646509441297,-25.8803504572708,
-215.608882620349));
#196835=CARTESIAN_POINT('Ctrl Pts',(-62.0637494272904,-25.9707796803734,
-215.630560795157));
#196836=CARTESIAN_POINT('Ctrl Pts',(-62.0622878127024,-26.10624205979,-215.664557073559));
#196837=CARTESIAN_POINT('Ctrl Pts',(-62.0615296291845,-26.1739278170651,
-215.681925290365));
#196838=CARTESIAN_POINT('Ctrl Pts',(-62.0605962917712,-26.2528128366554,
-215.702843946589));
#196839=CARTESIAN_POINT('Ctrl Pts',(-62.0601857362366,-26.2866029536357,
-215.71195050125));
#196840=CARTESIAN_POINT('Ctrl Pts',(-62.0599096760567,-26.3091257269047,
-215.718053065345));
#196841=CARTESIAN_POINT('Ctrl Pts',(-62.059836967416,-26.3186805305512,
-215.720581183794));
#196842=CARTESIAN_POINT('Ctrl Pts',(-62.0596235416337,-26.3318125162586,
-215.724256795808));
#196843=CARTESIAN_POINT('',(-61.6307906481739,-35.3347454198004,-216.138336341698));
#196844=CARTESIAN_POINT('Ctrl Pts',(-62.0596235416337,-26.3318125162586,
-215.724256795808));
#196845=CARTESIAN_POINT('Ctrl Pts',(-62.0594646122662,-26.3415802983989,
-215.726990681004));
#196846=CARTESIAN_POINT('Ctrl Pts',(-62.0591414109411,-26.3555304260684,
-215.731043606804));
#196847=CARTESIAN_POINT('Ctrl Pts',(-62.0586451088583,-26.3794896926403,
-215.737866697814));
#196848=CARTESIAN_POINT('Ctrl Pts',(-62.0578959089358,-26.4154258672405,
-215.748060296758));
#196849=CARTESIAN_POINT('Ctrl Pts',(-62.0561146300557,-26.4992579889169,
-215.771558827276));
#196850=CARTESIAN_POINT('Ctrl Pts',(-62.0524202151427,-26.6668475808658,
-215.817416048729));
#196851=CARTESIAN_POINT('Ctrl Pts',(-62.0445088892061,-27.0017357453129,
-215.904616215262));
#196852=CARTESIAN_POINT('Ctrl Pts',(-62.0368501484612,-27.2883096841957,
-215.971779454331));
#196853=CARTESIAN_POINT('Ctrl Pts',(-62.0203905608737,-27.8609439770147,
-216.096385682438));
#196854=CARTESIAN_POINT('Ctrl Pts',(-62.007903346956,-28.2419562872458,
-216.166476359143));
#196855=CARTESIAN_POINT('Ctrl Pts',(-61.9663758722878,-29.3820316599105,
-216.340372092763));
#196856=CARTESIAN_POINT('Ctrl Pts',(-61.9332872087863,-30.1378403279775,
-216.40779180649));
#196857=CARTESIAN_POINT('Ctrl Pts',(-61.858695018778,-31.6397584228355,
-216.459727323568));
#196858=CARTESIAN_POINT('Ctrl Pts',(-61.7860430758083,-32.9456419949789,
-216.432292162243));
#196859=CARTESIAN_POINT('Ctrl Pts',(-61.7040063394451,-34.235878888517,
-216.295897196999));
#196860=CARTESIAN_POINT('Ctrl Pts',(-61.6615453643437,-34.8774627313319,
-216.20733693376));
#196861=CARTESIAN_POINT('Ctrl Pts',(-61.6554459518943,-34.9690313914074,
-216.194201358865));
#196862=CARTESIAN_POINT('Ctrl Pts',(-61.6462397539745,-35.1062806936728,
-216.173780952623));
#196863=CARTESIAN_POINT('Ctrl Pts',(-61.6416227919041,-35.1748782865785,
-216.163391786615));
#196864=CARTESIAN_POINT('Ctrl Pts',(-61.6369852304075,-35.2434360370502,
-216.152736975617));
#196865=CARTESIAN_POINT('Ctrl Pts',(-61.6338889661978,-35.289132405245,
-216.145575037068));
#196866=CARTESIAN_POINT('Ctrl Pts',(-61.6318678984275,-35.3131377401504,
-216.142292059632));
#196867=CARTESIAN_POINT('Ctrl Pts',(-61.6307906481739,-35.3347454198004,
-216.138336341698));
#196868=CARTESIAN_POINT('Ctrl Pts',(-61.630817075809,-35.334740583441,-216.138302962291));
#196869=CARTESIAN_POINT('Ctrl Pts',(-61.630258520597,-35.3462277829799,
-216.136181498867));
#196870=CARTESIAN_POINT('Ctrl Pts',(-61.6313429993451,-35.3536573552358,
-216.132909291467));
#196871=CARTESIAN_POINT('Ctrl Pts',(-61.6316177861922,-35.3630846532595,
-216.130212116335));
#196872=CARTESIAN_POINT('Ctrl Pts',(-61.6317600130997,-35.367964127875,
-216.128816085622));
#196873=CARTESIAN_POINT('Ctrl Pts',(-61.6319021390161,-35.3728435113644,
-216.127421530594));
#196874=CARTESIAN_POINT('Ctrl Pts',(-61.6320441647623,-35.3777228018413,
-216.126028451162));
#196875=CARTESIAN_POINT('Ctrl Pts',(-61.6324606058031,-35.3920296219691,
-216.121943730863));
#196876=CARTESIAN_POINT('Ctrl Pts',(-61.632876179423,-35.4063356552158,
-216.117871702025));
#196877=CARTESIAN_POINT('Ctrl Pts',(-61.6332908867424,-35.4206408919241,
-216.113812378814));
#196878=CARTESIAN_POINT('Ctrl Pts',(-61.6339117798235,-35.4420584606094,
-216.107734825855));
#196879=CARTESIAN_POINT('Ctrl Pts',(-61.6345307316567,-35.4634742441022,
-216.101685752426));
#196880=CARTESIAN_POINT('Ctrl Pts',(-61.6351477473426,-35.4848882106408,
-216.095665204135));
#196881=CARTESIAN_POINT('Ctrl Pts',(-61.6353549667106,-35.4920799056225,
-216.093643255196));
#196882=CARTESIAN_POINT('Ctrl Pts',(-61.6355619677589,-35.4992713957634,
-216.091624523017));
#196883=CARTESIAN_POINT('Ctrl Pts',(-61.6357687506611,-35.5064626798289,
-216.089609009526));
#196884=CARTESIAN_POINT('Ctrl Pts',(-61.6374137485988,-35.5636707339529,
-216.073575210303));
#196885=CARTESIAN_POINT('Ctrl Pts',(-61.6390449413356,-35.6208657466514,
-216.057745105776));
#196886=CARTESIAN_POINT('Ctrl Pts',(-61.6406624176502,-35.6780470970208,
-216.042119664109));
#196887=CARTESIAN_POINT('Ctrl Pts',(-61.6434323883464,-35.7759716622587,
-216.015360684616));
#196888=CARTESIAN_POINT('Ctrl Pts',(-61.6461621322568,-35.873856159352,
-215.98920192936));
#196889=CARTESIAN_POINT('Ctrl Pts',(-61.6488520954094,-35.9716974699246,
-215.963648260647));
#196890=CARTESIAN_POINT('Ctrl Pts',(-61.6577684374166,-36.2960091939178,
-215.878946264054));
#196891=CARTESIAN_POINT('Ctrl Pts',(-61.6662440943207,-36.6196815346019,
-215.800922589524));
#196892=CARTESIAN_POINT('Ctrl Pts',(-61.6743064449508,-36.9432367142385,
-215.729666205912));
#196893=CARTESIAN_POINT('Ctrl Pts',(-61.690431146211,-37.5903470735117,
-215.587153438688));
#196894=CARTESIAN_POINT('Ctrl Pts',(-61.7049238227888,-38.2370578570965,
-215.47160642675));
#196895=CARTESIAN_POINT('Ctrl Pts',(-61.717722543651,-38.8825180264413,
-215.386359753546));
#196896=CARTESIAN_POINT('Ctrl Pts',(-61.7305212645132,-39.5279781957861,
-215.301113080342));
#196897=CARTESIAN_POINT('Ctrl Pts',(-61.7416182124067,-40.1722488053015,
-215.24609947756));
#196898=CARTESIAN_POINT('Ctrl Pts',(-61.7508074253462,-40.8140216533927,
-215.226712561206));
#196899=CARTESIAN_POINT('Ctrl Pts',(-61.7554020318159,-41.1349080774383,
-215.217019103028));
#196900=CARTESIAN_POINT('Ctrl Pts',(-61.759529053594,-41.4561062910276,
-215.216323666665));
#196901=CARTESIAN_POINT('Ctrl Pts',(-61.7630736382772,-41.7731288880566,
-215.225442248004));
#196902=CARTESIAN_POINT('Ctrl Pts',(-61.7666182229604,-42.0901514850857,
-215.234560829344));
#196903=CARTESIAN_POINT('Ctrl Pts',(-61.7695890991181,-42.4033483152362,
-215.253420330887));
#196904=CARTESIAN_POINT('Ctrl Pts',(-61.7719305274043,-42.7122677019303,
-215.28266947677));
#196905=CARTESIAN_POINT('Ctrl Pts',(-61.7766133839768,-43.3301064753184,
-215.341167768535));
#196906=CARTESIAN_POINT('Ctrl Pts',(-61.7788431881158,-43.9309400562982,
-215.44088331143));
#196907=CARTESIAN_POINT('Ctrl Pts',(-61.777662100194,-44.509800555182,-215.590007618605));
#196908=CARTESIAN_POINT('Ctrl Pts',(-61.7775373295268,-44.570951642519,
-215.605761178487));
#196909=CARTESIAN_POINT('Ctrl Pts',(-61.7773739523109,-44.631856455737,
-215.62206914929));
#196910=CARTESIAN_POINT('Ctrl Pts',(-61.7771699370815,-44.6925059899769,
-215.638946475185));
#196911=CARTESIAN_POINT('Ctrl Pts',(-61.7764083411934,-44.9189127932377,
-215.701950114888));
#196912=CARTESIAN_POINT('Ctrl Pts',(-61.7750804204424,-45.141762233653,
-215.772888079167));
#196913=CARTESIAN_POINT('Ctrl Pts',(-61.7730805145089,-45.3605857093514,
-215.852537712049));
#196914=CARTESIAN_POINT('Ctrl Pts',(-61.7715068721449,-45.5327687534799,
-215.915210678053));
#196915=CARTESIAN_POINT('Ctrl Pts',(-61.7695063242332,-45.7029161773407,
-215.983543948429));
#196916=CARTESIAN_POINT('Ctrl Pts',(-61.7670326019116,-45.8692783289489,
-216.057267272104));
#196917=CARTESIAN_POINT('Ctrl Pts',(-62.3685680449237,-46.7295402395799,
-213.857753233788));
#196918=CARTESIAN_POINT('Ctrl Pts',(-62.3741929604051,-46.5883034476749,
-213.791721439529));
#196919=CARTESIAN_POINT('Ctrl Pts',(-62.3797697215036,-46.4460138537357,
-213.72875854686));
#196920=CARTESIAN_POINT('Ctrl Pts',(-62.385275944621,-46.3032780419763,
-213.668964158759));
#196921=CARTESIAN_POINT('Ctrl Pts',(-62.3975426118317,-45.9852937059672,
-213.535755270514));
#196922=CARTESIAN_POINT('Ctrl Pts',(-62.409516407143,-45.6637866234507,
-213.417460800487));
#196923=CARTESIAN_POINT('Ctrl Pts',(-62.4212099404421,-45.3390922912232,
-213.312250045486));
#196924=CARTESIAN_POINT('Ctrl Pts',(-62.4220692464071,-45.3152319430017,
-213.304518573138));
#196925=CARTESIAN_POINT('Ctrl Pts',(-62.4229270385012,-45.2913543786762,
-213.296857777048));
#196926=CARTESIAN_POINT('Ctrl Pts',(-62.423783321531,-45.2674597292978,
-213.289266941101));
#196927=CARTESIAN_POINT('Ctrl Pts',(-62.4306555056665,-45.0756908577149,
-213.228345936535));
#196928=CARTESIAN_POINT('Ctrl Pts',(-62.4374306715991,-44.8828278915337,
-213.171905711604));
#196929=CARTESIAN_POINT('Ctrl Pts',(-62.4441103360269,-44.6889056159381,
-213.119707758193));
#196930=CARTESIAN_POINT('Ctrl Pts',(-62.4591991205405,-44.2508519591279,
-213.001797093728));
#196931=CARTESIAN_POINT('Ctrl Pts',(-62.4737962281636,-43.8075866319174,
-212.905453163029));
#196932=CARTESIAN_POINT('Ctrl Pts',(-62.4879106189022,-43.359734523307,
-212.828052803901));
#196933=CARTESIAN_POINT('Ctrl Pts',(-62.4903171672674,-43.2833743190478,
-212.814855797302));
#196934=CARTESIAN_POINT('Ctrl Pts',(-62.4927096782803,-43.2068808386599,
-212.802209607456));
#196935=CARTESIAN_POINT('Ctrl Pts',(-62.4950881915082,-43.13025726092,-212.790101352928));
#196936=CARTESIAN_POINT('Ctrl Pts',(-62.5008761037457,-42.9438002178896,
-212.760636932155));
#196937=CARTESIAN_POINT('Ctrl Pts',(-62.5065809373471,-42.7565658493217,
-212.734385263862));
#196938=CARTESIAN_POINT('Ctrl Pts',(-62.5122027551557,-42.5685838171507,
-212.711227872825));
#196939=CARTESIAN_POINT('Ctrl Pts',(-62.5175209296255,-42.390754994103,
-212.689321249381));
#196940=CARTESIAN_POINT('Ctrl Pts',(-62.5227648065832,-42.2122634170404,
-212.67017411522));
#196941=CARTESIAN_POINT('Ctrl Pts',(-62.527934793664,-42.0331254267329,
-212.653679770053));
#196942=CARTESIAN_POINT('Ctrl Pts',(-62.5385750526628,-41.6644446962783,
-212.619733049907));
#196943=CARTESIAN_POINT('Ctrl Pts',(-62.5489103696866,-41.2926330468704,
-212.597082683307));
#196944=CARTESIAN_POINT('Ctrl Pts',(-62.5588215912841,-40.9225569182789,
-212.584979442362));
#196945=CARTESIAN_POINT('Ctrl Pts',(-62.5635469131376,-40.7461176367338,
-212.579209042782));
#196946=CARTESIAN_POINT('Ctrl Pts',(-62.5681836632462,-40.5698182404518,
-212.575793047696));
#196947=CARTESIAN_POINT('Ctrl Pts',(-62.572734055004,-40.3936434675017,
-212.574637782408));
#196948=CARTESIAN_POINT('Ctrl Pts',(-62.5872728250111,-39.8307546787403,
-212.570946641685));
#196949=CARTESIAN_POINT('Ctrl Pts',(-62.6009299850174,-39.2692127837142,
-212.590224636131));
#196950=CARTESIAN_POINT('Ctrl Pts',(-62.6137680988131,-38.7088381795338,
-212.629502632766));
#196951=CARTESIAN_POINT('Ctrl Pts',(-62.6174709897936,-38.5472096022708,
-212.640831566424));
#196952=CARTESIAN_POINT('Ctrl Pts',(-62.6211056256317,-38.3856786969395,
-212.653829961882));
#196953=CARTESIAN_POINT('Ctrl Pts',(-62.6246729139128,-38.2242434316533,
-212.668455765861));
#196954=CARTESIAN_POINT('Ctrl Pts',(-62.6373436782579,-37.6508363946416,
-212.720405622718));
#196955=CARTESIAN_POINT('Ctrl Pts',(-62.64916746512,-37.0786070163147,-212.792770228131));
#196956=CARTESIAN_POINT('Ctrl Pts',(-62.6601855978901,-36.5075023878094,
-212.883581944343));
#196957=CARTESIAN_POINT('Ctrl Pts',(-62.6630243100177,-36.3603629705484,
-212.906978678211));
#196958=CARTESIAN_POINT('Ctrl Pts',(-62.6658095819956,-36.2132944881781,
-212.931604448248));
#196959=CARTESIAN_POINT('Ctrl Pts',(-62.6685426178708,-36.0662511671651,
-212.957447775203));
#196960=CARTESIAN_POINT('Ctrl Pts',(-62.6726066835548,-35.847595524766,
-212.99587719327));
#196961=CARTESIAN_POINT('Ctrl Pts',(-62.6765563106204,-35.6289441132953,
-213.037001059769));
#196962=CARTESIAN_POINT('Ctrl Pts',(-62.6803946782106,-35.4101865945473,
-213.080774391967));
#196963=CARTESIAN_POINT('Ctrl Pts',(-62.6828563633539,-35.2698894184043,
-213.108847826575));
#196964=CARTESIAN_POINT('Ctrl Pts',(-62.6852717293956,-35.1295761809559,
-213.138007694814));
#196965=CARTESIAN_POINT('Ctrl Pts',(-62.6876407845122,-34.9892589138455,
-213.168238544914));
#196966=CARTESIAN_POINT('Ctrl Pts',(-62.6883605905981,-34.9466253667763,
-213.177423789163));
#196967=CARTESIAN_POINT('Ctrl Pts',(-62.6890761418333,-34.9039903123168,
-213.186708083958));
#196968=CARTESIAN_POINT('Ctrl Pts',(-62.6897874443054,-34.8613537452901,
-213.196091056989));
#196969=CARTESIAN_POINT('Ctrl Pts',(-62.6905505729894,-34.8156106352014,
-213.206157682852));
#196970=CARTESIAN_POINT('Ctrl Pts',(-62.6913088108163,-34.7698657837897,
-213.216337913902));
#196971=CARTESIAN_POINT('Ctrl Pts',(-62.6920621645107,-34.7241191838736,
-213.226631336799));
#196972=CARTESIAN_POINT('Ctrl Pts',(-62.6922505029487,-34.712682533017,
-213.22920469272));
#196973=CARTESIAN_POINT('Ctrl Pts',(-62.6924385015881,-34.7012457426654,
-213.231787136791));
#196974=CARTESIAN_POINT('Ctrl Pts',(-62.6926262681682,-34.6898089068761,
-213.234372387595));
#196975=CARTESIAN_POINT('Ctrl Pts',(-62.6928140347405,-34.6783720715574,
-213.236957638293));
#196976=CARTESIAN_POINT('Ctrl Pts',(-62.6930017734618,-34.666935369537,
-213.23953379065));
#196977=CARTESIAN_POINT('Ctrl Pts',(-62.6931894847934,-34.6554988009796,
-213.242100818803));
#196978=CARTESIAN_POINT('Ctrl Pts',(-62.6935649074066,-34.6326256669197,
-213.247234874422));
#196979=CARTESIAN_POINT('Ctrl Pts',(-62.693940220454,-34.6097530667601,
-213.252332433528));
